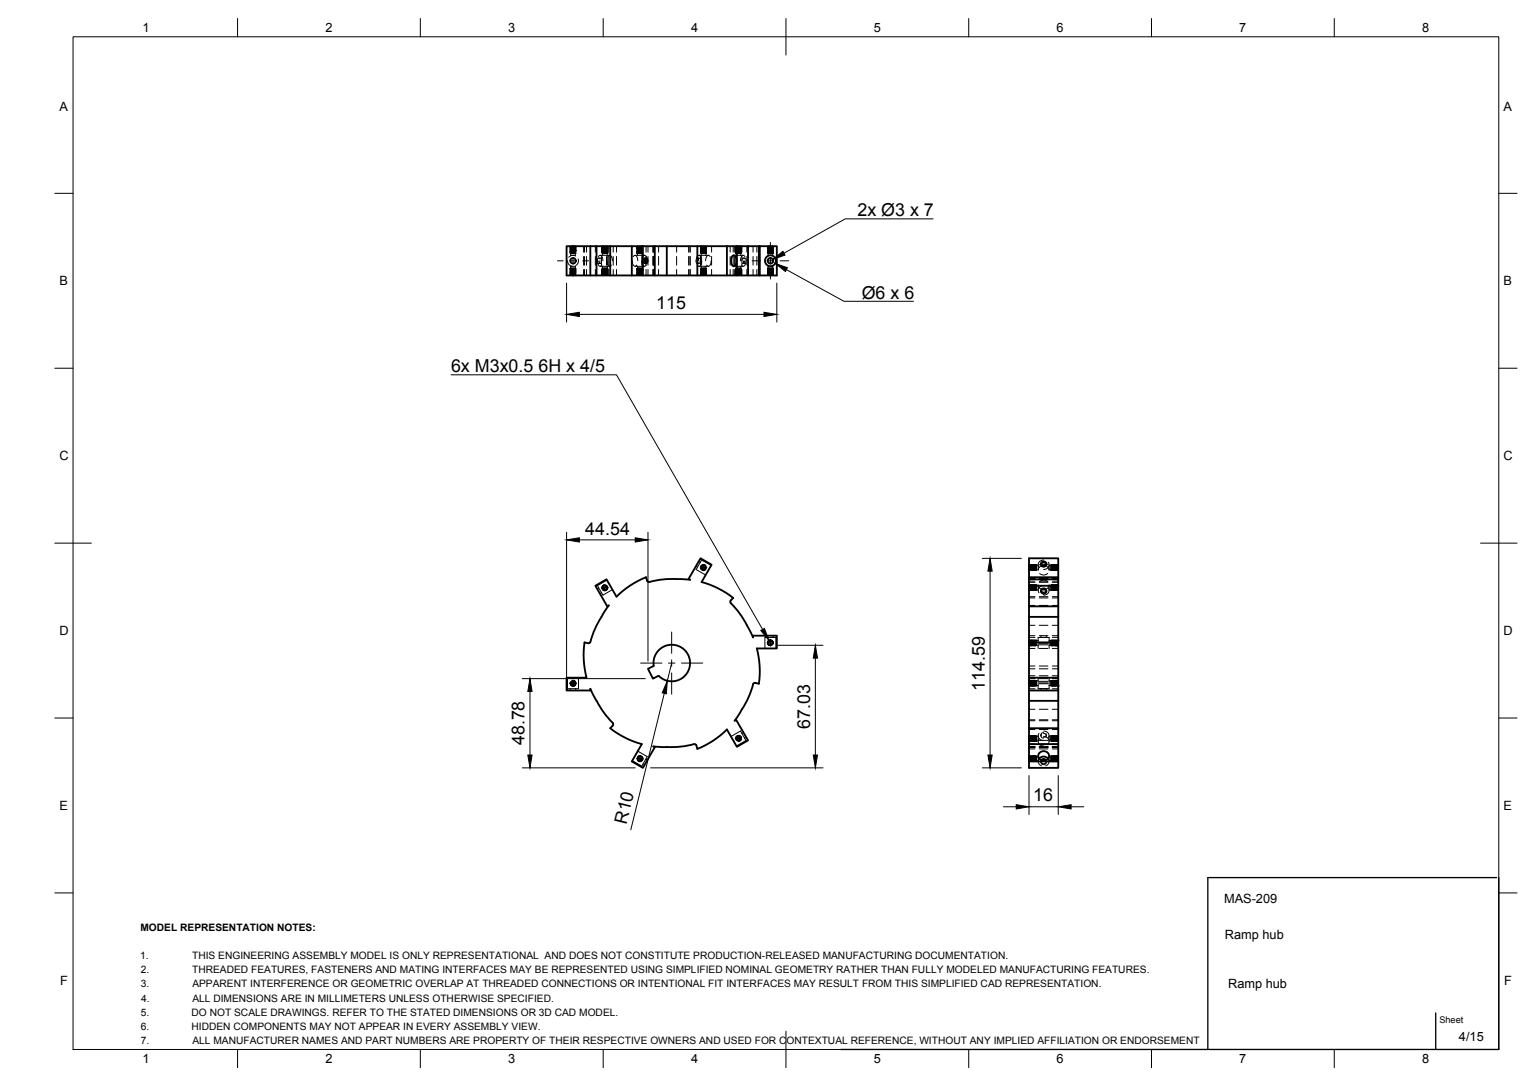
ISO-10303-21;
HEADER;
/* Generated by software containing ST-Developer
 * from STEP Tools, Inc. (www.steptools.com) 
 */

FILE_DESCRIPTION(
/* description */ ('Independent bearing-supported roller-ramp one-way clutch. Six logarit
hmic ramps with plain solid rollers, sprung guided plungers, native Co
il variants, removable shared keepers, rounded parallel key, shaft wit
h complete retaining lips, bronze journal/thrust support and bolted co
vers. Native rotor, roller planar/spin and plunger joints permit manua
l geometric engaged/released inspection. Automatic frictional torque s
witching/contact dynamics are not simulated; no capacity, hardness, fi
t, lubrication, speed, force or life rating. External input driver/cou
pling/anchors outside assembly.'),
/* implementation_level */ '2;1');

FILE_NAME(
/* name */ 'Ramp hub.step',
/* time_stamp */ '2026-11-08T07:04:38-08:00',
/* author */ (''),
/* organization */ (''),
/* preprocessor_version */ 'ST-DEVELOPER v20.2',
/* originating_system */ 'Autodesk Translation Framework v15.17.0.0',
/* authorisation */ '');

FILE_SCHEMA (('AUTOMOTIVE_DESIGN { 1 0 10303 214 3 1 1 }'));
ENDSEC;

DATA;
#10=MECHANICAL_DESIGN_GEOMETRIC_PRESENTATION_REPRESENTATION('',(#301),#99526);
#256=(
BOUNDED_SURFACE()
B_SPLINE_SURFACE(5,1,((#70021,#70022),(#70023,#70024),(#70025,#70026),(#70027,
#70028),(#70029,#70030),(#70031,#70032),(#70033,#70034),(#70035,#70036),
(#70037,#70038),(#70039,#70040),(#70041,#70042),(#70043,#70044),(#70045,
#70046),(#70047,#70048),(#70049,#70050),(#70051,#70052),(#70053,#70054),
(#70055,#70056),(#70057,#70058),(#70059,#70060),(#70061,#70062),(#70063,
#70064),(#70065,#70066),(#70067,#70068),(#70069,#70070),(#70071,#70072),
(#70073,#70074),(#70075,#70076),(#70077,#70078),(#70079,#70080),(#70081,
#70082),(#70083,#70084),(#70085,#70086),(#70087,#70088),(#70089,#70090),
(#70091,#70092),(#70093,#70094),(#70095,#70096),(#70097,#70098),(#70099,
#70100),(#70101,#70102),(#70103,#70104),(#70105,#70106),(#70107,#70108),
(#70109,#70110),(#70111,#70112),(#70113,#70114),(#70115,#70116),(#70117,
#70118),(#70119,#70120),(#70121,#70122),(#70123,#70124),(#70125,#70126),
(#70127,#70128),(#70129,#70130),(#70131,#70132),(#70133,#70134),(#70135,
#70136),(#70137,#70138),(#70139,#70140),(#70141,#70142),(#70143,#70144),
(#70145,#70146),(#70147,#70148),(#70149,#70150),(#70151,#70152),(#70153,
#70154),(#70155,#70156),(#70157,#70158),(#70159,#70160),(#70161,#70162),
(#70163,#70164),(#70165,#70166),(#70167,#70168),(#70169,#70170),(#70171,
#70172),(#70173,#70174),(#70175,#70176),(#70177,#70178),(#70179,#70180),
(#70181,#70182),(#70183,#70184),(#70185,#70186),(#70187,#70188),(#70189,
#70190),(#70191,#70192),(#70193,#70194),(#70195,#70196),(#70197,#70198),
(#70199,#70200),(#70201,#70202),(#70203,#70204),(#70205,#70206),(#70207,
#70208),(#70209,#70210),(#70211,#70212),(#70213,#70214),(#70215,#70216),
(#70217,#70218),(#70219,#70220),(#70221,#70222),(#70223,#70224),(#70225,
#70226),(#70227,#70228),(#70229,#70230),(#70231,#70232),(#70233,#70234),
(#70235,#70236),(#70237,#70238),(#70239,#70240),(#70241,#70242),(#70243,
#70244),(#70245,#70246),(#70247,#70248),(#70249,#70250),(#70251,#70252),
(#70253,#70254),(#70255,#70256),(#70257,#70258),(#70259,#70260),(#70261,
#70262),(#70263,#70264),(#70265,#70266),(#70267,#70268),(#70269,#70270),
(#70271,#70272),(#70273,#70274),(#70275,#70276),(#70277,#70278),(#70279,
#70280),(#70281,#70282),(#70283,#70284),(#70285,#70286),(#70287,#70288),
(#70289,#70290),(#70291,#70292),(#70293,#70294),(#70295,#70296),(#70297,
#70298),(#70299,#70300),(#70301,#70302),(#70303,#70304),(#70305,#70306),
(#70307,#70308),(#70309,#70310),(#70311,#70312),(#70313,#70314),(#70315,
#70316),(#70317,#70318),(#70319,#70320),(#70321,#70322),(#70323,#70324),
(#70325,#70326),(#70327,#70328),(#70329,#70330),(#70331,#70332),(#70333,
#70334),(#70335,#70336),(#70337,#70338),(#70339,#70340),(#70341,#70342),
(#70343,#70344),(#70345,#70346),(#70347,#70348),(#70349,#70350),(#70351,
#70352),(#70353,#70354),(#70355,#70356),(#70357,#70358),(#70359,#70360),
(#70361,#70362),(#70363,#70364),(#70365,#70366),(#70367,#70368),(#70369,
#70370),(#70371,#70372),(#70373,#70374),(#70375,#70376),(#70377,#70378),
(#70379,#70380),(#70381,#70382),(#70383,#70384),(#70385,#70386),(#70387,
#70388),(#70389,#70390),(#70391,#70392),(#70393,#70394),(#70395,#70396),
(#70397,#70398),(#70399,#70400),(#70401,#70402),(#70403,#70404),(#70405,
#70406),(#70407,#70408),(#70409,#70410),(#70411,#70412),(#70413,#70414),
(#70415,#70416),(#70417,#70418),(#70419,#70420),(#70421,#70422),(#70423,
#70424),(#70425,#70426),(#70427,#70428),(#70429,#70430),(#70431,#70432),
(#70433,#70434),(#70435,#70436),(#70437,#70438),(#70439,#70440),(#70441,
#70442),(#70443,#70444),(#70445,#70446),(#70447,#70448),(#70449,#70450),
(#70451,#70452),(#70453,#70454),(#70455,#70456),(#70457,#70458),(#70459,
#70460),(#70461,#70462),(#70463,#70464),(#70465,#70466),(#70467,#70468),
(#70469,#70470),(#70471,#70472),(#70473,#70474),(#70475,#70476),(#70477,
#70478),(#70479,#70480),(#70481,#70482),(#70483,#70484),(#70485,#70486),
(#70487,#70488),(#70489,#70490),(#70491,#70492),(#70493,#70494),(#70495,
#70496),(#70497,#70498),(#70499,#70500),(#70501,#70502),(#70503,#70504),
(#70505,#70506),(#70507,#70508),(#70509,#70510),(#70511,#70512),(#70513,
#70514),(#70515,#70516),(#70517,#70518),(#70519,#70520),(#70521,#70522),
(#70523,#70524),(#70525,#70526),(#70527,#70528),(#70529,#70530),(#70531,
#70532),(#70533,#70534),(#70535,#70536),(#70537,#70538),(#70539,#70540),
(#70541,#70542),(#70543,#70544),(#70545,#70546),(#70547,#70548),(#70549,
#70550),(#70551,#70552),(#70553,#70554),(#70555,#70556),(#70557,#70558),
(#70559,#70560),(#70561,#70562),(#70563,#70564),(#70565,#70566),(#70567,
#70568),(#70569,#70570),(#70571,#70572),(#70573,#70574),(#70575,#70576),
(#70577,#70578),(#70579,#70580),(#70581,#70582),(#70583,#70584),(#70585,
#70586),(#70587,#70588),(#70589,#70590),(#70591,#70592),(#70593,#70594),
(#70595,#70596),(#70597,#70598),(#70599,#70600),(#70601,#70602),(#70603,
#70604),(#70605,#70606),(#70607,#70608),(#70609,#70610),(#70611,#70612),
(#70613,#70614),(#70615,#70616),(#70617,#70618),(#70619,#70620),(#70621,
#70622),(#70623,#70624),(#70625,#70626),(#70627,#70628),(#70629,#70630),
(#70631,#70632),(#70633,#70634),(#70635,#70636),(#70637,#70638),(#70639,
#70640),(#70641,#70642),(#70643,#70644),(#70645,#70646),(#70647,#70648),
(#70649,#70650),(#70651,#70652),(#70653,#70654),(#70655,#70656),(#70657,
#70658),(#70659,#70660),(#70661,#70662),(#70663,#70664),(#70665,#70666),
(#70667,#70668),(#70669,#70670),(#70671,#70672),(#70673,#70674),(#70675,
#70676),(#70677,#70678),(#70679,#70680),(#70681,#70682),(#70683,#70684),
(#70685,#70686),(#70687,#70688),(#70689,#70690),(#70691,#70692),(#70693,
#70694),(#70695,#70696),(#70697,#70698),(#70699,#70700),(#70701,#70702),
(#70703,#70704),(#70705,#70706),(#70707,#70708),(#70709,#70710),(#70711,
#70712),(#70713,#70714),(#70715,#70716),(#70717,#70718),(#70719,#70720),
(#70721,#70722),(#70723,#70724),(#70725,#70726),(#70727,#70728),(#70729,
#70730),(#70731,#70732),(#70733,#70734),(#70735,#70736),(#70737,#70738),
(#70739,#70740),(#70741,#70742),(#70743,#70744),(#70745,#70746),(#70747,
#70748),(#70749,#70750),(#70751,#70752),(#70753,#70754),(#70755,#70756),
(#70757,#70758),(#70759,#70760),(#70761,#70762),(#70763,#70764),(#70765,
#70766),(#70767,#70768),(#70769,#70770),(#70771,#70772),(#70773,#70774),
(#70775,#70776),(#70777,#70778),(#70779,#70780),(#70781,#70782),(#70783,
#70784),(#70785,#70786),(#70787,#70788),(#70789,#70790),(#70791,#70792),
(#70793,#70794),(#70795,#70796),(#70797,#70798),(#70799,#70800),(#70801,
#70802),(#70803,#70804),(#70805,#70806),(#70807,#70808),(#70809,#70810),
(#70811,#70812),(#70813,#70814),(#70815,#70816),(#70817,#70818),(#70819,
#70820),(#70821,#70822),(#70823,#70824),(#70825,#70826),(#70827,#70828),
(#70829,#70830),(#70831,#70832),(#70833,#70834),(#70835,#70836),(#70837,
#70838),(#70839,#70840),(#70841,#70842),(#70843,#70844),(#70845,#70846),
(#70847,#70848),(#70849,#70850),(#70851,#70852),(#70853,#70854),(#70855,
#70856),(#70857,#70858),(#70859,#70860),(#70861,#70862),(#70863,#70864),
(#70865,#70866),(#70867,#70868),(#70869,#70870),(#70871,#70872),(#70873,
#70874),(#70875,#70876),(#70877,#70878),(#70879,#70880),(#70881,#70882),
(#70883,#70884),(#70885,#70886),(#70887,#70888),(#70889,#70890),(#70891,
#70892),(#70893,#70894),(#70895,#70896),(#70897,#70898),(#70899,#70900),
(#70901,#70902),(#70903,#70904),(#70905,#70906),(#70907,#70908),(#70909,
#70910),(#70911,#70912),(#70913,#70914),(#70915,#70916),(#70917,#70918),
(#70919,#70920),(#70921,#70922),(#70923,#70924),(#70925,#70926),(#70927,
#70928),(#70929,#70930),(#70931,#70932),(#70933,#70934),(#70935,#70936),
(#70937,#70938),(#70939,#70940),(#70941,#70942),(#70943,#70944),(#70945,
#70946),(#70947,#70948),(#70949,#70950),(#70951,#70952),(#70953,#70954),
(#70955,#70956),(#70957,#70958),(#70959,#70960),(#70961,#70962),(#70963,
#70964),(#70965,#70966),(#70967,#70968),(#70969,#70970),(#70971,#70972),
(#70973,#70974),(#70975,#70976),(#70977,#70978),(#70979,#70980),(#70981,
#70982),(#70983,#70984),(#70985,#70986),(#70987,#70988),(#70989,#70990),
(#70991,#70992),(#70993,#70994),(#70995,#70996),(#70997,#70998),(#70999,
#71000),(#71001,#71002),(#71003,#71004),(#71005,#71006),(#71007,#71008),
(#71009,#71010),(#71011,#71012),(#71013,#71014),(#71015,#71016),(#71017,
#71018),(#71019,#71020),(#71021,#71022),(#71023,#71024),(#71025,#71026),
(#71027,#71028),(#71029,#71030),(#71031,#71032),(#71033,#71034),(#71035,
#71036),(#71037,#71038),(#71039,#71040),(#71041,#71042),(#71043,#71044),
(#71045,#71046),(#71047,#71048),(#71049,#71050),(#71051,#71052),(#71053,
#71054),(#71055,#71056),(#71057,#71058),(#71059,#71060),(#71061,#71062),
(#71063,#71064),(#71065,#71066),(#71067,#71068),(#71069,#71070),(#71071,
#71072),(#71073,#71074),(#71075,#71076),(#71077,#71078),(#71079,#71080),
(#71081,#71082),(#71083,#71084),(#71085,#71086),(#71087,#71088),(#71089,
#71090),(#71091,#71092),(#71093,#71094),(#71095,#71096),(#71097,#71098),
(#71099,#71100),(#71101,#71102),(#71103,#71104),(#71105,#71106),(#71107,
#71108),(#71109,#71110),(#71111,#71112),(#71113,#71114),(#71115,#71116),
(#71117,#71118),(#71119,#71120),(#71121,#71122),(#71123,#71124),(#71125,
#71126),(#71127,#71128),(#71129,#71130),(#71131,#71132),(#71133,#71134),
(#71135,#71136),(#71137,#71138),(#71139,#71140),(#71141,#71142),(#71143,
#71144),(#71145,#71146),(#71147,#71148),(#71149,#71150),(#71151,#71152),
(#71153,#71154),(#71155,#71156),(#71157,#71158),(#71159,#71160),(#71161,
#71162),(#71163,#71164),(#71165,#71166),(#71167,#71168),(#71169,#71170),
(#71171,#71172),(#71173,#71174),(#71175,#71176),(#71177,#71178),(#71179,
#71180),(#71181,#71182),(#71183,#71184),(#71185,#71186),(#71187,#71188),
(#71189,#71190),(#71191,#71192),(#71193,#71194),(#71195,#71196),(#71197,
#71198),(#71199,#71200),(#71201,#71202),(#71203,#71204),(#71205,#71206),
(#71207,#71208),(#71209,#71210),(#71211,#71212),(#71213,#71214),(#71215,
#71216),(#71217,#71218),(#71219,#71220),(#71221,#71222),(#71223,#71224),
(#71225,#71226),(#71227,#71228),(#71229,#71230),(#71231,#71232),(#71233,
#71234),(#71235,#71236),(#71237,#71238),(#71239,#71240),(#71241,#71242),
(#71243,#71244),(#71245,#71246),(#71247,#71248),(#71249,#71250),(#71251,
#71252),(#71253,#71254),(#71255,#71256),(#71257,#71258),(#71259,#71260),
(#71261,#71262),(#71263,#71264),(#71265,#71266),(#71267,#71268),(#71269,
#71270),(#71271,#71272),(#71273,#71274),(#71275,#71276),(#71277,#71278),
(#71279,#71280),(#71281,#71282),(#71283,#71284),(#71285,#71286),(#71287,
#71288),(#71289,#71290),(#71291,#71292),(#71293,#71294),(#71295,#71296),
(#71297,#71298),(#71299,#71300),(#71301,#71302),(#71303,#71304),(#71305,
#71306),(#71307,#71308),(#71309,#71310),(#71311,#71312),(#71313,#71314),
(#71315,#71316),(#71317,#71318),(#71319,#71320),(#71321,#71322),(#71323,
#71324),(#71325,#71326),(#71327,#71328),(#71329,#71330),(#71331,#71332),
(#71333,#71334),(#71335,#71336),(#71337,#71338),(#71339,#71340),(#71341,
#71342),(#71343,#71344),(#71345,#71346),(#71347,#71348),(#71349,#71350),
(#71351,#71352),(#71353,#71354),(#71355,#71356),(#71357,#71358),(#71359,
#71360),(#71361,#71362),(#71363,#71364),(#71365,#71366),(#71367,#71368),
(#71369,#71370),(#71371,#71372),(#71373,#71374),(#71375,#71376),(#71377,
#71378),(#71379,#71380),(#71381,#71382),(#71383,#71384),(#71385,#71386),
(#71387,#71388),(#71389,#71390),(#71391,#71392),(#71393,#71394),(#71395,
#71396),(#71397,#71398),(#71399,#71400),(#71401,#71402),(#71403,#71404),
(#71405,#71406),(#71407,#71408),(#71409,#71410),(#71411,#71412),(#71413,
#71414),(#71415,#71416),(#71417,#71418),(#71419,#71420),(#71421,#71422),
(#71423,#71424),(#71425,#71426),(#71427,#71428),(#71429,#71430),(#71431,
#71432),(#71433,#71434),(#71435,#71436),(#71437,#71438),(#71439,#71440),
(#71441,#71442),(#71443,#71444),(#71445,#71446),(#71447,#71448),(#71449,
#71450),(#71451,#71452),(#71453,#71454),(#71455,#71456),(#71457,#71458),
(#71459,#71460),(#71461,#71462),(#71463,#71464),(#71465,#71466),(#71467,
#71468),(#71469,#71470),(#71471,#71472),(#71473,#71474),(#71475,#71476),
(#71477,#71478),(#71479,#71480),(#71481,#71482),(#71483,#71484),(#71485,
#71486),(#71487,#71488),(#71489,#71490),(#71491,#71492),(#71493,#71494),
(#71495,#71496),(#71497,#71498),(#71499,#71500),(#71501,#71502),(#71503,
#71504),(#71505,#71506),(#71507,#71508),(#71509,#71510),(#71511,#71512),
(#71513,#71514),(#71515,#71516),(#71517,#71518),(#71519,#71520),(#71521,
#71522),(#71523,#71524),(#71525,#71526),(#71527,#71528),(#71529,#71530),
(#71531,#71532),(#71533,#71534),(#71535,#71536),(#71537,#71538),(#71539,
#71540),(#71541,#71542),(#71543,#71544),(#71545,#71546),(#71547,#71548),
(#71549,#71550),(#71551,#71552),(#71553,#71554),(#71555,#71556),(#71557,
#71558),(#71559,#71560),(#71561,#71562),(#71563,#71564),(#71565,#71566),
(#71567,#71568),(#71569,#71570),(#71571,#71572),(#71573,#71574),(#71575,
#71576),(#71577,#71578),(#71579,#71580),(#71581,#71582),(#71583,#71584),
(#71585,#71586),(#71587,#71588),(#71589,#71590),(#71591,#71592),(#71593,
#71594),(#71595,#71596),(#71597,#71598),(#71599,#71600),(#71601,#71602),
(#71603,#71604),(#71605,#71606),(#71607,#71608),(#71609,#71610),(#71611,
#71612),(#71613,#71614),(#71615,#71616),(#71617,#71618),(#71619,#71620),
(#71621,#71622),(#71623,#71624),(#71625,#71626),(#71627,#71628),(#71629,
#71630),(#71631,#71632),(#71633,#71634),(#71635,#71636),(#71637,#71638),
(#71639,#71640),(#71641,#71642),(#71643,#71644),(#71645,#71646),(#71647,
#71648),(#71649,#71650),(#71651,#71652),(#71653,#71654),(#71655,#71656),
(#71657,#71658),(#71659,#71660),(#71661,#71662),(#71663,#71664),(#71665,
#71666),(#71667,#71668),(#71669,#71670),(#71671,#71672),(#71673,#71674),
(#71675,#71676),(#71677,#71678),(#71679,#71680),(#71681,#71682),(#71683,
#71684),(#71685,#71686),(#71687,#71688),(#71689,#71690),(#71691,#71692),
(#71693,#71694),(#71695,#71696),(#71697,#71698),(#71699,#71700),(#71701,
#71702),(#71703,#71704),(#71705,#71706),(#71707,#71708),(#71709,#71710),
(#71711,#71712),(#71713,#71714),(#71715,#71716),(#71717,#71718),(#71719,
#71720),(#71721,#71722),(#71723,#71724),(#71725,#71726),(#71727,#71728),
(#71729,#71730),(#71731,#71732),(#71733,#71734),(#71735,#71736),(#71737,
#71738),(#71739,#71740),(#71741,#71742),(#71743,#71744),(#71745,#71746),
(#71747,#71748),(#71749,#71750),(#71751,#71752),(#71753,#71754),(#71755,
#71756),(#71757,#71758),(#71759,#71760),(#71761,#71762),(#71763,#71764),
(#71765,#71766),(#71767,#71768),(#71769,#71770),(#71771,#71772),(#71773,
#71774),(#71775,#71776),(#71777,#71778),(#71779,#71780),(#71781,#71782),
(#71783,#71784),(#71785,#71786),(#71787,#71788),(#71789,#71790),(#71791,
#71792),(#71793,#71794),(#71795,#71796),(#71797,#71798),(#71799,#71800),
(#71801,#71802),(#71803,#71804),(#71805,#71806),(#71807,#71808),(#71809,
#71810),(#71811,#71812),(#71813,#71814),(#71815,#71816),(#71817,#71818),
(#71819,#71820),(#71821,#71822),(#71823,#71824),(#71825,#71826),(#71827,
#71828),(#71829,#71830),(#71831,#71832),(#71833,#71834),(#71835,#71836),
(#71837,#71838),(#71839,#71840),(#71841,#71842),(#71843,#71844),(#71845,
#71846),(#71847,#71848),(#71849,#71850),(#71851,#71852),(#71853,#71854),
(#71855,#71856),(#71857,#71858),(#71859,#71860),(#71861,#71862),(#71863,
#71864),(#71865,#71866),(#71867,#71868),(#71869,#71870),(#71871,#71872),
(#71873,#71874),(#71875,#71876),(#71877,#71878),(#71879,#71880),(#71881,
#71882),(#71883,#71884),(#71885,#71886),(#71887,#71888),(#71889,#71890),
(#71891,#71892),(#71893,#71894),(#71895,#71896),(#71897,#71898),(#71899,
#71900),(#71901,#71902),(#71903,#71904),(#71905,#71906),(#71907,#71908),
(#71909,#71910),(#71911,#71912),(#71913,#71914),(#71915,#71916),(#71917,
#71918),(#71919,#71920),(#71921,#71922),(#71923,#71924),(#71925,#71926),
(#71927,#71928),(#71929,#71930),(#71931,#71932),(#71933,#71934),(#71935,
#71936),(#71937,#71938),(#71939,#71940),(#71941,#71942),(#71943,#71944),
(#71945,#71946),(#71947,#71948),(#71949,#71950),(#71951,#71952),(#71953,
#71954),(#71955,#71956),(#71957,#71958),(#71959,#71960),(#71961,#71962),
(#71963,#71964),(#71965,#71966),(#71967,#71968),(#71969,#71970),(#71971,
#71972),(#71973,#71974),(#71975,#71976),(#71977,#71978),(#71979,#71980),
(#71981,#71982),(#71983,#71984),(#71985,#71986),(#71987,#71988),(#71989,
#71990),(#71991,#71992),(#71993,#71994),(#71995,#71996),(#71997,#71998),
(#71999,#72000),(#72001,#72002),(#72003,#72004),(#72005,#72006),(#72007,
#72008),(#72009,#72010),(#72011,#72012),(#72013,#72014),(#72015,#72016),
(#72017,#72018),(#72019,#72020),(#72021,#72022),(#72023,#72024),(#72025,
#72026),(#72027,#72028),(#72029,#72030)),.UNSPECIFIED.,.F.,.F.,.F.)
B_SPLINE_SURFACE_WITH_KNOTS((6,1,1,1,1,1,1,1,1,1,1,1,1,1,1,1,1,1,1,1,1,
1,1,1,1,1,1,1,1,1,1,1,1,1,1,1,1,1,1,1,1,1,1,1,1,1,1,1,1,1,1,1,1,1,1,1,1,
1,1,1,1,1,1,1,1,1,1,1,1,1,1,1,1,1,1,1,1,1,1,1,1,1,1,1,1,1,1,1,1,1,1,1,1,
1,1,1,1,1,1,1,1,1,1,1,1,1,1,1,1,1,1,1,1,1,1,1,1,1,1,1,1,1,1,1,1,1,1,1,1,
1,1,1,1,1,1,1,1,1,1,1,1,1,1,1,1,1,1,1,1,1,1,1,1,1,1,1,1,1,1,1,1,1,1,1,1,
1,1,1,1,1,1,1,1,1,1,1,1,1,1,1,1,1,1,1,1,1,1,1,1,1,1,1,1,1,1,1,1,1,1,1,1,
1,1,1,1,1,1,1,1,1,1,1,1,1,1,1,1,1,1,1,1,1,1,1,1,1,1,1,1,1,1,1,1,1,1,1,1,
1,1,1,1,1,1,1,1,1,1,1,1,1,1,1,1,1,1,1,1,1,1,1,1,1,1,1,1,1,1,1,1,1,1,1,1,
1,1,1,1,1,1,1,1,1,1,1,1,1,1,1,1,1,1,1,1,1,1,1,1,1,1,1,1,1,1,1,1,1,1,1,1,
1,1,1,1,1,1,1,1,1,1,1,1,1,1,1,1,1,1,1,1,1,1,1,1,1,1,1,1,1,1,1,1,1,1,1,1,
1,1,1,1,1,1,1,1,1,1,1,1,1,1,1,1,1,1,1,1,1,1,1,1,1,1,1,1,1,1,1,1,1,1,1,1,
1,1,1,1,1,1,1,1,1,1,1,1,1,1,1,1,1,1,1,1,1,1,1,1,1,1,1,1,1,1,1,1,1,1,1,1,
1,1,1,1,1,1,1,1,1,1,1,1,1,1,1,1,1,1,1,1,1,1,1,1,1,1,1,1,1,1,1,1,1,1,1,1,
1,1,1,1,1,1,1,1,1,1,1,1,1,1,1,1,1,1,1,1,1,1,1,1,1,1,1,1,1,1,1,1,1,1,1,1,
1,1,1,1,1,1,1,1,1,1,1,1,1,1,1,1,1,1,1,1,1,1,1,1,1,1,1,1,1,1,1,1,1,1,1,1,
1,1,1,1,1,1,1,1,1,1,1,1,1,1,1,1,1,1,1,1,1,1,1,1,1,1,1,1,1,1,1,1,1,1,1,1,
1,1,1,1,1,1,1,1,1,1,1,1,1,1,1,1,1,1,1,1,1,1,1,1,1,1,1,1,1,1,1,1,1,1,1,1,
1,1,1,1,1,1,1,1,1,1,1,1,1,1,1,1,1,1,1,1,1,1,1,1,1,1,1,1,1,1,1,1,1,1,1,1,
1,1,1,1,1,1,1,1,1,1,1,1,1,1,1,1,1,1,1,1,1,1,1,1,1,1,1,1,1,1,1,1,1,1,1,1,
1,1,1,1,1,1,1,1,1,1,1,1,1,1,1,1,1,1,1,1,1,1,1,1,1,1,1,1,1,1,1,1,1,1,1,1,
1,1,1,1,1,1,1,1,1,1,1,1,1,1,1,1,1,1,1,1,1,1,1,1,1,1,1,1,1,1,1,1,1,1,1,1,
1,1,1,1,1,1,1,1,1,1,1,1,1,1,1,1,1,1,1,1,1,1,1,1,1,1,1,1,1,1,1,1,1,1,1,1,
1,1,1,1,1,1,1,1,1,1,1,1,1,1,1,1,1,1,1,1,1,1,1,1,1,1,1,1,1,1,1,1,1,1,1,1,
1,1,1,1,1,1,1,1,1,1,1,1,1,1,1,1,1,1,1,1,1,1,1,1,1,1,1,1,1,1,1,1,1,1,1,1,
1,1,1,1,1,1,1,1,1,1,1,1,1,1,1,1,1,1,1,1,1,1,1,1,1,1,1,1,1,1,1,1,1,1,1,1,
1,1,1,1,1,1,1,1,1,1,1,1,1,1,1,1,1,1,1,1,1,1,1,1,1,1,1,1,1,1,1,1,1,1,1,1,
1,1,1,1,1,1,1,1,1,1,1,1,1,1,1,1,1,1,1,1,1,1,1,1,1,1,1,1,1,1,1,1,1,1,1,1,
1,1,1,1,1,1,1,1,1,1,1,1,1,1,1,1,1,1,1,1,1,1,1,1,1,1,1,1,1,1,1,1,1,1,1,1,
1,1,1,1,1,1,1,6),(2,2),(-1.,-0.999000000000001,-0.998000000000001,-0.997000000000001,
-0.996000000000001,-0.995000000000001,-0.994000000000001,-0.993000000000001,
-0.992000000000001,-0.991000000000001,-0.990000000000001,-0.989000000000001,
-0.988000000000001,-0.987000000000001,-0.986000000000001,-0.985000000000001,
-0.984000000000001,-0.983000000000001,-0.982000000000001,-0.981000000000001,
-0.980000000000001,-0.979000000000001,-0.978000000000001,-0.977000000000001,
-0.976000000000001,-0.975000000000001,-0.974000000000001,-0.973000000000001,
-0.972000000000001,-0.971000000000001,-0.970000000000001,-0.969000000000001,
-0.968000000000001,-0.967000000000001,-0.966000000000001,-0.965000000000001,
-0.964000000000001,-0.963000000000001,-0.962000000000001,-0.961000000000001,
-0.960000000000001,-0.959000000000001,-0.958000000000001,-0.957000000000001,
-0.956000000000001,-0.955000000000001,-0.954000000000001,-0.953000000000001,
-0.952000000000001,-0.951000000000001,-0.950000000000001,-0.949000000000001,
-0.948000000000001,-0.947000000000001,-0.946000000000001,-0.945000000000001,
-0.944000000000001,-0.943000000000001,-0.942000000000001,-0.941000000000001,
-0.940000000000001,-0.939000000000001,-0.938000000000001,-0.937000000000001,
-0.936000000000001,-0.935000000000001,-0.934000000000001,-0.933000000000001,
-0.932000000000001,-0.931000000000001,-0.930000000000001,-0.929000000000001,
-0.928000000000001,-0.927000000000001,-0.926000000000001,-0.925000000000001,
-0.924000000000001,-0.923000000000001,-0.922000000000001,-0.921000000000001,
-0.920000000000001,-0.919000000000001,-0.918000000000001,-0.917000000000001,
-0.916000000000001,-0.915000000000001,-0.914000000000001,-0.913000000000001,
-0.912000000000001,-0.911000000000001,-0.910000000000001,-0.909000000000001,
-0.908000000000001,-0.907000000000001,-0.906000000000001,-0.905000000000001,
-0.904000000000001,-0.903000000000001,-0.902000000000001,-0.901000000000001,
-0.900000000000001,-0.899000000000001,-0.898000000000001,-0.897000000000001,
-0.896000000000001,-0.895000000000001,-0.894000000000001,-0.893000000000001,
-0.892000000000001,-0.891000000000001,-0.890000000000001,-0.889000000000001,
-0.888000000000001,-0.887000000000001,-0.886000000000001,-0.885000000000001,
-0.884000000000001,-0.883000000000001,-0.882000000000001,-0.881000000000001,
-0.880000000000001,-0.879000000000001,-0.878000000000001,-0.877000000000001,
-0.876000000000001,-0.875000000000001,-0.874000000000001,-0.873000000000001,
-0.872000000000001,-0.871000000000001,-0.870000000000001,-0.869000000000001,
-0.868000000000001,-0.867000000000001,-0.866000000000001,-0.865000000000001,
-0.864000000000001,-0.863000000000001,-0.862000000000001,-0.861000000000001,
-0.860000000000001,-0.859000000000001,-0.858000000000001,-0.857000000000001,
-0.856000000000001,-0.855000000000001,-0.854000000000001,-0.853000000000001,
-0.852000000000001,-0.851000000000001,-0.850000000000001,-0.849000000000001,
-0.848000000000001,-0.847000000000001,-0.846000000000001,-0.845000000000001,
-0.844000000000001,-0.843000000000001,-0.842000000000001,-0.841000000000001,
-0.840000000000001,-0.839000000000001,-0.838000000000001,-0.837000000000001,
-0.836000000000001,-0.835000000000001,-0.834000000000001,-0.833000000000001,
-0.832000000000001,-0.831000000000001,-0.830000000000001,-0.829000000000001,
-0.828000000000001,-0.827000000000001,-0.826000000000001,-0.825000000000001,
-0.824000000000001,-0.823000000000001,-0.822000000000001,-0.821000000000001,
-0.820000000000001,-0.819000000000001,-0.818000000000001,-0.817000000000001,
-0.816000000000001,-0.815000000000001,-0.814000000000001,-0.813000000000001,
-0.812000000000001,-0.811000000000001,-0.810000000000001,-0.809000000000001,
-0.808000000000001,-0.807000000000001,-0.806000000000001,-0.805000000000001,
-0.804000000000001,-0.803000000000001,-0.802000000000001,-0.801000000000001,
-0.800000000000001,-0.799000000000001,-0.798000000000001,-0.797000000000001,
-0.796000000000001,-0.795000000000001,-0.794000000000001,-0.793000000000001,
-0.792000000000001,-0.791000000000001,-0.790000000000001,-0.789000000000001,
-0.788000000000001,-0.787000000000001,-0.786000000000001,-0.785000000000001,
-0.784000000000001,-0.783000000000001,-0.782000000000001,-0.781000000000001,
-0.780000000000001,-0.779000000000001,-0.778000000000001,-0.777000000000001,
-0.776000000000001,-0.775000000000001,-0.774000000000001,-0.773000000000001,
-0.772000000000001,-0.771000000000001,-0.770000000000001,-0.769000000000001,
-0.768000000000001,-0.767000000000001,-0.766000000000001,-0.765000000000001,
-0.764000000000001,-0.763000000000001,-0.762000000000001,-0.761000000000001,
-0.760000000000001,-0.759000000000001,-0.758000000000001,-0.757000000000001,
-0.756000000000001,-0.755000000000001,-0.754000000000001,-0.753000000000001,
-0.752000000000001,-0.751000000000001,-0.750000000000001,-0.749000000000001,
-0.748000000000001,-0.747000000000001,-0.746000000000001,-0.745000000000001,
-0.744000000000001,-0.743000000000001,-0.742000000000001,-0.741000000000001,
-0.740000000000001,-0.739000000000001,-0.738000000000001,-0.737000000000001,
-0.736000000000001,-0.735000000000001,-0.734000000000001,-0.733000000000001,
-0.732000000000001,-0.731000000000001,-0.730000000000001,-0.729000000000001,
-0.728000000000001,-0.727000000000001,-0.726000000000001,-0.725000000000001,
-0.724000000000001,-0.723000000000001,-0.722000000000001,-0.721000000000001,
-0.720000000000001,-0.719000000000001,-0.718000000000001,-0.717000000000001,
-0.716000000000001,-0.715000000000001,-0.714000000000001,-0.713000000000001,
-0.712000000000001,-0.711000000000001,-0.710000000000001,-0.709000000000001,
-0.708000000000001,-0.707000000000001,-0.706000000000001,-0.705000000000001,
-0.704000000000001,-0.703000000000001,-0.702000000000001,-0.701000000000001,
-0.700000000000001,-0.699000000000001,-0.698000000000001,-0.697000000000001,
-0.696000000000001,-0.695000000000001,-0.694000000000001,-0.693000000000001,
-0.692000000000001,-0.691000000000001,-0.690000000000001,-0.689000000000001,
-0.688000000000001,-0.687,-0.686,-0.685,-0.684,-0.683,-0.682,-0.681,-0.68,
-0.679,-0.678,-0.677,-0.676,-0.675,-0.674,-0.673,-0.672,-0.671,-0.67,-0.669,
-0.668,-0.667,-0.666,-0.665,-0.664,-0.663,-0.662,-0.661,-0.66,-0.659,-0.658,
-0.657,-0.656,-0.655,-0.654,-0.653,-0.652,-0.651,-0.65,-0.649,-0.648,-0.647,
-0.646,-0.645,-0.644,-0.643,-0.642,-0.641,-0.64,-0.639,-0.638,-0.637,-0.636,
-0.635,-0.634,-0.633,-0.632,-0.631,-0.63,-0.629,-0.628,-0.627,-0.626,-0.625,
-0.624,-0.623,-0.622,-0.621,-0.62,-0.619,-0.618,-0.617,-0.616,-0.615,-0.614,
-0.613,-0.612,-0.611,-0.61,-0.609,-0.608,-0.607,-0.606,-0.605,-0.604,-0.603,
-0.602,-0.601,-0.6,-0.599,-0.598,-0.597,-0.596,-0.595,-0.594,-0.593,-0.592,
-0.591,-0.59,-0.589,-0.588,-0.587,-0.586,-0.585,-0.584,-0.583,-0.582,-0.581,
-0.58,-0.579,-0.578,-0.577,-0.576,-0.575,-0.574,-0.573,-0.572,-0.571,-0.57,
-0.569,-0.568,-0.567,-0.566,-0.565,-0.564,-0.563,-0.562,-0.561,-0.56,-0.559,
-0.558,-0.557,-0.556,-0.555,-0.554,-0.553,-0.552,-0.551,-0.55,-0.549,-0.548,
-0.547,-0.546,-0.545,-0.544,-0.543,-0.542,-0.541,-0.54,-0.539,-0.538,-0.537,
-0.536,-0.535,-0.534,-0.533,-0.532,-0.531,-0.53,-0.529,-0.528,-0.527,-0.526,
-0.525,-0.524,-0.523,-0.522,-0.521,-0.52,-0.519,-0.518,-0.517,-0.516,-0.515,
-0.514,-0.513,-0.512,-0.511,-0.51,-0.509,-0.508,-0.507,-0.506,-0.505,-0.504,
-0.503,-0.502,-0.501,-0.5,-0.499,-0.498,-0.497,-0.496,-0.495,-0.494,-0.493,
-0.492,-0.491,-0.49,-0.489,-0.488,-0.487,-0.486,-0.485,-0.484,-0.483,-0.482,
-0.481,-0.48,-0.479,-0.478,-0.477,-0.476,-0.475,-0.474,-0.473,-0.472,-0.471,
-0.47,-0.469,-0.468,-0.467,-0.466,-0.465,-0.464,-0.463,-0.462,-0.461,-0.46,
-0.459,-0.458,-0.457,-0.456,-0.455,-0.454,-0.453,-0.452,-0.451,-0.45,-0.449,
-0.448,-0.447,-0.446,-0.445,-0.444,-0.443,-0.442,-0.441,-0.44,-0.439,-0.438,
-0.437,-0.436,-0.435,-0.434,-0.433,-0.432,-0.431,-0.43,-0.429,-0.428,-0.427,
-0.426,-0.425,-0.424,-0.423,-0.422,-0.421,-0.42,-0.419,-0.418,-0.417,-0.416,
-0.415,-0.414,-0.413,-0.412,-0.411,-0.41,-0.409,-0.408,-0.407,-0.406,-0.405,
-0.404,-0.403,-0.402,-0.401,-0.4,-0.399,-0.398,-0.397,-0.396,-0.395,-0.394,
-0.393,-0.392,-0.391,-0.39,-0.389,-0.388,-0.387,-0.386,-0.385,-0.384,-0.383,
-0.382,-0.381,-0.38,-0.379,-0.378,-0.377,-0.376,-0.375,-0.374,-0.373,-0.372,
-0.371,-0.37,-0.369,-0.368,-0.367,-0.366,-0.365,-0.364,-0.363,-0.362,-0.361,
-0.36,-0.359,-0.358,-0.357,-0.356,-0.355,-0.354,-0.353,-0.352,-0.351,-0.35,
-0.349,-0.348,-0.347,-0.346,-0.345,-0.344,-0.343,-0.342,-0.341,-0.34,-0.339,
-0.338,-0.337,-0.336,-0.335,-0.334,-0.333,-0.332,-0.331,-0.33,-0.329,-0.328,
-0.327,-0.326,-0.325,-0.324,-0.323,-0.322,-0.321,-0.32,-0.319,-0.318,-0.317,
-0.316,-0.315,-0.314,-0.313,-0.312,-0.311,-0.31,-0.309,-0.308,-0.307,-0.306,
-0.305,-0.304,-0.303,-0.302,-0.301,-0.3,-0.299,-0.298,-0.297,-0.296,-0.295,
-0.294,-0.293,-0.292,-0.291,-0.29,-0.289,-0.288,-0.287,-0.286,-0.285,-0.284,
-0.283,-0.282,-0.281,-0.28,-0.279,-0.278,-0.277,-0.276,-0.275,-0.274,-0.273,
-0.272,-0.271,-0.27,-0.269,-0.268,-0.267,-0.266,-0.265,-0.264,-0.263,-0.262,
-0.261,-0.26,-0.259,-0.258,-0.257,-0.256,-0.255,-0.254,-0.253,-0.252,-0.251,
-0.25,-0.249,-0.248,-0.247,-0.246,-0.245,-0.244,-0.243,-0.242,-0.241,-0.24,
-0.239,-0.238,-0.237,-0.236,-0.235,-0.234,-0.233,-0.232,-0.231,-0.23,-0.229,
-0.228,-0.227,-0.226,-0.225,-0.224,-0.223,-0.222,-0.221,-0.22,-0.219,-0.218,
-0.217,-0.216,-0.215,-0.214,-0.213,-0.212,-0.211,-0.21,-0.209,-0.208,-0.207,
-0.206,-0.205,-0.204,-0.203,-0.202,-0.201,-0.2,-0.199,-0.198,-0.197,-0.196,
-0.195,-0.194,-0.193,-0.192,-0.191,-0.19,-0.189,-0.188,-0.187,-0.186,-0.185,
-0.184,-0.183,-0.182,-0.181,-0.18,-0.179,-0.178,-0.177,-0.176,-0.175,-0.174,
-0.173,-0.172,-0.171,-0.17,-0.169,-0.168,-0.167,-0.166,-0.165,-0.164,-0.163,
-0.162,-0.161,-0.16,-0.159,-0.158,-0.157,-0.156,-0.155,-0.154,-0.153,-0.152,
-0.151,-0.15,-0.149,-0.148,-0.147,-0.146,-0.145,-0.144,-0.143,-0.142,-0.141,
-0.14,-0.139,-0.138,-0.137,-0.136,-0.135,-0.134,-0.133,-0.132,-0.131,-0.13,
-0.129,-0.128,-0.127,-0.126,-0.125,-0.124,-0.123,-0.122,-0.121,-0.12,-0.119,
-0.118,-0.117,-0.116,-0.115,-0.114,-0.113,-0.112,-0.111,-0.11,-0.109,-0.108,
-0.107,-0.106,-0.105,-0.104,-0.103,-0.102,-0.101,-0.1,-0.0990000000000001,
-0.0980000000000001,-0.0970000000000001,-0.0960000000000001,-0.0950000000000001,
-0.0940000000000001,-0.0930000000000001,-0.0920000000000001,-0.0910000000000001,
-0.0900000000000001,-0.0890000000000001,-0.0880000000000001,-0.0870000000000001,
-0.0860000000000001,-0.0850000000000001,-0.0840000000000001,-0.0830000000000001,
-0.0820000000000001,-0.0810000000000001,-0.0800000000000001,-0.0790000000000001,
-0.0780000000000001,-0.0770000000000001,-0.0760000000000001,-0.0750000000000001,
-0.0740000000000001,-0.0730000000000001,-0.0720000000000001,-0.071,-0.07,
-0.069,-0.068,-0.067,-0.066,-0.065,-0.064,-0.063,-0.062,-0.061,-0.06,-0.059,
-0.058,-0.057,-0.056,-0.055,-0.054,-0.053,-0.052,-0.051,-0.05,-0.049,-0.048,
-0.047,-0.046,-0.045,-0.044,-0.043,-0.042,-0.041,-0.04,-0.039,-0.038,-0.037,
-0.036,-0.035,-0.034,-0.033,-0.032,-0.031,-0.03,-0.029,-0.028,-0.027,-0.026,
-0.025,-0.024,-0.023,-0.022,-0.021,-0.02,-0.019,-0.018,-0.017,-0.016,-0.015,
-0.014,-0.013,-0.012,-0.011,-0.01,-0.009,-0.008,-0.007,-0.006,-0.005,-0.004,
-0.003,-0.002,-0.001,0.),(0.,2.),.UNSPECIFIED.)
GEOMETRIC_REPRESENTATION_ITEM()
RATIONAL_B_SPLINE_SURFACE(((1.,1.),(1.,1.),(1.,1.),(1.,1.),(1.,1.),(1.,
1.),(1.,1.),(1.,1.),(1.,1.),(1.,1.),(1.,1.),(1.,1.),(1.,1.),(1.,1.),(1.,
1.),(1.,1.),(1.,1.),(1.,1.),(1.,1.),(1.,1.),(1.,1.),(1.,1.),(1.,1.),(1.,
1.),(1.,1.),(1.,1.),(1.,1.),(1.,1.),(1.,1.),(1.,1.),(1.,1.),(1.,1.),(1.,
1.),(1.,1.),(1.,1.),(1.,1.),(1.,1.),(1.,1.),(1.,1.),(1.,1.),(1.,1.),(1.,
1.),(1.,1.),(1.,1.),(1.,1.),(1.,1.),(1.,1.),(1.,1.),(1.,1.),(1.,1.),(1.,
1.),(1.,1.),(1.,1.),(1.,1.),(1.,1.),(1.,1.),(1.,1.),(1.,1.),(1.,1.),(1.,
1.),(1.,1.),(1.,1.),(1.,1.),(1.,1.),(1.,1.),(1.,1.),(1.,1.),(1.,1.),(1.,
1.),(1.,1.),(1.,1.),(1.,1.),(1.,1.),(1.,1.),(1.,1.),(1.,1.),(1.,1.),(1.,
1.),(1.,1.),(1.,1.),(1.,1.),(1.,1.),(1.,1.),(1.,1.),(1.,1.),(1.,1.),(1.,
1.),(1.,1.),(1.,1.),(1.,1.),(1.,1.),(1.,1.),(1.,1.),(1.,1.),(1.,1.),(1.,
1.),(1.,1.),(1.,1.),(1.,1.),(1.,1.),(1.,1.),(1.,1.),(1.,1.),(1.,1.),(1.,
1.),(1.,1.),(1.,1.),(1.,1.),(1.,1.),(1.,1.),(1.,1.),(1.,1.),(1.,1.),(1.,
1.),(1.,1.),(1.,1.),(1.,1.),(1.,1.),(1.,1.),(1.,1.),(1.,1.),(1.,1.),(1.,
1.),(1.,1.),(1.,1.),(1.,1.),(1.,1.),(1.,1.),(1.,1.),(1.,1.),(1.,1.),(1.,
1.),(1.,1.),(1.,1.),(1.,1.),(1.,1.),(1.,1.),(1.,1.),(1.,1.),(1.,1.),(1.,
1.),(1.,1.),(1.,1.),(1.,1.),(1.,1.),(1.,1.),(1.,1.),(1.,1.),(1.,1.),(1.,
1.),(1.,1.),(1.,1.),(1.,1.),(1.,1.),(1.,1.),(1.,1.),(1.,1.),(1.,1.),(1.,
1.),(1.,1.),(1.,1.),(1.,1.),(1.,1.),(1.,1.),(1.,1.),(1.,1.),(1.,1.),(1.,
1.),(1.,1.),(1.,1.),(1.,1.),(1.,1.),(1.,1.),(1.,1.),(1.,1.),(1.,1.),(1.,
1.),(1.,1.),(1.,1.),(1.,1.),(1.,1.),(1.,1.),(1.,1.),(1.,1.),(1.,1.),(1.,
1.),(1.,1.),(1.,1.),(1.,1.),(1.,1.),(1.,1.),(1.,1.),(1.,1.),(1.,1.),(1.,
1.),(1.,1.),(1.,1.),(1.,1.),(1.,1.),(1.,1.),(1.,1.),(1.,1.),(1.,1.),(1.,
1.),(1.,1.),(1.,1.),(1.,1.),(1.,1.),(1.,1.),(1.,1.),(1.,1.),(1.,1.),(1.,
1.),(1.,1.),(1.,1.),(1.,1.),(1.,1.),(1.,1.),(1.,1.),(1.,1.),(1.,1.),(1.,
1.),(1.,1.),(1.,1.),(1.,1.),(1.,1.),(1.,1.),(1.,1.),(1.,1.),(1.,1.),(1.,
1.),(1.,1.),(1.,1.),(1.,1.),(1.,1.),(1.,1.),(1.,1.),(1.,1.),(1.,1.),(1.,
1.),(1.,1.),(1.,1.),(1.,1.),(1.,1.),(1.,1.),(1.,1.),(1.,1.),(1.,1.),(1.,
1.),(1.,1.),(1.,1.),(1.,1.),(1.,1.),(1.,1.),(1.,1.),(1.,1.),(1.,1.),(1.,
1.),(1.,1.),(1.,1.),(1.,1.),(1.,1.),(1.,1.),(1.,1.),(1.,1.),(1.,1.),(1.,
1.),(1.,1.),(1.,1.),(1.,1.),(1.,1.),(1.,1.),(1.,1.),(1.,1.),(1.,1.),(1.,
1.),(1.,1.),(1.,1.),(1.,1.),(1.,1.),(1.,1.),(1.,1.),(1.,1.),(1.,1.),(1.,
1.),(1.,1.),(1.,1.),(1.,1.),(1.,1.),(1.,1.),(1.,1.),(1.,1.),(1.,1.),(1.,
1.),(1.,1.),(1.,1.),(1.,1.),(1.,1.),(1.,1.),(1.,1.),(1.,1.),(1.,1.),(1.,
1.),(1.,1.),(1.,1.),(1.,1.),(1.,1.),(1.,1.),(1.,1.),(1.,1.),(1.,1.),(1.,
1.),(1.,1.),(1.,1.),(1.,1.),(1.,1.),(1.,1.),(1.,1.),(1.,1.),(1.,1.),(1.,
1.),(1.,1.),(1.,1.),(1.,1.),(1.,1.),(1.,1.),(1.,1.),(1.,1.),(1.,1.),(1.,
1.),(1.,1.),(1.,1.),(1.,1.),(1.,1.),(1.,1.),(1.,1.),(1.,1.),(1.,1.),(1.,
1.),(1.,1.),(1.,1.),(1.,1.),(1.,1.),(1.,1.),(1.,1.),(1.,1.),(1.,1.),(1.,
1.),(1.,1.),(1.,1.),(1.,1.),(1.,1.),(1.,1.),(1.,1.),(1.,1.),(1.,1.),(1.,
1.),(1.,1.),(1.,1.),(1.,1.),(1.,1.),(1.,1.),(1.,1.),(1.,1.),(1.,1.),(1.,
1.),(1.,1.),(1.,1.),(1.,1.),(1.,1.),(1.,1.),(1.,1.),(1.,1.),(1.,1.),(1.,
1.),(1.,1.),(1.,1.),(1.,1.),(1.,1.),(1.,1.),(1.,1.),(1.,1.),(1.,1.),(1.,
1.),(1.,1.),(1.,1.),(1.,1.),(1.,1.),(1.,1.),(1.,1.),(1.,1.),(1.,1.),(1.,
1.),(1.,1.),(1.,1.),(1.,1.),(1.,1.),(1.,1.),(1.,1.),(1.,1.),(1.,1.),(1.,
1.),(1.,1.),(1.,1.),(1.,1.),(1.,1.),(1.,1.),(1.,1.),(1.,1.),(1.,1.),(1.,
1.),(1.,1.),(1.,1.),(1.,1.),(1.,1.),(1.,1.),(1.,1.),(1.,1.),(1.,1.),(1.,
1.),(1.,1.),(1.,1.),(1.,1.),(1.,1.),(1.,1.),(1.,1.),(1.,1.),(1.,1.),(1.,
1.),(1.,1.),(1.,1.),(1.,1.),(1.,1.),(1.,1.),(1.,1.),(1.,1.),(1.,1.),(1.,
1.),(1.,1.),(1.,1.),(1.,1.),(1.,1.),(1.,1.),(1.,1.),(1.,1.),(1.,1.),(1.,
1.),(1.,1.),(1.,1.),(1.,1.),(1.,1.),(1.,1.),(1.,1.),(1.,1.),(1.,1.),(1.,
1.),(1.,1.),(1.,1.),(1.,1.),(1.,1.),(1.,1.),(1.,1.),(1.,1.),(1.,1.),(1.,
1.),(1.,1.),(1.,1.),(1.,1.),(1.,1.),(1.,1.),(1.,1.),(1.,1.),(1.,1.),(1.,
1.),(1.,1.),(1.,1.),(1.,1.),(1.,1.),(1.,1.),(1.,1.),(1.,1.),(1.,1.),(1.,
1.),(1.,1.),(1.,1.),(1.,1.),(1.,1.),(1.,1.),(1.,1.),(1.,1.),(1.,1.),(1.,
1.),(1.,1.),(1.,1.),(1.,1.),(1.,1.),(1.,1.),(1.,1.),(1.,1.),(1.,1.),(1.,
1.),(1.,1.),(1.,1.),(1.,1.),(1.,1.),(1.,1.),(1.,1.),(1.,1.),(1.,1.),(1.,
1.),(1.,1.),(1.,1.),(1.,1.),(1.,1.),(1.,1.),(1.,1.),(1.,1.),(1.,1.),(1.,
1.),(1.,1.),(1.,1.),(1.,1.),(1.,1.),(1.,1.),(1.,1.),(1.,1.),(1.,1.),(1.,
1.),(1.,1.),(1.,1.),(1.,1.),(1.,1.),(1.,1.),(1.,1.),(1.,1.),(1.,1.),(1.,
1.),(1.,1.),(1.,1.),(1.,1.),(1.,1.),(1.,1.),(1.,1.),(1.,1.),(1.,1.),(1.,
1.),(1.,1.),(1.,1.),(1.,1.),(1.,1.),(1.,1.),(1.,1.),(1.,1.),(1.,1.),(1.,
1.),(1.,1.),(1.,1.),(1.,1.),(1.,1.),(1.,1.),(1.,1.),(1.,1.),(1.,1.),(1.,
1.),(1.,1.),(1.,1.),(1.,1.),(1.,1.),(1.,1.),(1.,1.),(1.,1.),(1.,1.),(1.,
1.),(1.,1.),(1.,1.),(1.,1.),(1.,1.),(1.,1.),(1.,1.),(1.,1.),(1.,1.),(1.,
1.),(1.,1.),(1.,1.),(1.,1.),(1.,1.),(1.,1.),(1.,1.),(1.,1.),(1.,1.),(1.,
1.),(1.,1.),(1.,1.),(1.,1.),(1.,1.),(1.,1.),(1.,1.),(1.,1.),(1.,1.),(1.,
1.),(1.,1.),(1.,1.),(1.,1.),(1.,1.),(1.,1.),(1.,1.),(1.,1.),(1.,1.),(1.,
1.),(1.,1.),(1.,1.),(1.,1.),(1.,1.),(1.,1.),(1.,1.),(1.,1.),(1.,1.),(1.,
1.),(1.,1.),(1.,1.),(1.,1.),(1.,1.),(1.,1.),(1.,1.),(1.,1.),(1.,1.),(1.,
1.),(1.,1.),(1.,1.),(1.,1.),(1.,1.),(1.,1.),(1.,1.),(1.,1.),(1.,1.),(1.,
1.),(1.,1.),(1.,1.),(1.,1.),(1.,1.),(1.,1.),(1.,1.),(1.,1.),(1.,1.),(1.,
1.),(1.,1.),(1.,1.),(1.,1.),(1.,1.),(1.,1.),(1.,1.),(1.,1.),(1.,1.),(1.,
1.),(1.,1.),(1.,1.),(1.,1.),(1.,1.),(1.,1.),(1.,1.),(1.,1.),(1.,1.),(1.,
1.),(1.,1.),(1.,1.),(1.,1.),(1.,1.),(1.,1.),(1.,1.),(1.,1.),(1.,1.),(1.,
1.),(1.,1.),(1.,1.),(1.,1.),(1.,1.),(1.,1.),(1.,1.),(1.,1.),(1.,1.),(1.,
1.),(1.,1.),(1.,1.),(1.,1.),(1.,1.),(1.,1.),(1.,1.),(1.,1.),(1.,1.),(1.,
1.),(1.,1.),(1.,1.),(1.,1.),(1.,1.),(1.,1.),(1.,1.),(1.,1.),(1.,1.),(1.,
1.),(1.,1.),(1.,1.),(1.,1.),(1.,1.),(1.,1.),(1.,1.),(1.,1.),(1.,1.),(1.,
1.),(1.,1.),(1.,1.),(1.,1.),(1.,1.),(1.,1.),(1.,1.),(1.,1.),(1.,1.),(1.,
1.),(1.,1.),(1.,1.),(1.,1.),(1.,1.),(1.,1.),(1.,1.),(1.,1.),(1.,1.),(1.,
1.),(1.,1.),(1.,1.),(1.,1.),(1.,1.),(1.,1.),(1.,1.),(1.,1.),(1.,1.),(1.,
1.),(1.,1.),(1.,1.),(1.,1.),(1.,1.),(1.,1.),(1.,1.),(1.,1.),(1.,1.),(1.,
1.),(1.,1.),(1.,1.),(1.,1.),(1.,1.),(1.,1.),(1.,1.),(1.,1.),(1.,1.),(1.,
1.),(1.,1.),(1.,1.),(1.,1.),(1.,1.),(1.,1.),(1.,1.),(1.,1.),(1.,1.),(1.,
1.),(1.,1.),(1.,1.),(1.,1.),(1.,1.),(1.,1.),(1.,1.),(1.,1.),(1.,1.),(1.,
1.),(1.,1.),(1.,1.),(1.,1.),(1.,1.),(1.,1.),(1.,1.),(1.,1.),(1.,1.),(1.,
1.),(1.,1.),(1.,1.),(1.,1.),(1.,1.),(1.,1.),(1.,1.),(1.,1.),(1.,1.),(1.,
1.),(1.,1.),(1.,1.),(1.,1.),(1.,1.),(1.,1.),(1.,1.),(1.,1.),(1.,1.),(1.,
1.),(1.,1.),(1.,1.),(1.,1.),(1.,1.),(1.,1.),(1.,1.),(1.,1.),(1.,1.),(1.,
1.),(1.,1.),(1.,1.),(1.,1.),(1.,1.),(1.,1.),(1.,1.),(1.,1.),(1.,1.),(1.,
1.),(1.,1.),(1.,1.),(1.,1.),(1.,1.),(1.,1.),(1.,1.),(1.,1.),(1.,1.),(1.,
1.),(1.,1.),(1.,1.),(1.,1.),(1.,1.),(1.,1.),(1.,1.),(1.,1.),(1.,1.),(1.,
1.),(1.,1.),(1.,1.),(1.,1.),(1.,1.),(1.,1.),(1.,1.),(1.,1.),(1.,1.),(1.,
1.),(1.,1.),(1.,1.),(1.,1.),(1.,1.),(1.,1.),(1.,1.),(1.,1.),(1.,1.),(1.,
1.),(1.,1.),(1.,1.),(1.,1.),(1.,1.),(1.,1.),(1.,1.),(1.,1.),(1.,1.),(1.,
1.),(1.,1.),(1.,1.),(1.,1.),(1.,1.),(1.,1.),(1.,1.),(1.,1.),(1.,1.),(1.,
1.),(1.,1.),(1.,1.),(1.,1.),(1.,1.),(1.,1.),(1.,1.),(1.,1.),(1.,1.),(1.,
1.),(1.,1.),(1.,1.),(1.,1.),(1.,1.),(1.,1.),(1.,1.),(1.,1.),(1.,1.),(1.,
1.),(1.,1.),(1.,1.),(1.,1.),(1.,1.),(1.,1.),(1.,1.),(1.,1.),(1.,1.),(1.,
1.),(1.,1.),(1.,1.),(1.,1.),(1.,1.),(1.,1.),(1.,1.),(1.,1.),(1.,1.),(1.,
1.),(1.,1.),(1.,1.),(1.,1.),(1.,1.),(1.,1.),(1.,1.),(1.,1.),(1.,1.),(1.,
1.),(1.,1.),(1.,1.),(1.,1.),(1.,1.),(1.,1.),(1.,1.),(1.,1.),(1.,1.),(1.,
1.),(1.,1.),(1.,1.),(1.,1.),(1.,1.),(1.,1.),(1.,1.),(1.,1.),(1.,1.),(1.,
1.),(1.,1.),(1.,1.),(1.,1.),(1.,1.),(1.,1.),(1.,1.),(1.,1.),(1.,1.),(1.,
1.),(1.,1.),(1.,1.),(1.,1.),(1.,1.),(1.,1.),(1.,1.),(1.,1.),(1.,1.),(1.,
1.),(1.,1.),(1.,1.),(1.,1.),(1.,1.),(1.,1.),(1.,1.),(1.,1.),(1.,1.),(1.,
1.),(1.,1.),(1.,1.),(1.,1.),(1.,1.),(1.,1.),(1.,1.),(1.,1.),(1.,1.),(1.,
1.),(1.,1.),(1.,1.),(1.,1.),(1.,1.),(1.,1.),(1.,1.),(1.,1.),(1.,1.),(1.,
1.),(1.,1.),(1.,1.),(1.,1.),(1.,1.),(1.,1.),(1.,1.),(1.,1.),(1.,1.),(1.,
1.),(1.,1.),(1.,1.),(1.,1.),(1.,1.),(1.,1.),(1.,1.),(1.,1.),(1.,1.),(1.,
1.),(1.,1.),(1.,1.),(1.,1.),(1.,1.),(1.,1.),(1.,1.),(1.,1.),(1.,1.),(1.,
1.)))
REPRESENTATION_ITEM('')
SURFACE()
);
#257=(
BOUNDED_SURFACE()
B_SPLINE_SURFACE(5,1,((#72061,#72062),(#72063,#72064),(#72065,#72066),(#72067,
#72068),(#72069,#72070),(#72071,#72072),(#72073,#72074),(#72075,#72076),
(#72077,#72078),(#72079,#72080),(#72081,#72082),(#72083,#72084),(#72085,
#72086),(#72087,#72088),(#72089,#72090),(#72091,#72092),(#72093,#72094),
(#72095,#72096),(#72097,#72098),(#72099,#72100),(#72101,#72102),(#72103,
#72104),(#72105,#72106),(#72107,#72108),(#72109,#72110),(#72111,#72112),
(#72113,#72114),(#72115,#72116),(#72117,#72118),(#72119,#72120),(#72121,
#72122),(#72123,#72124),(#72125,#72126),(#72127,#72128),(#72129,#72130),
(#72131,#72132),(#72133,#72134),(#72135,#72136),(#72137,#72138),(#72139,
#72140),(#72141,#72142),(#72143,#72144),(#72145,#72146),(#72147,#72148),
(#72149,#72150),(#72151,#72152),(#72153,#72154),(#72155,#72156),(#72157,
#72158),(#72159,#72160),(#72161,#72162),(#72163,#72164),(#72165,#72166),
(#72167,#72168),(#72169,#72170),(#72171,#72172),(#72173,#72174),(#72175,
#72176),(#72177,#72178),(#72179,#72180),(#72181,#72182),(#72183,#72184),
(#72185,#72186),(#72187,#72188),(#72189,#72190),(#72191,#72192),(#72193,
#72194),(#72195,#72196),(#72197,#72198),(#72199,#72200),(#72201,#72202),
(#72203,#72204),(#72205,#72206),(#72207,#72208),(#72209,#72210),(#72211,
#72212),(#72213,#72214),(#72215,#72216),(#72217,#72218),(#72219,#72220),
(#72221,#72222),(#72223,#72224),(#72225,#72226),(#72227,#72228),(#72229,
#72230),(#72231,#72232),(#72233,#72234),(#72235,#72236),(#72237,#72238),
(#72239,#72240),(#72241,#72242),(#72243,#72244),(#72245,#72246),(#72247,
#72248),(#72249,#72250),(#72251,#72252),(#72253,#72254),(#72255,#72256),
(#72257,#72258),(#72259,#72260),(#72261,#72262),(#72263,#72264),(#72265,
#72266),(#72267,#72268),(#72269,#72270),(#72271,#72272),(#72273,#72274),
(#72275,#72276),(#72277,#72278),(#72279,#72280),(#72281,#72282),(#72283,
#72284),(#72285,#72286),(#72287,#72288),(#72289,#72290),(#72291,#72292),
(#72293,#72294),(#72295,#72296),(#72297,#72298),(#72299,#72300),(#72301,
#72302),(#72303,#72304),(#72305,#72306),(#72307,#72308),(#72309,#72310),
(#72311,#72312),(#72313,#72314),(#72315,#72316),(#72317,#72318),(#72319,
#72320),(#72321,#72322),(#72323,#72324),(#72325,#72326),(#72327,#72328),
(#72329,#72330),(#72331,#72332),(#72333,#72334),(#72335,#72336),(#72337,
#72338),(#72339,#72340),(#72341,#72342),(#72343,#72344),(#72345,#72346),
(#72347,#72348),(#72349,#72350),(#72351,#72352),(#72353,#72354),(#72355,
#72356),(#72357,#72358),(#72359,#72360),(#72361,#72362),(#72363,#72364),
(#72365,#72366),(#72367,#72368),(#72369,#72370),(#72371,#72372),(#72373,
#72374),(#72375,#72376),(#72377,#72378),(#72379,#72380),(#72381,#72382),
(#72383,#72384),(#72385,#72386),(#72387,#72388),(#72389,#72390),(#72391,
#72392),(#72393,#72394),(#72395,#72396),(#72397,#72398),(#72399,#72400),
(#72401,#72402),(#72403,#72404),(#72405,#72406),(#72407,#72408),(#72409,
#72410),(#72411,#72412),(#72413,#72414),(#72415,#72416),(#72417,#72418),
(#72419,#72420),(#72421,#72422),(#72423,#72424),(#72425,#72426),(#72427,
#72428),(#72429,#72430),(#72431,#72432),(#72433,#72434),(#72435,#72436),
(#72437,#72438),(#72439,#72440),(#72441,#72442),(#72443,#72444),(#72445,
#72446),(#72447,#72448),(#72449,#72450),(#72451,#72452),(#72453,#72454),
(#72455,#72456),(#72457,#72458),(#72459,#72460),(#72461,#72462),(#72463,
#72464),(#72465,#72466),(#72467,#72468),(#72469,#72470),(#72471,#72472),
(#72473,#72474),(#72475,#72476),(#72477,#72478),(#72479,#72480),(#72481,
#72482),(#72483,#72484),(#72485,#72486),(#72487,#72488),(#72489,#72490),
(#72491,#72492),(#72493,#72494),(#72495,#72496),(#72497,#72498),(#72499,
#72500),(#72501,#72502),(#72503,#72504),(#72505,#72506),(#72507,#72508),
(#72509,#72510),(#72511,#72512),(#72513,#72514),(#72515,#72516),(#72517,
#72518),(#72519,#72520),(#72521,#72522),(#72523,#72524),(#72525,#72526),
(#72527,#72528),(#72529,#72530),(#72531,#72532),(#72533,#72534),(#72535,
#72536),(#72537,#72538),(#72539,#72540),(#72541,#72542),(#72543,#72544),
(#72545,#72546),(#72547,#72548),(#72549,#72550),(#72551,#72552),(#72553,
#72554),(#72555,#72556),(#72557,#72558),(#72559,#72560),(#72561,#72562),
(#72563,#72564),(#72565,#72566),(#72567,#72568),(#72569,#72570),(#72571,
#72572),(#72573,#72574),(#72575,#72576),(#72577,#72578),(#72579,#72580),
(#72581,#72582),(#72583,#72584),(#72585,#72586),(#72587,#72588),(#72589,
#72590),(#72591,#72592),(#72593,#72594),(#72595,#72596),(#72597,#72598),
(#72599,#72600),(#72601,#72602),(#72603,#72604),(#72605,#72606),(#72607,
#72608),(#72609,#72610),(#72611,#72612),(#72613,#72614),(#72615,#72616),
(#72617,#72618),(#72619,#72620),(#72621,#72622),(#72623,#72624),(#72625,
#72626),(#72627,#72628),(#72629,#72630),(#72631,#72632),(#72633,#72634),
(#72635,#72636),(#72637,#72638),(#72639,#72640),(#72641,#72642),(#72643,
#72644),(#72645,#72646),(#72647,#72648),(#72649,#72650),(#72651,#72652),
(#72653,#72654),(#72655,#72656),(#72657,#72658),(#72659,#72660),(#72661,
#72662),(#72663,#72664),(#72665,#72666),(#72667,#72668),(#72669,#72670),
(#72671,#72672),(#72673,#72674),(#72675,#72676),(#72677,#72678),(#72679,
#72680),(#72681,#72682),(#72683,#72684),(#72685,#72686),(#72687,#72688),
(#72689,#72690),(#72691,#72692),(#72693,#72694),(#72695,#72696),(#72697,
#72698),(#72699,#72700),(#72701,#72702),(#72703,#72704),(#72705,#72706),
(#72707,#72708),(#72709,#72710),(#72711,#72712),(#72713,#72714),(#72715,
#72716),(#72717,#72718),(#72719,#72720),(#72721,#72722),(#72723,#72724),
(#72725,#72726),(#72727,#72728),(#72729,#72730),(#72731,#72732),(#72733,
#72734),(#72735,#72736),(#72737,#72738),(#72739,#72740),(#72741,#72742),
(#72743,#72744),(#72745,#72746),(#72747,#72748),(#72749,#72750),(#72751,
#72752),(#72753,#72754),(#72755,#72756),(#72757,#72758),(#72759,#72760),
(#72761,#72762),(#72763,#72764),(#72765,#72766),(#72767,#72768),(#72769,
#72770),(#72771,#72772),(#72773,#72774),(#72775,#72776),(#72777,#72778),
(#72779,#72780),(#72781,#72782),(#72783,#72784),(#72785,#72786),(#72787,
#72788),(#72789,#72790),(#72791,#72792),(#72793,#72794),(#72795,#72796),
(#72797,#72798),(#72799,#72800),(#72801,#72802),(#72803,#72804),(#72805,
#72806),(#72807,#72808),(#72809,#72810),(#72811,#72812),(#72813,#72814),
(#72815,#72816),(#72817,#72818),(#72819,#72820),(#72821,#72822),(#72823,
#72824),(#72825,#72826),(#72827,#72828),(#72829,#72830),(#72831,#72832),
(#72833,#72834),(#72835,#72836),(#72837,#72838),(#72839,#72840),(#72841,
#72842),(#72843,#72844),(#72845,#72846),(#72847,#72848),(#72849,#72850),
(#72851,#72852),(#72853,#72854),(#72855,#72856),(#72857,#72858),(#72859,
#72860),(#72861,#72862),(#72863,#72864),(#72865,#72866),(#72867,#72868),
(#72869,#72870),(#72871,#72872),(#72873,#72874),(#72875,#72876),(#72877,
#72878),(#72879,#72880),(#72881,#72882),(#72883,#72884),(#72885,#72886),
(#72887,#72888),(#72889,#72890),(#72891,#72892),(#72893,#72894),(#72895,
#72896),(#72897,#72898),(#72899,#72900),(#72901,#72902),(#72903,#72904),
(#72905,#72906),(#72907,#72908),(#72909,#72910),(#72911,#72912),(#72913,
#72914),(#72915,#72916),(#72917,#72918),(#72919,#72920),(#72921,#72922),
(#72923,#72924),(#72925,#72926),(#72927,#72928),(#72929,#72930),(#72931,
#72932),(#72933,#72934),(#72935,#72936),(#72937,#72938),(#72939,#72940),
(#72941,#72942),(#72943,#72944),(#72945,#72946),(#72947,#72948),(#72949,
#72950),(#72951,#72952),(#72953,#72954),(#72955,#72956),(#72957,#72958),
(#72959,#72960),(#72961,#72962),(#72963,#72964),(#72965,#72966),(#72967,
#72968),(#72969,#72970),(#72971,#72972),(#72973,#72974),(#72975,#72976),
(#72977,#72978),(#72979,#72980),(#72981,#72982),(#72983,#72984),(#72985,
#72986),(#72987,#72988),(#72989,#72990),(#72991,#72992),(#72993,#72994),
(#72995,#72996),(#72997,#72998),(#72999,#73000),(#73001,#73002),(#73003,
#73004),(#73005,#73006),(#73007,#73008),(#73009,#73010),(#73011,#73012),
(#73013,#73014),(#73015,#73016),(#73017,#73018),(#73019,#73020),(#73021,
#73022),(#73023,#73024),(#73025,#73026),(#73027,#73028),(#73029,#73030),
(#73031,#73032),(#73033,#73034),(#73035,#73036),(#73037,#73038),(#73039,
#73040),(#73041,#73042),(#73043,#73044),(#73045,#73046),(#73047,#73048),
(#73049,#73050),(#73051,#73052),(#73053,#73054),(#73055,#73056),(#73057,
#73058),(#73059,#73060),(#73061,#73062),(#73063,#73064),(#73065,#73066),
(#73067,#73068),(#73069,#73070),(#73071,#73072),(#73073,#73074),(#73075,
#73076),(#73077,#73078),(#73079,#73080),(#73081,#73082),(#73083,#73084),
(#73085,#73086),(#73087,#73088),(#73089,#73090),(#73091,#73092),(#73093,
#73094),(#73095,#73096),(#73097,#73098),(#73099,#73100),(#73101,#73102),
(#73103,#73104),(#73105,#73106),(#73107,#73108),(#73109,#73110),(#73111,
#73112),(#73113,#73114),(#73115,#73116),(#73117,#73118),(#73119,#73120),
(#73121,#73122),(#73123,#73124),(#73125,#73126),(#73127,#73128),(#73129,
#73130),(#73131,#73132),(#73133,#73134),(#73135,#73136),(#73137,#73138),
(#73139,#73140),(#73141,#73142),(#73143,#73144),(#73145,#73146),(#73147,
#73148),(#73149,#73150),(#73151,#73152),(#73153,#73154),(#73155,#73156),
(#73157,#73158),(#73159,#73160),(#73161,#73162),(#73163,#73164),(#73165,
#73166),(#73167,#73168),(#73169,#73170),(#73171,#73172),(#73173,#73174),
(#73175,#73176),(#73177,#73178),(#73179,#73180),(#73181,#73182),(#73183,
#73184),(#73185,#73186),(#73187,#73188),(#73189,#73190),(#73191,#73192),
(#73193,#73194),(#73195,#73196),(#73197,#73198),(#73199,#73200),(#73201,
#73202),(#73203,#73204),(#73205,#73206),(#73207,#73208),(#73209,#73210),
(#73211,#73212),(#73213,#73214),(#73215,#73216),(#73217,#73218),(#73219,
#73220),(#73221,#73222),(#73223,#73224),(#73225,#73226),(#73227,#73228),
(#73229,#73230),(#73231,#73232),(#73233,#73234),(#73235,#73236),(#73237,
#73238),(#73239,#73240),(#73241,#73242),(#73243,#73244),(#73245,#73246),
(#73247,#73248),(#73249,#73250),(#73251,#73252),(#73253,#73254),(#73255,
#73256),(#73257,#73258),(#73259,#73260),(#73261,#73262),(#73263,#73264),
(#73265,#73266),(#73267,#73268),(#73269,#73270),(#73271,#73272),(#73273,
#73274),(#73275,#73276),(#73277,#73278),(#73279,#73280),(#73281,#73282),
(#73283,#73284),(#73285,#73286),(#73287,#73288),(#73289,#73290),(#73291,
#73292),(#73293,#73294),(#73295,#73296),(#73297,#73298),(#73299,#73300),
(#73301,#73302),(#73303,#73304),(#73305,#73306),(#73307,#73308),(#73309,
#73310),(#73311,#73312),(#73313,#73314),(#73315,#73316),(#73317,#73318),
(#73319,#73320),(#73321,#73322),(#73323,#73324),(#73325,#73326),(#73327,
#73328),(#73329,#73330),(#73331,#73332),(#73333,#73334),(#73335,#73336),
(#73337,#73338),(#73339,#73340),(#73341,#73342),(#73343,#73344),(#73345,
#73346),(#73347,#73348),(#73349,#73350),(#73351,#73352),(#73353,#73354),
(#73355,#73356),(#73357,#73358),(#73359,#73360),(#73361,#73362),(#73363,
#73364),(#73365,#73366),(#73367,#73368),(#73369,#73370),(#73371,#73372),
(#73373,#73374),(#73375,#73376),(#73377,#73378),(#73379,#73380),(#73381,
#73382),(#73383,#73384),(#73385,#73386),(#73387,#73388),(#73389,#73390),
(#73391,#73392),(#73393,#73394),(#73395,#73396),(#73397,#73398),(#73399,
#73400),(#73401,#73402),(#73403,#73404),(#73405,#73406),(#73407,#73408),
(#73409,#73410),(#73411,#73412),(#73413,#73414),(#73415,#73416),(#73417,
#73418),(#73419,#73420),(#73421,#73422),(#73423,#73424),(#73425,#73426),
(#73427,#73428),(#73429,#73430),(#73431,#73432),(#73433,#73434),(#73435,
#73436),(#73437,#73438),(#73439,#73440),(#73441,#73442),(#73443,#73444),
(#73445,#73446),(#73447,#73448),(#73449,#73450),(#73451,#73452),(#73453,
#73454),(#73455,#73456),(#73457,#73458),(#73459,#73460),(#73461,#73462),
(#73463,#73464),(#73465,#73466),(#73467,#73468),(#73469,#73470),(#73471,
#73472),(#73473,#73474),(#73475,#73476),(#73477,#73478),(#73479,#73480),
(#73481,#73482),(#73483,#73484),(#73485,#73486),(#73487,#73488),(#73489,
#73490),(#73491,#73492),(#73493,#73494),(#73495,#73496),(#73497,#73498),
(#73499,#73500),(#73501,#73502),(#73503,#73504),(#73505,#73506),(#73507,
#73508),(#73509,#73510),(#73511,#73512),(#73513,#73514),(#73515,#73516),
(#73517,#73518),(#73519,#73520),(#73521,#73522),(#73523,#73524),(#73525,
#73526),(#73527,#73528),(#73529,#73530),(#73531,#73532),(#73533,#73534),
(#73535,#73536),(#73537,#73538),(#73539,#73540),(#73541,#73542),(#73543,
#73544),(#73545,#73546),(#73547,#73548),(#73549,#73550),(#73551,#73552),
(#73553,#73554),(#73555,#73556),(#73557,#73558),(#73559,#73560),(#73561,
#73562),(#73563,#73564),(#73565,#73566),(#73567,#73568),(#73569,#73570),
(#73571,#73572),(#73573,#73574),(#73575,#73576),(#73577,#73578),(#73579,
#73580),(#73581,#73582),(#73583,#73584),(#73585,#73586),(#73587,#73588),
(#73589,#73590),(#73591,#73592),(#73593,#73594),(#73595,#73596),(#73597,
#73598),(#73599,#73600),(#73601,#73602),(#73603,#73604),(#73605,#73606),
(#73607,#73608),(#73609,#73610),(#73611,#73612),(#73613,#73614),(#73615,
#73616),(#73617,#73618),(#73619,#73620),(#73621,#73622),(#73623,#73624),
(#73625,#73626),(#73627,#73628),(#73629,#73630),(#73631,#73632),(#73633,
#73634),(#73635,#73636),(#73637,#73638),(#73639,#73640),(#73641,#73642),
(#73643,#73644),(#73645,#73646),(#73647,#73648),(#73649,#73650),(#73651,
#73652),(#73653,#73654),(#73655,#73656),(#73657,#73658),(#73659,#73660),
(#73661,#73662),(#73663,#73664),(#73665,#73666),(#73667,#73668),(#73669,
#73670),(#73671,#73672),(#73673,#73674),(#73675,#73676),(#73677,#73678),
(#73679,#73680),(#73681,#73682),(#73683,#73684),(#73685,#73686),(#73687,
#73688),(#73689,#73690),(#73691,#73692),(#73693,#73694),(#73695,#73696),
(#73697,#73698),(#73699,#73700),(#73701,#73702),(#73703,#73704),(#73705,
#73706),(#73707,#73708),(#73709,#73710),(#73711,#73712),(#73713,#73714),
(#73715,#73716),(#73717,#73718),(#73719,#73720),(#73721,#73722),(#73723,
#73724),(#73725,#73726),(#73727,#73728),(#73729,#73730),(#73731,#73732),
(#73733,#73734),(#73735,#73736),(#73737,#73738),(#73739,#73740),(#73741,
#73742),(#73743,#73744),(#73745,#73746),(#73747,#73748),(#73749,#73750),
(#73751,#73752),(#73753,#73754),(#73755,#73756),(#73757,#73758),(#73759,
#73760),(#73761,#73762),(#73763,#73764),(#73765,#73766),(#73767,#73768),
(#73769,#73770),(#73771,#73772),(#73773,#73774),(#73775,#73776),(#73777,
#73778),(#73779,#73780),(#73781,#73782),(#73783,#73784),(#73785,#73786),
(#73787,#73788),(#73789,#73790),(#73791,#73792),(#73793,#73794),(#73795,
#73796),(#73797,#73798),(#73799,#73800),(#73801,#73802),(#73803,#73804),
(#73805,#73806),(#73807,#73808),(#73809,#73810),(#73811,#73812),(#73813,
#73814),(#73815,#73816),(#73817,#73818),(#73819,#73820),(#73821,#73822),
(#73823,#73824),(#73825,#73826),(#73827,#73828),(#73829,#73830),(#73831,
#73832),(#73833,#73834),(#73835,#73836),(#73837,#73838),(#73839,#73840),
(#73841,#73842),(#73843,#73844),(#73845,#73846),(#73847,#73848),(#73849,
#73850),(#73851,#73852),(#73853,#73854),(#73855,#73856),(#73857,#73858),
(#73859,#73860),(#73861,#73862),(#73863,#73864),(#73865,#73866),(#73867,
#73868),(#73869,#73870),(#73871,#73872),(#73873,#73874),(#73875,#73876),
(#73877,#73878),(#73879,#73880),(#73881,#73882),(#73883,#73884),(#73885,
#73886),(#73887,#73888),(#73889,#73890),(#73891,#73892),(#73893,#73894),
(#73895,#73896),(#73897,#73898),(#73899,#73900),(#73901,#73902),(#73903,
#73904),(#73905,#73906),(#73907,#73908),(#73909,#73910),(#73911,#73912),
(#73913,#73914),(#73915,#73916),(#73917,#73918),(#73919,#73920),(#73921,
#73922),(#73923,#73924),(#73925,#73926),(#73927,#73928),(#73929,#73930),
(#73931,#73932),(#73933,#73934),(#73935,#73936),(#73937,#73938),(#73939,
#73940),(#73941,#73942),(#73943,#73944),(#73945,#73946),(#73947,#73948),
(#73949,#73950),(#73951,#73952),(#73953,#73954),(#73955,#73956),(#73957,
#73958),(#73959,#73960),(#73961,#73962),(#73963,#73964),(#73965,#73966),
(#73967,#73968),(#73969,#73970),(#73971,#73972),(#73973,#73974),(#73975,
#73976),(#73977,#73978),(#73979,#73980),(#73981,#73982),(#73983,#73984),
(#73985,#73986),(#73987,#73988),(#73989,#73990),(#73991,#73992),(#73993,
#73994),(#73995,#73996),(#73997,#73998),(#73999,#74000),(#74001,#74002),
(#74003,#74004),(#74005,#74006),(#74007,#74008),(#74009,#74010),(#74011,
#74012),(#74013,#74014),(#74015,#74016),(#74017,#74018),(#74019,#74020),
(#74021,#74022),(#74023,#74024),(#74025,#74026),(#74027,#74028),(#74029,
#74030),(#74031,#74032),(#74033,#74034),(#74035,#74036),(#74037,#74038),
(#74039,#74040),(#74041,#74042),(#74043,#74044),(#74045,#74046),(#74047,
#74048),(#74049,#74050),(#74051,#74052),(#74053,#74054),(#74055,#74056),
(#74057,#74058),(#74059,#74060),(#74061,#74062),(#74063,#74064),(#74065,
#74066),(#74067,#74068),(#74069,#74070)),.UNSPECIFIED.,.F.,.F.,.F.)
B_SPLINE_SURFACE_WITH_KNOTS((6,1,1,1,1,1,1,1,1,1,1,1,1,1,1,1,1,1,1,1,1,
1,1,1,1,1,1,1,1,1,1,1,1,1,1,1,1,1,1,1,1,1,1,1,1,1,1,1,1,1,1,1,1,1,1,1,1,
1,1,1,1,1,1,1,1,1,1,1,1,1,1,1,1,1,1,1,1,1,1,1,1,1,1,1,1,1,1,1,1,1,1,1,1,
1,1,1,1,1,1,1,1,1,1,1,1,1,1,1,1,1,1,1,1,1,1,1,1,1,1,1,1,1,1,1,1,1,1,1,1,
1,1,1,1,1,1,1,1,1,1,1,1,1,1,1,1,1,1,1,1,1,1,1,1,1,1,1,1,1,1,1,1,1,1,1,1,
1,1,1,1,1,1,1,1,1,1,1,1,1,1,1,1,1,1,1,1,1,1,1,1,1,1,1,1,1,1,1,1,1,1,1,1,
1,1,1,1,1,1,1,1,1,1,1,1,1,1,1,1,1,1,1,1,1,1,1,1,1,1,1,1,1,1,1,1,1,1,1,1,
1,1,1,1,1,1,1,1,1,1,1,1,1,1,1,1,1,1,1,1,1,1,1,1,1,1,1,1,1,1,1,1,1,1,1,1,
1,1,1,1,1,1,1,1,1,1,1,1,1,1,1,1,1,1,1,1,1,1,1,1,1,1,1,1,1,1,1,1,1,1,1,1,
1,1,1,1,1,1,1,1,1,1,1,1,1,1,1,1,1,1,1,1,1,1,1,1,1,1,1,1,1,1,1,1,1,1,1,1,
1,1,1,1,1,1,1,1,1,1,1,1,1,1,1,1,1,1,1,1,1,1,1,1,1,1,1,1,1,1,1,1,1,1,1,1,
1,1,1,1,1,1,1,1,1,1,1,1,1,1,1,1,1,1,1,1,1,1,1,1,1,1,1,1,1,1,1,1,1,1,1,1,
1,1,1,1,1,1,1,1,1,1,1,1,1,1,1,1,1,1,1,1,1,1,1,1,1,1,1,1,1,1,1,1,1,1,1,1,
1,1,1,1,1,1,1,1,1,1,1,1,1,1,1,1,1,1,1,1,1,1,1,1,1,1,1,1,1,1,1,1,1,1,1,1,
1,1,1,1,1,1,1,1,1,1,1,1,1,1,1,1,1,1,1,1,1,1,1,1,1,1,1,1,1,1,1,1,1,1,1,1,
1,1,1,1,1,1,1,1,1,1,1,1,1,1,1,1,1,1,1,1,1,1,1,1,1,1,1,1,1,1,1,1,1,1,1,1,
1,1,1,1,1,1,1,1,1,1,1,1,1,1,1,1,1,1,1,1,1,1,1,1,1,1,1,1,1,1,1,1,1,1,1,1,
1,1,1,1,1,1,1,1,1,1,1,1,1,1,1,1,1,1,1,1,1,1,1,1,1,1,1,1,1,1,1,1,1,1,1,1,
1,1,1,1,1,1,1,1,1,1,1,1,1,1,1,1,1,1,1,1,1,1,1,1,1,1,1,1,1,1,1,1,1,1,1,1,
1,1,1,1,1,1,1,1,1,1,1,1,1,1,1,1,1,1,1,1,1,1,1,1,1,1,1,1,1,1,1,1,1,1,1,1,
1,1,1,1,1,1,1,1,1,1,1,1,1,1,1,1,1,1,1,1,1,1,1,1,1,1,1,1,1,1,1,1,1,1,1,1,
1,1,1,1,1,1,1,1,1,1,1,1,1,1,1,1,1,1,1,1,1,1,1,1,1,1,1,1,1,1,1,1,1,1,1,1,
1,1,1,1,1,1,1,1,1,1,1,1,1,1,1,1,1,1,1,1,1,1,1,1,1,1,1,1,1,1,1,1,1,1,1,1,
1,1,1,1,1,1,1,1,1,1,1,1,1,1,1,1,1,1,1,1,1,1,1,1,1,1,1,1,1,1,1,1,1,1,1,1,
1,1,1,1,1,1,1,1,1,1,1,1,1,1,1,1,1,1,1,1,1,1,1,1,1,1,1,1,1,1,1,1,1,1,1,1,
1,1,1,1,1,1,1,1,1,1,1,1,1,1,1,1,1,1,1,1,1,1,1,1,1,1,1,1,1,1,1,1,1,1,1,1,
1,1,1,1,1,1,1,1,1,1,1,1,1,1,1,1,1,1,1,1,1,1,1,1,1,1,1,1,1,1,1,1,1,1,1,1,
1,1,1,1,1,1,1,1,1,1,1,1,1,1,1,1,1,1,1,1,1,1,1,1,1,1,1,1,1,1,1,1,1,1,1,1,
1,1,1,1,1,1,1,6),(2,2),(-1.,-0.999000000000001,-0.998000000000001,-0.997000000000001,
-0.996000000000001,-0.995000000000001,-0.994000000000001,-0.993000000000001,
-0.992000000000001,-0.991000000000001,-0.990000000000001,-0.989000000000001,
-0.988000000000001,-0.987000000000001,-0.986000000000001,-0.985000000000001,
-0.984000000000001,-0.983000000000001,-0.982000000000001,-0.981000000000001,
-0.980000000000001,-0.979000000000001,-0.978000000000001,-0.977000000000001,
-0.976000000000001,-0.975000000000001,-0.974000000000001,-0.973000000000001,
-0.972000000000001,-0.971000000000001,-0.970000000000001,-0.969000000000001,
-0.968000000000001,-0.967000000000001,-0.966000000000001,-0.965000000000001,
-0.964000000000001,-0.963000000000001,-0.962000000000001,-0.961000000000001,
-0.960000000000001,-0.959000000000001,-0.958000000000001,-0.957000000000001,
-0.956000000000001,-0.955000000000001,-0.954000000000001,-0.953000000000001,
-0.952000000000001,-0.951000000000001,-0.950000000000001,-0.949000000000001,
-0.948000000000001,-0.947000000000001,-0.946000000000001,-0.945000000000001,
-0.944000000000001,-0.943000000000001,-0.942000000000001,-0.941000000000001,
-0.940000000000001,-0.939000000000001,-0.938000000000001,-0.937000000000001,
-0.936000000000001,-0.935000000000001,-0.934000000000001,-0.933000000000001,
-0.932000000000001,-0.931000000000001,-0.930000000000001,-0.929000000000001,
-0.928000000000001,-0.927000000000001,-0.926000000000001,-0.925000000000001,
-0.924000000000001,-0.923000000000001,-0.922000000000001,-0.921000000000001,
-0.920000000000001,-0.919000000000001,-0.918000000000001,-0.917000000000001,
-0.916000000000001,-0.915000000000001,-0.914000000000001,-0.913000000000001,
-0.912000000000001,-0.911000000000001,-0.910000000000001,-0.909000000000001,
-0.908000000000001,-0.907000000000001,-0.906000000000001,-0.905000000000001,
-0.904000000000001,-0.903000000000001,-0.902000000000001,-0.901000000000001,
-0.900000000000001,-0.899000000000001,-0.898000000000001,-0.897000000000001,
-0.896000000000001,-0.895000000000001,-0.894000000000001,-0.893000000000001,
-0.892000000000001,-0.891000000000001,-0.890000000000001,-0.889000000000001,
-0.888000000000001,-0.887000000000001,-0.886000000000001,-0.885000000000001,
-0.884000000000001,-0.883000000000001,-0.882000000000001,-0.881000000000001,
-0.880000000000001,-0.879000000000001,-0.878000000000001,-0.877000000000001,
-0.876000000000001,-0.875000000000001,-0.874000000000001,-0.873000000000001,
-0.872000000000001,-0.871000000000001,-0.870000000000001,-0.869000000000001,
-0.868000000000001,-0.867000000000001,-0.866000000000001,-0.865000000000001,
-0.864000000000001,-0.863000000000001,-0.862000000000001,-0.861000000000001,
-0.860000000000001,-0.859000000000001,-0.858000000000001,-0.857000000000001,
-0.856000000000001,-0.855000000000001,-0.854000000000001,-0.853000000000001,
-0.852000000000001,-0.851000000000001,-0.850000000000001,-0.849000000000001,
-0.848000000000001,-0.847000000000001,-0.846000000000001,-0.845000000000001,
-0.844000000000001,-0.843000000000001,-0.842000000000001,-0.841000000000001,
-0.840000000000001,-0.839000000000001,-0.838000000000001,-0.837000000000001,
-0.836000000000001,-0.835000000000001,-0.834000000000001,-0.833000000000001,
-0.832000000000001,-0.831000000000001,-0.830000000000001,-0.829000000000001,
-0.828000000000001,-0.827000000000001,-0.826000000000001,-0.825000000000001,
-0.824000000000001,-0.823000000000001,-0.822000000000001,-0.821000000000001,
-0.820000000000001,-0.819000000000001,-0.818000000000001,-0.817000000000001,
-0.816000000000001,-0.815000000000001,-0.814000000000001,-0.813000000000001,
-0.812000000000001,-0.811000000000001,-0.810000000000001,-0.809000000000001,
-0.808000000000001,-0.807000000000001,-0.806000000000001,-0.805000000000001,
-0.804000000000001,-0.803000000000001,-0.802000000000001,-0.801000000000001,
-0.800000000000001,-0.799000000000001,-0.798000000000001,-0.797000000000001,
-0.796000000000001,-0.795000000000001,-0.794000000000001,-0.793000000000001,
-0.792000000000001,-0.791000000000001,-0.790000000000001,-0.789000000000001,
-0.788000000000001,-0.787000000000001,-0.786000000000001,-0.785000000000001,
-0.784000000000001,-0.783000000000001,-0.782000000000001,-0.781000000000001,
-0.780000000000001,-0.779000000000001,-0.778000000000001,-0.777000000000001,
-0.776000000000001,-0.775000000000001,-0.774000000000001,-0.773000000000001,
-0.772000000000001,-0.771000000000001,-0.770000000000001,-0.769000000000001,
-0.768000000000001,-0.767000000000001,-0.766000000000001,-0.765000000000001,
-0.764000000000001,-0.763000000000001,-0.762000000000001,-0.761000000000001,
-0.760000000000001,-0.759000000000001,-0.758000000000001,-0.757000000000001,
-0.756000000000001,-0.755000000000001,-0.754000000000001,-0.753000000000001,
-0.752000000000001,-0.751000000000001,-0.750000000000001,-0.749000000000001,
-0.748000000000001,-0.747000000000001,-0.746000000000001,-0.745000000000001,
-0.744000000000001,-0.743000000000001,-0.742000000000001,-0.741000000000001,
-0.740000000000001,-0.739000000000001,-0.738000000000001,-0.737000000000001,
-0.736000000000001,-0.735000000000001,-0.734000000000001,-0.733000000000001,
-0.732000000000001,-0.731000000000001,-0.730000000000001,-0.729000000000001,
-0.728000000000001,-0.727000000000001,-0.726000000000001,-0.725000000000001,
-0.724000000000001,-0.723000000000001,-0.722000000000001,-0.721000000000001,
-0.720000000000001,-0.719000000000001,-0.718000000000001,-0.717000000000001,
-0.716000000000001,-0.715000000000001,-0.714000000000001,-0.713000000000001,
-0.712000000000001,-0.711000000000001,-0.710000000000001,-0.709000000000001,
-0.708000000000001,-0.707000000000001,-0.706000000000001,-0.705000000000001,
-0.704000000000001,-0.703000000000001,-0.702000000000001,-0.701000000000001,
-0.700000000000001,-0.699000000000001,-0.698000000000001,-0.697000000000001,
-0.696000000000001,-0.695000000000001,-0.694000000000001,-0.693000000000001,
-0.692000000000001,-0.691000000000001,-0.690000000000001,-0.689000000000001,
-0.688000000000001,-0.687,-0.686,-0.685,-0.684,-0.683,-0.682,-0.681,-0.68,
-0.679,-0.678,-0.677,-0.676,-0.675,-0.674,-0.673,-0.672,-0.671,-0.67,-0.669,
-0.668,-0.667,-0.666,-0.665,-0.664,-0.663,-0.662,-0.661,-0.66,-0.659,-0.658,
-0.657,-0.656,-0.655,-0.654,-0.653,-0.652,-0.651,-0.65,-0.649,-0.648,-0.647,
-0.646,-0.645,-0.644,-0.643,-0.642,-0.641,-0.64,-0.639,-0.638,-0.637,-0.636,
-0.635,-0.634,-0.633,-0.632,-0.631,-0.63,-0.629,-0.628,-0.627,-0.626,-0.625,
-0.624,-0.623,-0.622,-0.621,-0.62,-0.619,-0.618,-0.617,-0.616,-0.615,-0.614,
-0.613,-0.612,-0.611,-0.61,-0.609,-0.608,-0.607,-0.606,-0.605,-0.604,-0.603,
-0.602,-0.601,-0.6,-0.599,-0.598,-0.597,-0.596,-0.595,-0.594,-0.593,-0.592,
-0.591,-0.59,-0.589,-0.588,-0.587,-0.586,-0.585,-0.584,-0.583,-0.582,-0.581,
-0.58,-0.579,-0.578,-0.577,-0.576,-0.575,-0.574,-0.573,-0.572,-0.571,-0.57,
-0.569,-0.568,-0.567,-0.566,-0.565,-0.564,-0.563,-0.562,-0.561,-0.56,-0.559,
-0.558,-0.557,-0.556,-0.555,-0.554,-0.553,-0.552,-0.551,-0.55,-0.549,-0.548,
-0.547,-0.546,-0.545,-0.544,-0.543,-0.542,-0.541,-0.54,-0.539,-0.538,-0.537,
-0.536,-0.535,-0.534,-0.533,-0.532,-0.531,-0.53,-0.529,-0.528,-0.527,-0.526,
-0.525,-0.524,-0.523,-0.522,-0.521,-0.52,-0.519,-0.518,-0.517,-0.516,-0.515,
-0.514,-0.513,-0.512,-0.511,-0.51,-0.509,-0.508,-0.507,-0.506,-0.505,-0.504,
-0.503,-0.502,-0.501,-0.5,-0.499,-0.498,-0.497,-0.496,-0.495,-0.494,-0.493,
-0.492,-0.491,-0.49,-0.489,-0.488,-0.487,-0.486,-0.485,-0.484,-0.483,-0.482,
-0.481,-0.48,-0.479,-0.478,-0.477,-0.476,-0.475,-0.474,-0.473,-0.472,-0.471,
-0.47,-0.469,-0.468,-0.467,-0.466,-0.465,-0.464,-0.463,-0.462,-0.461,-0.46,
-0.459,-0.458,-0.457,-0.456,-0.455,-0.454,-0.453,-0.452,-0.451,-0.45,-0.449,
-0.448,-0.447,-0.446,-0.445,-0.444,-0.443,-0.442,-0.441,-0.44,-0.439,-0.438,
-0.437,-0.436,-0.435,-0.434,-0.433,-0.432,-0.431,-0.43,-0.429,-0.428,-0.427,
-0.426,-0.425,-0.424,-0.423,-0.422,-0.421,-0.42,-0.419,-0.418,-0.417,-0.416,
-0.415,-0.414,-0.413,-0.412,-0.411,-0.41,-0.409,-0.408,-0.407,-0.406,-0.405,
-0.404,-0.403,-0.402,-0.401,-0.4,-0.399,-0.398,-0.397,-0.396,-0.395,-0.394,
-0.393,-0.392,-0.391,-0.39,-0.389,-0.388,-0.387,-0.386,-0.385,-0.384,-0.383,
-0.382,-0.381,-0.38,-0.379,-0.378,-0.377,-0.376,-0.375,-0.374,-0.373,-0.372,
-0.371,-0.37,-0.369,-0.368,-0.367,-0.366,-0.365,-0.364,-0.363,-0.362,-0.361,
-0.36,-0.359,-0.358,-0.357,-0.356,-0.355,-0.354,-0.353,-0.352,-0.351,-0.35,
-0.349,-0.348,-0.347,-0.346,-0.345,-0.344,-0.343,-0.342,-0.341,-0.34,-0.339,
-0.338,-0.337,-0.336,-0.335,-0.334,-0.333,-0.332,-0.331,-0.33,-0.329,-0.328,
-0.327,-0.326,-0.325,-0.324,-0.323,-0.322,-0.321,-0.32,-0.319,-0.318,-0.317,
-0.316,-0.315,-0.314,-0.313,-0.312,-0.311,-0.31,-0.309,-0.308,-0.307,-0.306,
-0.305,-0.304,-0.303,-0.302,-0.301,-0.3,-0.299,-0.298,-0.297,-0.296,-0.295,
-0.294,-0.293,-0.292,-0.291,-0.29,-0.289,-0.288,-0.287,-0.286,-0.285,-0.284,
-0.283,-0.282,-0.281,-0.28,-0.279,-0.278,-0.277,-0.276,-0.275,-0.274,-0.273,
-0.272,-0.271,-0.27,-0.269,-0.268,-0.267,-0.266,-0.265,-0.264,-0.263,-0.262,
-0.261,-0.26,-0.259,-0.258,-0.257,-0.256,-0.255,-0.254,-0.253,-0.252,-0.251,
-0.25,-0.249,-0.248,-0.247,-0.246,-0.245,-0.244,-0.243,-0.242,-0.241,-0.24,
-0.239,-0.238,-0.237,-0.236,-0.235,-0.234,-0.233,-0.232,-0.231,-0.23,-0.229,
-0.228,-0.227,-0.226,-0.225,-0.224,-0.223,-0.222,-0.221,-0.22,-0.219,-0.218,
-0.217,-0.216,-0.215,-0.214,-0.213,-0.212,-0.211,-0.21,-0.209,-0.208,-0.207,
-0.206,-0.205,-0.204,-0.203,-0.202,-0.201,-0.2,-0.199,-0.198,-0.197,-0.196,
-0.195,-0.194,-0.193,-0.192,-0.191,-0.19,-0.189,-0.188,-0.187,-0.186,-0.185,
-0.184,-0.183,-0.182,-0.181,-0.18,-0.179,-0.178,-0.177,-0.176,-0.175,-0.174,
-0.173,-0.172,-0.171,-0.17,-0.169,-0.168,-0.167,-0.166,-0.165,-0.164,-0.163,
-0.162,-0.161,-0.16,-0.159,-0.158,-0.157,-0.156,-0.155,-0.154,-0.153,-0.152,
-0.151,-0.15,-0.149,-0.148,-0.147,-0.146,-0.145,-0.144,-0.143,-0.142,-0.141,
-0.14,-0.139,-0.138,-0.137,-0.136,-0.135,-0.134,-0.133,-0.132,-0.131,-0.13,
-0.129,-0.128,-0.127,-0.126,-0.125,-0.124,-0.123,-0.122,-0.121,-0.12,-0.119,
-0.118,-0.117,-0.116,-0.115,-0.114,-0.113,-0.112,-0.111,-0.11,-0.109,-0.108,
-0.107,-0.106,-0.105,-0.104,-0.103,-0.102,-0.101,-0.1,-0.0990000000000001,
-0.0980000000000001,-0.0970000000000001,-0.0960000000000001,-0.0950000000000001,
-0.0940000000000001,-0.0930000000000001,-0.0920000000000001,-0.0910000000000001,
-0.0900000000000001,-0.0890000000000001,-0.0880000000000001,-0.0870000000000001,
-0.0860000000000001,-0.0850000000000001,-0.0840000000000001,-0.0830000000000001,
-0.0820000000000001,-0.0810000000000001,-0.0800000000000001,-0.0790000000000001,
-0.0780000000000001,-0.0770000000000001,-0.0760000000000001,-0.0750000000000001,
-0.0740000000000001,-0.0730000000000001,-0.0720000000000001,-0.071,-0.07,
-0.069,-0.068,-0.067,-0.066,-0.065,-0.064,-0.063,-0.062,-0.061,-0.06,-0.059,
-0.058,-0.057,-0.056,-0.055,-0.054,-0.053,-0.052,-0.051,-0.05,-0.049,-0.048,
-0.047,-0.046,-0.045,-0.044,-0.043,-0.042,-0.041,-0.04,-0.039,-0.038,-0.037,
-0.036,-0.035,-0.034,-0.033,-0.032,-0.031,-0.03,-0.029,-0.028,-0.027,-0.026,
-0.025,-0.024,-0.023,-0.022,-0.021,-0.02,-0.019,-0.018,-0.017,-0.016,-0.015,
-0.014,-0.013,-0.012,-0.011,-0.01,-0.009,-0.008,-0.007,-0.006,-0.005,-0.004,
-0.003,-0.002,-0.001,0.),(0.,2.),.UNSPECIFIED.)
GEOMETRIC_REPRESENTATION_ITEM()
RATIONAL_B_SPLINE_SURFACE(((1.,1.),(1.,1.),(1.,1.),(1.,1.),(1.,1.),(1.,
1.),(1.,1.),(1.,1.),(1.,1.),(1.,1.),(1.,1.),(1.,1.),(1.,1.),(1.,1.),(1.,
1.),(1.,1.),(1.,1.),(1.,1.),(1.,1.),(1.,1.),(1.,1.),(1.,1.),(1.,1.),(1.,
1.),(1.,1.),(1.,1.),(1.,1.),(1.,1.),(1.,1.),(1.,1.),(1.,1.),(1.,1.),(1.,
1.),(1.,1.),(1.,1.),(1.,1.),(1.,1.),(1.,1.),(1.,1.),(1.,1.),(1.,1.),(1.,
1.),(1.,1.),(1.,1.),(1.,1.),(1.,1.),(1.,1.),(1.,1.),(1.,1.),(1.,1.),(1.,
1.),(1.,1.),(1.,1.),(1.,1.),(1.,1.),(1.,1.),(1.,1.),(1.,1.),(1.,1.),(1.,
1.),(1.,1.),(1.,1.),(1.,1.),(1.,1.),(1.,1.),(1.,1.),(1.,1.),(1.,1.),(1.,
1.),(1.,1.),(1.,1.),(1.,1.),(1.,1.),(1.,1.),(1.,1.),(1.,1.),(1.,1.),(1.,
1.),(1.,1.),(1.,1.),(1.,1.),(1.,1.),(1.,1.),(1.,1.),(1.,1.),(1.,1.),(1.,
1.),(1.,1.),(1.,1.),(1.,1.),(1.,1.),(1.,1.),(1.,1.),(1.,1.),(1.,1.),(1.,
1.),(1.,1.),(1.,1.),(1.,1.),(1.,1.),(1.,1.),(1.,1.),(1.,1.),(1.,1.),(1.,
1.),(1.,1.),(1.,1.),(1.,1.),(1.,1.),(1.,1.),(1.,1.),(1.,1.),(1.,1.),(1.,
1.),(1.,1.),(1.,1.),(1.,1.),(1.,1.),(1.,1.),(1.,1.),(1.,1.),(1.,1.),(1.,
1.),(1.,1.),(1.,1.),(1.,1.),(1.,1.),(1.,1.),(1.,1.),(1.,1.),(1.,1.),(1.,
1.),(1.,1.),(1.,1.),(1.,1.),(1.,1.),(1.,1.),(1.,1.),(1.,1.),(1.,1.),(1.,
1.),(1.,1.),(1.,1.),(1.,1.),(1.,1.),(1.,1.),(1.,1.),(1.,1.),(1.,1.),(1.,
1.),(1.,1.),(1.,1.),(1.,1.),(1.,1.),(1.,1.),(1.,1.),(1.,1.),(1.,1.),(1.,
1.),(1.,1.),(1.,1.),(1.,1.),(1.,1.),(1.,1.),(1.,1.),(1.,1.),(1.,1.),(1.,
1.),(1.,1.),(1.,1.),(1.,1.),(1.,1.),(1.,1.),(1.,1.),(1.,1.),(1.,1.),(1.,
1.),(1.,1.),(1.,1.),(1.,1.),(1.,1.),(1.,1.),(1.,1.),(1.,1.),(1.,1.),(1.,
1.),(1.,1.),(1.,1.),(1.,1.),(1.,1.),(1.,1.),(1.,1.),(1.,1.),(1.,1.),(1.,
1.),(1.,1.),(1.,1.),(1.,1.),(1.,1.),(1.,1.),(1.,1.),(1.,1.),(1.,1.),(1.,
1.),(1.,1.),(1.,1.),(1.,1.),(1.,1.),(1.,1.),(1.,1.),(1.,1.),(1.,1.),(1.,
1.),(1.,1.),(1.,1.),(1.,1.),(1.,1.),(1.,1.),(1.,1.),(1.,1.),(1.,1.),(1.,
1.),(1.,1.),(1.,1.),(1.,1.),(1.,1.),(1.,1.),(1.,1.),(1.,1.),(1.,1.),(1.,
1.),(1.,1.),(1.,1.),(1.,1.),(1.,1.),(1.,1.),(1.,1.),(1.,1.),(1.,1.),(1.,
1.),(1.,1.),(1.,1.),(1.,1.),(1.,1.),(1.,1.),(1.,1.),(1.,1.),(1.,1.),(1.,
1.),(1.,1.),(1.,1.),(1.,1.),(1.,1.),(1.,1.),(1.,1.),(1.,1.),(1.,1.),(1.,
1.),(1.,1.),(1.,1.),(1.,1.),(1.,1.),(1.,1.),(1.,1.),(1.,1.),(1.,1.),(1.,
1.),(1.,1.),(1.,1.),(1.,1.),(1.,1.),(1.,1.),(1.,1.),(1.,1.),(1.,1.),(1.,
1.),(1.,1.),(1.,1.),(1.,1.),(1.,1.),(1.,1.),(1.,1.),(1.,1.),(1.,1.),(1.,
1.),(1.,1.),(1.,1.),(1.,1.),(1.,1.),(1.,1.),(1.,1.),(1.,1.),(1.,1.),(1.,
1.),(1.,1.),(1.,1.),(1.,1.),(1.,1.),(1.,1.),(1.,1.),(1.,1.),(1.,1.),(1.,
1.),(1.,1.),(1.,1.),(1.,1.),(1.,1.),(1.,1.),(1.,1.),(1.,1.),(1.,1.),(1.,
1.),(1.,1.),(1.,1.),(1.,1.),(1.,1.),(1.,1.),(1.,1.),(1.,1.),(1.,1.),(1.,
1.),(1.,1.),(1.,1.),(1.,1.),(1.,1.),(1.,1.),(1.,1.),(1.,1.),(1.,1.),(1.,
1.),(1.,1.),(1.,1.),(1.,1.),(1.,1.),(1.,1.),(1.,1.),(1.,1.),(1.,1.),(1.,
1.),(1.,1.),(1.,1.),(1.,1.),(1.,1.),(1.,1.),(1.,1.),(1.,1.),(1.,1.),(1.,
1.),(1.,1.),(1.,1.),(1.,1.),(1.,1.),(1.,1.),(1.,1.),(1.,1.),(1.,1.),(1.,
1.),(1.,1.),(1.,1.),(1.,1.),(1.,1.),(1.,1.),(1.,1.),(1.,1.),(1.,1.),(1.,
1.),(1.,1.),(1.,1.),(1.,1.),(1.,1.),(1.,1.),(1.,1.),(1.,1.),(1.,1.),(1.,
1.),(1.,1.),(1.,1.),(1.,1.),(1.,1.),(1.,1.),(1.,1.),(1.,1.),(1.,1.),(1.,
1.),(1.,1.),(1.,1.),(1.,1.),(1.,1.),(1.,1.),(1.,1.),(1.,1.),(1.,1.),(1.,
1.),(1.,1.),(1.,1.),(1.,1.),(1.,1.),(1.,1.),(1.,1.),(1.,1.),(1.,1.),(1.,
1.),(1.,1.),(1.,1.),(1.,1.),(1.,1.),(1.,1.),(1.,1.),(1.,1.),(1.,1.),(1.,
1.),(1.,1.),(1.,1.),(1.,1.),(1.,1.),(1.,1.),(1.,1.),(1.,1.),(1.,1.),(1.,
1.),(1.,1.),(1.,1.),(1.,1.),(1.,1.),(1.,1.),(1.,1.),(1.,1.),(1.,1.),(1.,
1.),(1.,1.),(1.,1.),(1.,1.),(1.,1.),(1.,1.),(1.,1.),(1.,1.),(1.,1.),(1.,
1.),(1.,1.),(1.,1.),(1.,1.),(1.,1.),(1.,1.),(1.,1.),(1.,1.),(1.,1.),(1.,
1.),(1.,1.),(1.,1.),(1.,1.),(1.,1.),(1.,1.),(1.,1.),(1.,1.),(1.,1.),(1.,
1.),(1.,1.),(1.,1.),(1.,1.),(1.,1.),(1.,1.),(1.,1.),(1.,1.),(1.,1.),(1.,
1.),(1.,1.),(1.,1.),(1.,1.),(1.,1.),(1.,1.),(1.,1.),(1.,1.),(1.,1.),(1.,
1.),(1.,1.),(1.,1.),(1.,1.),(1.,1.),(1.,1.),(1.,1.),(1.,1.),(1.,1.),(1.,
1.),(1.,1.),(1.,1.),(1.,1.),(1.,1.),(1.,1.),(1.,1.),(1.,1.),(1.,1.),(1.,
1.),(1.,1.),(1.,1.),(1.,1.),(1.,1.),(1.,1.),(1.,1.),(1.,1.),(1.,1.),(1.,
1.),(1.,1.),(1.,1.),(1.,1.),(1.,1.),(1.,1.),(1.,1.),(1.,1.),(1.,1.),(1.,
1.),(1.,1.),(1.,1.),(1.,1.),(1.,1.),(1.,1.),(1.,1.),(1.,1.),(1.,1.),(1.,
1.),(1.,1.),(1.,1.),(1.,1.),(1.,1.),(1.,1.),(1.,1.),(1.,1.),(1.,1.),(1.,
1.),(1.,1.),(1.,1.),(1.,1.),(1.,1.),(1.,1.),(1.,1.),(1.,1.),(1.,1.),(1.,
1.),(1.,1.),(1.,1.),(1.,1.),(1.,1.),(1.,1.),(1.,1.),(1.,1.),(1.,1.),(1.,
1.),(1.,1.),(1.,1.),(1.,1.),(1.,1.),(1.,1.),(1.,1.),(1.,1.),(1.,1.),(1.,
1.),(1.,1.),(1.,1.),(1.,1.),(1.,1.),(1.,1.),(1.,1.),(1.,1.),(1.,1.),(1.,
1.),(1.,1.),(1.,1.),(1.,1.),(1.,1.),(1.,1.),(1.,1.),(1.,1.),(1.,1.),(1.,
1.),(1.,1.),(1.,1.),(1.,1.),(1.,1.),(1.,1.),(1.,1.),(1.,1.),(1.,1.),(1.,
1.),(1.,1.),(1.,1.),(1.,1.),(1.,1.),(1.,1.),(1.,1.),(1.,1.),(1.,1.),(1.,
1.),(1.,1.),(1.,1.),(1.,1.),(1.,1.),(1.,1.),(1.,1.),(1.,1.),(1.,1.),(1.,
1.),(1.,1.),(1.,1.),(1.,1.),(1.,1.),(1.,1.),(1.,1.),(1.,1.),(1.,1.),(1.,
1.),(1.,1.),(1.,1.),(1.,1.),(1.,1.),(1.,1.),(1.,1.),(1.,1.),(1.,1.),(1.,
1.),(1.,1.),(1.,1.),(1.,1.),(1.,1.),(1.,1.),(1.,1.),(1.,1.),(1.,1.),(1.,
1.),(1.,1.),(1.,1.),(1.,1.),(1.,1.),(1.,1.),(1.,1.),(1.,1.),(1.,1.),(1.,
1.),(1.,1.),(1.,1.),(1.,1.),(1.,1.),(1.,1.),(1.,1.),(1.,1.),(1.,1.),(1.,
1.),(1.,1.),(1.,1.),(1.,1.),(1.,1.),(1.,1.),(1.,1.),(1.,1.),(1.,1.),(1.,
1.),(1.,1.),(1.,1.),(1.,1.),(1.,1.),(1.,1.),(1.,1.),(1.,1.),(1.,1.),(1.,
1.),(1.,1.),(1.,1.),(1.,1.),(1.,1.),(1.,1.),(1.,1.),(1.,1.),(1.,1.),(1.,
1.),(1.,1.),(1.,1.),(1.,1.),(1.,1.),(1.,1.),(1.,1.),(1.,1.),(1.,1.),(1.,
1.),(1.,1.),(1.,1.),(1.,1.),(1.,1.),(1.,1.),(1.,1.),(1.,1.),(1.,1.),(1.,
1.),(1.,1.),(1.,1.),(1.,1.),(1.,1.),(1.,1.),(1.,1.),(1.,1.),(1.,1.),(1.,
1.),(1.,1.),(1.,1.),(1.,1.),(1.,1.),(1.,1.),(1.,1.),(1.,1.),(1.,1.),(1.,
1.),(1.,1.),(1.,1.),(1.,1.),(1.,1.),(1.,1.),(1.,1.),(1.,1.),(1.,1.),(1.,
1.),(1.,1.),(1.,1.),(1.,1.),(1.,1.),(1.,1.),(1.,1.),(1.,1.),(1.,1.),(1.,
1.),(1.,1.),(1.,1.),(1.,1.),(1.,1.),(1.,1.),(1.,1.),(1.,1.),(1.,1.),(1.,
1.),(1.,1.),(1.,1.),(1.,1.),(1.,1.),(1.,1.),(1.,1.),(1.,1.),(1.,1.),(1.,
1.),(1.,1.),(1.,1.),(1.,1.),(1.,1.),(1.,1.),(1.,1.),(1.,1.),(1.,1.),(1.,
1.),(1.,1.),(1.,1.),(1.,1.),(1.,1.),(1.,1.),(1.,1.),(1.,1.),(1.,1.),(1.,
1.),(1.,1.),(1.,1.),(1.,1.),(1.,1.),(1.,1.),(1.,1.),(1.,1.),(1.,1.),(1.,
1.),(1.,1.),(1.,1.),(1.,1.),(1.,1.),(1.,1.),(1.,1.),(1.,1.),(1.,1.),(1.,
1.),(1.,1.),(1.,1.),(1.,1.),(1.,1.),(1.,1.),(1.,1.),(1.,1.),(1.,1.),(1.,
1.),(1.,1.),(1.,1.),(1.,1.),(1.,1.),(1.,1.),(1.,1.),(1.,1.),(1.,1.),(1.,
1.),(1.,1.),(1.,1.),(1.,1.),(1.,1.),(1.,1.),(1.,1.),(1.,1.),(1.,1.),(1.,
1.),(1.,1.),(1.,1.),(1.,1.),(1.,1.),(1.,1.),(1.,1.),(1.,1.),(1.,1.),(1.,
1.),(1.,1.),(1.,1.),(1.,1.),(1.,1.),(1.,1.),(1.,1.),(1.,1.),(1.,1.),(1.,
1.),(1.,1.),(1.,1.),(1.,1.),(1.,1.),(1.,1.),(1.,1.),(1.,1.),(1.,1.),(1.,
1.),(1.,1.),(1.,1.),(1.,1.),(1.,1.),(1.,1.),(1.,1.),(1.,1.),(1.,1.),(1.,
1.),(1.,1.),(1.,1.),(1.,1.),(1.,1.),(1.,1.),(1.,1.),(1.,1.),(1.,1.),(1.,
1.),(1.,1.),(1.,1.),(1.,1.),(1.,1.),(1.,1.),(1.,1.),(1.,1.),(1.,1.),(1.,
1.),(1.,1.),(1.,1.),(1.,1.),(1.,1.),(1.,1.),(1.,1.),(1.,1.),(1.,1.),(1.,
1.),(1.,1.),(1.,1.),(1.,1.),(1.,1.),(1.,1.),(1.,1.),(1.,1.),(1.,1.),(1.,
1.),(1.,1.),(1.,1.),(1.,1.),(1.,1.),(1.,1.),(1.,1.),(1.,1.),(1.,1.),(1.,
1.),(1.,1.),(1.,1.),(1.,1.),(1.,1.),(1.,1.),(1.,1.),(1.,1.),(1.,1.),(1.,
1.),(1.,1.),(1.,1.),(1.,1.),(1.,1.),(1.,1.),(1.,1.),(1.,1.),(1.,1.),(1.,
1.),(1.,1.),(1.,1.),(1.,1.),(1.,1.),(1.,1.),(1.,1.),(1.,1.),(1.,1.),(1.,
1.),(1.,1.),(1.,1.),(1.,1.),(1.,1.),(1.,1.),(1.,1.),(1.,1.),(1.,1.),(1.,
1.),(1.,1.),(1.,1.),(1.,1.),(1.,1.),(1.,1.),(1.,1.),(1.,1.),(1.,1.),(1.,
1.),(1.,1.),(1.,1.),(1.,1.),(1.,1.),(1.,1.),(1.,1.),(1.,1.),(1.,1.),(1.,
1.),(1.,1.),(1.,1.),(1.,1.),(1.,1.),(1.,1.),(1.,1.),(1.,1.),(1.,1.),(1.,
1.),(1.,1.),(1.,1.),(1.,1.),(1.,1.),(1.,1.),(1.,1.),(1.,1.),(1.,1.),(1.,
1.),(1.,1.),(1.,1.),(1.,1.),(1.,1.),(1.,1.),(1.,1.),(1.,1.),(1.,1.),(1.,
1.),(1.,1.),(1.,1.),(1.,1.),(1.,1.),(1.,1.),(1.,1.),(1.,1.),(1.,1.),(1.,
1.),(1.,1.),(1.,1.),(1.,1.),(1.,1.),(1.,1.),(1.,1.),(1.,1.),(1.,1.),(1.,
1.),(1.,1.),(1.,1.),(1.,1.),(1.,1.),(1.,1.),(1.,1.),(1.,1.),(1.,1.),(1.,
1.),(1.,1.),(1.,1.),(1.,1.),(1.,1.),(1.,1.),(1.,1.),(1.,1.),(1.,1.),(1.,
1.)))
REPRESENTATION_ITEM('')
SURFACE()
);
#258=(
BOUNDED_SURFACE()
B_SPLINE_SURFACE(5,1,((#74101,#74102),(#74103,#74104),(#74105,#74106),(#74107,
#74108),(#74109,#74110),(#74111,#74112),(#74113,#74114),(#74115,#74116),
(#74117,#74118),(#74119,#74120),(#74121,#74122),(#74123,#74124),(#74125,
#74126),(#74127,#74128),(#74129,#74130),(#74131,#74132),(#74133,#74134),
(#74135,#74136),(#74137,#74138),(#74139,#74140),(#74141,#74142),(#74143,
#74144),(#74145,#74146),(#74147,#74148),(#74149,#74150),(#74151,#74152),
(#74153,#74154),(#74155,#74156),(#74157,#74158),(#74159,#74160),(#74161,
#74162),(#74163,#74164),(#74165,#74166),(#74167,#74168),(#74169,#74170),
(#74171,#74172),(#74173,#74174),(#74175,#74176),(#74177,#74178),(#74179,
#74180),(#74181,#74182),(#74183,#74184),(#74185,#74186),(#74187,#74188),
(#74189,#74190),(#74191,#74192),(#74193,#74194),(#74195,#74196),(#74197,
#74198),(#74199,#74200),(#74201,#74202),(#74203,#74204),(#74205,#74206),
(#74207,#74208),(#74209,#74210),(#74211,#74212),(#74213,#74214),(#74215,
#74216),(#74217,#74218),(#74219,#74220),(#74221,#74222),(#74223,#74224),
(#74225,#74226),(#74227,#74228),(#74229,#74230),(#74231,#74232),(#74233,
#74234),(#74235,#74236),(#74237,#74238),(#74239,#74240),(#74241,#74242),
(#74243,#74244),(#74245,#74246),(#74247,#74248),(#74249,#74250),(#74251,
#74252),(#74253,#74254),(#74255,#74256),(#74257,#74258),(#74259,#74260),
(#74261,#74262),(#74263,#74264),(#74265,#74266),(#74267,#74268),(#74269,
#74270),(#74271,#74272),(#74273,#74274),(#74275,#74276),(#74277,#74278),
(#74279,#74280),(#74281,#74282),(#74283,#74284),(#74285,#74286),(#74287,
#74288),(#74289,#74290),(#74291,#74292),(#74293,#74294),(#74295,#74296),
(#74297,#74298),(#74299,#74300),(#74301,#74302),(#74303,#74304),(#74305,
#74306),(#74307,#74308),(#74309,#74310),(#74311,#74312),(#74313,#74314),
(#74315,#74316),(#74317,#74318),(#74319,#74320),(#74321,#74322),(#74323,
#74324),(#74325,#74326),(#74327,#74328),(#74329,#74330),(#74331,#74332),
(#74333,#74334),(#74335,#74336),(#74337,#74338),(#74339,#74340),(#74341,
#74342),(#74343,#74344),(#74345,#74346),(#74347,#74348),(#74349,#74350),
(#74351,#74352),(#74353,#74354),(#74355,#74356),(#74357,#74358),(#74359,
#74360),(#74361,#74362),(#74363,#74364),(#74365,#74366),(#74367,#74368),
(#74369,#74370),(#74371,#74372),(#74373,#74374),(#74375,#74376),(#74377,
#74378),(#74379,#74380),(#74381,#74382),(#74383,#74384),(#74385,#74386),
(#74387,#74388),(#74389,#74390),(#74391,#74392),(#74393,#74394),(#74395,
#74396),(#74397,#74398),(#74399,#74400),(#74401,#74402),(#74403,#74404),
(#74405,#74406),(#74407,#74408),(#74409,#74410),(#74411,#74412),(#74413,
#74414),(#74415,#74416),(#74417,#74418),(#74419,#74420),(#74421,#74422),
(#74423,#74424),(#74425,#74426),(#74427,#74428),(#74429,#74430),(#74431,
#74432),(#74433,#74434),(#74435,#74436),(#74437,#74438),(#74439,#74440),
(#74441,#74442),(#74443,#74444),(#74445,#74446),(#74447,#74448),(#74449,
#74450),(#74451,#74452),(#74453,#74454),(#74455,#74456),(#74457,#74458),
(#74459,#74460),(#74461,#74462),(#74463,#74464),(#74465,#74466),(#74467,
#74468),(#74469,#74470),(#74471,#74472),(#74473,#74474),(#74475,#74476),
(#74477,#74478),(#74479,#74480),(#74481,#74482),(#74483,#74484),(#74485,
#74486),(#74487,#74488),(#74489,#74490),(#74491,#74492),(#74493,#74494),
(#74495,#74496),(#74497,#74498),(#74499,#74500),(#74501,#74502),(#74503,
#74504),(#74505,#74506),(#74507,#74508),(#74509,#74510),(#74511,#74512),
(#74513,#74514),(#74515,#74516),(#74517,#74518),(#74519,#74520),(#74521,
#74522),(#74523,#74524),(#74525,#74526),(#74527,#74528),(#74529,#74530),
(#74531,#74532),(#74533,#74534),(#74535,#74536),(#74537,#74538),(#74539,
#74540),(#74541,#74542),(#74543,#74544),(#74545,#74546),(#74547,#74548),
(#74549,#74550),(#74551,#74552),(#74553,#74554),(#74555,#74556),(#74557,
#74558),(#74559,#74560),(#74561,#74562),(#74563,#74564),(#74565,#74566),
(#74567,#74568),(#74569,#74570),(#74571,#74572),(#74573,#74574),(#74575,
#74576),(#74577,#74578),(#74579,#74580),(#74581,#74582),(#74583,#74584),
(#74585,#74586),(#74587,#74588),(#74589,#74590),(#74591,#74592),(#74593,
#74594),(#74595,#74596),(#74597,#74598),(#74599,#74600),(#74601,#74602),
(#74603,#74604),(#74605,#74606),(#74607,#74608),(#74609,#74610),(#74611,
#74612),(#74613,#74614),(#74615,#74616),(#74617,#74618),(#74619,#74620),
(#74621,#74622),(#74623,#74624),(#74625,#74626),(#74627,#74628),(#74629,
#74630),(#74631,#74632),(#74633,#74634),(#74635,#74636),(#74637,#74638),
(#74639,#74640),(#74641,#74642),(#74643,#74644),(#74645,#74646),(#74647,
#74648),(#74649,#74650),(#74651,#74652),(#74653,#74654),(#74655,#74656),
(#74657,#74658),(#74659,#74660),(#74661,#74662),(#74663,#74664),(#74665,
#74666),(#74667,#74668),(#74669,#74670),(#74671,#74672),(#74673,#74674),
(#74675,#74676),(#74677,#74678),(#74679,#74680),(#74681,#74682),(#74683,
#74684),(#74685,#74686),(#74687,#74688),(#74689,#74690),(#74691,#74692),
(#74693,#74694),(#74695,#74696),(#74697,#74698),(#74699,#74700),(#74701,
#74702),(#74703,#74704),(#74705,#74706),(#74707,#74708),(#74709,#74710),
(#74711,#74712),(#74713,#74714),(#74715,#74716),(#74717,#74718),(#74719,
#74720),(#74721,#74722),(#74723,#74724),(#74725,#74726),(#74727,#74728),
(#74729,#74730),(#74731,#74732),(#74733,#74734),(#74735,#74736),(#74737,
#74738),(#74739,#74740),(#74741,#74742),(#74743,#74744),(#74745,#74746),
(#74747,#74748),(#74749,#74750),(#74751,#74752),(#74753,#74754),(#74755,
#74756),(#74757,#74758),(#74759,#74760),(#74761,#74762),(#74763,#74764),
(#74765,#74766),(#74767,#74768),(#74769,#74770),(#74771,#74772),(#74773,
#74774),(#74775,#74776),(#74777,#74778),(#74779,#74780),(#74781,#74782),
(#74783,#74784),(#74785,#74786),(#74787,#74788),(#74789,#74790),(#74791,
#74792),(#74793,#74794),(#74795,#74796),(#74797,#74798),(#74799,#74800),
(#74801,#74802),(#74803,#74804),(#74805,#74806),(#74807,#74808),(#74809,
#74810),(#74811,#74812),(#74813,#74814),(#74815,#74816),(#74817,#74818),
(#74819,#74820),(#74821,#74822),(#74823,#74824),(#74825,#74826),(#74827,
#74828),(#74829,#74830),(#74831,#74832),(#74833,#74834),(#74835,#74836),
(#74837,#74838),(#74839,#74840),(#74841,#74842),(#74843,#74844),(#74845,
#74846),(#74847,#74848),(#74849,#74850),(#74851,#74852),(#74853,#74854),
(#74855,#74856),(#74857,#74858),(#74859,#74860),(#74861,#74862),(#74863,
#74864),(#74865,#74866),(#74867,#74868),(#74869,#74870),(#74871,#74872),
(#74873,#74874),(#74875,#74876),(#74877,#74878),(#74879,#74880),(#74881,
#74882),(#74883,#74884),(#74885,#74886),(#74887,#74888),(#74889,#74890),
(#74891,#74892),(#74893,#74894),(#74895,#74896),(#74897,#74898),(#74899,
#74900),(#74901,#74902),(#74903,#74904),(#74905,#74906),(#74907,#74908),
(#74909,#74910),(#74911,#74912),(#74913,#74914),(#74915,#74916),(#74917,
#74918),(#74919,#74920),(#74921,#74922),(#74923,#74924),(#74925,#74926),
(#74927,#74928),(#74929,#74930),(#74931,#74932),(#74933,#74934),(#74935,
#74936),(#74937,#74938),(#74939,#74940),(#74941,#74942),(#74943,#74944),
(#74945,#74946),(#74947,#74948),(#74949,#74950),(#74951,#74952),(#74953,
#74954),(#74955,#74956),(#74957,#74958),(#74959,#74960),(#74961,#74962),
(#74963,#74964),(#74965,#74966),(#74967,#74968),(#74969,#74970),(#74971,
#74972),(#74973,#74974),(#74975,#74976),(#74977,#74978),(#74979,#74980),
(#74981,#74982),(#74983,#74984),(#74985,#74986),(#74987,#74988),(#74989,
#74990),(#74991,#74992),(#74993,#74994),(#74995,#74996),(#74997,#74998),
(#74999,#75000),(#75001,#75002),(#75003,#75004),(#75005,#75006),(#75007,
#75008),(#75009,#75010),(#75011,#75012),(#75013,#75014),(#75015,#75016),
(#75017,#75018),(#75019,#75020),(#75021,#75022),(#75023,#75024),(#75025,
#75026),(#75027,#75028),(#75029,#75030),(#75031,#75032),(#75033,#75034),
(#75035,#75036),(#75037,#75038),(#75039,#75040),(#75041,#75042),(#75043,
#75044),(#75045,#75046),(#75047,#75048),(#75049,#75050),(#75051,#75052),
(#75053,#75054),(#75055,#75056),(#75057,#75058),(#75059,#75060),(#75061,
#75062),(#75063,#75064),(#75065,#75066),(#75067,#75068),(#75069,#75070),
(#75071,#75072),(#75073,#75074),(#75075,#75076),(#75077,#75078),(#75079,
#75080),(#75081,#75082),(#75083,#75084),(#75085,#75086),(#75087,#75088),
(#75089,#75090),(#75091,#75092),(#75093,#75094),(#75095,#75096),(#75097,
#75098),(#75099,#75100),(#75101,#75102),(#75103,#75104),(#75105,#75106),
(#75107,#75108),(#75109,#75110),(#75111,#75112),(#75113,#75114),(#75115,
#75116),(#75117,#75118),(#75119,#75120),(#75121,#75122),(#75123,#75124),
(#75125,#75126),(#75127,#75128),(#75129,#75130),(#75131,#75132),(#75133,
#75134),(#75135,#75136),(#75137,#75138),(#75139,#75140),(#75141,#75142),
(#75143,#75144),(#75145,#75146),(#75147,#75148),(#75149,#75150),(#75151,
#75152),(#75153,#75154),(#75155,#75156),(#75157,#75158),(#75159,#75160),
(#75161,#75162),(#75163,#75164),(#75165,#75166),(#75167,#75168),(#75169,
#75170),(#75171,#75172),(#75173,#75174),(#75175,#75176),(#75177,#75178),
(#75179,#75180),(#75181,#75182),(#75183,#75184),(#75185,#75186),(#75187,
#75188),(#75189,#75190),(#75191,#75192),(#75193,#75194),(#75195,#75196),
(#75197,#75198),(#75199,#75200),(#75201,#75202),(#75203,#75204),(#75205,
#75206),(#75207,#75208),(#75209,#75210),(#75211,#75212),(#75213,#75214),
(#75215,#75216),(#75217,#75218),(#75219,#75220),(#75221,#75222),(#75223,
#75224),(#75225,#75226),(#75227,#75228),(#75229,#75230),(#75231,#75232),
(#75233,#75234),(#75235,#75236),(#75237,#75238),(#75239,#75240),(#75241,
#75242),(#75243,#75244),(#75245,#75246),(#75247,#75248),(#75249,#75250),
(#75251,#75252),(#75253,#75254),(#75255,#75256),(#75257,#75258),(#75259,
#75260),(#75261,#75262),(#75263,#75264),(#75265,#75266),(#75267,#75268),
(#75269,#75270),(#75271,#75272),(#75273,#75274),(#75275,#75276),(#75277,
#75278),(#75279,#75280),(#75281,#75282),(#75283,#75284),(#75285,#75286),
(#75287,#75288),(#75289,#75290),(#75291,#75292),(#75293,#75294),(#75295,
#75296),(#75297,#75298),(#75299,#75300),(#75301,#75302),(#75303,#75304),
(#75305,#75306),(#75307,#75308),(#75309,#75310),(#75311,#75312),(#75313,
#75314),(#75315,#75316),(#75317,#75318),(#75319,#75320),(#75321,#75322),
(#75323,#75324),(#75325,#75326),(#75327,#75328),(#75329,#75330),(#75331,
#75332),(#75333,#75334),(#75335,#75336),(#75337,#75338),(#75339,#75340),
(#75341,#75342),(#75343,#75344),(#75345,#75346),(#75347,#75348),(#75349,
#75350),(#75351,#75352),(#75353,#75354),(#75355,#75356),(#75357,#75358),
(#75359,#75360),(#75361,#75362),(#75363,#75364),(#75365,#75366),(#75367,
#75368),(#75369,#75370),(#75371,#75372),(#75373,#75374),(#75375,#75376),
(#75377,#75378),(#75379,#75380),(#75381,#75382),(#75383,#75384),(#75385,
#75386),(#75387,#75388),(#75389,#75390),(#75391,#75392),(#75393,#75394),
(#75395,#75396),(#75397,#75398),(#75399,#75400),(#75401,#75402),(#75403,
#75404),(#75405,#75406),(#75407,#75408),(#75409,#75410),(#75411,#75412),
(#75413,#75414),(#75415,#75416),(#75417,#75418),(#75419,#75420),(#75421,
#75422),(#75423,#75424),(#75425,#75426),(#75427,#75428),(#75429,#75430),
(#75431,#75432),(#75433,#75434),(#75435,#75436),(#75437,#75438),(#75439,
#75440),(#75441,#75442),(#75443,#75444),(#75445,#75446),(#75447,#75448),
(#75449,#75450),(#75451,#75452),(#75453,#75454),(#75455,#75456),(#75457,
#75458),(#75459,#75460),(#75461,#75462),(#75463,#75464),(#75465,#75466),
(#75467,#75468),(#75469,#75470),(#75471,#75472),(#75473,#75474),(#75475,
#75476),(#75477,#75478),(#75479,#75480),(#75481,#75482),(#75483,#75484),
(#75485,#75486),(#75487,#75488),(#75489,#75490),(#75491,#75492),(#75493,
#75494),(#75495,#75496),(#75497,#75498),(#75499,#75500),(#75501,#75502),
(#75503,#75504),(#75505,#75506),(#75507,#75508),(#75509,#75510),(#75511,
#75512),(#75513,#75514),(#75515,#75516),(#75517,#75518),(#75519,#75520),
(#75521,#75522),(#75523,#75524),(#75525,#75526),(#75527,#75528),(#75529,
#75530),(#75531,#75532),(#75533,#75534),(#75535,#75536),(#75537,#75538),
(#75539,#75540),(#75541,#75542),(#75543,#75544),(#75545,#75546),(#75547,
#75548),(#75549,#75550),(#75551,#75552),(#75553,#75554),(#75555,#75556),
(#75557,#75558),(#75559,#75560),(#75561,#75562),(#75563,#75564),(#75565,
#75566),(#75567,#75568),(#75569,#75570),(#75571,#75572),(#75573,#75574),
(#75575,#75576),(#75577,#75578),(#75579,#75580),(#75581,#75582),(#75583,
#75584),(#75585,#75586),(#75587,#75588),(#75589,#75590),(#75591,#75592),
(#75593,#75594),(#75595,#75596),(#75597,#75598),(#75599,#75600),(#75601,
#75602),(#75603,#75604),(#75605,#75606),(#75607,#75608),(#75609,#75610),
(#75611,#75612),(#75613,#75614),(#75615,#75616),(#75617,#75618),(#75619,
#75620),(#75621,#75622),(#75623,#75624),(#75625,#75626),(#75627,#75628),
(#75629,#75630),(#75631,#75632),(#75633,#75634),(#75635,#75636),(#75637,
#75638),(#75639,#75640),(#75641,#75642),(#75643,#75644),(#75645,#75646),
(#75647,#75648),(#75649,#75650),(#75651,#75652),(#75653,#75654),(#75655,
#75656),(#75657,#75658),(#75659,#75660),(#75661,#75662),(#75663,#75664),
(#75665,#75666),(#75667,#75668),(#75669,#75670),(#75671,#75672),(#75673,
#75674),(#75675,#75676),(#75677,#75678),(#75679,#75680),(#75681,#75682),
(#75683,#75684),(#75685,#75686),(#75687,#75688),(#75689,#75690),(#75691,
#75692),(#75693,#75694),(#75695,#75696),(#75697,#75698),(#75699,#75700),
(#75701,#75702),(#75703,#75704),(#75705,#75706),(#75707,#75708),(#75709,
#75710),(#75711,#75712),(#75713,#75714),(#75715,#75716),(#75717,#75718),
(#75719,#75720),(#75721,#75722),(#75723,#75724),(#75725,#75726),(#75727,
#75728),(#75729,#75730),(#75731,#75732),(#75733,#75734),(#75735,#75736),
(#75737,#75738),(#75739,#75740),(#75741,#75742),(#75743,#75744),(#75745,
#75746),(#75747,#75748),(#75749,#75750),(#75751,#75752),(#75753,#75754),
(#75755,#75756),(#75757,#75758),(#75759,#75760),(#75761,#75762),(#75763,
#75764),(#75765,#75766),(#75767,#75768),(#75769,#75770),(#75771,#75772),
(#75773,#75774),(#75775,#75776),(#75777,#75778),(#75779,#75780),(#75781,
#75782),(#75783,#75784),(#75785,#75786),(#75787,#75788),(#75789,#75790),
(#75791,#75792),(#75793,#75794),(#75795,#75796),(#75797,#75798),(#75799,
#75800),(#75801,#75802),(#75803,#75804),(#75805,#75806),(#75807,#75808),
(#75809,#75810),(#75811,#75812),(#75813,#75814),(#75815,#75816),(#75817,
#75818),(#75819,#75820),(#75821,#75822),(#75823,#75824),(#75825,#75826),
(#75827,#75828),(#75829,#75830),(#75831,#75832),(#75833,#75834),(#75835,
#75836),(#75837,#75838),(#75839,#75840),(#75841,#75842),(#75843,#75844),
(#75845,#75846),(#75847,#75848),(#75849,#75850),(#75851,#75852),(#75853,
#75854),(#75855,#75856),(#75857,#75858),(#75859,#75860),(#75861,#75862),
(#75863,#75864),(#75865,#75866),(#75867,#75868),(#75869,#75870),(#75871,
#75872),(#75873,#75874),(#75875,#75876),(#75877,#75878),(#75879,#75880),
(#75881,#75882),(#75883,#75884),(#75885,#75886),(#75887,#75888),(#75889,
#75890),(#75891,#75892),(#75893,#75894),(#75895,#75896),(#75897,#75898),
(#75899,#75900),(#75901,#75902),(#75903,#75904),(#75905,#75906),(#75907,
#75908),(#75909,#75910),(#75911,#75912),(#75913,#75914),(#75915,#75916),
(#75917,#75918),(#75919,#75920),(#75921,#75922),(#75923,#75924),(#75925,
#75926),(#75927,#75928),(#75929,#75930),(#75931,#75932),(#75933,#75934),
(#75935,#75936),(#75937,#75938),(#75939,#75940),(#75941,#75942),(#75943,
#75944),(#75945,#75946),(#75947,#75948),(#75949,#75950),(#75951,#75952),
(#75953,#75954),(#75955,#75956),(#75957,#75958),(#75959,#75960),(#75961,
#75962),(#75963,#75964),(#75965,#75966),(#75967,#75968),(#75969,#75970),
(#75971,#75972),(#75973,#75974),(#75975,#75976),(#75977,#75978),(#75979,
#75980),(#75981,#75982),(#75983,#75984),(#75985,#75986),(#75987,#75988),
(#75989,#75990),(#75991,#75992),(#75993,#75994),(#75995,#75996),(#75997,
#75998),(#75999,#76000),(#76001,#76002),(#76003,#76004),(#76005,#76006),
(#76007,#76008),(#76009,#76010),(#76011,#76012),(#76013,#76014),(#76015,
#76016),(#76017,#76018),(#76019,#76020),(#76021,#76022),(#76023,#76024),
(#76025,#76026),(#76027,#76028),(#76029,#76030),(#76031,#76032),(#76033,
#76034),(#76035,#76036),(#76037,#76038),(#76039,#76040),(#76041,#76042),
(#76043,#76044),(#76045,#76046),(#76047,#76048),(#76049,#76050),(#76051,
#76052),(#76053,#76054),(#76055,#76056),(#76057,#76058),(#76059,#76060),
(#76061,#76062),(#76063,#76064),(#76065,#76066),(#76067,#76068),(#76069,
#76070),(#76071,#76072),(#76073,#76074),(#76075,#76076),(#76077,#76078),
(#76079,#76080),(#76081,#76082),(#76083,#76084),(#76085,#76086),(#76087,
#76088),(#76089,#76090),(#76091,#76092),(#76093,#76094),(#76095,#76096),
(#76097,#76098),(#76099,#76100),(#76101,#76102),(#76103,#76104),(#76105,
#76106),(#76107,#76108),(#76109,#76110)),.UNSPECIFIED.,.F.,.F.,.F.)
B_SPLINE_SURFACE_WITH_KNOTS((6,1,1,1,1,1,1,1,1,1,1,1,1,1,1,1,1,1,1,1,1,
1,1,1,1,1,1,1,1,1,1,1,1,1,1,1,1,1,1,1,1,1,1,1,1,1,1,1,1,1,1,1,1,1,1,1,1,
1,1,1,1,1,1,1,1,1,1,1,1,1,1,1,1,1,1,1,1,1,1,1,1,1,1,1,1,1,1,1,1,1,1,1,1,
1,1,1,1,1,1,1,1,1,1,1,1,1,1,1,1,1,1,1,1,1,1,1,1,1,1,1,1,1,1,1,1,1,1,1,1,
1,1,1,1,1,1,1,1,1,1,1,1,1,1,1,1,1,1,1,1,1,1,1,1,1,1,1,1,1,1,1,1,1,1,1,1,
1,1,1,1,1,1,1,1,1,1,1,1,1,1,1,1,1,1,1,1,1,1,1,1,1,1,1,1,1,1,1,1,1,1,1,1,
1,1,1,1,1,1,1,1,1,1,1,1,1,1,1,1,1,1,1,1,1,1,1,1,1,1,1,1,1,1,1,1,1,1,1,1,
1,1,1,1,1,1,1,1,1,1,1,1,1,1,1,1,1,1,1,1,1,1,1,1,1,1,1,1,1,1,1,1,1,1,1,1,
1,1,1,1,1,1,1,1,1,1,1,1,1,1,1,1,1,1,1,1,1,1,1,1,1,1,1,1,1,1,1,1,1,1,1,1,
1,1,1,1,1,1,1,1,1,1,1,1,1,1,1,1,1,1,1,1,1,1,1,1,1,1,1,1,1,1,1,1,1,1,1,1,
1,1,1,1,1,1,1,1,1,1,1,1,1,1,1,1,1,1,1,1,1,1,1,1,1,1,1,1,1,1,1,1,1,1,1,1,
1,1,1,1,1,1,1,1,1,1,1,1,1,1,1,1,1,1,1,1,1,1,1,1,1,1,1,1,1,1,1,1,1,1,1,1,
1,1,1,1,1,1,1,1,1,1,1,1,1,1,1,1,1,1,1,1,1,1,1,1,1,1,1,1,1,1,1,1,1,1,1,1,
1,1,1,1,1,1,1,1,1,1,1,1,1,1,1,1,1,1,1,1,1,1,1,1,1,1,1,1,1,1,1,1,1,1,1,1,
1,1,1,1,1,1,1,1,1,1,1,1,1,1,1,1,1,1,1,1,1,1,1,1,1,1,1,1,1,1,1,1,1,1,1,1,
1,1,1,1,1,1,1,1,1,1,1,1,1,1,1,1,1,1,1,1,1,1,1,1,1,1,1,1,1,1,1,1,1,1,1,1,
1,1,1,1,1,1,1,1,1,1,1,1,1,1,1,1,1,1,1,1,1,1,1,1,1,1,1,1,1,1,1,1,1,1,1,1,
1,1,1,1,1,1,1,1,1,1,1,1,1,1,1,1,1,1,1,1,1,1,1,1,1,1,1,1,1,1,1,1,1,1,1,1,
1,1,1,1,1,1,1,1,1,1,1,1,1,1,1,1,1,1,1,1,1,1,1,1,1,1,1,1,1,1,1,1,1,1,1,1,
1,1,1,1,1,1,1,1,1,1,1,1,1,1,1,1,1,1,1,1,1,1,1,1,1,1,1,1,1,1,1,1,1,1,1,1,
1,1,1,1,1,1,1,1,1,1,1,1,1,1,1,1,1,1,1,1,1,1,1,1,1,1,1,1,1,1,1,1,1,1,1,1,
1,1,1,1,1,1,1,1,1,1,1,1,1,1,1,1,1,1,1,1,1,1,1,1,1,1,1,1,1,1,1,1,1,1,1,1,
1,1,1,1,1,1,1,1,1,1,1,1,1,1,1,1,1,1,1,1,1,1,1,1,1,1,1,1,1,1,1,1,1,1,1,1,
1,1,1,1,1,1,1,1,1,1,1,1,1,1,1,1,1,1,1,1,1,1,1,1,1,1,1,1,1,1,1,1,1,1,1,1,
1,1,1,1,1,1,1,1,1,1,1,1,1,1,1,1,1,1,1,1,1,1,1,1,1,1,1,1,1,1,1,1,1,1,1,1,
1,1,1,1,1,1,1,1,1,1,1,1,1,1,1,1,1,1,1,1,1,1,1,1,1,1,1,1,1,1,1,1,1,1,1,1,
1,1,1,1,1,1,1,1,1,1,1,1,1,1,1,1,1,1,1,1,1,1,1,1,1,1,1,1,1,1,1,1,1,1,1,1,
1,1,1,1,1,1,1,1,1,1,1,1,1,1,1,1,1,1,1,1,1,1,1,1,1,1,1,1,1,1,1,1,1,1,1,1,
1,1,1,1,1,1,1,6),(2,2),(-1.,-0.999000000000001,-0.998000000000001,-0.997000000000001,
-0.996000000000001,-0.995000000000001,-0.994000000000001,-0.993000000000001,
-0.992000000000001,-0.991000000000001,-0.990000000000001,-0.989000000000001,
-0.988000000000001,-0.987000000000001,-0.986000000000001,-0.985000000000001,
-0.984000000000001,-0.983000000000001,-0.982000000000001,-0.981000000000001,
-0.980000000000001,-0.979000000000001,-0.978000000000001,-0.977000000000001,
-0.976000000000001,-0.975000000000001,-0.974000000000001,-0.973000000000001,
-0.972000000000001,-0.971000000000001,-0.970000000000001,-0.969000000000001,
-0.968000000000001,-0.967000000000001,-0.966000000000001,-0.965000000000001,
-0.964000000000001,-0.963000000000001,-0.962000000000001,-0.961000000000001,
-0.960000000000001,-0.959000000000001,-0.958000000000001,-0.957000000000001,
-0.956000000000001,-0.955000000000001,-0.954000000000001,-0.953000000000001,
-0.952000000000001,-0.951000000000001,-0.950000000000001,-0.949000000000001,
-0.948000000000001,-0.947000000000001,-0.946000000000001,-0.945000000000001,
-0.944000000000001,-0.943000000000001,-0.942000000000001,-0.941000000000001,
-0.940000000000001,-0.939000000000001,-0.938000000000001,-0.937000000000001,
-0.936000000000001,-0.935000000000001,-0.934000000000001,-0.933000000000001,
-0.932000000000001,-0.931000000000001,-0.930000000000001,-0.929000000000001,
-0.928000000000001,-0.927000000000001,-0.926000000000001,-0.925000000000001,
-0.924000000000001,-0.923000000000001,-0.922000000000001,-0.921000000000001,
-0.920000000000001,-0.919000000000001,-0.918000000000001,-0.917000000000001,
-0.916000000000001,-0.915000000000001,-0.914000000000001,-0.913000000000001,
-0.912000000000001,-0.911000000000001,-0.910000000000001,-0.909000000000001,
-0.908000000000001,-0.907000000000001,-0.906000000000001,-0.905000000000001,
-0.904000000000001,-0.903000000000001,-0.902000000000001,-0.901000000000001,
-0.900000000000001,-0.899000000000001,-0.898000000000001,-0.897000000000001,
-0.896000000000001,-0.895000000000001,-0.894000000000001,-0.893000000000001,
-0.892000000000001,-0.891000000000001,-0.890000000000001,-0.889000000000001,
-0.888000000000001,-0.887000000000001,-0.886000000000001,-0.885000000000001,
-0.884000000000001,-0.883000000000001,-0.882000000000001,-0.881000000000001,
-0.880000000000001,-0.879000000000001,-0.878000000000001,-0.877000000000001,
-0.876000000000001,-0.875000000000001,-0.874000000000001,-0.873000000000001,
-0.872000000000001,-0.871000000000001,-0.870000000000001,-0.869000000000001,
-0.868000000000001,-0.867000000000001,-0.866000000000001,-0.865000000000001,
-0.864000000000001,-0.863000000000001,-0.862000000000001,-0.861000000000001,
-0.860000000000001,-0.859000000000001,-0.858000000000001,-0.857000000000001,
-0.856000000000001,-0.855000000000001,-0.854000000000001,-0.853000000000001,
-0.852000000000001,-0.851000000000001,-0.850000000000001,-0.849000000000001,
-0.848000000000001,-0.847000000000001,-0.846000000000001,-0.845000000000001,
-0.844000000000001,-0.843000000000001,-0.842000000000001,-0.841000000000001,
-0.840000000000001,-0.839000000000001,-0.838000000000001,-0.837000000000001,
-0.836000000000001,-0.835000000000001,-0.834000000000001,-0.833000000000001,
-0.832000000000001,-0.831000000000001,-0.830000000000001,-0.829000000000001,
-0.828000000000001,-0.827000000000001,-0.826000000000001,-0.825000000000001,
-0.824000000000001,-0.823000000000001,-0.822000000000001,-0.821000000000001,
-0.820000000000001,-0.819000000000001,-0.818000000000001,-0.817000000000001,
-0.816000000000001,-0.815000000000001,-0.814000000000001,-0.813000000000001,
-0.812000000000001,-0.811000000000001,-0.810000000000001,-0.809000000000001,
-0.808000000000001,-0.807000000000001,-0.806000000000001,-0.805000000000001,
-0.804000000000001,-0.803000000000001,-0.802000000000001,-0.801000000000001,
-0.800000000000001,-0.799000000000001,-0.798000000000001,-0.797000000000001,
-0.796000000000001,-0.795000000000001,-0.794000000000001,-0.793000000000001,
-0.792000000000001,-0.791000000000001,-0.790000000000001,-0.789000000000001,
-0.788000000000001,-0.787000000000001,-0.786000000000001,-0.785000000000001,
-0.784000000000001,-0.783000000000001,-0.782000000000001,-0.781000000000001,
-0.780000000000001,-0.779000000000001,-0.778000000000001,-0.777000000000001,
-0.776000000000001,-0.775000000000001,-0.774000000000001,-0.773000000000001,
-0.772000000000001,-0.771000000000001,-0.770000000000001,-0.769000000000001,
-0.768000000000001,-0.767000000000001,-0.766000000000001,-0.765000000000001,
-0.764000000000001,-0.763000000000001,-0.762000000000001,-0.761000000000001,
-0.760000000000001,-0.759000000000001,-0.758000000000001,-0.757000000000001,
-0.756000000000001,-0.755000000000001,-0.754000000000001,-0.753000000000001,
-0.752000000000001,-0.751000000000001,-0.750000000000001,-0.749000000000001,
-0.748000000000001,-0.747000000000001,-0.746000000000001,-0.745000000000001,
-0.744000000000001,-0.743000000000001,-0.742000000000001,-0.741000000000001,
-0.740000000000001,-0.739000000000001,-0.738000000000001,-0.737000000000001,
-0.736000000000001,-0.735000000000001,-0.734000000000001,-0.733000000000001,
-0.732000000000001,-0.731000000000001,-0.730000000000001,-0.729000000000001,
-0.728000000000001,-0.727000000000001,-0.726000000000001,-0.725000000000001,
-0.724000000000001,-0.723000000000001,-0.722000000000001,-0.721000000000001,
-0.720000000000001,-0.719000000000001,-0.718000000000001,-0.717000000000001,
-0.716000000000001,-0.715000000000001,-0.714000000000001,-0.713000000000001,
-0.712000000000001,-0.711000000000001,-0.710000000000001,-0.709000000000001,
-0.708000000000001,-0.707000000000001,-0.706000000000001,-0.705000000000001,
-0.704000000000001,-0.703000000000001,-0.702000000000001,-0.701000000000001,
-0.700000000000001,-0.699000000000001,-0.698000000000001,-0.697000000000001,
-0.696000000000001,-0.695000000000001,-0.694000000000001,-0.693000000000001,
-0.692000000000001,-0.691000000000001,-0.690000000000001,-0.689000000000001,
-0.688000000000001,-0.687,-0.686,-0.685,-0.684,-0.683,-0.682,-0.681,-0.68,
-0.679,-0.678,-0.677,-0.676,-0.675,-0.674,-0.673,-0.672,-0.671,-0.67,-0.669,
-0.668,-0.667,-0.666,-0.665,-0.664,-0.663,-0.662,-0.661,-0.66,-0.659,-0.658,
-0.657,-0.656,-0.655,-0.654,-0.653,-0.652,-0.651,-0.65,-0.649,-0.648,-0.647,
-0.646,-0.645,-0.644,-0.643,-0.642,-0.641,-0.64,-0.639,-0.638,-0.637,-0.636,
-0.635,-0.634,-0.633,-0.632,-0.631,-0.63,-0.629,-0.628,-0.627,-0.626,-0.625,
-0.624,-0.623,-0.622,-0.621,-0.62,-0.619,-0.618,-0.617,-0.616,-0.615,-0.614,
-0.613,-0.612,-0.611,-0.61,-0.609,-0.608,-0.607,-0.606,-0.605,-0.604,-0.603,
-0.602,-0.601,-0.6,-0.599,-0.598,-0.597,-0.596,-0.595,-0.594,-0.593,-0.592,
-0.591,-0.59,-0.589,-0.588,-0.587,-0.586,-0.585,-0.584,-0.583,-0.582,-0.581,
-0.58,-0.579,-0.578,-0.577,-0.576,-0.575,-0.574,-0.573,-0.572,-0.571,-0.57,
-0.569,-0.568,-0.567,-0.566,-0.565,-0.564,-0.563,-0.562,-0.561,-0.56,-0.559,
-0.558,-0.557,-0.556,-0.555,-0.554,-0.553,-0.552,-0.551,-0.55,-0.549,-0.548,
-0.547,-0.546,-0.545,-0.544,-0.543,-0.542,-0.541,-0.54,-0.539,-0.538,-0.537,
-0.536,-0.535,-0.534,-0.533,-0.532,-0.531,-0.53,-0.529,-0.528,-0.527,-0.526,
-0.525,-0.524,-0.523,-0.522,-0.521,-0.52,-0.519,-0.518,-0.517,-0.516,-0.515,
-0.514,-0.513,-0.512,-0.511,-0.51,-0.509,-0.508,-0.507,-0.506,-0.505,-0.504,
-0.503,-0.502,-0.501,-0.5,-0.499,-0.498,-0.497,-0.496,-0.495,-0.494,-0.493,
-0.492,-0.491,-0.49,-0.489,-0.488,-0.487,-0.486,-0.485,-0.484,-0.483,-0.482,
-0.481,-0.48,-0.479,-0.478,-0.477,-0.476,-0.475,-0.474,-0.473,-0.472,-0.471,
-0.47,-0.469,-0.468,-0.467,-0.466,-0.465,-0.464,-0.463,-0.462,-0.461,-0.46,
-0.459,-0.458,-0.457,-0.456,-0.455,-0.454,-0.453,-0.452,-0.451,-0.45,-0.449,
-0.448,-0.447,-0.446,-0.445,-0.444,-0.443,-0.442,-0.441,-0.44,-0.439,-0.438,
-0.437,-0.436,-0.435,-0.434,-0.433,-0.432,-0.431,-0.43,-0.429,-0.428,-0.427,
-0.426,-0.425,-0.424,-0.423,-0.422,-0.421,-0.42,-0.419,-0.418,-0.417,-0.416,
-0.415,-0.414,-0.413,-0.412,-0.411,-0.41,-0.409,-0.408,-0.407,-0.406,-0.405,
-0.404,-0.403,-0.402,-0.401,-0.4,-0.399,-0.398,-0.397,-0.396,-0.395,-0.394,
-0.393,-0.392,-0.391,-0.39,-0.389,-0.388,-0.387,-0.386,-0.385,-0.384,-0.383,
-0.382,-0.381,-0.38,-0.379,-0.378,-0.377,-0.376,-0.375,-0.374,-0.373,-0.372,
-0.371,-0.37,-0.369,-0.368,-0.367,-0.366,-0.365,-0.364,-0.363,-0.362,-0.361,
-0.36,-0.359,-0.358,-0.357,-0.356,-0.355,-0.354,-0.353,-0.352,-0.351,-0.35,
-0.349,-0.348,-0.347,-0.346,-0.345,-0.344,-0.343,-0.342,-0.341,-0.34,-0.339,
-0.338,-0.337,-0.336,-0.335,-0.334,-0.333,-0.332,-0.331,-0.33,-0.329,-0.328,
-0.327,-0.326,-0.325,-0.324,-0.323,-0.322,-0.321,-0.32,-0.319,-0.318,-0.317,
-0.316,-0.315,-0.314,-0.313,-0.312,-0.311,-0.31,-0.309,-0.308,-0.307,-0.306,
-0.305,-0.304,-0.303,-0.302,-0.301,-0.3,-0.299,-0.298,-0.297,-0.296,-0.295,
-0.294,-0.293,-0.292,-0.291,-0.29,-0.289,-0.288,-0.287,-0.286,-0.285,-0.284,
-0.283,-0.282,-0.281,-0.28,-0.279,-0.278,-0.277,-0.276,-0.275,-0.274,-0.273,
-0.272,-0.271,-0.27,-0.269,-0.268,-0.267,-0.266,-0.265,-0.264,-0.263,-0.262,
-0.261,-0.26,-0.259,-0.258,-0.257,-0.256,-0.255,-0.254,-0.253,-0.252,-0.251,
-0.25,-0.249,-0.248,-0.247,-0.246,-0.245,-0.244,-0.243,-0.242,-0.241,-0.24,
-0.239,-0.238,-0.237,-0.236,-0.235,-0.234,-0.233,-0.232,-0.231,-0.23,-0.229,
-0.228,-0.227,-0.226,-0.225,-0.224,-0.223,-0.222,-0.221,-0.22,-0.219,-0.218,
-0.217,-0.216,-0.215,-0.214,-0.213,-0.212,-0.211,-0.21,-0.209,-0.208,-0.207,
-0.206,-0.205,-0.204,-0.203,-0.202,-0.201,-0.2,-0.199,-0.198,-0.197,-0.196,
-0.195,-0.194,-0.193,-0.192,-0.191,-0.19,-0.189,-0.188,-0.187,-0.186,-0.185,
-0.184,-0.183,-0.182,-0.181,-0.18,-0.179,-0.178,-0.177,-0.176,-0.175,-0.174,
-0.173,-0.172,-0.171,-0.17,-0.169,-0.168,-0.167,-0.166,-0.165,-0.164,-0.163,
-0.162,-0.161,-0.16,-0.159,-0.158,-0.157,-0.156,-0.155,-0.154,-0.153,-0.152,
-0.151,-0.15,-0.149,-0.148,-0.147,-0.146,-0.145,-0.144,-0.143,-0.142,-0.141,
-0.14,-0.139,-0.138,-0.137,-0.136,-0.135,-0.134,-0.133,-0.132,-0.131,-0.13,
-0.129,-0.128,-0.127,-0.126,-0.125,-0.124,-0.123,-0.122,-0.121,-0.12,-0.119,
-0.118,-0.117,-0.116,-0.115,-0.114,-0.113,-0.112,-0.111,-0.11,-0.109,-0.108,
-0.107,-0.106,-0.105,-0.104,-0.103,-0.102,-0.101,-0.1,-0.0990000000000001,
-0.0980000000000001,-0.0970000000000001,-0.0960000000000001,-0.0950000000000001,
-0.0940000000000001,-0.0930000000000001,-0.0920000000000001,-0.0910000000000001,
-0.0900000000000001,-0.0890000000000001,-0.0880000000000001,-0.0870000000000001,
-0.0860000000000001,-0.0850000000000001,-0.0840000000000001,-0.0830000000000001,
-0.0820000000000001,-0.0810000000000001,-0.0800000000000001,-0.0790000000000001,
-0.0780000000000001,-0.0770000000000001,-0.0760000000000001,-0.0750000000000001,
-0.0740000000000001,-0.0730000000000001,-0.0720000000000001,-0.071,-0.07,
-0.069,-0.068,-0.067,-0.066,-0.065,-0.064,-0.063,-0.062,-0.061,-0.06,-0.059,
-0.058,-0.057,-0.056,-0.055,-0.054,-0.053,-0.052,-0.051,-0.05,-0.049,-0.048,
-0.047,-0.046,-0.045,-0.044,-0.043,-0.042,-0.041,-0.04,-0.039,-0.038,-0.037,
-0.036,-0.035,-0.034,-0.033,-0.032,-0.031,-0.03,-0.029,-0.028,-0.027,-0.026,
-0.025,-0.024,-0.023,-0.022,-0.021,-0.02,-0.019,-0.018,-0.017,-0.016,-0.015,
-0.014,-0.013,-0.012,-0.011,-0.01,-0.009,-0.008,-0.007,-0.006,-0.005,-0.004,
-0.003,-0.002,-0.001,0.),(0.,2.),.UNSPECIFIED.)
GEOMETRIC_REPRESENTATION_ITEM()
RATIONAL_B_SPLINE_SURFACE(((1.,1.),(1.,1.),(1.,1.),(1.,1.),(1.,1.),(1.,
1.),(1.,1.),(1.,1.),(1.,1.),(1.,1.),(1.,1.),(1.,1.),(1.,1.),(1.,1.),(1.,
1.),(1.,1.),(1.,1.),(1.,1.),(1.,1.),(1.,1.),(1.,1.),(1.,1.),(1.,1.),(1.,
1.),(1.,1.),(1.,1.),(1.,1.),(1.,1.),(1.,1.),(1.,1.),(1.,1.),(1.,1.),(1.,
1.),(1.,1.),(1.,1.),(1.,1.),(1.,1.),(1.,1.),(1.,1.),(1.,1.),(1.,1.),(1.,
1.),(1.,1.),(1.,1.),(1.,1.),(1.,1.),(1.,1.),(1.,1.),(1.,1.),(1.,1.),(1.,
1.),(1.,1.),(1.,1.),(1.,1.),(1.,1.),(1.,1.),(1.,1.),(1.,1.),(1.,1.),(1.,
1.),(1.,1.),(1.,1.),(1.,1.),(1.,1.),(1.,1.),(1.,1.),(1.,1.),(1.,1.),(1.,
1.),(1.,1.),(1.,1.),(1.,1.),(1.,1.),(1.,1.),(1.,1.),(1.,1.),(1.,1.),(1.,
1.),(1.,1.),(1.,1.),(1.,1.),(1.,1.),(1.,1.),(1.,1.),(1.,1.),(1.,1.),(1.,
1.),(1.,1.),(1.,1.),(1.,1.),(1.,1.),(1.,1.),(1.,1.),(1.,1.),(1.,1.),(1.,
1.),(1.,1.),(1.,1.),(1.,1.),(1.,1.),(1.,1.),(1.,1.),(1.,1.),(1.,1.),(1.,
1.),(1.,1.),(1.,1.),(1.,1.),(1.,1.),(1.,1.),(1.,1.),(1.,1.),(1.,1.),(1.,
1.),(1.,1.),(1.,1.),(1.,1.),(1.,1.),(1.,1.),(1.,1.),(1.,1.),(1.,1.),(1.,
1.),(1.,1.),(1.,1.),(1.,1.),(1.,1.),(1.,1.),(1.,1.),(1.,1.),(1.,1.),(1.,
1.),(1.,1.),(1.,1.),(1.,1.),(1.,1.),(1.,1.),(1.,1.),(1.,1.),(1.,1.),(1.,
1.),(1.,1.),(1.,1.),(1.,1.),(1.,1.),(1.,1.),(1.,1.),(1.,1.),(1.,1.),(1.,
1.),(1.,1.),(1.,1.),(1.,1.),(1.,1.),(1.,1.),(1.,1.),(1.,1.),(1.,1.),(1.,
1.),(1.,1.),(1.,1.),(1.,1.),(1.,1.),(1.,1.),(1.,1.),(1.,1.),(1.,1.),(1.,
1.),(1.,1.),(1.,1.),(1.,1.),(1.,1.),(1.,1.),(1.,1.),(1.,1.),(1.,1.),(1.,
1.),(1.,1.),(1.,1.),(1.,1.),(1.,1.),(1.,1.),(1.,1.),(1.,1.),(1.,1.),(1.,
1.),(1.,1.),(1.,1.),(1.,1.),(1.,1.),(1.,1.),(1.,1.),(1.,1.),(1.,1.),(1.,
1.),(1.,1.),(1.,1.),(1.,1.),(1.,1.),(1.,1.),(1.,1.),(1.,1.),(1.,1.),(1.,
1.),(1.,1.),(1.,1.),(1.,1.),(1.,1.),(1.,1.),(1.,1.),(1.,1.),(1.,1.),(1.,
1.),(1.,1.),(1.,1.),(1.,1.),(1.,1.),(1.,1.),(1.,1.),(1.,1.),(1.,1.),(1.,
1.),(1.,1.),(1.,1.),(1.,1.),(1.,1.),(1.,1.),(1.,1.),(1.,1.),(1.,1.),(1.,
1.),(1.,1.),(1.,1.),(1.,1.),(1.,1.),(1.,1.),(1.,1.),(1.,1.),(1.,1.),(1.,
1.),(1.,1.),(1.,1.),(1.,1.),(1.,1.),(1.,1.),(1.,1.),(1.,1.),(1.,1.),(1.,
1.),(1.,1.),(1.,1.),(1.,1.),(1.,1.),(1.,1.),(1.,1.),(1.,1.),(1.,1.),(1.,
1.),(1.,1.),(1.,1.),(1.,1.),(1.,1.),(1.,1.),(1.,1.),(1.,1.),(1.,1.),(1.,
1.),(1.,1.),(1.,1.),(1.,1.),(1.,1.),(1.,1.),(1.,1.),(1.,1.),(1.,1.),(1.,
1.),(1.,1.),(1.,1.),(1.,1.),(1.,1.),(1.,1.),(1.,1.),(1.,1.),(1.,1.),(1.,
1.),(1.,1.),(1.,1.),(1.,1.),(1.,1.),(1.,1.),(1.,1.),(1.,1.),(1.,1.),(1.,
1.),(1.,1.),(1.,1.),(1.,1.),(1.,1.),(1.,1.),(1.,1.),(1.,1.),(1.,1.),(1.,
1.),(1.,1.),(1.,1.),(1.,1.),(1.,1.),(1.,1.),(1.,1.),(1.,1.),(1.,1.),(1.,
1.),(1.,1.),(1.,1.),(1.,1.),(1.,1.),(1.,1.),(1.,1.),(1.,1.),(1.,1.),(1.,
1.),(1.,1.),(1.,1.),(1.,1.),(1.,1.),(1.,1.),(1.,1.),(1.,1.),(1.,1.),(1.,
1.),(1.,1.),(1.,1.),(1.,1.),(1.,1.),(1.,1.),(1.,1.),(1.,1.),(1.,1.),(1.,
1.),(1.,1.),(1.,1.),(1.,1.),(1.,1.),(1.,1.),(1.,1.),(1.,1.),(1.,1.),(1.,
1.),(1.,1.),(1.,1.),(1.,1.),(1.,1.),(1.,1.),(1.,1.),(1.,1.),(1.,1.),(1.,
1.),(1.,1.),(1.,1.),(1.,1.),(1.,1.),(1.,1.),(1.,1.),(1.,1.),(1.,1.),(1.,
1.),(1.,1.),(1.,1.),(1.,1.),(1.,1.),(1.,1.),(1.,1.),(1.,1.),(1.,1.),(1.,
1.),(1.,1.),(1.,1.),(1.,1.),(1.,1.),(1.,1.),(1.,1.),(1.,1.),(1.,1.),(1.,
1.),(1.,1.),(1.,1.),(1.,1.),(1.,1.),(1.,1.),(1.,1.),(1.,1.),(1.,1.),(1.,
1.),(1.,1.),(1.,1.),(1.,1.),(1.,1.),(1.,1.),(1.,1.),(1.,1.),(1.,1.),(1.,
1.),(1.,1.),(1.,1.),(1.,1.),(1.,1.),(1.,1.),(1.,1.),(1.,1.),(1.,1.),(1.,
1.),(1.,1.),(1.,1.),(1.,1.),(1.,1.),(1.,1.),(1.,1.),(1.,1.),(1.,1.),(1.,
1.),(1.,1.),(1.,1.),(1.,1.),(1.,1.),(1.,1.),(1.,1.),(1.,1.),(1.,1.),(1.,
1.),(1.,1.),(1.,1.),(1.,1.),(1.,1.),(1.,1.),(1.,1.),(1.,1.),(1.,1.),(1.,
1.),(1.,1.),(1.,1.),(1.,1.),(1.,1.),(1.,1.),(1.,1.),(1.,1.),(1.,1.),(1.,
1.),(1.,1.),(1.,1.),(1.,1.),(1.,1.),(1.,1.),(1.,1.),(1.,1.),(1.,1.),(1.,
1.),(1.,1.),(1.,1.),(1.,1.),(1.,1.),(1.,1.),(1.,1.),(1.,1.),(1.,1.),(1.,
1.),(1.,1.),(1.,1.),(1.,1.),(1.,1.),(1.,1.),(1.,1.),(1.,1.),(1.,1.),(1.,
1.),(1.,1.),(1.,1.),(1.,1.),(1.,1.),(1.,1.),(1.,1.),(1.,1.),(1.,1.),(1.,
1.),(1.,1.),(1.,1.),(1.,1.),(1.,1.),(1.,1.),(1.,1.),(1.,1.),(1.,1.),(1.,
1.),(1.,1.),(1.,1.),(1.,1.),(1.,1.),(1.,1.),(1.,1.),(1.,1.),(1.,1.),(1.,
1.),(1.,1.),(1.,1.),(1.,1.),(1.,1.),(1.,1.),(1.,1.),(1.,1.),(1.,1.),(1.,
1.),(1.,1.),(1.,1.),(1.,1.),(1.,1.),(1.,1.),(1.,1.),(1.,1.),(1.,1.),(1.,
1.),(1.,1.),(1.,1.),(1.,1.),(1.,1.),(1.,1.),(1.,1.),(1.,1.),(1.,1.),(1.,
1.),(1.,1.),(1.,1.),(1.,1.),(1.,1.),(1.,1.),(1.,1.),(1.,1.),(1.,1.),(1.,
1.),(1.,1.),(1.,1.),(1.,1.),(1.,1.),(1.,1.),(1.,1.),(1.,1.),(1.,1.),(1.,
1.),(1.,1.),(1.,1.),(1.,1.),(1.,1.),(1.,1.),(1.,1.),(1.,1.),(1.,1.),(1.,
1.),(1.,1.),(1.,1.),(1.,1.),(1.,1.),(1.,1.),(1.,1.),(1.,1.),(1.,1.),(1.,
1.),(1.,1.),(1.,1.),(1.,1.),(1.,1.),(1.,1.),(1.,1.),(1.,1.),(1.,1.),(1.,
1.),(1.,1.),(1.,1.),(1.,1.),(1.,1.),(1.,1.),(1.,1.),(1.,1.),(1.,1.),(1.,
1.),(1.,1.),(1.,1.),(1.,1.),(1.,1.),(1.,1.),(1.,1.),(1.,1.),(1.,1.),(1.,
1.),(1.,1.),(1.,1.),(1.,1.),(1.,1.),(1.,1.),(1.,1.),(1.,1.),(1.,1.),(1.,
1.),(1.,1.),(1.,1.),(1.,1.),(1.,1.),(1.,1.),(1.,1.),(1.,1.),(1.,1.),(1.,
1.),(1.,1.),(1.,1.),(1.,1.),(1.,1.),(1.,1.),(1.,1.),(1.,1.),(1.,1.),(1.,
1.),(1.,1.),(1.,1.),(1.,1.),(1.,1.),(1.,1.),(1.,1.),(1.,1.),(1.,1.),(1.,
1.),(1.,1.),(1.,1.),(1.,1.),(1.,1.),(1.,1.),(1.,1.),(1.,1.),(1.,1.),(1.,
1.),(1.,1.),(1.,1.),(1.,1.),(1.,1.),(1.,1.),(1.,1.),(1.,1.),(1.,1.),(1.,
1.),(1.,1.),(1.,1.),(1.,1.),(1.,1.),(1.,1.),(1.,1.),(1.,1.),(1.,1.),(1.,
1.),(1.,1.),(1.,1.),(1.,1.),(1.,1.),(1.,1.),(1.,1.),(1.,1.),(1.,1.),(1.,
1.),(1.,1.),(1.,1.),(1.,1.),(1.,1.),(1.,1.),(1.,1.),(1.,1.),(1.,1.),(1.,
1.),(1.,1.),(1.,1.),(1.,1.),(1.,1.),(1.,1.),(1.,1.),(1.,1.),(1.,1.),(1.,
1.),(1.,1.),(1.,1.),(1.,1.),(1.,1.),(1.,1.),(1.,1.),(1.,1.),(1.,1.),(1.,
1.),(1.,1.),(1.,1.),(1.,1.),(1.,1.),(1.,1.),(1.,1.),(1.,1.),(1.,1.),(1.,
1.),(1.,1.),(1.,1.),(1.,1.),(1.,1.),(1.,1.),(1.,1.),(1.,1.),(1.,1.),(1.,
1.),(1.,1.),(1.,1.),(1.,1.),(1.,1.),(1.,1.),(1.,1.),(1.,1.),(1.,1.),(1.,
1.),(1.,1.),(1.,1.),(1.,1.),(1.,1.),(1.,1.),(1.,1.),(1.,1.),(1.,1.),(1.,
1.),(1.,1.),(1.,1.),(1.,1.),(1.,1.),(1.,1.),(1.,1.),(1.,1.),(1.,1.),(1.,
1.),(1.,1.),(1.,1.),(1.,1.),(1.,1.),(1.,1.),(1.,1.),(1.,1.),(1.,1.),(1.,
1.),(1.,1.),(1.,1.),(1.,1.),(1.,1.),(1.,1.),(1.,1.),(1.,1.),(1.,1.),(1.,
1.),(1.,1.),(1.,1.),(1.,1.),(1.,1.),(1.,1.),(1.,1.),(1.,1.),(1.,1.),(1.,
1.),(1.,1.),(1.,1.),(1.,1.),(1.,1.),(1.,1.),(1.,1.),(1.,1.),(1.,1.),(1.,
1.),(1.,1.),(1.,1.),(1.,1.),(1.,1.),(1.,1.),(1.,1.),(1.,1.),(1.,1.),(1.,
1.),(1.,1.),(1.,1.),(1.,1.),(1.,1.),(1.,1.),(1.,1.),(1.,1.),(1.,1.),(1.,
1.),(1.,1.),(1.,1.),(1.,1.),(1.,1.),(1.,1.),(1.,1.),(1.,1.),(1.,1.),(1.,
1.),(1.,1.),(1.,1.),(1.,1.),(1.,1.),(1.,1.),(1.,1.),(1.,1.),(1.,1.),(1.,
1.),(1.,1.),(1.,1.),(1.,1.),(1.,1.),(1.,1.),(1.,1.),(1.,1.),(1.,1.),(1.,
1.),(1.,1.),(1.,1.),(1.,1.),(1.,1.),(1.,1.),(1.,1.),(1.,1.),(1.,1.),(1.,
1.),(1.,1.),(1.,1.),(1.,1.),(1.,1.),(1.,1.),(1.,1.),(1.,1.),(1.,1.),(1.,
1.),(1.,1.),(1.,1.),(1.,1.),(1.,1.),(1.,1.),(1.,1.),(1.,1.),(1.,1.),(1.,
1.),(1.,1.),(1.,1.),(1.,1.),(1.,1.),(1.,1.),(1.,1.),(1.,1.),(1.,1.),(1.,
1.),(1.,1.),(1.,1.),(1.,1.),(1.,1.),(1.,1.),(1.,1.),(1.,1.),(1.,1.),(1.,
1.),(1.,1.),(1.,1.),(1.,1.),(1.,1.),(1.,1.),(1.,1.),(1.,1.),(1.,1.),(1.,
1.),(1.,1.),(1.,1.),(1.,1.),(1.,1.),(1.,1.),(1.,1.),(1.,1.),(1.,1.),(1.,
1.),(1.,1.),(1.,1.),(1.,1.),(1.,1.),(1.,1.),(1.,1.),(1.,1.),(1.,1.),(1.,
1.),(1.,1.),(1.,1.),(1.,1.),(1.,1.),(1.,1.),(1.,1.),(1.,1.),(1.,1.),(1.,
1.),(1.,1.),(1.,1.),(1.,1.),(1.,1.),(1.,1.),(1.,1.),(1.,1.),(1.,1.),(1.,
1.),(1.,1.),(1.,1.),(1.,1.),(1.,1.),(1.,1.),(1.,1.),(1.,1.),(1.,1.),(1.,
1.),(1.,1.),(1.,1.),(1.,1.),(1.,1.),(1.,1.),(1.,1.),(1.,1.),(1.,1.),(1.,
1.),(1.,1.),(1.,1.),(1.,1.),(1.,1.),(1.,1.),(1.,1.),(1.,1.),(1.,1.),(1.,
1.),(1.,1.),(1.,1.),(1.,1.),(1.,1.),(1.,1.),(1.,1.),(1.,1.),(1.,1.),(1.,
1.),(1.,1.),(1.,1.),(1.,1.),(1.,1.),(1.,1.),(1.,1.),(1.,1.),(1.,1.),(1.,
1.),(1.,1.),(1.,1.),(1.,1.),(1.,1.),(1.,1.),(1.,1.),(1.,1.),(1.,1.),(1.,
1.),(1.,1.),(1.,1.),(1.,1.),(1.,1.),(1.,1.),(1.,1.),(1.,1.),(1.,1.),(1.,
1.),(1.,1.),(1.,1.),(1.,1.),(1.,1.),(1.,1.),(1.,1.),(1.,1.),(1.,1.),(1.,
1.),(1.,1.),(1.,1.),(1.,1.),(1.,1.),(1.,1.),(1.,1.),(1.,1.),(1.,1.),(1.,
1.),(1.,1.),(1.,1.),(1.,1.),(1.,1.),(1.,1.),(1.,1.),(1.,1.),(1.,1.),(1.,
1.),(1.,1.),(1.,1.),(1.,1.),(1.,1.),(1.,1.),(1.,1.),(1.,1.),(1.,1.),(1.,
1.)))
REPRESENTATION_ITEM('')
SURFACE()
);
#259=(
BOUNDED_SURFACE()
B_SPLINE_SURFACE(5,1,((#76117,#76118),(#76119,#76120),(#76121,#76122),(#76123,
#76124),(#76125,#76126),(#76127,#76128),(#76129,#76130),(#76131,#76132),
(#76133,#76134),(#76135,#76136),(#76137,#76138),(#76139,#76140),(#76141,
#76142),(#76143,#76144),(#76145,#76146),(#76147,#76148),(#76149,#76150),
(#76151,#76152),(#76153,#76154),(#76155,#76156),(#76157,#76158),(#76159,
#76160),(#76161,#76162),(#76163,#76164),(#76165,#76166),(#76167,#76168),
(#76169,#76170),(#76171,#76172),(#76173,#76174),(#76175,#76176),(#76177,
#76178),(#76179,#76180),(#76181,#76182),(#76183,#76184),(#76185,#76186),
(#76187,#76188),(#76189,#76190),(#76191,#76192),(#76193,#76194),(#76195,
#76196),(#76197,#76198),(#76199,#76200),(#76201,#76202),(#76203,#76204),
(#76205,#76206),(#76207,#76208),(#76209,#76210),(#76211,#76212),(#76213,
#76214),(#76215,#76216),(#76217,#76218),(#76219,#76220),(#76221,#76222),
(#76223,#76224),(#76225,#76226),(#76227,#76228),(#76229,#76230),(#76231,
#76232),(#76233,#76234),(#76235,#76236),(#76237,#76238),(#76239,#76240),
(#76241,#76242),(#76243,#76244),(#76245,#76246),(#76247,#76248),(#76249,
#76250),(#76251,#76252),(#76253,#76254),(#76255,#76256),(#76257,#76258),
(#76259,#76260),(#76261,#76262),(#76263,#76264),(#76265,#76266),(#76267,
#76268),(#76269,#76270),(#76271,#76272),(#76273,#76274),(#76275,#76276),
(#76277,#76278),(#76279,#76280),(#76281,#76282),(#76283,#76284),(#76285,
#76286),(#76287,#76288),(#76289,#76290),(#76291,#76292),(#76293,#76294),
(#76295,#76296),(#76297,#76298),(#76299,#76300),(#76301,#76302),(#76303,
#76304),(#76305,#76306),(#76307,#76308),(#76309,#76310),(#76311,#76312),
(#76313,#76314),(#76315,#76316),(#76317,#76318),(#76319,#76320),(#76321,
#76322),(#76323,#76324),(#76325,#76326),(#76327,#76328),(#76329,#76330),
(#76331,#76332),(#76333,#76334),(#76335,#76336),(#76337,#76338),(#76339,
#76340),(#76341,#76342),(#76343,#76344),(#76345,#76346),(#76347,#76348),
(#76349,#76350),(#76351,#76352),(#76353,#76354),(#76355,#76356),(#76357,
#76358),(#76359,#76360),(#76361,#76362),(#76363,#76364),(#76365,#76366),
(#76367,#76368),(#76369,#76370),(#76371,#76372),(#76373,#76374),(#76375,
#76376),(#76377,#76378),(#76379,#76380),(#76381,#76382),(#76383,#76384),
(#76385,#76386),(#76387,#76388),(#76389,#76390),(#76391,#76392),(#76393,
#76394),(#76395,#76396),(#76397,#76398),(#76399,#76400),(#76401,#76402),
(#76403,#76404),(#76405,#76406),(#76407,#76408),(#76409,#76410),(#76411,
#76412),(#76413,#76414),(#76415,#76416),(#76417,#76418),(#76419,#76420),
(#76421,#76422),(#76423,#76424),(#76425,#76426),(#76427,#76428),(#76429,
#76430),(#76431,#76432),(#76433,#76434),(#76435,#76436),(#76437,#76438),
(#76439,#76440),(#76441,#76442),(#76443,#76444),(#76445,#76446),(#76447,
#76448),(#76449,#76450),(#76451,#76452),(#76453,#76454),(#76455,#76456),
(#76457,#76458),(#76459,#76460),(#76461,#76462),(#76463,#76464),(#76465,
#76466),(#76467,#76468),(#76469,#76470),(#76471,#76472),(#76473,#76474),
(#76475,#76476),(#76477,#76478),(#76479,#76480),(#76481,#76482),(#76483,
#76484),(#76485,#76486),(#76487,#76488),(#76489,#76490),(#76491,#76492),
(#76493,#76494),(#76495,#76496),(#76497,#76498),(#76499,#76500),(#76501,
#76502),(#76503,#76504),(#76505,#76506),(#76507,#76508),(#76509,#76510),
(#76511,#76512),(#76513,#76514),(#76515,#76516),(#76517,#76518),(#76519,
#76520),(#76521,#76522),(#76523,#76524),(#76525,#76526),(#76527,#76528),
(#76529,#76530),(#76531,#76532),(#76533,#76534),(#76535,#76536),(#76537,
#76538),(#76539,#76540),(#76541,#76542),(#76543,#76544),(#76545,#76546),
(#76547,#76548),(#76549,#76550),(#76551,#76552),(#76553,#76554),(#76555,
#76556),(#76557,#76558),(#76559,#76560),(#76561,#76562),(#76563,#76564),
(#76565,#76566),(#76567,#76568),(#76569,#76570),(#76571,#76572),(#76573,
#76574),(#76575,#76576),(#76577,#76578),(#76579,#76580),(#76581,#76582),
(#76583,#76584),(#76585,#76586),(#76587,#76588),(#76589,#76590),(#76591,
#76592),(#76593,#76594),(#76595,#76596),(#76597,#76598),(#76599,#76600),
(#76601,#76602),(#76603,#76604),(#76605,#76606),(#76607,#76608),(#76609,
#76610),(#76611,#76612),(#76613,#76614),(#76615,#76616),(#76617,#76618),
(#76619,#76620),(#76621,#76622),(#76623,#76624),(#76625,#76626),(#76627,
#76628),(#76629,#76630),(#76631,#76632),(#76633,#76634),(#76635,#76636),
(#76637,#76638),(#76639,#76640),(#76641,#76642),(#76643,#76644),(#76645,
#76646),(#76647,#76648),(#76649,#76650),(#76651,#76652),(#76653,#76654),
(#76655,#76656),(#76657,#76658),(#76659,#76660),(#76661,#76662),(#76663,
#76664),(#76665,#76666),(#76667,#76668),(#76669,#76670),(#76671,#76672),
(#76673,#76674),(#76675,#76676),(#76677,#76678),(#76679,#76680),(#76681,
#76682),(#76683,#76684),(#76685,#76686),(#76687,#76688),(#76689,#76690),
(#76691,#76692),(#76693,#76694),(#76695,#76696),(#76697,#76698),(#76699,
#76700),(#76701,#76702),(#76703,#76704),(#76705,#76706),(#76707,#76708),
(#76709,#76710),(#76711,#76712),(#76713,#76714),(#76715,#76716),(#76717,
#76718),(#76719,#76720),(#76721,#76722),(#76723,#76724),(#76725,#76726),
(#76727,#76728),(#76729,#76730),(#76731,#76732),(#76733,#76734),(#76735,
#76736),(#76737,#76738),(#76739,#76740),(#76741,#76742),(#76743,#76744),
(#76745,#76746),(#76747,#76748),(#76749,#76750),(#76751,#76752),(#76753,
#76754),(#76755,#76756),(#76757,#76758),(#76759,#76760),(#76761,#76762),
(#76763,#76764),(#76765,#76766),(#76767,#76768),(#76769,#76770),(#76771,
#76772),(#76773,#76774),(#76775,#76776),(#76777,#76778),(#76779,#76780),
(#76781,#76782),(#76783,#76784),(#76785,#76786),(#76787,#76788),(#76789,
#76790),(#76791,#76792),(#76793,#76794),(#76795,#76796),(#76797,#76798),
(#76799,#76800),(#76801,#76802),(#76803,#76804),(#76805,#76806),(#76807,
#76808),(#76809,#76810),(#76811,#76812),(#76813,#76814),(#76815,#76816),
(#76817,#76818),(#76819,#76820),(#76821,#76822),(#76823,#76824),(#76825,
#76826),(#76827,#76828),(#76829,#76830),(#76831,#76832),(#76833,#76834),
(#76835,#76836),(#76837,#76838),(#76839,#76840),(#76841,#76842),(#76843,
#76844),(#76845,#76846),(#76847,#76848),(#76849,#76850),(#76851,#76852),
(#76853,#76854),(#76855,#76856),(#76857,#76858),(#76859,#76860),(#76861,
#76862),(#76863,#76864),(#76865,#76866),(#76867,#76868),(#76869,#76870),
(#76871,#76872),(#76873,#76874),(#76875,#76876),(#76877,#76878),(#76879,
#76880),(#76881,#76882),(#76883,#76884),(#76885,#76886),(#76887,#76888),
(#76889,#76890),(#76891,#76892),(#76893,#76894),(#76895,#76896),(#76897,
#76898),(#76899,#76900),(#76901,#76902),(#76903,#76904),(#76905,#76906),
(#76907,#76908),(#76909,#76910),(#76911,#76912),(#76913,#76914),(#76915,
#76916),(#76917,#76918),(#76919,#76920),(#76921,#76922),(#76923,#76924),
(#76925,#76926),(#76927,#76928),(#76929,#76930),(#76931,#76932),(#76933,
#76934),(#76935,#76936),(#76937,#76938),(#76939,#76940),(#76941,#76942),
(#76943,#76944),(#76945,#76946),(#76947,#76948),(#76949,#76950),(#76951,
#76952),(#76953,#76954),(#76955,#76956),(#76957,#76958),(#76959,#76960),
(#76961,#76962),(#76963,#76964),(#76965,#76966),(#76967,#76968),(#76969,
#76970),(#76971,#76972),(#76973,#76974),(#76975,#76976),(#76977,#76978),
(#76979,#76980),(#76981,#76982),(#76983,#76984),(#76985,#76986),(#76987,
#76988),(#76989,#76990),(#76991,#76992),(#76993,#76994),(#76995,#76996),
(#76997,#76998),(#76999,#77000),(#77001,#77002),(#77003,#77004),(#77005,
#77006),(#77007,#77008),(#77009,#77010),(#77011,#77012),(#77013,#77014),
(#77015,#77016),(#77017,#77018),(#77019,#77020),(#77021,#77022),(#77023,
#77024),(#77025,#77026),(#77027,#77028),(#77029,#77030),(#77031,#77032),
(#77033,#77034),(#77035,#77036),(#77037,#77038),(#77039,#77040),(#77041,
#77042),(#77043,#77044),(#77045,#77046),(#77047,#77048),(#77049,#77050),
(#77051,#77052),(#77053,#77054),(#77055,#77056),(#77057,#77058),(#77059,
#77060),(#77061,#77062),(#77063,#77064),(#77065,#77066),(#77067,#77068),
(#77069,#77070),(#77071,#77072),(#77073,#77074),(#77075,#77076),(#77077,
#77078),(#77079,#77080),(#77081,#77082),(#77083,#77084),(#77085,#77086),
(#77087,#77088),(#77089,#77090),(#77091,#77092),(#77093,#77094),(#77095,
#77096),(#77097,#77098),(#77099,#77100),(#77101,#77102),(#77103,#77104),
(#77105,#77106),(#77107,#77108),(#77109,#77110),(#77111,#77112),(#77113,
#77114),(#77115,#77116),(#77117,#77118),(#77119,#77120),(#77121,#77122),
(#77123,#77124),(#77125,#77126),(#77127,#77128),(#77129,#77130),(#77131,
#77132),(#77133,#77134),(#77135,#77136),(#77137,#77138),(#77139,#77140),
(#77141,#77142),(#77143,#77144),(#77145,#77146),(#77147,#77148),(#77149,
#77150),(#77151,#77152),(#77153,#77154),(#77155,#77156),(#77157,#77158),
(#77159,#77160),(#77161,#77162),(#77163,#77164),(#77165,#77166),(#77167,
#77168),(#77169,#77170),(#77171,#77172),(#77173,#77174),(#77175,#77176),
(#77177,#77178),(#77179,#77180),(#77181,#77182),(#77183,#77184),(#77185,
#77186),(#77187,#77188),(#77189,#77190),(#77191,#77192),(#77193,#77194),
(#77195,#77196),(#77197,#77198),(#77199,#77200),(#77201,#77202),(#77203,
#77204),(#77205,#77206),(#77207,#77208),(#77209,#77210),(#77211,#77212),
(#77213,#77214),(#77215,#77216),(#77217,#77218),(#77219,#77220),(#77221,
#77222),(#77223,#77224),(#77225,#77226),(#77227,#77228),(#77229,#77230),
(#77231,#77232),(#77233,#77234),(#77235,#77236),(#77237,#77238),(#77239,
#77240),(#77241,#77242),(#77243,#77244),(#77245,#77246),(#77247,#77248),
(#77249,#77250),(#77251,#77252),(#77253,#77254),(#77255,#77256),(#77257,
#77258),(#77259,#77260),(#77261,#77262),(#77263,#77264),(#77265,#77266),
(#77267,#77268),(#77269,#77270),(#77271,#77272),(#77273,#77274),(#77275,
#77276),(#77277,#77278),(#77279,#77280),(#77281,#77282),(#77283,#77284),
(#77285,#77286),(#77287,#77288),(#77289,#77290),(#77291,#77292),(#77293,
#77294),(#77295,#77296),(#77297,#77298),(#77299,#77300),(#77301,#77302),
(#77303,#77304),(#77305,#77306),(#77307,#77308),(#77309,#77310),(#77311,
#77312),(#77313,#77314),(#77315,#77316),(#77317,#77318),(#77319,#77320),
(#77321,#77322),(#77323,#77324),(#77325,#77326),(#77327,#77328),(#77329,
#77330),(#77331,#77332),(#77333,#77334),(#77335,#77336),(#77337,#77338),
(#77339,#77340),(#77341,#77342),(#77343,#77344),(#77345,#77346),(#77347,
#77348),(#77349,#77350),(#77351,#77352),(#77353,#77354),(#77355,#77356),
(#77357,#77358),(#77359,#77360),(#77361,#77362),(#77363,#77364),(#77365,
#77366),(#77367,#77368),(#77369,#77370),(#77371,#77372),(#77373,#77374),
(#77375,#77376),(#77377,#77378),(#77379,#77380),(#77381,#77382),(#77383,
#77384),(#77385,#77386),(#77387,#77388),(#77389,#77390),(#77391,#77392),
(#77393,#77394),(#77395,#77396),(#77397,#77398),(#77399,#77400),(#77401,
#77402),(#77403,#77404),(#77405,#77406),(#77407,#77408),(#77409,#77410),
(#77411,#77412),(#77413,#77414),(#77415,#77416),(#77417,#77418),(#77419,
#77420),(#77421,#77422),(#77423,#77424),(#77425,#77426),(#77427,#77428),
(#77429,#77430),(#77431,#77432),(#77433,#77434),(#77435,#77436),(#77437,
#77438),(#77439,#77440),(#77441,#77442),(#77443,#77444),(#77445,#77446),
(#77447,#77448),(#77449,#77450),(#77451,#77452),(#77453,#77454),(#77455,
#77456),(#77457,#77458),(#77459,#77460),(#77461,#77462),(#77463,#77464),
(#77465,#77466),(#77467,#77468),(#77469,#77470),(#77471,#77472),(#77473,
#77474),(#77475,#77476),(#77477,#77478),(#77479,#77480),(#77481,#77482),
(#77483,#77484),(#77485,#77486),(#77487,#77488),(#77489,#77490),(#77491,
#77492),(#77493,#77494),(#77495,#77496),(#77497,#77498),(#77499,#77500),
(#77501,#77502),(#77503,#77504),(#77505,#77506),(#77507,#77508),(#77509,
#77510),(#77511,#77512),(#77513,#77514),(#77515,#77516),(#77517,#77518),
(#77519,#77520),(#77521,#77522),(#77523,#77524),(#77525,#77526),(#77527,
#77528),(#77529,#77530),(#77531,#77532),(#77533,#77534),(#77535,#77536),
(#77537,#77538),(#77539,#77540),(#77541,#77542),(#77543,#77544),(#77545,
#77546),(#77547,#77548),(#77549,#77550),(#77551,#77552),(#77553,#77554),
(#77555,#77556),(#77557,#77558),(#77559,#77560),(#77561,#77562),(#77563,
#77564),(#77565,#77566),(#77567,#77568),(#77569,#77570),(#77571,#77572),
(#77573,#77574),(#77575,#77576),(#77577,#77578),(#77579,#77580),(#77581,
#77582),(#77583,#77584),(#77585,#77586),(#77587,#77588),(#77589,#77590),
(#77591,#77592),(#77593,#77594),(#77595,#77596),(#77597,#77598),(#77599,
#77600),(#77601,#77602),(#77603,#77604),(#77605,#77606),(#77607,#77608),
(#77609,#77610),(#77611,#77612),(#77613,#77614),(#77615,#77616),(#77617,
#77618),(#77619,#77620),(#77621,#77622),(#77623,#77624),(#77625,#77626),
(#77627,#77628),(#77629,#77630),(#77631,#77632),(#77633,#77634),(#77635,
#77636),(#77637,#77638),(#77639,#77640),(#77641,#77642),(#77643,#77644),
(#77645,#77646),(#77647,#77648),(#77649,#77650),(#77651,#77652),(#77653,
#77654),(#77655,#77656),(#77657,#77658),(#77659,#77660),(#77661,#77662),
(#77663,#77664),(#77665,#77666),(#77667,#77668),(#77669,#77670),(#77671,
#77672),(#77673,#77674),(#77675,#77676),(#77677,#77678),(#77679,#77680),
(#77681,#77682),(#77683,#77684),(#77685,#77686),(#77687,#77688),(#77689,
#77690),(#77691,#77692),(#77693,#77694),(#77695,#77696),(#77697,#77698),
(#77699,#77700),(#77701,#77702),(#77703,#77704),(#77705,#77706),(#77707,
#77708),(#77709,#77710),(#77711,#77712),(#77713,#77714),(#77715,#77716),
(#77717,#77718),(#77719,#77720),(#77721,#77722),(#77723,#77724),(#77725,
#77726),(#77727,#77728),(#77729,#77730),(#77731,#77732),(#77733,#77734),
(#77735,#77736),(#77737,#77738),(#77739,#77740),(#77741,#77742),(#77743,
#77744),(#77745,#77746),(#77747,#77748),(#77749,#77750),(#77751,#77752),
(#77753,#77754),(#77755,#77756),(#77757,#77758),(#77759,#77760),(#77761,
#77762),(#77763,#77764),(#77765,#77766),(#77767,#77768),(#77769,#77770),
(#77771,#77772),(#77773,#77774),(#77775,#77776),(#77777,#77778),(#77779,
#77780),(#77781,#77782),(#77783,#77784),(#77785,#77786),(#77787,#77788),
(#77789,#77790),(#77791,#77792),(#77793,#77794),(#77795,#77796),(#77797,
#77798),(#77799,#77800),(#77801,#77802),(#77803,#77804),(#77805,#77806),
(#77807,#77808),(#77809,#77810),(#77811,#77812),(#77813,#77814),(#77815,
#77816),(#77817,#77818),(#77819,#77820),(#77821,#77822),(#77823,#77824),
(#77825,#77826),(#77827,#77828),(#77829,#77830),(#77831,#77832),(#77833,
#77834),(#77835,#77836),(#77837,#77838),(#77839,#77840),(#77841,#77842),
(#77843,#77844),(#77845,#77846),(#77847,#77848),(#77849,#77850),(#77851,
#77852),(#77853,#77854),(#77855,#77856),(#77857,#77858),(#77859,#77860),
(#77861,#77862),(#77863,#77864),(#77865,#77866),(#77867,#77868),(#77869,
#77870),(#77871,#77872),(#77873,#77874),(#77875,#77876),(#77877,#77878),
(#77879,#77880),(#77881,#77882),(#77883,#77884),(#77885,#77886),(#77887,
#77888),(#77889,#77890),(#77891,#77892),(#77893,#77894),(#77895,#77896),
(#77897,#77898),(#77899,#77900),(#77901,#77902),(#77903,#77904),(#77905,
#77906),(#77907,#77908),(#77909,#77910),(#77911,#77912),(#77913,#77914),
(#77915,#77916),(#77917,#77918),(#77919,#77920),(#77921,#77922),(#77923,
#77924),(#77925,#77926),(#77927,#77928),(#77929,#77930),(#77931,#77932),
(#77933,#77934),(#77935,#77936),(#77937,#77938),(#77939,#77940),(#77941,
#77942),(#77943,#77944),(#77945,#77946),(#77947,#77948),(#77949,#77950),
(#77951,#77952),(#77953,#77954),(#77955,#77956),(#77957,#77958),(#77959,
#77960),(#77961,#77962),(#77963,#77964),(#77965,#77966),(#77967,#77968),
(#77969,#77970),(#77971,#77972),(#77973,#77974),(#77975,#77976),(#77977,
#77978),(#77979,#77980),(#77981,#77982),(#77983,#77984),(#77985,#77986),
(#77987,#77988),(#77989,#77990),(#77991,#77992),(#77993,#77994),(#77995,
#77996),(#77997,#77998),(#77999,#78000),(#78001,#78002),(#78003,#78004),
(#78005,#78006),(#78007,#78008),(#78009,#78010),(#78011,#78012),(#78013,
#78014),(#78015,#78016),(#78017,#78018),(#78019,#78020),(#78021,#78022),
(#78023,#78024),(#78025,#78026),(#78027,#78028),(#78029,#78030),(#78031,
#78032),(#78033,#78034),(#78035,#78036),(#78037,#78038),(#78039,#78040),
(#78041,#78042),(#78043,#78044),(#78045,#78046),(#78047,#78048),(#78049,
#78050),(#78051,#78052),(#78053,#78054),(#78055,#78056),(#78057,#78058),
(#78059,#78060),(#78061,#78062),(#78063,#78064),(#78065,#78066),(#78067,
#78068),(#78069,#78070),(#78071,#78072),(#78073,#78074),(#78075,#78076),
(#78077,#78078),(#78079,#78080),(#78081,#78082),(#78083,#78084),(#78085,
#78086),(#78087,#78088),(#78089,#78090),(#78091,#78092),(#78093,#78094),
(#78095,#78096),(#78097,#78098),(#78099,#78100),(#78101,#78102),(#78103,
#78104),(#78105,#78106),(#78107,#78108),(#78109,#78110),(#78111,#78112),
(#78113,#78114),(#78115,#78116),(#78117,#78118),(#78119,#78120),(#78121,
#78122),(#78123,#78124),(#78125,#78126)),.UNSPECIFIED.,.F.,.F.,.F.)
B_SPLINE_SURFACE_WITH_KNOTS((6,1,1,1,1,1,1,1,1,1,1,1,1,1,1,1,1,1,1,1,1,
1,1,1,1,1,1,1,1,1,1,1,1,1,1,1,1,1,1,1,1,1,1,1,1,1,1,1,1,1,1,1,1,1,1,1,1,
1,1,1,1,1,1,1,1,1,1,1,1,1,1,1,1,1,1,1,1,1,1,1,1,1,1,1,1,1,1,1,1,1,1,1,1,
1,1,1,1,1,1,1,1,1,1,1,1,1,1,1,1,1,1,1,1,1,1,1,1,1,1,1,1,1,1,1,1,1,1,1,1,
1,1,1,1,1,1,1,1,1,1,1,1,1,1,1,1,1,1,1,1,1,1,1,1,1,1,1,1,1,1,1,1,1,1,1,1,
1,1,1,1,1,1,1,1,1,1,1,1,1,1,1,1,1,1,1,1,1,1,1,1,1,1,1,1,1,1,1,1,1,1,1,1,
1,1,1,1,1,1,1,1,1,1,1,1,1,1,1,1,1,1,1,1,1,1,1,1,1,1,1,1,1,1,1,1,1,1,1,1,
1,1,1,1,1,1,1,1,1,1,1,1,1,1,1,1,1,1,1,1,1,1,1,1,1,1,1,1,1,1,1,1,1,1,1,1,
1,1,1,1,1,1,1,1,1,1,1,1,1,1,1,1,1,1,1,1,1,1,1,1,1,1,1,1,1,1,1,1,1,1,1,1,
1,1,1,1,1,1,1,1,1,1,1,1,1,1,1,1,1,1,1,1,1,1,1,1,1,1,1,1,1,1,1,1,1,1,1,1,
1,1,1,1,1,1,1,1,1,1,1,1,1,1,1,1,1,1,1,1,1,1,1,1,1,1,1,1,1,1,1,1,1,1,1,1,
1,1,1,1,1,1,1,1,1,1,1,1,1,1,1,1,1,1,1,1,1,1,1,1,1,1,1,1,1,1,1,1,1,1,1,1,
1,1,1,1,1,1,1,1,1,1,1,1,1,1,1,1,1,1,1,1,1,1,1,1,1,1,1,1,1,1,1,1,1,1,1,1,
1,1,1,1,1,1,1,1,1,1,1,1,1,1,1,1,1,1,1,1,1,1,1,1,1,1,1,1,1,1,1,1,1,1,1,1,
1,1,1,1,1,1,1,1,1,1,1,1,1,1,1,1,1,1,1,1,1,1,1,1,1,1,1,1,1,1,1,1,1,1,1,1,
1,1,1,1,1,1,1,1,1,1,1,1,1,1,1,1,1,1,1,1,1,1,1,1,1,1,1,1,1,1,1,1,1,1,1,1,
1,1,1,1,1,1,1,1,1,1,1,1,1,1,1,1,1,1,1,1,1,1,1,1,1,1,1,1,1,1,1,1,1,1,1,1,
1,1,1,1,1,1,1,1,1,1,1,1,1,1,1,1,1,1,1,1,1,1,1,1,1,1,1,1,1,1,1,1,1,1,1,1,
1,1,1,1,1,1,1,1,1,1,1,1,1,1,1,1,1,1,1,1,1,1,1,1,1,1,1,1,1,1,1,1,1,1,1,1,
1,1,1,1,1,1,1,1,1,1,1,1,1,1,1,1,1,1,1,1,1,1,1,1,1,1,1,1,1,1,1,1,1,1,1,1,
1,1,1,1,1,1,1,1,1,1,1,1,1,1,1,1,1,1,1,1,1,1,1,1,1,1,1,1,1,1,1,1,1,1,1,1,
1,1,1,1,1,1,1,1,1,1,1,1,1,1,1,1,1,1,1,1,1,1,1,1,1,1,1,1,1,1,1,1,1,1,1,1,
1,1,1,1,1,1,1,1,1,1,1,1,1,1,1,1,1,1,1,1,1,1,1,1,1,1,1,1,1,1,1,1,1,1,1,1,
1,1,1,1,1,1,1,1,1,1,1,1,1,1,1,1,1,1,1,1,1,1,1,1,1,1,1,1,1,1,1,1,1,1,1,1,
1,1,1,1,1,1,1,1,1,1,1,1,1,1,1,1,1,1,1,1,1,1,1,1,1,1,1,1,1,1,1,1,1,1,1,1,
1,1,1,1,1,1,1,1,1,1,1,1,1,1,1,1,1,1,1,1,1,1,1,1,1,1,1,1,1,1,1,1,1,1,1,1,
1,1,1,1,1,1,1,1,1,1,1,1,1,1,1,1,1,1,1,1,1,1,1,1,1,1,1,1,1,1,1,1,1,1,1,1,
1,1,1,1,1,1,1,1,1,1,1,1,1,1,1,1,1,1,1,1,1,1,1,1,1,1,1,1,1,1,1,1,1,1,1,1,
1,1,1,1,1,1,1,6),(2,2),(-1.,-0.999000000000001,-0.998000000000001,-0.997000000000001,
-0.996000000000001,-0.995000000000001,-0.994000000000001,-0.993000000000001,
-0.992000000000001,-0.991000000000001,-0.990000000000001,-0.989000000000001,
-0.988000000000001,-0.987000000000001,-0.986000000000001,-0.985000000000001,
-0.984000000000001,-0.983000000000001,-0.982000000000001,-0.981000000000001,
-0.980000000000001,-0.979000000000001,-0.978000000000001,-0.977000000000001,
-0.976000000000001,-0.975000000000001,-0.974000000000001,-0.973000000000001,
-0.972000000000001,-0.971000000000001,-0.970000000000001,-0.969000000000001,
-0.968000000000001,-0.967000000000001,-0.966000000000001,-0.965000000000001,
-0.964000000000001,-0.963000000000001,-0.962000000000001,-0.961000000000001,
-0.960000000000001,-0.959000000000001,-0.958000000000001,-0.957000000000001,
-0.956000000000001,-0.955000000000001,-0.954000000000001,-0.953000000000001,
-0.952000000000001,-0.951000000000001,-0.950000000000001,-0.949000000000001,
-0.948000000000001,-0.947000000000001,-0.946000000000001,-0.945000000000001,
-0.944000000000001,-0.943000000000001,-0.942000000000001,-0.941000000000001,
-0.940000000000001,-0.939000000000001,-0.938000000000001,-0.937000000000001,
-0.936000000000001,-0.935000000000001,-0.934000000000001,-0.933000000000001,
-0.932000000000001,-0.931000000000001,-0.930000000000001,-0.929000000000001,
-0.928000000000001,-0.927000000000001,-0.926000000000001,-0.925000000000001,
-0.924000000000001,-0.923000000000001,-0.922000000000001,-0.921000000000001,
-0.920000000000001,-0.919000000000001,-0.918000000000001,-0.917000000000001,
-0.916000000000001,-0.915000000000001,-0.914000000000001,-0.913000000000001,
-0.912000000000001,-0.911000000000001,-0.910000000000001,-0.909000000000001,
-0.908000000000001,-0.907000000000001,-0.906000000000001,-0.905000000000001,
-0.904000000000001,-0.903000000000001,-0.902000000000001,-0.901000000000001,
-0.900000000000001,-0.899000000000001,-0.898000000000001,-0.897000000000001,
-0.896000000000001,-0.895000000000001,-0.894000000000001,-0.893000000000001,
-0.892000000000001,-0.891000000000001,-0.890000000000001,-0.889000000000001,
-0.888000000000001,-0.887000000000001,-0.886000000000001,-0.885000000000001,
-0.884000000000001,-0.883000000000001,-0.882000000000001,-0.881000000000001,
-0.880000000000001,-0.879000000000001,-0.878000000000001,-0.877000000000001,
-0.876000000000001,-0.875000000000001,-0.874000000000001,-0.873000000000001,
-0.872000000000001,-0.871000000000001,-0.870000000000001,-0.869000000000001,
-0.868000000000001,-0.867000000000001,-0.866000000000001,-0.865000000000001,
-0.864000000000001,-0.863000000000001,-0.862000000000001,-0.861000000000001,
-0.860000000000001,-0.859000000000001,-0.858000000000001,-0.857000000000001,
-0.856000000000001,-0.855000000000001,-0.854000000000001,-0.853000000000001,
-0.852000000000001,-0.851000000000001,-0.850000000000001,-0.849000000000001,
-0.848000000000001,-0.847000000000001,-0.846000000000001,-0.845000000000001,
-0.844000000000001,-0.843000000000001,-0.842000000000001,-0.841000000000001,
-0.840000000000001,-0.839000000000001,-0.838000000000001,-0.837000000000001,
-0.836000000000001,-0.835000000000001,-0.834000000000001,-0.833000000000001,
-0.832000000000001,-0.831000000000001,-0.830000000000001,-0.829000000000001,
-0.828000000000001,-0.827000000000001,-0.826000000000001,-0.825000000000001,
-0.824000000000001,-0.823000000000001,-0.822000000000001,-0.821000000000001,
-0.820000000000001,-0.819000000000001,-0.818000000000001,-0.817000000000001,
-0.816000000000001,-0.815000000000001,-0.814000000000001,-0.813000000000001,
-0.812000000000001,-0.811000000000001,-0.810000000000001,-0.809000000000001,
-0.808000000000001,-0.807000000000001,-0.806000000000001,-0.805000000000001,
-0.804000000000001,-0.803000000000001,-0.802000000000001,-0.801000000000001,
-0.800000000000001,-0.799000000000001,-0.798000000000001,-0.797000000000001,
-0.796000000000001,-0.795000000000001,-0.794000000000001,-0.793000000000001,
-0.792000000000001,-0.791000000000001,-0.790000000000001,-0.789000000000001,
-0.788000000000001,-0.787000000000001,-0.786000000000001,-0.785000000000001,
-0.784000000000001,-0.783000000000001,-0.782000000000001,-0.781000000000001,
-0.780000000000001,-0.779000000000001,-0.778000000000001,-0.777000000000001,
-0.776000000000001,-0.775000000000001,-0.774000000000001,-0.773000000000001,
-0.772000000000001,-0.771000000000001,-0.770000000000001,-0.769000000000001,
-0.768000000000001,-0.767000000000001,-0.766000000000001,-0.765000000000001,
-0.764000000000001,-0.763000000000001,-0.762000000000001,-0.761000000000001,
-0.760000000000001,-0.759000000000001,-0.758000000000001,-0.757000000000001,
-0.756000000000001,-0.755000000000001,-0.754000000000001,-0.753000000000001,
-0.752000000000001,-0.751000000000001,-0.750000000000001,-0.749000000000001,
-0.748000000000001,-0.747000000000001,-0.746000000000001,-0.745000000000001,
-0.744000000000001,-0.743000000000001,-0.742000000000001,-0.741000000000001,
-0.740000000000001,-0.739000000000001,-0.738000000000001,-0.737000000000001,
-0.736000000000001,-0.735000000000001,-0.734000000000001,-0.733000000000001,
-0.732000000000001,-0.731000000000001,-0.730000000000001,-0.729000000000001,
-0.728000000000001,-0.727000000000001,-0.726000000000001,-0.725000000000001,
-0.724000000000001,-0.723000000000001,-0.722000000000001,-0.721000000000001,
-0.720000000000001,-0.719000000000001,-0.718000000000001,-0.717000000000001,
-0.716000000000001,-0.715000000000001,-0.714000000000001,-0.713000000000001,
-0.712000000000001,-0.711000000000001,-0.710000000000001,-0.709000000000001,
-0.708000000000001,-0.707000000000001,-0.706000000000001,-0.705000000000001,
-0.704000000000001,-0.703000000000001,-0.702000000000001,-0.701000000000001,
-0.700000000000001,-0.699000000000001,-0.698000000000001,-0.697000000000001,
-0.696000000000001,-0.695000000000001,-0.694000000000001,-0.693000000000001,
-0.692000000000001,-0.691000000000001,-0.690000000000001,-0.689000000000001,
-0.688000000000001,-0.687,-0.686,-0.685,-0.684,-0.683,-0.682,-0.681,-0.68,
-0.679,-0.678,-0.677,-0.676,-0.675,-0.674,-0.673,-0.672,-0.671,-0.67,-0.669,
-0.668,-0.667,-0.666,-0.665,-0.664,-0.663,-0.662,-0.661,-0.66,-0.659,-0.658,
-0.657,-0.656,-0.655,-0.654,-0.653,-0.652,-0.651,-0.65,-0.649,-0.648,-0.647,
-0.646,-0.645,-0.644,-0.643,-0.642,-0.641,-0.64,-0.639,-0.638,-0.637,-0.636,
-0.635,-0.634,-0.633,-0.632,-0.631,-0.63,-0.629,-0.628,-0.627,-0.626,-0.625,
-0.624,-0.623,-0.622,-0.621,-0.62,-0.619,-0.618,-0.617,-0.616,-0.615,-0.614,
-0.613,-0.612,-0.611,-0.61,-0.609,-0.608,-0.607,-0.606,-0.605,-0.604,-0.603,
-0.602,-0.601,-0.6,-0.599,-0.598,-0.597,-0.596,-0.595,-0.594,-0.593,-0.592,
-0.591,-0.59,-0.589,-0.588,-0.587,-0.586,-0.585,-0.584,-0.583,-0.582,-0.581,
-0.58,-0.579,-0.578,-0.577,-0.576,-0.575,-0.574,-0.573,-0.572,-0.571,-0.57,
-0.569,-0.568,-0.567,-0.566,-0.565,-0.564,-0.563,-0.562,-0.561,-0.56,-0.559,
-0.558,-0.557,-0.556,-0.555,-0.554,-0.553,-0.552,-0.551,-0.55,-0.549,-0.548,
-0.547,-0.546,-0.545,-0.544,-0.543,-0.542,-0.541,-0.54,-0.539,-0.538,-0.537,
-0.536,-0.535,-0.534,-0.533,-0.532,-0.531,-0.53,-0.529,-0.528,-0.527,-0.526,
-0.525,-0.524,-0.523,-0.522,-0.521,-0.52,-0.519,-0.518,-0.517,-0.516,-0.515,
-0.514,-0.513,-0.512,-0.511,-0.51,-0.509,-0.508,-0.507,-0.506,-0.505,-0.504,
-0.503,-0.502,-0.501,-0.5,-0.499,-0.498,-0.497,-0.496,-0.495,-0.494,-0.493,
-0.492,-0.491,-0.49,-0.489,-0.488,-0.487,-0.486,-0.485,-0.484,-0.483,-0.482,
-0.481,-0.48,-0.479,-0.478,-0.477,-0.476,-0.475,-0.474,-0.473,-0.472,-0.471,
-0.47,-0.469,-0.468,-0.467,-0.466,-0.465,-0.464,-0.463,-0.462,-0.461,-0.46,
-0.459,-0.458,-0.457,-0.456,-0.455,-0.454,-0.453,-0.452,-0.451,-0.45,-0.449,
-0.448,-0.447,-0.446,-0.445,-0.444,-0.443,-0.442,-0.441,-0.44,-0.439,-0.438,
-0.437,-0.436,-0.435,-0.434,-0.433,-0.432,-0.431,-0.43,-0.429,-0.428,-0.427,
-0.426,-0.425,-0.424,-0.423,-0.422,-0.421,-0.42,-0.419,-0.418,-0.417,-0.416,
-0.415,-0.414,-0.413,-0.412,-0.411,-0.41,-0.409,-0.408,-0.407,-0.406,-0.405,
-0.404,-0.403,-0.402,-0.401,-0.4,-0.399,-0.398,-0.397,-0.396,-0.395,-0.394,
-0.393,-0.392,-0.391,-0.39,-0.389,-0.388,-0.387,-0.386,-0.385,-0.384,-0.383,
-0.382,-0.381,-0.38,-0.379,-0.378,-0.377,-0.376,-0.375,-0.374,-0.373,-0.372,
-0.371,-0.37,-0.369,-0.368,-0.367,-0.366,-0.365,-0.364,-0.363,-0.362,-0.361,
-0.36,-0.359,-0.358,-0.357,-0.356,-0.355,-0.354,-0.353,-0.352,-0.351,-0.35,
-0.349,-0.348,-0.347,-0.346,-0.345,-0.344,-0.343,-0.342,-0.341,-0.34,-0.339,
-0.338,-0.337,-0.336,-0.335,-0.334,-0.333,-0.332,-0.331,-0.33,-0.329,-0.328,
-0.327,-0.326,-0.325,-0.324,-0.323,-0.322,-0.321,-0.32,-0.319,-0.318,-0.317,
-0.316,-0.315,-0.314,-0.313,-0.312,-0.311,-0.31,-0.309,-0.308,-0.307,-0.306,
-0.305,-0.304,-0.303,-0.302,-0.301,-0.3,-0.299,-0.298,-0.297,-0.296,-0.295,
-0.294,-0.293,-0.292,-0.291,-0.29,-0.289,-0.288,-0.287,-0.286,-0.285,-0.284,
-0.283,-0.282,-0.281,-0.28,-0.279,-0.278,-0.277,-0.276,-0.275,-0.274,-0.273,
-0.272,-0.271,-0.27,-0.269,-0.268,-0.267,-0.266,-0.265,-0.264,-0.263,-0.262,
-0.261,-0.26,-0.259,-0.258,-0.257,-0.256,-0.255,-0.254,-0.253,-0.252,-0.251,
-0.25,-0.249,-0.248,-0.247,-0.246,-0.245,-0.244,-0.243,-0.242,-0.241,-0.24,
-0.239,-0.238,-0.237,-0.236,-0.235,-0.234,-0.233,-0.232,-0.231,-0.23,-0.229,
-0.228,-0.227,-0.226,-0.225,-0.224,-0.223,-0.222,-0.221,-0.22,-0.219,-0.218,
-0.217,-0.216,-0.215,-0.214,-0.213,-0.212,-0.211,-0.21,-0.209,-0.208,-0.207,
-0.206,-0.205,-0.204,-0.203,-0.202,-0.201,-0.2,-0.199,-0.198,-0.197,-0.196,
-0.195,-0.194,-0.193,-0.192,-0.191,-0.19,-0.189,-0.188,-0.187,-0.186,-0.185,
-0.184,-0.183,-0.182,-0.181,-0.18,-0.179,-0.178,-0.177,-0.176,-0.175,-0.174,
-0.173,-0.172,-0.171,-0.17,-0.169,-0.168,-0.167,-0.166,-0.165,-0.164,-0.163,
-0.162,-0.161,-0.16,-0.159,-0.158,-0.157,-0.156,-0.155,-0.154,-0.153,-0.152,
-0.151,-0.15,-0.149,-0.148,-0.147,-0.146,-0.145,-0.144,-0.143,-0.142,-0.141,
-0.14,-0.139,-0.138,-0.137,-0.136,-0.135,-0.134,-0.133,-0.132,-0.131,-0.13,
-0.129,-0.128,-0.127,-0.126,-0.125,-0.124,-0.123,-0.122,-0.121,-0.12,-0.119,
-0.118,-0.117,-0.116,-0.115,-0.114,-0.113,-0.112,-0.111,-0.11,-0.109,-0.108,
-0.107,-0.106,-0.105,-0.104,-0.103,-0.102,-0.101,-0.1,-0.0990000000000001,
-0.0980000000000001,-0.0970000000000001,-0.0960000000000001,-0.0950000000000001,
-0.0940000000000001,-0.0930000000000001,-0.0920000000000001,-0.0910000000000001,
-0.0900000000000001,-0.0890000000000001,-0.0880000000000001,-0.0870000000000001,
-0.0860000000000001,-0.0850000000000001,-0.0840000000000001,-0.0830000000000001,
-0.0820000000000001,-0.0810000000000001,-0.0800000000000001,-0.0790000000000001,
-0.0780000000000001,-0.0770000000000001,-0.0760000000000001,-0.0750000000000001,
-0.0740000000000001,-0.0730000000000001,-0.0720000000000001,-0.071,-0.07,
-0.069,-0.068,-0.067,-0.066,-0.065,-0.064,-0.063,-0.062,-0.061,-0.06,-0.059,
-0.058,-0.057,-0.056,-0.055,-0.054,-0.053,-0.052,-0.051,-0.05,-0.049,-0.048,
-0.047,-0.046,-0.045,-0.044,-0.043,-0.042,-0.041,-0.04,-0.039,-0.038,-0.037,
-0.036,-0.035,-0.034,-0.033,-0.032,-0.031,-0.03,-0.029,-0.028,-0.027,-0.026,
-0.025,-0.024,-0.023,-0.022,-0.021,-0.02,-0.019,-0.018,-0.017,-0.016,-0.015,
-0.014,-0.013,-0.012,-0.011,-0.01,-0.009,-0.008,-0.007,-0.006,-0.005,-0.004,
-0.003,-0.002,-0.001,0.),(0.,2.),.UNSPECIFIED.)
GEOMETRIC_REPRESENTATION_ITEM()
RATIONAL_B_SPLINE_SURFACE(((1.,1.),(1.,1.),(1.,1.),(1.,1.),(1.,1.),(1.,
1.),(1.,1.),(1.,1.),(1.,1.),(1.,1.),(1.,1.),(1.,1.),(1.,1.),(1.,1.),(1.,
1.),(1.,1.),(1.,1.),(1.,1.),(1.,1.),(1.,1.),(1.,1.),(1.,1.),(1.,1.),(1.,
1.),(1.,1.),(1.,1.),(1.,1.),(1.,1.),(1.,1.),(1.,1.),(1.,1.),(1.,1.),(1.,
1.),(1.,1.),(1.,1.),(1.,1.),(1.,1.),(1.,1.),(1.,1.),(1.,1.),(1.,1.),(1.,
1.),(1.,1.),(1.,1.),(1.,1.),(1.,1.),(1.,1.),(1.,1.),(1.,1.),(1.,1.),(1.,
1.),(1.,1.),(1.,1.),(1.,1.),(1.,1.),(1.,1.),(1.,1.),(1.,1.),(1.,1.),(1.,
1.),(1.,1.),(1.,1.),(1.,1.),(1.,1.),(1.,1.),(1.,1.),(1.,1.),(1.,1.),(1.,
1.),(1.,1.),(1.,1.),(1.,1.),(1.,1.),(1.,1.),(1.,1.),(1.,1.),(1.,1.),(1.,
1.),(1.,1.),(1.,1.),(1.,1.),(1.,1.),(1.,1.),(1.,1.),(1.,1.),(1.,1.),(1.,
1.),(1.,1.),(1.,1.),(1.,1.),(1.,1.),(1.,1.),(1.,1.),(1.,1.),(1.,1.),(1.,
1.),(1.,1.),(1.,1.),(1.,1.),(1.,1.),(1.,1.),(1.,1.),(1.,1.),(1.,1.),(1.,
1.),(1.,1.),(1.,1.),(1.,1.),(1.,1.),(1.,1.),(1.,1.),(1.,1.),(1.,1.),(1.,
1.),(1.,1.),(1.,1.),(1.,1.),(1.,1.),(1.,1.),(1.,1.),(1.,1.),(1.,1.),(1.,
1.),(1.,1.),(1.,1.),(1.,1.),(1.,1.),(1.,1.),(1.,1.),(1.,1.),(1.,1.),(1.,
1.),(1.,1.),(1.,1.),(1.,1.),(1.,1.),(1.,1.),(1.,1.),(1.,1.),(1.,1.),(1.,
1.),(1.,1.),(1.,1.),(1.,1.),(1.,1.),(1.,1.),(1.,1.),(1.,1.),(1.,1.),(1.,
1.),(1.,1.),(1.,1.),(1.,1.),(1.,1.),(1.,1.),(1.,1.),(1.,1.),(1.,1.),(1.,
1.),(1.,1.),(1.,1.),(1.,1.),(1.,1.),(1.,1.),(1.,1.),(1.,1.),(1.,1.),(1.,
1.),(1.,1.),(1.,1.),(1.,1.),(1.,1.),(1.,1.),(1.,1.),(1.,1.),(1.,1.),(1.,
1.),(1.,1.),(1.,1.),(1.,1.),(1.,1.),(1.,1.),(1.,1.),(1.,1.),(1.,1.),(1.,
1.),(1.,1.),(1.,1.),(1.,1.),(1.,1.),(1.,1.),(1.,1.),(1.,1.),(1.,1.),(1.,
1.),(1.,1.),(1.,1.),(1.,1.),(1.,1.),(1.,1.),(1.,1.),(1.,1.),(1.,1.),(1.,
1.),(1.,1.),(1.,1.),(1.,1.),(1.,1.),(1.,1.),(1.,1.),(1.,1.),(1.,1.),(1.,
1.),(1.,1.),(1.,1.),(1.,1.),(1.,1.),(1.,1.),(1.,1.),(1.,1.),(1.,1.),(1.,
1.),(1.,1.),(1.,1.),(1.,1.),(1.,1.),(1.,1.),(1.,1.),(1.,1.),(1.,1.),(1.,
1.),(1.,1.),(1.,1.),(1.,1.),(1.,1.),(1.,1.),(1.,1.),(1.,1.),(1.,1.),(1.,
1.),(1.,1.),(1.,1.),(1.,1.),(1.,1.),(1.,1.),(1.,1.),(1.,1.),(1.,1.),(1.,
1.),(1.,1.),(1.,1.),(1.,1.),(1.,1.),(1.,1.),(1.,1.),(1.,1.),(1.,1.),(1.,
1.),(1.,1.),(1.,1.),(1.,1.),(1.,1.),(1.,1.),(1.,1.),(1.,1.),(1.,1.),(1.,
1.),(1.,1.),(1.,1.),(1.,1.),(1.,1.),(1.,1.),(1.,1.),(1.,1.),(1.,1.),(1.,
1.),(1.,1.),(1.,1.),(1.,1.),(1.,1.),(1.,1.),(1.,1.),(1.,1.),(1.,1.),(1.,
1.),(1.,1.),(1.,1.),(1.,1.),(1.,1.),(1.,1.),(1.,1.),(1.,1.),(1.,1.),(1.,
1.),(1.,1.),(1.,1.),(1.,1.),(1.,1.),(1.,1.),(1.,1.),(1.,1.),(1.,1.),(1.,
1.),(1.,1.),(1.,1.),(1.,1.),(1.,1.),(1.,1.),(1.,1.),(1.,1.),(1.,1.),(1.,
1.),(1.,1.),(1.,1.),(1.,1.),(1.,1.),(1.,1.),(1.,1.),(1.,1.),(1.,1.),(1.,
1.),(1.,1.),(1.,1.),(1.,1.),(1.,1.),(1.,1.),(1.,1.),(1.,1.),(1.,1.),(1.,
1.),(1.,1.),(1.,1.),(1.,1.),(1.,1.),(1.,1.),(1.,1.),(1.,1.),(1.,1.),(1.,
1.),(1.,1.),(1.,1.),(1.,1.),(1.,1.),(1.,1.),(1.,1.),(1.,1.),(1.,1.),(1.,
1.),(1.,1.),(1.,1.),(1.,1.),(1.,1.),(1.,1.),(1.,1.),(1.,1.),(1.,1.),(1.,
1.),(1.,1.),(1.,1.),(1.,1.),(1.,1.),(1.,1.),(1.,1.),(1.,1.),(1.,1.),(1.,
1.),(1.,1.),(1.,1.),(1.,1.),(1.,1.),(1.,1.),(1.,1.),(1.,1.),(1.,1.),(1.,
1.),(1.,1.),(1.,1.),(1.,1.),(1.,1.),(1.,1.),(1.,1.),(1.,1.),(1.,1.),(1.,
1.),(1.,1.),(1.,1.),(1.,1.),(1.,1.),(1.,1.),(1.,1.),(1.,1.),(1.,1.),(1.,
1.),(1.,1.),(1.,1.),(1.,1.),(1.,1.),(1.,1.),(1.,1.),(1.,1.),(1.,1.),(1.,
1.),(1.,1.),(1.,1.),(1.,1.),(1.,1.),(1.,1.),(1.,1.),(1.,1.),(1.,1.),(1.,
1.),(1.,1.),(1.,1.),(1.,1.),(1.,1.),(1.,1.),(1.,1.),(1.,1.),(1.,1.),(1.,
1.),(1.,1.),(1.,1.),(1.,1.),(1.,1.),(1.,1.),(1.,1.),(1.,1.),(1.,1.),(1.,
1.),(1.,1.),(1.,1.),(1.,1.),(1.,1.),(1.,1.),(1.,1.),(1.,1.),(1.,1.),(1.,
1.),(1.,1.),(1.,1.),(1.,1.),(1.,1.),(1.,1.),(1.,1.),(1.,1.),(1.,1.),(1.,
1.),(1.,1.),(1.,1.),(1.,1.),(1.,1.),(1.,1.),(1.,1.),(1.,1.),(1.,1.),(1.,
1.),(1.,1.),(1.,1.),(1.,1.),(1.,1.),(1.,1.),(1.,1.),(1.,1.),(1.,1.),(1.,
1.),(1.,1.),(1.,1.),(1.,1.),(1.,1.),(1.,1.),(1.,1.),(1.,1.),(1.,1.),(1.,
1.),(1.,1.),(1.,1.),(1.,1.),(1.,1.),(1.,1.),(1.,1.),(1.,1.),(1.,1.),(1.,
1.),(1.,1.),(1.,1.),(1.,1.),(1.,1.),(1.,1.),(1.,1.),(1.,1.),(1.,1.),(1.,
1.),(1.,1.),(1.,1.),(1.,1.),(1.,1.),(1.,1.),(1.,1.),(1.,1.),(1.,1.),(1.,
1.),(1.,1.),(1.,1.),(1.,1.),(1.,1.),(1.,1.),(1.,1.),(1.,1.),(1.,1.),(1.,
1.),(1.,1.),(1.,1.),(1.,1.),(1.,1.),(1.,1.),(1.,1.),(1.,1.),(1.,1.),(1.,
1.),(1.,1.),(1.,1.),(1.,1.),(1.,1.),(1.,1.),(1.,1.),(1.,1.),(1.,1.),(1.,
1.),(1.,1.),(1.,1.),(1.,1.),(1.,1.),(1.,1.),(1.,1.),(1.,1.),(1.,1.),(1.,
1.),(1.,1.),(1.,1.),(1.,1.),(1.,1.),(1.,1.),(1.,1.),(1.,1.),(1.,1.),(1.,
1.),(1.,1.),(1.,1.),(1.,1.),(1.,1.),(1.,1.),(1.,1.),(1.,1.),(1.,1.),(1.,
1.),(1.,1.),(1.,1.),(1.,1.),(1.,1.),(1.,1.),(1.,1.),(1.,1.),(1.,1.),(1.,
1.),(1.,1.),(1.,1.),(1.,1.),(1.,1.),(1.,1.),(1.,1.),(1.,1.),(1.,1.),(1.,
1.),(1.,1.),(1.,1.),(1.,1.),(1.,1.),(1.,1.),(1.,1.),(1.,1.),(1.,1.),(1.,
1.),(1.,1.),(1.,1.),(1.,1.),(1.,1.),(1.,1.),(1.,1.),(1.,1.),(1.,1.),(1.,
1.),(1.,1.),(1.,1.),(1.,1.),(1.,1.),(1.,1.),(1.,1.),(1.,1.),(1.,1.),(1.,
1.),(1.,1.),(1.,1.),(1.,1.),(1.,1.),(1.,1.),(1.,1.),(1.,1.),(1.,1.),(1.,
1.),(1.,1.),(1.,1.),(1.,1.),(1.,1.),(1.,1.),(1.,1.),(1.,1.),(1.,1.),(1.,
1.),(1.,1.),(1.,1.),(1.,1.),(1.,1.),(1.,1.),(1.,1.),(1.,1.),(1.,1.),(1.,
1.),(1.,1.),(1.,1.),(1.,1.),(1.,1.),(1.,1.),(1.,1.),(1.,1.),(1.,1.),(1.,
1.),(1.,1.),(1.,1.),(1.,1.),(1.,1.),(1.,1.),(1.,1.),(1.,1.),(1.,1.),(1.,
1.),(1.,1.),(1.,1.),(1.,1.),(1.,1.),(1.,1.),(1.,1.),(1.,1.),(1.,1.),(1.,
1.),(1.,1.),(1.,1.),(1.,1.),(1.,1.),(1.,1.),(1.,1.),(1.,1.),(1.,1.),(1.,
1.),(1.,1.),(1.,1.),(1.,1.),(1.,1.),(1.,1.),(1.,1.),(1.,1.),(1.,1.),(1.,
1.),(1.,1.),(1.,1.),(1.,1.),(1.,1.),(1.,1.),(1.,1.),(1.,1.),(1.,1.),(1.,
1.),(1.,1.),(1.,1.),(1.,1.),(1.,1.),(1.,1.),(1.,1.),(1.,1.),(1.,1.),(1.,
1.),(1.,1.),(1.,1.),(1.,1.),(1.,1.),(1.,1.),(1.,1.),(1.,1.),(1.,1.),(1.,
1.),(1.,1.),(1.,1.),(1.,1.),(1.,1.),(1.,1.),(1.,1.),(1.,1.),(1.,1.),(1.,
1.),(1.,1.),(1.,1.),(1.,1.),(1.,1.),(1.,1.),(1.,1.),(1.,1.),(1.,1.),(1.,
1.),(1.,1.),(1.,1.),(1.,1.),(1.,1.),(1.,1.),(1.,1.),(1.,1.),(1.,1.),(1.,
1.),(1.,1.),(1.,1.),(1.,1.),(1.,1.),(1.,1.),(1.,1.),(1.,1.),(1.,1.),(1.,
1.),(1.,1.),(1.,1.),(1.,1.),(1.,1.),(1.,1.),(1.,1.),(1.,1.),(1.,1.),(1.,
1.),(1.,1.),(1.,1.),(1.,1.),(1.,1.),(1.,1.),(1.,1.),(1.,1.),(1.,1.),(1.,
1.),(1.,1.),(1.,1.),(1.,1.),(1.,1.),(1.,1.),(1.,1.),(1.,1.),(1.,1.),(1.,
1.),(1.,1.),(1.,1.),(1.,1.),(1.,1.),(1.,1.),(1.,1.),(1.,1.),(1.,1.),(1.,
1.),(1.,1.),(1.,1.),(1.,1.),(1.,1.),(1.,1.),(1.,1.),(1.,1.),(1.,1.),(1.,
1.),(1.,1.),(1.,1.),(1.,1.),(1.,1.),(1.,1.),(1.,1.),(1.,1.),(1.,1.),(1.,
1.),(1.,1.),(1.,1.),(1.,1.),(1.,1.),(1.,1.),(1.,1.),(1.,1.),(1.,1.),(1.,
1.),(1.,1.),(1.,1.),(1.,1.),(1.,1.),(1.,1.),(1.,1.),(1.,1.),(1.,1.),(1.,
1.),(1.,1.),(1.,1.),(1.,1.),(1.,1.),(1.,1.),(1.,1.),(1.,1.),(1.,1.),(1.,
1.),(1.,1.),(1.,1.),(1.,1.),(1.,1.),(1.,1.),(1.,1.),(1.,1.),(1.,1.),(1.,
1.),(1.,1.),(1.,1.),(1.,1.),(1.,1.),(1.,1.),(1.,1.),(1.,1.),(1.,1.),(1.,
1.),(1.,1.),(1.,1.),(1.,1.),(1.,1.),(1.,1.),(1.,1.),(1.,1.),(1.,1.),(1.,
1.),(1.,1.),(1.,1.),(1.,1.),(1.,1.),(1.,1.),(1.,1.),(1.,1.),(1.,1.),(1.,
1.),(1.,1.),(1.,1.),(1.,1.),(1.,1.),(1.,1.),(1.,1.),(1.,1.),(1.,1.),(1.,
1.),(1.,1.),(1.,1.),(1.,1.),(1.,1.),(1.,1.),(1.,1.),(1.,1.),(1.,1.),(1.,
1.),(1.,1.),(1.,1.),(1.,1.),(1.,1.),(1.,1.),(1.,1.),(1.,1.),(1.,1.),(1.,
1.),(1.,1.),(1.,1.),(1.,1.),(1.,1.),(1.,1.),(1.,1.),(1.,1.),(1.,1.),(1.,
1.),(1.,1.),(1.,1.),(1.,1.),(1.,1.),(1.,1.),(1.,1.),(1.,1.),(1.,1.),(1.,
1.),(1.,1.),(1.,1.),(1.,1.),(1.,1.),(1.,1.),(1.,1.),(1.,1.),(1.,1.),(1.,
1.),(1.,1.),(1.,1.),(1.,1.),(1.,1.),(1.,1.),(1.,1.),(1.,1.),(1.,1.),(1.,
1.),(1.,1.),(1.,1.),(1.,1.),(1.,1.),(1.,1.),(1.,1.),(1.,1.),(1.,1.),(1.,
1.),(1.,1.),(1.,1.),(1.,1.),(1.,1.),(1.,1.),(1.,1.),(1.,1.),(1.,1.),(1.,
1.),(1.,1.),(1.,1.),(1.,1.),(1.,1.),(1.,1.),(1.,1.),(1.,1.),(1.,1.),(1.,
1.),(1.,1.),(1.,1.),(1.,1.),(1.,1.),(1.,1.),(1.,1.),(1.,1.),(1.,1.),(1.,
1.),(1.,1.),(1.,1.),(1.,1.),(1.,1.),(1.,1.),(1.,1.),(1.,1.),(1.,1.),(1.,
1.),(1.,1.),(1.,1.),(1.,1.),(1.,1.),(1.,1.),(1.,1.),(1.,1.),(1.,1.),(1.,
1.),(1.,1.),(1.,1.),(1.,1.),(1.,1.),(1.,1.),(1.,1.),(1.,1.),(1.,1.),(1.,
1.),(1.,1.),(1.,1.),(1.,1.),(1.,1.),(1.,1.),(1.,1.),(1.,1.),(1.,1.),(1.,
1.),(1.,1.),(1.,1.),(1.,1.),(1.,1.),(1.,1.),(1.,1.),(1.,1.),(1.,1.),(1.,
1.),(1.,1.),(1.,1.),(1.,1.),(1.,1.),(1.,1.),(1.,1.),(1.,1.),(1.,1.),(1.,
1.)))
REPRESENTATION_ITEM('')
SURFACE()
);
#260=(
BOUNDED_SURFACE()
B_SPLINE_SURFACE(5,1,((#78157,#78158),(#78159,#78160),(#78161,#78162),(#78163,
#78164),(#78165,#78166),(#78167,#78168),(#78169,#78170),(#78171,#78172),
(#78173,#78174),(#78175,#78176),(#78177,#78178),(#78179,#78180),(#78181,
#78182),(#78183,#78184),(#78185,#78186),(#78187,#78188),(#78189,#78190),
(#78191,#78192),(#78193,#78194),(#78195,#78196),(#78197,#78198),(#78199,
#78200),(#78201,#78202),(#78203,#78204),(#78205,#78206),(#78207,#78208),
(#78209,#78210),(#78211,#78212),(#78213,#78214),(#78215,#78216),(#78217,
#78218),(#78219,#78220),(#78221,#78222),(#78223,#78224),(#78225,#78226),
(#78227,#78228),(#78229,#78230),(#78231,#78232),(#78233,#78234),(#78235,
#78236),(#78237,#78238),(#78239,#78240),(#78241,#78242),(#78243,#78244),
(#78245,#78246),(#78247,#78248),(#78249,#78250),(#78251,#78252),(#78253,
#78254),(#78255,#78256),(#78257,#78258),(#78259,#78260),(#78261,#78262),
(#78263,#78264),(#78265,#78266),(#78267,#78268),(#78269,#78270),(#78271,
#78272),(#78273,#78274),(#78275,#78276),(#78277,#78278),(#78279,#78280),
(#78281,#78282),(#78283,#78284),(#78285,#78286),(#78287,#78288),(#78289,
#78290),(#78291,#78292),(#78293,#78294),(#78295,#78296),(#78297,#78298),
(#78299,#78300),(#78301,#78302),(#78303,#78304),(#78305,#78306),(#78307,
#78308),(#78309,#78310),(#78311,#78312),(#78313,#78314),(#78315,#78316),
(#78317,#78318),(#78319,#78320),(#78321,#78322),(#78323,#78324),(#78325,
#78326),(#78327,#78328),(#78329,#78330),(#78331,#78332),(#78333,#78334),
(#78335,#78336),(#78337,#78338),(#78339,#78340),(#78341,#78342),(#78343,
#78344),(#78345,#78346),(#78347,#78348),(#78349,#78350),(#78351,#78352),
(#78353,#78354),(#78355,#78356),(#78357,#78358),(#78359,#78360),(#78361,
#78362),(#78363,#78364),(#78365,#78366),(#78367,#78368),(#78369,#78370),
(#78371,#78372),(#78373,#78374),(#78375,#78376),(#78377,#78378),(#78379,
#78380),(#78381,#78382),(#78383,#78384),(#78385,#78386),(#78387,#78388),
(#78389,#78390),(#78391,#78392),(#78393,#78394),(#78395,#78396),(#78397,
#78398),(#78399,#78400),(#78401,#78402),(#78403,#78404),(#78405,#78406),
(#78407,#78408),(#78409,#78410),(#78411,#78412),(#78413,#78414),(#78415,
#78416),(#78417,#78418),(#78419,#78420),(#78421,#78422),(#78423,#78424),
(#78425,#78426),(#78427,#78428),(#78429,#78430),(#78431,#78432),(#78433,
#78434),(#78435,#78436),(#78437,#78438),(#78439,#78440),(#78441,#78442),
(#78443,#78444),(#78445,#78446),(#78447,#78448),(#78449,#78450),(#78451,
#78452),(#78453,#78454),(#78455,#78456),(#78457,#78458),(#78459,#78460),
(#78461,#78462),(#78463,#78464),(#78465,#78466),(#78467,#78468),(#78469,
#78470),(#78471,#78472),(#78473,#78474),(#78475,#78476),(#78477,#78478),
(#78479,#78480),(#78481,#78482),(#78483,#78484),(#78485,#78486),(#78487,
#78488),(#78489,#78490),(#78491,#78492),(#78493,#78494),(#78495,#78496),
(#78497,#78498),(#78499,#78500),(#78501,#78502),(#78503,#78504),(#78505,
#78506),(#78507,#78508),(#78509,#78510),(#78511,#78512),(#78513,#78514),
(#78515,#78516),(#78517,#78518),(#78519,#78520),(#78521,#78522),(#78523,
#78524),(#78525,#78526),(#78527,#78528),(#78529,#78530),(#78531,#78532),
(#78533,#78534),(#78535,#78536),(#78537,#78538),(#78539,#78540),(#78541,
#78542),(#78543,#78544),(#78545,#78546),(#78547,#78548),(#78549,#78550),
(#78551,#78552),(#78553,#78554),(#78555,#78556),(#78557,#78558),(#78559,
#78560),(#78561,#78562),(#78563,#78564),(#78565,#78566),(#78567,#78568),
(#78569,#78570),(#78571,#78572),(#78573,#78574),(#78575,#78576),(#78577,
#78578),(#78579,#78580),(#78581,#78582),(#78583,#78584),(#78585,#78586),
(#78587,#78588),(#78589,#78590),(#78591,#78592),(#78593,#78594),(#78595,
#78596),(#78597,#78598),(#78599,#78600),(#78601,#78602),(#78603,#78604),
(#78605,#78606),(#78607,#78608),(#78609,#78610),(#78611,#78612),(#78613,
#78614),(#78615,#78616),(#78617,#78618),(#78619,#78620),(#78621,#78622),
(#78623,#78624),(#78625,#78626),(#78627,#78628),(#78629,#78630),(#78631,
#78632),(#78633,#78634),(#78635,#78636),(#78637,#78638),(#78639,#78640),
(#78641,#78642),(#78643,#78644),(#78645,#78646),(#78647,#78648),(#78649,
#78650),(#78651,#78652),(#78653,#78654),(#78655,#78656),(#78657,#78658),
(#78659,#78660),(#78661,#78662),(#78663,#78664),(#78665,#78666),(#78667,
#78668),(#78669,#78670),(#78671,#78672),(#78673,#78674),(#78675,#78676),
(#78677,#78678),(#78679,#78680),(#78681,#78682),(#78683,#78684),(#78685,
#78686),(#78687,#78688),(#78689,#78690),(#78691,#78692),(#78693,#78694),
(#78695,#78696),(#78697,#78698),(#78699,#78700),(#78701,#78702),(#78703,
#78704),(#78705,#78706),(#78707,#78708),(#78709,#78710),(#78711,#78712),
(#78713,#78714),(#78715,#78716),(#78717,#78718),(#78719,#78720),(#78721,
#78722),(#78723,#78724),(#78725,#78726),(#78727,#78728),(#78729,#78730),
(#78731,#78732),(#78733,#78734),(#78735,#78736),(#78737,#78738),(#78739,
#78740),(#78741,#78742),(#78743,#78744),(#78745,#78746),(#78747,#78748),
(#78749,#78750),(#78751,#78752),(#78753,#78754),(#78755,#78756),(#78757,
#78758),(#78759,#78760),(#78761,#78762),(#78763,#78764),(#78765,#78766),
(#78767,#78768),(#78769,#78770),(#78771,#78772),(#78773,#78774),(#78775,
#78776),(#78777,#78778),(#78779,#78780),(#78781,#78782),(#78783,#78784),
(#78785,#78786),(#78787,#78788),(#78789,#78790),(#78791,#78792),(#78793,
#78794),(#78795,#78796),(#78797,#78798),(#78799,#78800),(#78801,#78802),
(#78803,#78804),(#78805,#78806),(#78807,#78808),(#78809,#78810),(#78811,
#78812),(#78813,#78814),(#78815,#78816),(#78817,#78818),(#78819,#78820),
(#78821,#78822),(#78823,#78824),(#78825,#78826),(#78827,#78828),(#78829,
#78830),(#78831,#78832),(#78833,#78834),(#78835,#78836),(#78837,#78838),
(#78839,#78840),(#78841,#78842),(#78843,#78844),(#78845,#78846),(#78847,
#78848),(#78849,#78850),(#78851,#78852),(#78853,#78854),(#78855,#78856),
(#78857,#78858),(#78859,#78860),(#78861,#78862),(#78863,#78864),(#78865,
#78866),(#78867,#78868),(#78869,#78870),(#78871,#78872),(#78873,#78874),
(#78875,#78876),(#78877,#78878),(#78879,#78880),(#78881,#78882),(#78883,
#78884),(#78885,#78886),(#78887,#78888),(#78889,#78890),(#78891,#78892),
(#78893,#78894),(#78895,#78896),(#78897,#78898),(#78899,#78900),(#78901,
#78902),(#78903,#78904),(#78905,#78906),(#78907,#78908),(#78909,#78910),
(#78911,#78912),(#78913,#78914),(#78915,#78916),(#78917,#78918),(#78919,
#78920),(#78921,#78922),(#78923,#78924),(#78925,#78926),(#78927,#78928),
(#78929,#78930),(#78931,#78932),(#78933,#78934),(#78935,#78936),(#78937,
#78938),(#78939,#78940),(#78941,#78942),(#78943,#78944),(#78945,#78946),
(#78947,#78948),(#78949,#78950),(#78951,#78952),(#78953,#78954),(#78955,
#78956),(#78957,#78958),(#78959,#78960),(#78961,#78962),(#78963,#78964),
(#78965,#78966),(#78967,#78968),(#78969,#78970),(#78971,#78972),(#78973,
#78974),(#78975,#78976),(#78977,#78978),(#78979,#78980),(#78981,#78982),
(#78983,#78984),(#78985,#78986),(#78987,#78988),(#78989,#78990),(#78991,
#78992),(#78993,#78994),(#78995,#78996),(#78997,#78998),(#78999,#79000),
(#79001,#79002),(#79003,#79004),(#79005,#79006),(#79007,#79008),(#79009,
#79010),(#79011,#79012),(#79013,#79014),(#79015,#79016),(#79017,#79018),
(#79019,#79020),(#79021,#79022),(#79023,#79024),(#79025,#79026),(#79027,
#79028),(#79029,#79030),(#79031,#79032),(#79033,#79034),(#79035,#79036),
(#79037,#79038),(#79039,#79040),(#79041,#79042),(#79043,#79044),(#79045,
#79046),(#79047,#79048),(#79049,#79050),(#79051,#79052),(#79053,#79054),
(#79055,#79056),(#79057,#79058),(#79059,#79060),(#79061,#79062),(#79063,
#79064),(#79065,#79066),(#79067,#79068),(#79069,#79070),(#79071,#79072),
(#79073,#79074),(#79075,#79076),(#79077,#79078),(#79079,#79080),(#79081,
#79082),(#79083,#79084),(#79085,#79086),(#79087,#79088),(#79089,#79090),
(#79091,#79092),(#79093,#79094),(#79095,#79096),(#79097,#79098),(#79099,
#79100),(#79101,#79102),(#79103,#79104),(#79105,#79106),(#79107,#79108),
(#79109,#79110),(#79111,#79112),(#79113,#79114),(#79115,#79116),(#79117,
#79118),(#79119,#79120),(#79121,#79122),(#79123,#79124),(#79125,#79126),
(#79127,#79128),(#79129,#79130),(#79131,#79132),(#79133,#79134),(#79135,
#79136),(#79137,#79138),(#79139,#79140),(#79141,#79142),(#79143,#79144),
(#79145,#79146),(#79147,#79148),(#79149,#79150),(#79151,#79152),(#79153,
#79154),(#79155,#79156),(#79157,#79158),(#79159,#79160),(#79161,#79162),
(#79163,#79164),(#79165,#79166),(#79167,#79168),(#79169,#79170),(#79171,
#79172),(#79173,#79174),(#79175,#79176),(#79177,#79178),(#79179,#79180),
(#79181,#79182),(#79183,#79184),(#79185,#79186),(#79187,#79188),(#79189,
#79190),(#79191,#79192),(#79193,#79194),(#79195,#79196),(#79197,#79198),
(#79199,#79200),(#79201,#79202),(#79203,#79204),(#79205,#79206),(#79207,
#79208),(#79209,#79210),(#79211,#79212),(#79213,#79214),(#79215,#79216),
(#79217,#79218),(#79219,#79220),(#79221,#79222),(#79223,#79224),(#79225,
#79226),(#79227,#79228),(#79229,#79230),(#79231,#79232),(#79233,#79234),
(#79235,#79236),(#79237,#79238),(#79239,#79240),(#79241,#79242),(#79243,
#79244),(#79245,#79246),(#79247,#79248),(#79249,#79250),(#79251,#79252),
(#79253,#79254),(#79255,#79256),(#79257,#79258),(#79259,#79260),(#79261,
#79262),(#79263,#79264),(#79265,#79266),(#79267,#79268),(#79269,#79270),
(#79271,#79272),(#79273,#79274),(#79275,#79276),(#79277,#79278),(#79279,
#79280),(#79281,#79282),(#79283,#79284),(#79285,#79286),(#79287,#79288),
(#79289,#79290),(#79291,#79292),(#79293,#79294),(#79295,#79296),(#79297,
#79298),(#79299,#79300),(#79301,#79302),(#79303,#79304),(#79305,#79306),
(#79307,#79308),(#79309,#79310),(#79311,#79312),(#79313,#79314),(#79315,
#79316),(#79317,#79318),(#79319,#79320),(#79321,#79322),(#79323,#79324),
(#79325,#79326),(#79327,#79328),(#79329,#79330),(#79331,#79332),(#79333,
#79334),(#79335,#79336),(#79337,#79338),(#79339,#79340),(#79341,#79342),
(#79343,#79344),(#79345,#79346),(#79347,#79348),(#79349,#79350),(#79351,
#79352),(#79353,#79354),(#79355,#79356),(#79357,#79358),(#79359,#79360),
(#79361,#79362),(#79363,#79364),(#79365,#79366),(#79367,#79368),(#79369,
#79370),(#79371,#79372),(#79373,#79374),(#79375,#79376),(#79377,#79378),
(#79379,#79380),(#79381,#79382),(#79383,#79384),(#79385,#79386),(#79387,
#79388),(#79389,#79390),(#79391,#79392),(#79393,#79394),(#79395,#79396),
(#79397,#79398),(#79399,#79400),(#79401,#79402),(#79403,#79404),(#79405,
#79406),(#79407,#79408),(#79409,#79410),(#79411,#79412),(#79413,#79414),
(#79415,#79416),(#79417,#79418),(#79419,#79420),(#79421,#79422),(#79423,
#79424),(#79425,#79426),(#79427,#79428),(#79429,#79430),(#79431,#79432),
(#79433,#79434),(#79435,#79436),(#79437,#79438),(#79439,#79440),(#79441,
#79442),(#79443,#79444),(#79445,#79446),(#79447,#79448),(#79449,#79450),
(#79451,#79452),(#79453,#79454),(#79455,#79456),(#79457,#79458),(#79459,
#79460),(#79461,#79462),(#79463,#79464),(#79465,#79466),(#79467,#79468),
(#79469,#79470),(#79471,#79472),(#79473,#79474),(#79475,#79476),(#79477,
#79478),(#79479,#79480),(#79481,#79482),(#79483,#79484),(#79485,#79486),
(#79487,#79488),(#79489,#79490),(#79491,#79492),(#79493,#79494),(#79495,
#79496),(#79497,#79498),(#79499,#79500),(#79501,#79502),(#79503,#79504),
(#79505,#79506),(#79507,#79508),(#79509,#79510),(#79511,#79512),(#79513,
#79514),(#79515,#79516),(#79517,#79518),(#79519,#79520),(#79521,#79522),
(#79523,#79524),(#79525,#79526),(#79527,#79528),(#79529,#79530),(#79531,
#79532),(#79533,#79534),(#79535,#79536),(#79537,#79538),(#79539,#79540),
(#79541,#79542),(#79543,#79544),(#79545,#79546),(#79547,#79548),(#79549,
#79550),(#79551,#79552),(#79553,#79554),(#79555,#79556),(#79557,#79558),
(#79559,#79560),(#79561,#79562),(#79563,#79564),(#79565,#79566),(#79567,
#79568),(#79569,#79570),(#79571,#79572),(#79573,#79574),(#79575,#79576),
(#79577,#79578),(#79579,#79580),(#79581,#79582),(#79583,#79584),(#79585,
#79586),(#79587,#79588),(#79589,#79590),(#79591,#79592),(#79593,#79594),
(#79595,#79596),(#79597,#79598),(#79599,#79600),(#79601,#79602),(#79603,
#79604),(#79605,#79606),(#79607,#79608),(#79609,#79610),(#79611,#79612),
(#79613,#79614),(#79615,#79616),(#79617,#79618),(#79619,#79620),(#79621,
#79622),(#79623,#79624),(#79625,#79626),(#79627,#79628),(#79629,#79630),
(#79631,#79632),(#79633,#79634),(#79635,#79636),(#79637,#79638),(#79639,
#79640),(#79641,#79642),(#79643,#79644),(#79645,#79646),(#79647,#79648),
(#79649,#79650),(#79651,#79652),(#79653,#79654),(#79655,#79656),(#79657,
#79658),(#79659,#79660),(#79661,#79662),(#79663,#79664),(#79665,#79666),
(#79667,#79668),(#79669,#79670),(#79671,#79672),(#79673,#79674),(#79675,
#79676),(#79677,#79678),(#79679,#79680),(#79681,#79682),(#79683,#79684),
(#79685,#79686),(#79687,#79688),(#79689,#79690),(#79691,#79692),(#79693,
#79694),(#79695,#79696),(#79697,#79698),(#79699,#79700),(#79701,#79702),
(#79703,#79704),(#79705,#79706),(#79707,#79708),(#79709,#79710),(#79711,
#79712),(#79713,#79714),(#79715,#79716),(#79717,#79718),(#79719,#79720),
(#79721,#79722),(#79723,#79724),(#79725,#79726),(#79727,#79728),(#79729,
#79730),(#79731,#79732),(#79733,#79734),(#79735,#79736),(#79737,#79738),
(#79739,#79740),(#79741,#79742),(#79743,#79744),(#79745,#79746),(#79747,
#79748),(#79749,#79750),(#79751,#79752),(#79753,#79754),(#79755,#79756),
(#79757,#79758),(#79759,#79760),(#79761,#79762),(#79763,#79764),(#79765,
#79766),(#79767,#79768),(#79769,#79770),(#79771,#79772),(#79773,#79774),
(#79775,#79776),(#79777,#79778),(#79779,#79780),(#79781,#79782),(#79783,
#79784),(#79785,#79786),(#79787,#79788),(#79789,#79790),(#79791,#79792),
(#79793,#79794),(#79795,#79796),(#79797,#79798),(#79799,#79800),(#79801,
#79802),(#79803,#79804),(#79805,#79806),(#79807,#79808),(#79809,#79810),
(#79811,#79812),(#79813,#79814),(#79815,#79816),(#79817,#79818),(#79819,
#79820),(#79821,#79822),(#79823,#79824),(#79825,#79826),(#79827,#79828),
(#79829,#79830),(#79831,#79832),(#79833,#79834),(#79835,#79836),(#79837,
#79838),(#79839,#79840),(#79841,#79842),(#79843,#79844),(#79845,#79846),
(#79847,#79848),(#79849,#79850),(#79851,#79852),(#79853,#79854),(#79855,
#79856),(#79857,#79858),(#79859,#79860),(#79861,#79862),(#79863,#79864),
(#79865,#79866),(#79867,#79868),(#79869,#79870),(#79871,#79872),(#79873,
#79874),(#79875,#79876),(#79877,#79878),(#79879,#79880),(#79881,#79882),
(#79883,#79884),(#79885,#79886),(#79887,#79888),(#79889,#79890),(#79891,
#79892),(#79893,#79894),(#79895,#79896),(#79897,#79898),(#79899,#79900),
(#79901,#79902),(#79903,#79904),(#79905,#79906),(#79907,#79908),(#79909,
#79910),(#79911,#79912),(#79913,#79914),(#79915,#79916),(#79917,#79918),
(#79919,#79920),(#79921,#79922),(#79923,#79924),(#79925,#79926),(#79927,
#79928),(#79929,#79930),(#79931,#79932),(#79933,#79934),(#79935,#79936),
(#79937,#79938),(#79939,#79940),(#79941,#79942),(#79943,#79944),(#79945,
#79946),(#79947,#79948),(#79949,#79950),(#79951,#79952),(#79953,#79954),
(#79955,#79956),(#79957,#79958),(#79959,#79960),(#79961,#79962),(#79963,
#79964),(#79965,#79966),(#79967,#79968),(#79969,#79970),(#79971,#79972),
(#79973,#79974),(#79975,#79976),(#79977,#79978),(#79979,#79980),(#79981,
#79982),(#79983,#79984),(#79985,#79986),(#79987,#79988),(#79989,#79990),
(#79991,#79992),(#79993,#79994),(#79995,#79996),(#79997,#79998),(#79999,
#80000),(#80001,#80002),(#80003,#80004),(#80005,#80006),(#80007,#80008),
(#80009,#80010),(#80011,#80012),(#80013,#80014),(#80015,#80016),(#80017,
#80018),(#80019,#80020),(#80021,#80022),(#80023,#80024),(#80025,#80026),
(#80027,#80028),(#80029,#80030),(#80031,#80032),(#80033,#80034),(#80035,
#80036),(#80037,#80038),(#80039,#80040),(#80041,#80042),(#80043,#80044),
(#80045,#80046),(#80047,#80048),(#80049,#80050),(#80051,#80052),(#80053,
#80054),(#80055,#80056),(#80057,#80058),(#80059,#80060),(#80061,#80062),
(#80063,#80064),(#80065,#80066),(#80067,#80068),(#80069,#80070),(#80071,
#80072),(#80073,#80074),(#80075,#80076),(#80077,#80078),(#80079,#80080),
(#80081,#80082),(#80083,#80084),(#80085,#80086),(#80087,#80088),(#80089,
#80090),(#80091,#80092),(#80093,#80094),(#80095,#80096),(#80097,#80098),
(#80099,#80100),(#80101,#80102),(#80103,#80104),(#80105,#80106),(#80107,
#80108),(#80109,#80110),(#80111,#80112),(#80113,#80114),(#80115,#80116),
(#80117,#80118),(#80119,#80120),(#80121,#80122),(#80123,#80124),(#80125,
#80126),(#80127,#80128),(#80129,#80130),(#80131,#80132),(#80133,#80134),
(#80135,#80136),(#80137,#80138),(#80139,#80140),(#80141,#80142),(#80143,
#80144),(#80145,#80146),(#80147,#80148),(#80149,#80150),(#80151,#80152),
(#80153,#80154),(#80155,#80156),(#80157,#80158),(#80159,#80160),(#80161,
#80162),(#80163,#80164),(#80165,#80166)),.UNSPECIFIED.,.F.,.F.,.F.)
B_SPLINE_SURFACE_WITH_KNOTS((6,1,1,1,1,1,1,1,1,1,1,1,1,1,1,1,1,1,1,1,1,
1,1,1,1,1,1,1,1,1,1,1,1,1,1,1,1,1,1,1,1,1,1,1,1,1,1,1,1,1,1,1,1,1,1,1,1,
1,1,1,1,1,1,1,1,1,1,1,1,1,1,1,1,1,1,1,1,1,1,1,1,1,1,1,1,1,1,1,1,1,1,1,1,
1,1,1,1,1,1,1,1,1,1,1,1,1,1,1,1,1,1,1,1,1,1,1,1,1,1,1,1,1,1,1,1,1,1,1,1,
1,1,1,1,1,1,1,1,1,1,1,1,1,1,1,1,1,1,1,1,1,1,1,1,1,1,1,1,1,1,1,1,1,1,1,1,
1,1,1,1,1,1,1,1,1,1,1,1,1,1,1,1,1,1,1,1,1,1,1,1,1,1,1,1,1,1,1,1,1,1,1,1,
1,1,1,1,1,1,1,1,1,1,1,1,1,1,1,1,1,1,1,1,1,1,1,1,1,1,1,1,1,1,1,1,1,1,1,1,
1,1,1,1,1,1,1,1,1,1,1,1,1,1,1,1,1,1,1,1,1,1,1,1,1,1,1,1,1,1,1,1,1,1,1,1,
1,1,1,1,1,1,1,1,1,1,1,1,1,1,1,1,1,1,1,1,1,1,1,1,1,1,1,1,1,1,1,1,1,1,1,1,
1,1,1,1,1,1,1,1,1,1,1,1,1,1,1,1,1,1,1,1,1,1,1,1,1,1,1,1,1,1,1,1,1,1,1,1,
1,1,1,1,1,1,1,1,1,1,1,1,1,1,1,1,1,1,1,1,1,1,1,1,1,1,1,1,1,1,1,1,1,1,1,1,
1,1,1,1,1,1,1,1,1,1,1,1,1,1,1,1,1,1,1,1,1,1,1,1,1,1,1,1,1,1,1,1,1,1,1,1,
1,1,1,1,1,1,1,1,1,1,1,1,1,1,1,1,1,1,1,1,1,1,1,1,1,1,1,1,1,1,1,1,1,1,1,1,
1,1,1,1,1,1,1,1,1,1,1,1,1,1,1,1,1,1,1,1,1,1,1,1,1,1,1,1,1,1,1,1,1,1,1,1,
1,1,1,1,1,1,1,1,1,1,1,1,1,1,1,1,1,1,1,1,1,1,1,1,1,1,1,1,1,1,1,1,1,1,1,1,
1,1,1,1,1,1,1,1,1,1,1,1,1,1,1,1,1,1,1,1,1,1,1,1,1,1,1,1,1,1,1,1,1,1,1,1,
1,1,1,1,1,1,1,1,1,1,1,1,1,1,1,1,1,1,1,1,1,1,1,1,1,1,1,1,1,1,1,1,1,1,1,1,
1,1,1,1,1,1,1,1,1,1,1,1,1,1,1,1,1,1,1,1,1,1,1,1,1,1,1,1,1,1,1,1,1,1,1,1,
1,1,1,1,1,1,1,1,1,1,1,1,1,1,1,1,1,1,1,1,1,1,1,1,1,1,1,1,1,1,1,1,1,1,1,1,
1,1,1,1,1,1,1,1,1,1,1,1,1,1,1,1,1,1,1,1,1,1,1,1,1,1,1,1,1,1,1,1,1,1,1,1,
1,1,1,1,1,1,1,1,1,1,1,1,1,1,1,1,1,1,1,1,1,1,1,1,1,1,1,1,1,1,1,1,1,1,1,1,
1,1,1,1,1,1,1,1,1,1,1,1,1,1,1,1,1,1,1,1,1,1,1,1,1,1,1,1,1,1,1,1,1,1,1,1,
1,1,1,1,1,1,1,1,1,1,1,1,1,1,1,1,1,1,1,1,1,1,1,1,1,1,1,1,1,1,1,1,1,1,1,1,
1,1,1,1,1,1,1,1,1,1,1,1,1,1,1,1,1,1,1,1,1,1,1,1,1,1,1,1,1,1,1,1,1,1,1,1,
1,1,1,1,1,1,1,1,1,1,1,1,1,1,1,1,1,1,1,1,1,1,1,1,1,1,1,1,1,1,1,1,1,1,1,1,
1,1,1,1,1,1,1,1,1,1,1,1,1,1,1,1,1,1,1,1,1,1,1,1,1,1,1,1,1,1,1,1,1,1,1,1,
1,1,1,1,1,1,1,1,1,1,1,1,1,1,1,1,1,1,1,1,1,1,1,1,1,1,1,1,1,1,1,1,1,1,1,1,
1,1,1,1,1,1,1,1,1,1,1,1,1,1,1,1,1,1,1,1,1,1,1,1,1,1,1,1,1,1,1,1,1,1,1,1,
1,1,1,1,1,1,1,6),(2,2),(-1.,-0.999000000000001,-0.998000000000001,-0.997000000000001,
-0.996000000000001,-0.995000000000001,-0.994000000000001,-0.993000000000001,
-0.992000000000001,-0.991000000000001,-0.990000000000001,-0.989000000000001,
-0.988000000000001,-0.987000000000001,-0.986000000000001,-0.985000000000001,
-0.984000000000001,-0.983000000000001,-0.982000000000001,-0.981000000000001,
-0.980000000000001,-0.979000000000001,-0.978000000000001,-0.977000000000001,
-0.976000000000001,-0.975000000000001,-0.974000000000001,-0.973000000000001,
-0.972000000000001,-0.971000000000001,-0.970000000000001,-0.969000000000001,
-0.968000000000001,-0.967000000000001,-0.966000000000001,-0.965000000000001,
-0.964000000000001,-0.963000000000001,-0.962000000000001,-0.961000000000001,
-0.960000000000001,-0.959000000000001,-0.958000000000001,-0.957000000000001,
-0.956000000000001,-0.955000000000001,-0.954000000000001,-0.953000000000001,
-0.952000000000001,-0.951000000000001,-0.950000000000001,-0.949000000000001,
-0.948000000000001,-0.947000000000001,-0.946000000000001,-0.945000000000001,
-0.944000000000001,-0.943000000000001,-0.942000000000001,-0.941000000000001,
-0.940000000000001,-0.939000000000001,-0.938000000000001,-0.937000000000001,
-0.936000000000001,-0.935000000000001,-0.934000000000001,-0.933000000000001,
-0.932000000000001,-0.931000000000001,-0.930000000000001,-0.929000000000001,
-0.928000000000001,-0.927000000000001,-0.926000000000001,-0.925000000000001,
-0.924000000000001,-0.923000000000001,-0.922000000000001,-0.921000000000001,
-0.920000000000001,-0.919000000000001,-0.918000000000001,-0.917000000000001,
-0.916000000000001,-0.915000000000001,-0.914000000000001,-0.913000000000001,
-0.912000000000001,-0.911000000000001,-0.910000000000001,-0.909000000000001,
-0.908000000000001,-0.907000000000001,-0.906000000000001,-0.905000000000001,
-0.904000000000001,-0.903000000000001,-0.902000000000001,-0.901000000000001,
-0.900000000000001,-0.899000000000001,-0.898000000000001,-0.897000000000001,
-0.896000000000001,-0.895000000000001,-0.894000000000001,-0.893000000000001,
-0.892000000000001,-0.891000000000001,-0.890000000000001,-0.889000000000001,
-0.888000000000001,-0.887000000000001,-0.886000000000001,-0.885000000000001,
-0.884000000000001,-0.883000000000001,-0.882000000000001,-0.881000000000001,
-0.880000000000001,-0.879000000000001,-0.878000000000001,-0.877000000000001,
-0.876000000000001,-0.875000000000001,-0.874000000000001,-0.873000000000001,
-0.872000000000001,-0.871000000000001,-0.870000000000001,-0.869000000000001,
-0.868000000000001,-0.867000000000001,-0.866000000000001,-0.865000000000001,
-0.864000000000001,-0.863000000000001,-0.862000000000001,-0.861000000000001,
-0.860000000000001,-0.859000000000001,-0.858000000000001,-0.857000000000001,
-0.856000000000001,-0.855000000000001,-0.854000000000001,-0.853000000000001,
-0.852000000000001,-0.851000000000001,-0.850000000000001,-0.849000000000001,
-0.848000000000001,-0.847000000000001,-0.846000000000001,-0.845000000000001,
-0.844000000000001,-0.843000000000001,-0.842000000000001,-0.841000000000001,
-0.840000000000001,-0.839000000000001,-0.838000000000001,-0.837000000000001,
-0.836000000000001,-0.835000000000001,-0.834000000000001,-0.833000000000001,
-0.832000000000001,-0.831000000000001,-0.830000000000001,-0.829000000000001,
-0.828000000000001,-0.827000000000001,-0.826000000000001,-0.825000000000001,
-0.824000000000001,-0.823000000000001,-0.822000000000001,-0.821000000000001,
-0.820000000000001,-0.819000000000001,-0.818000000000001,-0.817000000000001,
-0.816000000000001,-0.815000000000001,-0.814000000000001,-0.813000000000001,
-0.812000000000001,-0.811000000000001,-0.810000000000001,-0.809000000000001,
-0.808000000000001,-0.807000000000001,-0.806000000000001,-0.805000000000001,
-0.804000000000001,-0.803000000000001,-0.802000000000001,-0.801000000000001,
-0.800000000000001,-0.799000000000001,-0.798000000000001,-0.797000000000001,
-0.796000000000001,-0.795000000000001,-0.794000000000001,-0.793000000000001,
-0.792000000000001,-0.791000000000001,-0.790000000000001,-0.789000000000001,
-0.788000000000001,-0.787000000000001,-0.786000000000001,-0.785000000000001,
-0.784000000000001,-0.783000000000001,-0.782000000000001,-0.781000000000001,
-0.780000000000001,-0.779000000000001,-0.778000000000001,-0.777000000000001,
-0.776000000000001,-0.775000000000001,-0.774000000000001,-0.773000000000001,
-0.772000000000001,-0.771000000000001,-0.770000000000001,-0.769000000000001,
-0.768000000000001,-0.767000000000001,-0.766000000000001,-0.765000000000001,
-0.764000000000001,-0.763000000000001,-0.762000000000001,-0.761000000000001,
-0.760000000000001,-0.759000000000001,-0.758000000000001,-0.757000000000001,
-0.756000000000001,-0.755000000000001,-0.754000000000001,-0.753000000000001,
-0.752000000000001,-0.751000000000001,-0.750000000000001,-0.749000000000001,
-0.748000000000001,-0.747000000000001,-0.746000000000001,-0.745000000000001,
-0.744000000000001,-0.743000000000001,-0.742000000000001,-0.741000000000001,
-0.740000000000001,-0.739000000000001,-0.738000000000001,-0.737000000000001,
-0.736000000000001,-0.735000000000001,-0.734000000000001,-0.733000000000001,
-0.732000000000001,-0.731000000000001,-0.730000000000001,-0.729000000000001,
-0.728000000000001,-0.727000000000001,-0.726000000000001,-0.725000000000001,
-0.724000000000001,-0.723000000000001,-0.722000000000001,-0.721000000000001,
-0.720000000000001,-0.719000000000001,-0.718000000000001,-0.717000000000001,
-0.716000000000001,-0.715000000000001,-0.714000000000001,-0.713000000000001,
-0.712000000000001,-0.711000000000001,-0.710000000000001,-0.709000000000001,
-0.708000000000001,-0.707000000000001,-0.706000000000001,-0.705000000000001,
-0.704000000000001,-0.703000000000001,-0.702000000000001,-0.701000000000001,
-0.700000000000001,-0.699000000000001,-0.698000000000001,-0.697000000000001,
-0.696000000000001,-0.695000000000001,-0.694000000000001,-0.693000000000001,
-0.692000000000001,-0.691000000000001,-0.690000000000001,-0.689000000000001,
-0.688000000000001,-0.687,-0.686,-0.685,-0.684,-0.683,-0.682,-0.681,-0.68,
-0.679,-0.678,-0.677,-0.676,-0.675,-0.674,-0.673,-0.672,-0.671,-0.67,-0.669,
-0.668,-0.667,-0.666,-0.665,-0.664,-0.663,-0.662,-0.661,-0.66,-0.659,-0.658,
-0.657,-0.656,-0.655,-0.654,-0.653,-0.652,-0.651,-0.65,-0.649,-0.648,-0.647,
-0.646,-0.645,-0.644,-0.643,-0.642,-0.641,-0.64,-0.639,-0.638,-0.637,-0.636,
-0.635,-0.634,-0.633,-0.632,-0.631,-0.63,-0.629,-0.628,-0.627,-0.626,-0.625,
-0.624,-0.623,-0.622,-0.621,-0.62,-0.619,-0.618,-0.617,-0.616,-0.615,-0.614,
-0.613,-0.612,-0.611,-0.61,-0.609,-0.608,-0.607,-0.606,-0.605,-0.604,-0.603,
-0.602,-0.601,-0.6,-0.599,-0.598,-0.597,-0.596,-0.595,-0.594,-0.593,-0.592,
-0.591,-0.59,-0.589,-0.588,-0.587,-0.586,-0.585,-0.584,-0.583,-0.582,-0.581,
-0.58,-0.579,-0.578,-0.577,-0.576,-0.575,-0.574,-0.573,-0.572,-0.571,-0.57,
-0.569,-0.568,-0.567,-0.566,-0.565,-0.564,-0.563,-0.562,-0.561,-0.56,-0.559,
-0.558,-0.557,-0.556,-0.555,-0.554,-0.553,-0.552,-0.551,-0.55,-0.549,-0.548,
-0.547,-0.546,-0.545,-0.544,-0.543,-0.542,-0.541,-0.54,-0.539,-0.538,-0.537,
-0.536,-0.535,-0.534,-0.533,-0.532,-0.531,-0.53,-0.529,-0.528,-0.527,-0.526,
-0.525,-0.524,-0.523,-0.522,-0.521,-0.52,-0.519,-0.518,-0.517,-0.516,-0.515,
-0.514,-0.513,-0.512,-0.511,-0.51,-0.509,-0.508,-0.507,-0.506,-0.505,-0.504,
-0.503,-0.502,-0.501,-0.5,-0.499,-0.498,-0.497,-0.496,-0.495,-0.494,-0.493,
-0.492,-0.491,-0.49,-0.489,-0.488,-0.487,-0.486,-0.485,-0.484,-0.483,-0.482,
-0.481,-0.48,-0.479,-0.478,-0.477,-0.476,-0.475,-0.474,-0.473,-0.472,-0.471,
-0.47,-0.469,-0.468,-0.467,-0.466,-0.465,-0.464,-0.463,-0.462,-0.461,-0.46,
-0.459,-0.458,-0.457,-0.456,-0.455,-0.454,-0.453,-0.452,-0.451,-0.45,-0.449,
-0.448,-0.447,-0.446,-0.445,-0.444,-0.443,-0.442,-0.441,-0.44,-0.439,-0.438,
-0.437,-0.436,-0.435,-0.434,-0.433,-0.432,-0.431,-0.43,-0.429,-0.428,-0.427,
-0.426,-0.425,-0.424,-0.423,-0.422,-0.421,-0.42,-0.419,-0.418,-0.417,-0.416,
-0.415,-0.414,-0.413,-0.412,-0.411,-0.41,-0.409,-0.408,-0.407,-0.406,-0.405,
-0.404,-0.403,-0.402,-0.401,-0.4,-0.399,-0.398,-0.397,-0.396,-0.395,-0.394,
-0.393,-0.392,-0.391,-0.39,-0.389,-0.388,-0.387,-0.386,-0.385,-0.384,-0.383,
-0.382,-0.381,-0.38,-0.379,-0.378,-0.377,-0.376,-0.375,-0.374,-0.373,-0.372,
-0.371,-0.37,-0.369,-0.368,-0.367,-0.366,-0.365,-0.364,-0.363,-0.362,-0.361,
-0.36,-0.359,-0.358,-0.357,-0.356,-0.355,-0.354,-0.353,-0.352,-0.351,-0.35,
-0.349,-0.348,-0.347,-0.346,-0.345,-0.344,-0.343,-0.342,-0.341,-0.34,-0.339,
-0.338,-0.337,-0.336,-0.335,-0.334,-0.333,-0.332,-0.331,-0.33,-0.329,-0.328,
-0.327,-0.326,-0.325,-0.324,-0.323,-0.322,-0.321,-0.32,-0.319,-0.318,-0.317,
-0.316,-0.315,-0.314,-0.313,-0.312,-0.311,-0.31,-0.309,-0.308,-0.307,-0.306,
-0.305,-0.304,-0.303,-0.302,-0.301,-0.3,-0.299,-0.298,-0.297,-0.296,-0.295,
-0.294,-0.293,-0.292,-0.291,-0.29,-0.289,-0.288,-0.287,-0.286,-0.285,-0.284,
-0.283,-0.282,-0.281,-0.28,-0.279,-0.278,-0.277,-0.276,-0.275,-0.274,-0.273,
-0.272,-0.271,-0.27,-0.269,-0.268,-0.267,-0.266,-0.265,-0.264,-0.263,-0.262,
-0.261,-0.26,-0.259,-0.258,-0.257,-0.256,-0.255,-0.254,-0.253,-0.252,-0.251,
-0.25,-0.249,-0.248,-0.247,-0.246,-0.245,-0.244,-0.243,-0.242,-0.241,-0.24,
-0.239,-0.238,-0.237,-0.236,-0.235,-0.234,-0.233,-0.232,-0.231,-0.23,-0.229,
-0.228,-0.227,-0.226,-0.225,-0.224,-0.223,-0.222,-0.221,-0.22,-0.219,-0.218,
-0.217,-0.216,-0.215,-0.214,-0.213,-0.212,-0.211,-0.21,-0.209,-0.208,-0.207,
-0.206,-0.205,-0.204,-0.203,-0.202,-0.201,-0.2,-0.199,-0.198,-0.197,-0.196,
-0.195,-0.194,-0.193,-0.192,-0.191,-0.19,-0.189,-0.188,-0.187,-0.186,-0.185,
-0.184,-0.183,-0.182,-0.181,-0.18,-0.179,-0.178,-0.177,-0.176,-0.175,-0.174,
-0.173,-0.172,-0.171,-0.17,-0.169,-0.168,-0.167,-0.166,-0.165,-0.164,-0.163,
-0.162,-0.161,-0.16,-0.159,-0.158,-0.157,-0.156,-0.155,-0.154,-0.153,-0.152,
-0.151,-0.15,-0.149,-0.148,-0.147,-0.146,-0.145,-0.144,-0.143,-0.142,-0.141,
-0.14,-0.139,-0.138,-0.137,-0.136,-0.135,-0.134,-0.133,-0.132,-0.131,-0.13,
-0.129,-0.128,-0.127,-0.126,-0.125,-0.124,-0.123,-0.122,-0.121,-0.12,-0.119,
-0.118,-0.117,-0.116,-0.115,-0.114,-0.113,-0.112,-0.111,-0.11,-0.109,-0.108,
-0.107,-0.106,-0.105,-0.104,-0.103,-0.102,-0.101,-0.1,-0.0990000000000001,
-0.0980000000000001,-0.0970000000000001,-0.0960000000000001,-0.0950000000000001,
-0.0940000000000001,-0.0930000000000001,-0.0920000000000001,-0.0910000000000001,
-0.0900000000000001,-0.0890000000000001,-0.0880000000000001,-0.0870000000000001,
-0.0860000000000001,-0.0850000000000001,-0.0840000000000001,-0.0830000000000001,
-0.0820000000000001,-0.0810000000000001,-0.0800000000000001,-0.0790000000000001,
-0.0780000000000001,-0.0770000000000001,-0.0760000000000001,-0.0750000000000001,
-0.0740000000000001,-0.0730000000000001,-0.0720000000000001,-0.071,-0.07,
-0.069,-0.068,-0.067,-0.066,-0.065,-0.064,-0.063,-0.062,-0.061,-0.06,-0.059,
-0.058,-0.057,-0.056,-0.055,-0.054,-0.053,-0.052,-0.051,-0.05,-0.049,-0.048,
-0.047,-0.046,-0.045,-0.044,-0.043,-0.042,-0.041,-0.04,-0.039,-0.038,-0.037,
-0.036,-0.035,-0.034,-0.033,-0.032,-0.031,-0.03,-0.029,-0.028,-0.027,-0.026,
-0.025,-0.024,-0.023,-0.022,-0.021,-0.02,-0.019,-0.018,-0.017,-0.016,-0.015,
-0.014,-0.013,-0.012,-0.011,-0.01,-0.009,-0.008,-0.007,-0.006,-0.005,-0.004,
-0.003,-0.002,-0.001,0.),(0.,2.),.UNSPECIFIED.)
GEOMETRIC_REPRESENTATION_ITEM()
RATIONAL_B_SPLINE_SURFACE(((1.,1.),(1.,1.),(1.,1.),(1.,1.),(1.,1.),(1.,
1.),(1.,1.),(1.,1.),(1.,1.),(1.,1.),(1.,1.),(1.,1.),(1.,1.),(1.,1.),(1.,
1.),(1.,1.),(1.,1.),(1.,1.),(1.,1.),(1.,1.),(1.,1.),(1.,1.),(1.,1.),(1.,
1.),(1.,1.),(1.,1.),(1.,1.),(1.,1.),(1.,1.),(1.,1.),(1.,1.),(1.,1.),(1.,
1.),(1.,1.),(1.,1.),(1.,1.),(1.,1.),(1.,1.),(1.,1.),(1.,1.),(1.,1.),(1.,
1.),(1.,1.),(1.,1.),(1.,1.),(1.,1.),(1.,1.),(1.,1.),(1.,1.),(1.,1.),(1.,
1.),(1.,1.),(1.,1.),(1.,1.),(1.,1.),(1.,1.),(1.,1.),(1.,1.),(1.,1.),(1.,
1.),(1.,1.),(1.,1.),(1.,1.),(1.,1.),(1.,1.),(1.,1.),(1.,1.),(1.,1.),(1.,
1.),(1.,1.),(1.,1.),(1.,1.),(1.,1.),(1.,1.),(1.,1.),(1.,1.),(1.,1.),(1.,
1.),(1.,1.),(1.,1.),(1.,1.),(1.,1.),(1.,1.),(1.,1.),(1.,1.),(1.,1.),(1.,
1.),(1.,1.),(1.,1.),(1.,1.),(1.,1.),(1.,1.),(1.,1.),(1.,1.),(1.,1.),(1.,
1.),(1.,1.),(1.,1.),(1.,1.),(1.,1.),(1.,1.),(1.,1.),(1.,1.),(1.,1.),(1.,
1.),(1.,1.),(1.,1.),(1.,1.),(1.,1.),(1.,1.),(1.,1.),(1.,1.),(1.,1.),(1.,
1.),(1.,1.),(1.,1.),(1.,1.),(1.,1.),(1.,1.),(1.,1.),(1.,1.),(1.,1.),(1.,
1.),(1.,1.),(1.,1.),(1.,1.),(1.,1.),(1.,1.),(1.,1.),(1.,1.),(1.,1.),(1.,
1.),(1.,1.),(1.,1.),(1.,1.),(1.,1.),(1.,1.),(1.,1.),(1.,1.),(1.,1.),(1.,
1.),(1.,1.),(1.,1.),(1.,1.),(1.,1.),(1.,1.),(1.,1.),(1.,1.),(1.,1.),(1.,
1.),(1.,1.),(1.,1.),(1.,1.),(1.,1.),(1.,1.),(1.,1.),(1.,1.),(1.,1.),(1.,
1.),(1.,1.),(1.,1.),(1.,1.),(1.,1.),(1.,1.),(1.,1.),(1.,1.),(1.,1.),(1.,
1.),(1.,1.),(1.,1.),(1.,1.),(1.,1.),(1.,1.),(1.,1.),(1.,1.),(1.,1.),(1.,
1.),(1.,1.),(1.,1.),(1.,1.),(1.,1.),(1.,1.),(1.,1.),(1.,1.),(1.,1.),(1.,
1.),(1.,1.),(1.,1.),(1.,1.),(1.,1.),(1.,1.),(1.,1.),(1.,1.),(1.,1.),(1.,
1.),(1.,1.),(1.,1.),(1.,1.),(1.,1.),(1.,1.),(1.,1.),(1.,1.),(1.,1.),(1.,
1.),(1.,1.),(1.,1.),(1.,1.),(1.,1.),(1.,1.),(1.,1.),(1.,1.),(1.,1.),(1.,
1.),(1.,1.),(1.,1.),(1.,1.),(1.,1.),(1.,1.),(1.,1.),(1.,1.),(1.,1.),(1.,
1.),(1.,1.),(1.,1.),(1.,1.),(1.,1.),(1.,1.),(1.,1.),(1.,1.),(1.,1.),(1.,
1.),(1.,1.),(1.,1.),(1.,1.),(1.,1.),(1.,1.),(1.,1.),(1.,1.),(1.,1.),(1.,
1.),(1.,1.),(1.,1.),(1.,1.),(1.,1.),(1.,1.),(1.,1.),(1.,1.),(1.,1.),(1.,
1.),(1.,1.),(1.,1.),(1.,1.),(1.,1.),(1.,1.),(1.,1.),(1.,1.),(1.,1.),(1.,
1.),(1.,1.),(1.,1.),(1.,1.),(1.,1.),(1.,1.),(1.,1.),(1.,1.),(1.,1.),(1.,
1.),(1.,1.),(1.,1.),(1.,1.),(1.,1.),(1.,1.),(1.,1.),(1.,1.),(1.,1.),(1.,
1.),(1.,1.),(1.,1.),(1.,1.),(1.,1.),(1.,1.),(1.,1.),(1.,1.),(1.,1.),(1.,
1.),(1.,1.),(1.,1.),(1.,1.),(1.,1.),(1.,1.),(1.,1.),(1.,1.),(1.,1.),(1.,
1.),(1.,1.),(1.,1.),(1.,1.),(1.,1.),(1.,1.),(1.,1.),(1.,1.),(1.,1.),(1.,
1.),(1.,1.),(1.,1.),(1.,1.),(1.,1.),(1.,1.),(1.,1.),(1.,1.),(1.,1.),(1.,
1.),(1.,1.),(1.,1.),(1.,1.),(1.,1.),(1.,1.),(1.,1.),(1.,1.),(1.,1.),(1.,
1.),(1.,1.),(1.,1.),(1.,1.),(1.,1.),(1.,1.),(1.,1.),(1.,1.),(1.,1.),(1.,
1.),(1.,1.),(1.,1.),(1.,1.),(1.,1.),(1.,1.),(1.,1.),(1.,1.),(1.,1.),(1.,
1.),(1.,1.),(1.,1.),(1.,1.),(1.,1.),(1.,1.),(1.,1.),(1.,1.),(1.,1.),(1.,
1.),(1.,1.),(1.,1.),(1.,1.),(1.,1.),(1.,1.),(1.,1.),(1.,1.),(1.,1.),(1.,
1.),(1.,1.),(1.,1.),(1.,1.),(1.,1.),(1.,1.),(1.,1.),(1.,1.),(1.,1.),(1.,
1.),(1.,1.),(1.,1.),(1.,1.),(1.,1.),(1.,1.),(1.,1.),(1.,1.),(1.,1.),(1.,
1.),(1.,1.),(1.,1.),(1.,1.),(1.,1.),(1.,1.),(1.,1.),(1.,1.),(1.,1.),(1.,
1.),(1.,1.),(1.,1.),(1.,1.),(1.,1.),(1.,1.),(1.,1.),(1.,1.),(1.,1.),(1.,
1.),(1.,1.),(1.,1.),(1.,1.),(1.,1.),(1.,1.),(1.,1.),(1.,1.),(1.,1.),(1.,
1.),(1.,1.),(1.,1.),(1.,1.),(1.,1.),(1.,1.),(1.,1.),(1.,1.),(1.,1.),(1.,
1.),(1.,1.),(1.,1.),(1.,1.),(1.,1.),(1.,1.),(1.,1.),(1.,1.),(1.,1.),(1.,
1.),(1.,1.),(1.,1.),(1.,1.),(1.,1.),(1.,1.),(1.,1.),(1.,1.),(1.,1.),(1.,
1.),(1.,1.),(1.,1.),(1.,1.),(1.,1.),(1.,1.),(1.,1.),(1.,1.),(1.,1.),(1.,
1.),(1.,1.),(1.,1.),(1.,1.),(1.,1.),(1.,1.),(1.,1.),(1.,1.),(1.,1.),(1.,
1.),(1.,1.),(1.,1.),(1.,1.),(1.,1.),(1.,1.),(1.,1.),(1.,1.),(1.,1.),(1.,
1.),(1.,1.),(1.,1.),(1.,1.),(1.,1.),(1.,1.),(1.,1.),(1.,1.),(1.,1.),(1.,
1.),(1.,1.),(1.,1.),(1.,1.),(1.,1.),(1.,1.),(1.,1.),(1.,1.),(1.,1.),(1.,
1.),(1.,1.),(1.,1.),(1.,1.),(1.,1.),(1.,1.),(1.,1.),(1.,1.),(1.,1.),(1.,
1.),(1.,1.),(1.,1.),(1.,1.),(1.,1.),(1.,1.),(1.,1.),(1.,1.),(1.,1.),(1.,
1.),(1.,1.),(1.,1.),(1.,1.),(1.,1.),(1.,1.),(1.,1.),(1.,1.),(1.,1.),(1.,
1.),(1.,1.),(1.,1.),(1.,1.),(1.,1.),(1.,1.),(1.,1.),(1.,1.),(1.,1.),(1.,
1.),(1.,1.),(1.,1.),(1.,1.),(1.,1.),(1.,1.),(1.,1.),(1.,1.),(1.,1.),(1.,
1.),(1.,1.),(1.,1.),(1.,1.),(1.,1.),(1.,1.),(1.,1.),(1.,1.),(1.,1.),(1.,
1.),(1.,1.),(1.,1.),(1.,1.),(1.,1.),(1.,1.),(1.,1.),(1.,1.),(1.,1.),(1.,
1.),(1.,1.),(1.,1.),(1.,1.),(1.,1.),(1.,1.),(1.,1.),(1.,1.),(1.,1.),(1.,
1.),(1.,1.),(1.,1.),(1.,1.),(1.,1.),(1.,1.),(1.,1.),(1.,1.),(1.,1.),(1.,
1.),(1.,1.),(1.,1.),(1.,1.),(1.,1.),(1.,1.),(1.,1.),(1.,1.),(1.,1.),(1.,
1.),(1.,1.),(1.,1.),(1.,1.),(1.,1.),(1.,1.),(1.,1.),(1.,1.),(1.,1.),(1.,
1.),(1.,1.),(1.,1.),(1.,1.),(1.,1.),(1.,1.),(1.,1.),(1.,1.),(1.,1.),(1.,
1.),(1.,1.),(1.,1.),(1.,1.),(1.,1.),(1.,1.),(1.,1.),(1.,1.),(1.,1.),(1.,
1.),(1.,1.),(1.,1.),(1.,1.),(1.,1.),(1.,1.),(1.,1.),(1.,1.),(1.,1.),(1.,
1.),(1.,1.),(1.,1.),(1.,1.),(1.,1.),(1.,1.),(1.,1.),(1.,1.),(1.,1.),(1.,
1.),(1.,1.),(1.,1.),(1.,1.),(1.,1.),(1.,1.),(1.,1.),(1.,1.),(1.,1.),(1.,
1.),(1.,1.),(1.,1.),(1.,1.),(1.,1.),(1.,1.),(1.,1.),(1.,1.),(1.,1.),(1.,
1.),(1.,1.),(1.,1.),(1.,1.),(1.,1.),(1.,1.),(1.,1.),(1.,1.),(1.,1.),(1.,
1.),(1.,1.),(1.,1.),(1.,1.),(1.,1.),(1.,1.),(1.,1.),(1.,1.),(1.,1.),(1.,
1.),(1.,1.),(1.,1.),(1.,1.),(1.,1.),(1.,1.),(1.,1.),(1.,1.),(1.,1.),(1.,
1.),(1.,1.),(1.,1.),(1.,1.),(1.,1.),(1.,1.),(1.,1.),(1.,1.),(1.,1.),(1.,
1.),(1.,1.),(1.,1.),(1.,1.),(1.,1.),(1.,1.),(1.,1.),(1.,1.),(1.,1.),(1.,
1.),(1.,1.),(1.,1.),(1.,1.),(1.,1.),(1.,1.),(1.,1.),(1.,1.),(1.,1.),(1.,
1.),(1.,1.),(1.,1.),(1.,1.),(1.,1.),(1.,1.),(1.,1.),(1.,1.),(1.,1.),(1.,
1.),(1.,1.),(1.,1.),(1.,1.),(1.,1.),(1.,1.),(1.,1.),(1.,1.),(1.,1.),(1.,
1.),(1.,1.),(1.,1.),(1.,1.),(1.,1.),(1.,1.),(1.,1.),(1.,1.),(1.,1.),(1.,
1.),(1.,1.),(1.,1.),(1.,1.),(1.,1.),(1.,1.),(1.,1.),(1.,1.),(1.,1.),(1.,
1.),(1.,1.),(1.,1.),(1.,1.),(1.,1.),(1.,1.),(1.,1.),(1.,1.),(1.,1.),(1.,
1.),(1.,1.),(1.,1.),(1.,1.),(1.,1.),(1.,1.),(1.,1.),(1.,1.),(1.,1.),(1.,
1.),(1.,1.),(1.,1.),(1.,1.),(1.,1.),(1.,1.),(1.,1.),(1.,1.),(1.,1.),(1.,
1.),(1.,1.),(1.,1.),(1.,1.),(1.,1.),(1.,1.),(1.,1.),(1.,1.),(1.,1.),(1.,
1.),(1.,1.),(1.,1.),(1.,1.),(1.,1.),(1.,1.),(1.,1.),(1.,1.),(1.,1.),(1.,
1.),(1.,1.),(1.,1.),(1.,1.),(1.,1.),(1.,1.),(1.,1.),(1.,1.),(1.,1.),(1.,
1.),(1.,1.),(1.,1.),(1.,1.),(1.,1.),(1.,1.),(1.,1.),(1.,1.),(1.,1.),(1.,
1.),(1.,1.),(1.,1.),(1.,1.),(1.,1.),(1.,1.),(1.,1.),(1.,1.),(1.,1.),(1.,
1.),(1.,1.),(1.,1.),(1.,1.),(1.,1.),(1.,1.),(1.,1.),(1.,1.),(1.,1.),(1.,
1.),(1.,1.),(1.,1.),(1.,1.),(1.,1.),(1.,1.),(1.,1.),(1.,1.),(1.,1.),(1.,
1.),(1.,1.),(1.,1.),(1.,1.),(1.,1.),(1.,1.),(1.,1.),(1.,1.),(1.,1.),(1.,
1.),(1.,1.),(1.,1.),(1.,1.),(1.,1.),(1.,1.),(1.,1.),(1.,1.),(1.,1.),(1.,
1.),(1.,1.),(1.,1.),(1.,1.),(1.,1.),(1.,1.),(1.,1.),(1.,1.),(1.,1.),(1.,
1.),(1.,1.),(1.,1.),(1.,1.),(1.,1.),(1.,1.),(1.,1.),(1.,1.),(1.,1.),(1.,
1.),(1.,1.),(1.,1.),(1.,1.),(1.,1.),(1.,1.),(1.,1.),(1.,1.),(1.,1.),(1.,
1.),(1.,1.),(1.,1.),(1.,1.),(1.,1.),(1.,1.),(1.,1.),(1.,1.),(1.,1.),(1.,
1.),(1.,1.),(1.,1.),(1.,1.),(1.,1.),(1.,1.),(1.,1.),(1.,1.),(1.,1.),(1.,
1.),(1.,1.),(1.,1.),(1.,1.),(1.,1.),(1.,1.),(1.,1.),(1.,1.),(1.,1.),(1.,
1.),(1.,1.),(1.,1.),(1.,1.),(1.,1.),(1.,1.),(1.,1.),(1.,1.),(1.,1.),(1.,
1.),(1.,1.),(1.,1.),(1.,1.),(1.,1.),(1.,1.),(1.,1.),(1.,1.),(1.,1.),(1.,
1.),(1.,1.),(1.,1.),(1.,1.),(1.,1.),(1.,1.),(1.,1.),(1.,1.),(1.,1.),(1.,
1.),(1.,1.),(1.,1.),(1.,1.),(1.,1.),(1.,1.),(1.,1.),(1.,1.),(1.,1.),(1.,
1.),(1.,1.),(1.,1.),(1.,1.),(1.,1.),(1.,1.),(1.,1.),(1.,1.),(1.,1.),(1.,
1.),(1.,1.),(1.,1.),(1.,1.),(1.,1.),(1.,1.),(1.,1.),(1.,1.),(1.,1.),(1.,
1.),(1.,1.),(1.,1.),(1.,1.),(1.,1.),(1.,1.),(1.,1.),(1.,1.),(1.,1.),(1.,
1.),(1.,1.),(1.,1.),(1.,1.),(1.,1.),(1.,1.),(1.,1.),(1.,1.),(1.,1.),(1.,
1.),(1.,1.),(1.,1.),(1.,1.),(1.,1.),(1.,1.),(1.,1.),(1.,1.),(1.,1.),(1.,
1.),(1.,1.),(1.,1.),(1.,1.),(1.,1.),(1.,1.),(1.,1.),(1.,1.),(1.,1.),(1.,
1.),(1.,1.),(1.,1.),(1.,1.),(1.,1.),(1.,1.),(1.,1.),(1.,1.),(1.,1.),(1.,
1.),(1.,1.),(1.,1.),(1.,1.),(1.,1.),(1.,1.),(1.,1.),(1.,1.),(1.,1.),(1.,
1.),(1.,1.),(1.,1.),(1.,1.),(1.,1.),(1.,1.),(1.,1.),(1.,1.),(1.,1.),(1.,
1.),(1.,1.),(1.,1.),(1.,1.),(1.,1.),(1.,1.),(1.,1.),(1.,1.),(1.,1.),(1.,
1.)))
REPRESENTATION_ITEM('')
SURFACE()
);
#261=(
BOUNDED_SURFACE()
B_SPLINE_SURFACE(5,1,((#80173,#80174),(#80175,#80176),(#80177,#80178),(#80179,
#80180),(#80181,#80182),(#80183,#80184),(#80185,#80186),(#80187,#80188),
(#80189,#80190),(#80191,#80192),(#80193,#80194),(#80195,#80196),(#80197,
#80198),(#80199,#80200),(#80201,#80202),(#80203,#80204),(#80205,#80206),
(#80207,#80208),(#80209,#80210),(#80211,#80212),(#80213,#80214),(#80215,
#80216),(#80217,#80218),(#80219,#80220),(#80221,#80222),(#80223,#80224),
(#80225,#80226),(#80227,#80228),(#80229,#80230),(#80231,#80232),(#80233,
#80234),(#80235,#80236),(#80237,#80238),(#80239,#80240),(#80241,#80242),
(#80243,#80244),(#80245,#80246),(#80247,#80248),(#80249,#80250),(#80251,
#80252),(#80253,#80254),(#80255,#80256),(#80257,#80258),(#80259,#80260),
(#80261,#80262),(#80263,#80264),(#80265,#80266),(#80267,#80268),(#80269,
#80270),(#80271,#80272),(#80273,#80274),(#80275,#80276),(#80277,#80278),
(#80279,#80280),(#80281,#80282),(#80283,#80284),(#80285,#80286),(#80287,
#80288),(#80289,#80290),(#80291,#80292),(#80293,#80294),(#80295,#80296),
(#80297,#80298),(#80299,#80300),(#80301,#80302),(#80303,#80304),(#80305,
#80306),(#80307,#80308),(#80309,#80310),(#80311,#80312),(#80313,#80314),
(#80315,#80316),(#80317,#80318),(#80319,#80320),(#80321,#80322),(#80323,
#80324),(#80325,#80326),(#80327,#80328),(#80329,#80330),(#80331,#80332),
(#80333,#80334),(#80335,#80336),(#80337,#80338),(#80339,#80340),(#80341,
#80342),(#80343,#80344),(#80345,#80346),(#80347,#80348),(#80349,#80350),
(#80351,#80352),(#80353,#80354),(#80355,#80356),(#80357,#80358),(#80359,
#80360),(#80361,#80362),(#80363,#80364),(#80365,#80366),(#80367,#80368),
(#80369,#80370),(#80371,#80372),(#80373,#80374),(#80375,#80376),(#80377,
#80378),(#80379,#80380),(#80381,#80382),(#80383,#80384),(#80385,#80386),
(#80387,#80388),(#80389,#80390),(#80391,#80392),(#80393,#80394),(#80395,
#80396),(#80397,#80398),(#80399,#80400),(#80401,#80402),(#80403,#80404),
(#80405,#80406),(#80407,#80408),(#80409,#80410),(#80411,#80412),(#80413,
#80414),(#80415,#80416),(#80417,#80418),(#80419,#80420),(#80421,#80422),
(#80423,#80424),(#80425,#80426),(#80427,#80428),(#80429,#80430),(#80431,
#80432),(#80433,#80434),(#80435,#80436),(#80437,#80438),(#80439,#80440),
(#80441,#80442),(#80443,#80444),(#80445,#80446),(#80447,#80448),(#80449,
#80450),(#80451,#80452),(#80453,#80454),(#80455,#80456),(#80457,#80458),
(#80459,#80460),(#80461,#80462),(#80463,#80464),(#80465,#80466),(#80467,
#80468),(#80469,#80470),(#80471,#80472),(#80473,#80474),(#80475,#80476),
(#80477,#80478),(#80479,#80480),(#80481,#80482),(#80483,#80484),(#80485,
#80486),(#80487,#80488),(#80489,#80490),(#80491,#80492),(#80493,#80494),
(#80495,#80496),(#80497,#80498),(#80499,#80500),(#80501,#80502),(#80503,
#80504),(#80505,#80506),(#80507,#80508),(#80509,#80510),(#80511,#80512),
(#80513,#80514),(#80515,#80516),(#80517,#80518),(#80519,#80520),(#80521,
#80522),(#80523,#80524),(#80525,#80526),(#80527,#80528),(#80529,#80530),
(#80531,#80532),(#80533,#80534),(#80535,#80536),(#80537,#80538),(#80539,
#80540),(#80541,#80542),(#80543,#80544),(#80545,#80546),(#80547,#80548),
(#80549,#80550),(#80551,#80552),(#80553,#80554),(#80555,#80556),(#80557,
#80558),(#80559,#80560),(#80561,#80562),(#80563,#80564),(#80565,#80566),
(#80567,#80568),(#80569,#80570),(#80571,#80572),(#80573,#80574),(#80575,
#80576),(#80577,#80578),(#80579,#80580),(#80581,#80582),(#80583,#80584),
(#80585,#80586),(#80587,#80588),(#80589,#80590),(#80591,#80592),(#80593,
#80594),(#80595,#80596),(#80597,#80598),(#80599,#80600),(#80601,#80602),
(#80603,#80604),(#80605,#80606),(#80607,#80608),(#80609,#80610),(#80611,
#80612),(#80613,#80614),(#80615,#80616),(#80617,#80618),(#80619,#80620),
(#80621,#80622),(#80623,#80624),(#80625,#80626),(#80627,#80628),(#80629,
#80630),(#80631,#80632),(#80633,#80634),(#80635,#80636),(#80637,#80638),
(#80639,#80640),(#80641,#80642),(#80643,#80644),(#80645,#80646),(#80647,
#80648),(#80649,#80650),(#80651,#80652),(#80653,#80654),(#80655,#80656),
(#80657,#80658),(#80659,#80660),(#80661,#80662),(#80663,#80664),(#80665,
#80666),(#80667,#80668),(#80669,#80670),(#80671,#80672),(#80673,#80674),
(#80675,#80676),(#80677,#80678),(#80679,#80680),(#80681,#80682),(#80683,
#80684),(#80685,#80686),(#80687,#80688),(#80689,#80690),(#80691,#80692),
(#80693,#80694),(#80695,#80696),(#80697,#80698),(#80699,#80700),(#80701,
#80702),(#80703,#80704),(#80705,#80706),(#80707,#80708),(#80709,#80710),
(#80711,#80712),(#80713,#80714),(#80715,#80716),(#80717,#80718),(#80719,
#80720),(#80721,#80722),(#80723,#80724),(#80725,#80726),(#80727,#80728),
(#80729,#80730),(#80731,#80732),(#80733,#80734),(#80735,#80736),(#80737,
#80738),(#80739,#80740),(#80741,#80742),(#80743,#80744),(#80745,#80746),
(#80747,#80748),(#80749,#80750),(#80751,#80752),(#80753,#80754),(#80755,
#80756),(#80757,#80758),(#80759,#80760),(#80761,#80762),(#80763,#80764),
(#80765,#80766),(#80767,#80768),(#80769,#80770),(#80771,#80772),(#80773,
#80774),(#80775,#80776),(#80777,#80778),(#80779,#80780),(#80781,#80782),
(#80783,#80784),(#80785,#80786),(#80787,#80788),(#80789,#80790),(#80791,
#80792),(#80793,#80794),(#80795,#80796),(#80797,#80798),(#80799,#80800),
(#80801,#80802),(#80803,#80804),(#80805,#80806),(#80807,#80808),(#80809,
#80810),(#80811,#80812),(#80813,#80814),(#80815,#80816),(#80817,#80818),
(#80819,#80820),(#80821,#80822),(#80823,#80824),(#80825,#80826),(#80827,
#80828),(#80829,#80830),(#80831,#80832),(#80833,#80834),(#80835,#80836),
(#80837,#80838),(#80839,#80840),(#80841,#80842),(#80843,#80844),(#80845,
#80846),(#80847,#80848),(#80849,#80850),(#80851,#80852),(#80853,#80854),
(#80855,#80856),(#80857,#80858),(#80859,#80860),(#80861,#80862),(#80863,
#80864),(#80865,#80866),(#80867,#80868),(#80869,#80870),(#80871,#80872),
(#80873,#80874),(#80875,#80876),(#80877,#80878),(#80879,#80880),(#80881,
#80882),(#80883,#80884),(#80885,#80886),(#80887,#80888),(#80889,#80890),
(#80891,#80892),(#80893,#80894),(#80895,#80896),(#80897,#80898),(#80899,
#80900),(#80901,#80902),(#80903,#80904),(#80905,#80906),(#80907,#80908),
(#80909,#80910),(#80911,#80912),(#80913,#80914),(#80915,#80916),(#80917,
#80918),(#80919,#80920),(#80921,#80922),(#80923,#80924),(#80925,#80926),
(#80927,#80928),(#80929,#80930),(#80931,#80932),(#80933,#80934),(#80935,
#80936),(#80937,#80938),(#80939,#80940),(#80941,#80942),(#80943,#80944),
(#80945,#80946),(#80947,#80948),(#80949,#80950),(#80951,#80952),(#80953,
#80954),(#80955,#80956),(#80957,#80958),(#80959,#80960),(#80961,#80962),
(#80963,#80964),(#80965,#80966),(#80967,#80968),(#80969,#80970),(#80971,
#80972),(#80973,#80974),(#80975,#80976),(#80977,#80978),(#80979,#80980),
(#80981,#80982),(#80983,#80984),(#80985,#80986),(#80987,#80988),(#80989,
#80990),(#80991,#80992),(#80993,#80994),(#80995,#80996),(#80997,#80998),
(#80999,#81000),(#81001,#81002),(#81003,#81004),(#81005,#81006),(#81007,
#81008),(#81009,#81010),(#81011,#81012),(#81013,#81014),(#81015,#81016),
(#81017,#81018),(#81019,#81020),(#81021,#81022),(#81023,#81024),(#81025,
#81026),(#81027,#81028),(#81029,#81030),(#81031,#81032),(#81033,#81034),
(#81035,#81036),(#81037,#81038),(#81039,#81040),(#81041,#81042),(#81043,
#81044),(#81045,#81046),(#81047,#81048),(#81049,#81050),(#81051,#81052),
(#81053,#81054),(#81055,#81056),(#81057,#81058),(#81059,#81060),(#81061,
#81062),(#81063,#81064),(#81065,#81066),(#81067,#81068),(#81069,#81070),
(#81071,#81072),(#81073,#81074),(#81075,#81076),(#81077,#81078),(#81079,
#81080),(#81081,#81082),(#81083,#81084),(#81085,#81086),(#81087,#81088),
(#81089,#81090),(#81091,#81092),(#81093,#81094),(#81095,#81096),(#81097,
#81098),(#81099,#81100),(#81101,#81102),(#81103,#81104),(#81105,#81106),
(#81107,#81108),(#81109,#81110),(#81111,#81112),(#81113,#81114),(#81115,
#81116),(#81117,#81118),(#81119,#81120),(#81121,#81122),(#81123,#81124),
(#81125,#81126),(#81127,#81128),(#81129,#81130),(#81131,#81132),(#81133,
#81134),(#81135,#81136),(#81137,#81138),(#81139,#81140),(#81141,#81142),
(#81143,#81144),(#81145,#81146),(#81147,#81148),(#81149,#81150),(#81151,
#81152),(#81153,#81154),(#81155,#81156),(#81157,#81158),(#81159,#81160),
(#81161,#81162),(#81163,#81164),(#81165,#81166),(#81167,#81168),(#81169,
#81170),(#81171,#81172),(#81173,#81174),(#81175,#81176),(#81177,#81178),
(#81179,#81180),(#81181,#81182),(#81183,#81184),(#81185,#81186),(#81187,
#81188),(#81189,#81190),(#81191,#81192),(#81193,#81194),(#81195,#81196),
(#81197,#81198),(#81199,#81200),(#81201,#81202),(#81203,#81204),(#81205,
#81206),(#81207,#81208),(#81209,#81210),(#81211,#81212),(#81213,#81214),
(#81215,#81216),(#81217,#81218),(#81219,#81220),(#81221,#81222),(#81223,
#81224),(#81225,#81226),(#81227,#81228),(#81229,#81230),(#81231,#81232),
(#81233,#81234),(#81235,#81236),(#81237,#81238),(#81239,#81240),(#81241,
#81242),(#81243,#81244),(#81245,#81246),(#81247,#81248),(#81249,#81250),
(#81251,#81252),(#81253,#81254),(#81255,#81256),(#81257,#81258),(#81259,
#81260),(#81261,#81262),(#81263,#81264),(#81265,#81266),(#81267,#81268),
(#81269,#81270),(#81271,#81272),(#81273,#81274),(#81275,#81276),(#81277,
#81278),(#81279,#81280),(#81281,#81282),(#81283,#81284),(#81285,#81286),
(#81287,#81288),(#81289,#81290),(#81291,#81292),(#81293,#81294),(#81295,
#81296),(#81297,#81298),(#81299,#81300),(#81301,#81302),(#81303,#81304),
(#81305,#81306),(#81307,#81308),(#81309,#81310),(#81311,#81312),(#81313,
#81314),(#81315,#81316),(#81317,#81318),(#81319,#81320),(#81321,#81322),
(#81323,#81324),(#81325,#81326),(#81327,#81328),(#81329,#81330),(#81331,
#81332),(#81333,#81334),(#81335,#81336),(#81337,#81338),(#81339,#81340),
(#81341,#81342),(#81343,#81344),(#81345,#81346),(#81347,#81348),(#81349,
#81350),(#81351,#81352),(#81353,#81354),(#81355,#81356),(#81357,#81358),
(#81359,#81360),(#81361,#81362),(#81363,#81364),(#81365,#81366),(#81367,
#81368),(#81369,#81370),(#81371,#81372),(#81373,#81374),(#81375,#81376),
(#81377,#81378),(#81379,#81380),(#81381,#81382),(#81383,#81384),(#81385,
#81386),(#81387,#81388),(#81389,#81390),(#81391,#81392),(#81393,#81394),
(#81395,#81396),(#81397,#81398),(#81399,#81400),(#81401,#81402),(#81403,
#81404),(#81405,#81406),(#81407,#81408),(#81409,#81410),(#81411,#81412),
(#81413,#81414),(#81415,#81416),(#81417,#81418),(#81419,#81420),(#81421,
#81422),(#81423,#81424),(#81425,#81426),(#81427,#81428),(#81429,#81430),
(#81431,#81432),(#81433,#81434),(#81435,#81436),(#81437,#81438),(#81439,
#81440),(#81441,#81442),(#81443,#81444),(#81445,#81446),(#81447,#81448),
(#81449,#81450),(#81451,#81452),(#81453,#81454),(#81455,#81456),(#81457,
#81458),(#81459,#81460),(#81461,#81462),(#81463,#81464),(#81465,#81466),
(#81467,#81468),(#81469,#81470),(#81471,#81472),(#81473,#81474),(#81475,
#81476),(#81477,#81478),(#81479,#81480),(#81481,#81482),(#81483,#81484),
(#81485,#81486),(#81487,#81488),(#81489,#81490),(#81491,#81492),(#81493,
#81494),(#81495,#81496),(#81497,#81498),(#81499,#81500),(#81501,#81502),
(#81503,#81504),(#81505,#81506),(#81507,#81508),(#81509,#81510),(#81511,
#81512),(#81513,#81514),(#81515,#81516),(#81517,#81518),(#81519,#81520),
(#81521,#81522),(#81523,#81524),(#81525,#81526),(#81527,#81528),(#81529,
#81530),(#81531,#81532),(#81533,#81534),(#81535,#81536),(#81537,#81538),
(#81539,#81540),(#81541,#81542),(#81543,#81544),(#81545,#81546),(#81547,
#81548),(#81549,#81550),(#81551,#81552),(#81553,#81554),(#81555,#81556),
(#81557,#81558),(#81559,#81560),(#81561,#81562),(#81563,#81564),(#81565,
#81566),(#81567,#81568),(#81569,#81570),(#81571,#81572),(#81573,#81574),
(#81575,#81576),(#81577,#81578),(#81579,#81580),(#81581,#81582),(#81583,
#81584),(#81585,#81586),(#81587,#81588),(#81589,#81590),(#81591,#81592),
(#81593,#81594),(#81595,#81596),(#81597,#81598),(#81599,#81600),(#81601,
#81602),(#81603,#81604),(#81605,#81606),(#81607,#81608),(#81609,#81610),
(#81611,#81612),(#81613,#81614),(#81615,#81616),(#81617,#81618),(#81619,
#81620),(#81621,#81622),(#81623,#81624),(#81625,#81626),(#81627,#81628),
(#81629,#81630),(#81631,#81632),(#81633,#81634),(#81635,#81636),(#81637,
#81638),(#81639,#81640),(#81641,#81642),(#81643,#81644),(#81645,#81646),
(#81647,#81648),(#81649,#81650),(#81651,#81652),(#81653,#81654),(#81655,
#81656),(#81657,#81658),(#81659,#81660),(#81661,#81662),(#81663,#81664),
(#81665,#81666),(#81667,#81668),(#81669,#81670),(#81671,#81672),(#81673,
#81674),(#81675,#81676),(#81677,#81678),(#81679,#81680),(#81681,#81682),
(#81683,#81684),(#81685,#81686),(#81687,#81688),(#81689,#81690),(#81691,
#81692),(#81693,#81694),(#81695,#81696),(#81697,#81698),(#81699,#81700),
(#81701,#81702),(#81703,#81704),(#81705,#81706),(#81707,#81708),(#81709,
#81710),(#81711,#81712),(#81713,#81714),(#81715,#81716),(#81717,#81718),
(#81719,#81720),(#81721,#81722),(#81723,#81724),(#81725,#81726),(#81727,
#81728),(#81729,#81730),(#81731,#81732),(#81733,#81734),(#81735,#81736),
(#81737,#81738),(#81739,#81740),(#81741,#81742),(#81743,#81744),(#81745,
#81746),(#81747,#81748),(#81749,#81750),(#81751,#81752),(#81753,#81754),
(#81755,#81756),(#81757,#81758),(#81759,#81760),(#81761,#81762),(#81763,
#81764),(#81765,#81766),(#81767,#81768),(#81769,#81770),(#81771,#81772),
(#81773,#81774),(#81775,#81776),(#81777,#81778),(#81779,#81780),(#81781,
#81782),(#81783,#81784),(#81785,#81786),(#81787,#81788),(#81789,#81790),
(#81791,#81792),(#81793,#81794),(#81795,#81796),(#81797,#81798),(#81799,
#81800),(#81801,#81802),(#81803,#81804),(#81805,#81806),(#81807,#81808),
(#81809,#81810),(#81811,#81812),(#81813,#81814),(#81815,#81816),(#81817,
#81818),(#81819,#81820),(#81821,#81822),(#81823,#81824),(#81825,#81826),
(#81827,#81828),(#81829,#81830),(#81831,#81832),(#81833,#81834),(#81835,
#81836),(#81837,#81838),(#81839,#81840),(#81841,#81842),(#81843,#81844),
(#81845,#81846),(#81847,#81848),(#81849,#81850),(#81851,#81852),(#81853,
#81854),(#81855,#81856),(#81857,#81858),(#81859,#81860),(#81861,#81862),
(#81863,#81864),(#81865,#81866),(#81867,#81868),(#81869,#81870),(#81871,
#81872),(#81873,#81874),(#81875,#81876),(#81877,#81878),(#81879,#81880),
(#81881,#81882),(#81883,#81884),(#81885,#81886),(#81887,#81888),(#81889,
#81890),(#81891,#81892),(#81893,#81894),(#81895,#81896),(#81897,#81898),
(#81899,#81900),(#81901,#81902),(#81903,#81904),(#81905,#81906),(#81907,
#81908),(#81909,#81910),(#81911,#81912),(#81913,#81914),(#81915,#81916),
(#81917,#81918),(#81919,#81920),(#81921,#81922),(#81923,#81924),(#81925,
#81926),(#81927,#81928),(#81929,#81930),(#81931,#81932),(#81933,#81934),
(#81935,#81936),(#81937,#81938),(#81939,#81940),(#81941,#81942),(#81943,
#81944),(#81945,#81946),(#81947,#81948),(#81949,#81950),(#81951,#81952),
(#81953,#81954),(#81955,#81956),(#81957,#81958),(#81959,#81960),(#81961,
#81962),(#81963,#81964),(#81965,#81966),(#81967,#81968),(#81969,#81970),
(#81971,#81972),(#81973,#81974),(#81975,#81976),(#81977,#81978),(#81979,
#81980),(#81981,#81982),(#81983,#81984),(#81985,#81986),(#81987,#81988),
(#81989,#81990),(#81991,#81992),(#81993,#81994),(#81995,#81996),(#81997,
#81998),(#81999,#82000),(#82001,#82002),(#82003,#82004),(#82005,#82006),
(#82007,#82008),(#82009,#82010),(#82011,#82012),(#82013,#82014),(#82015,
#82016),(#82017,#82018),(#82019,#82020),(#82021,#82022),(#82023,#82024),
(#82025,#82026),(#82027,#82028),(#82029,#82030),(#82031,#82032),(#82033,
#82034),(#82035,#82036),(#82037,#82038),(#82039,#82040),(#82041,#82042),
(#82043,#82044),(#82045,#82046),(#82047,#82048),(#82049,#82050),(#82051,
#82052),(#82053,#82054),(#82055,#82056),(#82057,#82058),(#82059,#82060),
(#82061,#82062),(#82063,#82064),(#82065,#82066),(#82067,#82068),(#82069,
#82070),(#82071,#82072),(#82073,#82074),(#82075,#82076),(#82077,#82078),
(#82079,#82080),(#82081,#82082),(#82083,#82084),(#82085,#82086),(#82087,
#82088),(#82089,#82090),(#82091,#82092),(#82093,#82094),(#82095,#82096),
(#82097,#82098),(#82099,#82100),(#82101,#82102),(#82103,#82104),(#82105,
#82106),(#82107,#82108),(#82109,#82110),(#82111,#82112),(#82113,#82114),
(#82115,#82116),(#82117,#82118),(#82119,#82120),(#82121,#82122),(#82123,
#82124),(#82125,#82126),(#82127,#82128),(#82129,#82130),(#82131,#82132),
(#82133,#82134),(#82135,#82136),(#82137,#82138),(#82139,#82140),(#82141,
#82142),(#82143,#82144),(#82145,#82146),(#82147,#82148),(#82149,#82150),
(#82151,#82152),(#82153,#82154),(#82155,#82156),(#82157,#82158),(#82159,
#82160),(#82161,#82162),(#82163,#82164),(#82165,#82166),(#82167,#82168),
(#82169,#82170),(#82171,#82172),(#82173,#82174),(#82175,#82176),(#82177,
#82178),(#82179,#82180),(#82181,#82182)),.UNSPECIFIED.,.F.,.F.,.F.)
B_SPLINE_SURFACE_WITH_KNOTS((6,1,1,1,1,1,1,1,1,1,1,1,1,1,1,1,1,1,1,1,1,
1,1,1,1,1,1,1,1,1,1,1,1,1,1,1,1,1,1,1,1,1,1,1,1,1,1,1,1,1,1,1,1,1,1,1,1,
1,1,1,1,1,1,1,1,1,1,1,1,1,1,1,1,1,1,1,1,1,1,1,1,1,1,1,1,1,1,1,1,1,1,1,1,
1,1,1,1,1,1,1,1,1,1,1,1,1,1,1,1,1,1,1,1,1,1,1,1,1,1,1,1,1,1,1,1,1,1,1,1,
1,1,1,1,1,1,1,1,1,1,1,1,1,1,1,1,1,1,1,1,1,1,1,1,1,1,1,1,1,1,1,1,1,1,1,1,
1,1,1,1,1,1,1,1,1,1,1,1,1,1,1,1,1,1,1,1,1,1,1,1,1,1,1,1,1,1,1,1,1,1,1,1,
1,1,1,1,1,1,1,1,1,1,1,1,1,1,1,1,1,1,1,1,1,1,1,1,1,1,1,1,1,1,1,1,1,1,1,1,
1,1,1,1,1,1,1,1,1,1,1,1,1,1,1,1,1,1,1,1,1,1,1,1,1,1,1,1,1,1,1,1,1,1,1,1,
1,1,1,1,1,1,1,1,1,1,1,1,1,1,1,1,1,1,1,1,1,1,1,1,1,1,1,1,1,1,1,1,1,1,1,1,
1,1,1,1,1,1,1,1,1,1,1,1,1,1,1,1,1,1,1,1,1,1,1,1,1,1,1,1,1,1,1,1,1,1,1,1,
1,1,1,1,1,1,1,1,1,1,1,1,1,1,1,1,1,1,1,1,1,1,1,1,1,1,1,1,1,1,1,1,1,1,1,1,
1,1,1,1,1,1,1,1,1,1,1,1,1,1,1,1,1,1,1,1,1,1,1,1,1,1,1,1,1,1,1,1,1,1,1,1,
1,1,1,1,1,1,1,1,1,1,1,1,1,1,1,1,1,1,1,1,1,1,1,1,1,1,1,1,1,1,1,1,1,1,1,1,
1,1,1,1,1,1,1,1,1,1,1,1,1,1,1,1,1,1,1,1,1,1,1,1,1,1,1,1,1,1,1,1,1,1,1,1,
1,1,1,1,1,1,1,1,1,1,1,1,1,1,1,1,1,1,1,1,1,1,1,1,1,1,1,1,1,1,1,1,1,1,1,1,
1,1,1,1,1,1,1,1,1,1,1,1,1,1,1,1,1,1,1,1,1,1,1,1,1,1,1,1,1,1,1,1,1,1,1,1,
1,1,1,1,1,1,1,1,1,1,1,1,1,1,1,1,1,1,1,1,1,1,1,1,1,1,1,1,1,1,1,1,1,1,1,1,
1,1,1,1,1,1,1,1,1,1,1,1,1,1,1,1,1,1,1,1,1,1,1,1,1,1,1,1,1,1,1,1,1,1,1,1,
1,1,1,1,1,1,1,1,1,1,1,1,1,1,1,1,1,1,1,1,1,1,1,1,1,1,1,1,1,1,1,1,1,1,1,1,
1,1,1,1,1,1,1,1,1,1,1,1,1,1,1,1,1,1,1,1,1,1,1,1,1,1,1,1,1,1,1,1,1,1,1,1,
1,1,1,1,1,1,1,1,1,1,1,1,1,1,1,1,1,1,1,1,1,1,1,1,1,1,1,1,1,1,1,1,1,1,1,1,
1,1,1,1,1,1,1,1,1,1,1,1,1,1,1,1,1,1,1,1,1,1,1,1,1,1,1,1,1,1,1,1,1,1,1,1,
1,1,1,1,1,1,1,1,1,1,1,1,1,1,1,1,1,1,1,1,1,1,1,1,1,1,1,1,1,1,1,1,1,1,1,1,
1,1,1,1,1,1,1,1,1,1,1,1,1,1,1,1,1,1,1,1,1,1,1,1,1,1,1,1,1,1,1,1,1,1,1,1,
1,1,1,1,1,1,1,1,1,1,1,1,1,1,1,1,1,1,1,1,1,1,1,1,1,1,1,1,1,1,1,1,1,1,1,1,
1,1,1,1,1,1,1,1,1,1,1,1,1,1,1,1,1,1,1,1,1,1,1,1,1,1,1,1,1,1,1,1,1,1,1,1,
1,1,1,1,1,1,1,1,1,1,1,1,1,1,1,1,1,1,1,1,1,1,1,1,1,1,1,1,1,1,1,1,1,1,1,1,
1,1,1,1,1,1,1,1,1,1,1,1,1,1,1,1,1,1,1,1,1,1,1,1,1,1,1,1,1,1,1,1,1,1,1,1,
1,1,1,1,1,1,1,6),(2,2),(-1.,-0.999000000000001,-0.998000000000001,-0.997000000000001,
-0.996000000000001,-0.995000000000001,-0.994000000000001,-0.993000000000001,
-0.992000000000001,-0.991000000000001,-0.990000000000001,-0.989000000000001,
-0.988000000000001,-0.987000000000001,-0.986000000000001,-0.985000000000001,
-0.984000000000001,-0.983000000000001,-0.982000000000001,-0.981000000000001,
-0.980000000000001,-0.979000000000001,-0.978000000000001,-0.977000000000001,
-0.976000000000001,-0.975000000000001,-0.974000000000001,-0.973000000000001,
-0.972000000000001,-0.971000000000001,-0.970000000000001,-0.969000000000001,
-0.968000000000001,-0.967000000000001,-0.966000000000001,-0.965000000000001,
-0.964000000000001,-0.963000000000001,-0.962000000000001,-0.961000000000001,
-0.960000000000001,-0.959000000000001,-0.958000000000001,-0.957000000000001,
-0.956000000000001,-0.955000000000001,-0.954000000000001,-0.953000000000001,
-0.952000000000001,-0.951000000000001,-0.950000000000001,-0.949000000000001,
-0.948000000000001,-0.947000000000001,-0.946000000000001,-0.945000000000001,
-0.944000000000001,-0.943000000000001,-0.942000000000001,-0.941000000000001,
-0.940000000000001,-0.939000000000001,-0.938000000000001,-0.937000000000001,
-0.936000000000001,-0.935000000000001,-0.934000000000001,-0.933000000000001,
-0.932000000000001,-0.931000000000001,-0.930000000000001,-0.929000000000001,
-0.928000000000001,-0.927000000000001,-0.926000000000001,-0.925000000000001,
-0.924000000000001,-0.923000000000001,-0.922000000000001,-0.921000000000001,
-0.920000000000001,-0.919000000000001,-0.918000000000001,-0.917000000000001,
-0.916000000000001,-0.915000000000001,-0.914000000000001,-0.913000000000001,
-0.912000000000001,-0.911000000000001,-0.910000000000001,-0.909000000000001,
-0.908000000000001,-0.907000000000001,-0.906000000000001,-0.905000000000001,
-0.904000000000001,-0.903000000000001,-0.902000000000001,-0.901000000000001,
-0.900000000000001,-0.899000000000001,-0.898000000000001,-0.897000000000001,
-0.896000000000001,-0.895000000000001,-0.894000000000001,-0.893000000000001,
-0.892000000000001,-0.891000000000001,-0.890000000000001,-0.889000000000001,
-0.888000000000001,-0.887000000000001,-0.886000000000001,-0.885000000000001,
-0.884000000000001,-0.883000000000001,-0.882000000000001,-0.881000000000001,
-0.880000000000001,-0.879000000000001,-0.878000000000001,-0.877000000000001,
-0.876000000000001,-0.875000000000001,-0.874000000000001,-0.873000000000001,
-0.872000000000001,-0.871000000000001,-0.870000000000001,-0.869000000000001,
-0.868000000000001,-0.867000000000001,-0.866000000000001,-0.865000000000001,
-0.864000000000001,-0.863000000000001,-0.862000000000001,-0.861000000000001,
-0.860000000000001,-0.859000000000001,-0.858000000000001,-0.857000000000001,
-0.856000000000001,-0.855000000000001,-0.854000000000001,-0.853000000000001,
-0.852000000000001,-0.851000000000001,-0.850000000000001,-0.849000000000001,
-0.848000000000001,-0.847000000000001,-0.846000000000001,-0.845000000000001,
-0.844000000000001,-0.843000000000001,-0.842000000000001,-0.841000000000001,
-0.840000000000001,-0.839000000000001,-0.838000000000001,-0.837000000000001,
-0.836000000000001,-0.835000000000001,-0.834000000000001,-0.833000000000001,
-0.832000000000001,-0.831000000000001,-0.830000000000001,-0.829000000000001,
-0.828000000000001,-0.827000000000001,-0.826000000000001,-0.825000000000001,
-0.824000000000001,-0.823000000000001,-0.822000000000001,-0.821000000000001,
-0.820000000000001,-0.819000000000001,-0.818000000000001,-0.817000000000001,
-0.816000000000001,-0.815000000000001,-0.814000000000001,-0.813000000000001,
-0.812000000000001,-0.811000000000001,-0.810000000000001,-0.809000000000001,
-0.808000000000001,-0.807000000000001,-0.806000000000001,-0.805000000000001,
-0.804000000000001,-0.803000000000001,-0.802000000000001,-0.801000000000001,
-0.800000000000001,-0.799000000000001,-0.798000000000001,-0.797000000000001,
-0.796000000000001,-0.795000000000001,-0.794000000000001,-0.793000000000001,
-0.792000000000001,-0.791000000000001,-0.790000000000001,-0.789000000000001,
-0.788000000000001,-0.787000000000001,-0.786000000000001,-0.785000000000001,
-0.784000000000001,-0.783000000000001,-0.782000000000001,-0.781000000000001,
-0.780000000000001,-0.779000000000001,-0.778000000000001,-0.777000000000001,
-0.776000000000001,-0.775000000000001,-0.774000000000001,-0.773000000000001,
-0.772000000000001,-0.771000000000001,-0.770000000000001,-0.769000000000001,
-0.768000000000001,-0.767000000000001,-0.766000000000001,-0.765000000000001,
-0.764000000000001,-0.763000000000001,-0.762000000000001,-0.761000000000001,
-0.760000000000001,-0.759000000000001,-0.758000000000001,-0.757000000000001,
-0.756000000000001,-0.755000000000001,-0.754000000000001,-0.753000000000001,
-0.752000000000001,-0.751000000000001,-0.750000000000001,-0.749000000000001,
-0.748000000000001,-0.747000000000001,-0.746000000000001,-0.745000000000001,
-0.744000000000001,-0.743000000000001,-0.742000000000001,-0.741000000000001,
-0.740000000000001,-0.739000000000001,-0.738000000000001,-0.737000000000001,
-0.736000000000001,-0.735000000000001,-0.734000000000001,-0.733000000000001,
-0.732000000000001,-0.731000000000001,-0.730000000000001,-0.729000000000001,
-0.728000000000001,-0.727000000000001,-0.726000000000001,-0.725000000000001,
-0.724000000000001,-0.723000000000001,-0.722000000000001,-0.721000000000001,
-0.720000000000001,-0.719000000000001,-0.718000000000001,-0.717000000000001,
-0.716000000000001,-0.715000000000001,-0.714000000000001,-0.713000000000001,
-0.712000000000001,-0.711000000000001,-0.710000000000001,-0.709000000000001,
-0.708000000000001,-0.707000000000001,-0.706000000000001,-0.705000000000001,
-0.704000000000001,-0.703000000000001,-0.702000000000001,-0.701000000000001,
-0.700000000000001,-0.699000000000001,-0.698000000000001,-0.697000000000001,
-0.696000000000001,-0.695000000000001,-0.694000000000001,-0.693000000000001,
-0.692000000000001,-0.691000000000001,-0.690000000000001,-0.689000000000001,
-0.688000000000001,-0.687,-0.686,-0.685,-0.684,-0.683,-0.682,-0.681,-0.68,
-0.679,-0.678,-0.677,-0.676,-0.675,-0.674,-0.673,-0.672,-0.671,-0.67,-0.669,
-0.668,-0.667,-0.666,-0.665,-0.664,-0.663,-0.662,-0.661,-0.66,-0.659,-0.658,
-0.657,-0.656,-0.655,-0.654,-0.653,-0.652,-0.651,-0.65,-0.649,-0.648,-0.647,
-0.646,-0.645,-0.644,-0.643,-0.642,-0.641,-0.64,-0.639,-0.638,-0.637,-0.636,
-0.635,-0.634,-0.633,-0.632,-0.631,-0.63,-0.629,-0.628,-0.627,-0.626,-0.625,
-0.624,-0.623,-0.622,-0.621,-0.62,-0.619,-0.618,-0.617,-0.616,-0.615,-0.614,
-0.613,-0.612,-0.611,-0.61,-0.609,-0.608,-0.607,-0.606,-0.605,-0.604,-0.603,
-0.602,-0.601,-0.6,-0.599,-0.598,-0.597,-0.596,-0.595,-0.594,-0.593,-0.592,
-0.591,-0.59,-0.589,-0.588,-0.587,-0.586,-0.585,-0.584,-0.583,-0.582,-0.581,
-0.58,-0.579,-0.578,-0.577,-0.576,-0.575,-0.574,-0.573,-0.572,-0.571,-0.57,
-0.569,-0.568,-0.567,-0.566,-0.565,-0.564,-0.563,-0.562,-0.561,-0.56,-0.559,
-0.558,-0.557,-0.556,-0.555,-0.554,-0.553,-0.552,-0.551,-0.55,-0.549,-0.548,
-0.547,-0.546,-0.545,-0.544,-0.543,-0.542,-0.541,-0.54,-0.539,-0.538,-0.537,
-0.536,-0.535,-0.534,-0.533,-0.532,-0.531,-0.53,-0.529,-0.528,-0.527,-0.526,
-0.525,-0.524,-0.523,-0.522,-0.521,-0.52,-0.519,-0.518,-0.517,-0.516,-0.515,
-0.514,-0.513,-0.512,-0.511,-0.51,-0.509,-0.508,-0.507,-0.506,-0.505,-0.504,
-0.503,-0.502,-0.501,-0.5,-0.499,-0.498,-0.497,-0.496,-0.495,-0.494,-0.493,
-0.492,-0.491,-0.49,-0.489,-0.488,-0.487,-0.486,-0.485,-0.484,-0.483,-0.482,
-0.481,-0.48,-0.479,-0.478,-0.477,-0.476,-0.475,-0.474,-0.473,-0.472,-0.471,
-0.47,-0.469,-0.468,-0.467,-0.466,-0.465,-0.464,-0.463,-0.462,-0.461,-0.46,
-0.459,-0.458,-0.457,-0.456,-0.455,-0.454,-0.453,-0.452,-0.451,-0.45,-0.449,
-0.448,-0.447,-0.446,-0.445,-0.444,-0.443,-0.442,-0.441,-0.44,-0.439,-0.438,
-0.437,-0.436,-0.435,-0.434,-0.433,-0.432,-0.431,-0.43,-0.429,-0.428,-0.427,
-0.426,-0.425,-0.424,-0.423,-0.422,-0.421,-0.42,-0.419,-0.418,-0.417,-0.416,
-0.415,-0.414,-0.413,-0.412,-0.411,-0.41,-0.409,-0.408,-0.407,-0.406,-0.405,
-0.404,-0.403,-0.402,-0.401,-0.4,-0.399,-0.398,-0.397,-0.396,-0.395,-0.394,
-0.393,-0.392,-0.391,-0.39,-0.389,-0.388,-0.387,-0.386,-0.385,-0.384,-0.383,
-0.382,-0.381,-0.38,-0.379,-0.378,-0.377,-0.376,-0.375,-0.374,-0.373,-0.372,
-0.371,-0.37,-0.369,-0.368,-0.367,-0.366,-0.365,-0.364,-0.363,-0.362,-0.361,
-0.36,-0.359,-0.358,-0.357,-0.356,-0.355,-0.354,-0.353,-0.352,-0.351,-0.35,
-0.349,-0.348,-0.347,-0.346,-0.345,-0.344,-0.343,-0.342,-0.341,-0.34,-0.339,
-0.338,-0.337,-0.336,-0.335,-0.334,-0.333,-0.332,-0.331,-0.33,-0.329,-0.328,
-0.327,-0.326,-0.325,-0.324,-0.323,-0.322,-0.321,-0.32,-0.319,-0.318,-0.317,
-0.316,-0.315,-0.314,-0.313,-0.312,-0.311,-0.31,-0.309,-0.308,-0.307,-0.306,
-0.305,-0.304,-0.303,-0.302,-0.301,-0.3,-0.299,-0.298,-0.297,-0.296,-0.295,
-0.294,-0.293,-0.292,-0.291,-0.29,-0.289,-0.288,-0.287,-0.286,-0.285,-0.284,
-0.283,-0.282,-0.281,-0.28,-0.279,-0.278,-0.277,-0.276,-0.275,-0.274,-0.273,
-0.272,-0.271,-0.27,-0.269,-0.268,-0.267,-0.266,-0.265,-0.264,-0.263,-0.262,
-0.261,-0.26,-0.259,-0.258,-0.257,-0.256,-0.255,-0.254,-0.253,-0.252,-0.251,
-0.25,-0.249,-0.248,-0.247,-0.246,-0.245,-0.244,-0.243,-0.242,-0.241,-0.24,
-0.239,-0.238,-0.237,-0.236,-0.235,-0.234,-0.233,-0.232,-0.231,-0.23,-0.229,
-0.228,-0.227,-0.226,-0.225,-0.224,-0.223,-0.222,-0.221,-0.22,-0.219,-0.218,
-0.217,-0.216,-0.215,-0.214,-0.213,-0.212,-0.211,-0.21,-0.209,-0.208,-0.207,
-0.206,-0.205,-0.204,-0.203,-0.202,-0.201,-0.2,-0.199,-0.198,-0.197,-0.196,
-0.195,-0.194,-0.193,-0.192,-0.191,-0.19,-0.189,-0.188,-0.187,-0.186,-0.185,
-0.184,-0.183,-0.182,-0.181,-0.18,-0.179,-0.178,-0.177,-0.176,-0.175,-0.174,
-0.173,-0.172,-0.171,-0.17,-0.169,-0.168,-0.167,-0.166,-0.165,-0.164,-0.163,
-0.162,-0.161,-0.16,-0.159,-0.158,-0.157,-0.156,-0.155,-0.154,-0.153,-0.152,
-0.151,-0.15,-0.149,-0.148,-0.147,-0.146,-0.145,-0.144,-0.143,-0.142,-0.141,
-0.14,-0.139,-0.138,-0.137,-0.136,-0.135,-0.134,-0.133,-0.132,-0.131,-0.13,
-0.129,-0.128,-0.127,-0.126,-0.125,-0.124,-0.123,-0.122,-0.121,-0.12,-0.119,
-0.118,-0.117,-0.116,-0.115,-0.114,-0.113,-0.112,-0.111,-0.11,-0.109,-0.108,
-0.107,-0.106,-0.105,-0.104,-0.103,-0.102,-0.101,-0.1,-0.0990000000000001,
-0.0980000000000001,-0.0970000000000001,-0.0960000000000001,-0.0950000000000001,
-0.0940000000000001,-0.0930000000000001,-0.0920000000000001,-0.0910000000000001,
-0.0900000000000001,-0.0890000000000001,-0.0880000000000001,-0.0870000000000001,
-0.0860000000000001,-0.0850000000000001,-0.0840000000000001,-0.0830000000000001,
-0.0820000000000001,-0.0810000000000001,-0.0800000000000001,-0.0790000000000001,
-0.0780000000000001,-0.0770000000000001,-0.0760000000000001,-0.0750000000000001,
-0.0740000000000001,-0.0730000000000001,-0.0720000000000001,-0.071,-0.07,
-0.069,-0.068,-0.067,-0.066,-0.065,-0.064,-0.063,-0.062,-0.061,-0.06,-0.059,
-0.058,-0.057,-0.056,-0.055,-0.054,-0.053,-0.052,-0.051,-0.05,-0.049,-0.048,
-0.047,-0.046,-0.045,-0.044,-0.043,-0.042,-0.041,-0.04,-0.039,-0.038,-0.037,
-0.036,-0.035,-0.034,-0.033,-0.032,-0.031,-0.03,-0.029,-0.028,-0.027,-0.026,
-0.025,-0.024,-0.023,-0.022,-0.021,-0.02,-0.019,-0.018,-0.017,-0.016,-0.015,
-0.014,-0.013,-0.012,-0.011,-0.01,-0.009,-0.008,-0.007,-0.006,-0.005,-0.004,
-0.003,-0.002,-0.001,0.),(0.,2.),.UNSPECIFIED.)
GEOMETRIC_REPRESENTATION_ITEM()
RATIONAL_B_SPLINE_SURFACE(((1.,1.),(1.,1.),(1.,1.),(1.,1.),(1.,1.),(1.,
1.),(1.,1.),(1.,1.),(1.,1.),(1.,1.),(1.,1.),(1.,1.),(1.,1.),(1.,1.),(1.,
1.),(1.,1.),(1.,1.),(1.,1.),(1.,1.),(1.,1.),(1.,1.),(1.,1.),(1.,1.),(1.,
1.),(1.,1.),(1.,1.),(1.,1.),(1.,1.),(1.,1.),(1.,1.),(1.,1.),(1.,1.),(1.,
1.),(1.,1.),(1.,1.),(1.,1.),(1.,1.),(1.,1.),(1.,1.),(1.,1.),(1.,1.),(1.,
1.),(1.,1.),(1.,1.),(1.,1.),(1.,1.),(1.,1.),(1.,1.),(1.,1.),(1.,1.),(1.,
1.),(1.,1.),(1.,1.),(1.,1.),(1.,1.),(1.,1.),(1.,1.),(1.,1.),(1.,1.),(1.,
1.),(1.,1.),(1.,1.),(1.,1.),(1.,1.),(1.,1.),(1.,1.),(1.,1.),(1.,1.),(1.,
1.),(1.,1.),(1.,1.),(1.,1.),(1.,1.),(1.,1.),(1.,1.),(1.,1.),(1.,1.),(1.,
1.),(1.,1.),(1.,1.),(1.,1.),(1.,1.),(1.,1.),(1.,1.),(1.,1.),(1.,1.),(1.,
1.),(1.,1.),(1.,1.),(1.,1.),(1.,1.),(1.,1.),(1.,1.),(1.,1.),(1.,1.),(1.,
1.),(1.,1.),(1.,1.),(1.,1.),(1.,1.),(1.,1.),(1.,1.),(1.,1.),(1.,1.),(1.,
1.),(1.,1.),(1.,1.),(1.,1.),(1.,1.),(1.,1.),(1.,1.),(1.,1.),(1.,1.),(1.,
1.),(1.,1.),(1.,1.),(1.,1.),(1.,1.),(1.,1.),(1.,1.),(1.,1.),(1.,1.),(1.,
1.),(1.,1.),(1.,1.),(1.,1.),(1.,1.),(1.,1.),(1.,1.),(1.,1.),(1.,1.),(1.,
1.),(1.,1.),(1.,1.),(1.,1.),(1.,1.),(1.,1.),(1.,1.),(1.,1.),(1.,1.),(1.,
1.),(1.,1.),(1.,1.),(1.,1.),(1.,1.),(1.,1.),(1.,1.),(1.,1.),(1.,1.),(1.,
1.),(1.,1.),(1.,1.),(1.,1.),(1.,1.),(1.,1.),(1.,1.),(1.,1.),(1.,1.),(1.,
1.),(1.,1.),(1.,1.),(1.,1.),(1.,1.),(1.,1.),(1.,1.),(1.,1.),(1.,1.),(1.,
1.),(1.,1.),(1.,1.),(1.,1.),(1.,1.),(1.,1.),(1.,1.),(1.,1.),(1.,1.),(1.,
1.),(1.,1.),(1.,1.),(1.,1.),(1.,1.),(1.,1.),(1.,1.),(1.,1.),(1.,1.),(1.,
1.),(1.,1.),(1.,1.),(1.,1.),(1.,1.),(1.,1.),(1.,1.),(1.,1.),(1.,1.),(1.,
1.),(1.,1.),(1.,1.),(1.,1.),(1.,1.),(1.,1.),(1.,1.),(1.,1.),(1.,1.),(1.,
1.),(1.,1.),(1.,1.),(1.,1.),(1.,1.),(1.,1.),(1.,1.),(1.,1.),(1.,1.),(1.,
1.),(1.,1.),(1.,1.),(1.,1.),(1.,1.),(1.,1.),(1.,1.),(1.,1.),(1.,1.),(1.,
1.),(1.,1.),(1.,1.),(1.,1.),(1.,1.),(1.,1.),(1.,1.),(1.,1.),(1.,1.),(1.,
1.),(1.,1.),(1.,1.),(1.,1.),(1.,1.),(1.,1.),(1.,1.),(1.,1.),(1.,1.),(1.,
1.),(1.,1.),(1.,1.),(1.,1.),(1.,1.),(1.,1.),(1.,1.),(1.,1.),(1.,1.),(1.,
1.),(1.,1.),(1.,1.),(1.,1.),(1.,1.),(1.,1.),(1.,1.),(1.,1.),(1.,1.),(1.,
1.),(1.,1.),(1.,1.),(1.,1.),(1.,1.),(1.,1.),(1.,1.),(1.,1.),(1.,1.),(1.,
1.),(1.,1.),(1.,1.),(1.,1.),(1.,1.),(1.,1.),(1.,1.),(1.,1.),(1.,1.),(1.,
1.),(1.,1.),(1.,1.),(1.,1.),(1.,1.),(1.,1.),(1.,1.),(1.,1.),(1.,1.),(1.,
1.),(1.,1.),(1.,1.),(1.,1.),(1.,1.),(1.,1.),(1.,1.),(1.,1.),(1.,1.),(1.,
1.),(1.,1.),(1.,1.),(1.,1.),(1.,1.),(1.,1.),(1.,1.),(1.,1.),(1.,1.),(1.,
1.),(1.,1.),(1.,1.),(1.,1.),(1.,1.),(1.,1.),(1.,1.),(1.,1.),(1.,1.),(1.,
1.),(1.,1.),(1.,1.),(1.,1.),(1.,1.),(1.,1.),(1.,1.),(1.,1.),(1.,1.),(1.,
1.),(1.,1.),(1.,1.),(1.,1.),(1.,1.),(1.,1.),(1.,1.),(1.,1.),(1.,1.),(1.,
1.),(1.,1.),(1.,1.),(1.,1.),(1.,1.),(1.,1.),(1.,1.),(1.,1.),(1.,1.),(1.,
1.),(1.,1.),(1.,1.),(1.,1.),(1.,1.),(1.,1.),(1.,1.),(1.,1.),(1.,1.),(1.,
1.),(1.,1.),(1.,1.),(1.,1.),(1.,1.),(1.,1.),(1.,1.),(1.,1.),(1.,1.),(1.,
1.),(1.,1.),(1.,1.),(1.,1.),(1.,1.),(1.,1.),(1.,1.),(1.,1.),(1.,1.),(1.,
1.),(1.,1.),(1.,1.),(1.,1.),(1.,1.),(1.,1.),(1.,1.),(1.,1.),(1.,1.),(1.,
1.),(1.,1.),(1.,1.),(1.,1.),(1.,1.),(1.,1.),(1.,1.),(1.,1.),(1.,1.),(1.,
1.),(1.,1.),(1.,1.),(1.,1.),(1.,1.),(1.,1.),(1.,1.),(1.,1.),(1.,1.),(1.,
1.),(1.,1.),(1.,1.),(1.,1.),(1.,1.),(1.,1.),(1.,1.),(1.,1.),(1.,1.),(1.,
1.),(1.,1.),(1.,1.),(1.,1.),(1.,1.),(1.,1.),(1.,1.),(1.,1.),(1.,1.),(1.,
1.),(1.,1.),(1.,1.),(1.,1.),(1.,1.),(1.,1.),(1.,1.),(1.,1.),(1.,1.),(1.,
1.),(1.,1.),(1.,1.),(1.,1.),(1.,1.),(1.,1.),(1.,1.),(1.,1.),(1.,1.),(1.,
1.),(1.,1.),(1.,1.),(1.,1.),(1.,1.),(1.,1.),(1.,1.),(1.,1.),(1.,1.),(1.,
1.),(1.,1.),(1.,1.),(1.,1.),(1.,1.),(1.,1.),(1.,1.),(1.,1.),(1.,1.),(1.,
1.),(1.,1.),(1.,1.),(1.,1.),(1.,1.),(1.,1.),(1.,1.),(1.,1.),(1.,1.),(1.,
1.),(1.,1.),(1.,1.),(1.,1.),(1.,1.),(1.,1.),(1.,1.),(1.,1.),(1.,1.),(1.,
1.),(1.,1.),(1.,1.),(1.,1.),(1.,1.),(1.,1.),(1.,1.),(1.,1.),(1.,1.),(1.,
1.),(1.,1.),(1.,1.),(1.,1.),(1.,1.),(1.,1.),(1.,1.),(1.,1.),(1.,1.),(1.,
1.),(1.,1.),(1.,1.),(1.,1.),(1.,1.),(1.,1.),(1.,1.),(1.,1.),(1.,1.),(1.,
1.),(1.,1.),(1.,1.),(1.,1.),(1.,1.),(1.,1.),(1.,1.),(1.,1.),(1.,1.),(1.,
1.),(1.,1.),(1.,1.),(1.,1.),(1.,1.),(1.,1.),(1.,1.),(1.,1.),(1.,1.),(1.,
1.),(1.,1.),(1.,1.),(1.,1.),(1.,1.),(1.,1.),(1.,1.),(1.,1.),(1.,1.),(1.,
1.),(1.,1.),(1.,1.),(1.,1.),(1.,1.),(1.,1.),(1.,1.),(1.,1.),(1.,1.),(1.,
1.),(1.,1.),(1.,1.),(1.,1.),(1.,1.),(1.,1.),(1.,1.),(1.,1.),(1.,1.),(1.,
1.),(1.,1.),(1.,1.),(1.,1.),(1.,1.),(1.,1.),(1.,1.),(1.,1.),(1.,1.),(1.,
1.),(1.,1.),(1.,1.),(1.,1.),(1.,1.),(1.,1.),(1.,1.),(1.,1.),(1.,1.),(1.,
1.),(1.,1.),(1.,1.),(1.,1.),(1.,1.),(1.,1.),(1.,1.),(1.,1.),(1.,1.),(1.,
1.),(1.,1.),(1.,1.),(1.,1.),(1.,1.),(1.,1.),(1.,1.),(1.,1.),(1.,1.),(1.,
1.),(1.,1.),(1.,1.),(1.,1.),(1.,1.),(1.,1.),(1.,1.),(1.,1.),(1.,1.),(1.,
1.),(1.,1.),(1.,1.),(1.,1.),(1.,1.),(1.,1.),(1.,1.),(1.,1.),(1.,1.),(1.,
1.),(1.,1.),(1.,1.),(1.,1.),(1.,1.),(1.,1.),(1.,1.),(1.,1.),(1.,1.),(1.,
1.),(1.,1.),(1.,1.),(1.,1.),(1.,1.),(1.,1.),(1.,1.),(1.,1.),(1.,1.),(1.,
1.),(1.,1.),(1.,1.),(1.,1.),(1.,1.),(1.,1.),(1.,1.),(1.,1.),(1.,1.),(1.,
1.),(1.,1.),(1.,1.),(1.,1.),(1.,1.),(1.,1.),(1.,1.),(1.,1.),(1.,1.),(1.,
1.),(1.,1.),(1.,1.),(1.,1.),(1.,1.),(1.,1.),(1.,1.),(1.,1.),(1.,1.),(1.,
1.),(1.,1.),(1.,1.),(1.,1.),(1.,1.),(1.,1.),(1.,1.),(1.,1.),(1.,1.),(1.,
1.),(1.,1.),(1.,1.),(1.,1.),(1.,1.),(1.,1.),(1.,1.),(1.,1.),(1.,1.),(1.,
1.),(1.,1.),(1.,1.),(1.,1.),(1.,1.),(1.,1.),(1.,1.),(1.,1.),(1.,1.),(1.,
1.),(1.,1.),(1.,1.),(1.,1.),(1.,1.),(1.,1.),(1.,1.),(1.,1.),(1.,1.),(1.,
1.),(1.,1.),(1.,1.),(1.,1.),(1.,1.),(1.,1.),(1.,1.),(1.,1.),(1.,1.),(1.,
1.),(1.,1.),(1.,1.),(1.,1.),(1.,1.),(1.,1.),(1.,1.),(1.,1.),(1.,1.),(1.,
1.),(1.,1.),(1.,1.),(1.,1.),(1.,1.),(1.,1.),(1.,1.),(1.,1.),(1.,1.),(1.,
1.),(1.,1.),(1.,1.),(1.,1.),(1.,1.),(1.,1.),(1.,1.),(1.,1.),(1.,1.),(1.,
1.),(1.,1.),(1.,1.),(1.,1.),(1.,1.),(1.,1.),(1.,1.),(1.,1.),(1.,1.),(1.,
1.),(1.,1.),(1.,1.),(1.,1.),(1.,1.),(1.,1.),(1.,1.),(1.,1.),(1.,1.),(1.,
1.),(1.,1.),(1.,1.),(1.,1.),(1.,1.),(1.,1.),(1.,1.),(1.,1.),(1.,1.),(1.,
1.),(1.,1.),(1.,1.),(1.,1.),(1.,1.),(1.,1.),(1.,1.),(1.,1.),(1.,1.),(1.,
1.),(1.,1.),(1.,1.),(1.,1.),(1.,1.),(1.,1.),(1.,1.),(1.,1.),(1.,1.),(1.,
1.),(1.,1.),(1.,1.),(1.,1.),(1.,1.),(1.,1.),(1.,1.),(1.,1.),(1.,1.),(1.,
1.),(1.,1.),(1.,1.),(1.,1.),(1.,1.),(1.,1.),(1.,1.),(1.,1.),(1.,1.),(1.,
1.),(1.,1.),(1.,1.),(1.,1.),(1.,1.),(1.,1.),(1.,1.),(1.,1.),(1.,1.),(1.,
1.),(1.,1.),(1.,1.),(1.,1.),(1.,1.),(1.,1.),(1.,1.),(1.,1.),(1.,1.),(1.,
1.),(1.,1.),(1.,1.),(1.,1.),(1.,1.),(1.,1.),(1.,1.),(1.,1.),(1.,1.),(1.,
1.),(1.,1.),(1.,1.),(1.,1.),(1.,1.),(1.,1.),(1.,1.),(1.,1.),(1.,1.),(1.,
1.),(1.,1.),(1.,1.),(1.,1.),(1.,1.),(1.,1.),(1.,1.),(1.,1.),(1.,1.),(1.,
1.),(1.,1.),(1.,1.),(1.,1.),(1.,1.),(1.,1.),(1.,1.),(1.,1.),(1.,1.),(1.,
1.),(1.,1.),(1.,1.),(1.,1.),(1.,1.),(1.,1.),(1.,1.),(1.,1.),(1.,1.),(1.,
1.),(1.,1.),(1.,1.),(1.,1.),(1.,1.),(1.,1.),(1.,1.),(1.,1.),(1.,1.),(1.,
1.),(1.,1.),(1.,1.),(1.,1.),(1.,1.),(1.,1.),(1.,1.),(1.,1.),(1.,1.),(1.,
1.),(1.,1.),(1.,1.),(1.,1.),(1.,1.),(1.,1.),(1.,1.),(1.,1.),(1.,1.),(1.,
1.),(1.,1.),(1.,1.),(1.,1.),(1.,1.),(1.,1.),(1.,1.),(1.,1.),(1.,1.),(1.,
1.),(1.,1.),(1.,1.),(1.,1.),(1.,1.),(1.,1.),(1.,1.),(1.,1.),(1.,1.),(1.,
1.),(1.,1.),(1.,1.),(1.,1.),(1.,1.),(1.,1.),(1.,1.),(1.,1.),(1.,1.),(1.,
1.),(1.,1.),(1.,1.),(1.,1.),(1.,1.),(1.,1.),(1.,1.),(1.,1.),(1.,1.),(1.,
1.),(1.,1.),(1.,1.),(1.,1.),(1.,1.),(1.,1.),(1.,1.),(1.,1.),(1.,1.),(1.,
1.),(1.,1.),(1.,1.),(1.,1.),(1.,1.),(1.,1.),(1.,1.),(1.,1.),(1.,1.),(1.,
1.),(1.,1.),(1.,1.),(1.,1.),(1.,1.),(1.,1.),(1.,1.),(1.,1.),(1.,1.),(1.,
1.),(1.,1.),(1.,1.),(1.,1.),(1.,1.),(1.,1.),(1.,1.),(1.,1.),(1.,1.),(1.,
1.),(1.,1.),(1.,1.),(1.,1.),(1.,1.),(1.,1.),(1.,1.),(1.,1.),(1.,1.),(1.,
1.),(1.,1.),(1.,1.),(1.,1.),(1.,1.),(1.,1.),(1.,1.),(1.,1.),(1.,1.),(1.,
1.),(1.,1.),(1.,1.),(1.,1.),(1.,1.),(1.,1.),(1.,1.),(1.,1.),(1.,1.),(1.,
1.),(1.,1.),(1.,1.),(1.,1.),(1.,1.),(1.,1.),(1.,1.),(1.,1.),(1.,1.),(1.,
1.),(1.,1.),(1.,1.),(1.,1.),(1.,1.),(1.,1.),(1.,1.),(1.,1.),(1.,1.),(1.,
1.),(1.,1.),(1.,1.),(1.,1.),(1.,1.),(1.,1.),(1.,1.),(1.,1.),(1.,1.),(1.,
1.),(1.,1.),(1.,1.),(1.,1.),(1.,1.),(1.,1.),(1.,1.),(1.,1.),(1.,1.),(1.,
1.),(1.,1.),(1.,1.),(1.,1.),(1.,1.),(1.,1.),(1.,1.),(1.,1.),(1.,1.),(1.,
1.)))
REPRESENTATION_ITEM('')
SURFACE()
);
#262=(
BOUNDED_SURFACE()
B_SPLINE_SURFACE(5,1,((#82213,#82214),(#82215,#82216),(#82217,#82218),(#82219,
#82220),(#82221,#82222),(#82223,#82224),(#82225,#82226),(#82227,#82228),
(#82229,#82230),(#82231,#82232),(#82233,#82234),(#82235,#82236),(#82237,
#82238),(#82239,#82240),(#82241,#82242),(#82243,#82244),(#82245,#82246),
(#82247,#82248),(#82249,#82250),(#82251,#82252),(#82253,#82254),(#82255,
#82256),(#82257,#82258),(#82259,#82260),(#82261,#82262),(#82263,#82264),
(#82265,#82266),(#82267,#82268),(#82269,#82270),(#82271,#82272),(#82273,
#82274),(#82275,#82276),(#82277,#82278),(#82279,#82280),(#82281,#82282),
(#82283,#82284),(#82285,#82286),(#82287,#82288),(#82289,#82290),(#82291,
#82292),(#82293,#82294),(#82295,#82296),(#82297,#82298),(#82299,#82300),
(#82301,#82302),(#82303,#82304),(#82305,#82306),(#82307,#82308),(#82309,
#82310),(#82311,#82312),(#82313,#82314),(#82315,#82316),(#82317,#82318),
(#82319,#82320),(#82321,#82322),(#82323,#82324),(#82325,#82326),(#82327,
#82328),(#82329,#82330),(#82331,#82332),(#82333,#82334),(#82335,#82336),
(#82337,#82338),(#82339,#82340),(#82341,#82342),(#82343,#82344),(#82345,
#82346),(#82347,#82348),(#82349,#82350),(#82351,#82352),(#82353,#82354),
(#82355,#82356),(#82357,#82358),(#82359,#82360),(#82361,#82362),(#82363,
#82364),(#82365,#82366),(#82367,#82368),(#82369,#82370),(#82371,#82372),
(#82373,#82374),(#82375,#82376),(#82377,#82378),(#82379,#82380),(#82381,
#82382),(#82383,#82384),(#82385,#82386),(#82387,#82388),(#82389,#82390),
(#82391,#82392),(#82393,#82394),(#82395,#82396),(#82397,#82398),(#82399,
#82400),(#82401,#82402),(#82403,#82404),(#82405,#82406),(#82407,#82408),
(#82409,#82410),(#82411,#82412),(#82413,#82414),(#82415,#82416),(#82417,
#82418),(#82419,#82420),(#82421,#82422),(#82423,#82424),(#82425,#82426),
(#82427,#82428),(#82429,#82430),(#82431,#82432),(#82433,#82434),(#82435,
#82436),(#82437,#82438),(#82439,#82440),(#82441,#82442),(#82443,#82444),
(#82445,#82446),(#82447,#82448),(#82449,#82450),(#82451,#82452),(#82453,
#82454),(#82455,#82456),(#82457,#82458),(#82459,#82460),(#82461,#82462),
(#82463,#82464),(#82465,#82466),(#82467,#82468),(#82469,#82470),(#82471,
#82472),(#82473,#82474),(#82475,#82476),(#82477,#82478),(#82479,#82480),
(#82481,#82482),(#82483,#82484),(#82485,#82486),(#82487,#82488),(#82489,
#82490),(#82491,#82492),(#82493,#82494),(#82495,#82496),(#82497,#82498),
(#82499,#82500),(#82501,#82502),(#82503,#82504),(#82505,#82506),(#82507,
#82508),(#82509,#82510),(#82511,#82512),(#82513,#82514),(#82515,#82516),
(#82517,#82518),(#82519,#82520),(#82521,#82522),(#82523,#82524),(#82525,
#82526),(#82527,#82528),(#82529,#82530),(#82531,#82532),(#82533,#82534),
(#82535,#82536),(#82537,#82538),(#82539,#82540),(#82541,#82542),(#82543,
#82544),(#82545,#82546),(#82547,#82548),(#82549,#82550),(#82551,#82552),
(#82553,#82554),(#82555,#82556),(#82557,#82558),(#82559,#82560),(#82561,
#82562),(#82563,#82564),(#82565,#82566),(#82567,#82568),(#82569,#82570),
(#82571,#82572),(#82573,#82574),(#82575,#82576),(#82577,#82578),(#82579,
#82580),(#82581,#82582),(#82583,#82584),(#82585,#82586),(#82587,#82588),
(#82589,#82590),(#82591,#82592),(#82593,#82594),(#82595,#82596),(#82597,
#82598),(#82599,#82600),(#82601,#82602),(#82603,#82604),(#82605,#82606),
(#82607,#82608),(#82609,#82610),(#82611,#82612),(#82613,#82614),(#82615,
#82616),(#82617,#82618),(#82619,#82620),(#82621,#82622),(#82623,#82624),
(#82625,#82626),(#82627,#82628),(#82629,#82630),(#82631,#82632),(#82633,
#82634),(#82635,#82636),(#82637,#82638),(#82639,#82640),(#82641,#82642),
(#82643,#82644),(#82645,#82646),(#82647,#82648),(#82649,#82650),(#82651,
#82652),(#82653,#82654),(#82655,#82656),(#82657,#82658),(#82659,#82660),
(#82661,#82662),(#82663,#82664),(#82665,#82666),(#82667,#82668),(#82669,
#82670),(#82671,#82672),(#82673,#82674),(#82675,#82676),(#82677,#82678),
(#82679,#82680),(#82681,#82682),(#82683,#82684),(#82685,#82686),(#82687,
#82688),(#82689,#82690),(#82691,#82692),(#82693,#82694),(#82695,#82696),
(#82697,#82698),(#82699,#82700),(#82701,#82702),(#82703,#82704),(#82705,
#82706),(#82707,#82708),(#82709,#82710),(#82711,#82712),(#82713,#82714),
(#82715,#82716),(#82717,#82718),(#82719,#82720),(#82721,#82722),(#82723,
#82724),(#82725,#82726),(#82727,#82728),(#82729,#82730),(#82731,#82732),
(#82733,#82734),(#82735,#82736),(#82737,#82738),(#82739,#82740),(#82741,
#82742),(#82743,#82744),(#82745,#82746),(#82747,#82748),(#82749,#82750),
(#82751,#82752),(#82753,#82754),(#82755,#82756),(#82757,#82758),(#82759,
#82760),(#82761,#82762),(#82763,#82764),(#82765,#82766),(#82767,#82768),
(#82769,#82770),(#82771,#82772),(#82773,#82774),(#82775,#82776),(#82777,
#82778),(#82779,#82780),(#82781,#82782),(#82783,#82784),(#82785,#82786),
(#82787,#82788),(#82789,#82790),(#82791,#82792),(#82793,#82794),(#82795,
#82796),(#82797,#82798),(#82799,#82800),(#82801,#82802),(#82803,#82804),
(#82805,#82806),(#82807,#82808),(#82809,#82810),(#82811,#82812),(#82813,
#82814),(#82815,#82816),(#82817,#82818),(#82819,#82820),(#82821,#82822),
(#82823,#82824),(#82825,#82826),(#82827,#82828),(#82829,#82830),(#82831,
#82832),(#82833,#82834),(#82835,#82836),(#82837,#82838),(#82839,#82840),
(#82841,#82842),(#82843,#82844),(#82845,#82846),(#82847,#82848),(#82849,
#82850),(#82851,#82852),(#82853,#82854),(#82855,#82856),(#82857,#82858),
(#82859,#82860),(#82861,#82862),(#82863,#82864),(#82865,#82866),(#82867,
#82868),(#82869,#82870),(#82871,#82872),(#82873,#82874),(#82875,#82876),
(#82877,#82878),(#82879,#82880),(#82881,#82882),(#82883,#82884),(#82885,
#82886),(#82887,#82888),(#82889,#82890),(#82891,#82892),(#82893,#82894),
(#82895,#82896),(#82897,#82898),(#82899,#82900),(#82901,#82902),(#82903,
#82904),(#82905,#82906),(#82907,#82908),(#82909,#82910),(#82911,#82912),
(#82913,#82914),(#82915,#82916),(#82917,#82918),(#82919,#82920),(#82921,
#82922),(#82923,#82924),(#82925,#82926),(#82927,#82928),(#82929,#82930),
(#82931,#82932),(#82933,#82934),(#82935,#82936),(#82937,#82938),(#82939,
#82940),(#82941,#82942),(#82943,#82944),(#82945,#82946),(#82947,#82948),
(#82949,#82950),(#82951,#82952),(#82953,#82954),(#82955,#82956),(#82957,
#82958),(#82959,#82960),(#82961,#82962),(#82963,#82964),(#82965,#82966),
(#82967,#82968),(#82969,#82970),(#82971,#82972),(#82973,#82974),(#82975,
#82976),(#82977,#82978),(#82979,#82980),(#82981,#82982),(#82983,#82984),
(#82985,#82986),(#82987,#82988),(#82989,#82990),(#82991,#82992),(#82993,
#82994),(#82995,#82996),(#82997,#82998),(#82999,#83000),(#83001,#83002),
(#83003,#83004),(#83005,#83006),(#83007,#83008),(#83009,#83010),(#83011,
#83012),(#83013,#83014),(#83015,#83016),(#83017,#83018),(#83019,#83020),
(#83021,#83022),(#83023,#83024),(#83025,#83026),(#83027,#83028),(#83029,
#83030),(#83031,#83032),(#83033,#83034),(#83035,#83036),(#83037,#83038),
(#83039,#83040),(#83041,#83042),(#83043,#83044),(#83045,#83046),(#83047,
#83048),(#83049,#83050),(#83051,#83052),(#83053,#83054),(#83055,#83056),
(#83057,#83058),(#83059,#83060),(#83061,#83062),(#83063,#83064),(#83065,
#83066),(#83067,#83068),(#83069,#83070),(#83071,#83072),(#83073,#83074),
(#83075,#83076),(#83077,#83078),(#83079,#83080),(#83081,#83082),(#83083,
#83084),(#83085,#83086),(#83087,#83088),(#83089,#83090),(#83091,#83092),
(#83093,#83094),(#83095,#83096),(#83097,#83098),(#83099,#83100),(#83101,
#83102),(#83103,#83104),(#83105,#83106),(#83107,#83108),(#83109,#83110),
(#83111,#83112),(#83113,#83114),(#83115,#83116),(#83117,#83118),(#83119,
#83120),(#83121,#83122),(#83123,#83124),(#83125,#83126),(#83127,#83128),
(#83129,#83130),(#83131,#83132),(#83133,#83134),(#83135,#83136),(#83137,
#83138),(#83139,#83140),(#83141,#83142),(#83143,#83144),(#83145,#83146),
(#83147,#83148),(#83149,#83150),(#83151,#83152),(#83153,#83154),(#83155,
#83156),(#83157,#83158),(#83159,#83160),(#83161,#83162),(#83163,#83164),
(#83165,#83166),(#83167,#83168),(#83169,#83170),(#83171,#83172),(#83173,
#83174),(#83175,#83176),(#83177,#83178),(#83179,#83180),(#83181,#83182),
(#83183,#83184),(#83185,#83186),(#83187,#83188),(#83189,#83190),(#83191,
#83192),(#83193,#83194),(#83195,#83196),(#83197,#83198),(#83199,#83200),
(#83201,#83202),(#83203,#83204),(#83205,#83206),(#83207,#83208),(#83209,
#83210),(#83211,#83212),(#83213,#83214),(#83215,#83216),(#83217,#83218),
(#83219,#83220),(#83221,#83222),(#83223,#83224),(#83225,#83226),(#83227,
#83228),(#83229,#83230),(#83231,#83232),(#83233,#83234),(#83235,#83236),
(#83237,#83238),(#83239,#83240),(#83241,#83242),(#83243,#83244),(#83245,
#83246),(#83247,#83248),(#83249,#83250),(#83251,#83252),(#83253,#83254),
(#83255,#83256),(#83257,#83258),(#83259,#83260),(#83261,#83262),(#83263,
#83264),(#83265,#83266),(#83267,#83268),(#83269,#83270),(#83271,#83272),
(#83273,#83274),(#83275,#83276),(#83277,#83278),(#83279,#83280),(#83281,
#83282),(#83283,#83284),(#83285,#83286),(#83287,#83288),(#83289,#83290),
(#83291,#83292),(#83293,#83294),(#83295,#83296),(#83297,#83298),(#83299,
#83300),(#83301,#83302),(#83303,#83304),(#83305,#83306),(#83307,#83308),
(#83309,#83310),(#83311,#83312),(#83313,#83314),(#83315,#83316),(#83317,
#83318),(#83319,#83320),(#83321,#83322),(#83323,#83324),(#83325,#83326),
(#83327,#83328),(#83329,#83330),(#83331,#83332),(#83333,#83334),(#83335,
#83336),(#83337,#83338),(#83339,#83340),(#83341,#83342),(#83343,#83344),
(#83345,#83346),(#83347,#83348),(#83349,#83350),(#83351,#83352),(#83353,
#83354),(#83355,#83356),(#83357,#83358),(#83359,#83360),(#83361,#83362),
(#83363,#83364),(#83365,#83366),(#83367,#83368),(#83369,#83370),(#83371,
#83372),(#83373,#83374),(#83375,#83376),(#83377,#83378),(#83379,#83380),
(#83381,#83382),(#83383,#83384),(#83385,#83386),(#83387,#83388),(#83389,
#83390),(#83391,#83392),(#83393,#83394),(#83395,#83396),(#83397,#83398),
(#83399,#83400),(#83401,#83402),(#83403,#83404),(#83405,#83406),(#83407,
#83408),(#83409,#83410),(#83411,#83412),(#83413,#83414),(#83415,#83416),
(#83417,#83418),(#83419,#83420),(#83421,#83422),(#83423,#83424),(#83425,
#83426),(#83427,#83428),(#83429,#83430),(#83431,#83432),(#83433,#83434),
(#83435,#83436),(#83437,#83438),(#83439,#83440),(#83441,#83442),(#83443,
#83444),(#83445,#83446),(#83447,#83448),(#83449,#83450),(#83451,#83452),
(#83453,#83454),(#83455,#83456),(#83457,#83458),(#83459,#83460),(#83461,
#83462),(#83463,#83464),(#83465,#83466),(#83467,#83468),(#83469,#83470),
(#83471,#83472),(#83473,#83474),(#83475,#83476),(#83477,#83478),(#83479,
#83480),(#83481,#83482),(#83483,#83484),(#83485,#83486),(#83487,#83488),
(#83489,#83490),(#83491,#83492),(#83493,#83494),(#83495,#83496),(#83497,
#83498),(#83499,#83500),(#83501,#83502),(#83503,#83504),(#83505,#83506),
(#83507,#83508),(#83509,#83510),(#83511,#83512),(#83513,#83514),(#83515,
#83516),(#83517,#83518),(#83519,#83520),(#83521,#83522),(#83523,#83524),
(#83525,#83526),(#83527,#83528),(#83529,#83530),(#83531,#83532),(#83533,
#83534),(#83535,#83536),(#83537,#83538),(#83539,#83540),(#83541,#83542),
(#83543,#83544),(#83545,#83546),(#83547,#83548),(#83549,#83550),(#83551,
#83552),(#83553,#83554),(#83555,#83556),(#83557,#83558),(#83559,#83560),
(#83561,#83562),(#83563,#83564),(#83565,#83566),(#83567,#83568),(#83569,
#83570),(#83571,#83572),(#83573,#83574),(#83575,#83576),(#83577,#83578),
(#83579,#83580),(#83581,#83582),(#83583,#83584),(#83585,#83586),(#83587,
#83588),(#83589,#83590),(#83591,#83592),(#83593,#83594),(#83595,#83596),
(#83597,#83598),(#83599,#83600),(#83601,#83602),(#83603,#83604),(#83605,
#83606),(#83607,#83608),(#83609,#83610),(#83611,#83612),(#83613,#83614),
(#83615,#83616),(#83617,#83618),(#83619,#83620),(#83621,#83622),(#83623,
#83624),(#83625,#83626),(#83627,#83628),(#83629,#83630),(#83631,#83632),
(#83633,#83634),(#83635,#83636),(#83637,#83638),(#83639,#83640),(#83641,
#83642),(#83643,#83644),(#83645,#83646),(#83647,#83648),(#83649,#83650),
(#83651,#83652),(#83653,#83654),(#83655,#83656),(#83657,#83658),(#83659,
#83660),(#83661,#83662),(#83663,#83664),(#83665,#83666),(#83667,#83668),
(#83669,#83670),(#83671,#83672),(#83673,#83674),(#83675,#83676),(#83677,
#83678),(#83679,#83680),(#83681,#83682),(#83683,#83684),(#83685,#83686),
(#83687,#83688),(#83689,#83690),(#83691,#83692),(#83693,#83694),(#83695,
#83696),(#83697,#83698),(#83699,#83700),(#83701,#83702),(#83703,#83704),
(#83705,#83706),(#83707,#83708),(#83709,#83710),(#83711,#83712),(#83713,
#83714),(#83715,#83716),(#83717,#83718),(#83719,#83720),(#83721,#83722),
(#83723,#83724),(#83725,#83726),(#83727,#83728),(#83729,#83730),(#83731,
#83732),(#83733,#83734),(#83735,#83736),(#83737,#83738),(#83739,#83740),
(#83741,#83742),(#83743,#83744),(#83745,#83746),(#83747,#83748),(#83749,
#83750),(#83751,#83752),(#83753,#83754),(#83755,#83756),(#83757,#83758),
(#83759,#83760),(#83761,#83762),(#83763,#83764),(#83765,#83766),(#83767,
#83768),(#83769,#83770),(#83771,#83772),(#83773,#83774),(#83775,#83776),
(#83777,#83778),(#83779,#83780),(#83781,#83782),(#83783,#83784),(#83785,
#83786),(#83787,#83788),(#83789,#83790),(#83791,#83792),(#83793,#83794),
(#83795,#83796),(#83797,#83798),(#83799,#83800),(#83801,#83802),(#83803,
#83804),(#83805,#83806),(#83807,#83808),(#83809,#83810),(#83811,#83812),
(#83813,#83814),(#83815,#83816),(#83817,#83818),(#83819,#83820),(#83821,
#83822),(#83823,#83824),(#83825,#83826),(#83827,#83828),(#83829,#83830),
(#83831,#83832),(#83833,#83834),(#83835,#83836),(#83837,#83838),(#83839,
#83840),(#83841,#83842),(#83843,#83844),(#83845,#83846),(#83847,#83848),
(#83849,#83850),(#83851,#83852),(#83853,#83854),(#83855,#83856),(#83857,
#83858),(#83859,#83860),(#83861,#83862),(#83863,#83864),(#83865,#83866),
(#83867,#83868),(#83869,#83870),(#83871,#83872),(#83873,#83874),(#83875,
#83876),(#83877,#83878),(#83879,#83880),(#83881,#83882),(#83883,#83884),
(#83885,#83886),(#83887,#83888),(#83889,#83890),(#83891,#83892),(#83893,
#83894),(#83895,#83896),(#83897,#83898),(#83899,#83900),(#83901,#83902),
(#83903,#83904),(#83905,#83906),(#83907,#83908),(#83909,#83910),(#83911,
#83912),(#83913,#83914),(#83915,#83916),(#83917,#83918),(#83919,#83920),
(#83921,#83922),(#83923,#83924),(#83925,#83926),(#83927,#83928),(#83929,
#83930),(#83931,#83932),(#83933,#83934),(#83935,#83936),(#83937,#83938),
(#83939,#83940),(#83941,#83942),(#83943,#83944),(#83945,#83946),(#83947,
#83948),(#83949,#83950),(#83951,#83952),(#83953,#83954),(#83955,#83956),
(#83957,#83958),(#83959,#83960),(#83961,#83962),(#83963,#83964),(#83965,
#83966),(#83967,#83968),(#83969,#83970),(#83971,#83972),(#83973,#83974),
(#83975,#83976),(#83977,#83978),(#83979,#83980),(#83981,#83982),(#83983,
#83984),(#83985,#83986),(#83987,#83988),(#83989,#83990),(#83991,#83992),
(#83993,#83994),(#83995,#83996),(#83997,#83998),(#83999,#84000),(#84001,
#84002),(#84003,#84004),(#84005,#84006),(#84007,#84008),(#84009,#84010),
(#84011,#84012),(#84013,#84014),(#84015,#84016),(#84017,#84018),(#84019,
#84020),(#84021,#84022),(#84023,#84024),(#84025,#84026),(#84027,#84028),
(#84029,#84030),(#84031,#84032),(#84033,#84034),(#84035,#84036),(#84037,
#84038),(#84039,#84040),(#84041,#84042),(#84043,#84044),(#84045,#84046),
(#84047,#84048),(#84049,#84050),(#84051,#84052),(#84053,#84054),(#84055,
#84056),(#84057,#84058),(#84059,#84060),(#84061,#84062),(#84063,#84064),
(#84065,#84066),(#84067,#84068),(#84069,#84070),(#84071,#84072),(#84073,
#84074),(#84075,#84076),(#84077,#84078),(#84079,#84080),(#84081,#84082),
(#84083,#84084),(#84085,#84086),(#84087,#84088),(#84089,#84090),(#84091,
#84092),(#84093,#84094),(#84095,#84096),(#84097,#84098),(#84099,#84100),
(#84101,#84102),(#84103,#84104),(#84105,#84106),(#84107,#84108),(#84109,
#84110),(#84111,#84112),(#84113,#84114),(#84115,#84116),(#84117,#84118),
(#84119,#84120),(#84121,#84122),(#84123,#84124),(#84125,#84126),(#84127,
#84128),(#84129,#84130),(#84131,#84132),(#84133,#84134),(#84135,#84136),
(#84137,#84138),(#84139,#84140),(#84141,#84142),(#84143,#84144),(#84145,
#84146),(#84147,#84148),(#84149,#84150),(#84151,#84152),(#84153,#84154),
(#84155,#84156),(#84157,#84158),(#84159,#84160),(#84161,#84162),(#84163,
#84164),(#84165,#84166),(#84167,#84168),(#84169,#84170),(#84171,#84172),
(#84173,#84174),(#84175,#84176),(#84177,#84178),(#84179,#84180),(#84181,
#84182),(#84183,#84184),(#84185,#84186),(#84187,#84188),(#84189,#84190),
(#84191,#84192),(#84193,#84194),(#84195,#84196),(#84197,#84198),(#84199,
#84200),(#84201,#84202),(#84203,#84204),(#84205,#84206),(#84207,#84208),
(#84209,#84210),(#84211,#84212),(#84213,#84214),(#84215,#84216),(#84217,
#84218),(#84219,#84220),(#84221,#84222)),.UNSPECIFIED.,.F.,.F.,.F.)
B_SPLINE_SURFACE_WITH_KNOTS((6,1,1,1,1,1,1,1,1,1,1,1,1,1,1,1,1,1,1,1,1,
1,1,1,1,1,1,1,1,1,1,1,1,1,1,1,1,1,1,1,1,1,1,1,1,1,1,1,1,1,1,1,1,1,1,1,1,
1,1,1,1,1,1,1,1,1,1,1,1,1,1,1,1,1,1,1,1,1,1,1,1,1,1,1,1,1,1,1,1,1,1,1,1,
1,1,1,1,1,1,1,1,1,1,1,1,1,1,1,1,1,1,1,1,1,1,1,1,1,1,1,1,1,1,1,1,1,1,1,1,
1,1,1,1,1,1,1,1,1,1,1,1,1,1,1,1,1,1,1,1,1,1,1,1,1,1,1,1,1,1,1,1,1,1,1,1,
1,1,1,1,1,1,1,1,1,1,1,1,1,1,1,1,1,1,1,1,1,1,1,1,1,1,1,1,1,1,1,1,1,1,1,1,
1,1,1,1,1,1,1,1,1,1,1,1,1,1,1,1,1,1,1,1,1,1,1,1,1,1,1,1,1,1,1,1,1,1,1,1,
1,1,1,1,1,1,1,1,1,1,1,1,1,1,1,1,1,1,1,1,1,1,1,1,1,1,1,1,1,1,1,1,1,1,1,1,
1,1,1,1,1,1,1,1,1,1,1,1,1,1,1,1,1,1,1,1,1,1,1,1,1,1,1,1,1,1,1,1,1,1,1,1,
1,1,1,1,1,1,1,1,1,1,1,1,1,1,1,1,1,1,1,1,1,1,1,1,1,1,1,1,1,1,1,1,1,1,1,1,
1,1,1,1,1,1,1,1,1,1,1,1,1,1,1,1,1,1,1,1,1,1,1,1,1,1,1,1,1,1,1,1,1,1,1,1,
1,1,1,1,1,1,1,1,1,1,1,1,1,1,1,1,1,1,1,1,1,1,1,1,1,1,1,1,1,1,1,1,1,1,1,1,
1,1,1,1,1,1,1,1,1,1,1,1,1,1,1,1,1,1,1,1,1,1,1,1,1,1,1,1,1,1,1,1,1,1,1,1,
1,1,1,1,1,1,1,1,1,1,1,1,1,1,1,1,1,1,1,1,1,1,1,1,1,1,1,1,1,1,1,1,1,1,1,1,
1,1,1,1,1,1,1,1,1,1,1,1,1,1,1,1,1,1,1,1,1,1,1,1,1,1,1,1,1,1,1,1,1,1,1,1,
1,1,1,1,1,1,1,1,1,1,1,1,1,1,1,1,1,1,1,1,1,1,1,1,1,1,1,1,1,1,1,1,1,1,1,1,
1,1,1,1,1,1,1,1,1,1,1,1,1,1,1,1,1,1,1,1,1,1,1,1,1,1,1,1,1,1,1,1,1,1,1,1,
1,1,1,1,1,1,1,1,1,1,1,1,1,1,1,1,1,1,1,1,1,1,1,1,1,1,1,1,1,1,1,1,1,1,1,1,
1,1,1,1,1,1,1,1,1,1,1,1,1,1,1,1,1,1,1,1,1,1,1,1,1,1,1,1,1,1,1,1,1,1,1,1,
1,1,1,1,1,1,1,1,1,1,1,1,1,1,1,1,1,1,1,1,1,1,1,1,1,1,1,1,1,1,1,1,1,1,1,1,
1,1,1,1,1,1,1,1,1,1,1,1,1,1,1,1,1,1,1,1,1,1,1,1,1,1,1,1,1,1,1,1,1,1,1,1,
1,1,1,1,1,1,1,1,1,1,1,1,1,1,1,1,1,1,1,1,1,1,1,1,1,1,1,1,1,1,1,1,1,1,1,1,
1,1,1,1,1,1,1,1,1,1,1,1,1,1,1,1,1,1,1,1,1,1,1,1,1,1,1,1,1,1,1,1,1,1,1,1,
1,1,1,1,1,1,1,1,1,1,1,1,1,1,1,1,1,1,1,1,1,1,1,1,1,1,1,1,1,1,1,1,1,1,1,1,
1,1,1,1,1,1,1,1,1,1,1,1,1,1,1,1,1,1,1,1,1,1,1,1,1,1,1,1,1,1,1,1,1,1,1,1,
1,1,1,1,1,1,1,1,1,1,1,1,1,1,1,1,1,1,1,1,1,1,1,1,1,1,1,1,1,1,1,1,1,1,1,1,
1,1,1,1,1,1,1,1,1,1,1,1,1,1,1,1,1,1,1,1,1,1,1,1,1,1,1,1,1,1,1,1,1,1,1,1,
1,1,1,1,1,1,1,1,1,1,1,1,1,1,1,1,1,1,1,1,1,1,1,1,1,1,1,1,1,1,1,1,1,1,1,1,
1,1,1,1,1,1,1,6),(2,2),(-1.,-0.999000000000001,-0.998000000000001,-0.997000000000001,
-0.996000000000001,-0.995000000000001,-0.994000000000001,-0.993000000000001,
-0.992000000000001,-0.991000000000001,-0.990000000000001,-0.989000000000001,
-0.988000000000001,-0.987000000000001,-0.986000000000001,-0.985000000000001,
-0.984000000000001,-0.983000000000001,-0.982000000000001,-0.981000000000001,
-0.980000000000001,-0.979000000000001,-0.978000000000001,-0.977000000000001,
-0.976000000000001,-0.975000000000001,-0.974000000000001,-0.973000000000001,
-0.972000000000001,-0.971000000000001,-0.970000000000001,-0.969000000000001,
-0.968000000000001,-0.967000000000001,-0.966000000000001,-0.965000000000001,
-0.964000000000001,-0.963000000000001,-0.962000000000001,-0.961000000000001,
-0.960000000000001,-0.959000000000001,-0.958000000000001,-0.957000000000001,
-0.956000000000001,-0.955000000000001,-0.954000000000001,-0.953000000000001,
-0.952000000000001,-0.951000000000001,-0.950000000000001,-0.949000000000001,
-0.948000000000001,-0.947000000000001,-0.946000000000001,-0.945000000000001,
-0.944000000000001,-0.943000000000001,-0.942000000000001,-0.941000000000001,
-0.940000000000001,-0.939000000000001,-0.938000000000001,-0.937000000000001,
-0.936000000000001,-0.935000000000001,-0.934000000000001,-0.933000000000001,
-0.932000000000001,-0.931000000000001,-0.930000000000001,-0.929000000000001,
-0.928000000000001,-0.927000000000001,-0.926000000000001,-0.925000000000001,
-0.924000000000001,-0.923000000000001,-0.922000000000001,-0.921000000000001,
-0.920000000000001,-0.919000000000001,-0.918000000000001,-0.917000000000001,
-0.916000000000001,-0.915000000000001,-0.914000000000001,-0.913000000000001,
-0.912000000000001,-0.911000000000001,-0.910000000000001,-0.909000000000001,
-0.908000000000001,-0.907000000000001,-0.906000000000001,-0.905000000000001,
-0.904000000000001,-0.903000000000001,-0.902000000000001,-0.901000000000001,
-0.900000000000001,-0.899000000000001,-0.898000000000001,-0.897000000000001,
-0.896000000000001,-0.895000000000001,-0.894000000000001,-0.893000000000001,
-0.892000000000001,-0.891000000000001,-0.890000000000001,-0.889000000000001,
-0.888000000000001,-0.887000000000001,-0.886000000000001,-0.885000000000001,
-0.884000000000001,-0.883000000000001,-0.882000000000001,-0.881000000000001,
-0.880000000000001,-0.879000000000001,-0.878000000000001,-0.877000000000001,
-0.876000000000001,-0.875000000000001,-0.874000000000001,-0.873000000000001,
-0.872000000000001,-0.871000000000001,-0.870000000000001,-0.869000000000001,
-0.868000000000001,-0.867000000000001,-0.866000000000001,-0.865000000000001,
-0.864000000000001,-0.863000000000001,-0.862000000000001,-0.861000000000001,
-0.860000000000001,-0.859000000000001,-0.858000000000001,-0.857000000000001,
-0.856000000000001,-0.855000000000001,-0.854000000000001,-0.853000000000001,
-0.852000000000001,-0.851000000000001,-0.850000000000001,-0.849000000000001,
-0.848000000000001,-0.847000000000001,-0.846000000000001,-0.845000000000001,
-0.844000000000001,-0.843000000000001,-0.842000000000001,-0.841000000000001,
-0.840000000000001,-0.839000000000001,-0.838000000000001,-0.837000000000001,
-0.836000000000001,-0.835000000000001,-0.834000000000001,-0.833000000000001,
-0.832000000000001,-0.831000000000001,-0.830000000000001,-0.829000000000001,
-0.828000000000001,-0.827000000000001,-0.826000000000001,-0.825000000000001,
-0.824000000000001,-0.823000000000001,-0.822000000000001,-0.821000000000001,
-0.820000000000001,-0.819000000000001,-0.818000000000001,-0.817000000000001,
-0.816000000000001,-0.815000000000001,-0.814000000000001,-0.813000000000001,
-0.812000000000001,-0.811000000000001,-0.810000000000001,-0.809000000000001,
-0.808000000000001,-0.807000000000001,-0.806000000000001,-0.805000000000001,
-0.804000000000001,-0.803000000000001,-0.802000000000001,-0.801000000000001,
-0.800000000000001,-0.799000000000001,-0.798000000000001,-0.797000000000001,
-0.796000000000001,-0.795000000000001,-0.794000000000001,-0.793000000000001,
-0.792000000000001,-0.791000000000001,-0.790000000000001,-0.789000000000001,
-0.788000000000001,-0.787000000000001,-0.786000000000001,-0.785000000000001,
-0.784000000000001,-0.783000000000001,-0.782000000000001,-0.781000000000001,
-0.780000000000001,-0.779000000000001,-0.778000000000001,-0.777000000000001,
-0.776000000000001,-0.775000000000001,-0.774000000000001,-0.773000000000001,
-0.772000000000001,-0.771000000000001,-0.770000000000001,-0.769000000000001,
-0.768000000000001,-0.767000000000001,-0.766000000000001,-0.765000000000001,
-0.764000000000001,-0.763000000000001,-0.762000000000001,-0.761000000000001,
-0.760000000000001,-0.759000000000001,-0.758000000000001,-0.757000000000001,
-0.756000000000001,-0.755000000000001,-0.754000000000001,-0.753000000000001,
-0.752000000000001,-0.751000000000001,-0.750000000000001,-0.749000000000001,
-0.748000000000001,-0.747000000000001,-0.746000000000001,-0.745000000000001,
-0.744000000000001,-0.743000000000001,-0.742000000000001,-0.741000000000001,
-0.740000000000001,-0.739000000000001,-0.738000000000001,-0.737000000000001,
-0.736000000000001,-0.735000000000001,-0.734000000000001,-0.733000000000001,
-0.732000000000001,-0.731000000000001,-0.730000000000001,-0.729000000000001,
-0.728000000000001,-0.727000000000001,-0.726000000000001,-0.725000000000001,
-0.724000000000001,-0.723000000000001,-0.722000000000001,-0.721000000000001,
-0.720000000000001,-0.719000000000001,-0.718000000000001,-0.717000000000001,
-0.716000000000001,-0.715000000000001,-0.714000000000001,-0.713000000000001,
-0.712000000000001,-0.711000000000001,-0.710000000000001,-0.709000000000001,
-0.708000000000001,-0.707000000000001,-0.706000000000001,-0.705000000000001,
-0.704000000000001,-0.703000000000001,-0.702000000000001,-0.701000000000001,
-0.700000000000001,-0.699000000000001,-0.698000000000001,-0.697000000000001,
-0.696000000000001,-0.695000000000001,-0.694000000000001,-0.693000000000001,
-0.692000000000001,-0.691000000000001,-0.690000000000001,-0.689000000000001,
-0.688000000000001,-0.687,-0.686,-0.685,-0.684,-0.683,-0.682,-0.681,-0.68,
-0.679,-0.678,-0.677,-0.676,-0.675,-0.674,-0.673,-0.672,-0.671,-0.67,-0.669,
-0.668,-0.667,-0.666,-0.665,-0.664,-0.663,-0.662,-0.661,-0.66,-0.659,-0.658,
-0.657,-0.656,-0.655,-0.654,-0.653,-0.652,-0.651,-0.65,-0.649,-0.648,-0.647,
-0.646,-0.645,-0.644,-0.643,-0.642,-0.641,-0.64,-0.639,-0.638,-0.637,-0.636,
-0.635,-0.634,-0.633,-0.632,-0.631,-0.63,-0.629,-0.628,-0.627,-0.626,-0.625,
-0.624,-0.623,-0.622,-0.621,-0.62,-0.619,-0.618,-0.617,-0.616,-0.615,-0.614,
-0.613,-0.612,-0.611,-0.61,-0.609,-0.608,-0.607,-0.606,-0.605,-0.604,-0.603,
-0.602,-0.601,-0.6,-0.599,-0.598,-0.597,-0.596,-0.595,-0.594,-0.593,-0.592,
-0.591,-0.59,-0.589,-0.588,-0.587,-0.586,-0.585,-0.584,-0.583,-0.582,-0.581,
-0.58,-0.579,-0.578,-0.577,-0.576,-0.575,-0.574,-0.573,-0.572,-0.571,-0.57,
-0.569,-0.568,-0.567,-0.566,-0.565,-0.564,-0.563,-0.562,-0.561,-0.56,-0.559,
-0.558,-0.557,-0.556,-0.555,-0.554,-0.553,-0.552,-0.551,-0.55,-0.549,-0.548,
-0.547,-0.546,-0.545,-0.544,-0.543,-0.542,-0.541,-0.54,-0.539,-0.538,-0.537,
-0.536,-0.535,-0.534,-0.533,-0.532,-0.531,-0.53,-0.529,-0.528,-0.527,-0.526,
-0.525,-0.524,-0.523,-0.522,-0.521,-0.52,-0.519,-0.518,-0.517,-0.516,-0.515,
-0.514,-0.513,-0.512,-0.511,-0.51,-0.509,-0.508,-0.507,-0.506,-0.505,-0.504,
-0.503,-0.502,-0.501,-0.5,-0.499,-0.498,-0.497,-0.496,-0.495,-0.494,-0.493,
-0.492,-0.491,-0.49,-0.489,-0.488,-0.487,-0.486,-0.485,-0.484,-0.483,-0.482,
-0.481,-0.48,-0.479,-0.478,-0.477,-0.476,-0.475,-0.474,-0.473,-0.472,-0.471,
-0.47,-0.469,-0.468,-0.467,-0.466,-0.465,-0.464,-0.463,-0.462,-0.461,-0.46,
-0.459,-0.458,-0.457,-0.456,-0.455,-0.454,-0.453,-0.452,-0.451,-0.45,-0.449,
-0.448,-0.447,-0.446,-0.445,-0.444,-0.443,-0.442,-0.441,-0.44,-0.439,-0.438,
-0.437,-0.436,-0.435,-0.434,-0.433,-0.432,-0.431,-0.43,-0.429,-0.428,-0.427,
-0.426,-0.425,-0.424,-0.423,-0.422,-0.421,-0.42,-0.419,-0.418,-0.417,-0.416,
-0.415,-0.414,-0.413,-0.412,-0.411,-0.41,-0.409,-0.408,-0.407,-0.406,-0.405,
-0.404,-0.403,-0.402,-0.401,-0.4,-0.399,-0.398,-0.397,-0.396,-0.395,-0.394,
-0.393,-0.392,-0.391,-0.39,-0.389,-0.388,-0.387,-0.386,-0.385,-0.384,-0.383,
-0.382,-0.381,-0.38,-0.379,-0.378,-0.377,-0.376,-0.375,-0.374,-0.373,-0.372,
-0.371,-0.37,-0.369,-0.368,-0.367,-0.366,-0.365,-0.364,-0.363,-0.362,-0.361,
-0.36,-0.359,-0.358,-0.357,-0.356,-0.355,-0.354,-0.353,-0.352,-0.351,-0.35,
-0.349,-0.348,-0.347,-0.346,-0.345,-0.344,-0.343,-0.342,-0.341,-0.34,-0.339,
-0.338,-0.337,-0.336,-0.335,-0.334,-0.333,-0.332,-0.331,-0.33,-0.329,-0.328,
-0.327,-0.326,-0.325,-0.324,-0.323,-0.322,-0.321,-0.32,-0.319,-0.318,-0.317,
-0.316,-0.315,-0.314,-0.313,-0.312,-0.311,-0.31,-0.309,-0.308,-0.307,-0.306,
-0.305,-0.304,-0.303,-0.302,-0.301,-0.3,-0.299,-0.298,-0.297,-0.296,-0.295,
-0.294,-0.293,-0.292,-0.291,-0.29,-0.289,-0.288,-0.287,-0.286,-0.285,-0.284,
-0.283,-0.282,-0.281,-0.28,-0.279,-0.278,-0.277,-0.276,-0.275,-0.274,-0.273,
-0.272,-0.271,-0.27,-0.269,-0.268,-0.267,-0.266,-0.265,-0.264,-0.263,-0.262,
-0.261,-0.26,-0.259,-0.258,-0.257,-0.256,-0.255,-0.254,-0.253,-0.252,-0.251,
-0.25,-0.249,-0.248,-0.247,-0.246,-0.245,-0.244,-0.243,-0.242,-0.241,-0.24,
-0.239,-0.238,-0.237,-0.236,-0.235,-0.234,-0.233,-0.232,-0.231,-0.23,-0.229,
-0.228,-0.227,-0.226,-0.225,-0.224,-0.223,-0.222,-0.221,-0.22,-0.219,-0.218,
-0.217,-0.216,-0.215,-0.214,-0.213,-0.212,-0.211,-0.21,-0.209,-0.208,-0.207,
-0.206,-0.205,-0.204,-0.203,-0.202,-0.201,-0.2,-0.199,-0.198,-0.197,-0.196,
-0.195,-0.194,-0.193,-0.192,-0.191,-0.19,-0.189,-0.188,-0.187,-0.186,-0.185,
-0.184,-0.183,-0.182,-0.181,-0.18,-0.179,-0.178,-0.177,-0.176,-0.175,-0.174,
-0.173,-0.172,-0.171,-0.17,-0.169,-0.168,-0.167,-0.166,-0.165,-0.164,-0.163,
-0.162,-0.161,-0.16,-0.159,-0.158,-0.157,-0.156,-0.155,-0.154,-0.153,-0.152,
-0.151,-0.15,-0.149,-0.148,-0.147,-0.146,-0.145,-0.144,-0.143,-0.142,-0.141,
-0.14,-0.139,-0.138,-0.137,-0.136,-0.135,-0.134,-0.133,-0.132,-0.131,-0.13,
-0.129,-0.128,-0.127,-0.126,-0.125,-0.124,-0.123,-0.122,-0.121,-0.12,-0.119,
-0.118,-0.117,-0.116,-0.115,-0.114,-0.113,-0.112,-0.111,-0.11,-0.109,-0.108,
-0.107,-0.106,-0.105,-0.104,-0.103,-0.102,-0.101,-0.1,-0.0990000000000001,
-0.0980000000000001,-0.0970000000000001,-0.0960000000000001,-0.0950000000000001,
-0.0940000000000001,-0.0930000000000001,-0.0920000000000001,-0.0910000000000001,
-0.0900000000000001,-0.0890000000000001,-0.0880000000000001,-0.0870000000000001,
-0.0860000000000001,-0.0850000000000001,-0.0840000000000001,-0.0830000000000001,
-0.0820000000000001,-0.0810000000000001,-0.0800000000000001,-0.0790000000000001,
-0.0780000000000001,-0.0770000000000001,-0.0760000000000001,-0.0750000000000001,
-0.0740000000000001,-0.0730000000000001,-0.0720000000000001,-0.071,-0.07,
-0.069,-0.068,-0.067,-0.066,-0.065,-0.064,-0.063,-0.062,-0.061,-0.06,-0.059,
-0.058,-0.057,-0.056,-0.055,-0.054,-0.053,-0.052,-0.051,-0.05,-0.049,-0.048,
-0.047,-0.046,-0.045,-0.044,-0.043,-0.042,-0.041,-0.04,-0.039,-0.038,-0.037,
-0.036,-0.035,-0.034,-0.033,-0.032,-0.031,-0.03,-0.029,-0.028,-0.027,-0.026,
-0.025,-0.024,-0.023,-0.022,-0.021,-0.02,-0.019,-0.018,-0.017,-0.016,-0.015,
-0.014,-0.013,-0.012,-0.011,-0.01,-0.009,-0.008,-0.007,-0.006,-0.005,-0.004,
-0.003,-0.002,-0.001,0.),(0.,2.),.UNSPECIFIED.)
GEOMETRIC_REPRESENTATION_ITEM()
RATIONAL_B_SPLINE_SURFACE(((1.,1.),(1.,1.),(1.,1.),(1.,1.),(1.,1.),(1.,
1.),(1.,1.),(1.,1.),(1.,1.),(1.,1.),(1.,1.),(1.,1.),(1.,1.),(1.,1.),(1.,
1.),(1.,1.),(1.,1.),(1.,1.),(1.,1.),(1.,1.),(1.,1.),(1.,1.),(1.,1.),(1.,
1.),(1.,1.),(1.,1.),(1.,1.),(1.,1.),(1.,1.),(1.,1.),(1.,1.),(1.,1.),(1.,
1.),(1.,1.),(1.,1.),(1.,1.),(1.,1.),(1.,1.),(1.,1.),(1.,1.),(1.,1.),(1.,
1.),(1.,1.),(1.,1.),(1.,1.),(1.,1.),(1.,1.),(1.,1.),(1.,1.),(1.,1.),(1.,
1.),(1.,1.),(1.,1.),(1.,1.),(1.,1.),(1.,1.),(1.,1.),(1.,1.),(1.,1.),(1.,
1.),(1.,1.),(1.,1.),(1.,1.),(1.,1.),(1.,1.),(1.,1.),(1.,1.),(1.,1.),(1.,
1.),(1.,1.),(1.,1.),(1.,1.),(1.,1.),(1.,1.),(1.,1.),(1.,1.),(1.,1.),(1.,
1.),(1.,1.),(1.,1.),(1.,1.),(1.,1.),(1.,1.),(1.,1.),(1.,1.),(1.,1.),(1.,
1.),(1.,1.),(1.,1.),(1.,1.),(1.,1.),(1.,1.),(1.,1.),(1.,1.),(1.,1.),(1.,
1.),(1.,1.),(1.,1.),(1.,1.),(1.,1.),(1.,1.),(1.,1.),(1.,1.),(1.,1.),(1.,
1.),(1.,1.),(1.,1.),(1.,1.),(1.,1.),(1.,1.),(1.,1.),(1.,1.),(1.,1.),(1.,
1.),(1.,1.),(1.,1.),(1.,1.),(1.,1.),(1.,1.),(1.,1.),(1.,1.),(1.,1.),(1.,
1.),(1.,1.),(1.,1.),(1.,1.),(1.,1.),(1.,1.),(1.,1.),(1.,1.),(1.,1.),(1.,
1.),(1.,1.),(1.,1.),(1.,1.),(1.,1.),(1.,1.),(1.,1.),(1.,1.),(1.,1.),(1.,
1.),(1.,1.),(1.,1.),(1.,1.),(1.,1.),(1.,1.),(1.,1.),(1.,1.),(1.,1.),(1.,
1.),(1.,1.),(1.,1.),(1.,1.),(1.,1.),(1.,1.),(1.,1.),(1.,1.),(1.,1.),(1.,
1.),(1.,1.),(1.,1.),(1.,1.),(1.,1.),(1.,1.),(1.,1.),(1.,1.),(1.,1.),(1.,
1.),(1.,1.),(1.,1.),(1.,1.),(1.,1.),(1.,1.),(1.,1.),(1.,1.),(1.,1.),(1.,
1.),(1.,1.),(1.,1.),(1.,1.),(1.,1.),(1.,1.),(1.,1.),(1.,1.),(1.,1.),(1.,
1.),(1.,1.),(1.,1.),(1.,1.),(1.,1.),(1.,1.),(1.,1.),(1.,1.),(1.,1.),(1.,
1.),(1.,1.),(1.,1.),(1.,1.),(1.,1.),(1.,1.),(1.,1.),(1.,1.),(1.,1.),(1.,
1.),(1.,1.),(1.,1.),(1.,1.),(1.,1.),(1.,1.),(1.,1.),(1.,1.),(1.,1.),(1.,
1.),(1.,1.),(1.,1.),(1.,1.),(1.,1.),(1.,1.),(1.,1.),(1.,1.),(1.,1.),(1.,
1.),(1.,1.),(1.,1.),(1.,1.),(1.,1.),(1.,1.),(1.,1.),(1.,1.),(1.,1.),(1.,
1.),(1.,1.),(1.,1.),(1.,1.),(1.,1.),(1.,1.),(1.,1.),(1.,1.),(1.,1.),(1.,
1.),(1.,1.),(1.,1.),(1.,1.),(1.,1.),(1.,1.),(1.,1.),(1.,1.),(1.,1.),(1.,
1.),(1.,1.),(1.,1.),(1.,1.),(1.,1.),(1.,1.),(1.,1.),(1.,1.),(1.,1.),(1.,
1.),(1.,1.),(1.,1.),(1.,1.),(1.,1.),(1.,1.),(1.,1.),(1.,1.),(1.,1.),(1.,
1.),(1.,1.),(1.,1.),(1.,1.),(1.,1.),(1.,1.),(1.,1.),(1.,1.),(1.,1.),(1.,
1.),(1.,1.),(1.,1.),(1.,1.),(1.,1.),(1.,1.),(1.,1.),(1.,1.),(1.,1.),(1.,
1.),(1.,1.),(1.,1.),(1.,1.),(1.,1.),(1.,1.),(1.,1.),(1.,1.),(1.,1.),(1.,
1.),(1.,1.),(1.,1.),(1.,1.),(1.,1.),(1.,1.),(1.,1.),(1.,1.),(1.,1.),(1.,
1.),(1.,1.),(1.,1.),(1.,1.),(1.,1.),(1.,1.),(1.,1.),(1.,1.),(1.,1.),(1.,
1.),(1.,1.),(1.,1.),(1.,1.),(1.,1.),(1.,1.),(1.,1.),(1.,1.),(1.,1.),(1.,
1.),(1.,1.),(1.,1.),(1.,1.),(1.,1.),(1.,1.),(1.,1.),(1.,1.),(1.,1.),(1.,
1.),(1.,1.),(1.,1.),(1.,1.),(1.,1.),(1.,1.),(1.,1.),(1.,1.),(1.,1.),(1.,
1.),(1.,1.),(1.,1.),(1.,1.),(1.,1.),(1.,1.),(1.,1.),(1.,1.),(1.,1.),(1.,
1.),(1.,1.),(1.,1.),(1.,1.),(1.,1.),(1.,1.),(1.,1.),(1.,1.),(1.,1.),(1.,
1.),(1.,1.),(1.,1.),(1.,1.),(1.,1.),(1.,1.),(1.,1.),(1.,1.),(1.,1.),(1.,
1.),(1.,1.),(1.,1.),(1.,1.),(1.,1.),(1.,1.),(1.,1.),(1.,1.),(1.,1.),(1.,
1.),(1.,1.),(1.,1.),(1.,1.),(1.,1.),(1.,1.),(1.,1.),(1.,1.),(1.,1.),(1.,
1.),(1.,1.),(1.,1.),(1.,1.),(1.,1.),(1.,1.),(1.,1.),(1.,1.),(1.,1.),(1.,
1.),(1.,1.),(1.,1.),(1.,1.),(1.,1.),(1.,1.),(1.,1.),(1.,1.),(1.,1.),(1.,
1.),(1.,1.),(1.,1.),(1.,1.),(1.,1.),(1.,1.),(1.,1.),(1.,1.),(1.,1.),(1.,
1.),(1.,1.),(1.,1.),(1.,1.),(1.,1.),(1.,1.),(1.,1.),(1.,1.),(1.,1.),(1.,
1.),(1.,1.),(1.,1.),(1.,1.),(1.,1.),(1.,1.),(1.,1.),(1.,1.),(1.,1.),(1.,
1.),(1.,1.),(1.,1.),(1.,1.),(1.,1.),(1.,1.),(1.,1.),(1.,1.),(1.,1.),(1.,
1.),(1.,1.),(1.,1.),(1.,1.),(1.,1.),(1.,1.),(1.,1.),(1.,1.),(1.,1.),(1.,
1.),(1.,1.),(1.,1.),(1.,1.),(1.,1.),(1.,1.),(1.,1.),(1.,1.),(1.,1.),(1.,
1.),(1.,1.),(1.,1.),(1.,1.),(1.,1.),(1.,1.),(1.,1.),(1.,1.),(1.,1.),(1.,
1.),(1.,1.),(1.,1.),(1.,1.),(1.,1.),(1.,1.),(1.,1.),(1.,1.),(1.,1.),(1.,
1.),(1.,1.),(1.,1.),(1.,1.),(1.,1.),(1.,1.),(1.,1.),(1.,1.),(1.,1.),(1.,
1.),(1.,1.),(1.,1.),(1.,1.),(1.,1.),(1.,1.),(1.,1.),(1.,1.),(1.,1.),(1.,
1.),(1.,1.),(1.,1.),(1.,1.),(1.,1.),(1.,1.),(1.,1.),(1.,1.),(1.,1.),(1.,
1.),(1.,1.),(1.,1.),(1.,1.),(1.,1.),(1.,1.),(1.,1.),(1.,1.),(1.,1.),(1.,
1.),(1.,1.),(1.,1.),(1.,1.),(1.,1.),(1.,1.),(1.,1.),(1.,1.),(1.,1.),(1.,
1.),(1.,1.),(1.,1.),(1.,1.),(1.,1.),(1.,1.),(1.,1.),(1.,1.),(1.,1.),(1.,
1.),(1.,1.),(1.,1.),(1.,1.),(1.,1.),(1.,1.),(1.,1.),(1.,1.),(1.,1.),(1.,
1.),(1.,1.),(1.,1.),(1.,1.),(1.,1.),(1.,1.),(1.,1.),(1.,1.),(1.,1.),(1.,
1.),(1.,1.),(1.,1.),(1.,1.),(1.,1.),(1.,1.),(1.,1.),(1.,1.),(1.,1.),(1.,
1.),(1.,1.),(1.,1.),(1.,1.),(1.,1.),(1.,1.),(1.,1.),(1.,1.),(1.,1.),(1.,
1.),(1.,1.),(1.,1.),(1.,1.),(1.,1.),(1.,1.),(1.,1.),(1.,1.),(1.,1.),(1.,
1.),(1.,1.),(1.,1.),(1.,1.),(1.,1.),(1.,1.),(1.,1.),(1.,1.),(1.,1.),(1.,
1.),(1.,1.),(1.,1.),(1.,1.),(1.,1.),(1.,1.),(1.,1.),(1.,1.),(1.,1.),(1.,
1.),(1.,1.),(1.,1.),(1.,1.),(1.,1.),(1.,1.),(1.,1.),(1.,1.),(1.,1.),(1.,
1.),(1.,1.),(1.,1.),(1.,1.),(1.,1.),(1.,1.),(1.,1.),(1.,1.),(1.,1.),(1.,
1.),(1.,1.),(1.,1.),(1.,1.),(1.,1.),(1.,1.),(1.,1.),(1.,1.),(1.,1.),(1.,
1.),(1.,1.),(1.,1.),(1.,1.),(1.,1.),(1.,1.),(1.,1.),(1.,1.),(1.,1.),(1.,
1.),(1.,1.),(1.,1.),(1.,1.),(1.,1.),(1.,1.),(1.,1.),(1.,1.),(1.,1.),(1.,
1.),(1.,1.),(1.,1.),(1.,1.),(1.,1.),(1.,1.),(1.,1.),(1.,1.),(1.,1.),(1.,
1.),(1.,1.),(1.,1.),(1.,1.),(1.,1.),(1.,1.),(1.,1.),(1.,1.),(1.,1.),(1.,
1.),(1.,1.),(1.,1.),(1.,1.),(1.,1.),(1.,1.),(1.,1.),(1.,1.),(1.,1.),(1.,
1.),(1.,1.),(1.,1.),(1.,1.),(1.,1.),(1.,1.),(1.,1.),(1.,1.),(1.,1.),(1.,
1.),(1.,1.),(1.,1.),(1.,1.),(1.,1.),(1.,1.),(1.,1.),(1.,1.),(1.,1.),(1.,
1.),(1.,1.),(1.,1.),(1.,1.),(1.,1.),(1.,1.),(1.,1.),(1.,1.),(1.,1.),(1.,
1.),(1.,1.),(1.,1.),(1.,1.),(1.,1.),(1.,1.),(1.,1.),(1.,1.),(1.,1.),(1.,
1.),(1.,1.),(1.,1.),(1.,1.),(1.,1.),(1.,1.),(1.,1.),(1.,1.),(1.,1.),(1.,
1.),(1.,1.),(1.,1.),(1.,1.),(1.,1.),(1.,1.),(1.,1.),(1.,1.),(1.,1.),(1.,
1.),(1.,1.),(1.,1.),(1.,1.),(1.,1.),(1.,1.),(1.,1.),(1.,1.),(1.,1.),(1.,
1.),(1.,1.),(1.,1.),(1.,1.),(1.,1.),(1.,1.),(1.,1.),(1.,1.),(1.,1.),(1.,
1.),(1.,1.),(1.,1.),(1.,1.),(1.,1.),(1.,1.),(1.,1.),(1.,1.),(1.,1.),(1.,
1.),(1.,1.),(1.,1.),(1.,1.),(1.,1.),(1.,1.),(1.,1.),(1.,1.),(1.,1.),(1.,
1.),(1.,1.),(1.,1.),(1.,1.),(1.,1.),(1.,1.),(1.,1.),(1.,1.),(1.,1.),(1.,
1.),(1.,1.),(1.,1.),(1.,1.),(1.,1.),(1.,1.),(1.,1.),(1.,1.),(1.,1.),(1.,
1.),(1.,1.),(1.,1.),(1.,1.),(1.,1.),(1.,1.),(1.,1.),(1.,1.),(1.,1.),(1.,
1.),(1.,1.),(1.,1.),(1.,1.),(1.,1.),(1.,1.),(1.,1.),(1.,1.),(1.,1.),(1.,
1.),(1.,1.),(1.,1.),(1.,1.),(1.,1.),(1.,1.),(1.,1.),(1.,1.),(1.,1.),(1.,
1.),(1.,1.),(1.,1.),(1.,1.),(1.,1.),(1.,1.),(1.,1.),(1.,1.),(1.,1.),(1.,
1.),(1.,1.),(1.,1.),(1.,1.),(1.,1.),(1.,1.),(1.,1.),(1.,1.),(1.,1.),(1.,
1.),(1.,1.),(1.,1.),(1.,1.),(1.,1.),(1.,1.),(1.,1.),(1.,1.),(1.,1.),(1.,
1.),(1.,1.),(1.,1.),(1.,1.),(1.,1.),(1.,1.),(1.,1.),(1.,1.),(1.,1.),(1.,
1.),(1.,1.),(1.,1.),(1.,1.),(1.,1.),(1.,1.),(1.,1.),(1.,1.),(1.,1.),(1.,
1.),(1.,1.),(1.,1.),(1.,1.),(1.,1.),(1.,1.),(1.,1.),(1.,1.),(1.,1.),(1.,
1.),(1.,1.),(1.,1.),(1.,1.),(1.,1.),(1.,1.),(1.,1.),(1.,1.),(1.,1.),(1.,
1.),(1.,1.),(1.,1.),(1.,1.),(1.,1.),(1.,1.),(1.,1.),(1.,1.),(1.,1.),(1.,
1.),(1.,1.),(1.,1.),(1.,1.),(1.,1.),(1.,1.),(1.,1.),(1.,1.),(1.,1.),(1.,
1.),(1.,1.),(1.,1.),(1.,1.),(1.,1.),(1.,1.),(1.,1.),(1.,1.),(1.,1.),(1.,
1.),(1.,1.),(1.,1.),(1.,1.),(1.,1.),(1.,1.),(1.,1.),(1.,1.),(1.,1.),(1.,
1.),(1.,1.),(1.,1.),(1.,1.),(1.,1.),(1.,1.),(1.,1.),(1.,1.),(1.,1.),(1.,
1.),(1.,1.),(1.,1.),(1.,1.),(1.,1.),(1.,1.),(1.,1.),(1.,1.),(1.,1.),(1.,
1.),(1.,1.),(1.,1.),(1.,1.),(1.,1.),(1.,1.),(1.,1.),(1.,1.),(1.,1.),(1.,
1.),(1.,1.),(1.,1.),(1.,1.),(1.,1.),(1.,1.),(1.,1.),(1.,1.),(1.,1.),(1.,
1.),(1.,1.),(1.,1.),(1.,1.),(1.,1.),(1.,1.),(1.,1.),(1.,1.),(1.,1.),(1.,
1.),(1.,1.),(1.,1.),(1.,1.),(1.,1.),(1.,1.),(1.,1.),(1.,1.),(1.,1.),(1.,
1.),(1.,1.),(1.,1.),(1.,1.),(1.,1.),(1.,1.),(1.,1.),(1.,1.),(1.,1.),(1.,
1.),(1.,1.),(1.,1.),(1.,1.),(1.,1.),(1.,1.),(1.,1.),(1.,1.),(1.,1.),(1.,
1.),(1.,1.),(1.,1.),(1.,1.),(1.,1.),(1.,1.),(1.,1.),(1.,1.),(1.,1.),(1.,
1.),(1.,1.),(1.,1.),(1.,1.),(1.,1.),(1.,1.),(1.,1.),(1.,1.),(1.,1.),(1.,
1.),(1.,1.),(1.,1.),(1.,1.),(1.,1.),(1.,1.),(1.,1.),(1.,1.),(1.,1.),(1.,
1.),(1.,1.),(1.,1.),(1.,1.),(1.,1.),(1.,1.),(1.,1.),(1.,1.),(1.,1.),(1.,
1.)))
REPRESENTATION_ITEM('')
SURFACE()
);
#263=(
BOUNDED_SURFACE()
B_SPLINE_SURFACE(5,1,((#84229,#84230),(#84231,#84232),(#84233,#84234),(#84235,
#84236),(#84237,#84238),(#84239,#84240),(#84241,#84242),(#84243,#84244),
(#84245,#84246),(#84247,#84248),(#84249,#84250),(#84251,#84252),(#84253,
#84254),(#84255,#84256),(#84257,#84258),(#84259,#84260),(#84261,#84262),
(#84263,#84264),(#84265,#84266),(#84267,#84268),(#84269,#84270),(#84271,
#84272),(#84273,#84274),(#84275,#84276),(#84277,#84278),(#84279,#84280),
(#84281,#84282),(#84283,#84284),(#84285,#84286),(#84287,#84288),(#84289,
#84290),(#84291,#84292),(#84293,#84294),(#84295,#84296),(#84297,#84298),
(#84299,#84300),(#84301,#84302),(#84303,#84304),(#84305,#84306),(#84307,
#84308),(#84309,#84310),(#84311,#84312),(#84313,#84314),(#84315,#84316),
(#84317,#84318),(#84319,#84320),(#84321,#84322),(#84323,#84324),(#84325,
#84326),(#84327,#84328),(#84329,#84330),(#84331,#84332),(#84333,#84334),
(#84335,#84336),(#84337,#84338),(#84339,#84340),(#84341,#84342),(#84343,
#84344),(#84345,#84346),(#84347,#84348),(#84349,#84350),(#84351,#84352),
(#84353,#84354),(#84355,#84356),(#84357,#84358),(#84359,#84360),(#84361,
#84362),(#84363,#84364),(#84365,#84366),(#84367,#84368),(#84369,#84370),
(#84371,#84372),(#84373,#84374),(#84375,#84376),(#84377,#84378),(#84379,
#84380),(#84381,#84382),(#84383,#84384),(#84385,#84386),(#84387,#84388),
(#84389,#84390),(#84391,#84392),(#84393,#84394),(#84395,#84396),(#84397,
#84398),(#84399,#84400),(#84401,#84402),(#84403,#84404),(#84405,#84406),
(#84407,#84408),(#84409,#84410),(#84411,#84412),(#84413,#84414),(#84415,
#84416),(#84417,#84418),(#84419,#84420),(#84421,#84422),(#84423,#84424),
(#84425,#84426),(#84427,#84428),(#84429,#84430),(#84431,#84432),(#84433,
#84434),(#84435,#84436),(#84437,#84438),(#84439,#84440),(#84441,#84442),
(#84443,#84444),(#84445,#84446),(#84447,#84448),(#84449,#84450),(#84451,
#84452),(#84453,#84454),(#84455,#84456),(#84457,#84458),(#84459,#84460),
(#84461,#84462),(#84463,#84464),(#84465,#84466),(#84467,#84468),(#84469,
#84470),(#84471,#84472),(#84473,#84474),(#84475,#84476),(#84477,#84478),
(#84479,#84480),(#84481,#84482),(#84483,#84484),(#84485,#84486),(#84487,
#84488),(#84489,#84490),(#84491,#84492),(#84493,#84494),(#84495,#84496),
(#84497,#84498),(#84499,#84500),(#84501,#84502),(#84503,#84504),(#84505,
#84506),(#84507,#84508),(#84509,#84510),(#84511,#84512),(#84513,#84514),
(#84515,#84516),(#84517,#84518),(#84519,#84520),(#84521,#84522),(#84523,
#84524),(#84525,#84526),(#84527,#84528),(#84529,#84530),(#84531,#84532),
(#84533,#84534),(#84535,#84536),(#84537,#84538),(#84539,#84540),(#84541,
#84542),(#84543,#84544),(#84545,#84546),(#84547,#84548),(#84549,#84550),
(#84551,#84552),(#84553,#84554),(#84555,#84556),(#84557,#84558),(#84559,
#84560),(#84561,#84562),(#84563,#84564),(#84565,#84566),(#84567,#84568),
(#84569,#84570),(#84571,#84572),(#84573,#84574),(#84575,#84576),(#84577,
#84578),(#84579,#84580),(#84581,#84582),(#84583,#84584),(#84585,#84586),
(#84587,#84588),(#84589,#84590),(#84591,#84592),(#84593,#84594),(#84595,
#84596),(#84597,#84598),(#84599,#84600),(#84601,#84602),(#84603,#84604),
(#84605,#84606),(#84607,#84608),(#84609,#84610),(#84611,#84612),(#84613,
#84614),(#84615,#84616),(#84617,#84618),(#84619,#84620),(#84621,#84622),
(#84623,#84624),(#84625,#84626),(#84627,#84628),(#84629,#84630),(#84631,
#84632),(#84633,#84634),(#84635,#84636),(#84637,#84638),(#84639,#84640),
(#84641,#84642),(#84643,#84644),(#84645,#84646),(#84647,#84648),(#84649,
#84650),(#84651,#84652),(#84653,#84654),(#84655,#84656),(#84657,#84658),
(#84659,#84660),(#84661,#84662),(#84663,#84664),(#84665,#84666),(#84667,
#84668),(#84669,#84670),(#84671,#84672),(#84673,#84674),(#84675,#84676),
(#84677,#84678),(#84679,#84680),(#84681,#84682),(#84683,#84684),(#84685,
#84686),(#84687,#84688),(#84689,#84690),(#84691,#84692),(#84693,#84694),
(#84695,#84696),(#84697,#84698),(#84699,#84700),(#84701,#84702),(#84703,
#84704),(#84705,#84706),(#84707,#84708),(#84709,#84710),(#84711,#84712),
(#84713,#84714),(#84715,#84716),(#84717,#84718),(#84719,#84720),(#84721,
#84722),(#84723,#84724),(#84725,#84726),(#84727,#84728),(#84729,#84730),
(#84731,#84732),(#84733,#84734),(#84735,#84736),(#84737,#84738),(#84739,
#84740),(#84741,#84742),(#84743,#84744),(#84745,#84746),(#84747,#84748),
(#84749,#84750),(#84751,#84752),(#84753,#84754),(#84755,#84756),(#84757,
#84758),(#84759,#84760),(#84761,#84762),(#84763,#84764),(#84765,#84766),
(#84767,#84768),(#84769,#84770),(#84771,#84772),(#84773,#84774),(#84775,
#84776),(#84777,#84778),(#84779,#84780),(#84781,#84782),(#84783,#84784),
(#84785,#84786),(#84787,#84788),(#84789,#84790),(#84791,#84792),(#84793,
#84794),(#84795,#84796),(#84797,#84798),(#84799,#84800),(#84801,#84802),
(#84803,#84804),(#84805,#84806),(#84807,#84808),(#84809,#84810),(#84811,
#84812),(#84813,#84814),(#84815,#84816),(#84817,#84818),(#84819,#84820),
(#84821,#84822),(#84823,#84824),(#84825,#84826),(#84827,#84828),(#84829,
#84830),(#84831,#84832),(#84833,#84834),(#84835,#84836),(#84837,#84838),
(#84839,#84840),(#84841,#84842),(#84843,#84844),(#84845,#84846),(#84847,
#84848),(#84849,#84850),(#84851,#84852),(#84853,#84854),(#84855,#84856),
(#84857,#84858),(#84859,#84860),(#84861,#84862),(#84863,#84864),(#84865,
#84866),(#84867,#84868),(#84869,#84870),(#84871,#84872),(#84873,#84874),
(#84875,#84876),(#84877,#84878),(#84879,#84880),(#84881,#84882),(#84883,
#84884),(#84885,#84886),(#84887,#84888),(#84889,#84890),(#84891,#84892),
(#84893,#84894),(#84895,#84896),(#84897,#84898),(#84899,#84900),(#84901,
#84902),(#84903,#84904),(#84905,#84906),(#84907,#84908),(#84909,#84910),
(#84911,#84912),(#84913,#84914),(#84915,#84916),(#84917,#84918),(#84919,
#84920),(#84921,#84922),(#84923,#84924),(#84925,#84926),(#84927,#84928),
(#84929,#84930),(#84931,#84932),(#84933,#84934),(#84935,#84936),(#84937,
#84938),(#84939,#84940),(#84941,#84942),(#84943,#84944),(#84945,#84946),
(#84947,#84948),(#84949,#84950),(#84951,#84952),(#84953,#84954),(#84955,
#84956),(#84957,#84958),(#84959,#84960),(#84961,#84962),(#84963,#84964),
(#84965,#84966),(#84967,#84968),(#84969,#84970),(#84971,#84972),(#84973,
#84974),(#84975,#84976),(#84977,#84978),(#84979,#84980),(#84981,#84982),
(#84983,#84984),(#84985,#84986),(#84987,#84988),(#84989,#84990),(#84991,
#84992),(#84993,#84994),(#84995,#84996),(#84997,#84998),(#84999,#85000),
(#85001,#85002),(#85003,#85004),(#85005,#85006),(#85007,#85008),(#85009,
#85010),(#85011,#85012),(#85013,#85014),(#85015,#85016),(#85017,#85018),
(#85019,#85020),(#85021,#85022),(#85023,#85024),(#85025,#85026),(#85027,
#85028),(#85029,#85030),(#85031,#85032),(#85033,#85034),(#85035,#85036),
(#85037,#85038),(#85039,#85040),(#85041,#85042),(#85043,#85044),(#85045,
#85046),(#85047,#85048),(#85049,#85050),(#85051,#85052),(#85053,#85054),
(#85055,#85056),(#85057,#85058),(#85059,#85060),(#85061,#85062),(#85063,
#85064),(#85065,#85066),(#85067,#85068),(#85069,#85070),(#85071,#85072),
(#85073,#85074),(#85075,#85076),(#85077,#85078),(#85079,#85080),(#85081,
#85082),(#85083,#85084),(#85085,#85086),(#85087,#85088),(#85089,#85090),
(#85091,#85092),(#85093,#85094),(#85095,#85096),(#85097,#85098),(#85099,
#85100),(#85101,#85102),(#85103,#85104),(#85105,#85106),(#85107,#85108),
(#85109,#85110),(#85111,#85112),(#85113,#85114),(#85115,#85116),(#85117,
#85118),(#85119,#85120),(#85121,#85122),(#85123,#85124),(#85125,#85126),
(#85127,#85128),(#85129,#85130),(#85131,#85132),(#85133,#85134),(#85135,
#85136),(#85137,#85138),(#85139,#85140),(#85141,#85142),(#85143,#85144),
(#85145,#85146),(#85147,#85148),(#85149,#85150),(#85151,#85152),(#85153,
#85154),(#85155,#85156),(#85157,#85158),(#85159,#85160),(#85161,#85162),
(#85163,#85164),(#85165,#85166),(#85167,#85168),(#85169,#85170),(#85171,
#85172),(#85173,#85174),(#85175,#85176),(#85177,#85178),(#85179,#85180),
(#85181,#85182),(#85183,#85184),(#85185,#85186),(#85187,#85188),(#85189,
#85190),(#85191,#85192),(#85193,#85194),(#85195,#85196),(#85197,#85198),
(#85199,#85200),(#85201,#85202),(#85203,#85204),(#85205,#85206),(#85207,
#85208),(#85209,#85210),(#85211,#85212),(#85213,#85214),(#85215,#85216),
(#85217,#85218),(#85219,#85220),(#85221,#85222),(#85223,#85224),(#85225,
#85226),(#85227,#85228),(#85229,#85230),(#85231,#85232),(#85233,#85234),
(#85235,#85236),(#85237,#85238),(#85239,#85240),(#85241,#85242),(#85243,
#85244),(#85245,#85246),(#85247,#85248),(#85249,#85250),(#85251,#85252),
(#85253,#85254),(#85255,#85256),(#85257,#85258),(#85259,#85260),(#85261,
#85262),(#85263,#85264),(#85265,#85266),(#85267,#85268),(#85269,#85270),
(#85271,#85272),(#85273,#85274),(#85275,#85276),(#85277,#85278),(#85279,
#85280),(#85281,#85282),(#85283,#85284),(#85285,#85286),(#85287,#85288),
(#85289,#85290),(#85291,#85292),(#85293,#85294),(#85295,#85296),(#85297,
#85298),(#85299,#85300),(#85301,#85302),(#85303,#85304),(#85305,#85306),
(#85307,#85308),(#85309,#85310),(#85311,#85312),(#85313,#85314),(#85315,
#85316),(#85317,#85318),(#85319,#85320),(#85321,#85322),(#85323,#85324),
(#85325,#85326),(#85327,#85328),(#85329,#85330),(#85331,#85332),(#85333,
#85334),(#85335,#85336),(#85337,#85338),(#85339,#85340),(#85341,#85342),
(#85343,#85344),(#85345,#85346),(#85347,#85348),(#85349,#85350),(#85351,
#85352),(#85353,#85354),(#85355,#85356),(#85357,#85358),(#85359,#85360),
(#85361,#85362),(#85363,#85364),(#85365,#85366),(#85367,#85368),(#85369,
#85370),(#85371,#85372),(#85373,#85374),(#85375,#85376),(#85377,#85378),
(#85379,#85380),(#85381,#85382),(#85383,#85384),(#85385,#85386),(#85387,
#85388),(#85389,#85390),(#85391,#85392),(#85393,#85394),(#85395,#85396),
(#85397,#85398),(#85399,#85400),(#85401,#85402),(#85403,#85404),(#85405,
#85406),(#85407,#85408),(#85409,#85410),(#85411,#85412),(#85413,#85414),
(#85415,#85416),(#85417,#85418),(#85419,#85420),(#85421,#85422),(#85423,
#85424),(#85425,#85426),(#85427,#85428),(#85429,#85430),(#85431,#85432),
(#85433,#85434),(#85435,#85436),(#85437,#85438),(#85439,#85440),(#85441,
#85442),(#85443,#85444),(#85445,#85446),(#85447,#85448),(#85449,#85450),
(#85451,#85452),(#85453,#85454),(#85455,#85456),(#85457,#85458),(#85459,
#85460),(#85461,#85462),(#85463,#85464),(#85465,#85466),(#85467,#85468),
(#85469,#85470),(#85471,#85472),(#85473,#85474),(#85475,#85476),(#85477,
#85478),(#85479,#85480),(#85481,#85482),(#85483,#85484),(#85485,#85486),
(#85487,#85488),(#85489,#85490),(#85491,#85492),(#85493,#85494),(#85495,
#85496),(#85497,#85498),(#85499,#85500),(#85501,#85502),(#85503,#85504),
(#85505,#85506),(#85507,#85508),(#85509,#85510),(#85511,#85512),(#85513,
#85514),(#85515,#85516),(#85517,#85518),(#85519,#85520),(#85521,#85522),
(#85523,#85524),(#85525,#85526),(#85527,#85528),(#85529,#85530),(#85531,
#85532),(#85533,#85534),(#85535,#85536),(#85537,#85538),(#85539,#85540),
(#85541,#85542),(#85543,#85544),(#85545,#85546),(#85547,#85548),(#85549,
#85550),(#85551,#85552),(#85553,#85554),(#85555,#85556),(#85557,#85558),
(#85559,#85560),(#85561,#85562),(#85563,#85564),(#85565,#85566),(#85567,
#85568),(#85569,#85570),(#85571,#85572),(#85573,#85574),(#85575,#85576),
(#85577,#85578),(#85579,#85580),(#85581,#85582),(#85583,#85584),(#85585,
#85586),(#85587,#85588),(#85589,#85590),(#85591,#85592),(#85593,#85594),
(#85595,#85596),(#85597,#85598),(#85599,#85600),(#85601,#85602),(#85603,
#85604),(#85605,#85606),(#85607,#85608),(#85609,#85610),(#85611,#85612),
(#85613,#85614),(#85615,#85616),(#85617,#85618),(#85619,#85620),(#85621,
#85622),(#85623,#85624),(#85625,#85626),(#85627,#85628),(#85629,#85630),
(#85631,#85632),(#85633,#85634),(#85635,#85636),(#85637,#85638),(#85639,
#85640),(#85641,#85642),(#85643,#85644),(#85645,#85646),(#85647,#85648),
(#85649,#85650),(#85651,#85652),(#85653,#85654),(#85655,#85656),(#85657,
#85658),(#85659,#85660),(#85661,#85662),(#85663,#85664),(#85665,#85666),
(#85667,#85668),(#85669,#85670),(#85671,#85672),(#85673,#85674),(#85675,
#85676),(#85677,#85678),(#85679,#85680),(#85681,#85682),(#85683,#85684),
(#85685,#85686),(#85687,#85688),(#85689,#85690),(#85691,#85692),(#85693,
#85694),(#85695,#85696),(#85697,#85698),(#85699,#85700),(#85701,#85702),
(#85703,#85704),(#85705,#85706),(#85707,#85708),(#85709,#85710),(#85711,
#85712),(#85713,#85714),(#85715,#85716),(#85717,#85718),(#85719,#85720),
(#85721,#85722),(#85723,#85724),(#85725,#85726),(#85727,#85728),(#85729,
#85730),(#85731,#85732),(#85733,#85734),(#85735,#85736),(#85737,#85738),
(#85739,#85740),(#85741,#85742),(#85743,#85744),(#85745,#85746),(#85747,
#85748),(#85749,#85750),(#85751,#85752),(#85753,#85754),(#85755,#85756),
(#85757,#85758),(#85759,#85760),(#85761,#85762),(#85763,#85764),(#85765,
#85766),(#85767,#85768),(#85769,#85770),(#85771,#85772),(#85773,#85774),
(#85775,#85776),(#85777,#85778),(#85779,#85780),(#85781,#85782),(#85783,
#85784),(#85785,#85786),(#85787,#85788),(#85789,#85790),(#85791,#85792),
(#85793,#85794),(#85795,#85796),(#85797,#85798),(#85799,#85800),(#85801,
#85802),(#85803,#85804),(#85805,#85806),(#85807,#85808),(#85809,#85810),
(#85811,#85812),(#85813,#85814),(#85815,#85816),(#85817,#85818),(#85819,
#85820),(#85821,#85822),(#85823,#85824),(#85825,#85826),(#85827,#85828),
(#85829,#85830),(#85831,#85832),(#85833,#85834),(#85835,#85836),(#85837,
#85838),(#85839,#85840),(#85841,#85842),(#85843,#85844),(#85845,#85846),
(#85847,#85848),(#85849,#85850),(#85851,#85852),(#85853,#85854),(#85855,
#85856),(#85857,#85858),(#85859,#85860),(#85861,#85862),(#85863,#85864),
(#85865,#85866),(#85867,#85868),(#85869,#85870),(#85871,#85872),(#85873,
#85874),(#85875,#85876),(#85877,#85878),(#85879,#85880),(#85881,#85882),
(#85883,#85884),(#85885,#85886),(#85887,#85888),(#85889,#85890),(#85891,
#85892),(#85893,#85894),(#85895,#85896),(#85897,#85898),(#85899,#85900),
(#85901,#85902),(#85903,#85904),(#85905,#85906),(#85907,#85908),(#85909,
#85910),(#85911,#85912),(#85913,#85914),(#85915,#85916),(#85917,#85918),
(#85919,#85920),(#85921,#85922),(#85923,#85924),(#85925,#85926),(#85927,
#85928),(#85929,#85930),(#85931,#85932),(#85933,#85934),(#85935,#85936),
(#85937,#85938),(#85939,#85940),(#85941,#85942),(#85943,#85944),(#85945,
#85946),(#85947,#85948),(#85949,#85950),(#85951,#85952),(#85953,#85954),
(#85955,#85956),(#85957,#85958),(#85959,#85960),(#85961,#85962),(#85963,
#85964),(#85965,#85966),(#85967,#85968),(#85969,#85970),(#85971,#85972),
(#85973,#85974),(#85975,#85976),(#85977,#85978),(#85979,#85980),(#85981,
#85982),(#85983,#85984),(#85985,#85986),(#85987,#85988),(#85989,#85990),
(#85991,#85992),(#85993,#85994),(#85995,#85996),(#85997,#85998),(#85999,
#86000),(#86001,#86002),(#86003,#86004),(#86005,#86006),(#86007,#86008),
(#86009,#86010),(#86011,#86012),(#86013,#86014),(#86015,#86016),(#86017,
#86018),(#86019,#86020),(#86021,#86022),(#86023,#86024),(#86025,#86026),
(#86027,#86028),(#86029,#86030),(#86031,#86032),(#86033,#86034),(#86035,
#86036),(#86037,#86038),(#86039,#86040),(#86041,#86042),(#86043,#86044),
(#86045,#86046),(#86047,#86048),(#86049,#86050),(#86051,#86052),(#86053,
#86054),(#86055,#86056),(#86057,#86058),(#86059,#86060),(#86061,#86062),
(#86063,#86064),(#86065,#86066),(#86067,#86068),(#86069,#86070),(#86071,
#86072),(#86073,#86074),(#86075,#86076),(#86077,#86078),(#86079,#86080),
(#86081,#86082),(#86083,#86084),(#86085,#86086),(#86087,#86088),(#86089,
#86090),(#86091,#86092),(#86093,#86094),(#86095,#86096),(#86097,#86098),
(#86099,#86100),(#86101,#86102),(#86103,#86104),(#86105,#86106),(#86107,
#86108),(#86109,#86110),(#86111,#86112),(#86113,#86114),(#86115,#86116),
(#86117,#86118),(#86119,#86120),(#86121,#86122),(#86123,#86124),(#86125,
#86126),(#86127,#86128),(#86129,#86130),(#86131,#86132),(#86133,#86134),
(#86135,#86136),(#86137,#86138),(#86139,#86140),(#86141,#86142),(#86143,
#86144),(#86145,#86146),(#86147,#86148),(#86149,#86150),(#86151,#86152),
(#86153,#86154),(#86155,#86156),(#86157,#86158),(#86159,#86160),(#86161,
#86162),(#86163,#86164),(#86165,#86166),(#86167,#86168),(#86169,#86170),
(#86171,#86172),(#86173,#86174),(#86175,#86176),(#86177,#86178),(#86179,
#86180),(#86181,#86182),(#86183,#86184),(#86185,#86186),(#86187,#86188),
(#86189,#86190),(#86191,#86192),(#86193,#86194),(#86195,#86196),(#86197,
#86198),(#86199,#86200),(#86201,#86202),(#86203,#86204),(#86205,#86206),
(#86207,#86208),(#86209,#86210),(#86211,#86212),(#86213,#86214),(#86215,
#86216),(#86217,#86218),(#86219,#86220),(#86221,#86222),(#86223,#86224),
(#86225,#86226),(#86227,#86228),(#86229,#86230),(#86231,#86232),(#86233,
#86234),(#86235,#86236),(#86237,#86238)),.UNSPECIFIED.,.F.,.F.,.F.)
B_SPLINE_SURFACE_WITH_KNOTS((6,1,1,1,1,1,1,1,1,1,1,1,1,1,1,1,1,1,1,1,1,
1,1,1,1,1,1,1,1,1,1,1,1,1,1,1,1,1,1,1,1,1,1,1,1,1,1,1,1,1,1,1,1,1,1,1,1,
1,1,1,1,1,1,1,1,1,1,1,1,1,1,1,1,1,1,1,1,1,1,1,1,1,1,1,1,1,1,1,1,1,1,1,1,
1,1,1,1,1,1,1,1,1,1,1,1,1,1,1,1,1,1,1,1,1,1,1,1,1,1,1,1,1,1,1,1,1,1,1,1,
1,1,1,1,1,1,1,1,1,1,1,1,1,1,1,1,1,1,1,1,1,1,1,1,1,1,1,1,1,1,1,1,1,1,1,1,
1,1,1,1,1,1,1,1,1,1,1,1,1,1,1,1,1,1,1,1,1,1,1,1,1,1,1,1,1,1,1,1,1,1,1,1,
1,1,1,1,1,1,1,1,1,1,1,1,1,1,1,1,1,1,1,1,1,1,1,1,1,1,1,1,1,1,1,1,1,1,1,1,
1,1,1,1,1,1,1,1,1,1,1,1,1,1,1,1,1,1,1,1,1,1,1,1,1,1,1,1,1,1,1,1,1,1,1,1,
1,1,1,1,1,1,1,1,1,1,1,1,1,1,1,1,1,1,1,1,1,1,1,1,1,1,1,1,1,1,1,1,1,1,1,1,
1,1,1,1,1,1,1,1,1,1,1,1,1,1,1,1,1,1,1,1,1,1,1,1,1,1,1,1,1,1,1,1,1,1,1,1,
1,1,1,1,1,1,1,1,1,1,1,1,1,1,1,1,1,1,1,1,1,1,1,1,1,1,1,1,1,1,1,1,1,1,1,1,
1,1,1,1,1,1,1,1,1,1,1,1,1,1,1,1,1,1,1,1,1,1,1,1,1,1,1,1,1,1,1,1,1,1,1,1,
1,1,1,1,1,1,1,1,1,1,1,1,1,1,1,1,1,1,1,1,1,1,1,1,1,1,1,1,1,1,1,1,1,1,1,1,
1,1,1,1,1,1,1,1,1,1,1,1,1,1,1,1,1,1,1,1,1,1,1,1,1,1,1,1,1,1,1,1,1,1,1,1,
1,1,1,1,1,1,1,1,1,1,1,1,1,1,1,1,1,1,1,1,1,1,1,1,1,1,1,1,1,1,1,1,1,1,1,1,
1,1,1,1,1,1,1,1,1,1,1,1,1,1,1,1,1,1,1,1,1,1,1,1,1,1,1,1,1,1,1,1,1,1,1,1,
1,1,1,1,1,1,1,1,1,1,1,1,1,1,1,1,1,1,1,1,1,1,1,1,1,1,1,1,1,1,1,1,1,1,1,1,
1,1,1,1,1,1,1,1,1,1,1,1,1,1,1,1,1,1,1,1,1,1,1,1,1,1,1,1,1,1,1,1,1,1,1,1,
1,1,1,1,1,1,1,1,1,1,1,1,1,1,1,1,1,1,1,1,1,1,1,1,1,1,1,1,1,1,1,1,1,1,1,1,
1,1,1,1,1,1,1,1,1,1,1,1,1,1,1,1,1,1,1,1,1,1,1,1,1,1,1,1,1,1,1,1,1,1,1,1,
1,1,1,1,1,1,1,1,1,1,1,1,1,1,1,1,1,1,1,1,1,1,1,1,1,1,1,1,1,1,1,1,1,1,1,1,
1,1,1,1,1,1,1,1,1,1,1,1,1,1,1,1,1,1,1,1,1,1,1,1,1,1,1,1,1,1,1,1,1,1,1,1,
1,1,1,1,1,1,1,1,1,1,1,1,1,1,1,1,1,1,1,1,1,1,1,1,1,1,1,1,1,1,1,1,1,1,1,1,
1,1,1,1,1,1,1,1,1,1,1,1,1,1,1,1,1,1,1,1,1,1,1,1,1,1,1,1,1,1,1,1,1,1,1,1,
1,1,1,1,1,1,1,1,1,1,1,1,1,1,1,1,1,1,1,1,1,1,1,1,1,1,1,1,1,1,1,1,1,1,1,1,
1,1,1,1,1,1,1,1,1,1,1,1,1,1,1,1,1,1,1,1,1,1,1,1,1,1,1,1,1,1,1,1,1,1,1,1,
1,1,1,1,1,1,1,1,1,1,1,1,1,1,1,1,1,1,1,1,1,1,1,1,1,1,1,1,1,1,1,1,1,1,1,1,
1,1,1,1,1,1,1,1,1,1,1,1,1,1,1,1,1,1,1,1,1,1,1,1,1,1,1,1,1,1,1,1,1,1,1,1,
1,1,1,1,1,1,1,6),(2,2),(-1.,-0.999000000000001,-0.998000000000001,-0.997000000000001,
-0.996000000000001,-0.995000000000001,-0.994000000000001,-0.993000000000001,
-0.992000000000001,-0.991000000000001,-0.990000000000001,-0.989000000000001,
-0.988000000000001,-0.987000000000001,-0.986000000000001,-0.985000000000001,
-0.984000000000001,-0.983000000000001,-0.982000000000001,-0.981000000000001,
-0.980000000000001,-0.979000000000001,-0.978000000000001,-0.977000000000001,
-0.976000000000001,-0.975000000000001,-0.974000000000001,-0.973000000000001,
-0.972000000000001,-0.971000000000001,-0.970000000000001,-0.969000000000001,
-0.968000000000001,-0.967000000000001,-0.966000000000001,-0.965000000000001,
-0.964000000000001,-0.963000000000001,-0.962000000000001,-0.961000000000001,
-0.960000000000001,-0.959000000000001,-0.958000000000001,-0.957000000000001,
-0.956000000000001,-0.955000000000001,-0.954000000000001,-0.953000000000001,
-0.952000000000001,-0.951000000000001,-0.950000000000001,-0.949000000000001,
-0.948000000000001,-0.947000000000001,-0.946000000000001,-0.945000000000001,
-0.944000000000001,-0.943000000000001,-0.942000000000001,-0.941000000000001,
-0.940000000000001,-0.939000000000001,-0.938000000000001,-0.937000000000001,
-0.936000000000001,-0.935000000000001,-0.934000000000001,-0.933000000000001,
-0.932000000000001,-0.931000000000001,-0.930000000000001,-0.929000000000001,
-0.928000000000001,-0.927000000000001,-0.926000000000001,-0.925000000000001,
-0.924000000000001,-0.923000000000001,-0.922000000000001,-0.921000000000001,
-0.920000000000001,-0.919000000000001,-0.918000000000001,-0.917000000000001,
-0.916000000000001,-0.915000000000001,-0.914000000000001,-0.913000000000001,
-0.912000000000001,-0.911000000000001,-0.910000000000001,-0.909000000000001,
-0.908000000000001,-0.907000000000001,-0.906000000000001,-0.905000000000001,
-0.904000000000001,-0.903000000000001,-0.902000000000001,-0.901000000000001,
-0.900000000000001,-0.899000000000001,-0.898000000000001,-0.897000000000001,
-0.896000000000001,-0.895000000000001,-0.894000000000001,-0.893000000000001,
-0.892000000000001,-0.891000000000001,-0.890000000000001,-0.889000000000001,
-0.888000000000001,-0.887000000000001,-0.886000000000001,-0.885000000000001,
-0.884000000000001,-0.883000000000001,-0.882000000000001,-0.881000000000001,
-0.880000000000001,-0.879000000000001,-0.878000000000001,-0.877000000000001,
-0.876000000000001,-0.875000000000001,-0.874000000000001,-0.873000000000001,
-0.872000000000001,-0.871000000000001,-0.870000000000001,-0.869000000000001,
-0.868000000000001,-0.867000000000001,-0.866000000000001,-0.865000000000001,
-0.864000000000001,-0.863000000000001,-0.862000000000001,-0.861000000000001,
-0.860000000000001,-0.859000000000001,-0.858000000000001,-0.857000000000001,
-0.856000000000001,-0.855000000000001,-0.854000000000001,-0.853000000000001,
-0.852000000000001,-0.851000000000001,-0.850000000000001,-0.849000000000001,
-0.848000000000001,-0.847000000000001,-0.846000000000001,-0.845000000000001,
-0.844000000000001,-0.843000000000001,-0.842000000000001,-0.841000000000001,
-0.840000000000001,-0.839000000000001,-0.838000000000001,-0.837000000000001,
-0.836000000000001,-0.835000000000001,-0.834000000000001,-0.833000000000001,
-0.832000000000001,-0.831000000000001,-0.830000000000001,-0.829000000000001,
-0.828000000000001,-0.827000000000001,-0.826000000000001,-0.825000000000001,
-0.824000000000001,-0.823000000000001,-0.822000000000001,-0.821000000000001,
-0.820000000000001,-0.819000000000001,-0.818000000000001,-0.817000000000001,
-0.816000000000001,-0.815000000000001,-0.814000000000001,-0.813000000000001,
-0.812000000000001,-0.811000000000001,-0.810000000000001,-0.809000000000001,
-0.808000000000001,-0.807000000000001,-0.806000000000001,-0.805000000000001,
-0.804000000000001,-0.803000000000001,-0.802000000000001,-0.801000000000001,
-0.800000000000001,-0.799000000000001,-0.798000000000001,-0.797000000000001,
-0.796000000000001,-0.795000000000001,-0.794000000000001,-0.793000000000001,
-0.792000000000001,-0.791000000000001,-0.790000000000001,-0.789000000000001,
-0.788000000000001,-0.787000000000001,-0.786000000000001,-0.785000000000001,
-0.784000000000001,-0.783000000000001,-0.782000000000001,-0.781000000000001,
-0.780000000000001,-0.779000000000001,-0.778000000000001,-0.777000000000001,
-0.776000000000001,-0.775000000000001,-0.774000000000001,-0.773000000000001,
-0.772000000000001,-0.771000000000001,-0.770000000000001,-0.769000000000001,
-0.768000000000001,-0.767000000000001,-0.766000000000001,-0.765000000000001,
-0.764000000000001,-0.763000000000001,-0.762000000000001,-0.761000000000001,
-0.760000000000001,-0.759000000000001,-0.758000000000001,-0.757000000000001,
-0.756000000000001,-0.755000000000001,-0.754000000000001,-0.753000000000001,
-0.752000000000001,-0.751000000000001,-0.750000000000001,-0.749000000000001,
-0.748000000000001,-0.747000000000001,-0.746000000000001,-0.745000000000001,
-0.744000000000001,-0.743000000000001,-0.742000000000001,-0.741000000000001,
-0.740000000000001,-0.739000000000001,-0.738000000000001,-0.737000000000001,
-0.736000000000001,-0.735000000000001,-0.734000000000001,-0.733000000000001,
-0.732000000000001,-0.731000000000001,-0.730000000000001,-0.729000000000001,
-0.728000000000001,-0.727000000000001,-0.726000000000001,-0.725000000000001,
-0.724000000000001,-0.723000000000001,-0.722000000000001,-0.721000000000001,
-0.720000000000001,-0.719000000000001,-0.718000000000001,-0.717000000000001,
-0.716000000000001,-0.715000000000001,-0.714000000000001,-0.713000000000001,
-0.712000000000001,-0.711000000000001,-0.710000000000001,-0.709000000000001,
-0.708000000000001,-0.707000000000001,-0.706000000000001,-0.705000000000001,
-0.704000000000001,-0.703000000000001,-0.702000000000001,-0.701000000000001,
-0.700000000000001,-0.699000000000001,-0.698000000000001,-0.697000000000001,
-0.696000000000001,-0.695000000000001,-0.694000000000001,-0.693000000000001,
-0.692000000000001,-0.691000000000001,-0.690000000000001,-0.689000000000001,
-0.688000000000001,-0.687,-0.686,-0.685,-0.684,-0.683,-0.682,-0.681,-0.68,
-0.679,-0.678,-0.677,-0.676,-0.675,-0.674,-0.673,-0.672,-0.671,-0.67,-0.669,
-0.668,-0.667,-0.666,-0.665,-0.664,-0.663,-0.662,-0.661,-0.66,-0.659,-0.658,
-0.657,-0.656,-0.655,-0.654,-0.653,-0.652,-0.651,-0.65,-0.649,-0.648,-0.647,
-0.646,-0.645,-0.644,-0.643,-0.642,-0.641,-0.64,-0.639,-0.638,-0.637,-0.636,
-0.635,-0.634,-0.633,-0.632,-0.631,-0.63,-0.629,-0.628,-0.627,-0.626,-0.625,
-0.624,-0.623,-0.622,-0.621,-0.62,-0.619,-0.618,-0.617,-0.616,-0.615,-0.614,
-0.613,-0.612,-0.611,-0.61,-0.609,-0.608,-0.607,-0.606,-0.605,-0.604,-0.603,
-0.602,-0.601,-0.6,-0.599,-0.598,-0.597,-0.596,-0.595,-0.594,-0.593,-0.592,
-0.591,-0.59,-0.589,-0.588,-0.587,-0.586,-0.585,-0.584,-0.583,-0.582,-0.581,
-0.58,-0.579,-0.578,-0.577,-0.576,-0.575,-0.574,-0.573,-0.572,-0.571,-0.57,
-0.569,-0.568,-0.567,-0.566,-0.565,-0.564,-0.563,-0.562,-0.561,-0.56,-0.559,
-0.558,-0.557,-0.556,-0.555,-0.554,-0.553,-0.552,-0.551,-0.55,-0.549,-0.548,
-0.547,-0.546,-0.545,-0.544,-0.543,-0.542,-0.541,-0.54,-0.539,-0.538,-0.537,
-0.536,-0.535,-0.534,-0.533,-0.532,-0.531,-0.53,-0.529,-0.528,-0.527,-0.526,
-0.525,-0.524,-0.523,-0.522,-0.521,-0.52,-0.519,-0.518,-0.517,-0.516,-0.515,
-0.514,-0.513,-0.512,-0.511,-0.51,-0.509,-0.508,-0.507,-0.506,-0.505,-0.504,
-0.503,-0.502,-0.501,-0.5,-0.499,-0.498,-0.497,-0.496,-0.495,-0.494,-0.493,
-0.492,-0.491,-0.49,-0.489,-0.488,-0.487,-0.486,-0.485,-0.484,-0.483,-0.482,
-0.481,-0.48,-0.479,-0.478,-0.477,-0.476,-0.475,-0.474,-0.473,-0.472,-0.471,
-0.47,-0.469,-0.468,-0.467,-0.466,-0.465,-0.464,-0.463,-0.462,-0.461,-0.46,
-0.459,-0.458,-0.457,-0.456,-0.455,-0.454,-0.453,-0.452,-0.451,-0.45,-0.449,
-0.448,-0.447,-0.446,-0.445,-0.444,-0.443,-0.442,-0.441,-0.44,-0.439,-0.438,
-0.437,-0.436,-0.435,-0.434,-0.433,-0.432,-0.431,-0.43,-0.429,-0.428,-0.427,
-0.426,-0.425,-0.424,-0.423,-0.422,-0.421,-0.42,-0.419,-0.418,-0.417,-0.416,
-0.415,-0.414,-0.413,-0.412,-0.411,-0.41,-0.409,-0.408,-0.407,-0.406,-0.405,
-0.404,-0.403,-0.402,-0.401,-0.4,-0.399,-0.398,-0.397,-0.396,-0.395,-0.394,
-0.393,-0.392,-0.391,-0.39,-0.389,-0.388,-0.387,-0.386,-0.385,-0.384,-0.383,
-0.382,-0.381,-0.38,-0.379,-0.378,-0.377,-0.376,-0.375,-0.374,-0.373,-0.372,
-0.371,-0.37,-0.369,-0.368,-0.367,-0.366,-0.365,-0.364,-0.363,-0.362,-0.361,
-0.36,-0.359,-0.358,-0.357,-0.356,-0.355,-0.354,-0.353,-0.352,-0.351,-0.35,
-0.349,-0.348,-0.347,-0.346,-0.345,-0.344,-0.343,-0.342,-0.341,-0.34,-0.339,
-0.338,-0.337,-0.336,-0.335,-0.334,-0.333,-0.332,-0.331,-0.33,-0.329,-0.328,
-0.327,-0.326,-0.325,-0.324,-0.323,-0.322,-0.321,-0.32,-0.319,-0.318,-0.317,
-0.316,-0.315,-0.314,-0.313,-0.312,-0.311,-0.31,-0.309,-0.308,-0.307,-0.306,
-0.305,-0.304,-0.303,-0.302,-0.301,-0.3,-0.299,-0.298,-0.297,-0.296,-0.295,
-0.294,-0.293,-0.292,-0.291,-0.29,-0.289,-0.288,-0.287,-0.286,-0.285,-0.284,
-0.283,-0.282,-0.281,-0.28,-0.279,-0.278,-0.277,-0.276,-0.275,-0.274,-0.273,
-0.272,-0.271,-0.27,-0.269,-0.268,-0.267,-0.266,-0.265,-0.264,-0.263,-0.262,
-0.261,-0.26,-0.259,-0.258,-0.257,-0.256,-0.255,-0.254,-0.253,-0.252,-0.251,
-0.25,-0.249,-0.248,-0.247,-0.246,-0.245,-0.244,-0.243,-0.242,-0.241,-0.24,
-0.239,-0.238,-0.237,-0.236,-0.235,-0.234,-0.233,-0.232,-0.231,-0.23,-0.229,
-0.228,-0.227,-0.226,-0.225,-0.224,-0.223,-0.222,-0.221,-0.22,-0.219,-0.218,
-0.217,-0.216,-0.215,-0.214,-0.213,-0.212,-0.211,-0.21,-0.209,-0.208,-0.207,
-0.206,-0.205,-0.204,-0.203,-0.202,-0.201,-0.2,-0.199,-0.198,-0.197,-0.196,
-0.195,-0.194,-0.193,-0.192,-0.191,-0.19,-0.189,-0.188,-0.187,-0.186,-0.185,
-0.184,-0.183,-0.182,-0.181,-0.18,-0.179,-0.178,-0.177,-0.176,-0.175,-0.174,
-0.173,-0.172,-0.171,-0.17,-0.169,-0.168,-0.167,-0.166,-0.165,-0.164,-0.163,
-0.162,-0.161,-0.16,-0.159,-0.158,-0.157,-0.156,-0.155,-0.154,-0.153,-0.152,
-0.151,-0.15,-0.149,-0.148,-0.147,-0.146,-0.145,-0.144,-0.143,-0.142,-0.141,
-0.14,-0.139,-0.138,-0.137,-0.136,-0.135,-0.134,-0.133,-0.132,-0.131,-0.13,
-0.129,-0.128,-0.127,-0.126,-0.125,-0.124,-0.123,-0.122,-0.121,-0.12,-0.119,
-0.118,-0.117,-0.116,-0.115,-0.114,-0.113,-0.112,-0.111,-0.11,-0.109,-0.108,
-0.107,-0.106,-0.105,-0.104,-0.103,-0.102,-0.101,-0.1,-0.0990000000000001,
-0.0980000000000001,-0.0970000000000001,-0.0960000000000001,-0.0950000000000001,
-0.0940000000000001,-0.0930000000000001,-0.0920000000000001,-0.0910000000000001,
-0.0900000000000001,-0.0890000000000001,-0.0880000000000001,-0.0870000000000001,
-0.0860000000000001,-0.0850000000000001,-0.0840000000000001,-0.0830000000000001,
-0.0820000000000001,-0.0810000000000001,-0.0800000000000001,-0.0790000000000001,
-0.0780000000000001,-0.0770000000000001,-0.0760000000000001,-0.0750000000000001,
-0.0740000000000001,-0.0730000000000001,-0.0720000000000001,-0.071,-0.07,
-0.069,-0.068,-0.067,-0.066,-0.065,-0.064,-0.063,-0.062,-0.061,-0.06,-0.059,
-0.058,-0.057,-0.056,-0.055,-0.054,-0.053,-0.052,-0.051,-0.05,-0.049,-0.048,
-0.047,-0.046,-0.045,-0.044,-0.043,-0.042,-0.041,-0.04,-0.039,-0.038,-0.037,
-0.036,-0.035,-0.034,-0.033,-0.032,-0.031,-0.03,-0.029,-0.028,-0.027,-0.026,
-0.025,-0.024,-0.023,-0.022,-0.021,-0.02,-0.019,-0.018,-0.017,-0.016,-0.015,
-0.014,-0.013,-0.012,-0.011,-0.01,-0.009,-0.008,-0.007,-0.006,-0.005,-0.004,
-0.003,-0.002,-0.001,0.),(0.,2.),.UNSPECIFIED.)
GEOMETRIC_REPRESENTATION_ITEM()
RATIONAL_B_SPLINE_SURFACE(((1.,1.),(1.,1.),(1.,1.),(1.,1.),(1.,1.),(1.,
1.),(1.,1.),(1.,1.),(1.,1.),(1.,1.),(1.,1.),(1.,1.),(1.,1.),(1.,1.),(1.,
1.),(1.,1.),(1.,1.),(1.,1.),(1.,1.),(1.,1.),(1.,1.),(1.,1.),(1.,1.),(1.,
1.),(1.,1.),(1.,1.),(1.,1.),(1.,1.),(1.,1.),(1.,1.),(1.,1.),(1.,1.),(1.,
1.),(1.,1.),(1.,1.),(1.,1.),(1.,1.),(1.,1.),(1.,1.),(1.,1.),(1.,1.),(1.,
1.),(1.,1.),(1.,1.),(1.,1.),(1.,1.),(1.,1.),(1.,1.),(1.,1.),(1.,1.),(1.,
1.),(1.,1.),(1.,1.),(1.,1.),(1.,1.),(1.,1.),(1.,1.),(1.,1.),(1.,1.),(1.,
1.),(1.,1.),(1.,1.),(1.,1.),(1.,1.),(1.,1.),(1.,1.),(1.,1.),(1.,1.),(1.,
1.),(1.,1.),(1.,1.),(1.,1.),(1.,1.),(1.,1.),(1.,1.),(1.,1.),(1.,1.),(1.,
1.),(1.,1.),(1.,1.),(1.,1.),(1.,1.),(1.,1.),(1.,1.),(1.,1.),(1.,1.),(1.,
1.),(1.,1.),(1.,1.),(1.,1.),(1.,1.),(1.,1.),(1.,1.),(1.,1.),(1.,1.),(1.,
1.),(1.,1.),(1.,1.),(1.,1.),(1.,1.),(1.,1.),(1.,1.),(1.,1.),(1.,1.),(1.,
1.),(1.,1.),(1.,1.),(1.,1.),(1.,1.),(1.,1.),(1.,1.),(1.,1.),(1.,1.),(1.,
1.),(1.,1.),(1.,1.),(1.,1.),(1.,1.),(1.,1.),(1.,1.),(1.,1.),(1.,1.),(1.,
1.),(1.,1.),(1.,1.),(1.,1.),(1.,1.),(1.,1.),(1.,1.),(1.,1.),(1.,1.),(1.,
1.),(1.,1.),(1.,1.),(1.,1.),(1.,1.),(1.,1.),(1.,1.),(1.,1.),(1.,1.),(1.,
1.),(1.,1.),(1.,1.),(1.,1.),(1.,1.),(1.,1.),(1.,1.),(1.,1.),(1.,1.),(1.,
1.),(1.,1.),(1.,1.),(1.,1.),(1.,1.),(1.,1.),(1.,1.),(1.,1.),(1.,1.),(1.,
1.),(1.,1.),(1.,1.),(1.,1.),(1.,1.),(1.,1.),(1.,1.),(1.,1.),(1.,1.),(1.,
1.),(1.,1.),(1.,1.),(1.,1.),(1.,1.),(1.,1.),(1.,1.),(1.,1.),(1.,1.),(1.,
1.),(1.,1.),(1.,1.),(1.,1.),(1.,1.),(1.,1.),(1.,1.),(1.,1.),(1.,1.),(1.,
1.),(1.,1.),(1.,1.),(1.,1.),(1.,1.),(1.,1.),(1.,1.),(1.,1.),(1.,1.),(1.,
1.),(1.,1.),(1.,1.),(1.,1.),(1.,1.),(1.,1.),(1.,1.),(1.,1.),(1.,1.),(1.,
1.),(1.,1.),(1.,1.),(1.,1.),(1.,1.),(1.,1.),(1.,1.),(1.,1.),(1.,1.),(1.,
1.),(1.,1.),(1.,1.),(1.,1.),(1.,1.),(1.,1.),(1.,1.),(1.,1.),(1.,1.),(1.,
1.),(1.,1.),(1.,1.),(1.,1.),(1.,1.),(1.,1.),(1.,1.),(1.,1.),(1.,1.),(1.,
1.),(1.,1.),(1.,1.),(1.,1.),(1.,1.),(1.,1.),(1.,1.),(1.,1.),(1.,1.),(1.,
1.),(1.,1.),(1.,1.),(1.,1.),(1.,1.),(1.,1.),(1.,1.),(1.,1.),(1.,1.),(1.,
1.),(1.,1.),(1.,1.),(1.,1.),(1.,1.),(1.,1.),(1.,1.),(1.,1.),(1.,1.),(1.,
1.),(1.,1.),(1.,1.),(1.,1.),(1.,1.),(1.,1.),(1.,1.),(1.,1.),(1.,1.),(1.,
1.),(1.,1.),(1.,1.),(1.,1.),(1.,1.),(1.,1.),(1.,1.),(1.,1.),(1.,1.),(1.,
1.),(1.,1.),(1.,1.),(1.,1.),(1.,1.),(1.,1.),(1.,1.),(1.,1.),(1.,1.),(1.,
1.),(1.,1.),(1.,1.),(1.,1.),(1.,1.),(1.,1.),(1.,1.),(1.,1.),(1.,1.),(1.,
1.),(1.,1.),(1.,1.),(1.,1.),(1.,1.),(1.,1.),(1.,1.),(1.,1.),(1.,1.),(1.,
1.),(1.,1.),(1.,1.),(1.,1.),(1.,1.),(1.,1.),(1.,1.),(1.,1.),(1.,1.),(1.,
1.),(1.,1.),(1.,1.),(1.,1.),(1.,1.),(1.,1.),(1.,1.),(1.,1.),(1.,1.),(1.,
1.),(1.,1.),(1.,1.),(1.,1.),(1.,1.),(1.,1.),(1.,1.),(1.,1.),(1.,1.),(1.,
1.),(1.,1.),(1.,1.),(1.,1.),(1.,1.),(1.,1.),(1.,1.),(1.,1.),(1.,1.),(1.,
1.),(1.,1.),(1.,1.),(1.,1.),(1.,1.),(1.,1.),(1.,1.),(1.,1.),(1.,1.),(1.,
1.),(1.,1.),(1.,1.),(1.,1.),(1.,1.),(1.,1.),(1.,1.),(1.,1.),(1.,1.),(1.,
1.),(1.,1.),(1.,1.),(1.,1.),(1.,1.),(1.,1.),(1.,1.),(1.,1.),(1.,1.),(1.,
1.),(1.,1.),(1.,1.),(1.,1.),(1.,1.),(1.,1.),(1.,1.),(1.,1.),(1.,1.),(1.,
1.),(1.,1.),(1.,1.),(1.,1.),(1.,1.),(1.,1.),(1.,1.),(1.,1.),(1.,1.),(1.,
1.),(1.,1.),(1.,1.),(1.,1.),(1.,1.),(1.,1.),(1.,1.),(1.,1.),(1.,1.),(1.,
1.),(1.,1.),(1.,1.),(1.,1.),(1.,1.),(1.,1.),(1.,1.),(1.,1.),(1.,1.),(1.,
1.),(1.,1.),(1.,1.),(1.,1.),(1.,1.),(1.,1.),(1.,1.),(1.,1.),(1.,1.),(1.,
1.),(1.,1.),(1.,1.),(1.,1.),(1.,1.),(1.,1.),(1.,1.),(1.,1.),(1.,1.),(1.,
1.),(1.,1.),(1.,1.),(1.,1.),(1.,1.),(1.,1.),(1.,1.),(1.,1.),(1.,1.),(1.,
1.),(1.,1.),(1.,1.),(1.,1.),(1.,1.),(1.,1.),(1.,1.),(1.,1.),(1.,1.),(1.,
1.),(1.,1.),(1.,1.),(1.,1.),(1.,1.),(1.,1.),(1.,1.),(1.,1.),(1.,1.),(1.,
1.),(1.,1.),(1.,1.),(1.,1.),(1.,1.),(1.,1.),(1.,1.),(1.,1.),(1.,1.),(1.,
1.),(1.,1.),(1.,1.),(1.,1.),(1.,1.),(1.,1.),(1.,1.),(1.,1.),(1.,1.),(1.,
1.),(1.,1.),(1.,1.),(1.,1.),(1.,1.),(1.,1.),(1.,1.),(1.,1.),(1.,1.),(1.,
1.),(1.,1.),(1.,1.),(1.,1.),(1.,1.),(1.,1.),(1.,1.),(1.,1.),(1.,1.),(1.,
1.),(1.,1.),(1.,1.),(1.,1.),(1.,1.),(1.,1.),(1.,1.),(1.,1.),(1.,1.),(1.,
1.),(1.,1.),(1.,1.),(1.,1.),(1.,1.),(1.,1.),(1.,1.),(1.,1.),(1.,1.),(1.,
1.),(1.,1.),(1.,1.),(1.,1.),(1.,1.),(1.,1.),(1.,1.),(1.,1.),(1.,1.),(1.,
1.),(1.,1.),(1.,1.),(1.,1.),(1.,1.),(1.,1.),(1.,1.),(1.,1.),(1.,1.),(1.,
1.),(1.,1.),(1.,1.),(1.,1.),(1.,1.),(1.,1.),(1.,1.),(1.,1.),(1.,1.),(1.,
1.),(1.,1.),(1.,1.),(1.,1.),(1.,1.),(1.,1.),(1.,1.),(1.,1.),(1.,1.),(1.,
1.),(1.,1.),(1.,1.),(1.,1.),(1.,1.),(1.,1.),(1.,1.),(1.,1.),(1.,1.),(1.,
1.),(1.,1.),(1.,1.),(1.,1.),(1.,1.),(1.,1.),(1.,1.),(1.,1.),(1.,1.),(1.,
1.),(1.,1.),(1.,1.),(1.,1.),(1.,1.),(1.,1.),(1.,1.),(1.,1.),(1.,1.),(1.,
1.),(1.,1.),(1.,1.),(1.,1.),(1.,1.),(1.,1.),(1.,1.),(1.,1.),(1.,1.),(1.,
1.),(1.,1.),(1.,1.),(1.,1.),(1.,1.),(1.,1.),(1.,1.),(1.,1.),(1.,1.),(1.,
1.),(1.,1.),(1.,1.),(1.,1.),(1.,1.),(1.,1.),(1.,1.),(1.,1.),(1.,1.),(1.,
1.),(1.,1.),(1.,1.),(1.,1.),(1.,1.),(1.,1.),(1.,1.),(1.,1.),(1.,1.),(1.,
1.),(1.,1.),(1.,1.),(1.,1.),(1.,1.),(1.,1.),(1.,1.),(1.,1.),(1.,1.),(1.,
1.),(1.,1.),(1.,1.),(1.,1.),(1.,1.),(1.,1.),(1.,1.),(1.,1.),(1.,1.),(1.,
1.),(1.,1.),(1.,1.),(1.,1.),(1.,1.),(1.,1.),(1.,1.),(1.,1.),(1.,1.),(1.,
1.),(1.,1.),(1.,1.),(1.,1.),(1.,1.),(1.,1.),(1.,1.),(1.,1.),(1.,1.),(1.,
1.),(1.,1.),(1.,1.),(1.,1.),(1.,1.),(1.,1.),(1.,1.),(1.,1.),(1.,1.),(1.,
1.),(1.,1.),(1.,1.),(1.,1.),(1.,1.),(1.,1.),(1.,1.),(1.,1.),(1.,1.),(1.,
1.),(1.,1.),(1.,1.),(1.,1.),(1.,1.),(1.,1.),(1.,1.),(1.,1.),(1.,1.),(1.,
1.),(1.,1.),(1.,1.),(1.,1.),(1.,1.),(1.,1.),(1.,1.),(1.,1.),(1.,1.),(1.,
1.),(1.,1.),(1.,1.),(1.,1.),(1.,1.),(1.,1.),(1.,1.),(1.,1.),(1.,1.),(1.,
1.),(1.,1.),(1.,1.),(1.,1.),(1.,1.),(1.,1.),(1.,1.),(1.,1.),(1.,1.),(1.,
1.),(1.,1.),(1.,1.),(1.,1.),(1.,1.),(1.,1.),(1.,1.),(1.,1.),(1.,1.),(1.,
1.),(1.,1.),(1.,1.),(1.,1.),(1.,1.),(1.,1.),(1.,1.),(1.,1.),(1.,1.),(1.,
1.),(1.,1.),(1.,1.),(1.,1.),(1.,1.),(1.,1.),(1.,1.),(1.,1.),(1.,1.),(1.,
1.),(1.,1.),(1.,1.),(1.,1.),(1.,1.),(1.,1.),(1.,1.),(1.,1.),(1.,1.),(1.,
1.),(1.,1.),(1.,1.),(1.,1.),(1.,1.),(1.,1.),(1.,1.),(1.,1.),(1.,1.),(1.,
1.),(1.,1.),(1.,1.),(1.,1.),(1.,1.),(1.,1.),(1.,1.),(1.,1.),(1.,1.),(1.,
1.),(1.,1.),(1.,1.),(1.,1.),(1.,1.),(1.,1.),(1.,1.),(1.,1.),(1.,1.),(1.,
1.),(1.,1.),(1.,1.),(1.,1.),(1.,1.),(1.,1.),(1.,1.),(1.,1.),(1.,1.),(1.,
1.),(1.,1.),(1.,1.),(1.,1.),(1.,1.),(1.,1.),(1.,1.),(1.,1.),(1.,1.),(1.,
1.),(1.,1.),(1.,1.),(1.,1.),(1.,1.),(1.,1.),(1.,1.),(1.,1.),(1.,1.),(1.,
1.),(1.,1.),(1.,1.),(1.,1.),(1.,1.),(1.,1.),(1.,1.),(1.,1.),(1.,1.),(1.,
1.),(1.,1.),(1.,1.),(1.,1.),(1.,1.),(1.,1.),(1.,1.),(1.,1.),(1.,1.),(1.,
1.),(1.,1.),(1.,1.),(1.,1.),(1.,1.),(1.,1.),(1.,1.),(1.,1.),(1.,1.),(1.,
1.),(1.,1.),(1.,1.),(1.,1.),(1.,1.),(1.,1.),(1.,1.),(1.,1.),(1.,1.),(1.,
1.),(1.,1.),(1.,1.),(1.,1.),(1.,1.),(1.,1.),(1.,1.),(1.,1.),(1.,1.),(1.,
1.),(1.,1.),(1.,1.),(1.,1.),(1.,1.),(1.,1.),(1.,1.),(1.,1.),(1.,1.),(1.,
1.),(1.,1.),(1.,1.),(1.,1.),(1.,1.),(1.,1.),(1.,1.),(1.,1.),(1.,1.),(1.,
1.),(1.,1.),(1.,1.),(1.,1.),(1.,1.),(1.,1.),(1.,1.),(1.,1.),(1.,1.),(1.,
1.),(1.,1.),(1.,1.),(1.,1.),(1.,1.),(1.,1.),(1.,1.),(1.,1.),(1.,1.),(1.,
1.),(1.,1.),(1.,1.),(1.,1.),(1.,1.),(1.,1.),(1.,1.),(1.,1.),(1.,1.),(1.,
1.),(1.,1.),(1.,1.),(1.,1.),(1.,1.),(1.,1.),(1.,1.),(1.,1.),(1.,1.),(1.,
1.),(1.,1.),(1.,1.),(1.,1.),(1.,1.),(1.,1.),(1.,1.),(1.,1.),(1.,1.),(1.,
1.),(1.,1.),(1.,1.),(1.,1.),(1.,1.),(1.,1.),(1.,1.),(1.,1.),(1.,1.),(1.,
1.),(1.,1.),(1.,1.),(1.,1.),(1.,1.),(1.,1.),(1.,1.),(1.,1.),(1.,1.),(1.,
1.),(1.,1.),(1.,1.),(1.,1.),(1.,1.),(1.,1.),(1.,1.),(1.,1.),(1.,1.),(1.,
1.),(1.,1.),(1.,1.),(1.,1.),(1.,1.),(1.,1.),(1.,1.),(1.,1.),(1.,1.),(1.,
1.),(1.,1.),(1.,1.),(1.,1.),(1.,1.),(1.,1.),(1.,1.),(1.,1.),(1.,1.),(1.,
1.),(1.,1.),(1.,1.),(1.,1.),(1.,1.),(1.,1.),(1.,1.),(1.,1.),(1.,1.),(1.,
1.),(1.,1.),(1.,1.),(1.,1.),(1.,1.),(1.,1.),(1.,1.),(1.,1.),(1.,1.),(1.,
1.),(1.,1.),(1.,1.),(1.,1.),(1.,1.),(1.,1.),(1.,1.),(1.,1.),(1.,1.),(1.,
1.),(1.,1.),(1.,1.),(1.,1.),(1.,1.),(1.,1.),(1.,1.),(1.,1.),(1.,1.),(1.,
1.),(1.,1.),(1.,1.),(1.,1.),(1.,1.),(1.,1.),(1.,1.),(1.,1.),(1.,1.),(1.,
1.),(1.,1.),(1.,1.),(1.,1.),(1.,1.),(1.,1.),(1.,1.),(1.,1.),(1.,1.),(1.,
1.),(1.,1.),(1.,1.),(1.,1.),(1.,1.),(1.,1.),(1.,1.),(1.,1.),(1.,1.),(1.,
1.),(1.,1.),(1.,1.),(1.,1.),(1.,1.),(1.,1.),(1.,1.),(1.,1.),(1.,1.),(1.,
1.)))
REPRESENTATION_ITEM('')
SURFACE()
);
#264=(
BOUNDED_SURFACE()
B_SPLINE_SURFACE(5,1,((#86297,#86298),(#86299,#86300),(#86301,#86302),(#86303,
#86304),(#86305,#86306),(#86307,#86308),(#86309,#86310),(#86311,#86312),
(#86313,#86314),(#86315,#86316),(#86317,#86318),(#86319,#86320),(#86321,
#86322),(#86323,#86324),(#86325,#86326),(#86327,#86328),(#86329,#86330),
(#86331,#86332),(#86333,#86334),(#86335,#86336),(#86337,#86338),(#86339,
#86340),(#86341,#86342),(#86343,#86344),(#86345,#86346),(#86347,#86348),
(#86349,#86350),(#86351,#86352),(#86353,#86354),(#86355,#86356),(#86357,
#86358),(#86359,#86360),(#86361,#86362),(#86363,#86364),(#86365,#86366),
(#86367,#86368),(#86369,#86370),(#86371,#86372),(#86373,#86374),(#86375,
#86376),(#86377,#86378),(#86379,#86380),(#86381,#86382),(#86383,#86384),
(#86385,#86386),(#86387,#86388),(#86389,#86390),(#86391,#86392),(#86393,
#86394),(#86395,#86396),(#86397,#86398),(#86399,#86400),(#86401,#86402),
(#86403,#86404),(#86405,#86406),(#86407,#86408),(#86409,#86410),(#86411,
#86412),(#86413,#86414),(#86415,#86416),(#86417,#86418),(#86419,#86420),
(#86421,#86422),(#86423,#86424),(#86425,#86426),(#86427,#86428),(#86429,
#86430),(#86431,#86432),(#86433,#86434),(#86435,#86436),(#86437,#86438),
(#86439,#86440),(#86441,#86442),(#86443,#86444),(#86445,#86446),(#86447,
#86448),(#86449,#86450),(#86451,#86452),(#86453,#86454),(#86455,#86456),
(#86457,#86458),(#86459,#86460),(#86461,#86462),(#86463,#86464),(#86465,
#86466),(#86467,#86468),(#86469,#86470),(#86471,#86472),(#86473,#86474),
(#86475,#86476),(#86477,#86478),(#86479,#86480),(#86481,#86482),(#86483,
#86484),(#86485,#86486),(#86487,#86488),(#86489,#86490),(#86491,#86492),
(#86493,#86494),(#86495,#86496),(#86497,#86498),(#86499,#86500),(#86501,
#86502),(#86503,#86504),(#86505,#86506),(#86507,#86508),(#86509,#86510),
(#86511,#86512),(#86513,#86514),(#86515,#86516),(#86517,#86518),(#86519,
#86520),(#86521,#86522),(#86523,#86524),(#86525,#86526),(#86527,#86528),
(#86529,#86530),(#86531,#86532),(#86533,#86534),(#86535,#86536),(#86537,
#86538),(#86539,#86540),(#86541,#86542),(#86543,#86544),(#86545,#86546),
(#86547,#86548),(#86549,#86550),(#86551,#86552),(#86553,#86554),(#86555,
#86556),(#86557,#86558),(#86559,#86560),(#86561,#86562),(#86563,#86564),
(#86565,#86566),(#86567,#86568),(#86569,#86570),(#86571,#86572),(#86573,
#86574),(#86575,#86576),(#86577,#86578),(#86579,#86580),(#86581,#86582),
(#86583,#86584),(#86585,#86586),(#86587,#86588),(#86589,#86590),(#86591,
#86592),(#86593,#86594),(#86595,#86596),(#86597,#86598),(#86599,#86600),
(#86601,#86602),(#86603,#86604),(#86605,#86606),(#86607,#86608),(#86609,
#86610),(#86611,#86612),(#86613,#86614),(#86615,#86616),(#86617,#86618),
(#86619,#86620),(#86621,#86622),(#86623,#86624),(#86625,#86626),(#86627,
#86628),(#86629,#86630),(#86631,#86632),(#86633,#86634),(#86635,#86636),
(#86637,#86638),(#86639,#86640),(#86641,#86642),(#86643,#86644),(#86645,
#86646),(#86647,#86648),(#86649,#86650),(#86651,#86652),(#86653,#86654),
(#86655,#86656),(#86657,#86658),(#86659,#86660),(#86661,#86662),(#86663,
#86664),(#86665,#86666),(#86667,#86668),(#86669,#86670),(#86671,#86672),
(#86673,#86674),(#86675,#86676),(#86677,#86678),(#86679,#86680),(#86681,
#86682),(#86683,#86684),(#86685,#86686),(#86687,#86688),(#86689,#86690),
(#86691,#86692),(#86693,#86694),(#86695,#86696),(#86697,#86698),(#86699,
#86700),(#86701,#86702),(#86703,#86704),(#86705,#86706),(#86707,#86708),
(#86709,#86710),(#86711,#86712),(#86713,#86714),(#86715,#86716),(#86717,
#86718),(#86719,#86720),(#86721,#86722),(#86723,#86724),(#86725,#86726),
(#86727,#86728),(#86729,#86730),(#86731,#86732),(#86733,#86734),(#86735,
#86736),(#86737,#86738),(#86739,#86740),(#86741,#86742),(#86743,#86744),
(#86745,#86746),(#86747,#86748),(#86749,#86750),(#86751,#86752),(#86753,
#86754),(#86755,#86756),(#86757,#86758),(#86759,#86760),(#86761,#86762),
(#86763,#86764),(#86765,#86766),(#86767,#86768),(#86769,#86770),(#86771,
#86772),(#86773,#86774),(#86775,#86776),(#86777,#86778),(#86779,#86780),
(#86781,#86782),(#86783,#86784),(#86785,#86786),(#86787,#86788),(#86789,
#86790),(#86791,#86792),(#86793,#86794),(#86795,#86796),(#86797,#86798),
(#86799,#86800),(#86801,#86802),(#86803,#86804),(#86805,#86806),(#86807,
#86808),(#86809,#86810),(#86811,#86812),(#86813,#86814),(#86815,#86816),
(#86817,#86818),(#86819,#86820),(#86821,#86822),(#86823,#86824),(#86825,
#86826),(#86827,#86828),(#86829,#86830),(#86831,#86832),(#86833,#86834),
(#86835,#86836),(#86837,#86838),(#86839,#86840),(#86841,#86842),(#86843,
#86844),(#86845,#86846),(#86847,#86848),(#86849,#86850),(#86851,#86852),
(#86853,#86854),(#86855,#86856),(#86857,#86858),(#86859,#86860),(#86861,
#86862),(#86863,#86864),(#86865,#86866),(#86867,#86868),(#86869,#86870),
(#86871,#86872),(#86873,#86874),(#86875,#86876),(#86877,#86878),(#86879,
#86880),(#86881,#86882),(#86883,#86884),(#86885,#86886),(#86887,#86888),
(#86889,#86890),(#86891,#86892),(#86893,#86894),(#86895,#86896),(#86897,
#86898),(#86899,#86900),(#86901,#86902),(#86903,#86904),(#86905,#86906),
(#86907,#86908),(#86909,#86910),(#86911,#86912),(#86913,#86914),(#86915,
#86916),(#86917,#86918),(#86919,#86920),(#86921,#86922),(#86923,#86924),
(#86925,#86926),(#86927,#86928),(#86929,#86930),(#86931,#86932),(#86933,
#86934),(#86935,#86936),(#86937,#86938),(#86939,#86940),(#86941,#86942),
(#86943,#86944),(#86945,#86946),(#86947,#86948),(#86949,#86950),(#86951,
#86952),(#86953,#86954),(#86955,#86956),(#86957,#86958),(#86959,#86960),
(#86961,#86962),(#86963,#86964),(#86965,#86966),(#86967,#86968),(#86969,
#86970),(#86971,#86972),(#86973,#86974),(#86975,#86976),(#86977,#86978),
(#86979,#86980),(#86981,#86982),(#86983,#86984),(#86985,#86986),(#86987,
#86988),(#86989,#86990),(#86991,#86992),(#86993,#86994),(#86995,#86996),
(#86997,#86998),(#86999,#87000),(#87001,#87002),(#87003,#87004),(#87005,
#87006),(#87007,#87008),(#87009,#87010),(#87011,#87012),(#87013,#87014),
(#87015,#87016),(#87017,#87018),(#87019,#87020),(#87021,#87022),(#87023,
#87024),(#87025,#87026),(#87027,#87028),(#87029,#87030),(#87031,#87032),
(#87033,#87034),(#87035,#87036),(#87037,#87038),(#87039,#87040),(#87041,
#87042),(#87043,#87044),(#87045,#87046),(#87047,#87048),(#87049,#87050),
(#87051,#87052),(#87053,#87054),(#87055,#87056),(#87057,#87058),(#87059,
#87060),(#87061,#87062),(#87063,#87064),(#87065,#87066),(#87067,#87068),
(#87069,#87070),(#87071,#87072),(#87073,#87074),(#87075,#87076),(#87077,
#87078),(#87079,#87080),(#87081,#87082),(#87083,#87084),(#87085,#87086),
(#87087,#87088),(#87089,#87090),(#87091,#87092),(#87093,#87094),(#87095,
#87096),(#87097,#87098),(#87099,#87100),(#87101,#87102),(#87103,#87104),
(#87105,#87106),(#87107,#87108),(#87109,#87110),(#87111,#87112),(#87113,
#87114),(#87115,#87116),(#87117,#87118),(#87119,#87120),(#87121,#87122),
(#87123,#87124),(#87125,#87126),(#87127,#87128),(#87129,#87130),(#87131,
#87132),(#87133,#87134),(#87135,#87136),(#87137,#87138),(#87139,#87140),
(#87141,#87142),(#87143,#87144),(#87145,#87146),(#87147,#87148),(#87149,
#87150),(#87151,#87152),(#87153,#87154),(#87155,#87156),(#87157,#87158),
(#87159,#87160),(#87161,#87162),(#87163,#87164),(#87165,#87166),(#87167,
#87168),(#87169,#87170),(#87171,#87172),(#87173,#87174),(#87175,#87176),
(#87177,#87178),(#87179,#87180),(#87181,#87182),(#87183,#87184),(#87185,
#87186),(#87187,#87188),(#87189,#87190),(#87191,#87192),(#87193,#87194),
(#87195,#87196),(#87197,#87198),(#87199,#87200),(#87201,#87202),(#87203,
#87204),(#87205,#87206),(#87207,#87208),(#87209,#87210),(#87211,#87212),
(#87213,#87214),(#87215,#87216),(#87217,#87218),(#87219,#87220),(#87221,
#87222),(#87223,#87224),(#87225,#87226),(#87227,#87228),(#87229,#87230),
(#87231,#87232),(#87233,#87234),(#87235,#87236),(#87237,#87238),(#87239,
#87240),(#87241,#87242),(#87243,#87244),(#87245,#87246),(#87247,#87248),
(#87249,#87250),(#87251,#87252),(#87253,#87254),(#87255,#87256),(#87257,
#87258),(#87259,#87260),(#87261,#87262),(#87263,#87264),(#87265,#87266),
(#87267,#87268),(#87269,#87270),(#87271,#87272),(#87273,#87274),(#87275,
#87276),(#87277,#87278),(#87279,#87280),(#87281,#87282),(#87283,#87284),
(#87285,#87286),(#87287,#87288),(#87289,#87290),(#87291,#87292),(#87293,
#87294),(#87295,#87296),(#87297,#87298),(#87299,#87300),(#87301,#87302),
(#87303,#87304),(#87305,#87306),(#87307,#87308),(#87309,#87310),(#87311,
#87312),(#87313,#87314),(#87315,#87316),(#87317,#87318),(#87319,#87320),
(#87321,#87322),(#87323,#87324),(#87325,#87326),(#87327,#87328),(#87329,
#87330),(#87331,#87332),(#87333,#87334),(#87335,#87336),(#87337,#87338),
(#87339,#87340),(#87341,#87342),(#87343,#87344),(#87345,#87346),(#87347,
#87348),(#87349,#87350),(#87351,#87352),(#87353,#87354),(#87355,#87356),
(#87357,#87358),(#87359,#87360),(#87361,#87362),(#87363,#87364),(#87365,
#87366),(#87367,#87368),(#87369,#87370),(#87371,#87372),(#87373,#87374),
(#87375,#87376),(#87377,#87378),(#87379,#87380),(#87381,#87382),(#87383,
#87384),(#87385,#87386),(#87387,#87388),(#87389,#87390),(#87391,#87392),
(#87393,#87394),(#87395,#87396),(#87397,#87398),(#87399,#87400),(#87401,
#87402),(#87403,#87404),(#87405,#87406),(#87407,#87408),(#87409,#87410),
(#87411,#87412),(#87413,#87414),(#87415,#87416),(#87417,#87418),(#87419,
#87420),(#87421,#87422),(#87423,#87424),(#87425,#87426),(#87427,#87428),
(#87429,#87430),(#87431,#87432),(#87433,#87434),(#87435,#87436),(#87437,
#87438),(#87439,#87440),(#87441,#87442),(#87443,#87444),(#87445,#87446),
(#87447,#87448),(#87449,#87450),(#87451,#87452),(#87453,#87454),(#87455,
#87456),(#87457,#87458),(#87459,#87460),(#87461,#87462),(#87463,#87464),
(#87465,#87466),(#87467,#87468),(#87469,#87470),(#87471,#87472),(#87473,
#87474),(#87475,#87476),(#87477,#87478),(#87479,#87480),(#87481,#87482),
(#87483,#87484),(#87485,#87486),(#87487,#87488),(#87489,#87490),(#87491,
#87492),(#87493,#87494),(#87495,#87496),(#87497,#87498),(#87499,#87500),
(#87501,#87502),(#87503,#87504),(#87505,#87506),(#87507,#87508),(#87509,
#87510),(#87511,#87512),(#87513,#87514),(#87515,#87516),(#87517,#87518),
(#87519,#87520),(#87521,#87522),(#87523,#87524),(#87525,#87526),(#87527,
#87528),(#87529,#87530),(#87531,#87532),(#87533,#87534),(#87535,#87536),
(#87537,#87538),(#87539,#87540),(#87541,#87542),(#87543,#87544),(#87545,
#87546),(#87547,#87548),(#87549,#87550),(#87551,#87552),(#87553,#87554),
(#87555,#87556),(#87557,#87558),(#87559,#87560),(#87561,#87562),(#87563,
#87564),(#87565,#87566),(#87567,#87568),(#87569,#87570),(#87571,#87572),
(#87573,#87574),(#87575,#87576),(#87577,#87578),(#87579,#87580),(#87581,
#87582),(#87583,#87584),(#87585,#87586),(#87587,#87588),(#87589,#87590),
(#87591,#87592),(#87593,#87594),(#87595,#87596),(#87597,#87598),(#87599,
#87600),(#87601,#87602),(#87603,#87604),(#87605,#87606),(#87607,#87608),
(#87609,#87610),(#87611,#87612),(#87613,#87614),(#87615,#87616),(#87617,
#87618),(#87619,#87620),(#87621,#87622),(#87623,#87624),(#87625,#87626),
(#87627,#87628),(#87629,#87630),(#87631,#87632),(#87633,#87634),(#87635,
#87636),(#87637,#87638),(#87639,#87640),(#87641,#87642),(#87643,#87644),
(#87645,#87646),(#87647,#87648),(#87649,#87650),(#87651,#87652),(#87653,
#87654),(#87655,#87656),(#87657,#87658),(#87659,#87660),(#87661,#87662),
(#87663,#87664),(#87665,#87666),(#87667,#87668),(#87669,#87670),(#87671,
#87672),(#87673,#87674),(#87675,#87676),(#87677,#87678),(#87679,#87680),
(#87681,#87682),(#87683,#87684),(#87685,#87686),(#87687,#87688),(#87689,
#87690),(#87691,#87692),(#87693,#87694),(#87695,#87696),(#87697,#87698),
(#87699,#87700),(#87701,#87702),(#87703,#87704),(#87705,#87706),(#87707,
#87708),(#87709,#87710),(#87711,#87712),(#87713,#87714),(#87715,#87716),
(#87717,#87718),(#87719,#87720),(#87721,#87722),(#87723,#87724),(#87725,
#87726),(#87727,#87728),(#87729,#87730),(#87731,#87732),(#87733,#87734),
(#87735,#87736),(#87737,#87738),(#87739,#87740),(#87741,#87742),(#87743,
#87744),(#87745,#87746),(#87747,#87748),(#87749,#87750),(#87751,#87752),
(#87753,#87754),(#87755,#87756),(#87757,#87758),(#87759,#87760),(#87761,
#87762),(#87763,#87764),(#87765,#87766),(#87767,#87768),(#87769,#87770),
(#87771,#87772),(#87773,#87774),(#87775,#87776),(#87777,#87778),(#87779,
#87780),(#87781,#87782),(#87783,#87784),(#87785,#87786),(#87787,#87788),
(#87789,#87790),(#87791,#87792),(#87793,#87794),(#87795,#87796),(#87797,
#87798),(#87799,#87800),(#87801,#87802),(#87803,#87804),(#87805,#87806),
(#87807,#87808),(#87809,#87810),(#87811,#87812),(#87813,#87814),(#87815,
#87816),(#87817,#87818),(#87819,#87820),(#87821,#87822),(#87823,#87824),
(#87825,#87826),(#87827,#87828),(#87829,#87830),(#87831,#87832),(#87833,
#87834),(#87835,#87836),(#87837,#87838),(#87839,#87840),(#87841,#87842),
(#87843,#87844),(#87845,#87846),(#87847,#87848),(#87849,#87850),(#87851,
#87852),(#87853,#87854),(#87855,#87856),(#87857,#87858),(#87859,#87860),
(#87861,#87862),(#87863,#87864),(#87865,#87866),(#87867,#87868),(#87869,
#87870),(#87871,#87872),(#87873,#87874),(#87875,#87876),(#87877,#87878),
(#87879,#87880),(#87881,#87882),(#87883,#87884),(#87885,#87886),(#87887,
#87888),(#87889,#87890),(#87891,#87892),(#87893,#87894),(#87895,#87896),
(#87897,#87898),(#87899,#87900),(#87901,#87902),(#87903,#87904),(#87905,
#87906),(#87907,#87908),(#87909,#87910),(#87911,#87912),(#87913,#87914),
(#87915,#87916),(#87917,#87918),(#87919,#87920),(#87921,#87922),(#87923,
#87924),(#87925,#87926),(#87927,#87928),(#87929,#87930),(#87931,#87932),
(#87933,#87934),(#87935,#87936),(#87937,#87938),(#87939,#87940),(#87941,
#87942),(#87943,#87944),(#87945,#87946),(#87947,#87948),(#87949,#87950),
(#87951,#87952),(#87953,#87954),(#87955,#87956),(#87957,#87958),(#87959,
#87960),(#87961,#87962),(#87963,#87964),(#87965,#87966),(#87967,#87968),
(#87969,#87970),(#87971,#87972),(#87973,#87974),(#87975,#87976),(#87977,
#87978),(#87979,#87980),(#87981,#87982),(#87983,#87984),(#87985,#87986),
(#87987,#87988),(#87989,#87990),(#87991,#87992),(#87993,#87994),(#87995,
#87996),(#87997,#87998),(#87999,#88000),(#88001,#88002),(#88003,#88004),
(#88005,#88006),(#88007,#88008),(#88009,#88010),(#88011,#88012),(#88013,
#88014),(#88015,#88016),(#88017,#88018),(#88019,#88020),(#88021,#88022),
(#88023,#88024),(#88025,#88026),(#88027,#88028),(#88029,#88030),(#88031,
#88032),(#88033,#88034),(#88035,#88036),(#88037,#88038),(#88039,#88040),
(#88041,#88042),(#88043,#88044),(#88045,#88046),(#88047,#88048),(#88049,
#88050),(#88051,#88052),(#88053,#88054),(#88055,#88056),(#88057,#88058),
(#88059,#88060),(#88061,#88062),(#88063,#88064),(#88065,#88066),(#88067,
#88068),(#88069,#88070),(#88071,#88072),(#88073,#88074),(#88075,#88076),
(#88077,#88078),(#88079,#88080),(#88081,#88082),(#88083,#88084),(#88085,
#88086),(#88087,#88088),(#88089,#88090),(#88091,#88092),(#88093,#88094),
(#88095,#88096),(#88097,#88098),(#88099,#88100),(#88101,#88102),(#88103,
#88104),(#88105,#88106),(#88107,#88108),(#88109,#88110),(#88111,#88112),
(#88113,#88114),(#88115,#88116),(#88117,#88118),(#88119,#88120),(#88121,
#88122),(#88123,#88124),(#88125,#88126),(#88127,#88128),(#88129,#88130),
(#88131,#88132),(#88133,#88134),(#88135,#88136),(#88137,#88138),(#88139,
#88140),(#88141,#88142),(#88143,#88144),(#88145,#88146),(#88147,#88148),
(#88149,#88150),(#88151,#88152),(#88153,#88154),(#88155,#88156),(#88157,
#88158),(#88159,#88160),(#88161,#88162),(#88163,#88164),(#88165,#88166),
(#88167,#88168),(#88169,#88170),(#88171,#88172),(#88173,#88174),(#88175,
#88176),(#88177,#88178),(#88179,#88180),(#88181,#88182),(#88183,#88184),
(#88185,#88186),(#88187,#88188),(#88189,#88190),(#88191,#88192),(#88193,
#88194),(#88195,#88196),(#88197,#88198),(#88199,#88200),(#88201,#88202),
(#88203,#88204),(#88205,#88206),(#88207,#88208),(#88209,#88210),(#88211,
#88212),(#88213,#88214),(#88215,#88216),(#88217,#88218),(#88219,#88220),
(#88221,#88222),(#88223,#88224),(#88225,#88226),(#88227,#88228),(#88229,
#88230),(#88231,#88232),(#88233,#88234),(#88235,#88236),(#88237,#88238),
(#88239,#88240),(#88241,#88242),(#88243,#88244),(#88245,#88246),(#88247,
#88248),(#88249,#88250),(#88251,#88252),(#88253,#88254),(#88255,#88256),
(#88257,#88258),(#88259,#88260),(#88261,#88262),(#88263,#88264),(#88265,
#88266),(#88267,#88268),(#88269,#88270),(#88271,#88272),(#88273,#88274),
(#88275,#88276),(#88277,#88278),(#88279,#88280),(#88281,#88282),(#88283,
#88284),(#88285,#88286),(#88287,#88288),(#88289,#88290),(#88291,#88292),
(#88293,#88294),(#88295,#88296),(#88297,#88298),(#88299,#88300),(#88301,
#88302),(#88303,#88304),(#88305,#88306)),.UNSPECIFIED.,.F.,.F.,.F.)
B_SPLINE_SURFACE_WITH_KNOTS((6,1,1,1,1,1,1,1,1,1,1,1,1,1,1,1,1,1,1,1,1,
1,1,1,1,1,1,1,1,1,1,1,1,1,1,1,1,1,1,1,1,1,1,1,1,1,1,1,1,1,1,1,1,1,1,1,1,
1,1,1,1,1,1,1,1,1,1,1,1,1,1,1,1,1,1,1,1,1,1,1,1,1,1,1,1,1,1,1,1,1,1,1,1,
1,1,1,1,1,1,1,1,1,1,1,1,1,1,1,1,1,1,1,1,1,1,1,1,1,1,1,1,1,1,1,1,1,1,1,1,
1,1,1,1,1,1,1,1,1,1,1,1,1,1,1,1,1,1,1,1,1,1,1,1,1,1,1,1,1,1,1,1,1,1,1,1,
1,1,1,1,1,1,1,1,1,1,1,1,1,1,1,1,1,1,1,1,1,1,1,1,1,1,1,1,1,1,1,1,1,1,1,1,
1,1,1,1,1,1,1,1,1,1,1,1,1,1,1,1,1,1,1,1,1,1,1,1,1,1,1,1,1,1,1,1,1,1,1,1,
1,1,1,1,1,1,1,1,1,1,1,1,1,1,1,1,1,1,1,1,1,1,1,1,1,1,1,1,1,1,1,1,1,1,1,1,
1,1,1,1,1,1,1,1,1,1,1,1,1,1,1,1,1,1,1,1,1,1,1,1,1,1,1,1,1,1,1,1,1,1,1,1,
1,1,1,1,1,1,1,1,1,1,1,1,1,1,1,1,1,1,1,1,1,1,1,1,1,1,1,1,1,1,1,1,1,1,1,1,
1,1,1,1,1,1,1,1,1,1,1,1,1,1,1,1,1,1,1,1,1,1,1,1,1,1,1,1,1,1,1,1,1,1,1,1,
1,1,1,1,1,1,1,1,1,1,1,1,1,1,1,1,1,1,1,1,1,1,1,1,1,1,1,1,1,1,1,1,1,1,1,1,
1,1,1,1,1,1,1,1,1,1,1,1,1,1,1,1,1,1,1,1,1,1,1,1,1,1,1,1,1,1,1,1,1,1,1,1,
1,1,1,1,1,1,1,1,1,1,1,1,1,1,1,1,1,1,1,1,1,1,1,1,1,1,1,1,1,1,1,1,1,1,1,1,
1,1,1,1,1,1,1,1,1,1,1,1,1,1,1,1,1,1,1,1,1,1,1,1,1,1,1,1,1,1,1,1,1,1,1,1,
1,1,1,1,1,1,1,1,1,1,1,1,1,1,1,1,1,1,1,1,1,1,1,1,1,1,1,1,1,1,1,1,1,1,1,1,
1,1,1,1,1,1,1,1,1,1,1,1,1,1,1,1,1,1,1,1,1,1,1,1,1,1,1,1,1,1,1,1,1,1,1,1,
1,1,1,1,1,1,1,1,1,1,1,1,1,1,1,1,1,1,1,1,1,1,1,1,1,1,1,1,1,1,1,1,1,1,1,1,
1,1,1,1,1,1,1,1,1,1,1,1,1,1,1,1,1,1,1,1,1,1,1,1,1,1,1,1,1,1,1,1,1,1,1,1,
1,1,1,1,1,1,1,1,1,1,1,1,1,1,1,1,1,1,1,1,1,1,1,1,1,1,1,1,1,1,1,1,1,1,1,1,
1,1,1,1,1,1,1,1,1,1,1,1,1,1,1,1,1,1,1,1,1,1,1,1,1,1,1,1,1,1,1,1,1,1,1,1,
1,1,1,1,1,1,1,1,1,1,1,1,1,1,1,1,1,1,1,1,1,1,1,1,1,1,1,1,1,1,1,1,1,1,1,1,
1,1,1,1,1,1,1,1,1,1,1,1,1,1,1,1,1,1,1,1,1,1,1,1,1,1,1,1,1,1,1,1,1,1,1,1,
1,1,1,1,1,1,1,1,1,1,1,1,1,1,1,1,1,1,1,1,1,1,1,1,1,1,1,1,1,1,1,1,1,1,1,1,
1,1,1,1,1,1,1,1,1,1,1,1,1,1,1,1,1,1,1,1,1,1,1,1,1,1,1,1,1,1,1,1,1,1,1,1,
1,1,1,1,1,1,1,1,1,1,1,1,1,1,1,1,1,1,1,1,1,1,1,1,1,1,1,1,1,1,1,1,1,1,1,1,
1,1,1,1,1,1,1,1,1,1,1,1,1,1,1,1,1,1,1,1,1,1,1,1,1,1,1,1,1,1,1,1,1,1,1,1,
1,1,1,1,1,1,1,1,1,1,1,1,1,1,1,1,1,1,1,1,1,1,1,1,1,1,1,1,1,1,1,1,1,1,1,1,
1,1,1,1,1,1,1,6),(2,2),(-1.,-0.999000000000001,-0.998000000000001,-0.997000000000001,
-0.996000000000001,-0.995000000000001,-0.994000000000001,-0.993000000000001,
-0.992000000000001,-0.991000000000001,-0.990000000000001,-0.989000000000001,
-0.988000000000001,-0.987000000000001,-0.986000000000001,-0.985000000000001,
-0.984000000000001,-0.983000000000001,-0.982000000000001,-0.981000000000001,
-0.980000000000001,-0.979000000000001,-0.978000000000001,-0.977000000000001,
-0.976000000000001,-0.975000000000001,-0.974000000000001,-0.973000000000001,
-0.972000000000001,-0.971000000000001,-0.970000000000001,-0.969000000000001,
-0.968000000000001,-0.967000000000001,-0.966000000000001,-0.965000000000001,
-0.964000000000001,-0.963000000000001,-0.962000000000001,-0.961000000000001,
-0.960000000000001,-0.959000000000001,-0.958000000000001,-0.957000000000001,
-0.956000000000001,-0.955000000000001,-0.954000000000001,-0.953000000000001,
-0.952000000000001,-0.951000000000001,-0.950000000000001,-0.949000000000001,
-0.948000000000001,-0.947000000000001,-0.946000000000001,-0.945000000000001,
-0.944000000000001,-0.943000000000001,-0.942000000000001,-0.941000000000001,
-0.940000000000001,-0.939000000000001,-0.938000000000001,-0.937000000000001,
-0.936000000000001,-0.935000000000001,-0.934000000000001,-0.933000000000001,
-0.932000000000001,-0.931000000000001,-0.930000000000001,-0.929000000000001,
-0.928000000000001,-0.927000000000001,-0.926000000000001,-0.925000000000001,
-0.924000000000001,-0.923000000000001,-0.922000000000001,-0.921000000000001,
-0.920000000000001,-0.919000000000001,-0.918000000000001,-0.917000000000001,
-0.916000000000001,-0.915000000000001,-0.914000000000001,-0.913000000000001,
-0.912000000000001,-0.911000000000001,-0.910000000000001,-0.909000000000001,
-0.908000000000001,-0.907000000000001,-0.906000000000001,-0.905000000000001,
-0.904000000000001,-0.903000000000001,-0.902000000000001,-0.901000000000001,
-0.900000000000001,-0.899000000000001,-0.898000000000001,-0.897000000000001,
-0.896000000000001,-0.895000000000001,-0.894000000000001,-0.893000000000001,
-0.892000000000001,-0.891000000000001,-0.890000000000001,-0.889000000000001,
-0.888000000000001,-0.887000000000001,-0.886000000000001,-0.885000000000001,
-0.884000000000001,-0.883000000000001,-0.882000000000001,-0.881000000000001,
-0.880000000000001,-0.879000000000001,-0.878000000000001,-0.877000000000001,
-0.876000000000001,-0.875000000000001,-0.874000000000001,-0.873000000000001,
-0.872000000000001,-0.871000000000001,-0.870000000000001,-0.869000000000001,
-0.868000000000001,-0.867000000000001,-0.866000000000001,-0.865000000000001,
-0.864000000000001,-0.863000000000001,-0.862000000000001,-0.861000000000001,
-0.860000000000001,-0.859000000000001,-0.858000000000001,-0.857000000000001,
-0.856000000000001,-0.855000000000001,-0.854000000000001,-0.853000000000001,
-0.852000000000001,-0.851000000000001,-0.850000000000001,-0.849000000000001,
-0.848000000000001,-0.847000000000001,-0.846000000000001,-0.845000000000001,
-0.844000000000001,-0.843000000000001,-0.842000000000001,-0.841000000000001,
-0.840000000000001,-0.839000000000001,-0.838000000000001,-0.837000000000001,
-0.836000000000001,-0.835000000000001,-0.834000000000001,-0.833000000000001,
-0.832000000000001,-0.831000000000001,-0.830000000000001,-0.829000000000001,
-0.828000000000001,-0.827000000000001,-0.826000000000001,-0.825000000000001,
-0.824000000000001,-0.823000000000001,-0.822000000000001,-0.821000000000001,
-0.820000000000001,-0.819000000000001,-0.818000000000001,-0.817000000000001,
-0.816000000000001,-0.815000000000001,-0.814000000000001,-0.813000000000001,
-0.812000000000001,-0.811000000000001,-0.810000000000001,-0.809000000000001,
-0.808000000000001,-0.807000000000001,-0.806000000000001,-0.805000000000001,
-0.804000000000001,-0.803000000000001,-0.802000000000001,-0.801000000000001,
-0.800000000000001,-0.799000000000001,-0.798000000000001,-0.797000000000001,
-0.796000000000001,-0.795000000000001,-0.794000000000001,-0.793000000000001,
-0.792000000000001,-0.791000000000001,-0.790000000000001,-0.789000000000001,
-0.788000000000001,-0.787000000000001,-0.786000000000001,-0.785000000000001,
-0.784000000000001,-0.783000000000001,-0.782000000000001,-0.781000000000001,
-0.780000000000001,-0.779000000000001,-0.778000000000001,-0.777000000000001,
-0.776000000000001,-0.775000000000001,-0.774000000000001,-0.773000000000001,
-0.772000000000001,-0.771000000000001,-0.770000000000001,-0.769000000000001,
-0.768000000000001,-0.767000000000001,-0.766000000000001,-0.765000000000001,
-0.764000000000001,-0.763000000000001,-0.762000000000001,-0.761000000000001,
-0.760000000000001,-0.759000000000001,-0.758000000000001,-0.757000000000001,
-0.756000000000001,-0.755000000000001,-0.754000000000001,-0.753000000000001,
-0.752000000000001,-0.751000000000001,-0.750000000000001,-0.749000000000001,
-0.748000000000001,-0.747000000000001,-0.746000000000001,-0.745000000000001,
-0.744000000000001,-0.743000000000001,-0.742000000000001,-0.741000000000001,
-0.740000000000001,-0.739000000000001,-0.738000000000001,-0.737000000000001,
-0.736000000000001,-0.735000000000001,-0.734000000000001,-0.733000000000001,
-0.732000000000001,-0.731000000000001,-0.730000000000001,-0.729000000000001,
-0.728000000000001,-0.727000000000001,-0.726000000000001,-0.725000000000001,
-0.724000000000001,-0.723000000000001,-0.722000000000001,-0.721000000000001,
-0.720000000000001,-0.719000000000001,-0.718000000000001,-0.717000000000001,
-0.716000000000001,-0.715000000000001,-0.714000000000001,-0.713000000000001,
-0.712000000000001,-0.711000000000001,-0.710000000000001,-0.709000000000001,
-0.708000000000001,-0.707000000000001,-0.706000000000001,-0.705000000000001,
-0.704000000000001,-0.703000000000001,-0.702000000000001,-0.701000000000001,
-0.700000000000001,-0.699000000000001,-0.698000000000001,-0.697000000000001,
-0.696000000000001,-0.695000000000001,-0.694000000000001,-0.693000000000001,
-0.692000000000001,-0.691000000000001,-0.690000000000001,-0.689000000000001,
-0.688000000000001,-0.687,-0.686,-0.685,-0.684,-0.683,-0.682,-0.681,-0.68,
-0.679,-0.678,-0.677,-0.676,-0.675,-0.674,-0.673,-0.672,-0.671,-0.67,-0.669,
-0.668,-0.667,-0.666,-0.665,-0.664,-0.663,-0.662,-0.661,-0.66,-0.659,-0.658,
-0.657,-0.656,-0.655,-0.654,-0.653,-0.652,-0.651,-0.65,-0.649,-0.648,-0.647,
-0.646,-0.645,-0.644,-0.643,-0.642,-0.641,-0.64,-0.639,-0.638,-0.637,-0.636,
-0.635,-0.634,-0.633,-0.632,-0.631,-0.63,-0.629,-0.628,-0.627,-0.626,-0.625,
-0.624,-0.623,-0.622,-0.621,-0.62,-0.619,-0.618,-0.617,-0.616,-0.615,-0.614,
-0.613,-0.612,-0.611,-0.61,-0.609,-0.608,-0.607,-0.606,-0.605,-0.604,-0.603,
-0.602,-0.601,-0.6,-0.599,-0.598,-0.597,-0.596,-0.595,-0.594,-0.593,-0.592,
-0.591,-0.59,-0.589,-0.588,-0.587,-0.586,-0.585,-0.584,-0.583,-0.582,-0.581,
-0.58,-0.579,-0.578,-0.577,-0.576,-0.575,-0.574,-0.573,-0.572,-0.571,-0.57,
-0.569,-0.568,-0.567,-0.566,-0.565,-0.564,-0.563,-0.562,-0.561,-0.56,-0.559,
-0.558,-0.557,-0.556,-0.555,-0.554,-0.553,-0.552,-0.551,-0.55,-0.549,-0.548,
-0.547,-0.546,-0.545,-0.544,-0.543,-0.542,-0.541,-0.54,-0.539,-0.538,-0.537,
-0.536,-0.535,-0.534,-0.533,-0.532,-0.531,-0.53,-0.529,-0.528,-0.527,-0.526,
-0.525,-0.524,-0.523,-0.522,-0.521,-0.52,-0.519,-0.518,-0.517,-0.516,-0.515,
-0.514,-0.513,-0.512,-0.511,-0.51,-0.509,-0.508,-0.507,-0.506,-0.505,-0.504,
-0.503,-0.502,-0.501,-0.5,-0.499,-0.498,-0.497,-0.496,-0.495,-0.494,-0.493,
-0.492,-0.491,-0.49,-0.489,-0.488,-0.487,-0.486,-0.485,-0.484,-0.483,-0.482,
-0.481,-0.48,-0.479,-0.478,-0.477,-0.476,-0.475,-0.474,-0.473,-0.472,-0.471,
-0.47,-0.469,-0.468,-0.467,-0.466,-0.465,-0.464,-0.463,-0.462,-0.461,-0.46,
-0.459,-0.458,-0.457,-0.456,-0.455,-0.454,-0.453,-0.452,-0.451,-0.45,-0.449,
-0.448,-0.447,-0.446,-0.445,-0.444,-0.443,-0.442,-0.441,-0.44,-0.439,-0.438,
-0.437,-0.436,-0.435,-0.434,-0.433,-0.432,-0.431,-0.43,-0.429,-0.428,-0.427,
-0.426,-0.425,-0.424,-0.423,-0.422,-0.421,-0.42,-0.419,-0.418,-0.417,-0.416,
-0.415,-0.414,-0.413,-0.412,-0.411,-0.41,-0.409,-0.408,-0.407,-0.406,-0.405,
-0.404,-0.403,-0.402,-0.401,-0.4,-0.399,-0.398,-0.397,-0.396,-0.395,-0.394,
-0.393,-0.392,-0.391,-0.39,-0.389,-0.388,-0.387,-0.386,-0.385,-0.384,-0.383,
-0.382,-0.381,-0.38,-0.379,-0.378,-0.377,-0.376,-0.375,-0.374,-0.373,-0.372,
-0.371,-0.37,-0.369,-0.368,-0.367,-0.366,-0.365,-0.364,-0.363,-0.362,-0.361,
-0.36,-0.359,-0.358,-0.357,-0.356,-0.355,-0.354,-0.353,-0.352,-0.351,-0.35,
-0.349,-0.348,-0.347,-0.346,-0.345,-0.344,-0.343,-0.342,-0.341,-0.34,-0.339,
-0.338,-0.337,-0.336,-0.335,-0.334,-0.333,-0.332,-0.331,-0.33,-0.329,-0.328,
-0.327,-0.326,-0.325,-0.324,-0.323,-0.322,-0.321,-0.32,-0.319,-0.318,-0.317,
-0.316,-0.315,-0.314,-0.313,-0.312,-0.311,-0.31,-0.309,-0.308,-0.307,-0.306,
-0.305,-0.304,-0.303,-0.302,-0.301,-0.3,-0.299,-0.298,-0.297,-0.296,-0.295,
-0.294,-0.293,-0.292,-0.291,-0.29,-0.289,-0.288,-0.287,-0.286,-0.285,-0.284,
-0.283,-0.282,-0.281,-0.28,-0.279,-0.278,-0.277,-0.276,-0.275,-0.274,-0.273,
-0.272,-0.271,-0.27,-0.269,-0.268,-0.267,-0.266,-0.265,-0.264,-0.263,-0.262,
-0.261,-0.26,-0.259,-0.258,-0.257,-0.256,-0.255,-0.254,-0.253,-0.252,-0.251,
-0.25,-0.249,-0.248,-0.247,-0.246,-0.245,-0.244,-0.243,-0.242,-0.241,-0.24,
-0.239,-0.238,-0.237,-0.236,-0.235,-0.234,-0.233,-0.232,-0.231,-0.23,-0.229,
-0.228,-0.227,-0.226,-0.225,-0.224,-0.223,-0.222,-0.221,-0.22,-0.219,-0.218,
-0.217,-0.216,-0.215,-0.214,-0.213,-0.212,-0.211,-0.21,-0.209,-0.208,-0.207,
-0.206,-0.205,-0.204,-0.203,-0.202,-0.201,-0.2,-0.199,-0.198,-0.197,-0.196,
-0.195,-0.194,-0.193,-0.192,-0.191,-0.19,-0.189,-0.188,-0.187,-0.186,-0.185,
-0.184,-0.183,-0.182,-0.181,-0.18,-0.179,-0.178,-0.177,-0.176,-0.175,-0.174,
-0.173,-0.172,-0.171,-0.17,-0.169,-0.168,-0.167,-0.166,-0.165,-0.164,-0.163,
-0.162,-0.161,-0.16,-0.159,-0.158,-0.157,-0.156,-0.155,-0.154,-0.153,-0.152,
-0.151,-0.15,-0.149,-0.148,-0.147,-0.146,-0.145,-0.144,-0.143,-0.142,-0.141,
-0.14,-0.139,-0.138,-0.137,-0.136,-0.135,-0.134,-0.133,-0.132,-0.131,-0.13,
-0.129,-0.128,-0.127,-0.126,-0.125,-0.124,-0.123,-0.122,-0.121,-0.12,-0.119,
-0.118,-0.117,-0.116,-0.115,-0.114,-0.113,-0.112,-0.111,-0.11,-0.109,-0.108,
-0.107,-0.106,-0.105,-0.104,-0.103,-0.102,-0.101,-0.1,-0.0990000000000001,
-0.0980000000000001,-0.0970000000000001,-0.0960000000000001,-0.0950000000000001,
-0.0940000000000001,-0.0930000000000001,-0.0920000000000001,-0.0910000000000001,
-0.0900000000000001,-0.0890000000000001,-0.0880000000000001,-0.0870000000000001,
-0.0860000000000001,-0.0850000000000001,-0.0840000000000001,-0.0830000000000001,
-0.0820000000000001,-0.0810000000000001,-0.0800000000000001,-0.0790000000000001,
-0.0780000000000001,-0.0770000000000001,-0.0760000000000001,-0.0750000000000001,
-0.0740000000000001,-0.0730000000000001,-0.0720000000000001,-0.071,-0.07,
-0.069,-0.068,-0.067,-0.066,-0.065,-0.064,-0.063,-0.062,-0.061,-0.06,-0.059,
-0.058,-0.057,-0.056,-0.055,-0.054,-0.053,-0.052,-0.051,-0.05,-0.049,-0.048,
-0.047,-0.046,-0.045,-0.044,-0.043,-0.042,-0.041,-0.04,-0.039,-0.038,-0.037,
-0.036,-0.035,-0.034,-0.033,-0.032,-0.031,-0.03,-0.029,-0.028,-0.027,-0.026,
-0.025,-0.024,-0.023,-0.022,-0.021,-0.02,-0.019,-0.018,-0.017,-0.016,-0.015,
-0.014,-0.013,-0.012,-0.011,-0.01,-0.009,-0.008,-0.007,-0.006,-0.005,-0.004,
-0.003,-0.002,-0.001,0.),(0.,2.),.UNSPECIFIED.)
GEOMETRIC_REPRESENTATION_ITEM()
RATIONAL_B_SPLINE_SURFACE(((1.,1.),(1.,1.),(1.,1.),(1.,1.),(1.,1.),(1.,
1.),(1.,1.),(1.,1.),(1.,1.),(1.,1.),(1.,1.),(1.,1.),(1.,1.),(1.,1.),(1.,
1.),(1.,1.),(1.,1.),(1.,1.),(1.,1.),(1.,1.),(1.,1.),(1.,1.),(1.,1.),(1.,
1.),(1.,1.),(1.,1.),(1.,1.),(1.,1.),(1.,1.),(1.,1.),(1.,1.),(1.,1.),(1.,
1.),(1.,1.),(1.,1.),(1.,1.),(1.,1.),(1.,1.),(1.,1.),(1.,1.),(1.,1.),(1.,
1.),(1.,1.),(1.,1.),(1.,1.),(1.,1.),(1.,1.),(1.,1.),(1.,1.),(1.,1.),(1.,
1.),(1.,1.),(1.,1.),(1.,1.),(1.,1.),(1.,1.),(1.,1.),(1.,1.),(1.,1.),(1.,
1.),(1.,1.),(1.,1.),(1.,1.),(1.,1.),(1.,1.),(1.,1.),(1.,1.),(1.,1.),(1.,
1.),(1.,1.),(1.,1.),(1.,1.),(1.,1.),(1.,1.),(1.,1.),(1.,1.),(1.,1.),(1.,
1.),(1.,1.),(1.,1.),(1.,1.),(1.,1.),(1.,1.),(1.,1.),(1.,1.),(1.,1.),(1.,
1.),(1.,1.),(1.,1.),(1.,1.),(1.,1.),(1.,1.),(1.,1.),(1.,1.),(1.,1.),(1.,
1.),(1.,1.),(1.,1.),(1.,1.),(1.,1.),(1.,1.),(1.,1.),(1.,1.),(1.,1.),(1.,
1.),(1.,1.),(1.,1.),(1.,1.),(1.,1.),(1.,1.),(1.,1.),(1.,1.),(1.,1.),(1.,
1.),(1.,1.),(1.,1.),(1.,1.),(1.,1.),(1.,1.),(1.,1.),(1.,1.),(1.,1.),(1.,
1.),(1.,1.),(1.,1.),(1.,1.),(1.,1.),(1.,1.),(1.,1.),(1.,1.),(1.,1.),(1.,
1.),(1.,1.),(1.,1.),(1.,1.),(1.,1.),(1.,1.),(1.,1.),(1.,1.),(1.,1.),(1.,
1.),(1.,1.),(1.,1.),(1.,1.),(1.,1.),(1.,1.),(1.,1.),(1.,1.),(1.,1.),(1.,
1.),(1.,1.),(1.,1.),(1.,1.),(1.,1.),(1.,1.),(1.,1.),(1.,1.),(1.,1.),(1.,
1.),(1.,1.),(1.,1.),(1.,1.),(1.,1.),(1.,1.),(1.,1.),(1.,1.),(1.,1.),(1.,
1.),(1.,1.),(1.,1.),(1.,1.),(1.,1.),(1.,1.),(1.,1.),(1.,1.),(1.,1.),(1.,
1.),(1.,1.),(1.,1.),(1.,1.),(1.,1.),(1.,1.),(1.,1.),(1.,1.),(1.,1.),(1.,
1.),(1.,1.),(1.,1.),(1.,1.),(1.,1.),(1.,1.),(1.,1.),(1.,1.),(1.,1.),(1.,
1.),(1.,1.),(1.,1.),(1.,1.),(1.,1.),(1.,1.),(1.,1.),(1.,1.),(1.,1.),(1.,
1.),(1.,1.),(1.,1.),(1.,1.),(1.,1.),(1.,1.),(1.,1.),(1.,1.),(1.,1.),(1.,
1.),(1.,1.),(1.,1.),(1.,1.),(1.,1.),(1.,1.),(1.,1.),(1.,1.),(1.,1.),(1.,
1.),(1.,1.),(1.,1.),(1.,1.),(1.,1.),(1.,1.),(1.,1.),(1.,1.),(1.,1.),(1.,
1.),(1.,1.),(1.,1.),(1.,1.),(1.,1.),(1.,1.),(1.,1.),(1.,1.),(1.,1.),(1.,
1.),(1.,1.),(1.,1.),(1.,1.),(1.,1.),(1.,1.),(1.,1.),(1.,1.),(1.,1.),(1.,
1.),(1.,1.),(1.,1.),(1.,1.),(1.,1.),(1.,1.),(1.,1.),(1.,1.),(1.,1.),(1.,
1.),(1.,1.),(1.,1.),(1.,1.),(1.,1.),(1.,1.),(1.,1.),(1.,1.),(1.,1.),(1.,
1.),(1.,1.),(1.,1.),(1.,1.),(1.,1.),(1.,1.),(1.,1.),(1.,1.),(1.,1.),(1.,
1.),(1.,1.),(1.,1.),(1.,1.),(1.,1.),(1.,1.),(1.,1.),(1.,1.),(1.,1.),(1.,
1.),(1.,1.),(1.,1.),(1.,1.),(1.,1.),(1.,1.),(1.,1.),(1.,1.),(1.,1.),(1.,
1.),(1.,1.),(1.,1.),(1.,1.),(1.,1.),(1.,1.),(1.,1.),(1.,1.),(1.,1.),(1.,
1.),(1.,1.),(1.,1.),(1.,1.),(1.,1.),(1.,1.),(1.,1.),(1.,1.),(1.,1.),(1.,
1.),(1.,1.),(1.,1.),(1.,1.),(1.,1.),(1.,1.),(1.,1.),(1.,1.),(1.,1.),(1.,
1.),(1.,1.),(1.,1.),(1.,1.),(1.,1.),(1.,1.),(1.,1.),(1.,1.),(1.,1.),(1.,
1.),(1.,1.),(1.,1.),(1.,1.),(1.,1.),(1.,1.),(1.,1.),(1.,1.),(1.,1.),(1.,
1.),(1.,1.),(1.,1.),(1.,1.),(1.,1.),(1.,1.),(1.,1.),(1.,1.),(1.,1.),(1.,
1.),(1.,1.),(1.,1.),(1.,1.),(1.,1.),(1.,1.),(1.,1.),(1.,1.),(1.,1.),(1.,
1.),(1.,1.),(1.,1.),(1.,1.),(1.,1.),(1.,1.),(1.,1.),(1.,1.),(1.,1.),(1.,
1.),(1.,1.),(1.,1.),(1.,1.),(1.,1.),(1.,1.),(1.,1.),(1.,1.),(1.,1.),(1.,
1.),(1.,1.),(1.,1.),(1.,1.),(1.,1.),(1.,1.),(1.,1.),(1.,1.),(1.,1.),(1.,
1.),(1.,1.),(1.,1.),(1.,1.),(1.,1.),(1.,1.),(1.,1.),(1.,1.),(1.,1.),(1.,
1.),(1.,1.),(1.,1.),(1.,1.),(1.,1.),(1.,1.),(1.,1.),(1.,1.),(1.,1.),(1.,
1.),(1.,1.),(1.,1.),(1.,1.),(1.,1.),(1.,1.),(1.,1.),(1.,1.),(1.,1.),(1.,
1.),(1.,1.),(1.,1.),(1.,1.),(1.,1.),(1.,1.),(1.,1.),(1.,1.),(1.,1.),(1.,
1.),(1.,1.),(1.,1.),(1.,1.),(1.,1.),(1.,1.),(1.,1.),(1.,1.),(1.,1.),(1.,
1.),(1.,1.),(1.,1.),(1.,1.),(1.,1.),(1.,1.),(1.,1.),(1.,1.),(1.,1.),(1.,
1.),(1.,1.),(1.,1.),(1.,1.),(1.,1.),(1.,1.),(1.,1.),(1.,1.),(1.,1.),(1.,
1.),(1.,1.),(1.,1.),(1.,1.),(1.,1.),(1.,1.),(1.,1.),(1.,1.),(1.,1.),(1.,
1.),(1.,1.),(1.,1.),(1.,1.),(1.,1.),(1.,1.),(1.,1.),(1.,1.),(1.,1.),(1.,
1.),(1.,1.),(1.,1.),(1.,1.),(1.,1.),(1.,1.),(1.,1.),(1.,1.),(1.,1.),(1.,
1.),(1.,1.),(1.,1.),(1.,1.),(1.,1.),(1.,1.),(1.,1.),(1.,1.),(1.,1.),(1.,
1.),(1.,1.),(1.,1.),(1.,1.),(1.,1.),(1.,1.),(1.,1.),(1.,1.),(1.,1.),(1.,
1.),(1.,1.),(1.,1.),(1.,1.),(1.,1.),(1.,1.),(1.,1.),(1.,1.),(1.,1.),(1.,
1.),(1.,1.),(1.,1.),(1.,1.),(1.,1.),(1.,1.),(1.,1.),(1.,1.),(1.,1.),(1.,
1.),(1.,1.),(1.,1.),(1.,1.),(1.,1.),(1.,1.),(1.,1.),(1.,1.),(1.,1.),(1.,
1.),(1.,1.),(1.,1.),(1.,1.),(1.,1.),(1.,1.),(1.,1.),(1.,1.),(1.,1.),(1.,
1.),(1.,1.),(1.,1.),(1.,1.),(1.,1.),(1.,1.),(1.,1.),(1.,1.),(1.,1.),(1.,
1.),(1.,1.),(1.,1.),(1.,1.),(1.,1.),(1.,1.),(1.,1.),(1.,1.),(1.,1.),(1.,
1.),(1.,1.),(1.,1.),(1.,1.),(1.,1.),(1.,1.),(1.,1.),(1.,1.),(1.,1.),(1.,
1.),(1.,1.),(1.,1.),(1.,1.),(1.,1.),(1.,1.),(1.,1.),(1.,1.),(1.,1.),(1.,
1.),(1.,1.),(1.,1.),(1.,1.),(1.,1.),(1.,1.),(1.,1.),(1.,1.),(1.,1.),(1.,
1.),(1.,1.),(1.,1.),(1.,1.),(1.,1.),(1.,1.),(1.,1.),(1.,1.),(1.,1.),(1.,
1.),(1.,1.),(1.,1.),(1.,1.),(1.,1.),(1.,1.),(1.,1.),(1.,1.),(1.,1.),(1.,
1.),(1.,1.),(1.,1.),(1.,1.),(1.,1.),(1.,1.),(1.,1.),(1.,1.),(1.,1.),(1.,
1.),(1.,1.),(1.,1.),(1.,1.),(1.,1.),(1.,1.),(1.,1.),(1.,1.),(1.,1.),(1.,
1.),(1.,1.),(1.,1.),(1.,1.),(1.,1.),(1.,1.),(1.,1.),(1.,1.),(1.,1.),(1.,
1.),(1.,1.),(1.,1.),(1.,1.),(1.,1.),(1.,1.),(1.,1.),(1.,1.),(1.,1.),(1.,
1.),(1.,1.),(1.,1.),(1.,1.),(1.,1.),(1.,1.),(1.,1.),(1.,1.),(1.,1.),(1.,
1.),(1.,1.),(1.,1.),(1.,1.),(1.,1.),(1.,1.),(1.,1.),(1.,1.),(1.,1.),(1.,
1.),(1.,1.),(1.,1.),(1.,1.),(1.,1.),(1.,1.),(1.,1.),(1.,1.),(1.,1.),(1.,
1.),(1.,1.),(1.,1.),(1.,1.),(1.,1.),(1.,1.),(1.,1.),(1.,1.),(1.,1.),(1.,
1.),(1.,1.),(1.,1.),(1.,1.),(1.,1.),(1.,1.),(1.,1.),(1.,1.),(1.,1.),(1.,
1.),(1.,1.),(1.,1.),(1.,1.),(1.,1.),(1.,1.),(1.,1.),(1.,1.),(1.,1.),(1.,
1.),(1.,1.),(1.,1.),(1.,1.),(1.,1.),(1.,1.),(1.,1.),(1.,1.),(1.,1.),(1.,
1.),(1.,1.),(1.,1.),(1.,1.),(1.,1.),(1.,1.),(1.,1.),(1.,1.),(1.,1.),(1.,
1.),(1.,1.),(1.,1.),(1.,1.),(1.,1.),(1.,1.),(1.,1.),(1.,1.),(1.,1.),(1.,
1.),(1.,1.),(1.,1.),(1.,1.),(1.,1.),(1.,1.),(1.,1.),(1.,1.),(1.,1.),(1.,
1.),(1.,1.),(1.,1.),(1.,1.),(1.,1.),(1.,1.),(1.,1.),(1.,1.),(1.,1.),(1.,
1.),(1.,1.),(1.,1.),(1.,1.),(1.,1.),(1.,1.),(1.,1.),(1.,1.),(1.,1.),(1.,
1.),(1.,1.),(1.,1.),(1.,1.),(1.,1.),(1.,1.),(1.,1.),(1.,1.),(1.,1.),(1.,
1.),(1.,1.),(1.,1.),(1.,1.),(1.,1.),(1.,1.),(1.,1.),(1.,1.),(1.,1.),(1.,
1.),(1.,1.),(1.,1.),(1.,1.),(1.,1.),(1.,1.),(1.,1.),(1.,1.),(1.,1.),(1.,
1.),(1.,1.),(1.,1.),(1.,1.),(1.,1.),(1.,1.),(1.,1.),(1.,1.),(1.,1.),(1.,
1.),(1.,1.),(1.,1.),(1.,1.),(1.,1.),(1.,1.),(1.,1.),(1.,1.),(1.,1.),(1.,
1.),(1.,1.),(1.,1.),(1.,1.),(1.,1.),(1.,1.),(1.,1.),(1.,1.),(1.,1.),(1.,
1.),(1.,1.),(1.,1.),(1.,1.),(1.,1.),(1.,1.),(1.,1.),(1.,1.),(1.,1.),(1.,
1.),(1.,1.),(1.,1.),(1.,1.),(1.,1.),(1.,1.),(1.,1.),(1.,1.),(1.,1.),(1.,
1.),(1.,1.),(1.,1.),(1.,1.),(1.,1.),(1.,1.),(1.,1.),(1.,1.),(1.,1.),(1.,
1.),(1.,1.),(1.,1.),(1.,1.),(1.,1.),(1.,1.),(1.,1.),(1.,1.),(1.,1.),(1.,
1.),(1.,1.),(1.,1.),(1.,1.),(1.,1.),(1.,1.),(1.,1.),(1.,1.),(1.,1.),(1.,
1.),(1.,1.),(1.,1.),(1.,1.),(1.,1.),(1.,1.),(1.,1.),(1.,1.),(1.,1.),(1.,
1.),(1.,1.),(1.,1.),(1.,1.),(1.,1.),(1.,1.),(1.,1.),(1.,1.),(1.,1.),(1.,
1.),(1.,1.),(1.,1.),(1.,1.),(1.,1.),(1.,1.),(1.,1.),(1.,1.),(1.,1.),(1.,
1.),(1.,1.),(1.,1.),(1.,1.),(1.,1.),(1.,1.),(1.,1.),(1.,1.),(1.,1.),(1.,
1.),(1.,1.),(1.,1.),(1.,1.),(1.,1.),(1.,1.),(1.,1.),(1.,1.),(1.,1.),(1.,
1.),(1.,1.),(1.,1.),(1.,1.),(1.,1.),(1.,1.),(1.,1.),(1.,1.),(1.,1.),(1.,
1.),(1.,1.),(1.,1.),(1.,1.),(1.,1.),(1.,1.),(1.,1.),(1.,1.),(1.,1.),(1.,
1.),(1.,1.),(1.,1.),(1.,1.),(1.,1.),(1.,1.),(1.,1.),(1.,1.),(1.,1.),(1.,
1.),(1.,1.),(1.,1.),(1.,1.),(1.,1.),(1.,1.),(1.,1.),(1.,1.),(1.,1.),(1.,
1.),(1.,1.),(1.,1.),(1.,1.),(1.,1.),(1.,1.),(1.,1.),(1.,1.),(1.,1.),(1.,
1.),(1.,1.),(1.,1.),(1.,1.),(1.,1.),(1.,1.),(1.,1.),(1.,1.),(1.,1.),(1.,
1.),(1.,1.),(1.,1.),(1.,1.),(1.,1.),(1.,1.),(1.,1.),(1.,1.),(1.,1.),(1.,
1.),(1.,1.),(1.,1.),(1.,1.),(1.,1.),(1.,1.),(1.,1.),(1.,1.),(1.,1.),(1.,
1.),(1.,1.),(1.,1.),(1.,1.),(1.,1.),(1.,1.),(1.,1.),(1.,1.),(1.,1.),(1.,
1.),(1.,1.),(1.,1.),(1.,1.),(1.,1.),(1.,1.),(1.,1.),(1.,1.),(1.,1.),(1.,
1.),(1.,1.),(1.,1.),(1.,1.),(1.,1.),(1.,1.),(1.,1.),(1.,1.),(1.,1.),(1.,
1.),(1.,1.),(1.,1.),(1.,1.),(1.,1.),(1.,1.),(1.,1.),(1.,1.),(1.,1.),(1.,
1.),(1.,1.),(1.,1.),(1.,1.),(1.,1.),(1.,1.),(1.,1.),(1.,1.),(1.,1.),(1.,
1.),(1.,1.),(1.,1.),(1.,1.),(1.,1.),(1.,1.),(1.,1.),(1.,1.),(1.,1.),(1.,
1.)))
REPRESENTATION_ITEM('')
SURFACE()
);
#265=(
BOUNDED_SURFACE()
B_SPLINE_SURFACE(5,1,((#88405,#88406),(#88407,#88408),(#88409,#88410),(#88411,
#88412),(#88413,#88414),(#88415,#88416),(#88417,#88418),(#88419,#88420),
(#88421,#88422),(#88423,#88424),(#88425,#88426),(#88427,#88428),(#88429,
#88430),(#88431,#88432),(#88433,#88434),(#88435,#88436),(#88437,#88438),
(#88439,#88440),(#88441,#88442),(#88443,#88444),(#88445,#88446),(#88447,
#88448),(#88449,#88450),(#88451,#88452),(#88453,#88454),(#88455,#88456),
(#88457,#88458),(#88459,#88460),(#88461,#88462),(#88463,#88464),(#88465,
#88466),(#88467,#88468),(#88469,#88470),(#88471,#88472),(#88473,#88474),
(#88475,#88476),(#88477,#88478),(#88479,#88480),(#88481,#88482),(#88483,
#88484),(#88485,#88486),(#88487,#88488),(#88489,#88490),(#88491,#88492),
(#88493,#88494),(#88495,#88496),(#88497,#88498),(#88499,#88500),(#88501,
#88502),(#88503,#88504),(#88505,#88506),(#88507,#88508),(#88509,#88510),
(#88511,#88512),(#88513,#88514),(#88515,#88516),(#88517,#88518),(#88519,
#88520),(#88521,#88522),(#88523,#88524),(#88525,#88526),(#88527,#88528),
(#88529,#88530),(#88531,#88532),(#88533,#88534),(#88535,#88536),(#88537,
#88538),(#88539,#88540),(#88541,#88542),(#88543,#88544),(#88545,#88546),
(#88547,#88548),(#88549,#88550),(#88551,#88552),(#88553,#88554),(#88555,
#88556),(#88557,#88558),(#88559,#88560),(#88561,#88562),(#88563,#88564),
(#88565,#88566),(#88567,#88568),(#88569,#88570),(#88571,#88572),(#88573,
#88574),(#88575,#88576),(#88577,#88578),(#88579,#88580),(#88581,#88582),
(#88583,#88584),(#88585,#88586),(#88587,#88588),(#88589,#88590),(#88591,
#88592),(#88593,#88594),(#88595,#88596),(#88597,#88598),(#88599,#88600),
(#88601,#88602),(#88603,#88604),(#88605,#88606),(#88607,#88608),(#88609,
#88610),(#88611,#88612),(#88613,#88614),(#88615,#88616),(#88617,#88618),
(#88619,#88620),(#88621,#88622),(#88623,#88624),(#88625,#88626),(#88627,
#88628),(#88629,#88630),(#88631,#88632),(#88633,#88634),(#88635,#88636),
(#88637,#88638),(#88639,#88640),(#88641,#88642),(#88643,#88644),(#88645,
#88646),(#88647,#88648),(#88649,#88650),(#88651,#88652),(#88653,#88654),
(#88655,#88656),(#88657,#88658),(#88659,#88660),(#88661,#88662),(#88663,
#88664),(#88665,#88666),(#88667,#88668),(#88669,#88670),(#88671,#88672),
(#88673,#88674),(#88675,#88676),(#88677,#88678),(#88679,#88680),(#88681,
#88682),(#88683,#88684),(#88685,#88686),(#88687,#88688),(#88689,#88690),
(#88691,#88692),(#88693,#88694),(#88695,#88696),(#88697,#88698),(#88699,
#88700),(#88701,#88702),(#88703,#88704),(#88705,#88706),(#88707,#88708),
(#88709,#88710),(#88711,#88712),(#88713,#88714),(#88715,#88716),(#88717,
#88718),(#88719,#88720),(#88721,#88722),(#88723,#88724),(#88725,#88726),
(#88727,#88728),(#88729,#88730),(#88731,#88732),(#88733,#88734),(#88735,
#88736),(#88737,#88738),(#88739,#88740),(#88741,#88742),(#88743,#88744),
(#88745,#88746),(#88747,#88748),(#88749,#88750),(#88751,#88752),(#88753,
#88754),(#88755,#88756),(#88757,#88758),(#88759,#88760),(#88761,#88762),
(#88763,#88764),(#88765,#88766),(#88767,#88768),(#88769,#88770),(#88771,
#88772),(#88773,#88774),(#88775,#88776),(#88777,#88778),(#88779,#88780),
(#88781,#88782),(#88783,#88784),(#88785,#88786),(#88787,#88788),(#88789,
#88790),(#88791,#88792),(#88793,#88794),(#88795,#88796),(#88797,#88798),
(#88799,#88800),(#88801,#88802),(#88803,#88804),(#88805,#88806),(#88807,
#88808),(#88809,#88810),(#88811,#88812),(#88813,#88814),(#88815,#88816),
(#88817,#88818),(#88819,#88820),(#88821,#88822),(#88823,#88824),(#88825,
#88826),(#88827,#88828),(#88829,#88830),(#88831,#88832),(#88833,#88834),
(#88835,#88836),(#88837,#88838),(#88839,#88840),(#88841,#88842),(#88843,
#88844),(#88845,#88846),(#88847,#88848),(#88849,#88850),(#88851,#88852),
(#88853,#88854),(#88855,#88856),(#88857,#88858),(#88859,#88860),(#88861,
#88862),(#88863,#88864),(#88865,#88866),(#88867,#88868),(#88869,#88870),
(#88871,#88872),(#88873,#88874),(#88875,#88876),(#88877,#88878),(#88879,
#88880),(#88881,#88882),(#88883,#88884),(#88885,#88886),(#88887,#88888),
(#88889,#88890),(#88891,#88892),(#88893,#88894),(#88895,#88896),(#88897,
#88898),(#88899,#88900),(#88901,#88902),(#88903,#88904),(#88905,#88906),
(#88907,#88908),(#88909,#88910),(#88911,#88912),(#88913,#88914),(#88915,
#88916),(#88917,#88918),(#88919,#88920),(#88921,#88922),(#88923,#88924),
(#88925,#88926),(#88927,#88928),(#88929,#88930),(#88931,#88932),(#88933,
#88934),(#88935,#88936),(#88937,#88938),(#88939,#88940),(#88941,#88942),
(#88943,#88944),(#88945,#88946),(#88947,#88948),(#88949,#88950),(#88951,
#88952),(#88953,#88954),(#88955,#88956),(#88957,#88958),(#88959,#88960),
(#88961,#88962),(#88963,#88964),(#88965,#88966),(#88967,#88968),(#88969,
#88970),(#88971,#88972),(#88973,#88974),(#88975,#88976),(#88977,#88978),
(#88979,#88980),(#88981,#88982),(#88983,#88984),(#88985,#88986),(#88987,
#88988),(#88989,#88990),(#88991,#88992),(#88993,#88994),(#88995,#88996),
(#88997,#88998),(#88999,#89000),(#89001,#89002),(#89003,#89004),(#89005,
#89006),(#89007,#89008),(#89009,#89010),(#89011,#89012),(#89013,#89014),
(#89015,#89016),(#89017,#89018),(#89019,#89020),(#89021,#89022),(#89023,
#89024),(#89025,#89026),(#89027,#89028),(#89029,#89030),(#89031,#89032),
(#89033,#89034),(#89035,#89036),(#89037,#89038),(#89039,#89040),(#89041,
#89042),(#89043,#89044),(#89045,#89046),(#89047,#89048),(#89049,#89050),
(#89051,#89052),(#89053,#89054),(#89055,#89056),(#89057,#89058),(#89059,
#89060),(#89061,#89062),(#89063,#89064),(#89065,#89066),(#89067,#89068),
(#89069,#89070),(#89071,#89072),(#89073,#89074),(#89075,#89076),(#89077,
#89078),(#89079,#89080),(#89081,#89082),(#89083,#89084),(#89085,#89086),
(#89087,#89088),(#89089,#89090),(#89091,#89092),(#89093,#89094),(#89095,
#89096),(#89097,#89098),(#89099,#89100),(#89101,#89102),(#89103,#89104),
(#89105,#89106),(#89107,#89108),(#89109,#89110),(#89111,#89112),(#89113,
#89114),(#89115,#89116),(#89117,#89118),(#89119,#89120),(#89121,#89122),
(#89123,#89124),(#89125,#89126),(#89127,#89128),(#89129,#89130),(#89131,
#89132),(#89133,#89134),(#89135,#89136),(#89137,#89138),(#89139,#89140),
(#89141,#89142),(#89143,#89144),(#89145,#89146),(#89147,#89148),(#89149,
#89150),(#89151,#89152),(#89153,#89154),(#89155,#89156),(#89157,#89158),
(#89159,#89160),(#89161,#89162),(#89163,#89164),(#89165,#89166),(#89167,
#89168),(#89169,#89170),(#89171,#89172),(#89173,#89174),(#89175,#89176),
(#89177,#89178),(#89179,#89180),(#89181,#89182),(#89183,#89184),(#89185,
#89186),(#89187,#89188),(#89189,#89190),(#89191,#89192),(#89193,#89194),
(#89195,#89196),(#89197,#89198),(#89199,#89200),(#89201,#89202),(#89203,
#89204),(#89205,#89206),(#89207,#89208),(#89209,#89210),(#89211,#89212),
(#89213,#89214),(#89215,#89216),(#89217,#89218),(#89219,#89220),(#89221,
#89222),(#89223,#89224),(#89225,#89226),(#89227,#89228),(#89229,#89230),
(#89231,#89232),(#89233,#89234),(#89235,#89236),(#89237,#89238),(#89239,
#89240),(#89241,#89242),(#89243,#89244),(#89245,#89246),(#89247,#89248),
(#89249,#89250),(#89251,#89252),(#89253,#89254),(#89255,#89256),(#89257,
#89258),(#89259,#89260),(#89261,#89262),(#89263,#89264),(#89265,#89266),
(#89267,#89268),(#89269,#89270),(#89271,#89272),(#89273,#89274),(#89275,
#89276),(#89277,#89278),(#89279,#89280),(#89281,#89282),(#89283,#89284),
(#89285,#89286),(#89287,#89288),(#89289,#89290),(#89291,#89292),(#89293,
#89294),(#89295,#89296),(#89297,#89298),(#89299,#89300),(#89301,#89302),
(#89303,#89304),(#89305,#89306),(#89307,#89308),(#89309,#89310),(#89311,
#89312),(#89313,#89314),(#89315,#89316),(#89317,#89318),(#89319,#89320),
(#89321,#89322),(#89323,#89324),(#89325,#89326),(#89327,#89328),(#89329,
#89330),(#89331,#89332),(#89333,#89334),(#89335,#89336),(#89337,#89338),
(#89339,#89340),(#89341,#89342),(#89343,#89344),(#89345,#89346),(#89347,
#89348),(#89349,#89350),(#89351,#89352),(#89353,#89354),(#89355,#89356),
(#89357,#89358),(#89359,#89360),(#89361,#89362),(#89363,#89364),(#89365,
#89366),(#89367,#89368),(#89369,#89370),(#89371,#89372),(#89373,#89374),
(#89375,#89376),(#89377,#89378),(#89379,#89380),(#89381,#89382),(#89383,
#89384),(#89385,#89386),(#89387,#89388),(#89389,#89390),(#89391,#89392),
(#89393,#89394),(#89395,#89396),(#89397,#89398),(#89399,#89400),(#89401,
#89402),(#89403,#89404),(#89405,#89406),(#89407,#89408),(#89409,#89410),
(#89411,#89412),(#89413,#89414),(#89415,#89416),(#89417,#89418),(#89419,
#89420),(#89421,#89422),(#89423,#89424),(#89425,#89426),(#89427,#89428),
(#89429,#89430),(#89431,#89432),(#89433,#89434),(#89435,#89436),(#89437,
#89438),(#89439,#89440),(#89441,#89442),(#89443,#89444),(#89445,#89446),
(#89447,#89448),(#89449,#89450),(#89451,#89452),(#89453,#89454),(#89455,
#89456),(#89457,#89458),(#89459,#89460),(#89461,#89462),(#89463,#89464),
(#89465,#89466),(#89467,#89468),(#89469,#89470),(#89471,#89472),(#89473,
#89474),(#89475,#89476),(#89477,#89478),(#89479,#89480),(#89481,#89482),
(#89483,#89484),(#89485,#89486),(#89487,#89488),(#89489,#89490),(#89491,
#89492),(#89493,#89494),(#89495,#89496),(#89497,#89498),(#89499,#89500),
(#89501,#89502),(#89503,#89504),(#89505,#89506),(#89507,#89508),(#89509,
#89510),(#89511,#89512),(#89513,#89514),(#89515,#89516),(#89517,#89518),
(#89519,#89520),(#89521,#89522),(#89523,#89524),(#89525,#89526),(#89527,
#89528),(#89529,#89530),(#89531,#89532),(#89533,#89534),(#89535,#89536),
(#89537,#89538),(#89539,#89540),(#89541,#89542),(#89543,#89544),(#89545,
#89546),(#89547,#89548),(#89549,#89550),(#89551,#89552),(#89553,#89554),
(#89555,#89556),(#89557,#89558),(#89559,#89560),(#89561,#89562),(#89563,
#89564),(#89565,#89566),(#89567,#89568),(#89569,#89570),(#89571,#89572),
(#89573,#89574),(#89575,#89576),(#89577,#89578),(#89579,#89580),(#89581,
#89582),(#89583,#89584),(#89585,#89586),(#89587,#89588),(#89589,#89590),
(#89591,#89592),(#89593,#89594),(#89595,#89596),(#89597,#89598),(#89599,
#89600),(#89601,#89602),(#89603,#89604),(#89605,#89606),(#89607,#89608),
(#89609,#89610),(#89611,#89612),(#89613,#89614),(#89615,#89616),(#89617,
#89618),(#89619,#89620),(#89621,#89622),(#89623,#89624),(#89625,#89626),
(#89627,#89628),(#89629,#89630),(#89631,#89632),(#89633,#89634),(#89635,
#89636),(#89637,#89638),(#89639,#89640),(#89641,#89642),(#89643,#89644),
(#89645,#89646),(#89647,#89648),(#89649,#89650),(#89651,#89652),(#89653,
#89654),(#89655,#89656),(#89657,#89658),(#89659,#89660),(#89661,#89662),
(#89663,#89664),(#89665,#89666),(#89667,#89668),(#89669,#89670),(#89671,
#89672),(#89673,#89674),(#89675,#89676),(#89677,#89678),(#89679,#89680),
(#89681,#89682),(#89683,#89684),(#89685,#89686),(#89687,#89688),(#89689,
#89690),(#89691,#89692),(#89693,#89694),(#89695,#89696),(#89697,#89698),
(#89699,#89700),(#89701,#89702),(#89703,#89704),(#89705,#89706),(#89707,
#89708),(#89709,#89710),(#89711,#89712),(#89713,#89714),(#89715,#89716),
(#89717,#89718),(#89719,#89720),(#89721,#89722),(#89723,#89724),(#89725,
#89726),(#89727,#89728),(#89729,#89730),(#89731,#89732),(#89733,#89734),
(#89735,#89736),(#89737,#89738),(#89739,#89740),(#89741,#89742),(#89743,
#89744),(#89745,#89746),(#89747,#89748),(#89749,#89750),(#89751,#89752),
(#89753,#89754),(#89755,#89756),(#89757,#89758),(#89759,#89760),(#89761,
#89762),(#89763,#89764),(#89765,#89766),(#89767,#89768),(#89769,#89770),
(#89771,#89772),(#89773,#89774),(#89775,#89776),(#89777,#89778),(#89779,
#89780),(#89781,#89782),(#89783,#89784),(#89785,#89786),(#89787,#89788),
(#89789,#89790),(#89791,#89792),(#89793,#89794),(#89795,#89796),(#89797,
#89798),(#89799,#89800),(#89801,#89802),(#89803,#89804),(#89805,#89806),
(#89807,#89808),(#89809,#89810),(#89811,#89812),(#89813,#89814),(#89815,
#89816),(#89817,#89818),(#89819,#89820),(#89821,#89822),(#89823,#89824),
(#89825,#89826),(#89827,#89828),(#89829,#89830),(#89831,#89832),(#89833,
#89834),(#89835,#89836),(#89837,#89838),(#89839,#89840),(#89841,#89842),
(#89843,#89844),(#89845,#89846),(#89847,#89848),(#89849,#89850),(#89851,
#89852),(#89853,#89854),(#89855,#89856),(#89857,#89858),(#89859,#89860),
(#89861,#89862),(#89863,#89864),(#89865,#89866),(#89867,#89868),(#89869,
#89870),(#89871,#89872),(#89873,#89874),(#89875,#89876),(#89877,#89878),
(#89879,#89880),(#89881,#89882),(#89883,#89884),(#89885,#89886),(#89887,
#89888),(#89889,#89890),(#89891,#89892),(#89893,#89894),(#89895,#89896),
(#89897,#89898),(#89899,#89900),(#89901,#89902),(#89903,#89904),(#89905,
#89906),(#89907,#89908),(#89909,#89910),(#89911,#89912),(#89913,#89914),
(#89915,#89916),(#89917,#89918),(#89919,#89920),(#89921,#89922),(#89923,
#89924),(#89925,#89926),(#89927,#89928),(#89929,#89930),(#89931,#89932),
(#89933,#89934),(#89935,#89936),(#89937,#89938),(#89939,#89940),(#89941,
#89942),(#89943,#89944),(#89945,#89946),(#89947,#89948),(#89949,#89950),
(#89951,#89952),(#89953,#89954),(#89955,#89956),(#89957,#89958),(#89959,
#89960),(#89961,#89962),(#89963,#89964),(#89965,#89966),(#89967,#89968),
(#89969,#89970),(#89971,#89972),(#89973,#89974),(#89975,#89976),(#89977,
#89978),(#89979,#89980),(#89981,#89982),(#89983,#89984),(#89985,#89986),
(#89987,#89988),(#89989,#89990),(#89991,#89992),(#89993,#89994),(#89995,
#89996),(#89997,#89998),(#89999,#90000),(#90001,#90002),(#90003,#90004),
(#90005,#90006),(#90007,#90008),(#90009,#90010),(#90011,#90012),(#90013,
#90014),(#90015,#90016),(#90017,#90018),(#90019,#90020),(#90021,#90022),
(#90023,#90024),(#90025,#90026),(#90027,#90028),(#90029,#90030),(#90031,
#90032),(#90033,#90034),(#90035,#90036),(#90037,#90038),(#90039,#90040),
(#90041,#90042),(#90043,#90044),(#90045,#90046),(#90047,#90048),(#90049,
#90050),(#90051,#90052),(#90053,#90054),(#90055,#90056),(#90057,#90058),
(#90059,#90060),(#90061,#90062),(#90063,#90064),(#90065,#90066),(#90067,
#90068),(#90069,#90070),(#90071,#90072),(#90073,#90074),(#90075,#90076),
(#90077,#90078),(#90079,#90080),(#90081,#90082),(#90083,#90084),(#90085,
#90086),(#90087,#90088),(#90089,#90090),(#90091,#90092),(#90093,#90094),
(#90095,#90096),(#90097,#90098),(#90099,#90100),(#90101,#90102),(#90103,
#90104),(#90105,#90106),(#90107,#90108),(#90109,#90110),(#90111,#90112),
(#90113,#90114),(#90115,#90116),(#90117,#90118),(#90119,#90120),(#90121,
#90122),(#90123,#90124),(#90125,#90126),(#90127,#90128),(#90129,#90130),
(#90131,#90132),(#90133,#90134),(#90135,#90136),(#90137,#90138),(#90139,
#90140),(#90141,#90142),(#90143,#90144),(#90145,#90146),(#90147,#90148),
(#90149,#90150),(#90151,#90152),(#90153,#90154),(#90155,#90156),(#90157,
#90158),(#90159,#90160),(#90161,#90162),(#90163,#90164),(#90165,#90166),
(#90167,#90168),(#90169,#90170),(#90171,#90172),(#90173,#90174),(#90175,
#90176),(#90177,#90178),(#90179,#90180),(#90181,#90182),(#90183,#90184),
(#90185,#90186),(#90187,#90188),(#90189,#90190),(#90191,#90192),(#90193,
#90194),(#90195,#90196),(#90197,#90198),(#90199,#90200),(#90201,#90202),
(#90203,#90204),(#90205,#90206),(#90207,#90208),(#90209,#90210),(#90211,
#90212),(#90213,#90214),(#90215,#90216),(#90217,#90218),(#90219,#90220),
(#90221,#90222),(#90223,#90224),(#90225,#90226),(#90227,#90228),(#90229,
#90230),(#90231,#90232),(#90233,#90234),(#90235,#90236),(#90237,#90238),
(#90239,#90240),(#90241,#90242),(#90243,#90244),(#90245,#90246),(#90247,
#90248),(#90249,#90250),(#90251,#90252),(#90253,#90254),(#90255,#90256),
(#90257,#90258),(#90259,#90260),(#90261,#90262),(#90263,#90264),(#90265,
#90266),(#90267,#90268),(#90269,#90270),(#90271,#90272),(#90273,#90274),
(#90275,#90276),(#90277,#90278),(#90279,#90280),(#90281,#90282),(#90283,
#90284),(#90285,#90286),(#90287,#90288),(#90289,#90290),(#90291,#90292),
(#90293,#90294),(#90295,#90296),(#90297,#90298),(#90299,#90300),(#90301,
#90302),(#90303,#90304),(#90305,#90306),(#90307,#90308),(#90309,#90310),
(#90311,#90312),(#90313,#90314),(#90315,#90316),(#90317,#90318),(#90319,
#90320),(#90321,#90322),(#90323,#90324),(#90325,#90326),(#90327,#90328),
(#90329,#90330),(#90331,#90332),(#90333,#90334),(#90335,#90336),(#90337,
#90338),(#90339,#90340),(#90341,#90342),(#90343,#90344),(#90345,#90346),
(#90347,#90348),(#90349,#90350),(#90351,#90352),(#90353,#90354),(#90355,
#90356),(#90357,#90358),(#90359,#90360),(#90361,#90362),(#90363,#90364),
(#90365,#90366),(#90367,#90368),(#90369,#90370),(#90371,#90372),(#90373,
#90374),(#90375,#90376),(#90377,#90378),(#90379,#90380),(#90381,#90382),
(#90383,#90384),(#90385,#90386),(#90387,#90388),(#90389,#90390),(#90391,
#90392),(#90393,#90394),(#90395,#90396),(#90397,#90398),(#90399,#90400),
(#90401,#90402),(#90403,#90404),(#90405,#90406),(#90407,#90408),(#90409,
#90410),(#90411,#90412),(#90413,#90414)),.UNSPECIFIED.,.F.,.F.,.F.)
B_SPLINE_SURFACE_WITH_KNOTS((6,1,1,1,1,1,1,1,1,1,1,1,1,1,1,1,1,1,1,1,1,
1,1,1,1,1,1,1,1,1,1,1,1,1,1,1,1,1,1,1,1,1,1,1,1,1,1,1,1,1,1,1,1,1,1,1,1,
1,1,1,1,1,1,1,1,1,1,1,1,1,1,1,1,1,1,1,1,1,1,1,1,1,1,1,1,1,1,1,1,1,1,1,1,
1,1,1,1,1,1,1,1,1,1,1,1,1,1,1,1,1,1,1,1,1,1,1,1,1,1,1,1,1,1,1,1,1,1,1,1,
1,1,1,1,1,1,1,1,1,1,1,1,1,1,1,1,1,1,1,1,1,1,1,1,1,1,1,1,1,1,1,1,1,1,1,1,
1,1,1,1,1,1,1,1,1,1,1,1,1,1,1,1,1,1,1,1,1,1,1,1,1,1,1,1,1,1,1,1,1,1,1,1,
1,1,1,1,1,1,1,1,1,1,1,1,1,1,1,1,1,1,1,1,1,1,1,1,1,1,1,1,1,1,1,1,1,1,1,1,
1,1,1,1,1,1,1,1,1,1,1,1,1,1,1,1,1,1,1,1,1,1,1,1,1,1,1,1,1,1,1,1,1,1,1,1,
1,1,1,1,1,1,1,1,1,1,1,1,1,1,1,1,1,1,1,1,1,1,1,1,1,1,1,1,1,1,1,1,1,1,1,1,
1,1,1,1,1,1,1,1,1,1,1,1,1,1,1,1,1,1,1,1,1,1,1,1,1,1,1,1,1,1,1,1,1,1,1,1,
1,1,1,1,1,1,1,1,1,1,1,1,1,1,1,1,1,1,1,1,1,1,1,1,1,1,1,1,1,1,1,1,1,1,1,1,
1,1,1,1,1,1,1,1,1,1,1,1,1,1,1,1,1,1,1,1,1,1,1,1,1,1,1,1,1,1,1,1,1,1,1,1,
1,1,1,1,1,1,1,1,1,1,1,1,1,1,1,1,1,1,1,1,1,1,1,1,1,1,1,1,1,1,1,1,1,1,1,1,
1,1,1,1,1,1,1,1,1,1,1,1,1,1,1,1,1,1,1,1,1,1,1,1,1,1,1,1,1,1,1,1,1,1,1,1,
1,1,1,1,1,1,1,1,1,1,1,1,1,1,1,1,1,1,1,1,1,1,1,1,1,1,1,1,1,1,1,1,1,1,1,1,
1,1,1,1,1,1,1,1,1,1,1,1,1,1,1,1,1,1,1,1,1,1,1,1,1,1,1,1,1,1,1,1,1,1,1,1,
1,1,1,1,1,1,1,1,1,1,1,1,1,1,1,1,1,1,1,1,1,1,1,1,1,1,1,1,1,1,1,1,1,1,1,1,
1,1,1,1,1,1,1,1,1,1,1,1,1,1,1,1,1,1,1,1,1,1,1,1,1,1,1,1,1,1,1,1,1,1,1,1,
1,1,1,1,1,1,1,1,1,1,1,1,1,1,1,1,1,1,1,1,1,1,1,1,1,1,1,1,1,1,1,1,1,1,1,1,
1,1,1,1,1,1,1,1,1,1,1,1,1,1,1,1,1,1,1,1,1,1,1,1,1,1,1,1,1,1,1,1,1,1,1,1,
1,1,1,1,1,1,1,1,1,1,1,1,1,1,1,1,1,1,1,1,1,1,1,1,1,1,1,1,1,1,1,1,1,1,1,1,
1,1,1,1,1,1,1,1,1,1,1,1,1,1,1,1,1,1,1,1,1,1,1,1,1,1,1,1,1,1,1,1,1,1,1,1,
1,1,1,1,1,1,1,1,1,1,1,1,1,1,1,1,1,1,1,1,1,1,1,1,1,1,1,1,1,1,1,1,1,1,1,1,
1,1,1,1,1,1,1,1,1,1,1,1,1,1,1,1,1,1,1,1,1,1,1,1,1,1,1,1,1,1,1,1,1,1,1,1,
1,1,1,1,1,1,1,1,1,1,1,1,1,1,1,1,1,1,1,1,1,1,1,1,1,1,1,1,1,1,1,1,1,1,1,1,
1,1,1,1,1,1,1,1,1,1,1,1,1,1,1,1,1,1,1,1,1,1,1,1,1,1,1,1,1,1,1,1,1,1,1,1,
1,1,1,1,1,1,1,1,1,1,1,1,1,1,1,1,1,1,1,1,1,1,1,1,1,1,1,1,1,1,1,1,1,1,1,1,
1,1,1,1,1,1,1,1,1,1,1,1,1,1,1,1,1,1,1,1,1,1,1,1,1,1,1,1,1,1,1,1,1,1,1,1,
1,1,1,1,1,1,1,6),(2,2),(-1.,-0.999000000000001,-0.998000000000001,-0.997000000000001,
-0.996000000000001,-0.995000000000001,-0.994000000000001,-0.993000000000001,
-0.992000000000001,-0.991000000000001,-0.990000000000001,-0.989000000000001,
-0.988000000000001,-0.987000000000001,-0.986000000000001,-0.985000000000001,
-0.984000000000001,-0.983000000000001,-0.982000000000001,-0.981000000000001,
-0.980000000000001,-0.979000000000001,-0.978000000000001,-0.977000000000001,
-0.976000000000001,-0.975000000000001,-0.974000000000001,-0.973000000000001,
-0.972000000000001,-0.971000000000001,-0.970000000000001,-0.969000000000001,
-0.968000000000001,-0.967000000000001,-0.966000000000001,-0.965000000000001,
-0.964000000000001,-0.963000000000001,-0.962000000000001,-0.961000000000001,
-0.960000000000001,-0.959000000000001,-0.958000000000001,-0.957000000000001,
-0.956000000000001,-0.955000000000001,-0.954000000000001,-0.953000000000001,
-0.952000000000001,-0.951000000000001,-0.950000000000001,-0.949000000000001,
-0.948000000000001,-0.947000000000001,-0.946000000000001,-0.945000000000001,
-0.944000000000001,-0.943000000000001,-0.942000000000001,-0.941000000000001,
-0.940000000000001,-0.939000000000001,-0.938000000000001,-0.937000000000001,
-0.936000000000001,-0.935000000000001,-0.934000000000001,-0.933000000000001,
-0.932000000000001,-0.931000000000001,-0.930000000000001,-0.929000000000001,
-0.928000000000001,-0.927000000000001,-0.926000000000001,-0.925000000000001,
-0.924000000000001,-0.923000000000001,-0.922000000000001,-0.921000000000001,
-0.920000000000001,-0.919000000000001,-0.918000000000001,-0.917000000000001,
-0.916000000000001,-0.915000000000001,-0.914000000000001,-0.913000000000001,
-0.912000000000001,-0.911000000000001,-0.910000000000001,-0.909000000000001,
-0.908000000000001,-0.907000000000001,-0.906000000000001,-0.905000000000001,
-0.904000000000001,-0.903000000000001,-0.902000000000001,-0.901000000000001,
-0.900000000000001,-0.899000000000001,-0.898000000000001,-0.897000000000001,
-0.896000000000001,-0.895000000000001,-0.894000000000001,-0.893000000000001,
-0.892000000000001,-0.891000000000001,-0.890000000000001,-0.889000000000001,
-0.888000000000001,-0.887000000000001,-0.886000000000001,-0.885000000000001,
-0.884000000000001,-0.883000000000001,-0.882000000000001,-0.881000000000001,
-0.880000000000001,-0.879000000000001,-0.878000000000001,-0.877000000000001,
-0.876000000000001,-0.875000000000001,-0.874000000000001,-0.873000000000001,
-0.872000000000001,-0.871000000000001,-0.870000000000001,-0.869000000000001,
-0.868000000000001,-0.867000000000001,-0.866000000000001,-0.865000000000001,
-0.864000000000001,-0.863000000000001,-0.862000000000001,-0.861000000000001,
-0.860000000000001,-0.859000000000001,-0.858000000000001,-0.857000000000001,
-0.856000000000001,-0.855000000000001,-0.854000000000001,-0.853000000000001,
-0.852000000000001,-0.851000000000001,-0.850000000000001,-0.849000000000001,
-0.848000000000001,-0.847000000000001,-0.846000000000001,-0.845000000000001,
-0.844000000000001,-0.843000000000001,-0.842000000000001,-0.841000000000001,
-0.840000000000001,-0.839000000000001,-0.838000000000001,-0.837000000000001,
-0.836000000000001,-0.835000000000001,-0.834000000000001,-0.833000000000001,
-0.832000000000001,-0.831000000000001,-0.830000000000001,-0.829000000000001,
-0.828000000000001,-0.827000000000001,-0.826000000000001,-0.825000000000001,
-0.824000000000001,-0.823000000000001,-0.822000000000001,-0.821000000000001,
-0.820000000000001,-0.819000000000001,-0.818000000000001,-0.817000000000001,
-0.816000000000001,-0.815000000000001,-0.814000000000001,-0.813000000000001,
-0.812000000000001,-0.811000000000001,-0.810000000000001,-0.809000000000001,
-0.808000000000001,-0.807000000000001,-0.806000000000001,-0.805000000000001,
-0.804000000000001,-0.803000000000001,-0.802000000000001,-0.801000000000001,
-0.800000000000001,-0.799000000000001,-0.798000000000001,-0.797000000000001,
-0.796000000000001,-0.795000000000001,-0.794000000000001,-0.793000000000001,
-0.792000000000001,-0.791000000000001,-0.790000000000001,-0.789000000000001,
-0.788000000000001,-0.787000000000001,-0.786000000000001,-0.785000000000001,
-0.784000000000001,-0.783000000000001,-0.782000000000001,-0.781000000000001,
-0.780000000000001,-0.779000000000001,-0.778000000000001,-0.777000000000001,
-0.776000000000001,-0.775000000000001,-0.774000000000001,-0.773000000000001,
-0.772000000000001,-0.771000000000001,-0.770000000000001,-0.769000000000001,
-0.768000000000001,-0.767000000000001,-0.766000000000001,-0.765000000000001,
-0.764000000000001,-0.763000000000001,-0.762000000000001,-0.761000000000001,
-0.760000000000001,-0.759000000000001,-0.758000000000001,-0.757000000000001,
-0.756000000000001,-0.755000000000001,-0.754000000000001,-0.753000000000001,
-0.752000000000001,-0.751000000000001,-0.750000000000001,-0.749000000000001,
-0.748000000000001,-0.747000000000001,-0.746000000000001,-0.745000000000001,
-0.744000000000001,-0.743000000000001,-0.742000000000001,-0.741000000000001,
-0.740000000000001,-0.739000000000001,-0.738000000000001,-0.737000000000001,
-0.736000000000001,-0.735000000000001,-0.734000000000001,-0.733000000000001,
-0.732000000000001,-0.731000000000001,-0.730000000000001,-0.729000000000001,
-0.728000000000001,-0.727000000000001,-0.726000000000001,-0.725000000000001,
-0.724000000000001,-0.723000000000001,-0.722000000000001,-0.721000000000001,
-0.720000000000001,-0.719000000000001,-0.718000000000001,-0.717000000000001,
-0.716000000000001,-0.715000000000001,-0.714000000000001,-0.713000000000001,
-0.712000000000001,-0.711000000000001,-0.710000000000001,-0.709000000000001,
-0.708000000000001,-0.707000000000001,-0.706000000000001,-0.705000000000001,
-0.704000000000001,-0.703000000000001,-0.702000000000001,-0.701000000000001,
-0.700000000000001,-0.699000000000001,-0.698000000000001,-0.697000000000001,
-0.696000000000001,-0.695000000000001,-0.694000000000001,-0.693000000000001,
-0.692000000000001,-0.691000000000001,-0.690000000000001,-0.689000000000001,
-0.688000000000001,-0.687,-0.686,-0.685,-0.684,-0.683,-0.682,-0.681,-0.68,
-0.679,-0.678,-0.677,-0.676,-0.675,-0.674,-0.673,-0.672,-0.671,-0.67,-0.669,
-0.668,-0.667,-0.666,-0.665,-0.664,-0.663,-0.662,-0.661,-0.66,-0.659,-0.658,
-0.657,-0.656,-0.655,-0.654,-0.653,-0.652,-0.651,-0.65,-0.649,-0.648,-0.647,
-0.646,-0.645,-0.644,-0.643,-0.642,-0.641,-0.64,-0.639,-0.638,-0.637,-0.636,
-0.635,-0.634,-0.633,-0.632,-0.631,-0.63,-0.629,-0.628,-0.627,-0.626,-0.625,
-0.624,-0.623,-0.622,-0.621,-0.62,-0.619,-0.618,-0.617,-0.616,-0.615,-0.614,
-0.613,-0.612,-0.611,-0.61,-0.609,-0.608,-0.607,-0.606,-0.605,-0.604,-0.603,
-0.602,-0.601,-0.6,-0.599,-0.598,-0.597,-0.596,-0.595,-0.594,-0.593,-0.592,
-0.591,-0.59,-0.589,-0.588,-0.587,-0.586,-0.585,-0.584,-0.583,-0.582,-0.581,
-0.58,-0.579,-0.578,-0.577,-0.576,-0.575,-0.574,-0.573,-0.572,-0.571,-0.57,
-0.569,-0.568,-0.567,-0.566,-0.565,-0.564,-0.563,-0.562,-0.561,-0.56,-0.559,
-0.558,-0.557,-0.556,-0.555,-0.554,-0.553,-0.552,-0.551,-0.55,-0.549,-0.548,
-0.547,-0.546,-0.545,-0.544,-0.543,-0.542,-0.541,-0.54,-0.539,-0.538,-0.537,
-0.536,-0.535,-0.534,-0.533,-0.532,-0.531,-0.53,-0.529,-0.528,-0.527,-0.526,
-0.525,-0.524,-0.523,-0.522,-0.521,-0.52,-0.519,-0.518,-0.517,-0.516,-0.515,
-0.514,-0.513,-0.512,-0.511,-0.51,-0.509,-0.508,-0.507,-0.506,-0.505,-0.504,
-0.503,-0.502,-0.501,-0.5,-0.499,-0.498,-0.497,-0.496,-0.495,-0.494,-0.493,
-0.492,-0.491,-0.49,-0.489,-0.488,-0.487,-0.486,-0.485,-0.484,-0.483,-0.482,
-0.481,-0.48,-0.479,-0.478,-0.477,-0.476,-0.475,-0.474,-0.473,-0.472,-0.471,
-0.47,-0.469,-0.468,-0.467,-0.466,-0.465,-0.464,-0.463,-0.462,-0.461,-0.46,
-0.459,-0.458,-0.457,-0.456,-0.455,-0.454,-0.453,-0.452,-0.451,-0.45,-0.449,
-0.448,-0.447,-0.446,-0.445,-0.444,-0.443,-0.442,-0.441,-0.44,-0.439,-0.438,
-0.437,-0.436,-0.435,-0.434,-0.433,-0.432,-0.431,-0.43,-0.429,-0.428,-0.427,
-0.426,-0.425,-0.424,-0.423,-0.422,-0.421,-0.42,-0.419,-0.418,-0.417,-0.416,
-0.415,-0.414,-0.413,-0.412,-0.411,-0.41,-0.409,-0.408,-0.407,-0.406,-0.405,
-0.404,-0.403,-0.402,-0.401,-0.4,-0.399,-0.398,-0.397,-0.396,-0.395,-0.394,
-0.393,-0.392,-0.391,-0.39,-0.389,-0.388,-0.387,-0.386,-0.385,-0.384,-0.383,
-0.382,-0.381,-0.38,-0.379,-0.378,-0.377,-0.376,-0.375,-0.374,-0.373,-0.372,
-0.371,-0.37,-0.369,-0.368,-0.367,-0.366,-0.365,-0.364,-0.363,-0.362,-0.361,
-0.36,-0.359,-0.358,-0.357,-0.356,-0.355,-0.354,-0.353,-0.352,-0.351,-0.35,
-0.349,-0.348,-0.347,-0.346,-0.345,-0.344,-0.343,-0.342,-0.341,-0.34,-0.339,
-0.338,-0.337,-0.336,-0.335,-0.334,-0.333,-0.332,-0.331,-0.33,-0.329,-0.328,
-0.327,-0.326,-0.325,-0.324,-0.323,-0.322,-0.321,-0.32,-0.319,-0.318,-0.317,
-0.316,-0.315,-0.314,-0.313,-0.312,-0.311,-0.31,-0.309,-0.308,-0.307,-0.306,
-0.305,-0.304,-0.303,-0.302,-0.301,-0.3,-0.299,-0.298,-0.297,-0.296,-0.295,
-0.294,-0.293,-0.292,-0.291,-0.29,-0.289,-0.288,-0.287,-0.286,-0.285,-0.284,
-0.283,-0.282,-0.281,-0.28,-0.279,-0.278,-0.277,-0.276,-0.275,-0.274,-0.273,
-0.272,-0.271,-0.27,-0.269,-0.268,-0.267,-0.266,-0.265,-0.264,-0.263,-0.262,
-0.261,-0.26,-0.259,-0.258,-0.257,-0.256,-0.255,-0.254,-0.253,-0.252,-0.251,
-0.25,-0.249,-0.248,-0.247,-0.246,-0.245,-0.244,-0.243,-0.242,-0.241,-0.24,
-0.239,-0.238,-0.237,-0.236,-0.235,-0.234,-0.233,-0.232,-0.231,-0.23,-0.229,
-0.228,-0.227,-0.226,-0.225,-0.224,-0.223,-0.222,-0.221,-0.22,-0.219,-0.218,
-0.217,-0.216,-0.215,-0.214,-0.213,-0.212,-0.211,-0.21,-0.209,-0.208,-0.207,
-0.206,-0.205,-0.204,-0.203,-0.202,-0.201,-0.2,-0.199,-0.198,-0.197,-0.196,
-0.195,-0.194,-0.193,-0.192,-0.191,-0.19,-0.189,-0.188,-0.187,-0.186,-0.185,
-0.184,-0.183,-0.182,-0.181,-0.18,-0.179,-0.178,-0.177,-0.176,-0.175,-0.174,
-0.173,-0.172,-0.171,-0.17,-0.169,-0.168,-0.167,-0.166,-0.165,-0.164,-0.163,
-0.162,-0.161,-0.16,-0.159,-0.158,-0.157,-0.156,-0.155,-0.154,-0.153,-0.152,
-0.151,-0.15,-0.149,-0.148,-0.147,-0.146,-0.145,-0.144,-0.143,-0.142,-0.141,
-0.14,-0.139,-0.138,-0.137,-0.136,-0.135,-0.134,-0.133,-0.132,-0.131,-0.13,
-0.129,-0.128,-0.127,-0.126,-0.125,-0.124,-0.123,-0.122,-0.121,-0.12,-0.119,
-0.118,-0.117,-0.116,-0.115,-0.114,-0.113,-0.112,-0.111,-0.11,-0.109,-0.108,
-0.107,-0.106,-0.105,-0.104,-0.103,-0.102,-0.101,-0.1,-0.0990000000000001,
-0.0980000000000001,-0.0970000000000001,-0.0960000000000001,-0.0950000000000001,
-0.0940000000000001,-0.0930000000000001,-0.0920000000000001,-0.0910000000000001,
-0.0900000000000001,-0.0890000000000001,-0.0880000000000001,-0.0870000000000001,
-0.0860000000000001,-0.0850000000000001,-0.0840000000000001,-0.0830000000000001,
-0.0820000000000001,-0.0810000000000001,-0.0800000000000001,-0.0790000000000001,
-0.0780000000000001,-0.0770000000000001,-0.0760000000000001,-0.0750000000000001,
-0.0740000000000001,-0.0730000000000001,-0.0720000000000001,-0.071,-0.07,
-0.069,-0.068,-0.067,-0.066,-0.065,-0.064,-0.063,-0.062,-0.061,-0.06,-0.059,
-0.058,-0.057,-0.056,-0.055,-0.054,-0.053,-0.052,-0.051,-0.05,-0.049,-0.048,
-0.047,-0.046,-0.045,-0.044,-0.043,-0.042,-0.041,-0.04,-0.039,-0.038,-0.037,
-0.036,-0.035,-0.034,-0.033,-0.032,-0.031,-0.03,-0.029,-0.028,-0.027,-0.026,
-0.025,-0.024,-0.023,-0.022,-0.021,-0.02,-0.019,-0.018,-0.017,-0.016,-0.015,
-0.014,-0.013,-0.012,-0.011,-0.01,-0.009,-0.008,-0.007,-0.006,-0.005,-0.004,
-0.003,-0.002,-0.001,0.),(0.,2.),.UNSPECIFIED.)
GEOMETRIC_REPRESENTATION_ITEM()
RATIONAL_B_SPLINE_SURFACE(((1.,1.),(1.,1.),(1.,1.),(1.,1.),(1.,1.),(1.,
1.),(1.,1.),(1.,1.),(1.,1.),(1.,1.),(1.,1.),(1.,1.),(1.,1.),(1.,1.),(1.,
1.),(1.,1.),(1.,1.),(1.,1.),(1.,1.),(1.,1.),(1.,1.),(1.,1.),(1.,1.),(1.,
1.),(1.,1.),(1.,1.),(1.,1.),(1.,1.),(1.,1.),(1.,1.),(1.,1.),(1.,1.),(1.,
1.),(1.,1.),(1.,1.),(1.,1.),(1.,1.),(1.,1.),(1.,1.),(1.,1.),(1.,1.),(1.,
1.),(1.,1.),(1.,1.),(1.,1.),(1.,1.),(1.,1.),(1.,1.),(1.,1.),(1.,1.),(1.,
1.),(1.,1.),(1.,1.),(1.,1.),(1.,1.),(1.,1.),(1.,1.),(1.,1.),(1.,1.),(1.,
1.),(1.,1.),(1.,1.),(1.,1.),(1.,1.),(1.,1.),(1.,1.),(1.,1.),(1.,1.),(1.,
1.),(1.,1.),(1.,1.),(1.,1.),(1.,1.),(1.,1.),(1.,1.),(1.,1.),(1.,1.),(1.,
1.),(1.,1.),(1.,1.),(1.,1.),(1.,1.),(1.,1.),(1.,1.),(1.,1.),(1.,1.),(1.,
1.),(1.,1.),(1.,1.),(1.,1.),(1.,1.),(1.,1.),(1.,1.),(1.,1.),(1.,1.),(1.,
1.),(1.,1.),(1.,1.),(1.,1.),(1.,1.),(1.,1.),(1.,1.),(1.,1.),(1.,1.),(1.,
1.),(1.,1.),(1.,1.),(1.,1.),(1.,1.),(1.,1.),(1.,1.),(1.,1.),(1.,1.),(1.,
1.),(1.,1.),(1.,1.),(1.,1.),(1.,1.),(1.,1.),(1.,1.),(1.,1.),(1.,1.),(1.,
1.),(1.,1.),(1.,1.),(1.,1.),(1.,1.),(1.,1.),(1.,1.),(1.,1.),(1.,1.),(1.,
1.),(1.,1.),(1.,1.),(1.,1.),(1.,1.),(1.,1.),(1.,1.),(1.,1.),(1.,1.),(1.,
1.),(1.,1.),(1.,1.),(1.,1.),(1.,1.),(1.,1.),(1.,1.),(1.,1.),(1.,1.),(1.,
1.),(1.,1.),(1.,1.),(1.,1.),(1.,1.),(1.,1.),(1.,1.),(1.,1.),(1.,1.),(1.,
1.),(1.,1.),(1.,1.),(1.,1.),(1.,1.),(1.,1.),(1.,1.),(1.,1.),(1.,1.),(1.,
1.),(1.,1.),(1.,1.),(1.,1.),(1.,1.),(1.,1.),(1.,1.),(1.,1.),(1.,1.),(1.,
1.),(1.,1.),(1.,1.),(1.,1.),(1.,1.),(1.,1.),(1.,1.),(1.,1.),(1.,1.),(1.,
1.),(1.,1.),(1.,1.),(1.,1.),(1.,1.),(1.,1.),(1.,1.),(1.,1.),(1.,1.),(1.,
1.),(1.,1.),(1.,1.),(1.,1.),(1.,1.),(1.,1.),(1.,1.),(1.,1.),(1.,1.),(1.,
1.),(1.,1.),(1.,1.),(1.,1.),(1.,1.),(1.,1.),(1.,1.),(1.,1.),(1.,1.),(1.,
1.),(1.,1.),(1.,1.),(1.,1.),(1.,1.),(1.,1.),(1.,1.),(1.,1.),(1.,1.),(1.,
1.),(1.,1.),(1.,1.),(1.,1.),(1.,1.),(1.,1.),(1.,1.),(1.,1.),(1.,1.),(1.,
1.),(1.,1.),(1.,1.),(1.,1.),(1.,1.),(1.,1.),(1.,1.),(1.,1.),(1.,1.),(1.,
1.),(1.,1.),(1.,1.),(1.,1.),(1.,1.),(1.,1.),(1.,1.),(1.,1.),(1.,1.),(1.,
1.),(1.,1.),(1.,1.),(1.,1.),(1.,1.),(1.,1.),(1.,1.),(1.,1.),(1.,1.),(1.,
1.),(1.,1.),(1.,1.),(1.,1.),(1.,1.),(1.,1.),(1.,1.),(1.,1.),(1.,1.),(1.,
1.),(1.,1.),(1.,1.),(1.,1.),(1.,1.),(1.,1.),(1.,1.),(1.,1.),(1.,1.),(1.,
1.),(1.,1.),(1.,1.),(1.,1.),(1.,1.),(1.,1.),(1.,1.),(1.,1.),(1.,1.),(1.,
1.),(1.,1.),(1.,1.),(1.,1.),(1.,1.),(1.,1.),(1.,1.),(1.,1.),(1.,1.),(1.,
1.),(1.,1.),(1.,1.),(1.,1.),(1.,1.),(1.,1.),(1.,1.),(1.,1.),(1.,1.),(1.,
1.),(1.,1.),(1.,1.),(1.,1.),(1.,1.),(1.,1.),(1.,1.),(1.,1.),(1.,1.),(1.,
1.),(1.,1.),(1.,1.),(1.,1.),(1.,1.),(1.,1.),(1.,1.),(1.,1.),(1.,1.),(1.,
1.),(1.,1.),(1.,1.),(1.,1.),(1.,1.),(1.,1.),(1.,1.),(1.,1.),(1.,1.),(1.,
1.),(1.,1.),(1.,1.),(1.,1.),(1.,1.),(1.,1.),(1.,1.),(1.,1.),(1.,1.),(1.,
1.),(1.,1.),(1.,1.),(1.,1.),(1.,1.),(1.,1.),(1.,1.),(1.,1.),(1.,1.),(1.,
1.),(1.,1.),(1.,1.),(1.,1.),(1.,1.),(1.,1.),(1.,1.),(1.,1.),(1.,1.),(1.,
1.),(1.,1.),(1.,1.),(1.,1.),(1.,1.),(1.,1.),(1.,1.),(1.,1.),(1.,1.),(1.,
1.),(1.,1.),(1.,1.),(1.,1.),(1.,1.),(1.,1.),(1.,1.),(1.,1.),(1.,1.),(1.,
1.),(1.,1.),(1.,1.),(1.,1.),(1.,1.),(1.,1.),(1.,1.),(1.,1.),(1.,1.),(1.,
1.),(1.,1.),(1.,1.),(1.,1.),(1.,1.),(1.,1.),(1.,1.),(1.,1.),(1.,1.),(1.,
1.),(1.,1.),(1.,1.),(1.,1.),(1.,1.),(1.,1.),(1.,1.),(1.,1.),(1.,1.),(1.,
1.),(1.,1.),(1.,1.),(1.,1.),(1.,1.),(1.,1.),(1.,1.),(1.,1.),(1.,1.),(1.,
1.),(1.,1.),(1.,1.),(1.,1.),(1.,1.),(1.,1.),(1.,1.),(1.,1.),(1.,1.),(1.,
1.),(1.,1.),(1.,1.),(1.,1.),(1.,1.),(1.,1.),(1.,1.),(1.,1.),(1.,1.),(1.,
1.),(1.,1.),(1.,1.),(1.,1.),(1.,1.),(1.,1.),(1.,1.),(1.,1.),(1.,1.),(1.,
1.),(1.,1.),(1.,1.),(1.,1.),(1.,1.),(1.,1.),(1.,1.),(1.,1.),(1.,1.),(1.,
1.),(1.,1.),(1.,1.),(1.,1.),(1.,1.),(1.,1.),(1.,1.),(1.,1.),(1.,1.),(1.,
1.),(1.,1.),(1.,1.),(1.,1.),(1.,1.),(1.,1.),(1.,1.),(1.,1.),(1.,1.),(1.,
1.),(1.,1.),(1.,1.),(1.,1.),(1.,1.),(1.,1.),(1.,1.),(1.,1.),(1.,1.),(1.,
1.),(1.,1.),(1.,1.),(1.,1.),(1.,1.),(1.,1.),(1.,1.),(1.,1.),(1.,1.),(1.,
1.),(1.,1.),(1.,1.),(1.,1.),(1.,1.),(1.,1.),(1.,1.),(1.,1.),(1.,1.),(1.,
1.),(1.,1.),(1.,1.),(1.,1.),(1.,1.),(1.,1.),(1.,1.),(1.,1.),(1.,1.),(1.,
1.),(1.,1.),(1.,1.),(1.,1.),(1.,1.),(1.,1.),(1.,1.),(1.,1.),(1.,1.),(1.,
1.),(1.,1.),(1.,1.),(1.,1.),(1.,1.),(1.,1.),(1.,1.),(1.,1.),(1.,1.),(1.,
1.),(1.,1.),(1.,1.),(1.,1.),(1.,1.),(1.,1.),(1.,1.),(1.,1.),(1.,1.),(1.,
1.),(1.,1.),(1.,1.),(1.,1.),(1.,1.),(1.,1.),(1.,1.),(1.,1.),(1.,1.),(1.,
1.),(1.,1.),(1.,1.),(1.,1.),(1.,1.),(1.,1.),(1.,1.),(1.,1.),(1.,1.),(1.,
1.),(1.,1.),(1.,1.),(1.,1.),(1.,1.),(1.,1.),(1.,1.),(1.,1.),(1.,1.),(1.,
1.),(1.,1.),(1.,1.),(1.,1.),(1.,1.),(1.,1.),(1.,1.),(1.,1.),(1.,1.),(1.,
1.),(1.,1.),(1.,1.),(1.,1.),(1.,1.),(1.,1.),(1.,1.),(1.,1.),(1.,1.),(1.,
1.),(1.,1.),(1.,1.),(1.,1.),(1.,1.),(1.,1.),(1.,1.),(1.,1.),(1.,1.),(1.,
1.),(1.,1.),(1.,1.),(1.,1.),(1.,1.),(1.,1.),(1.,1.),(1.,1.),(1.,1.),(1.,
1.),(1.,1.),(1.,1.),(1.,1.),(1.,1.),(1.,1.),(1.,1.),(1.,1.),(1.,1.),(1.,
1.),(1.,1.),(1.,1.),(1.,1.),(1.,1.),(1.,1.),(1.,1.),(1.,1.),(1.,1.),(1.,
1.),(1.,1.),(1.,1.),(1.,1.),(1.,1.),(1.,1.),(1.,1.),(1.,1.),(1.,1.),(1.,
1.),(1.,1.),(1.,1.),(1.,1.),(1.,1.),(1.,1.),(1.,1.),(1.,1.),(1.,1.),(1.,
1.),(1.,1.),(1.,1.),(1.,1.),(1.,1.),(1.,1.),(1.,1.),(1.,1.),(1.,1.),(1.,
1.),(1.,1.),(1.,1.),(1.,1.),(1.,1.),(1.,1.),(1.,1.),(1.,1.),(1.,1.),(1.,
1.),(1.,1.),(1.,1.),(1.,1.),(1.,1.),(1.,1.),(1.,1.),(1.,1.),(1.,1.),(1.,
1.),(1.,1.),(1.,1.),(1.,1.),(1.,1.),(1.,1.),(1.,1.),(1.,1.),(1.,1.),(1.,
1.),(1.,1.),(1.,1.),(1.,1.),(1.,1.),(1.,1.),(1.,1.),(1.,1.),(1.,1.),(1.,
1.),(1.,1.),(1.,1.),(1.,1.),(1.,1.),(1.,1.),(1.,1.),(1.,1.),(1.,1.),(1.,
1.),(1.,1.),(1.,1.),(1.,1.),(1.,1.),(1.,1.),(1.,1.),(1.,1.),(1.,1.),(1.,
1.),(1.,1.),(1.,1.),(1.,1.),(1.,1.),(1.,1.),(1.,1.),(1.,1.),(1.,1.),(1.,
1.),(1.,1.),(1.,1.),(1.,1.),(1.,1.),(1.,1.),(1.,1.),(1.,1.),(1.,1.),(1.,
1.),(1.,1.),(1.,1.),(1.,1.),(1.,1.),(1.,1.),(1.,1.),(1.,1.),(1.,1.),(1.,
1.),(1.,1.),(1.,1.),(1.,1.),(1.,1.),(1.,1.),(1.,1.),(1.,1.),(1.,1.),(1.,
1.),(1.,1.),(1.,1.),(1.,1.),(1.,1.),(1.,1.),(1.,1.),(1.,1.),(1.,1.),(1.,
1.),(1.,1.),(1.,1.),(1.,1.),(1.,1.),(1.,1.),(1.,1.),(1.,1.),(1.,1.),(1.,
1.),(1.,1.),(1.,1.),(1.,1.),(1.,1.),(1.,1.),(1.,1.),(1.,1.),(1.,1.),(1.,
1.),(1.,1.),(1.,1.),(1.,1.),(1.,1.),(1.,1.),(1.,1.),(1.,1.),(1.,1.),(1.,
1.),(1.,1.),(1.,1.),(1.,1.),(1.,1.),(1.,1.),(1.,1.),(1.,1.),(1.,1.),(1.,
1.),(1.,1.),(1.,1.),(1.,1.),(1.,1.),(1.,1.),(1.,1.),(1.,1.),(1.,1.),(1.,
1.),(1.,1.),(1.,1.),(1.,1.),(1.,1.),(1.,1.),(1.,1.),(1.,1.),(1.,1.),(1.,
1.),(1.,1.),(1.,1.),(1.,1.),(1.,1.),(1.,1.),(1.,1.),(1.,1.),(1.,1.),(1.,
1.),(1.,1.),(1.,1.),(1.,1.),(1.,1.),(1.,1.),(1.,1.),(1.,1.),(1.,1.),(1.,
1.),(1.,1.),(1.,1.),(1.,1.),(1.,1.),(1.,1.),(1.,1.),(1.,1.),(1.,1.),(1.,
1.),(1.,1.),(1.,1.),(1.,1.),(1.,1.),(1.,1.),(1.,1.),(1.,1.),(1.,1.),(1.,
1.),(1.,1.),(1.,1.),(1.,1.),(1.,1.),(1.,1.),(1.,1.),(1.,1.),(1.,1.),(1.,
1.),(1.,1.),(1.,1.),(1.,1.),(1.,1.),(1.,1.),(1.,1.),(1.,1.),(1.,1.),(1.,
1.),(1.,1.),(1.,1.),(1.,1.),(1.,1.),(1.,1.),(1.,1.),(1.,1.),(1.,1.),(1.,
1.),(1.,1.),(1.,1.),(1.,1.),(1.,1.),(1.,1.),(1.,1.),(1.,1.),(1.,1.),(1.,
1.),(1.,1.),(1.,1.),(1.,1.),(1.,1.),(1.,1.),(1.,1.),(1.,1.),(1.,1.),(1.,
1.),(1.,1.),(1.,1.),(1.,1.),(1.,1.),(1.,1.),(1.,1.),(1.,1.),(1.,1.),(1.,
1.),(1.,1.),(1.,1.),(1.,1.),(1.,1.),(1.,1.),(1.,1.),(1.,1.),(1.,1.),(1.,
1.),(1.,1.),(1.,1.),(1.,1.),(1.,1.),(1.,1.),(1.,1.),(1.,1.),(1.,1.),(1.,
1.),(1.,1.),(1.,1.),(1.,1.),(1.,1.),(1.,1.),(1.,1.),(1.,1.),(1.,1.),(1.,
1.),(1.,1.),(1.,1.),(1.,1.),(1.,1.),(1.,1.),(1.,1.),(1.,1.),(1.,1.),(1.,
1.),(1.,1.),(1.,1.),(1.,1.),(1.,1.),(1.,1.),(1.,1.),(1.,1.),(1.,1.),(1.,
1.),(1.,1.),(1.,1.),(1.,1.),(1.,1.),(1.,1.),(1.,1.),(1.,1.),(1.,1.),(1.,
1.),(1.,1.),(1.,1.),(1.,1.),(1.,1.),(1.,1.),(1.,1.),(1.,1.),(1.,1.),(1.,
1.),(1.,1.),(1.,1.),(1.,1.),(1.,1.),(1.,1.),(1.,1.),(1.,1.),(1.,1.),(1.,
1.),(1.,1.),(1.,1.),(1.,1.),(1.,1.),(1.,1.),(1.,1.),(1.,1.),(1.,1.),(1.,
1.),(1.,1.),(1.,1.),(1.,1.),(1.,1.),(1.,1.),(1.,1.),(1.,1.),(1.,1.),(1.,
1.),(1.,1.),(1.,1.),(1.,1.),(1.,1.),(1.,1.),(1.,1.),(1.,1.),(1.,1.),(1.,
1.),(1.,1.),(1.,1.),(1.,1.),(1.,1.),(1.,1.),(1.,1.),(1.,1.),(1.,1.),(1.,
1.),(1.,1.),(1.,1.),(1.,1.),(1.,1.),(1.,1.),(1.,1.),(1.,1.),(1.,1.),(1.,
1.),(1.,1.),(1.,1.),(1.,1.),(1.,1.),(1.,1.),(1.,1.),(1.,1.),(1.,1.),(1.,
1.)))
REPRESENTATION_ITEM('')
SURFACE()
);
#266=(
BOUNDED_SURFACE()
B_SPLINE_SURFACE(5,1,((#90421,#90422),(#90423,#90424),(#90425,#90426),(#90427,
#90428),(#90429,#90430),(#90431,#90432),(#90433,#90434),(#90435,#90436),
(#90437,#90438),(#90439,#90440),(#90441,#90442),(#90443,#90444),(#90445,
#90446),(#90447,#90448),(#90449,#90450),(#90451,#90452),(#90453,#90454),
(#90455,#90456),(#90457,#90458),(#90459,#90460),(#90461,#90462),(#90463,
#90464),(#90465,#90466),(#90467,#90468),(#90469,#90470),(#90471,#90472),
(#90473,#90474),(#90475,#90476),(#90477,#90478),(#90479,#90480),(#90481,
#90482),(#90483,#90484),(#90485,#90486),(#90487,#90488),(#90489,#90490),
(#90491,#90492),(#90493,#90494),(#90495,#90496),(#90497,#90498),(#90499,
#90500),(#90501,#90502),(#90503,#90504),(#90505,#90506),(#90507,#90508),
(#90509,#90510),(#90511,#90512),(#90513,#90514),(#90515,#90516),(#90517,
#90518),(#90519,#90520),(#90521,#90522),(#90523,#90524),(#90525,#90526),
(#90527,#90528),(#90529,#90530),(#90531,#90532),(#90533,#90534),(#90535,
#90536),(#90537,#90538),(#90539,#90540),(#90541,#90542),(#90543,#90544),
(#90545,#90546),(#90547,#90548),(#90549,#90550),(#90551,#90552),(#90553,
#90554),(#90555,#90556),(#90557,#90558),(#90559,#90560),(#90561,#90562),
(#90563,#90564),(#90565,#90566),(#90567,#90568),(#90569,#90570),(#90571,
#90572),(#90573,#90574),(#90575,#90576),(#90577,#90578),(#90579,#90580),
(#90581,#90582),(#90583,#90584),(#90585,#90586),(#90587,#90588),(#90589,
#90590),(#90591,#90592),(#90593,#90594),(#90595,#90596),(#90597,#90598),
(#90599,#90600),(#90601,#90602),(#90603,#90604),(#90605,#90606),(#90607,
#90608),(#90609,#90610),(#90611,#90612),(#90613,#90614),(#90615,#90616),
(#90617,#90618),(#90619,#90620),(#90621,#90622),(#90623,#90624),(#90625,
#90626),(#90627,#90628),(#90629,#90630),(#90631,#90632),(#90633,#90634),
(#90635,#90636),(#90637,#90638),(#90639,#90640),(#90641,#90642),(#90643,
#90644),(#90645,#90646),(#90647,#90648),(#90649,#90650),(#90651,#90652),
(#90653,#90654),(#90655,#90656),(#90657,#90658),(#90659,#90660),(#90661,
#90662),(#90663,#90664),(#90665,#90666),(#90667,#90668),(#90669,#90670),
(#90671,#90672),(#90673,#90674),(#90675,#90676),(#90677,#90678),(#90679,
#90680),(#90681,#90682),(#90683,#90684),(#90685,#90686),(#90687,#90688),
(#90689,#90690),(#90691,#90692),(#90693,#90694),(#90695,#90696),(#90697,
#90698),(#90699,#90700),(#90701,#90702),(#90703,#90704),(#90705,#90706),
(#90707,#90708),(#90709,#90710),(#90711,#90712),(#90713,#90714),(#90715,
#90716),(#90717,#90718),(#90719,#90720),(#90721,#90722),(#90723,#90724),
(#90725,#90726),(#90727,#90728),(#90729,#90730),(#90731,#90732),(#90733,
#90734),(#90735,#90736),(#90737,#90738),(#90739,#90740),(#90741,#90742),
(#90743,#90744),(#90745,#90746),(#90747,#90748),(#90749,#90750),(#90751,
#90752),(#90753,#90754),(#90755,#90756),(#90757,#90758),(#90759,#90760),
(#90761,#90762),(#90763,#90764),(#90765,#90766),(#90767,#90768),(#90769,
#90770),(#90771,#90772),(#90773,#90774),(#90775,#90776),(#90777,#90778),
(#90779,#90780),(#90781,#90782),(#90783,#90784),(#90785,#90786),(#90787,
#90788),(#90789,#90790),(#90791,#90792),(#90793,#90794),(#90795,#90796),
(#90797,#90798),(#90799,#90800),(#90801,#90802),(#90803,#90804),(#90805,
#90806),(#90807,#90808),(#90809,#90810),(#90811,#90812),(#90813,#90814),
(#90815,#90816),(#90817,#90818),(#90819,#90820),(#90821,#90822),(#90823,
#90824),(#90825,#90826),(#90827,#90828),(#90829,#90830),(#90831,#90832),
(#90833,#90834),(#90835,#90836),(#90837,#90838),(#90839,#90840),(#90841,
#90842),(#90843,#90844),(#90845,#90846),(#90847,#90848),(#90849,#90850),
(#90851,#90852),(#90853,#90854),(#90855,#90856),(#90857,#90858),(#90859,
#90860),(#90861,#90862),(#90863,#90864),(#90865,#90866),(#90867,#90868),
(#90869,#90870),(#90871,#90872),(#90873,#90874),(#90875,#90876),(#90877,
#90878),(#90879,#90880),(#90881,#90882),(#90883,#90884),(#90885,#90886),
(#90887,#90888),(#90889,#90890),(#90891,#90892),(#90893,#90894),(#90895,
#90896),(#90897,#90898),(#90899,#90900),(#90901,#90902),(#90903,#90904),
(#90905,#90906),(#90907,#90908),(#90909,#90910),(#90911,#90912),(#90913,
#90914),(#90915,#90916),(#90917,#90918),(#90919,#90920),(#90921,#90922),
(#90923,#90924),(#90925,#90926),(#90927,#90928),(#90929,#90930),(#90931,
#90932),(#90933,#90934),(#90935,#90936),(#90937,#90938),(#90939,#90940),
(#90941,#90942),(#90943,#90944),(#90945,#90946),(#90947,#90948),(#90949,
#90950),(#90951,#90952),(#90953,#90954),(#90955,#90956),(#90957,#90958),
(#90959,#90960),(#90961,#90962),(#90963,#90964),(#90965,#90966),(#90967,
#90968),(#90969,#90970),(#90971,#90972),(#90973,#90974),(#90975,#90976),
(#90977,#90978),(#90979,#90980),(#90981,#90982),(#90983,#90984),(#90985,
#90986),(#90987,#90988),(#90989,#90990),(#90991,#90992),(#90993,#90994),
(#90995,#90996),(#90997,#90998),(#90999,#91000),(#91001,#91002),(#91003,
#91004),(#91005,#91006),(#91007,#91008),(#91009,#91010),(#91011,#91012),
(#91013,#91014),(#91015,#91016),(#91017,#91018),(#91019,#91020),(#91021,
#91022),(#91023,#91024),(#91025,#91026),(#91027,#91028),(#91029,#91030),
(#91031,#91032),(#91033,#91034),(#91035,#91036),(#91037,#91038),(#91039,
#91040),(#91041,#91042),(#91043,#91044),(#91045,#91046),(#91047,#91048),
(#91049,#91050),(#91051,#91052),(#91053,#91054),(#91055,#91056),(#91057,
#91058),(#91059,#91060),(#91061,#91062),(#91063,#91064),(#91065,#91066),
(#91067,#91068),(#91069,#91070),(#91071,#91072),(#91073,#91074),(#91075,
#91076),(#91077,#91078),(#91079,#91080),(#91081,#91082),(#91083,#91084),
(#91085,#91086),(#91087,#91088),(#91089,#91090),(#91091,#91092),(#91093,
#91094),(#91095,#91096),(#91097,#91098),(#91099,#91100),(#91101,#91102),
(#91103,#91104),(#91105,#91106),(#91107,#91108),(#91109,#91110),(#91111,
#91112),(#91113,#91114),(#91115,#91116),(#91117,#91118),(#91119,#91120),
(#91121,#91122),(#91123,#91124),(#91125,#91126),(#91127,#91128),(#91129,
#91130),(#91131,#91132),(#91133,#91134),(#91135,#91136),(#91137,#91138),
(#91139,#91140),(#91141,#91142),(#91143,#91144),(#91145,#91146),(#91147,
#91148),(#91149,#91150),(#91151,#91152),(#91153,#91154),(#91155,#91156),
(#91157,#91158),(#91159,#91160),(#91161,#91162),(#91163,#91164),(#91165,
#91166),(#91167,#91168),(#91169,#91170),(#91171,#91172),(#91173,#91174),
(#91175,#91176),(#91177,#91178),(#91179,#91180),(#91181,#91182),(#91183,
#91184),(#91185,#91186),(#91187,#91188),(#91189,#91190),(#91191,#91192),
(#91193,#91194),(#91195,#91196),(#91197,#91198),(#91199,#91200),(#91201,
#91202),(#91203,#91204),(#91205,#91206),(#91207,#91208),(#91209,#91210),
(#91211,#91212),(#91213,#91214),(#91215,#91216),(#91217,#91218),(#91219,
#91220),(#91221,#91222),(#91223,#91224),(#91225,#91226),(#91227,#91228),
(#91229,#91230),(#91231,#91232),(#91233,#91234),(#91235,#91236),(#91237,
#91238),(#91239,#91240),(#91241,#91242),(#91243,#91244),(#91245,#91246),
(#91247,#91248),(#91249,#91250),(#91251,#91252),(#91253,#91254),(#91255,
#91256),(#91257,#91258),(#91259,#91260),(#91261,#91262),(#91263,#91264),
(#91265,#91266),(#91267,#91268),(#91269,#91270),(#91271,#91272),(#91273,
#91274),(#91275,#91276),(#91277,#91278),(#91279,#91280),(#91281,#91282),
(#91283,#91284),(#91285,#91286),(#91287,#91288),(#91289,#91290),(#91291,
#91292),(#91293,#91294),(#91295,#91296),(#91297,#91298),(#91299,#91300),
(#91301,#91302),(#91303,#91304),(#91305,#91306),(#91307,#91308),(#91309,
#91310),(#91311,#91312),(#91313,#91314),(#91315,#91316),(#91317,#91318),
(#91319,#91320),(#91321,#91322),(#91323,#91324),(#91325,#91326),(#91327,
#91328),(#91329,#91330),(#91331,#91332),(#91333,#91334),(#91335,#91336),
(#91337,#91338),(#91339,#91340),(#91341,#91342),(#91343,#91344),(#91345,
#91346),(#91347,#91348),(#91349,#91350),(#91351,#91352),(#91353,#91354),
(#91355,#91356),(#91357,#91358),(#91359,#91360),(#91361,#91362),(#91363,
#91364),(#91365,#91366),(#91367,#91368),(#91369,#91370),(#91371,#91372),
(#91373,#91374),(#91375,#91376),(#91377,#91378),(#91379,#91380),(#91381,
#91382),(#91383,#91384),(#91385,#91386),(#91387,#91388),(#91389,#91390),
(#91391,#91392),(#91393,#91394),(#91395,#91396),(#91397,#91398),(#91399,
#91400),(#91401,#91402),(#91403,#91404),(#91405,#91406),(#91407,#91408),
(#91409,#91410),(#91411,#91412),(#91413,#91414),(#91415,#91416),(#91417,
#91418),(#91419,#91420),(#91421,#91422),(#91423,#91424),(#91425,#91426),
(#91427,#91428),(#91429,#91430),(#91431,#91432),(#91433,#91434),(#91435,
#91436),(#91437,#91438),(#91439,#91440),(#91441,#91442),(#91443,#91444),
(#91445,#91446),(#91447,#91448),(#91449,#91450),(#91451,#91452),(#91453,
#91454),(#91455,#91456),(#91457,#91458),(#91459,#91460),(#91461,#91462),
(#91463,#91464),(#91465,#91466),(#91467,#91468),(#91469,#91470),(#91471,
#91472),(#91473,#91474),(#91475,#91476),(#91477,#91478),(#91479,#91480),
(#91481,#91482),(#91483,#91484),(#91485,#91486),(#91487,#91488),(#91489,
#91490),(#91491,#91492),(#91493,#91494),(#91495,#91496),(#91497,#91498),
(#91499,#91500),(#91501,#91502),(#91503,#91504),(#91505,#91506),(#91507,
#91508),(#91509,#91510),(#91511,#91512),(#91513,#91514),(#91515,#91516),
(#91517,#91518),(#91519,#91520),(#91521,#91522),(#91523,#91524),(#91525,
#91526),(#91527,#91528),(#91529,#91530),(#91531,#91532),(#91533,#91534),
(#91535,#91536),(#91537,#91538),(#91539,#91540),(#91541,#91542),(#91543,
#91544),(#91545,#91546),(#91547,#91548),(#91549,#91550),(#91551,#91552),
(#91553,#91554),(#91555,#91556),(#91557,#91558),(#91559,#91560),(#91561,
#91562),(#91563,#91564),(#91565,#91566),(#91567,#91568),(#91569,#91570),
(#91571,#91572),(#91573,#91574),(#91575,#91576),(#91577,#91578),(#91579,
#91580),(#91581,#91582),(#91583,#91584),(#91585,#91586),(#91587,#91588),
(#91589,#91590),(#91591,#91592),(#91593,#91594),(#91595,#91596),(#91597,
#91598),(#91599,#91600),(#91601,#91602),(#91603,#91604),(#91605,#91606),
(#91607,#91608),(#91609,#91610),(#91611,#91612),(#91613,#91614),(#91615,
#91616),(#91617,#91618),(#91619,#91620),(#91621,#91622),(#91623,#91624),
(#91625,#91626),(#91627,#91628),(#91629,#91630),(#91631,#91632),(#91633,
#91634),(#91635,#91636),(#91637,#91638),(#91639,#91640),(#91641,#91642),
(#91643,#91644),(#91645,#91646),(#91647,#91648),(#91649,#91650),(#91651,
#91652),(#91653,#91654),(#91655,#91656),(#91657,#91658),(#91659,#91660),
(#91661,#91662),(#91663,#91664),(#91665,#91666),(#91667,#91668),(#91669,
#91670),(#91671,#91672),(#91673,#91674),(#91675,#91676),(#91677,#91678),
(#91679,#91680),(#91681,#91682),(#91683,#91684),(#91685,#91686),(#91687,
#91688),(#91689,#91690),(#91691,#91692),(#91693,#91694),(#91695,#91696),
(#91697,#91698),(#91699,#91700),(#91701,#91702),(#91703,#91704),(#91705,
#91706),(#91707,#91708),(#91709,#91710),(#91711,#91712),(#91713,#91714),
(#91715,#91716),(#91717,#91718),(#91719,#91720),(#91721,#91722),(#91723,
#91724),(#91725,#91726),(#91727,#91728),(#91729,#91730),(#91731,#91732),
(#91733,#91734),(#91735,#91736),(#91737,#91738),(#91739,#91740),(#91741,
#91742),(#91743,#91744),(#91745,#91746),(#91747,#91748),(#91749,#91750),
(#91751,#91752),(#91753,#91754),(#91755,#91756),(#91757,#91758),(#91759,
#91760),(#91761,#91762),(#91763,#91764),(#91765,#91766),(#91767,#91768),
(#91769,#91770),(#91771,#91772),(#91773,#91774),(#91775,#91776),(#91777,
#91778),(#91779,#91780),(#91781,#91782),(#91783,#91784),(#91785,#91786),
(#91787,#91788),(#91789,#91790),(#91791,#91792),(#91793,#91794),(#91795,
#91796),(#91797,#91798),(#91799,#91800),(#91801,#91802),(#91803,#91804),
(#91805,#91806),(#91807,#91808),(#91809,#91810),(#91811,#91812),(#91813,
#91814),(#91815,#91816),(#91817,#91818),(#91819,#91820),(#91821,#91822),
(#91823,#91824),(#91825,#91826),(#91827,#91828),(#91829,#91830),(#91831,
#91832),(#91833,#91834),(#91835,#91836),(#91837,#91838),(#91839,#91840),
(#91841,#91842),(#91843,#91844),(#91845,#91846),(#91847,#91848),(#91849,
#91850),(#91851,#91852),(#91853,#91854),(#91855,#91856),(#91857,#91858),
(#91859,#91860),(#91861,#91862),(#91863,#91864),(#91865,#91866),(#91867,
#91868),(#91869,#91870),(#91871,#91872),(#91873,#91874),(#91875,#91876),
(#91877,#91878),(#91879,#91880),(#91881,#91882),(#91883,#91884),(#91885,
#91886),(#91887,#91888),(#91889,#91890),(#91891,#91892),(#91893,#91894),
(#91895,#91896),(#91897,#91898),(#91899,#91900),(#91901,#91902),(#91903,
#91904),(#91905,#91906),(#91907,#91908),(#91909,#91910),(#91911,#91912),
(#91913,#91914),(#91915,#91916),(#91917,#91918),(#91919,#91920),(#91921,
#91922),(#91923,#91924),(#91925,#91926),(#91927,#91928),(#91929,#91930),
(#91931,#91932),(#91933,#91934),(#91935,#91936),(#91937,#91938),(#91939,
#91940),(#91941,#91942),(#91943,#91944),(#91945,#91946),(#91947,#91948),
(#91949,#91950),(#91951,#91952),(#91953,#91954),(#91955,#91956),(#91957,
#91958),(#91959,#91960),(#91961,#91962),(#91963,#91964),(#91965,#91966),
(#91967,#91968),(#91969,#91970),(#91971,#91972),(#91973,#91974),(#91975,
#91976),(#91977,#91978),(#91979,#91980),(#91981,#91982),(#91983,#91984),
(#91985,#91986),(#91987,#91988),(#91989,#91990),(#91991,#91992),(#91993,
#91994),(#91995,#91996),(#91997,#91998),(#91999,#92000),(#92001,#92002),
(#92003,#92004),(#92005,#92006),(#92007,#92008),(#92009,#92010),(#92011,
#92012),(#92013,#92014),(#92015,#92016),(#92017,#92018),(#92019,#92020),
(#92021,#92022),(#92023,#92024),(#92025,#92026),(#92027,#92028),(#92029,
#92030),(#92031,#92032),(#92033,#92034),(#92035,#92036),(#92037,#92038),
(#92039,#92040),(#92041,#92042),(#92043,#92044),(#92045,#92046),(#92047,
#92048),(#92049,#92050),(#92051,#92052),(#92053,#92054),(#92055,#92056),
(#92057,#92058),(#92059,#92060),(#92061,#92062),(#92063,#92064),(#92065,
#92066),(#92067,#92068),(#92069,#92070),(#92071,#92072),(#92073,#92074),
(#92075,#92076),(#92077,#92078),(#92079,#92080),(#92081,#92082),(#92083,
#92084),(#92085,#92086),(#92087,#92088),(#92089,#92090),(#92091,#92092),
(#92093,#92094),(#92095,#92096),(#92097,#92098),(#92099,#92100),(#92101,
#92102),(#92103,#92104),(#92105,#92106),(#92107,#92108),(#92109,#92110),
(#92111,#92112),(#92113,#92114),(#92115,#92116),(#92117,#92118),(#92119,
#92120),(#92121,#92122),(#92123,#92124),(#92125,#92126),(#92127,#92128),
(#92129,#92130),(#92131,#92132),(#92133,#92134),(#92135,#92136),(#92137,
#92138),(#92139,#92140),(#92141,#92142),(#92143,#92144),(#92145,#92146),
(#92147,#92148),(#92149,#92150),(#92151,#92152),(#92153,#92154),(#92155,
#92156),(#92157,#92158),(#92159,#92160),(#92161,#92162),(#92163,#92164),
(#92165,#92166),(#92167,#92168),(#92169,#92170),(#92171,#92172),(#92173,
#92174),(#92175,#92176),(#92177,#92178),(#92179,#92180),(#92181,#92182),
(#92183,#92184),(#92185,#92186),(#92187,#92188),(#92189,#92190),(#92191,
#92192),(#92193,#92194),(#92195,#92196),(#92197,#92198),(#92199,#92200),
(#92201,#92202),(#92203,#92204),(#92205,#92206),(#92207,#92208),(#92209,
#92210),(#92211,#92212),(#92213,#92214),(#92215,#92216),(#92217,#92218),
(#92219,#92220),(#92221,#92222),(#92223,#92224),(#92225,#92226),(#92227,
#92228),(#92229,#92230),(#92231,#92232),(#92233,#92234),(#92235,#92236),
(#92237,#92238),(#92239,#92240),(#92241,#92242),(#92243,#92244),(#92245,
#92246),(#92247,#92248),(#92249,#92250),(#92251,#92252),(#92253,#92254),
(#92255,#92256),(#92257,#92258),(#92259,#92260),(#92261,#92262),(#92263,
#92264),(#92265,#92266),(#92267,#92268),(#92269,#92270),(#92271,#92272),
(#92273,#92274),(#92275,#92276),(#92277,#92278),(#92279,#92280),(#92281,
#92282),(#92283,#92284),(#92285,#92286),(#92287,#92288),(#92289,#92290),
(#92291,#92292),(#92293,#92294),(#92295,#92296),(#92297,#92298),(#92299,
#92300),(#92301,#92302),(#92303,#92304),(#92305,#92306),(#92307,#92308),
(#92309,#92310),(#92311,#92312),(#92313,#92314),(#92315,#92316),(#92317,
#92318),(#92319,#92320),(#92321,#92322),(#92323,#92324),(#92325,#92326),
(#92327,#92328),(#92329,#92330),(#92331,#92332),(#92333,#92334),(#92335,
#92336),(#92337,#92338),(#92339,#92340),(#92341,#92342),(#92343,#92344),
(#92345,#92346),(#92347,#92348),(#92349,#92350),(#92351,#92352),(#92353,
#92354),(#92355,#92356),(#92357,#92358),(#92359,#92360),(#92361,#92362),
(#92363,#92364),(#92365,#92366),(#92367,#92368),(#92369,#92370),(#92371,
#92372),(#92373,#92374),(#92375,#92376),(#92377,#92378),(#92379,#92380),
(#92381,#92382),(#92383,#92384),(#92385,#92386),(#92387,#92388),(#92389,
#92390),(#92391,#92392),(#92393,#92394),(#92395,#92396),(#92397,#92398),
(#92399,#92400),(#92401,#92402),(#92403,#92404),(#92405,#92406),(#92407,
#92408),(#92409,#92410),(#92411,#92412),(#92413,#92414),(#92415,#92416),
(#92417,#92418),(#92419,#92420),(#92421,#92422),(#92423,#92424),(#92425,
#92426),(#92427,#92428),(#92429,#92430)),.UNSPECIFIED.,.F.,.F.,.F.)
B_SPLINE_SURFACE_WITH_KNOTS((6,1,1,1,1,1,1,1,1,1,1,1,1,1,1,1,1,1,1,1,1,
1,1,1,1,1,1,1,1,1,1,1,1,1,1,1,1,1,1,1,1,1,1,1,1,1,1,1,1,1,1,1,1,1,1,1,1,
1,1,1,1,1,1,1,1,1,1,1,1,1,1,1,1,1,1,1,1,1,1,1,1,1,1,1,1,1,1,1,1,1,1,1,1,
1,1,1,1,1,1,1,1,1,1,1,1,1,1,1,1,1,1,1,1,1,1,1,1,1,1,1,1,1,1,1,1,1,1,1,1,
1,1,1,1,1,1,1,1,1,1,1,1,1,1,1,1,1,1,1,1,1,1,1,1,1,1,1,1,1,1,1,1,1,1,1,1,
1,1,1,1,1,1,1,1,1,1,1,1,1,1,1,1,1,1,1,1,1,1,1,1,1,1,1,1,1,1,1,1,1,1,1,1,
1,1,1,1,1,1,1,1,1,1,1,1,1,1,1,1,1,1,1,1,1,1,1,1,1,1,1,1,1,1,1,1,1,1,1,1,
1,1,1,1,1,1,1,1,1,1,1,1,1,1,1,1,1,1,1,1,1,1,1,1,1,1,1,1,1,1,1,1,1,1,1,1,
1,1,1,1,1,1,1,1,1,1,1,1,1,1,1,1,1,1,1,1,1,1,1,1,1,1,1,1,1,1,1,1,1,1,1,1,
1,1,1,1,1,1,1,1,1,1,1,1,1,1,1,1,1,1,1,1,1,1,1,1,1,1,1,1,1,1,1,1,1,1,1,1,
1,1,1,1,1,1,1,1,1,1,1,1,1,1,1,1,1,1,1,1,1,1,1,1,1,1,1,1,1,1,1,1,1,1,1,1,
1,1,1,1,1,1,1,1,1,1,1,1,1,1,1,1,1,1,1,1,1,1,1,1,1,1,1,1,1,1,1,1,1,1,1,1,
1,1,1,1,1,1,1,1,1,1,1,1,1,1,1,1,1,1,1,1,1,1,1,1,1,1,1,1,1,1,1,1,1,1,1,1,
1,1,1,1,1,1,1,1,1,1,1,1,1,1,1,1,1,1,1,1,1,1,1,1,1,1,1,1,1,1,1,1,1,1,1,1,
1,1,1,1,1,1,1,1,1,1,1,1,1,1,1,1,1,1,1,1,1,1,1,1,1,1,1,1,1,1,1,1,1,1,1,1,
1,1,1,1,1,1,1,1,1,1,1,1,1,1,1,1,1,1,1,1,1,1,1,1,1,1,1,1,1,1,1,1,1,1,1,1,
1,1,1,1,1,1,1,1,1,1,1,1,1,1,1,1,1,1,1,1,1,1,1,1,1,1,1,1,1,1,1,1,1,1,1,1,
1,1,1,1,1,1,1,1,1,1,1,1,1,1,1,1,1,1,1,1,1,1,1,1,1,1,1,1,1,1,1,1,1,1,1,1,
1,1,1,1,1,1,1,1,1,1,1,1,1,1,1,1,1,1,1,1,1,1,1,1,1,1,1,1,1,1,1,1,1,1,1,1,
1,1,1,1,1,1,1,1,1,1,1,1,1,1,1,1,1,1,1,1,1,1,1,1,1,1,1,1,1,1,1,1,1,1,1,1,
1,1,1,1,1,1,1,1,1,1,1,1,1,1,1,1,1,1,1,1,1,1,1,1,1,1,1,1,1,1,1,1,1,1,1,1,
1,1,1,1,1,1,1,1,1,1,1,1,1,1,1,1,1,1,1,1,1,1,1,1,1,1,1,1,1,1,1,1,1,1,1,1,
1,1,1,1,1,1,1,1,1,1,1,1,1,1,1,1,1,1,1,1,1,1,1,1,1,1,1,1,1,1,1,1,1,1,1,1,
1,1,1,1,1,1,1,1,1,1,1,1,1,1,1,1,1,1,1,1,1,1,1,1,1,1,1,1,1,1,1,1,1,1,1,1,
1,1,1,1,1,1,1,1,1,1,1,1,1,1,1,1,1,1,1,1,1,1,1,1,1,1,1,1,1,1,1,1,1,1,1,1,
1,1,1,1,1,1,1,1,1,1,1,1,1,1,1,1,1,1,1,1,1,1,1,1,1,1,1,1,1,1,1,1,1,1,1,1,
1,1,1,1,1,1,1,1,1,1,1,1,1,1,1,1,1,1,1,1,1,1,1,1,1,1,1,1,1,1,1,1,1,1,1,1,
1,1,1,1,1,1,1,1,1,1,1,1,1,1,1,1,1,1,1,1,1,1,1,1,1,1,1,1,1,1,1,1,1,1,1,1,
1,1,1,1,1,1,1,6),(2,2),(-1.,-0.999000000000001,-0.998000000000001,-0.997000000000001,
-0.996000000000001,-0.995000000000001,-0.994000000000001,-0.993000000000001,
-0.992000000000001,-0.991000000000001,-0.990000000000001,-0.989000000000001,
-0.988000000000001,-0.987000000000001,-0.986000000000001,-0.985000000000001,
-0.984000000000001,-0.983000000000001,-0.982000000000001,-0.981000000000001,
-0.980000000000001,-0.979000000000001,-0.978000000000001,-0.977000000000001,
-0.976000000000001,-0.975000000000001,-0.974000000000001,-0.973000000000001,
-0.972000000000001,-0.971000000000001,-0.970000000000001,-0.969000000000001,
-0.968000000000001,-0.967000000000001,-0.966000000000001,-0.965000000000001,
-0.964000000000001,-0.963000000000001,-0.962000000000001,-0.961000000000001,
-0.960000000000001,-0.959000000000001,-0.958000000000001,-0.957000000000001,
-0.956000000000001,-0.955000000000001,-0.954000000000001,-0.953000000000001,
-0.952000000000001,-0.951000000000001,-0.950000000000001,-0.949000000000001,
-0.948000000000001,-0.947000000000001,-0.946000000000001,-0.945000000000001,
-0.944000000000001,-0.943000000000001,-0.942000000000001,-0.941000000000001,
-0.940000000000001,-0.939000000000001,-0.938000000000001,-0.937000000000001,
-0.936000000000001,-0.935000000000001,-0.934000000000001,-0.933000000000001,
-0.932000000000001,-0.931000000000001,-0.930000000000001,-0.929000000000001,
-0.928000000000001,-0.927000000000001,-0.926000000000001,-0.925000000000001,
-0.924000000000001,-0.923000000000001,-0.922000000000001,-0.921000000000001,
-0.920000000000001,-0.919000000000001,-0.918000000000001,-0.917000000000001,
-0.916000000000001,-0.915000000000001,-0.914000000000001,-0.913000000000001,
-0.912000000000001,-0.911000000000001,-0.910000000000001,-0.909000000000001,
-0.908000000000001,-0.907000000000001,-0.906000000000001,-0.905000000000001,
-0.904000000000001,-0.903000000000001,-0.902000000000001,-0.901000000000001,
-0.900000000000001,-0.899000000000001,-0.898000000000001,-0.897000000000001,
-0.896000000000001,-0.895000000000001,-0.894000000000001,-0.893000000000001,
-0.892000000000001,-0.891000000000001,-0.890000000000001,-0.889000000000001,
-0.888000000000001,-0.887000000000001,-0.886000000000001,-0.885000000000001,
-0.884000000000001,-0.883000000000001,-0.882000000000001,-0.881000000000001,
-0.880000000000001,-0.879000000000001,-0.878000000000001,-0.877000000000001,
-0.876000000000001,-0.875000000000001,-0.874000000000001,-0.873000000000001,
-0.872000000000001,-0.871000000000001,-0.870000000000001,-0.869000000000001,
-0.868000000000001,-0.867000000000001,-0.866000000000001,-0.865000000000001,
-0.864000000000001,-0.863000000000001,-0.862000000000001,-0.861000000000001,
-0.860000000000001,-0.859000000000001,-0.858000000000001,-0.857000000000001,
-0.856000000000001,-0.855000000000001,-0.854000000000001,-0.853000000000001,
-0.852000000000001,-0.851000000000001,-0.850000000000001,-0.849000000000001,
-0.848000000000001,-0.847000000000001,-0.846000000000001,-0.845000000000001,
-0.844000000000001,-0.843000000000001,-0.842000000000001,-0.841000000000001,
-0.840000000000001,-0.839000000000001,-0.838000000000001,-0.837000000000001,
-0.836000000000001,-0.835000000000001,-0.834000000000001,-0.833000000000001,
-0.832000000000001,-0.831000000000001,-0.830000000000001,-0.829000000000001,
-0.828000000000001,-0.827000000000001,-0.826000000000001,-0.825000000000001,
-0.824000000000001,-0.823000000000001,-0.822000000000001,-0.821000000000001,
-0.820000000000001,-0.819000000000001,-0.818000000000001,-0.817000000000001,
-0.816000000000001,-0.815000000000001,-0.814000000000001,-0.813000000000001,
-0.812000000000001,-0.811000000000001,-0.810000000000001,-0.809000000000001,
-0.808000000000001,-0.807000000000001,-0.806000000000001,-0.805000000000001,
-0.804000000000001,-0.803000000000001,-0.802000000000001,-0.801000000000001,
-0.800000000000001,-0.799000000000001,-0.798000000000001,-0.797000000000001,
-0.796000000000001,-0.795000000000001,-0.794000000000001,-0.793000000000001,
-0.792000000000001,-0.791000000000001,-0.790000000000001,-0.789000000000001,
-0.788000000000001,-0.787000000000001,-0.786000000000001,-0.785000000000001,
-0.784000000000001,-0.783000000000001,-0.782000000000001,-0.781000000000001,
-0.780000000000001,-0.779000000000001,-0.778000000000001,-0.777000000000001,
-0.776000000000001,-0.775000000000001,-0.774000000000001,-0.773000000000001,
-0.772000000000001,-0.771000000000001,-0.770000000000001,-0.769000000000001,
-0.768000000000001,-0.767000000000001,-0.766000000000001,-0.765000000000001,
-0.764000000000001,-0.763000000000001,-0.762000000000001,-0.761000000000001,
-0.760000000000001,-0.759000000000001,-0.758000000000001,-0.757000000000001,
-0.756000000000001,-0.755000000000001,-0.754000000000001,-0.753000000000001,
-0.752000000000001,-0.751000000000001,-0.750000000000001,-0.749000000000001,
-0.748000000000001,-0.747000000000001,-0.746000000000001,-0.745000000000001,
-0.744000000000001,-0.743000000000001,-0.742000000000001,-0.741000000000001,
-0.740000000000001,-0.739000000000001,-0.738000000000001,-0.737000000000001,
-0.736000000000001,-0.735000000000001,-0.734000000000001,-0.733000000000001,
-0.732000000000001,-0.731000000000001,-0.730000000000001,-0.729000000000001,
-0.728000000000001,-0.727000000000001,-0.726000000000001,-0.725000000000001,
-0.724000000000001,-0.723000000000001,-0.722000000000001,-0.721000000000001,
-0.720000000000001,-0.719000000000001,-0.718000000000001,-0.717000000000001,
-0.716000000000001,-0.715000000000001,-0.714000000000001,-0.713000000000001,
-0.712000000000001,-0.711000000000001,-0.710000000000001,-0.709000000000001,
-0.708000000000001,-0.707000000000001,-0.706000000000001,-0.705000000000001,
-0.704000000000001,-0.703000000000001,-0.702000000000001,-0.701000000000001,
-0.700000000000001,-0.699000000000001,-0.698000000000001,-0.697000000000001,
-0.696000000000001,-0.695000000000001,-0.694000000000001,-0.693000000000001,
-0.692000000000001,-0.691000000000001,-0.690000000000001,-0.689000000000001,
-0.688000000000001,-0.687,-0.686,-0.685,-0.684,-0.683,-0.682,-0.681,-0.68,
-0.679,-0.678,-0.677,-0.676,-0.675,-0.674,-0.673,-0.672,-0.671,-0.67,-0.669,
-0.668,-0.667,-0.666,-0.665,-0.664,-0.663,-0.662,-0.661,-0.66,-0.659,-0.658,
-0.657,-0.656,-0.655,-0.654,-0.653,-0.652,-0.651,-0.65,-0.649,-0.648,-0.647,
-0.646,-0.645,-0.644,-0.643,-0.642,-0.641,-0.64,-0.639,-0.638,-0.637,-0.636,
-0.635,-0.634,-0.633,-0.632,-0.631,-0.63,-0.629,-0.628,-0.627,-0.626,-0.625,
-0.624,-0.623,-0.622,-0.621,-0.62,-0.619,-0.618,-0.617,-0.616,-0.615,-0.614,
-0.613,-0.612,-0.611,-0.61,-0.609,-0.608,-0.607,-0.606,-0.605,-0.604,-0.603,
-0.602,-0.601,-0.6,-0.599,-0.598,-0.597,-0.596,-0.595,-0.594,-0.593,-0.592,
-0.591,-0.59,-0.589,-0.588,-0.587,-0.586,-0.585,-0.584,-0.583,-0.582,-0.581,
-0.58,-0.579,-0.578,-0.577,-0.576,-0.575,-0.574,-0.573,-0.572,-0.571,-0.57,
-0.569,-0.568,-0.567,-0.566,-0.565,-0.564,-0.563,-0.562,-0.561,-0.56,-0.559,
-0.558,-0.557,-0.556,-0.555,-0.554,-0.553,-0.552,-0.551,-0.55,-0.549,-0.548,
-0.547,-0.546,-0.545,-0.544,-0.543,-0.542,-0.541,-0.54,-0.539,-0.538,-0.537,
-0.536,-0.535,-0.534,-0.533,-0.532,-0.531,-0.53,-0.529,-0.528,-0.527,-0.526,
-0.525,-0.524,-0.523,-0.522,-0.521,-0.52,-0.519,-0.518,-0.517,-0.516,-0.515,
-0.514,-0.513,-0.512,-0.511,-0.51,-0.509,-0.508,-0.507,-0.506,-0.505,-0.504,
-0.503,-0.502,-0.501,-0.5,-0.499,-0.498,-0.497,-0.496,-0.495,-0.494,-0.493,
-0.492,-0.491,-0.49,-0.489,-0.488,-0.487,-0.486,-0.485,-0.484,-0.483,-0.482,
-0.481,-0.48,-0.479,-0.478,-0.477,-0.476,-0.475,-0.474,-0.473,-0.472,-0.471,
-0.47,-0.469,-0.468,-0.467,-0.466,-0.465,-0.464,-0.463,-0.462,-0.461,-0.46,
-0.459,-0.458,-0.457,-0.456,-0.455,-0.454,-0.453,-0.452,-0.451,-0.45,-0.449,
-0.448,-0.447,-0.446,-0.445,-0.444,-0.443,-0.442,-0.441,-0.44,-0.439,-0.438,
-0.437,-0.436,-0.435,-0.434,-0.433,-0.432,-0.431,-0.43,-0.429,-0.428,-0.427,
-0.426,-0.425,-0.424,-0.423,-0.422,-0.421,-0.42,-0.419,-0.418,-0.417,-0.416,
-0.415,-0.414,-0.413,-0.412,-0.411,-0.41,-0.409,-0.408,-0.407,-0.406,-0.405,
-0.404,-0.403,-0.402,-0.401,-0.4,-0.399,-0.398,-0.397,-0.396,-0.395,-0.394,
-0.393,-0.392,-0.391,-0.39,-0.389,-0.388,-0.387,-0.386,-0.385,-0.384,-0.383,
-0.382,-0.381,-0.38,-0.379,-0.378,-0.377,-0.376,-0.375,-0.374,-0.373,-0.372,
-0.371,-0.37,-0.369,-0.368,-0.367,-0.366,-0.365,-0.364,-0.363,-0.362,-0.361,
-0.36,-0.359,-0.358,-0.357,-0.356,-0.355,-0.354,-0.353,-0.352,-0.351,-0.35,
-0.349,-0.348,-0.347,-0.346,-0.345,-0.344,-0.343,-0.342,-0.341,-0.34,-0.339,
-0.338,-0.337,-0.336,-0.335,-0.334,-0.333,-0.332,-0.331,-0.33,-0.329,-0.328,
-0.327,-0.326,-0.325,-0.324,-0.323,-0.322,-0.321,-0.32,-0.319,-0.318,-0.317,
-0.316,-0.315,-0.314,-0.313,-0.312,-0.311,-0.31,-0.309,-0.308,-0.307,-0.306,
-0.305,-0.304,-0.303,-0.302,-0.301,-0.3,-0.299,-0.298,-0.297,-0.296,-0.295,
-0.294,-0.293,-0.292,-0.291,-0.29,-0.289,-0.288,-0.287,-0.286,-0.285,-0.284,
-0.283,-0.282,-0.281,-0.28,-0.279,-0.278,-0.277,-0.276,-0.275,-0.274,-0.273,
-0.272,-0.271,-0.27,-0.269,-0.268,-0.267,-0.266,-0.265,-0.264,-0.263,-0.262,
-0.261,-0.26,-0.259,-0.258,-0.257,-0.256,-0.255,-0.254,-0.253,-0.252,-0.251,
-0.25,-0.249,-0.248,-0.247,-0.246,-0.245,-0.244,-0.243,-0.242,-0.241,-0.24,
-0.239,-0.238,-0.237,-0.236,-0.235,-0.234,-0.233,-0.232,-0.231,-0.23,-0.229,
-0.228,-0.227,-0.226,-0.225,-0.224,-0.223,-0.222,-0.221,-0.22,-0.219,-0.218,
-0.217,-0.216,-0.215,-0.214,-0.213,-0.212,-0.211,-0.21,-0.209,-0.208,-0.207,
-0.206,-0.205,-0.204,-0.203,-0.202,-0.201,-0.2,-0.199,-0.198,-0.197,-0.196,
-0.195,-0.194,-0.193,-0.192,-0.191,-0.19,-0.189,-0.188,-0.187,-0.186,-0.185,
-0.184,-0.183,-0.182,-0.181,-0.18,-0.179,-0.178,-0.177,-0.176,-0.175,-0.174,
-0.173,-0.172,-0.171,-0.17,-0.169,-0.168,-0.167,-0.166,-0.165,-0.164,-0.163,
-0.162,-0.161,-0.16,-0.159,-0.158,-0.157,-0.156,-0.155,-0.154,-0.153,-0.152,
-0.151,-0.15,-0.149,-0.148,-0.147,-0.146,-0.145,-0.144,-0.143,-0.142,-0.141,
-0.14,-0.139,-0.138,-0.137,-0.136,-0.135,-0.134,-0.133,-0.132,-0.131,-0.13,
-0.129,-0.128,-0.127,-0.126,-0.125,-0.124,-0.123,-0.122,-0.121,-0.12,-0.119,
-0.118,-0.117,-0.116,-0.115,-0.114,-0.113,-0.112,-0.111,-0.11,-0.109,-0.108,
-0.107,-0.106,-0.105,-0.104,-0.103,-0.102,-0.101,-0.1,-0.0990000000000001,
-0.0980000000000001,-0.0970000000000001,-0.0960000000000001,-0.0950000000000001,
-0.0940000000000001,-0.0930000000000001,-0.0920000000000001,-0.0910000000000001,
-0.0900000000000001,-0.0890000000000001,-0.0880000000000001,-0.0870000000000001,
-0.0860000000000001,-0.0850000000000001,-0.0840000000000001,-0.0830000000000001,
-0.0820000000000001,-0.0810000000000001,-0.0800000000000001,-0.0790000000000001,
-0.0780000000000001,-0.0770000000000001,-0.0760000000000001,-0.0750000000000001,
-0.0740000000000001,-0.0730000000000001,-0.0720000000000001,-0.071,-0.07,
-0.069,-0.068,-0.067,-0.066,-0.065,-0.064,-0.063,-0.062,-0.061,-0.06,-0.059,
-0.058,-0.057,-0.056,-0.055,-0.054,-0.053,-0.052,-0.051,-0.05,-0.049,-0.048,
-0.047,-0.046,-0.045,-0.044,-0.043,-0.042,-0.041,-0.04,-0.039,-0.038,-0.037,
-0.036,-0.035,-0.034,-0.033,-0.032,-0.031,-0.03,-0.029,-0.028,-0.027,-0.026,
-0.025,-0.024,-0.023,-0.022,-0.021,-0.02,-0.019,-0.018,-0.017,-0.016,-0.015,
-0.014,-0.013,-0.012,-0.011,-0.01,-0.009,-0.008,-0.007,-0.006,-0.005,-0.004,
-0.003,-0.002,-0.001,0.),(0.,2.),.UNSPECIFIED.)
GEOMETRIC_REPRESENTATION_ITEM()
RATIONAL_B_SPLINE_SURFACE(((1.,1.),(1.,1.),(1.,1.),(1.,1.),(1.,1.),(1.,
1.),(1.,1.),(1.,1.),(1.,1.),(1.,1.),(1.,1.),(1.,1.),(1.,1.),(1.,1.),(1.,
1.),(1.,1.),(1.,1.),(1.,1.),(1.,1.),(1.,1.),(1.,1.),(1.,1.),(1.,1.),(1.,
1.),(1.,1.),(1.,1.),(1.,1.),(1.,1.),(1.,1.),(1.,1.),(1.,1.),(1.,1.),(1.,
1.),(1.,1.),(1.,1.),(1.,1.),(1.,1.),(1.,1.),(1.,1.),(1.,1.),(1.,1.),(1.,
1.),(1.,1.),(1.,1.),(1.,1.),(1.,1.),(1.,1.),(1.,1.),(1.,1.),(1.,1.),(1.,
1.),(1.,1.),(1.,1.),(1.,1.),(1.,1.),(1.,1.),(1.,1.),(1.,1.),(1.,1.),(1.,
1.),(1.,1.),(1.,1.),(1.,1.),(1.,1.),(1.,1.),(1.,1.),(1.,1.),(1.,1.),(1.,
1.),(1.,1.),(1.,1.),(1.,1.),(1.,1.),(1.,1.),(1.,1.),(1.,1.),(1.,1.),(1.,
1.),(1.,1.),(1.,1.),(1.,1.),(1.,1.),(1.,1.),(1.,1.),(1.,1.),(1.,1.),(1.,
1.),(1.,1.),(1.,1.),(1.,1.),(1.,1.),(1.,1.),(1.,1.),(1.,1.),(1.,1.),(1.,
1.),(1.,1.),(1.,1.),(1.,1.),(1.,1.),(1.,1.),(1.,1.),(1.,1.),(1.,1.),(1.,
1.),(1.,1.),(1.,1.),(1.,1.),(1.,1.),(1.,1.),(1.,1.),(1.,1.),(1.,1.),(1.,
1.),(1.,1.),(1.,1.),(1.,1.),(1.,1.),(1.,1.),(1.,1.),(1.,1.),(1.,1.),(1.,
1.),(1.,1.),(1.,1.),(1.,1.),(1.,1.),(1.,1.),(1.,1.),(1.,1.),(1.,1.),(1.,
1.),(1.,1.),(1.,1.),(1.,1.),(1.,1.),(1.,1.),(1.,1.),(1.,1.),(1.,1.),(1.,
1.),(1.,1.),(1.,1.),(1.,1.),(1.,1.),(1.,1.),(1.,1.),(1.,1.),(1.,1.),(1.,
1.),(1.,1.),(1.,1.),(1.,1.),(1.,1.),(1.,1.),(1.,1.),(1.,1.),(1.,1.),(1.,
1.),(1.,1.),(1.,1.),(1.,1.),(1.,1.),(1.,1.),(1.,1.),(1.,1.),(1.,1.),(1.,
1.),(1.,1.),(1.,1.),(1.,1.),(1.,1.),(1.,1.),(1.,1.),(1.,1.),(1.,1.),(1.,
1.),(1.,1.),(1.,1.),(1.,1.),(1.,1.),(1.,1.),(1.,1.),(1.,1.),(1.,1.),(1.,
1.),(1.,1.),(1.,1.),(1.,1.),(1.,1.),(1.,1.),(1.,1.),(1.,1.),(1.,1.),(1.,
1.),(1.,1.),(1.,1.),(1.,1.),(1.,1.),(1.,1.),(1.,1.),(1.,1.),(1.,1.),(1.,
1.),(1.,1.),(1.,1.),(1.,1.),(1.,1.),(1.,1.),(1.,1.),(1.,1.),(1.,1.),(1.,
1.),(1.,1.),(1.,1.),(1.,1.),(1.,1.),(1.,1.),(1.,1.),(1.,1.),(1.,1.),(1.,
1.),(1.,1.),(1.,1.),(1.,1.),(1.,1.),(1.,1.),(1.,1.),(1.,1.),(1.,1.),(1.,
1.),(1.,1.),(1.,1.),(1.,1.),(1.,1.),(1.,1.),(1.,1.),(1.,1.),(1.,1.),(1.,
1.),(1.,1.),(1.,1.),(1.,1.),(1.,1.),(1.,1.),(1.,1.),(1.,1.),(1.,1.),(1.,
1.),(1.,1.),(1.,1.),(1.,1.),(1.,1.),(1.,1.),(1.,1.),(1.,1.),(1.,1.),(1.,
1.),(1.,1.),(1.,1.),(1.,1.),(1.,1.),(1.,1.),(1.,1.),(1.,1.),(1.,1.),(1.,
1.),(1.,1.),(1.,1.),(1.,1.),(1.,1.),(1.,1.),(1.,1.),(1.,1.),(1.,1.),(1.,
1.),(1.,1.),(1.,1.),(1.,1.),(1.,1.),(1.,1.),(1.,1.),(1.,1.),(1.,1.),(1.,
1.),(1.,1.),(1.,1.),(1.,1.),(1.,1.),(1.,1.),(1.,1.),(1.,1.),(1.,1.),(1.,
1.),(1.,1.),(1.,1.),(1.,1.),(1.,1.),(1.,1.),(1.,1.),(1.,1.),(1.,1.),(1.,
1.),(1.,1.),(1.,1.),(1.,1.),(1.,1.),(1.,1.),(1.,1.),(1.,1.),(1.,1.),(1.,
1.),(1.,1.),(1.,1.),(1.,1.),(1.,1.),(1.,1.),(1.,1.),(1.,1.),(1.,1.),(1.,
1.),(1.,1.),(1.,1.),(1.,1.),(1.,1.),(1.,1.),(1.,1.),(1.,1.),(1.,1.),(1.,
1.),(1.,1.),(1.,1.),(1.,1.),(1.,1.),(1.,1.),(1.,1.),(1.,1.),(1.,1.),(1.,
1.),(1.,1.),(1.,1.),(1.,1.),(1.,1.),(1.,1.),(1.,1.),(1.,1.),(1.,1.),(1.,
1.),(1.,1.),(1.,1.),(1.,1.),(1.,1.),(1.,1.),(1.,1.),(1.,1.),(1.,1.),(1.,
1.),(1.,1.),(1.,1.),(1.,1.),(1.,1.),(1.,1.),(1.,1.),(1.,1.),(1.,1.),(1.,
1.),(1.,1.),(1.,1.),(1.,1.),(1.,1.),(1.,1.),(1.,1.),(1.,1.),(1.,1.),(1.,
1.),(1.,1.),(1.,1.),(1.,1.),(1.,1.),(1.,1.),(1.,1.),(1.,1.),(1.,1.),(1.,
1.),(1.,1.),(1.,1.),(1.,1.),(1.,1.),(1.,1.),(1.,1.),(1.,1.),(1.,1.),(1.,
1.),(1.,1.),(1.,1.),(1.,1.),(1.,1.),(1.,1.),(1.,1.),(1.,1.),(1.,1.),(1.,
1.),(1.,1.),(1.,1.),(1.,1.),(1.,1.),(1.,1.),(1.,1.),(1.,1.),(1.,1.),(1.,
1.),(1.,1.),(1.,1.),(1.,1.),(1.,1.),(1.,1.),(1.,1.),(1.,1.),(1.,1.),(1.,
1.),(1.,1.),(1.,1.),(1.,1.),(1.,1.),(1.,1.),(1.,1.),(1.,1.),(1.,1.),(1.,
1.),(1.,1.),(1.,1.),(1.,1.),(1.,1.),(1.,1.),(1.,1.),(1.,1.),(1.,1.),(1.,
1.),(1.,1.),(1.,1.),(1.,1.),(1.,1.),(1.,1.),(1.,1.),(1.,1.),(1.,1.),(1.,
1.),(1.,1.),(1.,1.),(1.,1.),(1.,1.),(1.,1.),(1.,1.),(1.,1.),(1.,1.),(1.,
1.),(1.,1.),(1.,1.),(1.,1.),(1.,1.),(1.,1.),(1.,1.),(1.,1.),(1.,1.),(1.,
1.),(1.,1.),(1.,1.),(1.,1.),(1.,1.),(1.,1.),(1.,1.),(1.,1.),(1.,1.),(1.,
1.),(1.,1.),(1.,1.),(1.,1.),(1.,1.),(1.,1.),(1.,1.),(1.,1.),(1.,1.),(1.,
1.),(1.,1.),(1.,1.),(1.,1.),(1.,1.),(1.,1.),(1.,1.),(1.,1.),(1.,1.),(1.,
1.),(1.,1.),(1.,1.),(1.,1.),(1.,1.),(1.,1.),(1.,1.),(1.,1.),(1.,1.),(1.,
1.),(1.,1.),(1.,1.),(1.,1.),(1.,1.),(1.,1.),(1.,1.),(1.,1.),(1.,1.),(1.,
1.),(1.,1.),(1.,1.),(1.,1.),(1.,1.),(1.,1.),(1.,1.),(1.,1.),(1.,1.),(1.,
1.),(1.,1.),(1.,1.),(1.,1.),(1.,1.),(1.,1.),(1.,1.),(1.,1.),(1.,1.),(1.,
1.),(1.,1.),(1.,1.),(1.,1.),(1.,1.),(1.,1.),(1.,1.),(1.,1.),(1.,1.),(1.,
1.),(1.,1.),(1.,1.),(1.,1.),(1.,1.),(1.,1.),(1.,1.),(1.,1.),(1.,1.),(1.,
1.),(1.,1.),(1.,1.),(1.,1.),(1.,1.),(1.,1.),(1.,1.),(1.,1.),(1.,1.),(1.,
1.),(1.,1.),(1.,1.),(1.,1.),(1.,1.),(1.,1.),(1.,1.),(1.,1.),(1.,1.),(1.,
1.),(1.,1.),(1.,1.),(1.,1.),(1.,1.),(1.,1.),(1.,1.),(1.,1.),(1.,1.),(1.,
1.),(1.,1.),(1.,1.),(1.,1.),(1.,1.),(1.,1.),(1.,1.),(1.,1.),(1.,1.),(1.,
1.),(1.,1.),(1.,1.),(1.,1.),(1.,1.),(1.,1.),(1.,1.),(1.,1.),(1.,1.),(1.,
1.),(1.,1.),(1.,1.),(1.,1.),(1.,1.),(1.,1.),(1.,1.),(1.,1.),(1.,1.),(1.,
1.),(1.,1.),(1.,1.),(1.,1.),(1.,1.),(1.,1.),(1.,1.),(1.,1.),(1.,1.),(1.,
1.),(1.,1.),(1.,1.),(1.,1.),(1.,1.),(1.,1.),(1.,1.),(1.,1.),(1.,1.),(1.,
1.),(1.,1.),(1.,1.),(1.,1.),(1.,1.),(1.,1.),(1.,1.),(1.,1.),(1.,1.),(1.,
1.),(1.,1.),(1.,1.),(1.,1.),(1.,1.),(1.,1.),(1.,1.),(1.,1.),(1.,1.),(1.,
1.),(1.,1.),(1.,1.),(1.,1.),(1.,1.),(1.,1.),(1.,1.),(1.,1.),(1.,1.),(1.,
1.),(1.,1.),(1.,1.),(1.,1.),(1.,1.),(1.,1.),(1.,1.),(1.,1.),(1.,1.),(1.,
1.),(1.,1.),(1.,1.),(1.,1.),(1.,1.),(1.,1.),(1.,1.),(1.,1.),(1.,1.),(1.,
1.),(1.,1.),(1.,1.),(1.,1.),(1.,1.),(1.,1.),(1.,1.),(1.,1.),(1.,1.),(1.,
1.),(1.,1.),(1.,1.),(1.,1.),(1.,1.),(1.,1.),(1.,1.),(1.,1.),(1.,1.),(1.,
1.),(1.,1.),(1.,1.),(1.,1.),(1.,1.),(1.,1.),(1.,1.),(1.,1.),(1.,1.),(1.,
1.),(1.,1.),(1.,1.),(1.,1.),(1.,1.),(1.,1.),(1.,1.),(1.,1.),(1.,1.),(1.,
1.),(1.,1.),(1.,1.),(1.,1.),(1.,1.),(1.,1.),(1.,1.),(1.,1.),(1.,1.),(1.,
1.),(1.,1.),(1.,1.),(1.,1.),(1.,1.),(1.,1.),(1.,1.),(1.,1.),(1.,1.),(1.,
1.),(1.,1.),(1.,1.),(1.,1.),(1.,1.),(1.,1.),(1.,1.),(1.,1.),(1.,1.),(1.,
1.),(1.,1.),(1.,1.),(1.,1.),(1.,1.),(1.,1.),(1.,1.),(1.,1.),(1.,1.),(1.,
1.),(1.,1.),(1.,1.),(1.,1.),(1.,1.),(1.,1.),(1.,1.),(1.,1.),(1.,1.),(1.,
1.),(1.,1.),(1.,1.),(1.,1.),(1.,1.),(1.,1.),(1.,1.),(1.,1.),(1.,1.),(1.,
1.),(1.,1.),(1.,1.),(1.,1.),(1.,1.),(1.,1.),(1.,1.),(1.,1.),(1.,1.),(1.,
1.),(1.,1.),(1.,1.),(1.,1.),(1.,1.),(1.,1.),(1.,1.),(1.,1.),(1.,1.),(1.,
1.),(1.,1.),(1.,1.),(1.,1.),(1.,1.),(1.,1.),(1.,1.),(1.,1.),(1.,1.),(1.,
1.),(1.,1.),(1.,1.),(1.,1.),(1.,1.),(1.,1.),(1.,1.),(1.,1.),(1.,1.),(1.,
1.),(1.,1.),(1.,1.),(1.,1.),(1.,1.),(1.,1.),(1.,1.),(1.,1.),(1.,1.),(1.,
1.),(1.,1.),(1.,1.),(1.,1.),(1.,1.),(1.,1.),(1.,1.),(1.,1.),(1.,1.),(1.,
1.),(1.,1.),(1.,1.),(1.,1.),(1.,1.),(1.,1.),(1.,1.),(1.,1.),(1.,1.),(1.,
1.),(1.,1.),(1.,1.),(1.,1.),(1.,1.),(1.,1.),(1.,1.),(1.,1.),(1.,1.),(1.,
1.),(1.,1.),(1.,1.),(1.,1.),(1.,1.),(1.,1.),(1.,1.),(1.,1.),(1.,1.),(1.,
1.),(1.,1.),(1.,1.),(1.,1.),(1.,1.),(1.,1.),(1.,1.),(1.,1.),(1.,1.),(1.,
1.),(1.,1.),(1.,1.),(1.,1.),(1.,1.),(1.,1.),(1.,1.),(1.,1.),(1.,1.),(1.,
1.),(1.,1.),(1.,1.),(1.,1.),(1.,1.),(1.,1.),(1.,1.),(1.,1.),(1.,1.),(1.,
1.),(1.,1.),(1.,1.),(1.,1.),(1.,1.),(1.,1.),(1.,1.),(1.,1.),(1.,1.),(1.,
1.),(1.,1.),(1.,1.),(1.,1.),(1.,1.),(1.,1.),(1.,1.),(1.,1.),(1.,1.),(1.,
1.),(1.,1.),(1.,1.),(1.,1.),(1.,1.),(1.,1.),(1.,1.),(1.,1.),(1.,1.),(1.,
1.),(1.,1.),(1.,1.),(1.,1.),(1.,1.),(1.,1.),(1.,1.),(1.,1.),(1.,1.),(1.,
1.),(1.,1.),(1.,1.),(1.,1.),(1.,1.),(1.,1.),(1.,1.),(1.,1.),(1.,1.),(1.,
1.),(1.,1.),(1.,1.),(1.,1.),(1.,1.),(1.,1.),(1.,1.),(1.,1.),(1.,1.),(1.,
1.),(1.,1.),(1.,1.),(1.,1.),(1.,1.),(1.,1.),(1.,1.),(1.,1.),(1.,1.),(1.,
1.),(1.,1.),(1.,1.),(1.,1.),(1.,1.),(1.,1.),(1.,1.),(1.,1.),(1.,1.),(1.,
1.),(1.,1.),(1.,1.),(1.,1.),(1.,1.),(1.,1.),(1.,1.),(1.,1.),(1.,1.),(1.,
1.),(1.,1.),(1.,1.),(1.,1.),(1.,1.),(1.,1.),(1.,1.),(1.,1.),(1.,1.),(1.,
1.),(1.,1.),(1.,1.),(1.,1.),(1.,1.),(1.,1.),(1.,1.),(1.,1.),(1.,1.),(1.,
1.),(1.,1.),(1.,1.),(1.,1.),(1.,1.),(1.,1.),(1.,1.),(1.,1.),(1.,1.),(1.,
1.),(1.,1.),(1.,1.),(1.,1.),(1.,1.),(1.,1.),(1.,1.),(1.,1.),(1.,1.),(1.,
1.),(1.,1.),(1.,1.),(1.,1.),(1.,1.),(1.,1.),(1.,1.),(1.,1.),(1.,1.),(1.,
1.),(1.,1.),(1.,1.),(1.,1.),(1.,1.),(1.,1.),(1.,1.),(1.,1.),(1.,1.),(1.,
1.),(1.,1.),(1.,1.),(1.,1.),(1.,1.),(1.,1.),(1.,1.),(1.,1.),(1.,1.),(1.,
1.)))
REPRESENTATION_ITEM('')
SURFACE()
);
#267=(
BOUNDED_SURFACE()
B_SPLINE_SURFACE(5,1,((#92433,#92434),(#92435,#92436),(#92437,#92438),(#92439,
#92440),(#92441,#92442),(#92443,#92444),(#92445,#92446),(#92447,#92448),
(#92449,#92450),(#92451,#92452),(#92453,#92454),(#92455,#92456),(#92457,
#92458),(#92459,#92460),(#92461,#92462),(#92463,#92464),(#92465,#92466),
(#92467,#92468),(#92469,#92470),(#92471,#92472),(#92473,#92474),(#92475,
#92476),(#92477,#92478),(#92479,#92480),(#92481,#92482),(#92483,#92484),
(#92485,#92486),(#92487,#92488),(#92489,#92490),(#92491,#92492),(#92493,
#92494),(#92495,#92496),(#92497,#92498),(#92499,#92500),(#92501,#92502),
(#92503,#92504),(#92505,#92506),(#92507,#92508),(#92509,#92510),(#92511,
#92512),(#92513,#92514),(#92515,#92516),(#92517,#92518),(#92519,#92520),
(#92521,#92522),(#92523,#92524),(#92525,#92526),(#92527,#92528),(#92529,
#92530),(#92531,#92532),(#92533,#92534),(#92535,#92536),(#92537,#92538),
(#92539,#92540),(#92541,#92542),(#92543,#92544),(#92545,#92546),(#92547,
#92548),(#92549,#92550),(#92551,#92552),(#92553,#92554),(#92555,#92556),
(#92557,#92558),(#92559,#92560),(#92561,#92562),(#92563,#92564),(#92565,
#92566),(#92567,#92568),(#92569,#92570),(#92571,#92572),(#92573,#92574),
(#92575,#92576),(#92577,#92578),(#92579,#92580),(#92581,#92582),(#92583,
#92584),(#92585,#92586),(#92587,#92588),(#92589,#92590),(#92591,#92592),
(#92593,#92594),(#92595,#92596),(#92597,#92598),(#92599,#92600),(#92601,
#92602),(#92603,#92604),(#92605,#92606),(#92607,#92608),(#92609,#92610),
(#92611,#92612),(#92613,#92614),(#92615,#92616),(#92617,#92618),(#92619,
#92620),(#92621,#92622),(#92623,#92624),(#92625,#92626),(#92627,#92628),
(#92629,#92630),(#92631,#92632),(#92633,#92634),(#92635,#92636),(#92637,
#92638),(#92639,#92640),(#92641,#92642),(#92643,#92644),(#92645,#92646),
(#92647,#92648),(#92649,#92650),(#92651,#92652),(#92653,#92654),(#92655,
#92656),(#92657,#92658),(#92659,#92660),(#92661,#92662),(#92663,#92664),
(#92665,#92666),(#92667,#92668),(#92669,#92670),(#92671,#92672),(#92673,
#92674),(#92675,#92676),(#92677,#92678),(#92679,#92680),(#92681,#92682),
(#92683,#92684),(#92685,#92686),(#92687,#92688),(#92689,#92690),(#92691,
#92692),(#92693,#92694),(#92695,#92696),(#92697,#92698),(#92699,#92700),
(#92701,#92702),(#92703,#92704),(#92705,#92706),(#92707,#92708),(#92709,
#92710),(#92711,#92712),(#92713,#92714),(#92715,#92716),(#92717,#92718),
(#92719,#92720),(#92721,#92722),(#92723,#92724),(#92725,#92726),(#92727,
#92728),(#92729,#92730),(#92731,#92732),(#92733,#92734),(#92735,#92736),
(#92737,#92738),(#92739,#92740),(#92741,#92742),(#92743,#92744),(#92745,
#92746),(#92747,#92748),(#92749,#92750),(#92751,#92752),(#92753,#92754),
(#92755,#92756),(#92757,#92758),(#92759,#92760),(#92761,#92762),(#92763,
#92764),(#92765,#92766),(#92767,#92768),(#92769,#92770),(#92771,#92772),
(#92773,#92774),(#92775,#92776),(#92777,#92778),(#92779,#92780),(#92781,
#92782),(#92783,#92784),(#92785,#92786),(#92787,#92788),(#92789,#92790),
(#92791,#92792),(#92793,#92794),(#92795,#92796),(#92797,#92798),(#92799,
#92800),(#92801,#92802),(#92803,#92804),(#92805,#92806),(#92807,#92808),
(#92809,#92810),(#92811,#92812),(#92813,#92814),(#92815,#92816),(#92817,
#92818),(#92819,#92820),(#92821,#92822),(#92823,#92824),(#92825,#92826),
(#92827,#92828),(#92829,#92830),(#92831,#92832),(#92833,#92834),(#92835,
#92836),(#92837,#92838),(#92839,#92840),(#92841,#92842),(#92843,#92844),
(#92845,#92846),(#92847,#92848),(#92849,#92850),(#92851,#92852),(#92853,
#92854),(#92855,#92856),(#92857,#92858),(#92859,#92860),(#92861,#92862),
(#92863,#92864),(#92865,#92866),(#92867,#92868),(#92869,#92870),(#92871,
#92872),(#92873,#92874),(#92875,#92876),(#92877,#92878),(#92879,#92880),
(#92881,#92882),(#92883,#92884),(#92885,#92886),(#92887,#92888),(#92889,
#92890),(#92891,#92892),(#92893,#92894),(#92895,#92896),(#92897,#92898),
(#92899,#92900),(#92901,#92902),(#92903,#92904),(#92905,#92906),(#92907,
#92908),(#92909,#92910),(#92911,#92912),(#92913,#92914),(#92915,#92916),
(#92917,#92918),(#92919,#92920),(#92921,#92922),(#92923,#92924),(#92925,
#92926),(#92927,#92928),(#92929,#92930),(#92931,#92932),(#92933,#92934),
(#92935,#92936),(#92937,#92938),(#92939,#92940),(#92941,#92942),(#92943,
#92944),(#92945,#92946),(#92947,#92948),(#92949,#92950),(#92951,#92952),
(#92953,#92954),(#92955,#92956),(#92957,#92958),(#92959,#92960),(#92961,
#92962),(#92963,#92964),(#92965,#92966),(#92967,#92968),(#92969,#92970),
(#92971,#92972),(#92973,#92974),(#92975,#92976),(#92977,#92978),(#92979,
#92980),(#92981,#92982),(#92983,#92984),(#92985,#92986),(#92987,#92988),
(#92989,#92990),(#92991,#92992),(#92993,#92994),(#92995,#92996),(#92997,
#92998),(#92999,#93000),(#93001,#93002),(#93003,#93004),(#93005,#93006),
(#93007,#93008),(#93009,#93010),(#93011,#93012),(#93013,#93014),(#93015,
#93016),(#93017,#93018),(#93019,#93020),(#93021,#93022),(#93023,#93024),
(#93025,#93026),(#93027,#93028),(#93029,#93030),(#93031,#93032),(#93033,
#93034),(#93035,#93036),(#93037,#93038),(#93039,#93040),(#93041,#93042),
(#93043,#93044),(#93045,#93046),(#93047,#93048),(#93049,#93050),(#93051,
#93052),(#93053,#93054),(#93055,#93056),(#93057,#93058),(#93059,#93060),
(#93061,#93062),(#93063,#93064),(#93065,#93066),(#93067,#93068),(#93069,
#93070),(#93071,#93072),(#93073,#93074),(#93075,#93076),(#93077,#93078),
(#93079,#93080),(#93081,#93082),(#93083,#93084),(#93085,#93086),(#93087,
#93088),(#93089,#93090),(#93091,#93092),(#93093,#93094),(#93095,#93096),
(#93097,#93098),(#93099,#93100),(#93101,#93102),(#93103,#93104),(#93105,
#93106),(#93107,#93108),(#93109,#93110),(#93111,#93112),(#93113,#93114),
(#93115,#93116),(#93117,#93118),(#93119,#93120),(#93121,#93122),(#93123,
#93124),(#93125,#93126),(#93127,#93128),(#93129,#93130),(#93131,#93132),
(#93133,#93134),(#93135,#93136),(#93137,#93138),(#93139,#93140),(#93141,
#93142),(#93143,#93144),(#93145,#93146),(#93147,#93148),(#93149,#93150),
(#93151,#93152),(#93153,#93154),(#93155,#93156),(#93157,#93158),(#93159,
#93160),(#93161,#93162),(#93163,#93164),(#93165,#93166),(#93167,#93168),
(#93169,#93170),(#93171,#93172),(#93173,#93174),(#93175,#93176),(#93177,
#93178),(#93179,#93180),(#93181,#93182),(#93183,#93184),(#93185,#93186),
(#93187,#93188),(#93189,#93190),(#93191,#93192),(#93193,#93194),(#93195,
#93196),(#93197,#93198),(#93199,#93200),(#93201,#93202),(#93203,#93204),
(#93205,#93206),(#93207,#93208),(#93209,#93210),(#93211,#93212),(#93213,
#93214),(#93215,#93216),(#93217,#93218),(#93219,#93220),(#93221,#93222),
(#93223,#93224),(#93225,#93226),(#93227,#93228),(#93229,#93230),(#93231,
#93232),(#93233,#93234),(#93235,#93236),(#93237,#93238),(#93239,#93240),
(#93241,#93242),(#93243,#93244),(#93245,#93246),(#93247,#93248),(#93249,
#93250),(#93251,#93252),(#93253,#93254),(#93255,#93256),(#93257,#93258),
(#93259,#93260),(#93261,#93262),(#93263,#93264),(#93265,#93266),(#93267,
#93268),(#93269,#93270),(#93271,#93272),(#93273,#93274),(#93275,#93276),
(#93277,#93278),(#93279,#93280),(#93281,#93282),(#93283,#93284),(#93285,
#93286),(#93287,#93288),(#93289,#93290),(#93291,#93292),(#93293,#93294),
(#93295,#93296),(#93297,#93298),(#93299,#93300),(#93301,#93302),(#93303,
#93304),(#93305,#93306),(#93307,#93308),(#93309,#93310),(#93311,#93312),
(#93313,#93314),(#93315,#93316),(#93317,#93318),(#93319,#93320),(#93321,
#93322),(#93323,#93324),(#93325,#93326),(#93327,#93328),(#93329,#93330),
(#93331,#93332),(#93333,#93334),(#93335,#93336),(#93337,#93338),(#93339,
#93340),(#93341,#93342),(#93343,#93344),(#93345,#93346),(#93347,#93348),
(#93349,#93350),(#93351,#93352),(#93353,#93354),(#93355,#93356),(#93357,
#93358),(#93359,#93360),(#93361,#93362),(#93363,#93364),(#93365,#93366),
(#93367,#93368),(#93369,#93370),(#93371,#93372),(#93373,#93374),(#93375,
#93376),(#93377,#93378),(#93379,#93380),(#93381,#93382),(#93383,#93384),
(#93385,#93386),(#93387,#93388),(#93389,#93390),(#93391,#93392),(#93393,
#93394),(#93395,#93396),(#93397,#93398),(#93399,#93400),(#93401,#93402),
(#93403,#93404),(#93405,#93406),(#93407,#93408),(#93409,#93410),(#93411,
#93412),(#93413,#93414),(#93415,#93416),(#93417,#93418),(#93419,#93420),
(#93421,#93422),(#93423,#93424),(#93425,#93426),(#93427,#93428),(#93429,
#93430),(#93431,#93432),(#93433,#93434),(#93435,#93436),(#93437,#93438),
(#93439,#93440),(#93441,#93442),(#93443,#93444),(#93445,#93446),(#93447,
#93448),(#93449,#93450),(#93451,#93452),(#93453,#93454),(#93455,#93456),
(#93457,#93458),(#93459,#93460),(#93461,#93462),(#93463,#93464),(#93465,
#93466),(#93467,#93468),(#93469,#93470),(#93471,#93472),(#93473,#93474),
(#93475,#93476),(#93477,#93478),(#93479,#93480),(#93481,#93482),(#93483,
#93484),(#93485,#93486),(#93487,#93488),(#93489,#93490),(#93491,#93492),
(#93493,#93494),(#93495,#93496),(#93497,#93498),(#93499,#93500),(#93501,
#93502),(#93503,#93504),(#93505,#93506),(#93507,#93508),(#93509,#93510),
(#93511,#93512),(#93513,#93514),(#93515,#93516),(#93517,#93518),(#93519,
#93520),(#93521,#93522),(#93523,#93524),(#93525,#93526),(#93527,#93528),
(#93529,#93530),(#93531,#93532),(#93533,#93534),(#93535,#93536),(#93537,
#93538),(#93539,#93540),(#93541,#93542),(#93543,#93544),(#93545,#93546),
(#93547,#93548),(#93549,#93550),(#93551,#93552),(#93553,#93554),(#93555,
#93556),(#93557,#93558),(#93559,#93560),(#93561,#93562),(#93563,#93564),
(#93565,#93566),(#93567,#93568),(#93569,#93570),(#93571,#93572),(#93573,
#93574),(#93575,#93576),(#93577,#93578),(#93579,#93580),(#93581,#93582),
(#93583,#93584),(#93585,#93586),(#93587,#93588),(#93589,#93590),(#93591,
#93592),(#93593,#93594),(#93595,#93596),(#93597,#93598),(#93599,#93600),
(#93601,#93602),(#93603,#93604),(#93605,#93606),(#93607,#93608),(#93609,
#93610),(#93611,#93612),(#93613,#93614),(#93615,#93616),(#93617,#93618),
(#93619,#93620),(#93621,#93622),(#93623,#93624),(#93625,#93626),(#93627,
#93628),(#93629,#93630),(#93631,#93632),(#93633,#93634),(#93635,#93636),
(#93637,#93638),(#93639,#93640),(#93641,#93642),(#93643,#93644),(#93645,
#93646),(#93647,#93648),(#93649,#93650),(#93651,#93652),(#93653,#93654),
(#93655,#93656),(#93657,#93658),(#93659,#93660),(#93661,#93662),(#93663,
#93664),(#93665,#93666),(#93667,#93668),(#93669,#93670),(#93671,#93672),
(#93673,#93674),(#93675,#93676),(#93677,#93678),(#93679,#93680),(#93681,
#93682),(#93683,#93684),(#93685,#93686),(#93687,#93688),(#93689,#93690),
(#93691,#93692),(#93693,#93694),(#93695,#93696),(#93697,#93698),(#93699,
#93700),(#93701,#93702),(#93703,#93704),(#93705,#93706),(#93707,#93708),
(#93709,#93710),(#93711,#93712),(#93713,#93714),(#93715,#93716),(#93717,
#93718),(#93719,#93720),(#93721,#93722),(#93723,#93724),(#93725,#93726),
(#93727,#93728),(#93729,#93730),(#93731,#93732),(#93733,#93734),(#93735,
#93736),(#93737,#93738),(#93739,#93740),(#93741,#93742),(#93743,#93744),
(#93745,#93746),(#93747,#93748),(#93749,#93750),(#93751,#93752),(#93753,
#93754),(#93755,#93756),(#93757,#93758),(#93759,#93760),(#93761,#93762),
(#93763,#93764),(#93765,#93766),(#93767,#93768),(#93769,#93770),(#93771,
#93772),(#93773,#93774),(#93775,#93776),(#93777,#93778),(#93779,#93780),
(#93781,#93782),(#93783,#93784),(#93785,#93786),(#93787,#93788),(#93789,
#93790),(#93791,#93792),(#93793,#93794),(#93795,#93796),(#93797,#93798),
(#93799,#93800),(#93801,#93802),(#93803,#93804),(#93805,#93806),(#93807,
#93808),(#93809,#93810),(#93811,#93812),(#93813,#93814),(#93815,#93816),
(#93817,#93818),(#93819,#93820),(#93821,#93822),(#93823,#93824),(#93825,
#93826),(#93827,#93828),(#93829,#93830),(#93831,#93832),(#93833,#93834),
(#93835,#93836),(#93837,#93838),(#93839,#93840),(#93841,#93842),(#93843,
#93844),(#93845,#93846),(#93847,#93848),(#93849,#93850),(#93851,#93852),
(#93853,#93854),(#93855,#93856),(#93857,#93858),(#93859,#93860),(#93861,
#93862),(#93863,#93864),(#93865,#93866),(#93867,#93868),(#93869,#93870),
(#93871,#93872),(#93873,#93874),(#93875,#93876),(#93877,#93878),(#93879,
#93880),(#93881,#93882),(#93883,#93884),(#93885,#93886),(#93887,#93888),
(#93889,#93890),(#93891,#93892),(#93893,#93894),(#93895,#93896),(#93897,
#93898),(#93899,#93900),(#93901,#93902),(#93903,#93904),(#93905,#93906),
(#93907,#93908),(#93909,#93910),(#93911,#93912),(#93913,#93914),(#93915,
#93916),(#93917,#93918),(#93919,#93920),(#93921,#93922),(#93923,#93924),
(#93925,#93926),(#93927,#93928),(#93929,#93930),(#93931,#93932),(#93933,
#93934),(#93935,#93936),(#93937,#93938),(#93939,#93940),(#93941,#93942),
(#93943,#93944),(#93945,#93946),(#93947,#93948),(#93949,#93950),(#93951,
#93952),(#93953,#93954),(#93955,#93956),(#93957,#93958),(#93959,#93960),
(#93961,#93962),(#93963,#93964),(#93965,#93966),(#93967,#93968),(#93969,
#93970),(#93971,#93972),(#93973,#93974),(#93975,#93976),(#93977,#93978),
(#93979,#93980),(#93981,#93982),(#93983,#93984),(#93985,#93986),(#93987,
#93988),(#93989,#93990),(#93991,#93992),(#93993,#93994),(#93995,#93996),
(#93997,#93998),(#93999,#94000),(#94001,#94002),(#94003,#94004),(#94005,
#94006),(#94007,#94008),(#94009,#94010),(#94011,#94012),(#94013,#94014),
(#94015,#94016),(#94017,#94018),(#94019,#94020),(#94021,#94022),(#94023,
#94024),(#94025,#94026),(#94027,#94028),(#94029,#94030),(#94031,#94032),
(#94033,#94034),(#94035,#94036),(#94037,#94038),(#94039,#94040),(#94041,
#94042),(#94043,#94044),(#94045,#94046),(#94047,#94048),(#94049,#94050),
(#94051,#94052),(#94053,#94054),(#94055,#94056),(#94057,#94058),(#94059,
#94060),(#94061,#94062),(#94063,#94064),(#94065,#94066),(#94067,#94068),
(#94069,#94070),(#94071,#94072),(#94073,#94074),(#94075,#94076),(#94077,
#94078),(#94079,#94080),(#94081,#94082),(#94083,#94084),(#94085,#94086),
(#94087,#94088),(#94089,#94090),(#94091,#94092),(#94093,#94094),(#94095,
#94096),(#94097,#94098),(#94099,#94100),(#94101,#94102),(#94103,#94104),
(#94105,#94106),(#94107,#94108),(#94109,#94110),(#94111,#94112),(#94113,
#94114),(#94115,#94116),(#94117,#94118),(#94119,#94120),(#94121,#94122),
(#94123,#94124),(#94125,#94126),(#94127,#94128),(#94129,#94130),(#94131,
#94132),(#94133,#94134),(#94135,#94136),(#94137,#94138),(#94139,#94140),
(#94141,#94142),(#94143,#94144),(#94145,#94146),(#94147,#94148),(#94149,
#94150),(#94151,#94152),(#94153,#94154),(#94155,#94156),(#94157,#94158),
(#94159,#94160),(#94161,#94162),(#94163,#94164),(#94165,#94166),(#94167,
#94168),(#94169,#94170),(#94171,#94172),(#94173,#94174),(#94175,#94176),
(#94177,#94178),(#94179,#94180),(#94181,#94182),(#94183,#94184),(#94185,
#94186),(#94187,#94188),(#94189,#94190),(#94191,#94192),(#94193,#94194),
(#94195,#94196),(#94197,#94198),(#94199,#94200),(#94201,#94202),(#94203,
#94204),(#94205,#94206),(#94207,#94208),(#94209,#94210),(#94211,#94212),
(#94213,#94214),(#94215,#94216),(#94217,#94218),(#94219,#94220),(#94221,
#94222),(#94223,#94224),(#94225,#94226),(#94227,#94228),(#94229,#94230),
(#94231,#94232),(#94233,#94234),(#94235,#94236),(#94237,#94238),(#94239,
#94240),(#94241,#94242),(#94243,#94244),(#94245,#94246),(#94247,#94248),
(#94249,#94250),(#94251,#94252),(#94253,#94254),(#94255,#94256),(#94257,
#94258),(#94259,#94260),(#94261,#94262),(#94263,#94264),(#94265,#94266),
(#94267,#94268),(#94269,#94270),(#94271,#94272),(#94273,#94274),(#94275,
#94276),(#94277,#94278),(#94279,#94280),(#94281,#94282),(#94283,#94284),
(#94285,#94286),(#94287,#94288),(#94289,#94290),(#94291,#94292),(#94293,
#94294),(#94295,#94296),(#94297,#94298),(#94299,#94300),(#94301,#94302),
(#94303,#94304),(#94305,#94306),(#94307,#94308),(#94309,#94310),(#94311,
#94312),(#94313,#94314),(#94315,#94316),(#94317,#94318),(#94319,#94320),
(#94321,#94322),(#94323,#94324),(#94325,#94326),(#94327,#94328),(#94329,
#94330),(#94331,#94332),(#94333,#94334),(#94335,#94336),(#94337,#94338),
(#94339,#94340),(#94341,#94342),(#94343,#94344),(#94345,#94346),(#94347,
#94348),(#94349,#94350),(#94351,#94352),(#94353,#94354),(#94355,#94356),
(#94357,#94358),(#94359,#94360),(#94361,#94362),(#94363,#94364),(#94365,
#94366),(#94367,#94368),(#94369,#94370),(#94371,#94372),(#94373,#94374),
(#94375,#94376),(#94377,#94378),(#94379,#94380),(#94381,#94382),(#94383,
#94384),(#94385,#94386),(#94387,#94388),(#94389,#94390),(#94391,#94392),
(#94393,#94394),(#94395,#94396),(#94397,#94398),(#94399,#94400),(#94401,
#94402),(#94403,#94404),(#94405,#94406),(#94407,#94408),(#94409,#94410),
(#94411,#94412),(#94413,#94414),(#94415,#94416),(#94417,#94418),(#94419,
#94420),(#94421,#94422),(#94423,#94424),(#94425,#94426),(#94427,#94428),
(#94429,#94430),(#94431,#94432),(#94433,#94434),(#94435,#94436),(#94437,
#94438),(#94439,#94440),(#94441,#94442)),.UNSPECIFIED.,.F.,.F.,.F.)
B_SPLINE_SURFACE_WITH_KNOTS((6,1,1,1,1,1,1,1,1,1,1,1,1,1,1,1,1,1,1,1,1,
1,1,1,1,1,1,1,1,1,1,1,1,1,1,1,1,1,1,1,1,1,1,1,1,1,1,1,1,1,1,1,1,1,1,1,1,
1,1,1,1,1,1,1,1,1,1,1,1,1,1,1,1,1,1,1,1,1,1,1,1,1,1,1,1,1,1,1,1,1,1,1,1,
1,1,1,1,1,1,1,1,1,1,1,1,1,1,1,1,1,1,1,1,1,1,1,1,1,1,1,1,1,1,1,1,1,1,1,1,
1,1,1,1,1,1,1,1,1,1,1,1,1,1,1,1,1,1,1,1,1,1,1,1,1,1,1,1,1,1,1,1,1,1,1,1,
1,1,1,1,1,1,1,1,1,1,1,1,1,1,1,1,1,1,1,1,1,1,1,1,1,1,1,1,1,1,1,1,1,1,1,1,
1,1,1,1,1,1,1,1,1,1,1,1,1,1,1,1,1,1,1,1,1,1,1,1,1,1,1,1,1,1,1,1,1,1,1,1,
1,1,1,1,1,1,1,1,1,1,1,1,1,1,1,1,1,1,1,1,1,1,1,1,1,1,1,1,1,1,1,1,1,1,1,1,
1,1,1,1,1,1,1,1,1,1,1,1,1,1,1,1,1,1,1,1,1,1,1,1,1,1,1,1,1,1,1,1,1,1,1,1,
1,1,1,1,1,1,1,1,1,1,1,1,1,1,1,1,1,1,1,1,1,1,1,1,1,1,1,1,1,1,1,1,1,1,1,1,
1,1,1,1,1,1,1,1,1,1,1,1,1,1,1,1,1,1,1,1,1,1,1,1,1,1,1,1,1,1,1,1,1,1,1,1,
1,1,1,1,1,1,1,1,1,1,1,1,1,1,1,1,1,1,1,1,1,1,1,1,1,1,1,1,1,1,1,1,1,1,1,1,
1,1,1,1,1,1,1,1,1,1,1,1,1,1,1,1,1,1,1,1,1,1,1,1,1,1,1,1,1,1,1,1,1,1,1,1,
1,1,1,1,1,1,1,1,1,1,1,1,1,1,1,1,1,1,1,1,1,1,1,1,1,1,1,1,1,1,1,1,1,1,1,1,
1,1,1,1,1,1,1,1,1,1,1,1,1,1,1,1,1,1,1,1,1,1,1,1,1,1,1,1,1,1,1,1,1,1,1,1,
1,1,1,1,1,1,1,1,1,1,1,1,1,1,1,1,1,1,1,1,1,1,1,1,1,1,1,1,1,1,1,1,1,1,1,1,
1,1,1,1,1,1,1,1,1,1,1,1,1,1,1,1,1,1,1,1,1,1,1,1,1,1,1,1,1,1,1,1,1,1,1,1,
1,1,1,1,1,1,1,1,1,1,1,1,1,1,1,1,1,1,1,1,1,1,1,1,1,1,1,1,1,1,1,1,1,1,1,1,
1,1,1,1,1,1,1,1,1,1,1,1,1,1,1,1,1,1,1,1,1,1,1,1,1,1,1,1,1,1,1,1,1,1,1,1,
1,1,1,1,1,1,1,1,1,1,1,1,1,1,1,1,1,1,1,1,1,1,1,1,1,1,1,1,1,1,1,1,1,1,1,1,
1,1,1,1,1,1,1,1,1,1,1,1,1,1,1,1,1,1,1,1,1,1,1,1,1,1,1,1,1,1,1,1,1,1,1,1,
1,1,1,1,1,1,1,1,1,1,1,1,1,1,1,1,1,1,1,1,1,1,1,1,1,1,1,1,1,1,1,1,1,1,1,1,
1,1,1,1,1,1,1,1,1,1,1,1,1,1,1,1,1,1,1,1,1,1,1,1,1,1,1,1,1,1,1,1,1,1,1,1,
1,1,1,1,1,1,1,1,1,1,1,1,1,1,1,1,1,1,1,1,1,1,1,1,1,1,1,1,1,1,1,1,1,1,1,1,
1,1,1,1,1,1,1,1,1,1,1,1,1,1,1,1,1,1,1,1,1,1,1,1,1,1,1,1,1,1,1,1,1,1,1,1,
1,1,1,1,1,1,1,1,1,1,1,1,1,1,1,1,1,1,1,1,1,1,1,1,1,1,1,1,1,1,1,1,1,1,1,1,
1,1,1,1,1,1,1,1,1,1,1,1,1,1,1,1,1,1,1,1,1,1,1,1,1,1,1,1,1,1,1,1,1,1,1,1,
1,1,1,1,1,1,1,1,1,1,1,1,1,1,1,1,1,1,1,1,1,1,1,1,1,1,1,1,1,1,1,1,1,1,1,1,
1,1,1,1,1,1,1,6),(2,2),(-1.,-0.999000000000001,-0.998000000000001,-0.997000000000001,
-0.996000000000001,-0.995000000000001,-0.994000000000001,-0.993000000000001,
-0.992000000000001,-0.991000000000001,-0.990000000000001,-0.989000000000001,
-0.988000000000001,-0.987000000000001,-0.986000000000001,-0.985000000000001,
-0.984000000000001,-0.983000000000001,-0.982000000000001,-0.981000000000001,
-0.980000000000001,-0.979000000000001,-0.978000000000001,-0.977000000000001,
-0.976000000000001,-0.975000000000001,-0.974000000000001,-0.973000000000001,
-0.972000000000001,-0.971000000000001,-0.970000000000001,-0.969000000000001,
-0.968000000000001,-0.967000000000001,-0.966000000000001,-0.965000000000001,
-0.964000000000001,-0.963000000000001,-0.962000000000001,-0.961000000000001,
-0.960000000000001,-0.959000000000001,-0.958000000000001,-0.957000000000001,
-0.956000000000001,-0.955000000000001,-0.954000000000001,-0.953000000000001,
-0.952000000000001,-0.951000000000001,-0.950000000000001,-0.949000000000001,
-0.948000000000001,-0.947000000000001,-0.946000000000001,-0.945000000000001,
-0.944000000000001,-0.943000000000001,-0.942000000000001,-0.941000000000001,
-0.940000000000001,-0.939000000000001,-0.938000000000001,-0.937000000000001,
-0.936000000000001,-0.935000000000001,-0.934000000000001,-0.933000000000001,
-0.932000000000001,-0.931000000000001,-0.930000000000001,-0.929000000000001,
-0.928000000000001,-0.927000000000001,-0.926000000000001,-0.925000000000001,
-0.924000000000001,-0.923000000000001,-0.922000000000001,-0.921000000000001,
-0.920000000000001,-0.919000000000001,-0.918000000000001,-0.917000000000001,
-0.916000000000001,-0.915000000000001,-0.914000000000001,-0.913000000000001,
-0.912000000000001,-0.911000000000001,-0.910000000000001,-0.909000000000001,
-0.908000000000001,-0.907000000000001,-0.906000000000001,-0.905000000000001,
-0.904000000000001,-0.903000000000001,-0.902000000000001,-0.901000000000001,
-0.900000000000001,-0.899000000000001,-0.898000000000001,-0.897000000000001,
-0.896000000000001,-0.895000000000001,-0.894000000000001,-0.893000000000001,
-0.892000000000001,-0.891000000000001,-0.890000000000001,-0.889000000000001,
-0.888000000000001,-0.887000000000001,-0.886000000000001,-0.885000000000001,
-0.884000000000001,-0.883000000000001,-0.882000000000001,-0.881000000000001,
-0.880000000000001,-0.879000000000001,-0.878000000000001,-0.877000000000001,
-0.876000000000001,-0.875000000000001,-0.874000000000001,-0.873000000000001,
-0.872000000000001,-0.871000000000001,-0.870000000000001,-0.869000000000001,
-0.868000000000001,-0.867000000000001,-0.866000000000001,-0.865000000000001,
-0.864000000000001,-0.863000000000001,-0.862000000000001,-0.861000000000001,
-0.860000000000001,-0.859000000000001,-0.858000000000001,-0.857000000000001,
-0.856000000000001,-0.855000000000001,-0.854000000000001,-0.853000000000001,
-0.852000000000001,-0.851000000000001,-0.850000000000001,-0.849000000000001,
-0.848000000000001,-0.847000000000001,-0.846000000000001,-0.845000000000001,
-0.844000000000001,-0.843000000000001,-0.842000000000001,-0.841000000000001,
-0.840000000000001,-0.839000000000001,-0.838000000000001,-0.837000000000001,
-0.836000000000001,-0.835000000000001,-0.834000000000001,-0.833000000000001,
-0.832000000000001,-0.831000000000001,-0.830000000000001,-0.829000000000001,
-0.828000000000001,-0.827000000000001,-0.826000000000001,-0.825000000000001,
-0.824000000000001,-0.823000000000001,-0.822000000000001,-0.821000000000001,
-0.820000000000001,-0.819000000000001,-0.818000000000001,-0.817000000000001,
-0.816000000000001,-0.815000000000001,-0.814000000000001,-0.813000000000001,
-0.812000000000001,-0.811000000000001,-0.810000000000001,-0.809000000000001,
-0.808000000000001,-0.807000000000001,-0.806000000000001,-0.805000000000001,
-0.804000000000001,-0.803000000000001,-0.802000000000001,-0.801000000000001,
-0.800000000000001,-0.799000000000001,-0.798000000000001,-0.797000000000001,
-0.796000000000001,-0.795000000000001,-0.794000000000001,-0.793000000000001,
-0.792000000000001,-0.791000000000001,-0.790000000000001,-0.789000000000001,
-0.788000000000001,-0.787000000000001,-0.786000000000001,-0.785000000000001,
-0.784000000000001,-0.783000000000001,-0.782000000000001,-0.781000000000001,
-0.780000000000001,-0.779000000000001,-0.778000000000001,-0.777000000000001,
-0.776000000000001,-0.775000000000001,-0.774000000000001,-0.773000000000001,
-0.772000000000001,-0.771000000000001,-0.770000000000001,-0.769000000000001,
-0.768000000000001,-0.767000000000001,-0.766000000000001,-0.765000000000001,
-0.764000000000001,-0.763000000000001,-0.762000000000001,-0.761000000000001,
-0.760000000000001,-0.759000000000001,-0.758000000000001,-0.757000000000001,
-0.756000000000001,-0.755000000000001,-0.754000000000001,-0.753000000000001,
-0.752000000000001,-0.751000000000001,-0.750000000000001,-0.749000000000001,
-0.748000000000001,-0.747000000000001,-0.746000000000001,-0.745000000000001,
-0.744000000000001,-0.743000000000001,-0.742000000000001,-0.741000000000001,
-0.740000000000001,-0.739000000000001,-0.738000000000001,-0.737000000000001,
-0.736000000000001,-0.735000000000001,-0.734000000000001,-0.733000000000001,
-0.732000000000001,-0.731000000000001,-0.730000000000001,-0.729000000000001,
-0.728000000000001,-0.727000000000001,-0.726000000000001,-0.725000000000001,
-0.724000000000001,-0.723000000000001,-0.722000000000001,-0.721000000000001,
-0.720000000000001,-0.719000000000001,-0.718000000000001,-0.717000000000001,
-0.716000000000001,-0.715000000000001,-0.714000000000001,-0.713000000000001,
-0.712000000000001,-0.711000000000001,-0.710000000000001,-0.709000000000001,
-0.708000000000001,-0.707000000000001,-0.706000000000001,-0.705000000000001,
-0.704000000000001,-0.703000000000001,-0.702000000000001,-0.701000000000001,
-0.700000000000001,-0.699000000000001,-0.698000000000001,-0.697000000000001,
-0.696000000000001,-0.695000000000001,-0.694000000000001,-0.693000000000001,
-0.692000000000001,-0.691000000000001,-0.690000000000001,-0.689000000000001,
-0.688000000000001,-0.687,-0.686,-0.685,-0.684,-0.683,-0.682,-0.681,-0.68,
-0.679,-0.678,-0.677,-0.676,-0.675,-0.674,-0.673,-0.672,-0.671,-0.67,-0.669,
-0.668,-0.667,-0.666,-0.665,-0.664,-0.663,-0.662,-0.661,-0.66,-0.659,-0.658,
-0.657,-0.656,-0.655,-0.654,-0.653,-0.652,-0.651,-0.65,-0.649,-0.648,-0.647,
-0.646,-0.645,-0.644,-0.643,-0.642,-0.641,-0.64,-0.639,-0.638,-0.637,-0.636,
-0.635,-0.634,-0.633,-0.632,-0.631,-0.63,-0.629,-0.628,-0.627,-0.626,-0.625,
-0.624,-0.623,-0.622,-0.621,-0.62,-0.619,-0.618,-0.617,-0.616,-0.615,-0.614,
-0.613,-0.612,-0.611,-0.61,-0.609,-0.608,-0.607,-0.606,-0.605,-0.604,-0.603,
-0.602,-0.601,-0.6,-0.599,-0.598,-0.597,-0.596,-0.595,-0.594,-0.593,-0.592,
-0.591,-0.59,-0.589,-0.588,-0.587,-0.586,-0.585,-0.584,-0.583,-0.582,-0.581,
-0.58,-0.579,-0.578,-0.577,-0.576,-0.575,-0.574,-0.573,-0.572,-0.571,-0.57,
-0.569,-0.568,-0.567,-0.566,-0.565,-0.564,-0.563,-0.562,-0.561,-0.56,-0.559,
-0.558,-0.557,-0.556,-0.555,-0.554,-0.553,-0.552,-0.551,-0.55,-0.549,-0.548,
-0.547,-0.546,-0.545,-0.544,-0.543,-0.542,-0.541,-0.54,-0.539,-0.538,-0.537,
-0.536,-0.535,-0.534,-0.533,-0.532,-0.531,-0.53,-0.529,-0.528,-0.527,-0.526,
-0.525,-0.524,-0.523,-0.522,-0.521,-0.52,-0.519,-0.518,-0.517,-0.516,-0.515,
-0.514,-0.513,-0.512,-0.511,-0.51,-0.509,-0.508,-0.507,-0.506,-0.505,-0.504,
-0.503,-0.502,-0.501,-0.5,-0.499,-0.498,-0.497,-0.496,-0.495,-0.494,-0.493,
-0.492,-0.491,-0.49,-0.489,-0.488,-0.487,-0.486,-0.485,-0.484,-0.483,-0.482,
-0.481,-0.48,-0.479,-0.478,-0.477,-0.476,-0.475,-0.474,-0.473,-0.472,-0.471,
-0.47,-0.469,-0.468,-0.467,-0.466,-0.465,-0.464,-0.463,-0.462,-0.461,-0.46,
-0.459,-0.458,-0.457,-0.456,-0.455,-0.454,-0.453,-0.452,-0.451,-0.45,-0.449,
-0.448,-0.447,-0.446,-0.445,-0.444,-0.443,-0.442,-0.441,-0.44,-0.439,-0.438,
-0.437,-0.436,-0.435,-0.434,-0.433,-0.432,-0.431,-0.43,-0.429,-0.428,-0.427,
-0.426,-0.425,-0.424,-0.423,-0.422,-0.421,-0.42,-0.419,-0.418,-0.417,-0.416,
-0.415,-0.414,-0.413,-0.412,-0.411,-0.41,-0.409,-0.408,-0.407,-0.406,-0.405,
-0.404,-0.403,-0.402,-0.401,-0.4,-0.399,-0.398,-0.397,-0.396,-0.395,-0.394,
-0.393,-0.392,-0.391,-0.39,-0.389,-0.388,-0.387,-0.386,-0.385,-0.384,-0.383,
-0.382,-0.381,-0.38,-0.379,-0.378,-0.377,-0.376,-0.375,-0.374,-0.373,-0.372,
-0.371,-0.37,-0.369,-0.368,-0.367,-0.366,-0.365,-0.364,-0.363,-0.362,-0.361,
-0.36,-0.359,-0.358,-0.357,-0.356,-0.355,-0.354,-0.353,-0.352,-0.351,-0.35,
-0.349,-0.348,-0.347,-0.346,-0.345,-0.344,-0.343,-0.342,-0.341,-0.34,-0.339,
-0.338,-0.337,-0.336,-0.335,-0.334,-0.333,-0.332,-0.331,-0.33,-0.329,-0.328,
-0.327,-0.326,-0.325,-0.324,-0.323,-0.322,-0.321,-0.32,-0.319,-0.318,-0.317,
-0.316,-0.315,-0.314,-0.313,-0.312,-0.311,-0.31,-0.309,-0.308,-0.307,-0.306,
-0.305,-0.304,-0.303,-0.302,-0.301,-0.3,-0.299,-0.298,-0.297,-0.296,-0.295,
-0.294,-0.293,-0.292,-0.291,-0.29,-0.289,-0.288,-0.287,-0.286,-0.285,-0.284,
-0.283,-0.282,-0.281,-0.28,-0.279,-0.278,-0.277,-0.276,-0.275,-0.274,-0.273,
-0.272,-0.271,-0.27,-0.269,-0.268,-0.267,-0.266,-0.265,-0.264,-0.263,-0.262,
-0.261,-0.26,-0.259,-0.258,-0.257,-0.256,-0.255,-0.254,-0.253,-0.252,-0.251,
-0.25,-0.249,-0.248,-0.247,-0.246,-0.245,-0.244,-0.243,-0.242,-0.241,-0.24,
-0.239,-0.238,-0.237,-0.236,-0.235,-0.234,-0.233,-0.232,-0.231,-0.23,-0.229,
-0.228,-0.227,-0.226,-0.225,-0.224,-0.223,-0.222,-0.221,-0.22,-0.219,-0.218,
-0.217,-0.216,-0.215,-0.214,-0.213,-0.212,-0.211,-0.21,-0.209,-0.208,-0.207,
-0.206,-0.205,-0.204,-0.203,-0.202,-0.201,-0.2,-0.199,-0.198,-0.197,-0.196,
-0.195,-0.194,-0.193,-0.192,-0.191,-0.19,-0.189,-0.188,-0.187,-0.186,-0.185,
-0.184,-0.183,-0.182,-0.181,-0.18,-0.179,-0.178,-0.177,-0.176,-0.175,-0.174,
-0.173,-0.172,-0.171,-0.17,-0.169,-0.168,-0.167,-0.166,-0.165,-0.164,-0.163,
-0.162,-0.161,-0.16,-0.159,-0.158,-0.157,-0.156,-0.155,-0.154,-0.153,-0.152,
-0.151,-0.15,-0.149,-0.148,-0.147,-0.146,-0.145,-0.144,-0.143,-0.142,-0.141,
-0.14,-0.139,-0.138,-0.137,-0.136,-0.135,-0.134,-0.133,-0.132,-0.131,-0.13,
-0.129,-0.128,-0.127,-0.126,-0.125,-0.124,-0.123,-0.122,-0.121,-0.12,-0.119,
-0.118,-0.117,-0.116,-0.115,-0.114,-0.113,-0.112,-0.111,-0.11,-0.109,-0.108,
-0.107,-0.106,-0.105,-0.104,-0.103,-0.102,-0.101,-0.1,-0.0990000000000001,
-0.0980000000000001,-0.0970000000000001,-0.0960000000000001,-0.0950000000000001,
-0.0940000000000001,-0.0930000000000001,-0.0920000000000001,-0.0910000000000001,
-0.0900000000000001,-0.0890000000000001,-0.0880000000000001,-0.0870000000000001,
-0.0860000000000001,-0.0850000000000001,-0.0840000000000001,-0.0830000000000001,
-0.0820000000000001,-0.0810000000000001,-0.0800000000000001,-0.0790000000000001,
-0.0780000000000001,-0.0770000000000001,-0.0760000000000001,-0.0750000000000001,
-0.0740000000000001,-0.0730000000000001,-0.0720000000000001,-0.071,-0.07,
-0.069,-0.068,-0.067,-0.066,-0.065,-0.064,-0.063,-0.062,-0.061,-0.06,-0.059,
-0.058,-0.057,-0.056,-0.055,-0.054,-0.053,-0.052,-0.051,-0.05,-0.049,-0.048,
-0.047,-0.046,-0.045,-0.044,-0.043,-0.042,-0.041,-0.04,-0.039,-0.038,-0.037,
-0.036,-0.035,-0.034,-0.033,-0.032,-0.031,-0.03,-0.029,-0.028,-0.027,-0.026,
-0.025,-0.024,-0.023,-0.022,-0.021,-0.02,-0.019,-0.018,-0.017,-0.016,-0.015,
-0.014,-0.013,-0.012,-0.011,-0.01,-0.009,-0.008,-0.007,-0.006,-0.005,-0.004,
-0.003,-0.002,-0.001,0.),(0.,2.),.UNSPECIFIED.)
GEOMETRIC_REPRESENTATION_ITEM()
RATIONAL_B_SPLINE_SURFACE(((1.,1.),(1.,1.),(1.,1.),(1.,1.),(1.,1.),(1.,
1.),(1.,1.),(1.,1.),(1.,1.),(1.,1.),(1.,1.),(1.,1.),(1.,1.),(1.,1.),(1.,
1.),(1.,1.),(1.,1.),(1.,1.),(1.,1.),(1.,1.),(1.,1.),(1.,1.),(1.,1.),(1.,
1.),(1.,1.),(1.,1.),(1.,1.),(1.,1.),(1.,1.),(1.,1.),(1.,1.),(1.,1.),(1.,
1.),(1.,1.),(1.,1.),(1.,1.),(1.,1.),(1.,1.),(1.,1.),(1.,1.),(1.,1.),(1.,
1.),(1.,1.),(1.,1.),(1.,1.),(1.,1.),(1.,1.),(1.,1.),(1.,1.),(1.,1.),(1.,
1.),(1.,1.),(1.,1.),(1.,1.),(1.,1.),(1.,1.),(1.,1.),(1.,1.),(1.,1.),(1.,
1.),(1.,1.),(1.,1.),(1.,1.),(1.,1.),(1.,1.),(1.,1.),(1.,1.),(1.,1.),(1.,
1.),(1.,1.),(1.,1.),(1.,1.),(1.,1.),(1.,1.),(1.,1.),(1.,1.),(1.,1.),(1.,
1.),(1.,1.),(1.,1.),(1.,1.),(1.,1.),(1.,1.),(1.,1.),(1.,1.),(1.,1.),(1.,
1.),(1.,1.),(1.,1.),(1.,1.),(1.,1.),(1.,1.),(1.,1.),(1.,1.),(1.,1.),(1.,
1.),(1.,1.),(1.,1.),(1.,1.),(1.,1.),(1.,1.),(1.,1.),(1.,1.),(1.,1.),(1.,
1.),(1.,1.),(1.,1.),(1.,1.),(1.,1.),(1.,1.),(1.,1.),(1.,1.),(1.,1.),(1.,
1.),(1.,1.),(1.,1.),(1.,1.),(1.,1.),(1.,1.),(1.,1.),(1.,1.),(1.,1.),(1.,
1.),(1.,1.),(1.,1.),(1.,1.),(1.,1.),(1.,1.),(1.,1.),(1.,1.),(1.,1.),(1.,
1.),(1.,1.),(1.,1.),(1.,1.),(1.,1.),(1.,1.),(1.,1.),(1.,1.),(1.,1.),(1.,
1.),(1.,1.),(1.,1.),(1.,1.),(1.,1.),(1.,1.),(1.,1.),(1.,1.),(1.,1.),(1.,
1.),(1.,1.),(1.,1.),(1.,1.),(1.,1.),(1.,1.),(1.,1.),(1.,1.),(1.,1.),(1.,
1.),(1.,1.),(1.,1.),(1.,1.),(1.,1.),(1.,1.),(1.,1.),(1.,1.),(1.,1.),(1.,
1.),(1.,1.),(1.,1.),(1.,1.),(1.,1.),(1.,1.),(1.,1.),(1.,1.),(1.,1.),(1.,
1.),(1.,1.),(1.,1.),(1.,1.),(1.,1.),(1.,1.),(1.,1.),(1.,1.),(1.,1.),(1.,
1.),(1.,1.),(1.,1.),(1.,1.),(1.,1.),(1.,1.),(1.,1.),(1.,1.),(1.,1.),(1.,
1.),(1.,1.),(1.,1.),(1.,1.),(1.,1.),(1.,1.),(1.,1.),(1.,1.),(1.,1.),(1.,
1.),(1.,1.),(1.,1.),(1.,1.),(1.,1.),(1.,1.),(1.,1.),(1.,1.),(1.,1.),(1.,
1.),(1.,1.),(1.,1.),(1.,1.),(1.,1.),(1.,1.),(1.,1.),(1.,1.),(1.,1.),(1.,
1.),(1.,1.),(1.,1.),(1.,1.),(1.,1.),(1.,1.),(1.,1.),(1.,1.),(1.,1.),(1.,
1.),(1.,1.),(1.,1.),(1.,1.),(1.,1.),(1.,1.),(1.,1.),(1.,1.),(1.,1.),(1.,
1.),(1.,1.),(1.,1.),(1.,1.),(1.,1.),(1.,1.),(1.,1.),(1.,1.),(1.,1.),(1.,
1.),(1.,1.),(1.,1.),(1.,1.),(1.,1.),(1.,1.),(1.,1.),(1.,1.),(1.,1.),(1.,
1.),(1.,1.),(1.,1.),(1.,1.),(1.,1.),(1.,1.),(1.,1.),(1.,1.),(1.,1.),(1.,
1.),(1.,1.),(1.,1.),(1.,1.),(1.,1.),(1.,1.),(1.,1.),(1.,1.),(1.,1.),(1.,
1.),(1.,1.),(1.,1.),(1.,1.),(1.,1.),(1.,1.),(1.,1.),(1.,1.),(1.,1.),(1.,
1.),(1.,1.),(1.,1.),(1.,1.),(1.,1.),(1.,1.),(1.,1.),(1.,1.),(1.,1.),(1.,
1.),(1.,1.),(1.,1.),(1.,1.),(1.,1.),(1.,1.),(1.,1.),(1.,1.),(1.,1.),(1.,
1.),(1.,1.),(1.,1.),(1.,1.),(1.,1.),(1.,1.),(1.,1.),(1.,1.),(1.,1.),(1.,
1.),(1.,1.),(1.,1.),(1.,1.),(1.,1.),(1.,1.),(1.,1.),(1.,1.),(1.,1.),(1.,
1.),(1.,1.),(1.,1.),(1.,1.),(1.,1.),(1.,1.),(1.,1.),(1.,1.),(1.,1.),(1.,
1.),(1.,1.),(1.,1.),(1.,1.),(1.,1.),(1.,1.),(1.,1.),(1.,1.),(1.,1.),(1.,
1.),(1.,1.),(1.,1.),(1.,1.),(1.,1.),(1.,1.),(1.,1.),(1.,1.),(1.,1.),(1.,
1.),(1.,1.),(1.,1.),(1.,1.),(1.,1.),(1.,1.),(1.,1.),(1.,1.),(1.,1.),(1.,
1.),(1.,1.),(1.,1.),(1.,1.),(1.,1.),(1.,1.),(1.,1.),(1.,1.),(1.,1.),(1.,
1.),(1.,1.),(1.,1.),(1.,1.),(1.,1.),(1.,1.),(1.,1.),(1.,1.),(1.,1.),(1.,
1.),(1.,1.),(1.,1.),(1.,1.),(1.,1.),(1.,1.),(1.,1.),(1.,1.),(1.,1.),(1.,
1.),(1.,1.),(1.,1.),(1.,1.),(1.,1.),(1.,1.),(1.,1.),(1.,1.),(1.,1.),(1.,
1.),(1.,1.),(1.,1.),(1.,1.),(1.,1.),(1.,1.),(1.,1.),(1.,1.),(1.,1.),(1.,
1.),(1.,1.),(1.,1.),(1.,1.),(1.,1.),(1.,1.),(1.,1.),(1.,1.),(1.,1.),(1.,
1.),(1.,1.),(1.,1.),(1.,1.),(1.,1.),(1.,1.),(1.,1.),(1.,1.),(1.,1.),(1.,
1.),(1.,1.),(1.,1.),(1.,1.),(1.,1.),(1.,1.),(1.,1.),(1.,1.),(1.,1.),(1.,
1.),(1.,1.),(1.,1.),(1.,1.),(1.,1.),(1.,1.),(1.,1.),(1.,1.),(1.,1.),(1.,
1.),(1.,1.),(1.,1.),(1.,1.),(1.,1.),(1.,1.),(1.,1.),(1.,1.),(1.,1.),(1.,
1.),(1.,1.),(1.,1.),(1.,1.),(1.,1.),(1.,1.),(1.,1.),(1.,1.),(1.,1.),(1.,
1.),(1.,1.),(1.,1.),(1.,1.),(1.,1.),(1.,1.),(1.,1.),(1.,1.),(1.,1.),(1.,
1.),(1.,1.),(1.,1.),(1.,1.),(1.,1.),(1.,1.),(1.,1.),(1.,1.),(1.,1.),(1.,
1.),(1.,1.),(1.,1.),(1.,1.),(1.,1.),(1.,1.),(1.,1.),(1.,1.),(1.,1.),(1.,
1.),(1.,1.),(1.,1.),(1.,1.),(1.,1.),(1.,1.),(1.,1.),(1.,1.),(1.,1.),(1.,
1.),(1.,1.),(1.,1.),(1.,1.),(1.,1.),(1.,1.),(1.,1.),(1.,1.),(1.,1.),(1.,
1.),(1.,1.),(1.,1.),(1.,1.),(1.,1.),(1.,1.),(1.,1.),(1.,1.),(1.,1.),(1.,
1.),(1.,1.),(1.,1.),(1.,1.),(1.,1.),(1.,1.),(1.,1.),(1.,1.),(1.,1.),(1.,
1.),(1.,1.),(1.,1.),(1.,1.),(1.,1.),(1.,1.),(1.,1.),(1.,1.),(1.,1.),(1.,
1.),(1.,1.),(1.,1.),(1.,1.),(1.,1.),(1.,1.),(1.,1.),(1.,1.),(1.,1.),(1.,
1.),(1.,1.),(1.,1.),(1.,1.),(1.,1.),(1.,1.),(1.,1.),(1.,1.),(1.,1.),(1.,
1.),(1.,1.),(1.,1.),(1.,1.),(1.,1.),(1.,1.),(1.,1.),(1.,1.),(1.,1.),(1.,
1.),(1.,1.),(1.,1.),(1.,1.),(1.,1.),(1.,1.),(1.,1.),(1.,1.),(1.,1.),(1.,
1.),(1.,1.),(1.,1.),(1.,1.),(1.,1.),(1.,1.),(1.,1.),(1.,1.),(1.,1.),(1.,
1.),(1.,1.),(1.,1.),(1.,1.),(1.,1.),(1.,1.),(1.,1.),(1.,1.),(1.,1.),(1.,
1.),(1.,1.),(1.,1.),(1.,1.),(1.,1.),(1.,1.),(1.,1.),(1.,1.),(1.,1.),(1.,
1.),(1.,1.),(1.,1.),(1.,1.),(1.,1.),(1.,1.),(1.,1.),(1.,1.),(1.,1.),(1.,
1.),(1.,1.),(1.,1.),(1.,1.),(1.,1.),(1.,1.),(1.,1.),(1.,1.),(1.,1.),(1.,
1.),(1.,1.),(1.,1.),(1.,1.),(1.,1.),(1.,1.),(1.,1.),(1.,1.),(1.,1.),(1.,
1.),(1.,1.),(1.,1.),(1.,1.),(1.,1.),(1.,1.),(1.,1.),(1.,1.),(1.,1.),(1.,
1.),(1.,1.),(1.,1.),(1.,1.),(1.,1.),(1.,1.),(1.,1.),(1.,1.),(1.,1.),(1.,
1.),(1.,1.),(1.,1.),(1.,1.),(1.,1.),(1.,1.),(1.,1.),(1.,1.),(1.,1.),(1.,
1.),(1.,1.),(1.,1.),(1.,1.),(1.,1.),(1.,1.),(1.,1.),(1.,1.),(1.,1.),(1.,
1.),(1.,1.),(1.,1.),(1.,1.),(1.,1.),(1.,1.),(1.,1.),(1.,1.),(1.,1.),(1.,
1.),(1.,1.),(1.,1.),(1.,1.),(1.,1.),(1.,1.),(1.,1.),(1.,1.),(1.,1.),(1.,
1.),(1.,1.),(1.,1.),(1.,1.),(1.,1.),(1.,1.),(1.,1.),(1.,1.),(1.,1.),(1.,
1.),(1.,1.),(1.,1.),(1.,1.),(1.,1.),(1.,1.),(1.,1.),(1.,1.),(1.,1.),(1.,
1.),(1.,1.),(1.,1.),(1.,1.),(1.,1.),(1.,1.),(1.,1.),(1.,1.),(1.,1.),(1.,
1.),(1.,1.),(1.,1.),(1.,1.),(1.,1.),(1.,1.),(1.,1.),(1.,1.),(1.,1.),(1.,
1.),(1.,1.),(1.,1.),(1.,1.),(1.,1.),(1.,1.),(1.,1.),(1.,1.),(1.,1.),(1.,
1.),(1.,1.),(1.,1.),(1.,1.),(1.,1.),(1.,1.),(1.,1.),(1.,1.),(1.,1.),(1.,
1.),(1.,1.),(1.,1.),(1.,1.),(1.,1.),(1.,1.),(1.,1.),(1.,1.),(1.,1.),(1.,
1.),(1.,1.),(1.,1.),(1.,1.),(1.,1.),(1.,1.),(1.,1.),(1.,1.),(1.,1.),(1.,
1.),(1.,1.),(1.,1.),(1.,1.),(1.,1.),(1.,1.),(1.,1.),(1.,1.),(1.,1.),(1.,
1.),(1.,1.),(1.,1.),(1.,1.),(1.,1.),(1.,1.),(1.,1.),(1.,1.),(1.,1.),(1.,
1.),(1.,1.),(1.,1.),(1.,1.),(1.,1.),(1.,1.),(1.,1.),(1.,1.),(1.,1.),(1.,
1.),(1.,1.),(1.,1.),(1.,1.),(1.,1.),(1.,1.),(1.,1.),(1.,1.),(1.,1.),(1.,
1.),(1.,1.),(1.,1.),(1.,1.),(1.,1.),(1.,1.),(1.,1.),(1.,1.),(1.,1.),(1.,
1.),(1.,1.),(1.,1.),(1.,1.),(1.,1.),(1.,1.),(1.,1.),(1.,1.),(1.,1.),(1.,
1.),(1.,1.),(1.,1.),(1.,1.),(1.,1.),(1.,1.),(1.,1.),(1.,1.),(1.,1.),(1.,
1.),(1.,1.),(1.,1.),(1.,1.),(1.,1.),(1.,1.),(1.,1.),(1.,1.),(1.,1.),(1.,
1.),(1.,1.),(1.,1.),(1.,1.),(1.,1.),(1.,1.),(1.,1.),(1.,1.),(1.,1.),(1.,
1.),(1.,1.),(1.,1.),(1.,1.),(1.,1.),(1.,1.),(1.,1.),(1.,1.),(1.,1.),(1.,
1.),(1.,1.),(1.,1.),(1.,1.),(1.,1.),(1.,1.),(1.,1.),(1.,1.),(1.,1.),(1.,
1.),(1.,1.),(1.,1.),(1.,1.),(1.,1.),(1.,1.),(1.,1.),(1.,1.),(1.,1.),(1.,
1.),(1.,1.),(1.,1.),(1.,1.),(1.,1.),(1.,1.),(1.,1.),(1.,1.),(1.,1.),(1.,
1.),(1.,1.),(1.,1.),(1.,1.),(1.,1.),(1.,1.),(1.,1.),(1.,1.),(1.,1.),(1.,
1.),(1.,1.),(1.,1.),(1.,1.),(1.,1.),(1.,1.),(1.,1.),(1.,1.),(1.,1.),(1.,
1.),(1.,1.),(1.,1.),(1.,1.),(1.,1.),(1.,1.),(1.,1.),(1.,1.),(1.,1.),(1.,
1.),(1.,1.),(1.,1.),(1.,1.),(1.,1.),(1.,1.),(1.,1.),(1.,1.),(1.,1.),(1.,
1.),(1.,1.),(1.,1.),(1.,1.),(1.,1.),(1.,1.),(1.,1.),(1.,1.),(1.,1.),(1.,
1.),(1.,1.),(1.,1.),(1.,1.),(1.,1.),(1.,1.),(1.,1.),(1.,1.),(1.,1.),(1.,
1.),(1.,1.),(1.,1.),(1.,1.),(1.,1.),(1.,1.),(1.,1.),(1.,1.),(1.,1.),(1.,
1.),(1.,1.),(1.,1.),(1.,1.),(1.,1.),(1.,1.),(1.,1.),(1.,1.),(1.,1.),(1.,
1.),(1.,1.),(1.,1.),(1.,1.),(1.,1.),(1.,1.),(1.,1.),(1.,1.),(1.,1.),(1.,
1.),(1.,1.),(1.,1.),(1.,1.),(1.,1.),(1.,1.),(1.,1.),(1.,1.),(1.,1.),(1.,
1.),(1.,1.),(1.,1.),(1.,1.),(1.,1.),(1.,1.),(1.,1.),(1.,1.),(1.,1.),(1.,
1.),(1.,1.),(1.,1.),(1.,1.),(1.,1.),(1.,1.),(1.,1.),(1.,1.),(1.,1.),(1.,
1.),(1.,1.),(1.,1.),(1.,1.),(1.,1.),(1.,1.),(1.,1.),(1.,1.),(1.,1.),(1.,
1.),(1.,1.),(1.,1.),(1.,1.),(1.,1.),(1.,1.),(1.,1.),(1.,1.),(1.,1.),(1.,
1.),(1.,1.),(1.,1.),(1.,1.),(1.,1.),(1.,1.),(1.,1.),(1.,1.),(1.,1.),(1.,
1.),(1.,1.),(1.,1.),(1.,1.),(1.,1.),(1.,1.),(1.,1.),(1.,1.),(1.,1.),(1.,
1.)))
REPRESENTATION_ITEM('')
SURFACE()
);
#269=SHAPE_REPRESENTATION_RELATIONSHIP('SRR','None',#99626,#285);
#285=ADVANCED_BREP_SHAPE_REPRESENTATION('',(#317),#99511);
#301=STYLED_ITEM('',(#99715),#317);
#317=MANIFOLD_SOLID_BREP('Gear blank',#18271);
#350=FACE_BOUND('',#2346,.T.);
#351=FACE_BOUND('',#2347,.T.);
#352=FACE_BOUND('',#2348,.T.);
#353=FACE_BOUND('',#2349,.T.);
#354=FACE_BOUND('',#2350,.T.);
#355=FACE_BOUND('',#2351,.T.);
#356=FACE_BOUND('',#2352,.T.);
#357=FACE_BOUND('',#2439,.T.);
#358=FACE_BOUND('',#2441,.T.);
#359=FACE_BOUND('',#2444,.T.);
#360=FACE_BOUND('',#2446,.T.);
#361=FACE_BOUND('',#2449,.T.);
#362=FACE_BOUND('',#2451,.T.);
#363=FACE_BOUND('',#2454,.T.);
#364=FACE_BOUND('',#2456,.T.);
#365=FACE_BOUND('',#2459,.T.);
#366=FACE_BOUND('',#2461,.T.);
#367=FACE_BOUND('',#2464,.T.);
#368=FACE_BOUND('',#2466,.T.);
#369=FACE_BOUND('',#2469,.T.);
#370=FACE_BOUND('',#2472,.T.);
#371=FACE_BOUND('',#2474,.T.);
#372=FACE_BOUND('',#2477,.T.);
#373=FACE_BOUND('',#2480,.T.);
#374=FACE_BOUND('',#2483,.T.);
#375=FACE_BOUND('',#2486,.T.);
#376=FACE_BOUND('',#2489,.T.);
#377=FACE_BOUND('',#2493,.T.);
#378=FACE_BOUND('',#2496,.T.);
#379=FACE_BOUND('',#2507,.T.);
#380=FACE_BOUND('',#2510,.T.);
#381=FACE_BOUND('',#2522,.T.);
#382=FACE_BOUND('',#2523,.T.);
#383=FACE_BOUND('',#2524,.T.);
#384=FACE_BOUND('',#2525,.T.);
#385=FACE_BOUND('',#2526,.T.);
#386=FACE_BOUND('',#2527,.T.);
#387=FACE_BOUND('',#2528,.T.);
#470=PLANE('',#19254);
#471=PLANE('',#19255);
#472=PLANE('',#19256);
#473=PLANE('',#19257);
#474=PLANE('',#19271);
#475=PLANE('',#19274);
#476=PLANE('',#19277);
#477=PLANE('',#19280);
#478=PLANE('',#19283);
#479=PLANE('',#19286);
#480=PLANE('',#19287);
#481=PLANE('',#19288);
#482=PLANE('',#19289);
#483=PLANE('',#19290);
#484=PLANE('',#19291);
#485=PLANE('',#19292);
#486=PLANE('',#19293);
#487=PLANE('',#19294);
#488=PLANE('',#19295);
#489=PLANE('',#19296);
#490=PLANE('',#19299);
#491=PLANE('',#19302);
#492=PLANE('',#19305);
#493=PLANE('',#19308);
#494=PLANE('',#19311);
#495=PLANE('',#19312);
#496=PLANE('',#19313);
#497=PLANE('',#19314);
#498=PLANE('',#19315);
#499=PLANE('',#19316);
#500=PLANE('',#19317);
#501=PLANE('',#19318);
#502=PLANE('',#19319);
#503=PLANE('',#19320);
#504=PLANE('',#19321);
#505=PLANE('',#19324);
#506=PLANE('',#19325);
#507=PLANE('',#19326);
#508=PLANE('',#19329);
#509=PLANE('',#19330);
#510=PLANE('',#19337);
#511=PLANE('',#19344);
#512=PLANE('',#19351);
#513=PLANE('',#19358);
#514=PLANE('',#19365);
#515=PLANE('',#19372);
#516=PLANE('',#19373);
#517=PLANE('',#19374);
#518=PLANE('',#19375);
#519=PLANE('',#19376);
#520=PLANE('',#19377);
#521=PLANE('',#19378);
#522=PLANE('',#19379);
#523=PLANE('',#19380);
#524=PLANE('',#19381);
#525=PLANE('',#19382);
#526=PLANE('',#19383);
#527=PLANE('',#19384);
#528=PLANE('',#19385);
#529=PLANE('',#19386);
#530=PLANE('',#19387);
#531=PLANE('',#19388);
#532=PLANE('',#19389);
#533=PLANE('',#19390);
#534=PLANE('',#19391);
#535=PLANE('',#19392);
#536=PLANE('',#19393);
#537=PLANE('',#19394);
#538=PLANE('',#19395);
#539=PLANE('',#19396);
#540=PLANE('',#19401);
#541=PLANE('',#19406);
#542=PLANE('',#19411);
#543=PLANE('',#19412);
#544=PLANE('',#19420);
#545=PLANE('',#19423);
#546=PLANE('',#19426);
#646=B_SPLINE_SURFACE_WITH_KNOTS('',3,3,((#60804,#60805,#60806,#60807,#60808,
#60809,#60810,#60811,#60812,#60813,#60814,#60815,#60816,#60817,#60818,#60819,
#60820,#60821,#60822,#60823,#60824,#60825,#60826,#60827,#60828,#60829,#60830,
#60831,#60832,#60833,#60834,#60835,#60836,#60837,#60838,#60839,#60840,#60841,
#60842,#60843,#60844,#60845,#60846,#60847,#60848,#60849,#60850,#60851,#60852,
#60853,#60854,#60855,#60856,#60857,#60858,#60859),(#60860,#60861,#60862,
#60863,#60864,#60865,#60866,#60867,#60868,#60869,#60870,#60871,#60872,#60873,
#60874,#60875,#60876,#60877,#60878,#60879,#60880,#60881,#60882,#60883,#60884,
#60885,#60886,#60887,#60888,#60889,#60890,#60891,#60892,#60893,#60894,#60895,
#60896,#60897,#60898,#60899,#60900,#60901,#60902,#60903,#60904,#60905,#60906,
#60907,#60908,#60909,#60910,#60911,#60912,#60913,#60914,#60915),(#60916,
#60917,#60918,#60919,#60920,#60921,#60922,#60923,#60924,#60925,#60926,#60927,
#60928,#60929,#60930,#60931,#60932,#60933,#60934,#60935,#60936,#60937,#60938,
#60939,#60940,#60941,#60942,#60943,#60944,#60945,#60946,#60947,#60948,#60949,
#60950,#60951,#60952,#60953,#60954,#60955,#60956,#60957,#60958,#60959,#60960,
#60961,#60962,#60963,#60964,#60965,#60966,#60967,#60968,#60969,#60970,#60971),
(#60972,#60973,#60974,#60975,#60976,#60977,#60978,#60979,#60980,#60981,
#60982,#60983,#60984,#60985,#60986,#60987,#60988,#60989,#60990,#60991,#60992,
#60993,#60994,#60995,#60996,#60997,#60998,#60999,#61000,#61001,#61002,#61003,
#61004,#61005,#61006,#61007,#61008,#61009,#61010,#61011,#61012,#61013,#61014,
#61015,#61016,#61017,#61018,#61019,#61020,#61021,#61022,#61023,#61024,#61025,
#61026,#61027)),.UNSPECIFIED.,.F.,.F.,.F.,(4,4),(4,1,1,1,1,1,1,1,1,1,1,
1,1,1,1,1,1,1,1,1,1,1,1,1,1,1,1,1,1,1,1,1,1,1,1,1,1,1,1,1,1,1,1,1,1,1,1,
1,1,1,1,1,1,4),(0.,0.0321584099938623),(11.8553612635793,12.8418906022434,
13.8284199409074,14.8149492795714,15.8014786182354,16.7880079568995,17.7745372955635,
18.7610666342275,19.7475959728916,20.7341253115556,21.7206546502196,22.7071839888837,
23.6937133275477,24.6802426662117,25.6667720048757,26.6533013435398,27.6398306822038,
28.6263600208678,29.6128893595319,30.5994186981959,31.5859480368599,32.572477375524,
33.559006714188,34.545536052852,35.5320653915161,36.5185947301801,37.5051240688441,
38.4916534075081,39.4781827461722,40.4647120848362,41.4512414235002,42.4377707621643,
43.4243001008283,44.4108294394923,45.3973587781564,46.3838881168204,47.3704174554844,
48.3569467941485,49.3434761328125,50.3300054714765,51.3165348101405,52.3030641488046,
53.2895934874686,54.2761228261326,55.2626521647967,56.2491815034607,57.2357108421247,
58.2222401807888,59.2087695194528,60.1952988581168,61.1818281967808,62.1683575354449,
63.1548868741089,64.1414162127729),.UNSPECIFIED.);
#647=B_SPLINE_SURFACE_WITH_KNOTS('',3,3,((#61135,#61136,#61137,#61138,#61139,
#61140,#61141,#61142,#61143,#61144,#61145,#61146,#61147,#61148,#61149,#61150,
#61151,#61152,#61153,#61154,#61155,#61156,#61157,#61158,#61159,#61160,#61161,
#61162,#61163,#61164,#61165,#61166,#61167,#61168,#61169,#61170,#61171,#61172,
#61173,#61174,#61175,#61176,#61177,#61178,#61179,#61180,#61181,#61182,#61183,
#61184,#61185,#61186,#61187,#61188,#61189,#61190),(#61191,#61192,#61193,
#61194,#61195,#61196,#61197,#61198,#61199,#61200,#61201,#61202,#61203,#61204,
#61205,#61206,#61207,#61208,#61209,#61210,#61211,#61212,#61213,#61214,#61215,
#61216,#61217,#61218,#61219,#61220,#61221,#61222,#61223,#61224,#61225,#61226,
#61227,#61228,#61229,#61230,#61231,#61232,#61233,#61234,#61235,#61236,#61237,
#61238,#61239,#61240,#61241,#61242,#61243,#61244,#61245,#61246),(#61247,
#61248,#61249,#61250,#61251,#61252,#61253,#61254,#61255,#61256,#61257,#61258,
#61259,#61260,#61261,#61262,#61263,#61264,#61265,#61266,#61267,#61268,#61269,
#61270,#61271,#61272,#61273,#61274,#61275,#61276,#61277,#61278,#61279,#61280,
#61281,#61282,#61283,#61284,#61285,#61286,#61287,#61288,#61289,#61290,#61291,
#61292,#61293,#61294,#61295,#61296,#61297,#61298,#61299,#61300,#61301,#61302),
(#61303,#61304,#61305,#61306,#61307,#61308,#61309,#61310,#61311,#61312,
#61313,#61314,#61315,#61316,#61317,#61318,#61319,#61320,#61321,#61322,#61323,
#61324,#61325,#61326,#61327,#61328,#61329,#61330,#61331,#61332,#61333,#61334,
#61335,#61336,#61337,#61338,#61339,#61340,#61341,#61342,#61343,#61344,#61345,
#61346,#61347,#61348,#61349,#61350,#61351,#61352,#61353,#61354,#61355,#61356,
#61357,#61358)),.UNSPECIFIED.,.F.,.F.,.F.,(4,4),(4,1,1,1,1,1,1,1,1,1,1,
1,1,1,1,1,1,1,1,1,1,1,1,1,1,1,1,1,1,1,1,1,1,1,1,1,1,1,1,1,1,1,1,1,1,1,1,
1,1,1,1,1,1,4),(0.,0.0321584099938623),(14.3984001269718,15.3849294656359,
16.3714588042999,17.3579881429639,18.3445174816279,19.331046820292,20.317576158956,
21.30410549762,22.2906348362841,23.2771641749481,24.2636935136121,25.2502228522762,
26.2367521909402,27.2232815296042,28.2098108682683,29.1963402069323,30.1828695455963,
31.1693988842603,32.1559282229244,33.1424575615884,34.1289869002524,35.1155162389165,
36.1020455775805,37.0885749162445,38.0751042549086,39.0616335935726,40.0481629322366,
41.0346922709007,42.0212216095647,43.0077509482287,43.9942802868927,44.9808096255568,
45.9673389642208,46.9538683028848,47.9403976415489,48.9269269802129,49.9134563188769,
50.899985657541,51.886514996205,52.873044334869,53.8595736735331,54.8461030121971,
55.8326323508611,56.8191616895252,57.8056910281892,58.7922203668532,59.7787497055172,
60.7652790441813,61.7518083828453,62.7383377215093,63.7248670601734,64.7113963988374,
65.6979257375014,66.6844550761655),.UNSPECIFIED.);
#648=B_SPLINE_SURFACE_WITH_KNOTS('',3,3,((#61645,#61646,#61647,#61648,#61649,
#61650,#61651,#61652,#61653,#61654,#61655,#61656,#61657,#61658,#61659,#61660,
#61661,#61662,#61663,#61664,#61665,#61666,#61667,#61668,#61669,#61670,#61671,
#61672,#61673,#61674,#61675,#61676,#61677,#61678,#61679,#61680,#61681,#61682,
#61683,#61684,#61685,#61686,#61687,#61688,#61689,#61690,#61691,#61692,#61693,
#61694,#61695,#61696,#61697,#61698,#61699,#61700),(#61701,#61702,#61703,
#61704,#61705,#61706,#61707,#61708,#61709,#61710,#61711,#61712,#61713,#61714,
#61715,#61716,#61717,#61718,#61719,#61720,#61721,#61722,#61723,#61724,#61725,
#61726,#61727,#61728,#61729,#61730,#61731,#61732,#61733,#61734,#61735,#61736,
#61737,#61738,#61739,#61740,#61741,#61742,#61743,#61744,#61745,#61746,#61747,
#61748,#61749,#61750,#61751,#61752,#61753,#61754,#61755,#61756),(#61757,
#61758,#61759,#61760,#61761,#61762,#61763,#61764,#61765,#61766,#61767,#61768,
#61769,#61770,#61771,#61772,#61773,#61774,#61775,#61776,#61777,#61778,#61779,
#61780,#61781,#61782,#61783,#61784,#61785,#61786,#61787,#61788,#61789,#61790,
#61791,#61792,#61793,#61794,#61795,#61796,#61797,#61798,#61799,#61800,#61801,
#61802,#61803,#61804,#61805,#61806,#61807,#61808,#61809,#61810,#61811,#61812),
(#61813,#61814,#61815,#61816,#61817,#61818,#61819,#61820,#61821,#61822,
#61823,#61824,#61825,#61826,#61827,#61828,#61829,#61830,#61831,#61832,#61833,
#61834,#61835,#61836,#61837,#61838,#61839,#61840,#61841,#61842,#61843,#61844,
#61845,#61846,#61847,#61848,#61849,#61850,#61851,#61852,#61853,#61854,#61855,
#61856,#61857,#61858,#61859,#61860,#61861,#61862,#61863,#61864,#61865,#61866,
#61867,#61868)),.UNSPECIFIED.,.F.,.F.,.F.,(4,4),(4,1,1,1,1,1,1,1,1,1,1,
1,1,1,1,1,1,1,1,1,1,1,1,1,1,1,1,1,1,1,1,1,1,1,1,1,1,1,1,1,1,1,1,1,1,1,1,
1,1,1,1,1,1,4),(0.,0.0321584099938627),(11.8553612635793,12.8418906022434,
13.8284199409074,14.8149492795714,15.8014786182355,16.7880079568995,17.7745372955635,
18.7610666342275,19.7475959728916,20.7341253115556,21.7206546502196,22.7071839888837,
23.6937133275477,24.6802426662117,25.6667720048758,26.6533013435398,27.6398306822038,
28.6263600208679,29.6128893595319,30.5994186981959,31.5859480368599,32.572477375524,
33.559006714188,34.545536052852,35.5320653915161,36.5185947301801,37.5051240688441,
38.4916534075082,39.4781827461722,40.4647120848362,41.4512414235002,42.4377707621643,
43.4243001008283,44.4108294394923,45.3973587781564,46.3838881168204,47.3704174554844,
48.3569467941485,49.3434761328125,50.3300054714765,51.3165348101406,52.3030641488046,
53.2895934874686,54.2761228261326,55.2626521647967,56.2491815034607,57.2357108421247,
58.2222401807888,59.2087695194528,60.1952988581168,61.1818281967809,62.1683575354449,
63.1548868741089,64.141416212773),.UNSPECIFIED.);
#649=B_SPLINE_SURFACE_WITH_KNOTS('',3,3,((#61976,#61977,#61978,#61979,#61980,
#61981,#61982,#61983,#61984,#61985,#61986,#61987,#61988,#61989,#61990,#61991,
#61992,#61993,#61994,#61995,#61996,#61997,#61998,#61999,#62000,#62001,#62002,
#62003,#62004,#62005,#62006,#62007,#62008,#62009,#62010,#62011,#62012,#62013,
#62014,#62015,#62016,#62017,#62018,#62019,#62020,#62021,#62022,#62023,#62024,
#62025,#62026,#62027,#62028,#62029,#62030,#62031),(#62032,#62033,#62034,
#62035,#62036,#62037,#62038,#62039,#62040,#62041,#62042,#62043,#62044,#62045,
#62046,#62047,#62048,#62049,#62050,#62051,#62052,#62053,#62054,#62055,#62056,
#62057,#62058,#62059,#62060,#62061,#62062,#62063,#62064,#62065,#62066,#62067,
#62068,#62069,#62070,#62071,#62072,#62073,#62074,#62075,#62076,#62077,#62078,
#62079,#62080,#62081,#62082,#62083,#62084,#62085,#62086,#62087),(#62088,
#62089,#62090,#62091,#62092,#62093,#62094,#62095,#62096,#62097,#62098,#62099,
#62100,#62101,#62102,#62103,#62104,#62105,#62106,#62107,#62108,#62109,#62110,
#62111,#62112,#62113,#62114,#62115,#62116,#62117,#62118,#62119,#62120,#62121,
#62122,#62123,#62124,#62125,#62126,#62127,#62128,#62129,#62130,#62131,#62132,
#62133,#62134,#62135,#62136,#62137,#62138,#62139,#62140,#62141,#62142,#62143),
(#62144,#62145,#62146,#62147,#62148,#62149,#62150,#62151,#62152,#62153,
#62154,#62155,#62156,#62157,#62158,#62159,#62160,#62161,#62162,#62163,#62164,
#62165,#62166,#62167,#62168,#62169,#62170,#62171,#62172,#62173,#62174,#62175,
#62176,#62177,#62178,#62179,#62180,#62181,#62182,#62183,#62184,#62185,#62186,
#62187,#62188,#62189,#62190,#62191,#62192,#62193,#62194,#62195,#62196,#62197,
#62198,#62199)),.UNSPECIFIED.,.F.,.F.,.F.,(4,4),(4,1,1,1,1,1,1,1,1,1,1,
1,1,1,1,1,1,1,1,1,1,1,1,1,1,1,1,1,1,1,1,1,1,1,1,1,1,1,1,1,1,1,1,1,1,1,1,
1,1,1,1,1,1,4),(0.,0.0321584099938627),(14.3984001269718,15.3849294656359,
16.3714588042999,17.3579881429639,18.344517481628,19.331046820292,20.317576158956,
21.3041054976201,22.2906348362841,23.2771641749481,24.2636935136121,25.2502228522762,
26.2367521909402,27.2232815296042,28.2098108682683,29.1963402069323,30.1828695455963,
31.1693988842604,32.1559282229244,33.1424575615884,34.1289869002525,35.1155162389165,
36.1020455775805,37.0885749162445,38.0751042549086,39.0616335935726,40.0481629322366,
41.0346922709007,42.0212216095647,43.0077509482287,43.9942802868928,44.9808096255568,
45.9673389642208,46.9538683028849,47.9403976415489,48.9269269802129,49.9134563188769,
50.899985657541,51.886514996205,52.873044334869,53.8595736735331,54.8461030121971,
55.8326323508611,56.8191616895252,57.8056910281892,58.7922203668532,59.7787497055173,
60.7652790441813,61.7518083828453,62.7383377215094,63.7248670601734,64.7113963988374,
65.6979257375014,66.6844550761655),.UNSPECIFIED.);
#650=B_SPLINE_SURFACE_WITH_KNOTS('',3,3,((#62486,#62487,#62488,#62489,#62490,
#62491,#62492,#62493,#62494,#62495,#62496,#62497,#62498,#62499,#62500,#62501,
#62502,#62503,#62504,#62505,#62506,#62507,#62508,#62509,#62510,#62511,#62512,
#62513,#62514,#62515,#62516,#62517,#62518,#62519,#62520,#62521,#62522,#62523,
#62524,#62525,#62526,#62527,#62528,#62529,#62530,#62531,#62532,#62533,#62534,
#62535,#62536,#62537,#62538,#62539,#62540,#62541),(#62542,#62543,#62544,
#62545,#62546,#62547,#62548,#62549,#62550,#62551,#62552,#62553,#62554,#62555,
#62556,#62557,#62558,#62559,#62560,#62561,#62562,#62563,#62564,#62565,#62566,
#62567,#62568,#62569,#62570,#62571,#62572,#62573,#62574,#62575,#62576,#62577,
#62578,#62579,#62580,#62581,#62582,#62583,#62584,#62585,#62586,#62587,#62588,
#62589,#62590,#62591,#62592,#62593,#62594,#62595,#62596,#62597),(#62598,
#62599,#62600,#62601,#62602,#62603,#62604,#62605,#62606,#62607,#62608,#62609,
#62610,#62611,#62612,#62613,#62614,#62615,#62616,#62617,#62618,#62619,#62620,
#62621,#62622,#62623,#62624,#62625,#62626,#62627,#62628,#62629,#62630,#62631,
#62632,#62633,#62634,#62635,#62636,#62637,#62638,#62639,#62640,#62641,#62642,
#62643,#62644,#62645,#62646,#62647,#62648,#62649,#62650,#62651,#62652,#62653),
(#62654,#62655,#62656,#62657,#62658,#62659,#62660,#62661,#62662,#62663,
#62664,#62665,#62666,#62667,#62668,#62669,#62670,#62671,#62672,#62673,#62674,
#62675,#62676,#62677,#62678,#62679,#62680,#62681,#62682,#62683,#62684,#62685,
#62686,#62687,#62688,#62689,#62690,#62691,#62692,#62693,#62694,#62695,#62696,
#62697,#62698,#62699,#62700,#62701,#62702,#62703,#62704,#62705,#62706,#62707,
#62708,#62709)),.UNSPECIFIED.,.F.,.F.,.F.,(4,4),(4,1,1,1,1,1,1,1,1,1,1,
1,1,1,1,1,1,1,1,1,1,1,1,1,1,1,1,1,1,1,1,1,1,1,1,1,1,1,1,1,1,1,1,1,1,1,1,
1,1,1,1,1,1,4),(0.,0.0321584099938621),(11.8553612635793,12.8418906022434,
13.8284199409074,14.8149492795714,15.8014786182354,16.7880079568995,17.7745372955635,
18.7610666342275,19.7475959728916,20.7341253115556,21.7206546502196,22.7071839888837,
23.6937133275477,24.6802426662117,25.6667720048758,26.6533013435398,27.6398306822038,
28.6263600208678,29.6128893595319,30.5994186981959,31.5859480368599,32.572477375524,
33.559006714188,34.545536052852,35.5320653915161,36.5185947301801,37.5051240688441,
38.4916534075081,39.4781827461722,40.4647120848362,41.4512414235002,42.4377707621643,
43.4243001008283,44.4108294394923,45.3973587781564,46.3838881168204,47.3704174554844,
48.3569467941485,49.3434761328125,50.3300054714765,51.3165348101405,52.3030641488046,
53.2895934874686,54.2761228261326,55.2626521647967,56.2491815034607,57.2357108421247,
58.2222401807888,59.2087695194528,60.1952988581168,61.1818281967808,62.1683575354449,
63.1548868741089,64.1414162127729),.UNSPECIFIED.);
#651=B_SPLINE_SURFACE_WITH_KNOTS('',3,3,((#62817,#62818,#62819,#62820,#62821,
#62822,#62823,#62824,#62825,#62826,#62827,#62828,#62829,#62830,#62831,#62832,
#62833,#62834,#62835,#62836,#62837,#62838,#62839,#62840,#62841,#62842,#62843,
#62844,#62845,#62846,#62847,#62848,#62849,#62850,#62851,#62852,#62853,#62854,
#62855,#62856,#62857,#62858,#62859,#62860,#62861,#62862,#62863,#62864,#62865,
#62866,#62867,#62868,#62869,#62870,#62871,#62872),(#62873,#62874,#62875,
#62876,#62877,#62878,#62879,#62880,#62881,#62882,#62883,#62884,#62885,#62886,
#62887,#62888,#62889,#62890,#62891,#62892,#62893,#62894,#62895,#62896,#62897,
#62898,#62899,#62900,#62901,#62902,#62903,#62904,#62905,#62906,#62907,#62908,
#62909,#62910,#62911,#62912,#62913,#62914,#62915,#62916,#62917,#62918,#62919,
#62920,#62921,#62922,#62923,#62924,#62925,#62926,#62927,#62928),(#62929,
#62930,#62931,#62932,#62933,#62934,#62935,#62936,#62937,#62938,#62939,#62940,
#62941,#62942,#62943,#62944,#62945,#62946,#62947,#62948,#62949,#62950,#62951,
#62952,#62953,#62954,#62955,#62956,#62957,#62958,#62959,#62960,#62961,#62962,
#62963,#62964,#62965,#62966,#62967,#62968,#62969,#62970,#62971,#62972,#62973,
#62974,#62975,#62976,#62977,#62978,#62979,#62980,#62981,#62982,#62983,#62984),
(#62985,#62986,#62987,#62988,#62989,#62990,#62991,#62992,#62993,#62994,
#62995,#62996,#62997,#62998,#62999,#63000,#63001,#63002,#63003,#63004,#63005,
#63006,#63007,#63008,#63009,#63010,#63011,#63012,#63013,#63014,#63015,#63016,
#63017,#63018,#63019,#63020,#63021,#63022,#63023,#63024,#63025,#63026,#63027,
#63028,#63029,#63030,#63031,#63032,#63033,#63034,#63035,#63036,#63037,#63038,
#63039,#63040)),.UNSPECIFIED.,.F.,.F.,.F.,(4,4),(4,1,1,1,1,1,1,1,1,1,1,
1,1,1,1,1,1,1,1,1,1,1,1,1,1,1,1,1,1,1,1,1,1,1,1,1,1,1,1,1,1,1,1,1,1,1,1,
1,1,1,1,1,1,4),(0.,0.0321584099938621),(14.3984001269718,15.3849294656359,
16.3714588042999,17.3579881429639,18.3445174816279,19.331046820292,20.317576158956,
21.30410549762,22.2906348362841,23.2771641749481,24.2636935136121,25.2502228522762,
26.2367521909402,27.2232815296042,28.2098108682683,29.1963402069323,30.1828695455963,
31.1693988842603,32.1559282229244,33.1424575615884,34.1289869002524,35.1155162389165,
36.1020455775805,37.0885749162445,38.0751042549086,39.0616335935726,40.0481629322366,
41.0346922709007,42.0212216095647,43.0077509482287,43.9942802868928,44.9808096255568,
45.9673389642208,46.9538683028848,47.9403976415489,48.9269269802129,49.9134563188769,
50.899985657541,51.886514996205,52.873044334869,53.8595736735331,54.8461030121971,
55.8326323508611,56.8191616895252,57.8056910281892,58.7922203668532,59.7787497055172,
60.7652790441813,61.7518083828453,62.7383377215093,63.7248670601734,64.7113963988374,
65.6979257375014,66.6844550761655),.UNSPECIFIED.);
#652=B_SPLINE_SURFACE_WITH_KNOTS('',3,3,((#63327,#63328,#63329,#63330,#63331,
#63332,#63333,#63334,#63335,#63336,#63337,#63338,#63339,#63340,#63341,#63342,
#63343,#63344,#63345,#63346,#63347,#63348,#63349,#63350,#63351,#63352,#63353,
#63354,#63355,#63356,#63357,#63358,#63359,#63360,#63361,#63362,#63363,#63364,
#63365,#63366,#63367,#63368,#63369,#63370,#63371,#63372,#63373,#63374,#63375,
#63376,#63377,#63378,#63379,#63380,#63381,#63382),(#63383,#63384,#63385,
#63386,#63387,#63388,#63389,#63390,#63391,#63392,#63393,#63394,#63395,#63396,
#63397,#63398,#63399,#63400,#63401,#63402,#63403,#63404,#63405,#63406,#63407,
#63408,#63409,#63410,#63411,#63412,#63413,#63414,#63415,#63416,#63417,#63418,
#63419,#63420,#63421,#63422,#63423,#63424,#63425,#63426,#63427,#63428,#63429,
#63430,#63431,#63432,#63433,#63434,#63435,#63436,#63437,#63438),(#63439,
#63440,#63441,#63442,#63443,#63444,#63445,#63446,#63447,#63448,#63449,#63450,
#63451,#63452,#63453,#63454,#63455,#63456,#63457,#63458,#63459,#63460,#63461,
#63462,#63463,#63464,#63465,#63466,#63467,#63468,#63469,#63470,#63471,#63472,
#63473,#63474,#63475,#63476,#63477,#63478,#63479,#63480,#63481,#63482,#63483,
#63484,#63485,#63486,#63487,#63488,#63489,#63490,#63491,#63492,#63493,#63494),
(#63495,#63496,#63497,#63498,#63499,#63500,#63501,#63502,#63503,#63504,
#63505,#63506,#63507,#63508,#63509,#63510,#63511,#63512,#63513,#63514,#63515,
#63516,#63517,#63518,#63519,#63520,#63521,#63522,#63523,#63524,#63525,#63526,
#63527,#63528,#63529,#63530,#63531,#63532,#63533,#63534,#63535,#63536,#63537,
#63538,#63539,#63540,#63541,#63542,#63543,#63544,#63545,#63546,#63547,#63548,
#63549,#63550)),.UNSPECIFIED.,.F.,.F.,.F.,(4,4),(4,1,1,1,1,1,1,1,1,1,1,
1,1,1,1,1,1,1,1,1,1,1,1,1,1,1,1,1,1,1,1,1,1,1,1,1,1,1,1,1,1,1,1,1,1,1,1,
1,1,1,1,1,1,4),(0.,0.0321584099938623),(11.8553612635793,12.8418906022434,
13.8284199409074,14.8149492795714,15.8014786182354,16.7880079568995,17.7745372955635,
18.7610666342275,19.7475959728916,20.7341253115556,21.7206546502196,22.7071839888837,
23.6937133275477,24.6802426662117,25.6667720048757,26.6533013435398,27.6398306822038,
28.6263600208678,29.6128893595319,30.5994186981959,31.5859480368599,32.572477375524,
33.559006714188,34.545536052852,35.5320653915161,36.5185947301801,37.5051240688441,
38.4916534075081,39.4781827461722,40.4647120848362,41.4512414235002,42.4377707621643,
43.4243001008283,44.4108294394923,45.3973587781564,46.3838881168204,47.3704174554844,
48.3569467941485,49.3434761328125,50.3300054714765,51.3165348101405,52.3030641488046,
53.2895934874686,54.2761228261326,55.2626521647967,56.2491815034607,57.2357108421247,
58.2222401807888,59.2087695194528,60.1952988581168,61.1818281967808,62.1683575354449,
63.1548868741089,64.1414162127729),.UNSPECIFIED.);
#653=B_SPLINE_SURFACE_WITH_KNOTS('',3,3,((#63658,#63659,#63660,#63661,#63662,
#63663,#63664,#63665,#63666,#63667,#63668,#63669,#63670,#63671,#63672,#63673,
#63674,#63675,#63676,#63677,#63678,#63679,#63680,#63681,#63682,#63683,#63684,
#63685,#63686,#63687,#63688,#63689,#63690,#63691,#63692,#63693,#63694,#63695,
#63696,#63697,#63698,#63699,#63700,#63701,#63702,#63703,#63704,#63705,#63706,
#63707,#63708,#63709,#63710,#63711,#63712,#63713),(#63714,#63715,#63716,
#63717,#63718,#63719,#63720,#63721,#63722,#63723,#63724,#63725,#63726,#63727,
#63728,#63729,#63730,#63731,#63732,#63733,#63734,#63735,#63736,#63737,#63738,
#63739,#63740,#63741,#63742,#63743,#63744,#63745,#63746,#63747,#63748,#63749,
#63750,#63751,#63752,#63753,#63754,#63755,#63756,#63757,#63758,#63759,#63760,
#63761,#63762,#63763,#63764,#63765,#63766,#63767,#63768,#63769),(#63770,
#63771,#63772,#63773,#63774,#63775,#63776,#63777,#63778,#63779,#63780,#63781,
#63782,#63783,#63784,#63785,#63786,#63787,#63788,#63789,#63790,#63791,#63792,
#63793,#63794,#63795,#63796,#63797,#63798,#63799,#63800,#63801,#63802,#63803,
#63804,#63805,#63806,#63807,#63808,#63809,#63810,#63811,#63812,#63813,#63814,
#63815,#63816,#63817,#63818,#63819,#63820,#63821,#63822,#63823,#63824,#63825),
(#63826,#63827,#63828,#63829,#63830,#63831,#63832,#63833,#63834,#63835,
#63836,#63837,#63838,#63839,#63840,#63841,#63842,#63843,#63844,#63845,#63846,
#63847,#63848,#63849,#63850,#63851,#63852,#63853,#63854,#63855,#63856,#63857,
#63858,#63859,#63860,#63861,#63862,#63863,#63864,#63865,#63866,#63867,#63868,
#63869,#63870,#63871,#63872,#63873,#63874,#63875,#63876,#63877,#63878,#63879,
#63880,#63881)),.UNSPECIFIED.,.F.,.F.,.F.,(4,4),(4,1,1,1,1,1,1,1,1,1,1,
1,1,1,1,1,1,1,1,1,1,1,1,1,1,1,1,1,1,1,1,1,1,1,1,1,1,1,1,1,1,1,1,1,1,1,1,
1,1,1,1,1,1,4),(0.,0.0321584099938623),(14.3984001269718,15.3849294656359,
16.3714588042999,17.3579881429639,18.3445174816279,19.331046820292,20.317576158956,
21.30410549762,22.2906348362841,23.2771641749481,24.2636935136121,25.2502228522762,
26.2367521909402,27.2232815296042,28.2098108682683,29.1963402069323,30.1828695455963,
31.1693988842603,32.1559282229244,33.1424575615884,34.1289869002524,35.1155162389165,
36.1020455775805,37.0885749162445,38.0751042549086,39.0616335935726,40.0481629322366,
41.0346922709007,42.0212216095647,43.0077509482287,43.9942802868928,44.9808096255568,
45.9673389642208,46.9538683028848,47.9403976415489,48.9269269802129,49.9134563188769,
50.899985657541,51.886514996205,52.873044334869,53.8595736735331,54.8461030121971,
55.8326323508611,56.8191616895252,57.8056910281892,58.7922203668532,59.7787497055172,
60.7652790441813,61.7518083828453,62.7383377215093,63.7248670601734,64.7113963988374,
65.6979257375014,66.6844550761655),.UNSPECIFIED.);
#654=B_SPLINE_SURFACE_WITH_KNOTS('',3,3,((#64168,#64169,#64170,#64171,#64172,
#64173,#64174,#64175,#64176,#64177,#64178,#64179,#64180,#64181,#64182,#64183,
#64184,#64185,#64186,#64187,#64188,#64189,#64190,#64191,#64192,#64193,#64194,
#64195,#64196,#64197,#64198,#64199,#64200,#64201,#64202,#64203,#64204,#64205,
#64206,#64207,#64208,#64209,#64210,#64211,#64212,#64213,#64214,#64215,#64216,
#64217,#64218,#64219,#64220,#64221,#64222,#64223),(#64224,#64225,#64226,
#64227,#64228,#64229,#64230,#64231,#64232,#64233,#64234,#64235,#64236,#64237,
#64238,#64239,#64240,#64241,#64242,#64243,#64244,#64245,#64246,#64247,#64248,
#64249,#64250,#64251,#64252,#64253,#64254,#64255,#64256,#64257,#64258,#64259,
#64260,#64261,#64262,#64263,#64264,#64265,#64266,#64267,#64268,#64269,#64270,
#64271,#64272,#64273,#64274,#64275,#64276,#64277,#64278,#64279),(#64280,
#64281,#64282,#64283,#64284,#64285,#64286,#64287,#64288,#64289,#64290,#64291,
#64292,#64293,#64294,#64295,#64296,#64297,#64298,#64299,#64300,#64301,#64302,
#64303,#64304,#64305,#64306,#64307,#64308,#64309,#64310,#64311,#64312,#64313,
#64314,#64315,#64316,#64317,#64318,#64319,#64320,#64321,#64322,#64323,#64324,
#64325,#64326,#64327,#64328,#64329,#64330,#64331,#64332,#64333,#64334,#64335),
(#64336,#64337,#64338,#64339,#64340,#64341,#64342,#64343,#64344,#64345,
#64346,#64347,#64348,#64349,#64350,#64351,#64352,#64353,#64354,#64355,#64356,
#64357,#64358,#64359,#64360,#64361,#64362,#64363,#64364,#64365,#64366,#64367,
#64368,#64369,#64370,#64371,#64372,#64373,#64374,#64375,#64376,#64377,#64378,
#64379,#64380,#64381,#64382,#64383,#64384,#64385,#64386,#64387,#64388,#64389,
#64390,#64391)),.UNSPECIFIED.,.F.,.F.,.F.,(4,4),(4,1,1,1,1,1,1,1,1,1,1,
1,1,1,1,1,1,1,1,1,1,1,1,1,1,1,1,1,1,1,1,1,1,1,1,1,1,1,1,1,1,1,1,1,1,1,1,
1,1,1,1,1,1,4),(0.,0.0321584099938627),(11.8553612635793,12.8418906022434,
13.8284199409074,14.8149492795714,15.8014786182355,16.7880079568995,17.7745372955635,
18.7610666342275,19.7475959728916,20.7341253115556,21.7206546502196,22.7071839888837,
23.6937133275477,24.6802426662117,25.6667720048758,26.6533013435398,27.6398306822038,
28.6263600208678,29.6128893595319,30.5994186981959,31.5859480368599,32.572477375524,
33.559006714188,34.545536052852,35.5320653915161,36.5185947301801,37.5051240688441,
38.4916534075082,39.4781827461722,40.4647120848362,41.4512414235002,42.4377707621643,
43.4243001008283,44.4108294394923,45.3973587781564,46.3838881168204,47.3704174554844,
48.3569467941485,49.3434761328125,50.3300054714765,51.3165348101406,52.3030641488046,
53.2895934874686,54.2761228261326,55.2626521647967,56.2491815034607,57.2357108421247,
58.2222401807888,59.2087695194528,60.1952988581168,61.1818281967809,62.1683575354449,
63.1548868741089,64.1414162127729),.UNSPECIFIED.);
#655=B_SPLINE_SURFACE_WITH_KNOTS('',3,3,((#64499,#64500,#64501,#64502,#64503,
#64504,#64505,#64506,#64507,#64508,#64509,#64510,#64511,#64512,#64513,#64514,
#64515,#64516,#64517,#64518,#64519,#64520,#64521,#64522,#64523,#64524,#64525,
#64526,#64527,#64528,#64529,#64530,#64531,#64532,#64533,#64534,#64535,#64536,
#64537,#64538,#64539,#64540,#64541,#64542,#64543,#64544,#64545,#64546,#64547,
#64548,#64549,#64550,#64551,#64552,#64553,#64554),(#64555,#64556,#64557,
#64558,#64559,#64560,#64561,#64562,#64563,#64564,#64565,#64566,#64567,#64568,
#64569,#64570,#64571,#64572,#64573,#64574,#64575,#64576,#64577,#64578,#64579,
#64580,#64581,#64582,#64583,#64584,#64585,#64586,#64587,#64588,#64589,#64590,
#64591,#64592,#64593,#64594,#64595,#64596,#64597,#64598,#64599,#64600,#64601,
#64602,#64603,#64604,#64605,#64606,#64607,#64608,#64609,#64610),(#64611,
#64612,#64613,#64614,#64615,#64616,#64617,#64618,#64619,#64620,#64621,#64622,
#64623,#64624,#64625,#64626,#64627,#64628,#64629,#64630,#64631,#64632,#64633,
#64634,#64635,#64636,#64637,#64638,#64639,#64640,#64641,#64642,#64643,#64644,
#64645,#64646,#64647,#64648,#64649,#64650,#64651,#64652,#64653,#64654,#64655,
#64656,#64657,#64658,#64659,#64660,#64661,#64662,#64663,#64664,#64665,#64666),
(#64667,#64668,#64669,#64670,#64671,#64672,#64673,#64674,#64675,#64676,
#64677,#64678,#64679,#64680,#64681,#64682,#64683,#64684,#64685,#64686,#64687,
#64688,#64689,#64690,#64691,#64692,#64693,#64694,#64695,#64696,#64697,#64698,
#64699,#64700,#64701,#64702,#64703,#64704,#64705,#64706,#64707,#64708,#64709,
#64710,#64711,#64712,#64713,#64714,#64715,#64716,#64717,#64718,#64719,#64720,
#64721,#64722)),.UNSPECIFIED.,.F.,.F.,.F.,(4,4),(4,1,1,1,1,1,1,1,1,1,1,
1,1,1,1,1,1,1,1,1,1,1,1,1,1,1,1,1,1,1,1,1,1,1,1,1,1,1,1,1,1,1,1,1,1,1,1,
1,1,1,1,1,1,4),(0.,0.0321584099938627),(14.3984001269718,15.3849294656359,
16.3714588042999,17.3579881429639,18.344517481628,19.331046820292,20.317576158956,
21.30410549762,22.2906348362841,23.2771641749481,24.2636935136121,25.2502228522762,
26.2367521909402,27.2232815296042,28.2098108682683,29.1963402069323,30.1828695455963,
31.1693988842604,32.1559282229244,33.1424575615884,34.1289869002524,35.1155162389165,
36.1020455775805,37.0885749162445,38.0751042549086,39.0616335935726,40.0481629322366,
41.0346922709007,42.0212216095647,43.0077509482287,43.9942802868928,44.9808096255568,
45.9673389642208,46.9538683028848,47.9403976415489,48.9269269802129,49.9134563188769,
50.899985657541,51.886514996205,52.873044334869,53.8595736735331,54.8461030121971,
55.8326323508611,56.8191616895252,57.8056910281892,58.7922203668532,59.7787497055172,
60.7652790441813,61.7518083828453,62.7383377215093,63.7248670601734,64.7113963988374,
65.6979257375014,66.6844550761655),.UNSPECIFIED.);
#656=B_SPLINE_SURFACE_WITH_KNOTS('',3,3,((#65029,#65030,#65031,#65032,#65033,
#65034,#65035,#65036,#65037,#65038,#65039,#65040,#65041,#65042,#65043,#65044,
#65045,#65046,#65047,#65048,#65049,#65050,#65051,#65052,#65053,#65054,#65055,
#65056,#65057,#65058,#65059,#65060,#65061,#65062,#65063,#65064,#65065,#65066,
#65067,#65068,#65069,#65070,#65071,#65072,#65073,#65074,#65075,#65076,#65077,
#65078,#65079,#65080,#65081,#65082,#65083,#65084),(#65085,#65086,#65087,
#65088,#65089,#65090,#65091,#65092,#65093,#65094,#65095,#65096,#65097,#65098,
#65099,#65100,#65101,#65102,#65103,#65104,#65105,#65106,#65107,#65108,#65109,
#65110,#65111,#65112,#65113,#65114,#65115,#65116,#65117,#65118,#65119,#65120,
#65121,#65122,#65123,#65124,#65125,#65126,#65127,#65128,#65129,#65130,#65131,
#65132,#65133,#65134,#65135,#65136,#65137,#65138,#65139,#65140),(#65141,
#65142,#65143,#65144,#65145,#65146,#65147,#65148,#65149,#65150,#65151,#65152,
#65153,#65154,#65155,#65156,#65157,#65158,#65159,#65160,#65161,#65162,#65163,
#65164,#65165,#65166,#65167,#65168,#65169,#65170,#65171,#65172,#65173,#65174,
#65175,#65176,#65177,#65178,#65179,#65180,#65181,#65182,#65183,#65184,#65185,
#65186,#65187,#65188,#65189,#65190,#65191,#65192,#65193,#65194,#65195,#65196),
(#65197,#65198,#65199,#65200,#65201,#65202,#65203,#65204,#65205,#65206,
#65207,#65208,#65209,#65210,#65211,#65212,#65213,#65214,#65215,#65216,#65217,
#65218,#65219,#65220,#65221,#65222,#65223,#65224,#65225,#65226,#65227,#65228,
#65229,#65230,#65231,#65232,#65233,#65234,#65235,#65236,#65237,#65238,#65239,
#65240,#65241,#65242,#65243,#65244,#65245,#65246,#65247,#65248,#65249,#65250,
#65251,#65252)),.UNSPECIFIED.,.F.,.F.,.F.,(4,4),(4,1,1,1,1,1,1,1,1,1,1,
1,1,1,1,1,1,1,1,1,1,1,1,1,1,1,1,1,1,1,1,1,1,1,1,1,1,1,1,1,1,1,1,1,1,1,1,
1,1,1,1,1,1,4),(0.,0.032158409993862),(11.8553612635794,12.8418906022434,
13.8284199409074,14.8149492795714,15.8014786182355,16.7880079568995,17.7745372955635,
18.7610666342276,19.7475959728916,20.7341253115556,21.7206546502197,22.7071839888837,
23.6937133275477,24.6802426662118,25.6667720048758,26.6533013435398,27.6398306822038,
28.6263600208679,29.6128893595319,30.5994186981959,31.58594803686,32.572477375524,
33.559006714188,34.5455360528521,35.5320653915161,36.5185947301801,37.5051240688441,
38.4916534075082,39.4781827461722,40.4647120848362,41.4512414235003,42.4377707621643,
43.4243001008283,44.4108294394924,45.3973587781564,46.3838881168204,47.3704174554844,
48.3569467941485,49.3434761328125,50.3300054714765,51.3165348101406,52.3030641488046,
53.2895934874686,54.2761228261327,55.2626521647967,56.2491815034607,57.2357108421248,
58.2222401807888,59.2087695194528,60.1952988581168,61.1818281967809,62.1683575354449,
63.1548868741089,64.141416212773),.UNSPECIFIED.);
#657=B_SPLINE_SURFACE_WITH_KNOTS('',3,3,((#65278,#65279,#65280,#65281,#65282,
#65283,#65284,#65285,#65286,#65287,#65288,#65289,#65290,#65291,#65292,#65293,
#65294,#65295,#65296,#65297,#65298,#65299,#65300,#65301,#65302,#65303,#65304,
#65305,#65306,#65307,#65308,#65309,#65310,#65311,#65312,#65313,#65314,#65315,
#65316,#65317,#65318,#65319,#65320,#65321,#65322,#65323,#65324,#65325,#65326,
#65327,#65328,#65329,#65330,#65331,#65332,#65333),(#65334,#65335,#65336,
#65337,#65338,#65339,#65340,#65341,#65342,#65343,#65344,#65345,#65346,#65347,
#65348,#65349,#65350,#65351,#65352,#65353,#65354,#65355,#65356,#65357,#65358,
#65359,#65360,#65361,#65362,#65363,#65364,#65365,#65366,#65367,#65368,#65369,
#65370,#65371,#65372,#65373,#65374,#65375,#65376,#65377,#65378,#65379,#65380,
#65381,#65382,#65383,#65384,#65385,#65386,#65387,#65388,#65389),(#65390,
#65391,#65392,#65393,#65394,#65395,#65396,#65397,#65398,#65399,#65400,#65401,
#65402,#65403,#65404,#65405,#65406,#65407,#65408,#65409,#65410,#65411,#65412,
#65413,#65414,#65415,#65416,#65417,#65418,#65419,#65420,#65421,#65422,#65423,
#65424,#65425,#65426,#65427,#65428,#65429,#65430,#65431,#65432,#65433,#65434,
#65435,#65436,#65437,#65438,#65439,#65440,#65441,#65442,#65443,#65444,#65445),
(#65446,#65447,#65448,#65449,#65450,#65451,#65452,#65453,#65454,#65455,
#65456,#65457,#65458,#65459,#65460,#65461,#65462,#65463,#65464,#65465,#65466,
#65467,#65468,#65469,#65470,#65471,#65472,#65473,#65474,#65475,#65476,#65477,
#65478,#65479,#65480,#65481,#65482,#65483,#65484,#65485,#65486,#65487,#65488,
#65489,#65490,#65491,#65492,#65493,#65494,#65495,#65496,#65497,#65498,#65499,
#65500,#65501)),.UNSPECIFIED.,.F.,.F.,.F.,(4,4),(4,1,1,1,1,1,1,1,1,1,1,
1,1,1,1,1,1,1,1,1,1,1,1,1,1,1,1,1,1,1,1,1,1,1,1,1,1,1,1,1,1,1,1,1,1,1,1,
1,1,1,1,1,1,4),(0.,0.032158409993862),(14.3984001269719,15.3849294656359,
16.3714588042999,17.357988142964,18.344517481628,19.331046820292,20.317576158956,
21.3041054976201,22.2906348362841,23.2771641749481,24.2636935136122,25.2502228522762,
26.2367521909402,27.2232815296043,28.2098108682683,29.1963402069323,30.1828695455963,
31.1693988842604,32.1559282229244,33.1424575615884,34.1289869002525,35.1155162389165,
36.1020455775805,37.0885749162446,38.0751042549086,39.0616335935726,40.0481629322367,
41.0346922709007,42.0212216095647,43.0077509482287,43.9942802868928,44.9808096255568,
45.9673389642208,46.9538683028849,47.9403976415489,48.9269269802129,49.913456318877,
50.899985657541,51.886514996205,52.873044334869,53.8595736735331,54.8461030121971,
55.8326323508611,56.8191616895252,57.8056910281892,58.7922203668532,59.7787497055173,
60.7652790441813,61.7518083828453,62.7383377215094,63.7248670601734,64.7113963988374,
65.6979257375014,66.6844550761655),.UNSPECIFIED.);
#658=B_SPLINE_SURFACE_WITH_KNOTS('',3,3,((#65709,#65710,#65711,#65712,#65713,
#65714,#65715,#65716,#65717,#65718,#65719,#65720,#65721,#65722,#65723,#65724,
#65725,#65726,#65727,#65728,#65729,#65730,#65731,#65732,#65733,#65734,#65735,
#65736,#65737,#65738,#65739,#65740,#65741,#65742,#65743,#65744,#65745,#65746,
#65747,#65748,#65749,#65750,#65751,#65752,#65753,#65754,#65755,#65756,#65757,
#65758,#65759,#65760,#65761,#65762,#65763,#65764),(#65765,#65766,#65767,
#65768,#65769,#65770,#65771,#65772,#65773,#65774,#65775,#65776,#65777,#65778,
#65779,#65780,#65781,#65782,#65783,#65784,#65785,#65786,#65787,#65788,#65789,
#65790,#65791,#65792,#65793,#65794,#65795,#65796,#65797,#65798,#65799,#65800,
#65801,#65802,#65803,#65804,#65805,#65806,#65807,#65808,#65809,#65810,#65811,
#65812,#65813,#65814,#65815,#65816,#65817,#65818,#65819,#65820),(#65821,
#65822,#65823,#65824,#65825,#65826,#65827,#65828,#65829,#65830,#65831,#65832,
#65833,#65834,#65835,#65836,#65837,#65838,#65839,#65840,#65841,#65842,#65843,
#65844,#65845,#65846,#65847,#65848,#65849,#65850,#65851,#65852,#65853,#65854,
#65855,#65856,#65857,#65858,#65859,#65860,#65861,#65862,#65863,#65864,#65865,
#65866,#65867,#65868,#65869,#65870,#65871,#65872,#65873,#65874,#65875,#65876),
(#65877,#65878,#65879,#65880,#65881,#65882,#65883,#65884,#65885,#65886,
#65887,#65888,#65889,#65890,#65891,#65892,#65893,#65894,#65895,#65896,#65897,
#65898,#65899,#65900,#65901,#65902,#65903,#65904,#65905,#65906,#65907,#65908,
#65909,#65910,#65911,#65912,#65913,#65914,#65915,#65916,#65917,#65918,#65919,
#65920,#65921,#65922,#65923,#65924,#65925,#65926,#65927,#65928,#65929,#65930,
#65931,#65932)),.UNSPECIFIED.,.F.,.F.,.F.,(4,4),(4,1,1,1,1,1,1,1,1,1,1,
1,1,1,1,1,1,1,1,1,1,1,1,1,1,1,1,1,1,1,1,1,1,1,1,1,1,1,1,1,1,1,1,1,1,1,1,
1,1,1,1,1,1,4),(0.,0.0321584099938627),(11.8553612635794,12.8418906022434,
13.8284199409074,14.8149492795714,15.8014786182355,16.7880079568995,17.7745372955635,
18.7610666342276,19.7475959728916,20.7341253115556,21.7206546502197,22.7071839888837,
23.6937133275477,24.6802426662118,25.6667720048758,26.6533013435398,27.6398306822038,
28.6263600208679,29.6128893595319,30.5994186981959,31.58594803686,32.572477375524,
33.559006714188,34.5455360528521,35.5320653915161,36.5185947301801,37.5051240688441,
38.4916534075082,39.4781827461722,40.4647120848362,41.4512414235003,42.4377707621643,
43.4243001008283,44.4108294394924,45.3973587781564,46.3838881168204,47.3704174554844,
48.3569467941485,49.3434761328125,50.3300054714765,51.3165348101406,52.3030641488046,
53.2895934874686,54.2761228261327,55.2626521647967,56.2491815034607,57.2357108421248,
58.2222401807888,59.2087695194528,60.1952988581168,61.1818281967809,62.1683575354449,
63.1548868741089,64.141416212773),.UNSPECIFIED.);
#659=B_SPLINE_SURFACE_WITH_KNOTS('',3,3,((#65958,#65959,#65960,#65961,#65962,
#65963,#65964,#65965,#65966,#65967,#65968,#65969,#65970,#65971,#65972,#65973,
#65974,#65975,#65976,#65977,#65978,#65979,#65980,#65981,#65982,#65983,#65984,
#65985,#65986,#65987,#65988,#65989,#65990,#65991,#65992,#65993,#65994,#65995,
#65996,#65997,#65998,#65999,#66000,#66001,#66002,#66003,#66004,#66005,#66006,
#66007,#66008,#66009,#66010,#66011,#66012,#66013),(#66014,#66015,#66016,
#66017,#66018,#66019,#66020,#66021,#66022,#66023,#66024,#66025,#66026,#66027,
#66028,#66029,#66030,#66031,#66032,#66033,#66034,#66035,#66036,#66037,#66038,
#66039,#66040,#66041,#66042,#66043,#66044,#66045,#66046,#66047,#66048,#66049,
#66050,#66051,#66052,#66053,#66054,#66055,#66056,#66057,#66058,#66059,#66060,
#66061,#66062,#66063,#66064,#66065,#66066,#66067,#66068,#66069),(#66070,
#66071,#66072,#66073,#66074,#66075,#66076,#66077,#66078,#66079,#66080,#66081,
#66082,#66083,#66084,#66085,#66086,#66087,#66088,#66089,#66090,#66091,#66092,
#66093,#66094,#66095,#66096,#66097,#66098,#66099,#66100,#66101,#66102,#66103,
#66104,#66105,#66106,#66107,#66108,#66109,#66110,#66111,#66112,#66113,#66114,
#66115,#66116,#66117,#66118,#66119,#66120,#66121,#66122,#66123,#66124,#66125),
(#66126,#66127,#66128,#66129,#66130,#66131,#66132,#66133,#66134,#66135,
#66136,#66137,#66138,#66139,#66140,#66141,#66142,#66143,#66144,#66145,#66146,
#66147,#66148,#66149,#66150,#66151,#66152,#66153,#66154,#66155,#66156,#66157,
#66158,#66159,#66160,#66161,#66162,#66163,#66164,#66165,#66166,#66167,#66168,
#66169,#66170,#66171,#66172,#66173,#66174,#66175,#66176,#66177,#66178,#66179,
#66180,#66181)),.UNSPECIFIED.,.F.,.F.,.F.,(4,4),(4,1,1,1,1,1,1,1,1,1,1,
1,1,1,1,1,1,1,1,1,1,1,1,1,1,1,1,1,1,1,1,1,1,1,1,1,1,1,1,1,1,1,1,1,1,1,1,
1,1,1,1,1,1,4),(0.,0.0321584099938627),(14.3984001269719,15.3849294656359,
16.3714588042999,17.357988142964,18.344517481628,19.331046820292,20.317576158956,
21.3041054976201,22.2906348362841,23.2771641749481,24.2636935136122,25.2502228522762,
26.2367521909402,27.2232815296043,28.2098108682683,29.1963402069323,30.1828695455963,
31.1693988842604,32.1559282229244,33.1424575615884,34.1289869002525,35.1155162389165,
36.1020455775805,37.0885749162446,38.0751042549086,39.0616335935726,40.0481629322367,
41.0346922709007,42.0212216095647,43.0077509482287,43.9942802868928,44.9808096255568,
45.9673389642208,46.9538683028849,47.9403976415489,48.9269269802129,49.913456318877,
50.899985657541,51.886514996205,52.873044334869,53.8595736735331,54.8461030121971,
55.8326323508611,56.8191616895252,57.8056910281892,58.7922203668532,59.7787497055173,
60.7652790441813,61.7518083828453,62.7383377215094,63.7248670601734,64.7113963988374,
65.6979257375014,66.6844550761655),.UNSPECIFIED.);
#660=B_SPLINE_SURFACE_WITH_KNOTS('',3,3,((#66389,#66390,#66391,#66392,#66393,
#66394,#66395,#66396,#66397,#66398,#66399,#66400,#66401,#66402,#66403,#66404,
#66405,#66406,#66407,#66408,#66409,#66410,#66411,#66412,#66413,#66414,#66415,
#66416,#66417,#66418,#66419,#66420,#66421,#66422,#66423,#66424,#66425,#66426,
#66427,#66428,#66429,#66430,#66431,#66432,#66433,#66434,#66435,#66436,#66437,
#66438,#66439,#66440,#66441,#66442,#66443,#66444),(#66445,#66446,#66447,
#66448,#66449,#66450,#66451,#66452,#66453,#66454,#66455,#66456,#66457,#66458,
#66459,#66460,#66461,#66462,#66463,#66464,#66465,#66466,#66467,#66468,#66469,
#66470,#66471,#66472,#66473,#66474,#66475,#66476,#66477,#66478,#66479,#66480,
#66481,#66482,#66483,#66484,#66485,#66486,#66487,#66488,#66489,#66490,#66491,
#66492,#66493,#66494,#66495,#66496,#66497,#66498,#66499,#66500),(#66501,
#66502,#66503,#66504,#66505,#66506,#66507,#66508,#66509,#66510,#66511,#66512,
#66513,#66514,#66515,#66516,#66517,#66518,#66519,#66520,#66521,#66522,#66523,
#66524,#66525,#66526,#66527,#66528,#66529,#66530,#66531,#66532,#66533,#66534,
#66535,#66536,#66537,#66538,#66539,#66540,#66541,#66542,#66543,#66544,#66545,
#66546,#66547,#66548,#66549,#66550,#66551,#66552,#66553,#66554,#66555,#66556),
(#66557,#66558,#66559,#66560,#66561,#66562,#66563,#66564,#66565,#66566,
#66567,#66568,#66569,#66570,#66571,#66572,#66573,#66574,#66575,#66576,#66577,
#66578,#66579,#66580,#66581,#66582,#66583,#66584,#66585,#66586,#66587,#66588,
#66589,#66590,#66591,#66592,#66593,#66594,#66595,#66596,#66597,#66598,#66599,
#66600,#66601,#66602,#66603,#66604,#66605,#66606,#66607,#66608,#66609,#66610,
#66611,#66612)),.UNSPECIFIED.,.F.,.F.,.F.,(4,4),(4,1,1,1,1,1,1,1,1,1,1,
1,1,1,1,1,1,1,1,1,1,1,1,1,1,1,1,1,1,1,1,1,1,1,1,1,1,1,1,1,1,1,1,1,1,1,1,
1,1,1,1,1,1,4),(0.,0.0321584099938621),(11.8553612635794,12.8418906022434,
13.8284199409074,14.8149492795714,15.8014786182355,16.7880079568995,17.7745372955635,
18.7610666342276,19.7475959728916,20.7341253115556,21.7206546502197,22.7071839888837,
23.6937133275477,24.6802426662117,25.6667720048758,26.6533013435398,27.6398306822038,
28.6263600208679,29.6128893595319,30.5994186981959,31.58594803686,32.572477375524,
33.559006714188,34.5455360528521,35.5320653915161,36.5185947301801,37.5051240688441,
38.4916534075082,39.4781827461722,40.4647120848362,41.4512414235003,42.4377707621643,
43.4243001008283,44.4108294394924,45.3973587781564,46.3838881168204,47.3704174554844,
48.3569467941485,49.3434761328125,50.3300054714765,51.3165348101406,52.3030641488046,
53.2895934874686,54.2761228261327,55.2626521647967,56.2491815034607,57.2357108421247,
58.2222401807888,59.2087695194528,60.1952988581168,61.1818281967809,62.1683575354449,
63.1548868741089,64.141416212773),.UNSPECIFIED.);
#661=B_SPLINE_SURFACE_WITH_KNOTS('',3,3,((#66638,#66639,#66640,#66641,#66642,
#66643,#66644,#66645,#66646,#66647,#66648,#66649,#66650,#66651,#66652,#66653,
#66654,#66655,#66656,#66657,#66658,#66659,#66660,#66661,#66662,#66663,#66664,
#66665,#66666,#66667,#66668,#66669,#66670,#66671,#66672,#66673,#66674,#66675,
#66676,#66677,#66678,#66679,#66680,#66681,#66682,#66683,#66684,#66685,#66686,
#66687,#66688,#66689,#66690,#66691,#66692,#66693),(#66694,#66695,#66696,
#66697,#66698,#66699,#66700,#66701,#66702,#66703,#66704,#66705,#66706,#66707,
#66708,#66709,#66710,#66711,#66712,#66713,#66714,#66715,#66716,#66717,#66718,
#66719,#66720,#66721,#66722,#66723,#66724,#66725,#66726,#66727,#66728,#66729,
#66730,#66731,#66732,#66733,#66734,#66735,#66736,#66737,#66738,#66739,#66740,
#66741,#66742,#66743,#66744,#66745,#66746,#66747,#66748,#66749),(#66750,
#66751,#66752,#66753,#66754,#66755,#66756,#66757,#66758,#66759,#66760,#66761,
#66762,#66763,#66764,#66765,#66766,#66767,#66768,#66769,#66770,#66771,#66772,
#66773,#66774,#66775,#66776,#66777,#66778,#66779,#66780,#66781,#66782,#66783,
#66784,#66785,#66786,#66787,#66788,#66789,#66790,#66791,#66792,#66793,#66794,
#66795,#66796,#66797,#66798,#66799,#66800,#66801,#66802,#66803,#66804,#66805),
(#66806,#66807,#66808,#66809,#66810,#66811,#66812,#66813,#66814,#66815,
#66816,#66817,#66818,#66819,#66820,#66821,#66822,#66823,#66824,#66825,#66826,
#66827,#66828,#66829,#66830,#66831,#66832,#66833,#66834,#66835,#66836,#66837,
#66838,#66839,#66840,#66841,#66842,#66843,#66844,#66845,#66846,#66847,#66848,
#66849,#66850,#66851,#66852,#66853,#66854,#66855,#66856,#66857,#66858,#66859,
#66860,#66861)),.UNSPECIFIED.,.F.,.F.,.F.,(4,4),(4,1,1,1,1,1,1,1,1,1,1,
1,1,1,1,1,1,1,1,1,1,1,1,1,1,1,1,1,1,1,1,1,1,1,1,1,1,1,1,1,1,1,1,1,1,1,1,
1,1,1,1,1,1,4),(0.,0.0321584099938621),(14.3984001269719,15.3849294656359,
16.3714588042999,17.357988142964,18.344517481628,19.331046820292,20.317576158956,
21.3041054976201,22.2906348362841,23.2771641749481,24.2636935136122,25.2502228522762,
26.2367521909402,27.2232815296043,28.2098108682683,29.1963402069323,30.1828695455963,
31.1693988842604,32.1559282229244,33.1424575615884,34.1289869002525,35.1155162389165,
36.1020455775805,37.0885749162446,38.0751042549086,39.0616335935726,40.0481629322367,
41.0346922709007,42.0212216095647,43.0077509482287,43.9942802868928,44.9808096255568,
45.9673389642208,46.9538683028849,47.9403976415489,48.9269269802129,49.913456318877,
50.899985657541,51.886514996205,52.873044334869,53.8595736735331,54.8461030121971,
55.8326323508611,56.8191616895252,57.8056910281892,58.7922203668532,59.7787497055173,
60.7652790441813,61.7518083828453,62.7383377215094,63.7248670601734,64.7113963988374,
65.6979257375014,66.6844550761655),.UNSPECIFIED.);
#662=B_SPLINE_SURFACE_WITH_KNOTS('',3,3,((#67069,#67070,#67071,#67072,#67073,
#67074,#67075,#67076,#67077,#67078,#67079,#67080,#67081,#67082,#67083,#67084,
#67085,#67086,#67087,#67088,#67089,#67090,#67091,#67092,#67093,#67094,#67095,
#67096,#67097,#67098,#67099,#67100,#67101,#67102,#67103,#67104,#67105,#67106,
#67107,#67108,#67109,#67110,#67111,#67112,#67113,#67114,#67115,#67116,#67117,
#67118,#67119,#67120,#67121,#67122,#67123,#67124),(#67125,#67126,#67127,
#67128,#67129,#67130,#67131,#67132,#67133,#67134,#67135,#67136,#67137,#67138,
#67139,#67140,#67141,#67142,#67143,#67144,#67145,#67146,#67147,#67148,#67149,
#67150,#67151,#67152,#67153,#67154,#67155,#67156,#67157,#67158,#67159,#67160,
#67161,#67162,#67163,#67164,#67165,#67166,#67167,#67168,#67169,#67170,#67171,
#67172,#67173,#67174,#67175,#67176,#67177,#67178,#67179,#67180),(#67181,
#67182,#67183,#67184,#67185,#67186,#67187,#67188,#67189,#67190,#67191,#67192,
#67193,#67194,#67195,#67196,#67197,#67198,#67199,#67200,#67201,#67202,#67203,
#67204,#67205,#67206,#67207,#67208,#67209,#67210,#67211,#67212,#67213,#67214,
#67215,#67216,#67217,#67218,#67219,#67220,#67221,#67222,#67223,#67224,#67225,
#67226,#67227,#67228,#67229,#67230,#67231,#67232,#67233,#67234,#67235,#67236),
(#67237,#67238,#67239,#67240,#67241,#67242,#67243,#67244,#67245,#67246,
#67247,#67248,#67249,#67250,#67251,#67252,#67253,#67254,#67255,#67256,#67257,
#67258,#67259,#67260,#67261,#67262,#67263,#67264,#67265,#67266,#67267,#67268,
#67269,#67270,#67271,#67272,#67273,#67274,#67275,#67276,#67277,#67278,#67279,
#67280,#67281,#67282,#67283,#67284,#67285,#67286,#67287,#67288,#67289,#67290,
#67291,#67292)),.UNSPECIFIED.,.F.,.F.,.F.,(4,4),(4,1,1,1,1,1,1,1,1,1,1,
1,1,1,1,1,1,1,1,1,1,1,1,1,1,1,1,1,1,1,1,1,1,1,1,1,1,1,1,1,1,1,1,1,1,1,1,
1,1,1,1,1,1,4),(0.,0.032158409993862),(11.8553612635794,12.8418906022434,
13.8284199409074,14.8149492795714,15.8014786182355,16.7880079568995,17.7745372955635,
18.7610666342276,19.7475959728916,20.7341253115556,21.7206546502197,22.7071839888837,
23.6937133275477,24.6802426662118,25.6667720048758,26.6533013435398,27.6398306822039,
28.6263600208679,29.6128893595319,30.5994186981959,31.58594803686,32.572477375524,
33.559006714188,34.5455360528521,35.5320653915161,36.5185947301801,37.5051240688442,
38.4916534075082,39.4781827461722,40.4647120848363,41.4512414235003,42.4377707621643,
43.4243001008283,44.4108294394924,45.3973587781564,46.3838881168204,47.3704174554845,
48.3569467941485,49.3434761328125,50.3300054714766,51.3165348101406,52.3030641488046,
53.2895934874687,54.2761228261327,55.2626521647967,56.2491815034607,57.2357108421248,
58.2222401807888,59.2087695194528,60.1952988581169,61.1818281967809,62.1683575354449,
63.154886874109,64.141416212773),.UNSPECIFIED.);
#663=B_SPLINE_SURFACE_WITH_KNOTS('',3,3,((#67318,#67319,#67320,#67321,#67322,
#67323,#67324,#67325,#67326,#67327,#67328,#67329,#67330,#67331,#67332,#67333,
#67334,#67335,#67336,#67337,#67338,#67339,#67340,#67341,#67342,#67343,#67344,
#67345,#67346,#67347,#67348,#67349,#67350,#67351,#67352,#67353,#67354,#67355,
#67356,#67357,#67358,#67359,#67360,#67361,#67362,#67363,#67364,#67365,#67366,
#67367,#67368,#67369,#67370,#67371,#67372,#67373),(#67374,#67375,#67376,
#67377,#67378,#67379,#67380,#67381,#67382,#67383,#67384,#67385,#67386,#67387,
#67388,#67389,#67390,#67391,#67392,#67393,#67394,#67395,#67396,#67397,#67398,
#67399,#67400,#67401,#67402,#67403,#67404,#67405,#67406,#67407,#67408,#67409,
#67410,#67411,#67412,#67413,#67414,#67415,#67416,#67417,#67418,#67419,#67420,
#67421,#67422,#67423,#67424,#67425,#67426,#67427,#67428,#67429),(#67430,
#67431,#67432,#67433,#67434,#67435,#67436,#67437,#67438,#67439,#67440,#67441,
#67442,#67443,#67444,#67445,#67446,#67447,#67448,#67449,#67450,#67451,#67452,
#67453,#67454,#67455,#67456,#67457,#67458,#67459,#67460,#67461,#67462,#67463,
#67464,#67465,#67466,#67467,#67468,#67469,#67470,#67471,#67472,#67473,#67474,
#67475,#67476,#67477,#67478,#67479,#67480,#67481,#67482,#67483,#67484,#67485),
(#67486,#67487,#67488,#67489,#67490,#67491,#67492,#67493,#67494,#67495,
#67496,#67497,#67498,#67499,#67500,#67501,#67502,#67503,#67504,#67505,#67506,
#67507,#67508,#67509,#67510,#67511,#67512,#67513,#67514,#67515,#67516,#67517,
#67518,#67519,#67520,#67521,#67522,#67523,#67524,#67525,#67526,#67527,#67528,
#67529,#67530,#67531,#67532,#67533,#67534,#67535,#67536,#67537,#67538,#67539,
#67540,#67541)),.UNSPECIFIED.,.F.,.F.,.F.,(4,4),(4,1,1,1,1,1,1,1,1,1,1,
1,1,1,1,1,1,1,1,1,1,1,1,1,1,1,1,1,1,1,1,1,1,1,1,1,1,1,1,1,1,1,1,1,1,1,1,
1,1,1,1,1,1,4),(0.,0.032158409993862),(14.3984001269719,15.3849294656359,
16.3714588042999,17.357988142964,18.344517481628,19.331046820292,20.317576158956,
21.3041054976201,22.2906348362841,23.2771641749481,24.2636935136122,25.2502228522762,
26.2367521909402,27.2232815296043,28.2098108682683,29.1963402069323,30.1828695455964,
31.1693988842604,32.1559282229244,33.1424575615884,34.1289869002525,35.1155162389165,
36.1020455775805,37.0885749162446,38.0751042549086,39.0616335935726,40.0481629322367,
41.0346922709007,42.0212216095647,43.0077509482288,43.9942802868928,44.9808096255568,
45.9673389642208,46.9538683028849,47.9403976415489,48.9269269802129,49.913456318877,
50.899985657541,51.886514996205,52.8730443348691,53.8595736735331,54.8461030121971,
55.8326323508612,56.8191616895252,57.8056910281892,58.7922203668532,59.7787497055173,
60.7652790441813,61.7518083828453,62.7383377215094,63.7248670601734,64.7113963988374,
65.6979257375015,66.6844550761655),.UNSPECIFIED.);
#664=B_SPLINE_SURFACE_WITH_KNOTS('',3,3,((#67749,#67750,#67751,#67752,#67753,
#67754,#67755,#67756,#67757,#67758,#67759,#67760,#67761,#67762,#67763,#67764,
#67765,#67766,#67767,#67768,#67769,#67770,#67771,#67772,#67773,#67774,#67775,
#67776,#67777,#67778,#67779,#67780,#67781,#67782,#67783,#67784,#67785,#67786,
#67787,#67788,#67789,#67790,#67791,#67792,#67793,#67794,#67795,#67796,#67797,
#67798,#67799,#67800,#67801,#67802,#67803,#67804),(#67805,#67806,#67807,
#67808,#67809,#67810,#67811,#67812,#67813,#67814,#67815,#67816,#67817,#67818,
#67819,#67820,#67821,#67822,#67823,#67824,#67825,#67826,#67827,#67828,#67829,
#67830,#67831,#67832,#67833,#67834,#67835,#67836,#67837,#67838,#67839,#67840,
#67841,#67842,#67843,#67844,#67845,#67846,#67847,#67848,#67849,#67850,#67851,
#67852,#67853,#67854,#67855,#67856,#67857,#67858,#67859,#67860),(#67861,
#67862,#67863,#67864,#67865,#67866,#67867,#67868,#67869,#67870,#67871,#67872,
#67873,#67874,#67875,#67876,#67877,#67878,#67879,#67880,#67881,#67882,#67883,
#67884,#67885,#67886,#67887,#67888,#67889,#67890,#67891,#67892,#67893,#67894,
#67895,#67896,#67897,#67898,#67899,#67900,#67901,#67902,#67903,#67904,#67905,
#67906,#67907,#67908,#67909,#67910,#67911,#67912,#67913,#67914,#67915,#67916),
(#67917,#67918,#67919,#67920,#67921,#67922,#67923,#67924,#67925,#67926,
#67927,#67928,#67929,#67930,#67931,#67932,#67933,#67934,#67935,#67936,#67937,
#67938,#67939,#67940,#67941,#67942,#67943,#67944,#67945,#67946,#67947,#67948,
#67949,#67950,#67951,#67952,#67953,#67954,#67955,#67956,#67957,#67958,#67959,
#67960,#67961,#67962,#67963,#67964,#67965,#67966,#67967,#67968,#67969,#67970,
#67971,#67972)),.UNSPECIFIED.,.F.,.F.,.F.,(4,4),(4,1,1,1,1,1,1,1,1,1,1,
1,1,1,1,1,1,1,1,1,1,1,1,1,1,1,1,1,1,1,1,1,1,1,1,1,1,1,1,1,1,1,1,1,1,1,1,
1,1,1,1,1,1,4),(0.,0.0321584099938627),(11.8553612635793,12.8418906022434,
13.8284199409074,14.8149492795714,15.8014786182354,16.7880079568995,17.7745372955635,
18.7610666342275,19.7475959728916,20.7341253115556,21.7206546502196,22.7071839888837,
23.6937133275477,24.6802426662117,25.6667720048758,26.6533013435398,27.6398306822038,
28.6263600208678,29.6128893595319,30.5994186981959,31.5859480368599,32.572477375524,
33.559006714188,34.545536052852,35.5320653915161,36.5185947301801,37.5051240688441,
38.4916534075082,39.4781827461722,40.4647120848362,41.4512414235002,42.4377707621643,
43.4243001008283,44.4108294394923,45.3973587781564,46.3838881168204,47.3704174554844,
48.3569467941485,49.3434761328125,50.3300054714765,51.3165348101405,52.3030641488046,
53.2895934874686,54.2761228261326,55.2626521647967,56.2491815034607,57.2357108421247,
58.2222401807888,59.2087695194528,60.1952988581168,61.1818281967808,62.1683575354449,
63.1548868741089,64.1414162127729),.UNSPECIFIED.);
#665=B_SPLINE_SURFACE_WITH_KNOTS('',3,3,((#67998,#67999,#68000,#68001,#68002,
#68003,#68004,#68005,#68006,#68007,#68008,#68009,#68010,#68011,#68012,#68013,
#68014,#68015,#68016,#68017,#68018,#68019,#68020,#68021,#68022,#68023,#68024,
#68025,#68026,#68027,#68028,#68029,#68030,#68031,#68032,#68033,#68034,#68035,
#68036,#68037,#68038,#68039,#68040,#68041,#68042,#68043,#68044,#68045,#68046,
#68047,#68048,#68049,#68050,#68051,#68052,#68053),(#68054,#68055,#68056,
#68057,#68058,#68059,#68060,#68061,#68062,#68063,#68064,#68065,#68066,#68067,
#68068,#68069,#68070,#68071,#68072,#68073,#68074,#68075,#68076,#68077,#68078,
#68079,#68080,#68081,#68082,#68083,#68084,#68085,#68086,#68087,#68088,#68089,
#68090,#68091,#68092,#68093,#68094,#68095,#68096,#68097,#68098,#68099,#68100,
#68101,#68102,#68103,#68104,#68105,#68106,#68107,#68108,#68109),(#68110,
#68111,#68112,#68113,#68114,#68115,#68116,#68117,#68118,#68119,#68120,#68121,
#68122,#68123,#68124,#68125,#68126,#68127,#68128,#68129,#68130,#68131,#68132,
#68133,#68134,#68135,#68136,#68137,#68138,#68139,#68140,#68141,#68142,#68143,
#68144,#68145,#68146,#68147,#68148,#68149,#68150,#68151,#68152,#68153,#68154,
#68155,#68156,#68157,#68158,#68159,#68160,#68161,#68162,#68163,#68164,#68165),
(#68166,#68167,#68168,#68169,#68170,#68171,#68172,#68173,#68174,#68175,
#68176,#68177,#68178,#68179,#68180,#68181,#68182,#68183,#68184,#68185,#68186,
#68187,#68188,#68189,#68190,#68191,#68192,#68193,#68194,#68195,#68196,#68197,
#68198,#68199,#68200,#68201,#68202,#68203,#68204,#68205,#68206,#68207,#68208,
#68209,#68210,#68211,#68212,#68213,#68214,#68215,#68216,#68217,#68218,#68219,
#68220,#68221)),.UNSPECIFIED.,.F.,.F.,.F.,(4,4),(4,1,1,1,1,1,1,1,1,1,1,
1,1,1,1,1,1,1,1,1,1,1,1,1,1,1,1,1,1,1,1,1,1,1,1,1,1,1,1,1,1,1,1,1,1,1,1,
1,1,1,1,1,1,4),(0.,0.0321584099938627),(14.3984001269718,15.3849294656359,
16.3714588042999,17.3579881429639,18.344517481628,19.331046820292,20.317576158956,
21.30410549762,22.2906348362841,23.2771641749481,24.2636935136121,25.2502228522762,
26.2367521909402,27.2232815296042,28.2098108682683,29.1963402069323,30.1828695455963,
31.1693988842603,32.1559282229244,33.1424575615884,34.1289869002524,35.1155162389165,
36.1020455775805,37.0885749162445,38.0751042549086,39.0616335935726,40.0481629322366,
41.0346922709006,42.0212216095647,43.0077509482287,43.9942802868927,44.9808096255568,
45.9673389642208,46.9538683028848,47.9403976415489,48.9269269802129,49.9134563188769,
50.899985657541,51.886514996205,52.873044334869,53.859573673533,54.8461030121971,
55.8326323508611,56.8191616895251,57.8056910281892,58.7922203668532,59.7787497055172,
60.7652790441813,61.7518083828453,62.7383377215093,63.7248670601733,64.7113963988374,
65.6979257375014,66.6844550761654),.UNSPECIFIED.);
#666=B_SPLINE_SURFACE_WITH_KNOTS('',3,3,((#68449,#68450,#68451,#68452,#68453,
#68454,#68455,#68456,#68457,#68458,#68459,#68460,#68461,#68462,#68463,#68464,
#68465,#68466,#68467,#68468,#68469,#68470,#68471,#68472,#68473,#68474,#68475,
#68476,#68477,#68478,#68479,#68480,#68481,#68482,#68483,#68484,#68485,#68486,
#68487,#68488,#68489,#68490,#68491,#68492,#68493,#68494,#68495,#68496,#68497,
#68498,#68499,#68500,#68501,#68502,#68503,#68504),(#68505,#68506,#68507,
#68508,#68509,#68510,#68511,#68512,#68513,#68514,#68515,#68516,#68517,#68518,
#68519,#68520,#68521,#68522,#68523,#68524,#68525,#68526,#68527,#68528,#68529,
#68530,#68531,#68532,#68533,#68534,#68535,#68536,#68537,#68538,#68539,#68540,
#68541,#68542,#68543,#68544,#68545,#68546,#68547,#68548,#68549,#68550,#68551,
#68552,#68553,#68554,#68555,#68556,#68557,#68558,#68559,#68560),(#68561,
#68562,#68563,#68564,#68565,#68566,#68567,#68568,#68569,#68570,#68571,#68572,
#68573,#68574,#68575,#68576,#68577,#68578,#68579,#68580,#68581,#68582,#68583,
#68584,#68585,#68586,#68587,#68588,#68589,#68590,#68591,#68592,#68593,#68594,
#68595,#68596,#68597,#68598,#68599,#68600,#68601,#68602,#68603,#68604,#68605,
#68606,#68607,#68608,#68609,#68610,#68611,#68612,#68613,#68614,#68615,#68616),
(#68617,#68618,#68619,#68620,#68621,#68622,#68623,#68624,#68625,#68626,
#68627,#68628,#68629,#68630,#68631,#68632,#68633,#68634,#68635,#68636,#68637,
#68638,#68639,#68640,#68641,#68642,#68643,#68644,#68645,#68646,#68647,#68648,
#68649,#68650,#68651,#68652,#68653,#68654,#68655,#68656,#68657,#68658,#68659,
#68660,#68661,#68662,#68663,#68664,#68665,#68666,#68667,#68668,#68669,#68670,
#68671,#68672)),.UNSPECIFIED.,.F.,.F.,.F.,(4,4),(4,1,1,1,1,1,1,1,1,1,1,
1,1,1,1,1,1,1,1,1,1,1,1,1,1,1,1,1,1,1,1,1,1,1,1,1,1,1,1,1,1,1,1,1,1,1,1,
1,1,1,1,1,1,4),(0.,0.0321584099938621),(11.8553612635793,12.8418906022434,
13.8284199409074,14.8149492795714,15.8014786182355,16.7880079568995,17.7745372955635,
18.7610666342275,19.7475959728916,20.7341253115556,21.7206546502196,22.7071839888837,
23.6937133275477,24.6802426662117,25.6667720048758,26.6533013435398,27.6398306822038,
28.6263600208679,29.6128893595319,30.5994186981959,31.5859480368599,32.572477375524,
33.559006714188,34.545536052852,35.5320653915161,36.5185947301801,37.5051240688441,
38.4916534075082,39.4781827461722,40.4647120848362,41.4512414235002,42.4377707621643,
43.4243001008283,44.4108294394923,45.3973587781564,46.3838881168204,47.3704174554844,
48.3569467941485,49.3434761328125,50.3300054714765,51.3165348101406,52.3030641488046,
53.2895934874686,54.2761228261326,55.2626521647967,56.2491815034607,57.2357108421247,
58.2222401807888,59.2087695194528,60.1952988581168,61.1818281967809,62.1683575354449,
63.1548868741089,64.141416212773),.UNSPECIFIED.);
#667=B_SPLINE_SURFACE_WITH_KNOTS('',3,3,((#68780,#68781,#68782,#68783,#68784,
#68785,#68786,#68787,#68788,#68789,#68790,#68791,#68792,#68793,#68794,#68795,
#68796,#68797,#68798,#68799,#68800,#68801,#68802,#68803,#68804,#68805,#68806,
#68807,#68808,#68809,#68810,#68811,#68812,#68813,#68814,#68815,#68816,#68817,
#68818,#68819,#68820,#68821,#68822,#68823,#68824,#68825,#68826,#68827,#68828,
#68829,#68830,#68831,#68832,#68833,#68834,#68835),(#68836,#68837,#68838,
#68839,#68840,#68841,#68842,#68843,#68844,#68845,#68846,#68847,#68848,#68849,
#68850,#68851,#68852,#68853,#68854,#68855,#68856,#68857,#68858,#68859,#68860,
#68861,#68862,#68863,#68864,#68865,#68866,#68867,#68868,#68869,#68870,#68871,
#68872,#68873,#68874,#68875,#68876,#68877,#68878,#68879,#68880,#68881,#68882,
#68883,#68884,#68885,#68886,#68887,#68888,#68889,#68890,#68891),(#68892,
#68893,#68894,#68895,#68896,#68897,#68898,#68899,#68900,#68901,#68902,#68903,
#68904,#68905,#68906,#68907,#68908,#68909,#68910,#68911,#68912,#68913,#68914,
#68915,#68916,#68917,#68918,#68919,#68920,#68921,#68922,#68923,#68924,#68925,
#68926,#68927,#68928,#68929,#68930,#68931,#68932,#68933,#68934,#68935,#68936,
#68937,#68938,#68939,#68940,#68941,#68942,#68943,#68944,#68945,#68946,#68947),
(#68948,#68949,#68950,#68951,#68952,#68953,#68954,#68955,#68956,#68957,
#68958,#68959,#68960,#68961,#68962,#68963,#68964,#68965,#68966,#68967,#68968,
#68969,#68970,#68971,#68972,#68973,#68974,#68975,#68976,#68977,#68978,#68979,
#68980,#68981,#68982,#68983,#68984,#68985,#68986,#68987,#68988,#68989,#68990,
#68991,#68992,#68993,#68994,#68995,#68996,#68997,#68998,#68999,#69000,#69001,
#69002,#69003)),.UNSPECIFIED.,.F.,.F.,.F.,(4,4),(4,1,1,1,1,1,1,1,1,1,1,
1,1,1,1,1,1,1,1,1,1,1,1,1,1,1,1,1,1,1,1,1,1,1,1,1,1,1,1,1,1,1,1,1,1,1,1,
1,1,1,1,1,1,4),(0.,0.0321584099938621),(14.3984001269718,15.3849294656359,
16.3714588042999,17.3579881429639,18.344517481628,19.331046820292,20.317576158956,
21.3041054976201,22.2906348362841,23.2771641749481,24.2636935136121,25.2502228522762,
26.2367521909402,27.2232815296042,28.2098108682683,29.1963402069323,30.1828695455963,
31.1693988842604,32.1559282229244,33.1424575615884,34.1289869002525,35.1155162389165,
36.1020455775805,37.0885749162445,38.0751042549086,39.0616335935726,40.0481629322366,
41.0346922709007,42.0212216095647,43.0077509482287,43.9942802868928,44.9808096255568,
45.9673389642208,46.9538683028849,47.9403976415489,48.9269269802129,49.9134563188769,
50.899985657541,51.886514996205,52.873044334869,53.8595736735331,54.8461030121971,
55.8326323508611,56.8191616895252,57.8056910281892,58.7922203668532,59.7787497055173,
60.7652790441813,61.7518083828453,62.7383377215094,63.7248670601734,64.7113963988374,
65.6979257375014,66.6844550761655),.UNSPECIFIED.);
#668=B_SPLINE_SURFACE_WITH_KNOTS('',3,3,((#69294,#69295,#69296,#69297,#69298,
#69299,#69300,#69301,#69302,#69303,#69304,#69305,#69306,#69307,#69308,#69309,
#69310,#69311,#69312,#69313,#69314,#69315,#69316,#69317,#69318,#69319,#69320,
#69321,#69322,#69323,#69324,#69325,#69326,#69327,#69328,#69329,#69330,#69331,
#69332,#69333,#69334,#69335,#69336,#69337,#69338,#69339,#69340,#69341,#69342,
#69343,#69344,#69345,#69346,#69347,#69348,#69349),(#69350,#69351,#69352,
#69353,#69354,#69355,#69356,#69357,#69358,#69359,#69360,#69361,#69362,#69363,
#69364,#69365,#69366,#69367,#69368,#69369,#69370,#69371,#69372,#69373,#69374,
#69375,#69376,#69377,#69378,#69379,#69380,#69381,#69382,#69383,#69384,#69385,
#69386,#69387,#69388,#69389,#69390,#69391,#69392,#69393,#69394,#69395,#69396,
#69397,#69398,#69399,#69400,#69401,#69402,#69403,#69404,#69405),(#69406,
#69407,#69408,#69409,#69410,#69411,#69412,#69413,#69414,#69415,#69416,#69417,
#69418,#69419,#69420,#69421,#69422,#69423,#69424,#69425,#69426,#69427,#69428,
#69429,#69430,#69431,#69432,#69433,#69434,#69435,#69436,#69437,#69438,#69439,
#69440,#69441,#69442,#69443,#69444,#69445,#69446,#69447,#69448,#69449,#69450,
#69451,#69452,#69453,#69454,#69455,#69456,#69457,#69458,#69459,#69460,#69461),
(#69462,#69463,#69464,#69465,#69466,#69467,#69468,#69469,#69470,#69471,
#69472,#69473,#69474,#69475,#69476,#69477,#69478,#69479,#69480,#69481,#69482,
#69483,#69484,#69485,#69486,#69487,#69488,#69489,#69490,#69491,#69492,#69493,
#69494,#69495,#69496,#69497,#69498,#69499,#69500,#69501,#69502,#69503,#69504,
#69505,#69506,#69507,#69508,#69509,#69510,#69511,#69512,#69513,#69514,#69515,
#69516,#69517)),.UNSPECIFIED.,.F.,.F.,.F.,(4,4),(4,1,1,1,1,1,1,1,1,1,1,
1,1,1,1,1,1,1,1,1,1,1,1,1,1,1,1,1,1,1,1,1,1,1,1,1,1,1,1,1,1,1,1,1,1,1,1,
1,1,1,1,1,1,4),(0.,0.0321584099938621),(11.8553612635794,12.8418906022434,
13.8284199409074,14.8149492795714,15.8014786182355,16.7880079568995,17.7745372955635,
18.7610666342276,19.7475959728916,20.7341253115556,21.7206546502197,22.7071839888837,
23.6937133275477,24.6802426662117,25.6667720048758,26.6533013435398,27.6398306822038,
28.6263600208679,29.6128893595319,30.5994186981959,31.58594803686,32.572477375524,
33.559006714188,34.5455360528521,35.5320653915161,36.5185947301801,37.5051240688441,
38.4916534075082,39.4781827461722,40.4647120848362,41.4512414235003,42.4377707621643,
43.4243001008283,44.4108294394924,45.3973587781564,46.3838881168204,47.3704174554844,
48.3569467941485,49.3434761328125,50.3300054714765,51.3165348101406,52.3030641488046,
53.2895934874686,54.2761228261327,55.2626521647967,56.2491815034607,57.2357108421248,
58.2222401807888,59.2087695194528,60.1952988581168,61.1818281967809,62.1683575354449,
63.1548868741089,64.141416212773),.UNSPECIFIED.);
#669=B_SPLINE_SURFACE_WITH_KNOTS('',3,3,((#69543,#69544,#69545,#69546,#69547,
#69548,#69549,#69550,#69551,#69552,#69553,#69554,#69555,#69556,#69557,#69558,
#69559,#69560,#69561,#69562,#69563,#69564,#69565,#69566,#69567,#69568,#69569,
#69570,#69571,#69572,#69573,#69574,#69575,#69576,#69577,#69578,#69579,#69580,
#69581,#69582,#69583,#69584,#69585,#69586,#69587,#69588,#69589,#69590,#69591,
#69592,#69593,#69594,#69595,#69596,#69597,#69598),(#69599,#69600,#69601,
#69602,#69603,#69604,#69605,#69606,#69607,#69608,#69609,#69610,#69611,#69612,
#69613,#69614,#69615,#69616,#69617,#69618,#69619,#69620,#69621,#69622,#69623,
#69624,#69625,#69626,#69627,#69628,#69629,#69630,#69631,#69632,#69633,#69634,
#69635,#69636,#69637,#69638,#69639,#69640,#69641,#69642,#69643,#69644,#69645,
#69646,#69647,#69648,#69649,#69650,#69651,#69652,#69653,#69654),(#69655,
#69656,#69657,#69658,#69659,#69660,#69661,#69662,#69663,#69664,#69665,#69666,
#69667,#69668,#69669,#69670,#69671,#69672,#69673,#69674,#69675,#69676,#69677,
#69678,#69679,#69680,#69681,#69682,#69683,#69684,#69685,#69686,#69687,#69688,
#69689,#69690,#69691,#69692,#69693,#69694,#69695,#69696,#69697,#69698,#69699,
#69700,#69701,#69702,#69703,#69704,#69705,#69706,#69707,#69708,#69709,#69710),
(#69711,#69712,#69713,#69714,#69715,#69716,#69717,#69718,#69719,#69720,
#69721,#69722,#69723,#69724,#69725,#69726,#69727,#69728,#69729,#69730,#69731,
#69732,#69733,#69734,#69735,#69736,#69737,#69738,#69739,#69740,#69741,#69742,
#69743,#69744,#69745,#69746,#69747,#69748,#69749,#69750,#69751,#69752,#69753,
#69754,#69755,#69756,#69757,#69758,#69759,#69760,#69761,#69762,#69763,#69764,
#69765,#69766)),.UNSPECIFIED.,.F.,.F.,.F.,(4,4),(4,1,1,1,1,1,1,1,1,1,1,
1,1,1,1,1,1,1,1,1,1,1,1,1,1,1,1,1,1,1,1,1,1,1,1,1,1,1,1,1,1,1,1,1,1,1,1,
1,1,1,1,1,1,4),(0.,0.0321584099938621),(14.3984001269719,15.3849294656359,
16.3714588042999,17.357988142964,18.344517481628,19.331046820292,20.317576158956,
21.3041054976201,22.2906348362841,23.2771641749481,24.2636935136122,25.2502228522762,
26.2367521909402,27.2232815296043,28.2098108682683,29.1963402069323,30.1828695455963,
31.1693988842604,32.1559282229244,33.1424575615884,34.1289869002525,35.1155162389165,
36.1020455775805,37.0885749162446,38.0751042549086,39.0616335935726,40.0481629322367,
41.0346922709007,42.0212216095647,43.0077509482287,43.9942802868928,44.9808096255568,
45.9673389642208,46.9538683028849,47.9403976415489,48.9269269802129,49.913456318877,
50.899985657541,51.886514996205,52.873044334869,53.8595736735331,54.8461030121971,
55.8326323508611,56.8191616895252,57.8056910281892,58.7922203668532,59.7787497055172,
60.7652790441813,61.7518083828453,62.7383377215093,63.7248670601734,64.7113963988374,
65.6979257375014,66.6844550761655),.UNSPECIFIED.);
#1135=FACE_OUTER_BOUND('',#2150,.T.);
#1136=FACE_OUTER_BOUND('',#2151,.T.);
#1137=FACE_OUTER_BOUND('',#2152,.T.);
#1138=FACE_OUTER_BOUND('',#2153,.T.);
#1139=FACE_OUTER_BOUND('',#2154,.T.);
#1140=FACE_OUTER_BOUND('',#2155,.T.);
#1141=FACE_OUTER_BOUND('',#2156,.T.);
#1142=FACE_OUTER_BOUND('',#2157,.T.);
#1143=FACE_OUTER_BOUND('',#2158,.T.);
#1144=FACE_OUTER_BOUND('',#2159,.T.);
#1145=FACE_OUTER_BOUND('',#2160,.T.);
#1146=FACE_OUTER_BOUND('',#2161,.T.);
#1147=FACE_OUTER_BOUND('',#2162,.T.);
#1148=FACE_OUTER_BOUND('',#2163,.T.);
#1149=FACE_OUTER_BOUND('',#2164,.T.);
#1150=FACE_OUTER_BOUND('',#2165,.T.);
#1151=FACE_OUTER_BOUND('',#2166,.T.);
#1152=FACE_OUTER_BOUND('',#2167,.T.);
#1153=FACE_OUTER_BOUND('',#2168,.T.);
#1154=FACE_OUTER_BOUND('',#2169,.T.);
#1155=FACE_OUTER_BOUND('',#2170,.T.);
#1156=FACE_OUTER_BOUND('',#2171,.T.);
#1157=FACE_OUTER_BOUND('',#2172,.T.);
#1158=FACE_OUTER_BOUND('',#2173,.T.);
#1159=FACE_OUTER_BOUND('',#2174,.T.);
#1160=FACE_OUTER_BOUND('',#2175,.T.);
#1161=FACE_OUTER_BOUND('',#2176,.T.);
#1162=FACE_OUTER_BOUND('',#2177,.T.);
#1163=FACE_OUTER_BOUND('',#2178,.T.);
#1164=FACE_OUTER_BOUND('',#2179,.T.);
#1165=FACE_OUTER_BOUND('',#2180,.T.);
#1166=FACE_OUTER_BOUND('',#2181,.T.);
#1167=FACE_OUTER_BOUND('',#2182,.T.);
#1168=FACE_OUTER_BOUND('',#2183,.T.);
#1169=FACE_OUTER_BOUND('',#2184,.T.);
#1170=FACE_OUTER_BOUND('',#2185,.T.);
#1171=FACE_OUTER_BOUND('',#2186,.T.);
#1172=FACE_OUTER_BOUND('',#2187,.T.);
#1173=FACE_OUTER_BOUND('',#2188,.T.);
#1174=FACE_OUTER_BOUND('',#2189,.T.);
#1175=FACE_OUTER_BOUND('',#2190,.T.);
#1176=FACE_OUTER_BOUND('',#2191,.T.);
#1177=FACE_OUTER_BOUND('',#2192,.T.);
#1178=FACE_OUTER_BOUND('',#2193,.T.);
#1179=FACE_OUTER_BOUND('',#2194,.T.);
#1180=FACE_OUTER_BOUND('',#2195,.T.);
#1181=FACE_OUTER_BOUND('',#2196,.T.);
#1182=FACE_OUTER_BOUND('',#2197,.T.);
#1183=FACE_OUTER_BOUND('',#2198,.T.);
#1184=FACE_OUTER_BOUND('',#2199,.T.);
#1185=FACE_OUTER_BOUND('',#2200,.T.);
#1186=FACE_OUTER_BOUND('',#2201,.T.);
#1187=FACE_OUTER_BOUND('',#2202,.T.);
#1188=FACE_OUTER_BOUND('',#2203,.T.);
#1189=FACE_OUTER_BOUND('',#2204,.T.);
#1190=FACE_OUTER_BOUND('',#2205,.T.);
#1191=FACE_OUTER_BOUND('',#2206,.T.);
#1192=FACE_OUTER_BOUND('',#2207,.T.);
#1193=FACE_OUTER_BOUND('',#2208,.T.);
#1194=FACE_OUTER_BOUND('',#2209,.T.);
#1195=FACE_OUTER_BOUND('',#2210,.T.);
#1196=FACE_OUTER_BOUND('',#2211,.T.);
#1197=FACE_OUTER_BOUND('',#2212,.T.);
#1198=FACE_OUTER_BOUND('',#2213,.T.);
#1199=FACE_OUTER_BOUND('',#2214,.T.);
#1200=FACE_OUTER_BOUND('',#2215,.T.);
#1201=FACE_OUTER_BOUND('',#2216,.T.);
#1202=FACE_OUTER_BOUND('',#2217,.T.);
#1203=FACE_OUTER_BOUND('',#2218,.T.);
#1204=FACE_OUTER_BOUND('',#2219,.T.);
#1205=FACE_OUTER_BOUND('',#2220,.T.);
#1206=FACE_OUTER_BOUND('',#2221,.T.);
#1207=FACE_OUTER_BOUND('',#2222,.T.);
#1208=FACE_OUTER_BOUND('',#2223,.T.);
#1209=FACE_OUTER_BOUND('',#2224,.T.);
#1210=FACE_OUTER_BOUND('',#2225,.T.);
#1211=FACE_OUTER_BOUND('',#2226,.T.);
#1212=FACE_OUTER_BOUND('',#2227,.T.);
#1213=FACE_OUTER_BOUND('',#2228,.T.);
#1214=FACE_OUTER_BOUND('',#2229,.T.);
#1215=FACE_OUTER_BOUND('',#2230,.T.);
#1216=FACE_OUTER_BOUND('',#2231,.T.);
#1217=FACE_OUTER_BOUND('',#2232,.T.);
#1218=FACE_OUTER_BOUND('',#2233,.T.);
#1219=FACE_OUTER_BOUND('',#2234,.T.);
#1220=FACE_OUTER_BOUND('',#2235,.T.);
#1221=FACE_OUTER_BOUND('',#2236,.T.);
#1222=FACE_OUTER_BOUND('',#2237,.T.);
#1223=FACE_OUTER_BOUND('',#2238,.T.);
#1224=FACE_OUTER_BOUND('',#2239,.T.);
#1225=FACE_OUTER_BOUND('',#2240,.T.);
#1226=FACE_OUTER_BOUND('',#2241,.T.);
#1227=FACE_OUTER_BOUND('',#2242,.T.);
#1228=FACE_OUTER_BOUND('',#2243,.T.);
#1229=FACE_OUTER_BOUND('',#2244,.T.);
#1230=FACE_OUTER_BOUND('',#2245,.T.);
#1231=FACE_OUTER_BOUND('',#2246,.T.);
#1232=FACE_OUTER_BOUND('',#2247,.T.);
#1233=FACE_OUTER_BOUND('',#2248,.T.);
#1234=FACE_OUTER_BOUND('',#2249,.T.);
#1235=FACE_OUTER_BOUND('',#2250,.T.);
#1236=FACE_OUTER_BOUND('',#2251,.T.);
#1237=FACE_OUTER_BOUND('',#2252,.T.);
#1238=FACE_OUTER_BOUND('',#2253,.T.);
#1239=FACE_OUTER_BOUND('',#2254,.T.);
#1240=FACE_OUTER_BOUND('',#2255,.T.);
#1241=FACE_OUTER_BOUND('',#2256,.T.);
#1242=FACE_OUTER_BOUND('',#2257,.T.);
#1243=FACE_OUTER_BOUND('',#2258,.T.);
#1244=FACE_OUTER_BOUND('',#2259,.T.);
#1245=FACE_OUTER_BOUND('',#2260,.T.);
#1246=FACE_OUTER_BOUND('',#2261,.T.);
#1247=FACE_OUTER_BOUND('',#2262,.T.);
#1248=FACE_OUTER_BOUND('',#2263,.T.);
#1249=FACE_OUTER_BOUND('',#2264,.T.);
#1250=FACE_OUTER_BOUND('',#2265,.T.);
#1251=FACE_OUTER_BOUND('',#2266,.T.);
#1252=FACE_OUTER_BOUND('',#2267,.T.);
#1253=FACE_OUTER_BOUND('',#2268,.T.);
#1254=FACE_OUTER_BOUND('',#2269,.T.);
#1255=FACE_OUTER_BOUND('',#2270,.T.);
#1256=FACE_OUTER_BOUND('',#2271,.T.);
#1257=FACE_OUTER_BOUND('',#2272,.T.);
#1258=FACE_OUTER_BOUND('',#2273,.T.);
#1259=FACE_OUTER_BOUND('',#2274,.T.);
#1260=FACE_OUTER_BOUND('',#2275,.T.);
#1261=FACE_OUTER_BOUND('',#2276,.T.);
#1262=FACE_OUTER_BOUND('',#2277,.T.);
#1263=FACE_OUTER_BOUND('',#2278,.T.);
#1264=FACE_OUTER_BOUND('',#2279,.T.);
#1265=FACE_OUTER_BOUND('',#2280,.T.);
#1266=FACE_OUTER_BOUND('',#2281,.T.);
#1267=FACE_OUTER_BOUND('',#2282,.T.);
#1268=FACE_OUTER_BOUND('',#2283,.T.);
#1269=FACE_OUTER_BOUND('',#2284,.T.);
#1270=FACE_OUTER_BOUND('',#2285,.T.);
#1271=FACE_OUTER_BOUND('',#2286,.T.);
#1272=FACE_OUTER_BOUND('',#2287,.T.);
#1273=FACE_OUTER_BOUND('',#2288,.T.);
#1274=FACE_OUTER_BOUND('',#2289,.T.);
#1275=FACE_OUTER_BOUND('',#2290,.T.);
#1276=FACE_OUTER_BOUND('',#2291,.T.);
#1277=FACE_OUTER_BOUND('',#2292,.T.);
#1278=FACE_OUTER_BOUND('',#2293,.T.);
#1279=FACE_OUTER_BOUND('',#2294,.T.);
#1280=FACE_OUTER_BOUND('',#2295,.T.);
#1281=FACE_OUTER_BOUND('',#2296,.T.);
#1282=FACE_OUTER_BOUND('',#2297,.T.);
#1283=FACE_OUTER_BOUND('',#2298,.T.);
#1284=FACE_OUTER_BOUND('',#2299,.T.);
#1285=FACE_OUTER_BOUND('',#2300,.T.);
#1286=FACE_OUTER_BOUND('',#2301,.T.);
#1287=FACE_OUTER_BOUND('',#2302,.T.);
#1288=FACE_OUTER_BOUND('',#2303,.T.);
#1289=FACE_OUTER_BOUND('',#2304,.T.);
#1290=FACE_OUTER_BOUND('',#2305,.T.);
#1291=FACE_OUTER_BOUND('',#2306,.T.);
#1292=FACE_OUTER_BOUND('',#2307,.T.);
#1293=FACE_OUTER_BOUND('',#2308,.T.);
#1294=FACE_OUTER_BOUND('',#2309,.T.);
#1295=FACE_OUTER_BOUND('',#2310,.T.);
#1296=FACE_OUTER_BOUND('',#2311,.T.);
#1297=FACE_OUTER_BOUND('',#2312,.T.);
#1298=FACE_OUTER_BOUND('',#2313,.T.);
#1299=FACE_OUTER_BOUND('',#2314,.T.);
#1300=FACE_OUTER_BOUND('',#2315,.T.);
#1301=FACE_OUTER_BOUND('',#2316,.T.);
#1302=FACE_OUTER_BOUND('',#2317,.T.);
#1303=FACE_OUTER_BOUND('',#2318,.T.);
#1304=FACE_OUTER_BOUND('',#2319,.T.);
#1305=FACE_OUTER_BOUND('',#2320,.T.);
#1306=FACE_OUTER_BOUND('',#2321,.T.);
#1307=FACE_OUTER_BOUND('',#2322,.T.);
#1308=FACE_OUTER_BOUND('',#2323,.T.);
#1309=FACE_OUTER_BOUND('',#2324,.T.);
#1310=FACE_OUTER_BOUND('',#2325,.T.);
#1311=FACE_OUTER_BOUND('',#2326,.T.);
#1312=FACE_OUTER_BOUND('',#2327,.T.);
#1313=FACE_OUTER_BOUND('',#2328,.T.);
#1314=FACE_OUTER_BOUND('',#2329,.T.);
#1315=FACE_OUTER_BOUND('',#2330,.T.);
#1316=FACE_OUTER_BOUND('',#2331,.T.);
#1317=FACE_OUTER_BOUND('',#2332,.T.);
#1318=FACE_OUTER_BOUND('',#2333,.T.);
#1319=FACE_OUTER_BOUND('',#2334,.T.);
#1320=FACE_OUTER_BOUND('',#2335,.T.);
#1321=FACE_OUTER_BOUND('',#2336,.T.);
#1322=FACE_OUTER_BOUND('',#2337,.T.);
#1323=FACE_OUTER_BOUND('',#2338,.T.);
#1324=FACE_OUTER_BOUND('',#2339,.T.);
#1325=FACE_OUTER_BOUND('',#2340,.T.);
#1326=FACE_OUTER_BOUND('',#2341,.T.);
#1327=FACE_OUTER_BOUND('',#2342,.T.);
#1328=FACE_OUTER_BOUND('',#2343,.T.);
#1329=FACE_OUTER_BOUND('',#2344,.T.);
#1330=FACE_OUTER_BOUND('',#2345,.T.);
#1331=FACE_OUTER_BOUND('',#2353,.T.);
#1332=FACE_OUTER_BOUND('',#2354,.T.);
#1333=FACE_OUTER_BOUND('',#2355,.T.);
#1334=FACE_OUTER_BOUND('',#2356,.T.);
#1335=FACE_OUTER_BOUND('',#2357,.T.);
#1336=FACE_OUTER_BOUND('',#2358,.T.);
#1337=FACE_OUTER_BOUND('',#2359,.T.);
#1338=FACE_OUTER_BOUND('',#2360,.T.);
#1339=FACE_OUTER_BOUND('',#2361,.T.);
#1340=FACE_OUTER_BOUND('',#2362,.T.);
#1341=FACE_OUTER_BOUND('',#2363,.T.);
#1342=FACE_OUTER_BOUND('',#2364,.T.);
#1343=FACE_OUTER_BOUND('',#2365,.T.);
#1344=FACE_OUTER_BOUND('',#2366,.T.);
#1345=FACE_OUTER_BOUND('',#2367,.T.);
#1346=FACE_OUTER_BOUND('',#2368,.T.);
#1347=FACE_OUTER_BOUND('',#2369,.T.);
#1348=FACE_OUTER_BOUND('',#2370,.T.);
#1349=FACE_OUTER_BOUND('',#2371,.T.);
#1350=FACE_OUTER_BOUND('',#2372,.T.);
#1351=FACE_OUTER_BOUND('',#2373,.T.);
#1352=FACE_OUTER_BOUND('',#2374,.T.);
#1353=FACE_OUTER_BOUND('',#2375,.T.);
#1354=FACE_OUTER_BOUND('',#2376,.T.);
#1355=FACE_OUTER_BOUND('',#2377,.T.);
#1356=FACE_OUTER_BOUND('',#2378,.T.);
#1357=FACE_OUTER_BOUND('',#2379,.T.);
#1358=FACE_OUTER_BOUND('',#2380,.T.);
#1359=FACE_OUTER_BOUND('',#2381,.T.);
#1360=FACE_OUTER_BOUND('',#2382,.T.);
#1361=FACE_OUTER_BOUND('',#2383,.T.);
#1362=FACE_OUTER_BOUND('',#2384,.T.);
#1363=FACE_OUTER_BOUND('',#2385,.T.);
#1364=FACE_OUTER_BOUND('',#2386,.T.);
#1365=FACE_OUTER_BOUND('',#2387,.T.);
#1366=FACE_OUTER_BOUND('',#2388,.T.);
#1367=FACE_OUTER_BOUND('',#2389,.T.);
#1368=FACE_OUTER_BOUND('',#2390,.T.);
#1369=FACE_OUTER_BOUND('',#2391,.T.);
#1370=FACE_OUTER_BOUND('',#2392,.T.);
#1371=FACE_OUTER_BOUND('',#2393,.T.);
#1372=FACE_OUTER_BOUND('',#2394,.T.);
#1373=FACE_OUTER_BOUND('',#2395,.T.);
#1374=FACE_OUTER_BOUND('',#2396,.T.);
#1375=FACE_OUTER_BOUND('',#2397,.T.);
#1376=FACE_OUTER_BOUND('',#2398,.T.);
#1377=FACE_OUTER_BOUND('',#2399,.T.);
#1378=FACE_OUTER_BOUND('',#2400,.T.);
#1379=FACE_OUTER_BOUND('',#2401,.T.);
#1380=FACE_OUTER_BOUND('',#2402,.T.);
#1381=FACE_OUTER_BOUND('',#2403,.T.);
#1382=FACE_OUTER_BOUND('',#2404,.T.);
#1383=FACE_OUTER_BOUND('',#2405,.T.);
#1384=FACE_OUTER_BOUND('',#2406,.T.);
#1385=FACE_OUTER_BOUND('',#2407,.T.);
#1386=FACE_OUTER_BOUND('',#2408,.T.);
#1387=FACE_OUTER_BOUND('',#2409,.T.);
#1388=FACE_OUTER_BOUND('',#2410,.T.);
#1389=FACE_OUTER_BOUND('',#2411,.T.);
#1390=FACE_OUTER_BOUND('',#2412,.T.);
#1391=FACE_OUTER_BOUND('',#2413,.T.);
#1392=FACE_OUTER_BOUND('',#2414,.T.);
#1393=FACE_OUTER_BOUND('',#2415,.T.);
#1394=FACE_OUTER_BOUND('',#2416,.T.);
#1395=FACE_OUTER_BOUND('',#2417,.T.);
#1396=FACE_OUTER_BOUND('',#2418,.T.);
#1397=FACE_OUTER_BOUND('',#2419,.T.);
#1398=FACE_OUTER_BOUND('',#2420,.T.);
#1399=FACE_OUTER_BOUND('',#2421,.T.);
#1400=FACE_OUTER_BOUND('',#2422,.T.);
#1401=FACE_OUTER_BOUND('',#2423,.T.);
#1402=FACE_OUTER_BOUND('',#2424,.T.);
#1403=FACE_OUTER_BOUND('',#2425,.T.);
#1404=FACE_OUTER_BOUND('',#2426,.T.);
#1405=FACE_OUTER_BOUND('',#2427,.T.);
#1406=FACE_OUTER_BOUND('',#2428,.T.);
#1407=FACE_OUTER_BOUND('',#2429,.T.);
#1408=FACE_OUTER_BOUND('',#2430,.T.);
#1409=FACE_OUTER_BOUND('',#2431,.T.);
#1410=FACE_OUTER_BOUND('',#2432,.T.);
#1411=FACE_OUTER_BOUND('',#2433,.T.);
#1412=FACE_OUTER_BOUND('',#2434,.T.);
#1413=FACE_OUTER_BOUND('',#2435,.T.);
#1414=FACE_OUTER_BOUND('',#2436,.T.);
#1415=FACE_OUTER_BOUND('',#2437,.T.);
#1416=FACE_OUTER_BOUND('',#2438,.T.);
#1417=FACE_OUTER_BOUND('',#2440,.T.);
#1418=FACE_OUTER_BOUND('',#2442,.T.);
#1419=FACE_OUTER_BOUND('',#2443,.T.);
#1420=FACE_OUTER_BOUND('',#2445,.T.);
#1421=FACE_OUTER_BOUND('',#2447,.T.);
#1422=FACE_OUTER_BOUND('',#2448,.T.);
#1423=FACE_OUTER_BOUND('',#2450,.T.);
#1424=FACE_OUTER_BOUND('',#2452,.T.);
#1425=FACE_OUTER_BOUND('',#2453,.T.);
#1426=FACE_OUTER_BOUND('',#2455,.T.);
#1427=FACE_OUTER_BOUND('',#2457,.T.);
#1428=FACE_OUTER_BOUND('',#2458,.T.);
#1429=FACE_OUTER_BOUND('',#2460,.T.);
#1430=FACE_OUTER_BOUND('',#2462,.T.);
#1431=FACE_OUTER_BOUND('',#2463,.T.);
#1432=FACE_OUTER_BOUND('',#2465,.T.);
#1433=FACE_OUTER_BOUND('',#2467,.T.);
#1434=FACE_OUTER_BOUND('',#2468,.T.);
#1435=FACE_OUTER_BOUND('',#2470,.T.);
#1436=FACE_OUTER_BOUND('',#2471,.T.);
#1437=FACE_OUTER_BOUND('',#2473,.T.);
#1438=FACE_OUTER_BOUND('',#2475,.T.);
#1439=FACE_OUTER_BOUND('',#2476,.T.);
#1440=FACE_OUTER_BOUND('',#2478,.T.);
#1441=FACE_OUTER_BOUND('',#2479,.T.);
#1442=FACE_OUTER_BOUND('',#2481,.T.);
#1443=FACE_OUTER_BOUND('',#2482,.T.);
#1444=FACE_OUTER_BOUND('',#2484,.T.);
#1445=FACE_OUTER_BOUND('',#2485,.T.);
#1446=FACE_OUTER_BOUND('',#2487,.T.);
#1447=FACE_OUTER_BOUND('',#2488,.T.);
#1448=FACE_OUTER_BOUND('',#2490,.T.);
#1449=FACE_OUTER_BOUND('',#2491,.T.);
#1450=FACE_OUTER_BOUND('',#2492,.T.);
#1451=FACE_OUTER_BOUND('',#2494,.T.);
#1452=FACE_OUTER_BOUND('',#2495,.T.);
#1453=FACE_OUTER_BOUND('',#2497,.T.);
#1454=FACE_OUTER_BOUND('',#2498,.T.);
#1455=FACE_OUTER_BOUND('',#2499,.T.);
#1456=FACE_OUTER_BOUND('',#2500,.T.);
#1457=FACE_OUTER_BOUND('',#2501,.T.);
#1458=FACE_OUTER_BOUND('',#2502,.T.);
#1459=FACE_OUTER_BOUND('',#2503,.T.);
#1460=FACE_OUTER_BOUND('',#2504,.T.);
#1461=FACE_OUTER_BOUND('',#2505,.T.);
#1462=FACE_OUTER_BOUND('',#2506,.T.);
#1463=FACE_OUTER_BOUND('',#2508,.T.);
#1464=FACE_OUTER_BOUND('',#2509,.T.);
#1465=FACE_OUTER_BOUND('',#2511,.T.);
#1466=FACE_OUTER_BOUND('',#2512,.T.);
#1467=FACE_OUTER_BOUND('',#2513,.T.);
#1468=FACE_OUTER_BOUND('',#2514,.T.);
#1469=FACE_OUTER_BOUND('',#2515,.T.);
#1470=FACE_OUTER_BOUND('',#2516,.T.);
#1471=FACE_OUTER_BOUND('',#2517,.T.);
#1472=FACE_OUTER_BOUND('',#2518,.T.);
#1473=FACE_OUTER_BOUND('',#2519,.T.);
#1474=FACE_OUTER_BOUND('',#2520,.T.);
#1475=FACE_OUTER_BOUND('',#2521,.T.);
#1476=FACE_OUTER_BOUND('',#2529,.T.);
#1477=FACE_OUTER_BOUND('',#2530,.T.);
#1478=FACE_OUTER_BOUND('',#2531,.T.);
#1479=FACE_OUTER_BOUND('',#2532,.T.);
#1480=FACE_OUTER_BOUND('',#2533,.T.);
#1481=FACE_OUTER_BOUND('',#2534,.T.);
#1482=FACE_OUTER_BOUND('',#2535,.T.);
#1483=FACE_OUTER_BOUND('',#2536,.T.);
#1484=FACE_OUTER_BOUND('',#2537,.T.);
#1485=FACE_OUTER_BOUND('',#2538,.T.);
#1486=FACE_OUTER_BOUND('',#2539,.T.);
#1487=FACE_OUTER_BOUND('',#2540,.T.);
#1488=FACE_OUTER_BOUND('',#2541,.T.);
#2150=EDGE_LOOP('',(#13678,#13679,#13680,#13681,#13682,#13683,#13684,#13685,
#13686,#13687));
#2151=EDGE_LOOP('',(#13688,#13689,#13690,#13691));
#2152=EDGE_LOOP('',(#13692,#13693,#13694,#13695));
#2153=EDGE_LOOP('',(#13696,#13697,#13698,#13699));
#2154=EDGE_LOOP('',(#13700,#13701,#13702,#13703));
#2155=EDGE_LOOP('',(#13704,#13705,#13706,#13707));
#2156=EDGE_LOOP('',(#13708,#13709,#13710,#13711));
#2157=EDGE_LOOP('',(#13712,#13713,#13714,#13715));
#2158=EDGE_LOOP('',(#13716,#13717,#13718,#13719));
#2159=EDGE_LOOP('',(#13720,#13721,#13722,#13723));
#2160=EDGE_LOOP('',(#13724,#13725,#13726,#13727));
#2161=EDGE_LOOP('',(#13728,#13729,#13730,#13731));
#2162=EDGE_LOOP('',(#13732,#13733,#13734,#13735));
#2163=EDGE_LOOP('',(#13736,#13737,#13738,#13739));
#2164=EDGE_LOOP('',(#13740,#13741,#13742,#13743));
#2165=EDGE_LOOP('',(#13744,#13745,#13746,#13747));
#2166=EDGE_LOOP('',(#13748,#13749,#13750,#13751,#13752,#13753,#13754,#13755,
#13756,#13757));
#2167=EDGE_LOOP('',(#13758,#13759,#13760,#13761));
#2168=EDGE_LOOP('',(#13762,#13763,#13764,#13765));
#2169=EDGE_LOOP('',(#13766,#13767,#13768,#13769));
#2170=EDGE_LOOP('',(#13770,#13771,#13772,#13773));
#2171=EDGE_LOOP('',(#13774,#13775,#13776,#13777));
#2172=EDGE_LOOP('',(#13778,#13779,#13780,#13781));
#2173=EDGE_LOOP('',(#13782,#13783,#13784,#13785));
#2174=EDGE_LOOP('',(#13786,#13787,#13788,#13789));
#2175=EDGE_LOOP('',(#13790,#13791,#13792,#13793));
#2176=EDGE_LOOP('',(#13794,#13795,#13796,#13797));
#2177=EDGE_LOOP('',(#13798,#13799,#13800,#13801));
#2178=EDGE_LOOP('',(#13802,#13803,#13804,#13805));
#2179=EDGE_LOOP('',(#13806,#13807,#13808,#13809));
#2180=EDGE_LOOP('',(#13810,#13811,#13812,#13813));
#2181=EDGE_LOOP('',(#13814,#13815,#13816,#13817));
#2182=EDGE_LOOP('',(#13818,#13819,#13820,#13821,#13822,#13823,#13824,#13825,
#13826,#13827));
#2183=EDGE_LOOP('',(#13828,#13829,#13830,#13831));
#2184=EDGE_LOOP('',(#13832,#13833,#13834,#13835));
#2185=EDGE_LOOP('',(#13836,#13837,#13838,#13839));
#2186=EDGE_LOOP('',(#13840,#13841,#13842,#13843));
#2187=EDGE_LOOP('',(#13844,#13845,#13846,#13847));
#2188=EDGE_LOOP('',(#13848,#13849,#13850,#13851));
#2189=EDGE_LOOP('',(#13852,#13853,#13854,#13855));
#2190=EDGE_LOOP('',(#13856,#13857,#13858,#13859));
#2191=EDGE_LOOP('',(#13860,#13861,#13862,#13863));
#2192=EDGE_LOOP('',(#13864,#13865,#13866,#13867));
#2193=EDGE_LOOP('',(#13868,#13869,#13870,#13871));
#2194=EDGE_LOOP('',(#13872,#13873,#13874,#13875));
#2195=EDGE_LOOP('',(#13876,#13877,#13878,#13879));
#2196=EDGE_LOOP('',(#13880,#13881,#13882,#13883));
#2197=EDGE_LOOP('',(#13884,#13885,#13886,#13887));
#2198=EDGE_LOOP('',(#13888,#13889,#13890,#13891,#13892,#13893,#13894,#13895,
#13896,#13897));
#2199=EDGE_LOOP('',(#13898,#13899,#13900,#13901));
#2200=EDGE_LOOP('',(#13902,#13903,#13904,#13905));
#2201=EDGE_LOOP('',(#13906,#13907,#13908,#13909));
#2202=EDGE_LOOP('',(#13910,#13911,#13912,#13913));
#2203=EDGE_LOOP('',(#13914,#13915,#13916,#13917));
#2204=EDGE_LOOP('',(#13918,#13919,#13920,#13921));
#2205=EDGE_LOOP('',(#13922,#13923,#13924,#13925));
#2206=EDGE_LOOP('',(#13926,#13927,#13928,#13929));
#2207=EDGE_LOOP('',(#13930,#13931,#13932,#13933));
#2208=EDGE_LOOP('',(#13934,#13935,#13936,#13937));
#2209=EDGE_LOOP('',(#13938,#13939,#13940,#13941));
#2210=EDGE_LOOP('',(#13942,#13943,#13944,#13945));
#2211=EDGE_LOOP('',(#13946,#13947,#13948,#13949));
#2212=EDGE_LOOP('',(#13950,#13951,#13952,#13953));
#2213=EDGE_LOOP('',(#13954,#13955,#13956,#13957));
#2214=EDGE_LOOP('',(#13958,#13959,#13960,#13961,#13962,#13963,#13964,#13965,
#13966,#13967));
#2215=EDGE_LOOP('',(#13968,#13969,#13970,#13971));
#2216=EDGE_LOOP('',(#13972,#13973,#13974,#13975));
#2217=EDGE_LOOP('',(#13976,#13977,#13978,#13979));
#2218=EDGE_LOOP('',(#13980,#13981,#13982,#13983));
#2219=EDGE_LOOP('',(#13984,#13985,#13986,#13987));
#2220=EDGE_LOOP('',(#13988,#13989,#13990,#13991));
#2221=EDGE_LOOP('',(#13992,#13993,#13994,#13995));
#2222=EDGE_LOOP('',(#13996,#13997,#13998,#13999));
#2223=EDGE_LOOP('',(#14000,#14001,#14002,#14003));
#2224=EDGE_LOOP('',(#14004,#14005,#14006,#14007));
#2225=EDGE_LOOP('',(#14008,#14009,#14010,#14011));
#2226=EDGE_LOOP('',(#14012,#14013,#14014,#14015));
#2227=EDGE_LOOP('',(#14016,#14017,#14018,#14019));
#2228=EDGE_LOOP('',(#14020,#14021,#14022,#14023));
#2229=EDGE_LOOP('',(#14024,#14025,#14026,#14027));
#2230=EDGE_LOOP('',(#14028,#14029,#14030,#14031,#14032,#14033,#14034,#14035,
#14036,#14037));
#2231=EDGE_LOOP('',(#14038,#14039,#14040,#14041));
#2232=EDGE_LOOP('',(#14042,#14043,#14044,#14045));
#2233=EDGE_LOOP('',(#14046,#14047,#14048,#14049));
#2234=EDGE_LOOP('',(#14050,#14051,#14052,#14053));
#2235=EDGE_LOOP('',(#14054,#14055,#14056,#14057));
#2236=EDGE_LOOP('',(#14058,#14059,#14060,#14061));
#2237=EDGE_LOOP('',(#14062,#14063,#14064,#14065));
#2238=EDGE_LOOP('',(#14066,#14067,#14068,#14069));
#2239=EDGE_LOOP('',(#14070,#14071,#14072,#14073));
#2240=EDGE_LOOP('',(#14074,#14075,#14076,#14077));
#2241=EDGE_LOOP('',(#14078,#14079,#14080,#14081));
#2242=EDGE_LOOP('',(#14082,#14083,#14084,#14085));
#2243=EDGE_LOOP('',(#14086,#14087,#14088,#14089));
#2244=EDGE_LOOP('',(#14090,#14091,#14092,#14093));
#2245=EDGE_LOOP('',(#14094,#14095,#14096,#14097));
#2246=EDGE_LOOP('',(#14098,#14099,#14100,#14101,#14102,#14103,#14104,#14105,
#14106,#14107));
#2247=EDGE_LOOP('',(#14108,#14109,#14110,#14111));
#2248=EDGE_LOOP('',(#14112,#14113,#14114,#14115));
#2249=EDGE_LOOP('',(#14116,#14117,#14118,#14119));
#2250=EDGE_LOOP('',(#14120,#14121,#14122,#14123));
#2251=EDGE_LOOP('',(#14124,#14125,#14126,#14127));
#2252=EDGE_LOOP('',(#14128,#14129,#14130,#14131));
#2253=EDGE_LOOP('',(#14132,#14133,#14134,#14135));
#2254=EDGE_LOOP('',(#14136,#14137,#14138,#14139));
#2255=EDGE_LOOP('',(#14140,#14141,#14142,#14143));
#2256=EDGE_LOOP('',(#14144,#14145,#14146,#14147));
#2257=EDGE_LOOP('',(#14148,#14149,#14150,#14151));
#2258=EDGE_LOOP('',(#14152,#14153,#14154,#14155));
#2259=EDGE_LOOP('',(#14156,#14157,#14158,#14159));
#2260=EDGE_LOOP('',(#14160,#14161,#14162,#14163));
#2261=EDGE_LOOP('',(#14164,#14165,#14166,#14167));
#2262=EDGE_LOOP('',(#14168,#14169,#14170,#14171,#14172,#14173,#14174,#14175,
#14176,#14177));
#2263=EDGE_LOOP('',(#14178,#14179,#14180,#14181));
#2264=EDGE_LOOP('',(#14182,#14183,#14184,#14185));
#2265=EDGE_LOOP('',(#14186,#14187,#14188,#14189));
#2266=EDGE_LOOP('',(#14190,#14191,#14192,#14193));
#2267=EDGE_LOOP('',(#14194,#14195,#14196,#14197));
#2268=EDGE_LOOP('',(#14198,#14199,#14200,#14201));
#2269=EDGE_LOOP('',(#14202,#14203,#14204,#14205));
#2270=EDGE_LOOP('',(#14206,#14207,#14208,#14209));
#2271=EDGE_LOOP('',(#14210,#14211,#14212,#14213));
#2272=EDGE_LOOP('',(#14214,#14215,#14216,#14217));
#2273=EDGE_LOOP('',(#14218,#14219,#14220,#14221));
#2274=EDGE_LOOP('',(#14222,#14223,#14224,#14225));
#2275=EDGE_LOOP('',(#14226,#14227,#14228,#14229));
#2276=EDGE_LOOP('',(#14230,#14231,#14232,#14233));
#2277=EDGE_LOOP('',(#14234,#14235,#14236,#14237));
#2278=EDGE_LOOP('',(#14238,#14239,#14240,#14241,#14242,#14243,#14244,#14245,
#14246,#14247));
#2279=EDGE_LOOP('',(#14248,#14249,#14250,#14251));
#2280=EDGE_LOOP('',(#14252,#14253,#14254,#14255));
#2281=EDGE_LOOP('',(#14256,#14257,#14258,#14259));
#2282=EDGE_LOOP('',(#14260,#14261,#14262,#14263));
#2283=EDGE_LOOP('',(#14264,#14265,#14266,#14267));
#2284=EDGE_LOOP('',(#14268,#14269,#14270,#14271));
#2285=EDGE_LOOP('',(#14272,#14273,#14274,#14275));
#2286=EDGE_LOOP('',(#14276,#14277,#14278,#14279));
#2287=EDGE_LOOP('',(#14280,#14281,#14282,#14283));
#2288=EDGE_LOOP('',(#14284,#14285,#14286,#14287));
#2289=EDGE_LOOP('',(#14288,#14289,#14290,#14291));
#2290=EDGE_LOOP('',(#14292,#14293,#14294,#14295));
#2291=EDGE_LOOP('',(#14296,#14297,#14298,#14299));
#2292=EDGE_LOOP('',(#14300,#14301,#14302,#14303));
#2293=EDGE_LOOP('',(#14304,#14305,#14306,#14307));
#2294=EDGE_LOOP('',(#14308,#14309,#14310,#14311,#14312,#14313,#14314,#14315,
#14316,#14317));
#2295=EDGE_LOOP('',(#14318,#14319,#14320,#14321));
#2296=EDGE_LOOP('',(#14322,#14323,#14324,#14325));
#2297=EDGE_LOOP('',(#14326,#14327,#14328,#14329));
#2298=EDGE_LOOP('',(#14330,#14331,#14332,#14333));
#2299=EDGE_LOOP('',(#14334,#14335,#14336,#14337));
#2300=EDGE_LOOP('',(#14338,#14339,#14340,#14341));
#2301=EDGE_LOOP('',(#14342,#14343,#14344,#14345));
#2302=EDGE_LOOP('',(#14346,#14347,#14348,#14349));
#2303=EDGE_LOOP('',(#14350,#14351,#14352,#14353));
#2304=EDGE_LOOP('',(#14354,#14355,#14356,#14357));
#2305=EDGE_LOOP('',(#14358,#14359,#14360,#14361));
#2306=EDGE_LOOP('',(#14362,#14363,#14364,#14365));
#2307=EDGE_LOOP('',(#14366,#14367,#14368,#14369));
#2308=EDGE_LOOP('',(#14370,#14371,#14372,#14373));
#2309=EDGE_LOOP('',(#14374,#14375,#14376,#14377));
#2310=EDGE_LOOP('',(#14378,#14379,#14380,#14381,#14382,#14383,#14384,#14385,
#14386,#14387));
#2311=EDGE_LOOP('',(#14388,#14389,#14390,#14391));
#2312=EDGE_LOOP('',(#14392,#14393,#14394,#14395));
#2313=EDGE_LOOP('',(#14396,#14397,#14398,#14399));
#2314=EDGE_LOOP('',(#14400,#14401,#14402,#14403));
#2315=EDGE_LOOP('',(#14404,#14405,#14406,#14407));
#2316=EDGE_LOOP('',(#14408,#14409,#14410,#14411));
#2317=EDGE_LOOP('',(#14412,#14413,#14414,#14415));
#2318=EDGE_LOOP('',(#14416,#14417,#14418,#14419));
#2319=EDGE_LOOP('',(#14420,#14421,#14422,#14423));
#2320=EDGE_LOOP('',(#14424,#14425,#14426,#14427));
#2321=EDGE_LOOP('',(#14428,#14429,#14430,#14431));
#2322=EDGE_LOOP('',(#14432,#14433,#14434,#14435));
#2323=EDGE_LOOP('',(#14436,#14437,#14438,#14439));
#2324=EDGE_LOOP('',(#14440,#14441,#14442,#14443));
#2325=EDGE_LOOP('',(#14444,#14445,#14446,#14447));
#2326=EDGE_LOOP('',(#14448,#14449,#14450,#14451,#14452,#14453,#14454,#14455,
#14456,#14457));
#2327=EDGE_LOOP('',(#14458,#14459,#14460,#14461));
#2328=EDGE_LOOP('',(#14462,#14463,#14464,#14465));
#2329=EDGE_LOOP('',(#14466,#14467,#14468,#14469));
#2330=EDGE_LOOP('',(#14470,#14471,#14472,#14473));
#2331=EDGE_LOOP('',(#14474,#14475,#14476,#14477));
#2332=EDGE_LOOP('',(#14478,#14479,#14480,#14481));
#2333=EDGE_LOOP('',(#14482,#14483,#14484,#14485));
#2334=EDGE_LOOP('',(#14486,#14487,#14488,#14489));
#2335=EDGE_LOOP('',(#14490,#14491,#14492,#14493));
#2336=EDGE_LOOP('',(#14494,#14495,#14496,#14497));
#2337=EDGE_LOOP('',(#14498,#14499,#14500,#14501));
#2338=EDGE_LOOP('',(#14502,#14503,#14504,#14505));
#2339=EDGE_LOOP('',(#14506,#14507,#14508,#14509));
#2340=EDGE_LOOP('',(#14510,#14511,#14512,#14513));
#2341=EDGE_LOOP('',(#14514,#14515,#14516,#14517));
#2342=EDGE_LOOP('',(#14518,#14519,#14520,#14521));
#2343=EDGE_LOOP('',(#14522,#14523,#14524,#14525));
#2344=EDGE_LOOP('',(#14526,#14527,#14528,#14529));
#2345=EDGE_LOOP('',(#14530,#14531,#14532,#14533,#14534,#14535,#14536,#14537,
#14538,#14539,#14540,#14541,#14542,#14543,#14544,#14545,#14546,#14547,#14548,
#14549,#14550,#14551,#14552,#14553,#14554,#14555,#14556,#14557,#14558,#14559,
#14560,#14561,#14562,#14563,#14564,#14565,#14566,#14567,#14568,#14569,#14570,
#14571,#14572,#14573,#14574,#14575,#14576,#14577,#14578,#14579,#14580,#14581,
#14582,#14583));
#2346=EDGE_LOOP('',(#14584,#14585,#14586,#14587));
#2347=EDGE_LOOP('',(#14588,#14589,#14590,#14591));
#2348=EDGE_LOOP('',(#14592,#14593,#14594,#14595));
#2349=EDGE_LOOP('',(#14596,#14597,#14598,#14599));
#2350=EDGE_LOOP('',(#14600,#14601,#14602,#14603));
#2351=EDGE_LOOP('',(#14604,#14605,#14606,#14607));
#2352=EDGE_LOOP('',(#14608,#14609,#14610,#14611));
#2353=EDGE_LOOP('',(#14612,#14613,#14614,#14615,#14616));
#2354=EDGE_LOOP('',(#14617,#14618,#14619,#14620));
#2355=EDGE_LOOP('',(#14621,#14622,#14623,#14624,#14625,#14626,#14627,#14628,
#14629,#14630,#14631,#14632,#14633,#14634,#14635,#14636,#14637,#14638,#14639,
#14640));
#2356=EDGE_LOOP('',(#14641,#14642,#14643,#14644,#14645,#14646,#14647,#14648,
#14649,#14650,#14651,#14652,#14653,#14654,#14655,#14656,#14657,#14658,#14659,
#14660));
#2357=EDGE_LOOP('',(#14661,#14662,#14663,#14664));
#2358=EDGE_LOOP('',(#14665,#14666,#14667,#14668,#14669));
#2359=EDGE_LOOP('',(#14670,#14671,#14672,#14673));
#2360=EDGE_LOOP('',(#14674,#14675,#14676,#14677,#14678,#14679,#14680,#14681,
#14682,#14683,#14684,#14685,#14686,#14687,#14688,#14689,#14690,#14691,#14692,
#14693));
#2361=EDGE_LOOP('',(#14694,#14695,#14696,#14697,#14698,#14699,#14700,#14701,
#14702,#14703,#14704,#14705,#14706,#14707,#14708,#14709,#14710,#14711,#14712,
#14713));
#2362=EDGE_LOOP('',(#14714,#14715,#14716,#14717));
#2363=EDGE_LOOP('',(#14718,#14719,#14720,#14721,#14722));
#2364=EDGE_LOOP('',(#14723,#14724,#14725,#14726));
#2365=EDGE_LOOP('',(#14727,#14728,#14729,#14730,#14731,#14732,#14733,#14734,
#14735,#14736,#14737,#14738,#14739,#14740,#14741,#14742,#14743,#14744,#14745,
#14746));
#2366=EDGE_LOOP('',(#14747,#14748,#14749,#14750,#14751,#14752,#14753,#14754,
#14755,#14756,#14757,#14758,#14759,#14760,#14761,#14762,#14763,#14764,#14765,
#14766));
#2367=EDGE_LOOP('',(#14767,#14768,#14769,#14770));
#2368=EDGE_LOOP('',(#14771,#14772,#14773,#14774,#14775));
#2369=EDGE_LOOP('',(#14776,#14777,#14778,#14779));
#2370=EDGE_LOOP('',(#14780,#14781,#14782,#14783,#14784,#14785,#14786,#14787,
#14788,#14789,#14790,#14791,#14792,#14793,#14794,#14795,#14796,#14797,#14798,
#14799));
#2371=EDGE_LOOP('',(#14800,#14801,#14802,#14803,#14804,#14805,#14806,#14807,
#14808,#14809,#14810,#14811,#14812,#14813,#14814,#14815,#14816,#14817,#14818,
#14819));
#2372=EDGE_LOOP('',(#14820,#14821,#14822,#14823));
#2373=EDGE_LOOP('',(#14824,#14825,#14826,#14827,#14828));
#2374=EDGE_LOOP('',(#14829,#14830,#14831,#14832));
#2375=EDGE_LOOP('',(#14833,#14834,#14835,#14836,#14837,#14838,#14839,#14840,
#14841,#14842,#14843,#14844,#14845,#14846,#14847,#14848,#14849,#14850,#14851,
#14852));
#2376=EDGE_LOOP('',(#14853,#14854,#14855,#14856,#14857,#14858,#14859,#14860,
#14861,#14862,#14863,#14864,#14865,#14866,#14867,#14868,#14869,#14870,#14871,
#14872));
#2377=EDGE_LOOP('',(#14873,#14874,#14875,#14876));
#2378=EDGE_LOOP('',(#14877,#14878,#14879));
#2379=EDGE_LOOP('',(#14880,#14881));
#2380=EDGE_LOOP('',(#14882,#14883,#14884));
#2381=EDGE_LOOP('',(#14885,#14886));
#2382=EDGE_LOOP('',(#14887,#14888,#14889));
#2383=EDGE_LOOP('',(#14890,#14891));
#2384=EDGE_LOOP('',(#14892,#14893,#14894));
#2385=EDGE_LOOP('',(#14895,#14896));
#2386=EDGE_LOOP('',(#14897,#14898,#14899));
#2387=EDGE_LOOP('',(#14900,#14901));
#2388=EDGE_LOOP('',(#14902,#14903,#14904,#14905,#14906));
#2389=EDGE_LOOP('',(#14907,#14908,#14909,#14910));
#2390=EDGE_LOOP('',(#14911,#14912,#14913,#14914,#14915,#14916,#14917,#14918,
#14919,#14920,#14921,#14922,#14923,#14924,#14925,#14926,#14927,#14928,#14929,
#14930));
#2391=EDGE_LOOP('',(#14931,#14932,#14933,#14934,#14935,#14936,#14937,#14938,
#14939,#14940,#14941,#14942,#14943,#14944,#14945,#14946,#14947,#14948,#14949,
#14950));
#2392=EDGE_LOOP('',(#14951,#14952,#14953,#14954));
#2393=EDGE_LOOP('',(#14955,#14956,#14957,#14958,#14959));
#2394=EDGE_LOOP('',(#14960,#14961,#14962,#14963));
#2395=EDGE_LOOP('',(#14964,#14965,#14966,#14967,#14968,#14969,#14970,#14971,
#14972,#14973,#14974,#14975,#14976,#14977,#14978,#14979,#14980,#14981,#14982,
#14983));
#2396=EDGE_LOOP('',(#14984,#14985,#14986,#14987,#14988,#14989,#14990,#14991,
#14992,#14993,#14994,#14995,#14996,#14997,#14998,#14999,#15000,#15001,#15002,
#15003));
#2397=EDGE_LOOP('',(#15004,#15005,#15006,#15007));
#2398=EDGE_LOOP('',(#15008,#15009,#15010,#15011,#15012));
#2399=EDGE_LOOP('',(#15013,#15014,#15015,#15016));
#2400=EDGE_LOOP('',(#15017,#15018,#15019,#15020,#15021,#15022,#15023,#15024,
#15025,#15026,#15027,#15028,#15029,#15030,#15031,#15032,#15033,#15034,#15035,
#15036));
#2401=EDGE_LOOP('',(#15037,#15038,#15039,#15040,#15041,#15042,#15043,#15044,
#15045,#15046,#15047,#15048,#15049,#15050,#15051,#15052,#15053,#15054,#15055,
#15056));
#2402=EDGE_LOOP('',(#15057,#15058,#15059,#15060));
#2403=EDGE_LOOP('',(#15061,#15062,#15063,#15064,#15065));
#2404=EDGE_LOOP('',(#15066,#15067,#15068,#15069));
#2405=EDGE_LOOP('',(#15070,#15071,#15072,#15073,#15074,#15075,#15076,#15077,
#15078,#15079,#15080,#15081,#15082,#15083,#15084,#15085,#15086,#15087,#15088,
#15089));
#2406=EDGE_LOOP('',(#15090,#15091,#15092,#15093,#15094,#15095,#15096,#15097,
#15098,#15099,#15100,#15101,#15102,#15103,#15104,#15105,#15106,#15107,#15108,
#15109));
#2407=EDGE_LOOP('',(#15110,#15111,#15112,#15113));
#2408=EDGE_LOOP('',(#15114,#15115,#15116,#15117,#15118));
#2409=EDGE_LOOP('',(#15119,#15120,#15121,#15122));
#2410=EDGE_LOOP('',(#15123,#15124,#15125,#15126,#15127,#15128,#15129,#15130,
#15131,#15132,#15133,#15134,#15135,#15136,#15137,#15138,#15139,#15140,#15141,
#15142));
#2411=EDGE_LOOP('',(#15143,#15144,#15145,#15146,#15147,#15148,#15149,#15150,
#15151,#15152,#15153,#15154,#15155,#15156,#15157,#15158,#15159,#15160,#15161,
#15162));
#2412=EDGE_LOOP('',(#15163,#15164,#15165,#15166));
#2413=EDGE_LOOP('',(#15167,#15168,#15169));
#2414=EDGE_LOOP('',(#15170,#15171));
#2415=EDGE_LOOP('',(#15172,#15173,#15174));
#2416=EDGE_LOOP('',(#15175,#15176));
#2417=EDGE_LOOP('',(#15177,#15178,#15179));
#2418=EDGE_LOOP('',(#15180,#15181));
#2419=EDGE_LOOP('',(#15182,#15183,#15184));
#2420=EDGE_LOOP('',(#15185,#15186));
#2421=EDGE_LOOP('',(#15187,#15188,#15189));
#2422=EDGE_LOOP('',(#15190,#15191));
#2423=EDGE_LOOP('',(#15192,#15193,#15194,#15195,#15196));
#2424=EDGE_LOOP('',(#15197,#15198,#15199,#15200));
#2425=EDGE_LOOP('',(#15201,#15202,#15203,#15204,#15205,#15206,#15207,#15208,
#15209,#15210,#15211,#15212,#15213,#15214,#15215,#15216,#15217,#15218,#15219,
#15220));
#2426=EDGE_LOOP('',(#15221,#15222,#15223,#15224,#15225,#15226,#15227,#15228,
#15229,#15230,#15231,#15232,#15233,#15234,#15235,#15236,#15237,#15238,#15239,
#15240));
#2427=EDGE_LOOP('',(#15241,#15242,#15243,#15244));
#2428=EDGE_LOOP('',(#15245,#15246,#15247));
#2429=EDGE_LOOP('',(#15248,#15249));
#2430=EDGE_LOOP('',(#15250,#15251,#15252,#15253,#15254));
#2431=EDGE_LOOP('',(#15255,#15256,#15257,#15258));
#2432=EDGE_LOOP('',(#15259,#15260,#15261,#15262,#15263,#15264,#15265,#15266,
#15267,#15268,#15269,#15270,#15271,#15272,#15273,#15274,#15275,#15276,#15277,
#15278));
#2433=EDGE_LOOP('',(#15279,#15280,#15281,#15282,#15283,#15284,#15285,#15286,
#15287,#15288,#15289,#15290,#15291,#15292,#15293,#15294,#15295,#15296,#15297,
#15298));
#2434=EDGE_LOOP('',(#15299,#15300,#15301,#15302));
#2435=EDGE_LOOP('',(#15303,#15304,#15305));
#2436=EDGE_LOOP('',(#15306,#15307));
#2437=EDGE_LOOP('',(#15308,#15309,#15310,#15311));
#2438=EDGE_LOOP('',(#15312,#15313,#15314,#15315,#15316,#15317,#15318,#15319));
#2439=EDGE_LOOP('',(#15320,#15321));
#2440=EDGE_LOOP('',(#15322));
#2441=EDGE_LOOP('',(#15323));
#2442=EDGE_LOOP('',(#15324,#15325,#15326,#15327));
#2443=EDGE_LOOP('',(#15328,#15329,#15330,#15331,#15332,#15333,#15334,#15335));
#2444=EDGE_LOOP('',(#15336,#15337));
#2445=EDGE_LOOP('',(#15338));
#2446=EDGE_LOOP('',(#15339));
#2447=EDGE_LOOP('',(#15340,#15341,#15342,#15343));
#2448=EDGE_LOOP('',(#15344,#15345,#15346,#15347,#15348,#15349,#15350,#15351));
#2449=EDGE_LOOP('',(#15352,#15353));
#2450=EDGE_LOOP('',(#15354));
#2451=EDGE_LOOP('',(#15355));
#2452=EDGE_LOOP('',(#15356,#15357,#15358,#15359));
#2453=EDGE_LOOP('',(#15360,#15361,#15362,#15363,#15364,#15365,#15366,#15367));
#2454=EDGE_LOOP('',(#15368,#15369));
#2455=EDGE_LOOP('',(#15370));
#2456=EDGE_LOOP('',(#15371));
#2457=EDGE_LOOP('',(#15372,#15373,#15374,#15375));
#2458=EDGE_LOOP('',(#15376,#15377,#15378,#15379,#15380,#15381,#15382,#15383));
#2459=EDGE_LOOP('',(#15384,#15385));
#2460=EDGE_LOOP('',(#15386));
#2461=EDGE_LOOP('',(#15387));
#2462=EDGE_LOOP('',(#15388,#15389,#15390,#15391));
#2463=EDGE_LOOP('',(#15392,#15393,#15394,#15395,#15396,#15397,#15398,#15399));
#2464=EDGE_LOOP('',(#15400,#15401));
#2465=EDGE_LOOP('',(#15402));
#2466=EDGE_LOOP('',(#15403));
#2467=EDGE_LOOP('',(#15404,#15405,#15406,#15407));
#2468=EDGE_LOOP('',(#15408,#15409,#15410,#15411));
#2469=EDGE_LOOP('',(#15412));
#2470=EDGE_LOOP('',(#15413,#15414,#15415,#15416));
#2471=EDGE_LOOP('',(#15417,#15418,#15419,#15420));
#2472=EDGE_LOOP('',(#15421));
#2473=EDGE_LOOP('',(#15422,#15423,#15424,#15425));
#2474=EDGE_LOOP('',(#15426));
#2475=EDGE_LOOP('',(#15427,#15428,#15429,#15430));
#2476=EDGE_LOOP('',(#15431,#15432,#15433,#15434));
#2477=EDGE_LOOP('',(#15435));
#2478=EDGE_LOOP('',(#15436,#15437,#15438,#15439));
#2479=EDGE_LOOP('',(#15440,#15441,#15442,#15443));
#2480=EDGE_LOOP('',(#15444));
#2481=EDGE_LOOP('',(#15445,#15446,#15447,#15448));
#2482=EDGE_LOOP('',(#15449,#15450,#15451,#15452));
#2483=EDGE_LOOP('',(#15453));
#2484=EDGE_LOOP('',(#15454,#15455,#15456,#15457));
#2485=EDGE_LOOP('',(#15458,#15459,#15460,#15461));
#2486=EDGE_LOOP('',(#15462));
#2487=EDGE_LOOP('',(#15463,#15464,#15465,#15466));
#2488=EDGE_LOOP('',(#15467,#15468,#15469,#15470));
#2489=EDGE_LOOP('',(#15471));
#2490=EDGE_LOOP('',(#15472,#15473,#15474,#15475));
#2491=EDGE_LOOP('',(#15476,#15477,#15478,#15479));
#2492=EDGE_LOOP('',(#15480,#15481,#15482,#15483));
#2493=EDGE_LOOP('',(#15484));
#2494=EDGE_LOOP('',(#15485,#15486,#15487,#15488));
#2495=EDGE_LOOP('',(#15489,#15490,#15491,#15492));
#2496=EDGE_LOOP('',(#15493));
#2497=EDGE_LOOP('',(#15494,#15495,#15496,#15497));
#2498=EDGE_LOOP('',(#15498,#15499,#15500,#15501));
#2499=EDGE_LOOP('',(#15502,#15503,#15504,#15505));
#2500=EDGE_LOOP('',(#15506,#15507,#15508,#15509));
#2501=EDGE_LOOP('',(#15510,#15511,#15512,#15513));
#2502=EDGE_LOOP('',(#15514,#15515,#15516,#15517));
#2503=EDGE_LOOP('',(#15518,#15519,#15520,#15521));
#2504=EDGE_LOOP('',(#15522,#15523,#15524,#15525));
#2505=EDGE_LOOP('',(#15526,#15527,#15528,#15529));
#2506=EDGE_LOOP('',(#15530,#15531,#15532,#15533));
#2507=EDGE_LOOP('',(#15534));
#2508=EDGE_LOOP('',(#15535,#15536,#15537,#15538));
#2509=EDGE_LOOP('',(#15539,#15540,#15541,#15542));
#2510=EDGE_LOOP('',(#15543));
#2511=EDGE_LOOP('',(#15544,#15545,#15546,#15547));
#2512=EDGE_LOOP('',(#15548,#15549,#15550,#15551));
#2513=EDGE_LOOP('',(#15552,#15553,#15554,#15555));
#2514=EDGE_LOOP('',(#15556,#15557,#15558,#15559));
#2515=EDGE_LOOP('',(#15560,#15561,#15562,#15563));
#2516=EDGE_LOOP('',(#15564,#15565,#15566,#15567));
#2517=EDGE_LOOP('',(#15568,#15569,#15570,#15571));
#2518=EDGE_LOOP('',(#15572,#15573,#15574,#15575));
#2519=EDGE_LOOP('',(#15576,#15577,#15578,#15579));
#2520=EDGE_LOOP('',(#15580,#15581,#15582,#15583));
#2521=EDGE_LOOP('',(#15584,#15585,#15586,#15587,#15588,#15589,#15590,#15591,
#15592,#15593,#15594,#15595,#15596,#15597,#15598,#15599,#15600,#15601,#15602,
#15603,#15604,#15605,#15606,#15607,#15608,#15609,#15610,#15611,#15612,#15613,
#15614,#15615,#15616,#15617,#15618,#15619,#15620,#15621,#15622,#15623,#15624,
#15625,#15626,#15627,#15628,#15629,#15630,#15631,#15632,#15633,#15634,#15635,
#15636,#15637));
#2522=EDGE_LOOP('',(#15638,#15639,#15640,#15641));
#2523=EDGE_LOOP('',(#15642,#15643,#15644,#15645));
#2524=EDGE_LOOP('',(#15646,#15647,#15648,#15649));
#2525=EDGE_LOOP('',(#15650,#15651,#15652,#15653));
#2526=EDGE_LOOP('',(#15654,#15655,#15656,#15657));
#2527=EDGE_LOOP('',(#15658,#15659,#15660,#15661));
#2528=EDGE_LOOP('',(#15662,#15663,#15664,#15665));
#2529=EDGE_LOOP('',(#15666,#15667,#15668,#15669));
#2530=EDGE_LOOP('',(#15670,#15671,#15672,#15673));
#2531=EDGE_LOOP('',(#15674,#15675,#15676,#15677));
#2532=EDGE_LOOP('',(#15678,#15679,#15680,#15681));
#2533=EDGE_LOOP('',(#15682,#15683,#15684,#15685));
#2534=EDGE_LOOP('',(#15686,#15687,#15688,#15689));
#2535=EDGE_LOOP('',(#15690,#15691,#15692,#15693));
#2536=EDGE_LOOP('',(#15694,#15695,#15696,#15697));
#2537=EDGE_LOOP('',(#15698,#15699,#15700,#15701));
#2538=EDGE_LOOP('',(#15702,#15703,#15704,#15705));
#2539=EDGE_LOOP('',(#15706,#15707,#15708,#15709));
#2540=EDGE_LOOP('',(#15710,#15711,#15712,#15713));
#2541=EDGE_LOOP('',(#15714,#15715,#15716,#15717));
#2849=CIRCLE('',#18967,1.2645);
#2850=CIRCLE('',#18968,1.2645);
#2851=CIRCLE('',#18969,1.2645);
#2852=CIRCLE('',#18970,1.2645);
#2853=CIRCLE('',#18971,1.2645);
#2854=CIRCLE('',#18979,1.2645);
#2855=CIRCLE('',#18981,1.543);
#2856=CIRCLE('',#18989,1.543);
#2857=CIRCLE('',#18991,1.2645);
#2858=CIRCLE('',#18992,1.2645);
#2859=CIRCLE('',#18993,1.2645);
#2860=CIRCLE('',#18994,1.2645);
#2861=CIRCLE('',#18995,1.2645);
#2862=CIRCLE('',#19003,1.2645);
#2863=CIRCLE('',#19005,1.54299999999999);
#2864=CIRCLE('',#19013,1.54299999999999);
#2865=CIRCLE('',#19015,1.2645);
#2866=CIRCLE('',#19016,1.2645);
#2867=CIRCLE('',#19017,1.2645);
#2868=CIRCLE('',#19018,1.2645);
#2869=CIRCLE('',#19019,1.2645);
#2870=CIRCLE('',#19027,1.2645);
#2871=CIRCLE('',#19029,1.543);
#2872=CIRCLE('',#19037,1.543);
#2873=CIRCLE('',#19039,1.2645);
#2874=CIRCLE('',#19040,1.2645);
#2875=CIRCLE('',#19041,1.2645);
#2876=CIRCLE('',#19042,1.2645);
#2877=CIRCLE('',#19043,1.2645);
#2878=CIRCLE('',#19051,1.2645);
#2879=CIRCLE('',#19053,1.543);
#2880=CIRCLE('',#19061,1.543);
#2881=CIRCLE('',#19063,1.2645);
#2882=CIRCLE('',#19064,1.2645);
#2883=CIRCLE('',#19065,1.2645);
#2884=CIRCLE('',#19066,1.2645);
#2885=CIRCLE('',#19067,1.2645);
#2886=CIRCLE('',#19075,1.2645);
#2887=CIRCLE('',#19077,1.54300000000001);
#2888=CIRCLE('',#19085,1.54300000000001);
#2889=CIRCLE('',#19087,1.2645);
#2890=CIRCLE('',#19088,1.2645);
#2891=CIRCLE('',#19089,1.2645);
#2892=CIRCLE('',#19090,1.2645);
#2893=CIRCLE('',#19091,1.2645);
#2894=CIRCLE('',#19099,1.2645);
#2895=CIRCLE('',#19101,1.54300000000001);
#2896=CIRCLE('',#19109,1.54300000000001);
#2897=CIRCLE('',#19111,1.2645);
#2898=CIRCLE('',#19112,1.2645);
#2899=CIRCLE('',#19113,1.2645);
#2900=CIRCLE('',#19114,1.2645);
#2901=CIRCLE('',#19115,1.2645);
#2902=CIRCLE('',#19123,1.2645);
#2903=CIRCLE('',#19125,1.543);
#2904=CIRCLE('',#19133,1.543);
#2905=CIRCLE('',#19135,1.2645);
#2906=CIRCLE('',#19136,1.2645);
#2907=CIRCLE('',#19137,1.2645);
#2908=CIRCLE('',#19138,1.2645);
#2909=CIRCLE('',#19139,1.2645);
#2910=CIRCLE('',#19147,1.2645);
#2911=CIRCLE('',#19149,1.54300000000001);
#2912=CIRCLE('',#19157,1.54300000000001);
#2913=CIRCLE('',#19159,1.2645);
#2914=CIRCLE('',#19160,1.2645);
#2915=CIRCLE('',#19161,1.2645);
#2916=CIRCLE('',#19162,1.2645);
#2917=CIRCLE('',#19163,1.2645);
#2918=CIRCLE('',#19171,1.2645);
#2919=CIRCLE('',#19173,1.54300000000001);
#2920=CIRCLE('',#19181,1.54300000000001);
#2921=CIRCLE('',#19183,1.2645);
#2922=CIRCLE('',#19184,1.2645);
#2923=CIRCLE('',#19185,1.2645);
#2924=CIRCLE('',#19186,1.2645);
#2925=CIRCLE('',#19187,1.2645);
#2926=CIRCLE('',#19195,1.2645);
#2927=CIRCLE('',#19197,1.543);
#2928=CIRCLE('',#19205,1.543);
#2929=CIRCLE('',#19207,1.2645);
#2930=CIRCLE('',#19208,1.2645);
#2931=CIRCLE('',#19209,1.2645);
#2932=CIRCLE('',#19210,1.2645);
#2933=CIRCLE('',#19211,1.2645);
#2934=CIRCLE('',#19219,1.2645);
#2935=CIRCLE('',#19221,1.54299999999999);
#2936=CIRCLE('',#19229,1.54299999999999);
#2937=CIRCLE('',#19231,1.2645);
#2938=CIRCLE('',#19232,1.2645);
#2939=CIRCLE('',#19233,1.2645);
#2940=CIRCLE('',#19234,1.2645);
#2941=CIRCLE('',#19235,1.2645);
#2942=CIRCLE('',#19243,1.2645);
#2943=CIRCLE('',#19245,1.543);
#2944=CIRCLE('',#19253,1.543);
#2945=CIRCLE('',#19258,1.);
#2946=CIRCLE('',#19259,45.9999999999998);
#2947=CIRCLE('',#19260,1.);
#2948=CIRCLE('',#19261,45.9999999999998);
#2949=CIRCLE('',#19262,1.);
#2950=CIRCLE('',#19263,45.9999999999998);
#2951=CIRCLE('',#19264,1.);
#2952=CIRCLE('',#19265,45.9999999999998);
#2953=CIRCLE('',#19266,1.);
#2954=CIRCLE('',#19267,45.9999999999998);
#2955=CIRCLE('',#19268,1.);
#2956=CIRCLE('',#19269,45.9999999999998);
#2957=CIRCLE('',#19270,10.);
#2958=CIRCLE('',#19332,1.5);
#2959=CIRCLE('',#19333,1.5);
#2960=CIRCLE('',#19335,3.);
#2961=CIRCLE('',#19336,3.);
#2962=CIRCLE('',#19339,1.5);
#2963=CIRCLE('',#19340,1.5);
#2964=CIRCLE('',#19342,3.);
#2965=CIRCLE('',#19343,3.);
#2966=CIRCLE('',#19346,1.5);
#2967=CIRCLE('',#19347,1.5);
#2968=CIRCLE('',#19349,3.);
#2969=CIRCLE('',#19350,3.);
#2970=CIRCLE('',#19353,1.5);
#2971=CIRCLE('',#19354,1.5);
#2972=CIRCLE('',#19356,3.);
#2973=CIRCLE('',#19357,3.);
#2974=CIRCLE('',#19360,1.5);
#2975=CIRCLE('',#19361,1.5);
#2976=CIRCLE('',#19363,3.);
#2977=CIRCLE('',#19364,3.);
#2978=CIRCLE('',#19367,1.5);
#2979=CIRCLE('',#19368,1.5);
#2980=CIRCLE('',#19370,3.);
#2981=CIRCLE('',#19371,3.);
#2982=CIRCLE('',#19398,45.9999999999998);
#2983=CIRCLE('',#19400,1.);
#2984=CIRCLE('',#19403,45.9999999999998);
#2985=CIRCLE('',#19405,1.);
#2986=CIRCLE('',#19408,45.9999999999998);
#2987=CIRCLE('',#19410,1.);
#2988=CIRCLE('',#19413,45.9999999999998);
#2989=CIRCLE('',#19414,1.);
#2990=CIRCLE('',#19415,45.9999999999998);
#2991=CIRCLE('',#19416,1.);
#2992=CIRCLE('',#19417,45.9999999999998);
#2993=CIRCLE('',#19418,1.);
#2994=CIRCLE('',#19419,10.);
#3993=B_SPLINE_CURVE_WITH_KNOTS('',3,(#52677,#52678,#52679,#52680),
 .UNSPECIFIED.,.F.,.F.,(4,4),(51.5750455984138,52.2860549491936),
 .UNSPECIFIED.);
#3994=B_SPLINE_CURVE_WITH_KNOTS('',3,(#52692,#52693,#52694,#52695,#52696,
#52697,#52698,#52699,#52700,#52701),.UNSPECIFIED.,.F.,.F.,(4,3,3,4),(-50.2654824574367,
-49.3264669332015,-48.3399375945375,-47.8348991546267),.UNSPECIFIED.);
#3995=B_SPLINE_CURVE_WITH_KNOTS('',3,(#52706,#52707,#52708,#52709,#52710,
#52711,#52712,#52713,#52714,#52715,#52716,#52717,#52718,#52719,#52720,#52721,
#52722,#52723,#52724,#52725,#52726,#52727,#52728,#52729,#52730),
 .UNSPECIFIED.,.F.,.F.,(4,3,3,3,3,3,3,3,4),(45.2918602912342,45.3803495785454,
46.3668789172094,47.3534082558734,48.3399375945375,49.3264669332015,50.3129962718655,
51.2995256105296,51.5750455984138),.UNSPECIFIED.);
#3996=B_SPLINE_CURVE_WITH_KNOTS('',3,(#52731,#52732,#52733,#52734,#52735,
#52736,#52737,#52738,#52739,#52740,#52741,#52742,#52743,#52744,#52745,#52746,
#52747,#52748,#52749,#52750,#52751,#52752),.UNSPECIFIED.,.F.,.F.,(4,3,3,
3,3,3,3,4),(-47.8348991546267,-47.3534082558735,-46.3668789172094,-45.3803495785454,
-44.3938202398814,-43.4072909012173,-42.4207615625533,-41.5517138474471),
 .UNSPECIFIED.);
#3997=B_SPLINE_CURVE_WITH_KNOTS('',3,(#52757,#52758,#52759,#52760,#52761,
#52762,#52763,#52764,#52765,#52766,#52767,#52768,#52769,#52770,#52771,#52772,
#52773,#52774,#52775,#52776,#52777,#52778),.UNSPECIFIED.,.F.,.F.,(4,3,3,
3,3,3,3,4),(39.0086749840546,39.4611735465612,40.4477028852252,41.4342322238893,
42.4207615625533,43.4072909012173,44.3938202398814,45.2918602912342),
 .UNSPECIFIED.);
#3998=B_SPLINE_CURVE_WITH_KNOTS('',3,(#52779,#52780,#52781,#52782,#52783,
#52784,#52785,#52786,#52787,#52788,#52789,#52790,#52791,#52792,#52793,#52794,
#52795,#52796,#52797,#52798,#52799,#52800,#52801,#52802,#52803),
 .UNSPECIFIED.,.F.,.F.,(4,3,3,3,3,3,3,3,4),(-41.5517138474471,-41.4342322238893,
-40.4477028852252,-39.4611735465612,-38.4746442078972,-37.4881148692332,
-36.5015855305691,-35.5150561919051,-35.2685285402675),.UNSPECIFIED.);
#3999=B_SPLINE_CURVE_WITH_KNOTS('',3,(#52808,#52809,#52810,#52811,#52812,
#52813,#52814,#52815,#52816,#52817,#52818,#52819,#52820,#52821,#52822,#52823,
#52824,#52825,#52826,#52827,#52828,#52829),.UNSPECIFIED.,.F.,.F.,(4,3,3,
3,3,3,3,4),(32.725489676875,33.541997514577,34.5285268532411,35.5150561919051,
36.5015855305691,37.4881148692331,38.4746442078972,39.0086749840546),
 .UNSPECIFIED.);
#4000=B_SPLINE_CURVE_WITH_KNOTS('',3,(#52830,#52831,#52832,#52833,#52834,
#52835,#52836,#52837,#52838,#52839,#52840,#52841,#52842,#52843,#52844,#52845,
#52846,#52847,#52848,#52849,#52850,#52851),.UNSPECIFIED.,.F.,.F.,(4,3,3,
3,3,3,3,4),(-35.2685285402675,-34.5285268532411,-33.541997514577,-32.555468175913,
-31.568938837249,-30.5824094985849,-29.5958801599209,-28.9853432330879),
 .UNSPECIFIED.);
#4001=B_SPLINE_CURVE_WITH_KNOTS('',3,(#52856,#52857,#52858,#52859,#52860,
#52861,#52862,#52863,#52864,#52865,#52866,#52867,#52868,#52869,#52870,#52871,
#52872,#52873,#52874,#52875,#52876,#52877,#52878,#52879,#52880),
 .UNSPECIFIED.,.F.,.F.,(4,3,3,3,3,3,3,3,4),(26.4423043696954,26.6362921439288,
27.6228214825928,28.6093508212569,29.5958801599209,30.5824094985849,31.568938837249,
32.555468175913,32.725489676875),.UNSPECIFIED.);
#4002=B_SPLINE_CURVE_WITH_KNOTS('',3,(#52881,#52882,#52883,#52884,#52885,
#52886,#52887,#52888,#52889,#52890,#52891,#52892,#52893,#52894,#52895,#52896,
#52897,#52898,#52899,#52900,#52901,#52902),.UNSPECIFIED.,.F.,.F.,(4,3,3,
3,3,3,3,4),(-28.9853432330879,-28.6093508212569,-27.6228214825929,-26.6362921439288,
-25.6497628052648,-24.6632334666008,-23.6767041279367,-22.7021579259083),
 .UNSPECIFIED.);
#4003=B_SPLINE_CURVE_WITH_KNOTS('',3,(#52907,#52908,#52909,#52910,#52911,
#52912,#52913,#52914,#52915,#52916,#52917,#52918,#52919,#52920,#52921,#52922,
#52923,#52924,#52925,#52926,#52927,#52928),.UNSPECIFIED.,.F.,.F.,(4,3,3,
3,3,3,3,4),(20.1591190625158,20.7171161119446,21.7036454506087,22.6901747892727,
23.6767041279367,24.6632334666008,25.6497628052648,26.4423043696954),
 .UNSPECIFIED.);
#4004=B_SPLINE_CURVE_WITH_KNOTS('',3,(#52929,#52930,#52931,#52932,#52933,
#52934,#52935,#52936,#52937,#52938,#52939,#52940,#52941,#52942,#52943,#52944,
#52945,#52946,#52947,#52948,#52949,#52950,#52951,#52952,#52953),
 .UNSPECIFIED.,.F.,.F.,(4,3,3,3,3,3,3,3,4),(-22.7021579259083,-22.6901747892727,
-21.7036454506087,-20.7171161119446,-19.7305867732806,-18.7440574346166,
-17.7575280959525,-16.7709987572885,-16.4189726187288),.UNSPECIFIED.);
#4005=B_SPLINE_CURVE_WITH_KNOTS('',3,(#52958,#52959,#52960,#52961,#52962,
#52963,#52964,#52965,#52966,#52967,#52968,#52969,#52970,#52971,#52972,#52973,
#52974,#52975,#52976,#52977,#52978,#52979),.UNSPECIFIED.,.F.,.F.,(4,3,3,
3,3,3,3,4),(13.8759337553362,14.7979400799604,15.7844694186245,16.7709987572885,
17.7575280959525,18.7440574346166,19.7305867732806,20.1591190625158),
 .UNSPECIFIED.);
#4006=B_SPLINE_CURVE_WITH_KNOTS('',3,(#52980,#52981,#52982,#52983,#52984,
#52985,#52986,#52987,#52988,#52989,#52990,#52991,#52992,#52993,#52994,#52995,
#52996,#52997,#52998,#52999,#53000,#53001),.UNSPECIFIED.,.F.,.F.,(4,3,3,
3,3,3,3,4),(-16.4189726187288,-15.7844694186245,-14.7979400799605,-13.8114107412964,
-12.8248814026324,-11.8383520639684,-10.8518227253043,-10.1357873115492),
 .UNSPECIFIED.);
#4007=B_SPLINE_CURVE_WITH_KNOTS('',3,(#53007,#53008,#53009,#53010,#53011,
#53012,#53013,#53014,#53015,#53016,#53017,#53018,#53019),.UNSPECIFIED.,
 .F.,.F.,(4,3,3,3,4),(-3.85260200436958,-2.95958801599209,-1.97305867732806,
-0.986529338664031,0.),.UNSPECIFIED.);
#4008=B_SPLINE_CURVE_WITH_KNOTS('',3,(#53022,#53023,#53024,#53025,#53026,
#53027,#53028,#53029,#53030,#53031,#53032,#53033,#53034,#53035,#53036,#53037,
#53038,#53039,#53040),.UNSPECIFIED.,.F.,.F.,(4,3,3,3,3,3,4),(2.02057249175696,
2.95958801599209,3.94611735465612,4.93264669332015,5.91917603198418,6.90570537064821,
7.59274844815664),.UNSPECIFIED.);
#4009=B_SPLINE_CURVE_WITH_KNOTS('',3,(#53046,#53047,#53048,#53049,#53050,
#53051,#53052,#53053),.UNSPECIFIED.,.F.,.F.,(4,1,1,1,1,4),(59.6902604182061,
60.1952988581168,61.1818281967809,62.1683575354449,63.1548868741089,64.141416212773),
 .UNSPECIFIED.);
#4010=B_SPLINE_CURVE_WITH_KNOTS('',3,(#53056,#53057,#53058,#53059,#53060,
#53061,#53062,#53063,#53064),.UNSPECIFIED.,.F.,.F.,(4,1,1,1,1,1,4),(59.6902604182061,
59.7787497055172,60.7652790441813,61.7518083828453,62.7383377215093,63.7248670601734,
64.6638825844085),.UNSPECIFIED.);
#4011=B_SPLINE_CURVE_WITH_KNOTS('',3,(#53069,#53070,#53071,#53072,#53073,
#53074,#53075,#53076,#53077,#53078),.UNSPECIFIED.,.F.,.F.,(4,1,1,1,1,1,
1,4),(53.4070751110265,54.2761228261327,55.2626521647967,56.2491815034607,
57.2357108421248,58.2222401807888,59.2087695194528,59.6902604182061),
 .UNSPECIFIED.);
#4012=B_SPLINE_CURVE_WITH_KNOTS('',3,(#53079,#53080,#53081,#53082,#53083,
#53084,#53085,#53086,#53087,#53088),.UNSPECIFIED.,.F.,.F.,(4,1,1,1,1,1,
1,4),(53.4070751110265,53.8595736735331,54.8461030121971,55.8326323508611,
56.8191616895252,57.8056910281892,58.7922203668532,59.6902604182061),
 .UNSPECIFIED.);
#4013=B_SPLINE_CURVE_WITH_KNOTS('',3,(#53093,#53094,#53095,#53096,#53097,
#53098,#53099,#53100,#53101,#53102,#53103),.UNSPECIFIED.,.F.,.F.,(4,1,1,
1,1,1,1,1,4),(47.1238898038469,47.3704174554844,48.3569467941485,49.3434761328125,
50.3300054714765,51.3165348101406,52.3030641488046,53.2895934874686,53.4070751110265),
 .UNSPECIFIED.);
#4014=B_SPLINE_CURVE_WITH_KNOTS('',3,(#53104,#53105,#53106,#53107,#53108,
#53109,#53110,#53111,#53112,#53113),.UNSPECIFIED.,.F.,.F.,(4,1,1,1,1,1,
1,4),(47.1238898038469,47.9403976415489,48.9269269802129,49.913456318877,
50.899985657541,51.886514996205,52.873044334869,53.4070751110265),
 .UNSPECIFIED.);
#4015=B_SPLINE_CURVE_WITH_KNOTS('',3,(#53118,#53119,#53120,#53121,#53122,
#53123,#53124,#53125,#53126,#53127),.UNSPECIFIED.,.F.,.F.,(4,1,1,1,1,1,
1,4),(40.8407044966673,41.4512414235003,42.4377707621643,43.4243001008283,
44.4108294394924,45.3973587781564,46.3838881168204,47.1238898038469),
 .UNSPECIFIED.);
#4016=B_SPLINE_CURVE_WITH_KNOTS('',3,(#53128,#53129,#53130,#53131,#53132,
#53133,#53134,#53135,#53136,#53137,#53138),.UNSPECIFIED.,.F.,.F.,(4,1,1,
1,1,1,1,1,4),(40.8407044966673,41.0346922709007,42.0212216095647,43.0077509482287,
43.9942802868928,44.9808096255568,45.9673389642208,46.9538683028849,47.1238898038469),
 .UNSPECIFIED.);
#4017=B_SPLINE_CURVE_WITH_KNOTS('',3,(#53143,#53144,#53145,#53146,#53147,
#53148,#53149,#53150,#53151,#53152),.UNSPECIFIED.,.F.,.F.,(4,1,1,1,1,1,
1,4),(34.5575191894877,35.5320653915161,36.5185947301801,37.5051240688441,
38.4916534075082,39.4781827461722,40.4647120848362,40.8407044966673),
 .UNSPECIFIED.);
#4018=B_SPLINE_CURVE_WITH_KNOTS('',3,(#53153,#53154,#53155,#53156,#53157,
#53158,#53159,#53160,#53161,#53162),.UNSPECIFIED.,.F.,.F.,(4,1,1,1,1,1,
1,4),(34.5575191894877,35.1155162389165,36.1020455775805,37.0885749162446,
38.0751042549086,39.0616335935726,40.0481629322367,40.8407044966673),
 .UNSPECIFIED.);
#4019=B_SPLINE_CURVE_WITH_KNOTS('',3,(#53167,#53168,#53169,#53170,#53171,
#53172,#53173,#53174,#53175,#53176,#53177),.UNSPECIFIED.,.F.,.F.,(4,1,1,
1,1,1,1,1,4),(28.2743338823081,28.6263600208679,29.6128893595319,30.5994186981959,
31.58594803686,32.572477375524,33.559006714188,34.5455360528521,34.5575191894877),
 .UNSPECIFIED.);
#4020=B_SPLINE_CURVE_WITH_KNOTS('',3,(#53178,#53179,#53180,#53181,#53182,
#53183,#53184,#53185,#53186,#53187),.UNSPECIFIED.,.F.,.F.,(4,1,1,1,1,1,
1,4),(28.2743338823081,29.1963402069323,30.1828695455963,31.1693988842604,
32.1559282229244,33.1424575615884,34.1289869002525,34.5575191894877),
 .UNSPECIFIED.);
#4021=B_SPLINE_CURVE_WITH_KNOTS('',3,(#53192,#53193,#53194,#53195,#53196,
#53197,#53198,#53199,#53200,#53201),.UNSPECIFIED.,.F.,.F.,(4,1,1,1,1,1,
1,4),(21.9911485751285,22.7071839888837,23.6937133275477,24.6802426662117,
25.6667720048758,26.6533013435398,27.6398306822038,28.2743338823081),
 .UNSPECIFIED.);
#4022=B_SPLINE_CURVE_WITH_KNOTS('',3,(#53202,#53203,#53204,#53205,#53206,
#53207,#53208,#53209,#53210,#53211,#53212),.UNSPECIFIED.,.F.,.F.,(4,1,1,
1,1,1,1,1,4),(21.9911485751285,22.2906348362841,23.2771641749481,24.2636935136122,
25.2502228522762,26.2367521909402,27.2232815296043,28.2098108682683,28.2743338823081),
 .UNSPECIFIED.);
#4023=B_SPLINE_CURVE_WITH_KNOTS('',3,(#53218,#53219,#53220,#53221,#53222),
 .UNSPECIFIED.,.F.,.F.,(4,1,4),(14.3984001269719,15.3849294656359,15.7079632679489),
 .UNSPECIFIED.);
#4024=B_SPLINE_CURVE_WITH_KNOTS('',3,(#53225,#53226,#53227,#53228,#53229),
 .UNSPECIFIED.,.F.,.F.,(4,1,4),(13.8759337553363,14.8149492795714,15.7079632679489),
 .UNSPECIFIED.);
#4025=B_SPLINE_CURVE_WITH_KNOTS('',3,(#53235,#53236,#53237,#53238),
 .UNSPECIFIED.,.F.,.F.,(4,4),(51.5750455984138,52.2860549491937),
 .UNSPECIFIED.);
#4026=B_SPLINE_CURVE_WITH_KNOTS('',3,(#53250,#53251,#53252,#53253,#53254,
#53255,#53256,#53257,#53258,#53259),.UNSPECIFIED.,.F.,.F.,(4,3,3,4),(-50.2654824574367,
-49.3264669332015,-48.3399375945375,-47.8348991546267),.UNSPECIFIED.);
#4027=B_SPLINE_CURVE_WITH_KNOTS('',3,(#53264,#53265,#53266,#53267,#53268,
#53269,#53270,#53271,#53272,#53273,#53274,#53275,#53276,#53277,#53278,#53279,
#53280,#53281,#53282,#53283,#53284,#53285,#53286,#53287,#53288),
 .UNSPECIFIED.,.F.,.F.,(4,3,3,3,3,3,3,3,4),(45.2918602912342,45.3803495785454,
46.3668789172095,47.3534082558735,48.3399375945375,49.3264669332015,50.3129962718656,
51.2995256105296,51.5750455984138),.UNSPECIFIED.);
#4028=B_SPLINE_CURVE_WITH_KNOTS('',3,(#53289,#53290,#53291,#53292,#53293,
#53294,#53295,#53296,#53297,#53298,#53299,#53300,#53301,#53302,#53303,#53304,
#53305,#53306,#53307,#53308,#53309,#53310),.UNSPECIFIED.,.F.,.F.,(4,3,3,
3,3,3,3,4),(-47.8348991546267,-47.3534082558735,-46.3668789172094,-45.3803495785454,
-44.3938202398814,-43.4072909012173,-42.4207615625533,-41.5517138474471),
 .UNSPECIFIED.);
#4029=B_SPLINE_CURVE_WITH_KNOTS('',3,(#53315,#53316,#53317,#53318,#53319,
#53320,#53321,#53322,#53323,#53324,#53325,#53326,#53327,#53328,#53329,#53330,
#53331,#53332,#53333,#53334,#53335,#53336),.UNSPECIFIED.,.F.,.F.,(4,3,3,
3,3,3,3,4),(39.0086749840546,39.4611735465612,40.4477028852253,41.4342322238893,
42.4207615625533,43.4072909012174,44.3938202398814,45.2918602912342),
 .UNSPECIFIED.);
#4030=B_SPLINE_CURVE_WITH_KNOTS('',3,(#53337,#53338,#53339,#53340,#53341,
#53342,#53343,#53344,#53345,#53346,#53347,#53348,#53349,#53350,#53351,#53352,
#53353,#53354,#53355,#53356,#53357,#53358,#53359,#53360,#53361),
 .UNSPECIFIED.,.F.,.F.,(4,3,3,3,3,3,3,3,4),(-41.5517138474471,-41.4342322238893,
-40.4477028852253,-39.4611735465612,-38.4746442078972,-37.4881148692332,
-36.5015855305691,-35.5150561919051,-35.2685285402676),.UNSPECIFIED.);
#4031=B_SPLINE_CURVE_WITH_KNOTS('',3,(#53366,#53367,#53368,#53369,#53370,
#53371,#53372,#53373,#53374,#53375,#53376,#53377,#53378,#53379,#53380,#53381,
#53382,#53383,#53384,#53385,#53386,#53387),.UNSPECIFIED.,.F.,.F.,(4,3,3,
3,3,3,3,4),(32.725489676875,33.541997514577,34.5285268532411,35.5150561919051,
36.5015855305691,37.4881148692332,38.4746442078972,39.0086749840546),
 .UNSPECIFIED.);
#4032=B_SPLINE_CURVE_WITH_KNOTS('',3,(#53388,#53389,#53390,#53391,#53392,
#53393,#53394,#53395,#53396,#53397,#53398,#53399,#53400,#53401,#53402,#53403,
#53404,#53405,#53406,#53407,#53408,#53409),.UNSPECIFIED.,.F.,.F.,(4,3,3,
3,3,3,3,4),(-35.2685285402676,-34.5285268532411,-33.541997514577,-32.555468175913,
-31.568938837249,-30.5824094985849,-29.5958801599209,-28.985343233088),
 .UNSPECIFIED.);
#4033=B_SPLINE_CURVE_WITH_KNOTS('',3,(#53414,#53415,#53416,#53417,#53418,
#53419,#53420,#53421,#53422,#53423,#53424,#53425,#53426,#53427,#53428,#53429,
#53430,#53431,#53432,#53433,#53434,#53435,#53436,#53437,#53438),
 .UNSPECIFIED.,.F.,.F.,(4,3,3,3,3,3,3,3,4),(26.4423043696954,26.6362921439288,
27.6228214825929,28.6093508212569,29.5958801599209,30.582409498585,31.568938837249,
32.555468175913,32.725489676875),.UNSPECIFIED.);
#4034=B_SPLINE_CURVE_WITH_KNOTS('',3,(#53439,#53440,#53441,#53442,#53443,
#53444,#53445,#53446,#53447,#53448,#53449,#53450,#53451,#53452,#53453,#53454,
#53455,#53456,#53457,#53458,#53459,#53460),.UNSPECIFIED.,.F.,.F.,(4,3,3,
3,3,3,3,4),(-28.985343233088,-28.6093508212569,-27.6228214825929,-26.6362921439288,
-25.6497628052648,-24.6632334666008,-23.6767041279367,-22.7021579259084),
 .UNSPECIFIED.);
#4035=B_SPLINE_CURVE_WITH_KNOTS('',3,(#53465,#53466,#53467,#53468,#53469,
#53470,#53471,#53472,#53473,#53474,#53475,#53476,#53477,#53478,#53479,#53480,
#53481,#53482,#53483,#53484,#53485,#53486),.UNSPECIFIED.,.F.,.F.,(4,3,3,
3,3,3,3,4),(20.1591190625159,20.7171161119446,21.7036454506087,22.6901747892727,
23.6767041279367,24.6632334666008,25.6497628052648,26.4423043696954),
 .UNSPECIFIED.);
#4036=B_SPLINE_CURVE_WITH_KNOTS('',3,(#53487,#53488,#53489,#53490,#53491,
#53492,#53493,#53494,#53495,#53496,#53497,#53498,#53499,#53500,#53501,#53502,
#53503,#53504,#53505,#53506,#53507,#53508,#53509,#53510,#53511),
 .UNSPECIFIED.,.F.,.F.,(4,3,3,3,3,3,3,3,4),(-22.7021579259084,-22.6901747892727,
-21.7036454506087,-20.7171161119446,-19.7305867732806,-18.7440574346166,
-17.7575280959526,-16.7709987572885,-16.4189726187288),.UNSPECIFIED.);
#4037=B_SPLINE_CURVE_WITH_KNOTS('',3,(#53516,#53517,#53518,#53519,#53520,
#53521,#53522,#53523,#53524,#53525,#53526,#53527,#53528,#53529,#53530,#53531,
#53532,#53533,#53534,#53535,#53536,#53537),.UNSPECIFIED.,.F.,.F.,(4,3,3,
3,3,3,3,4),(13.8759337553363,14.7979400799605,15.7844694186245,16.7709987572885,
17.7575280959526,18.7440574346166,19.7305867732806,20.1591190625159),
 .UNSPECIFIED.);
#4038=B_SPLINE_CURVE_WITH_KNOTS('',3,(#53538,#53539,#53540,#53541,#53542,
#53543,#53544,#53545,#53546,#53547,#53548,#53549,#53550,#53551,#53552,#53553,
#53554,#53555,#53556,#53557,#53558,#53559),.UNSPECIFIED.,.F.,.F.,(4,3,3,
3,3,3,3,4),(-16.4189726187288,-15.7844694186245,-14.7979400799605,-13.8114107412964,
-12.8248814026324,-11.8383520639684,-10.8518227253043,-10.1357873115492),
 .UNSPECIFIED.);
#4039=B_SPLINE_CURVE_WITH_KNOTS('',3,(#53565,#53566,#53567,#53568,#53569,
#53570,#53571,#53572,#53573,#53574,#53575,#53576,#53577),.UNSPECIFIED.,
 .F.,.F.,(4,3,3,3,4),(-3.85260200436962,-2.9595880159921,-1.97305867732806,
-0.986529338664032,0.),.UNSPECIFIED.);
#4040=B_SPLINE_CURVE_WITH_KNOTS('',3,(#53580,#53581,#53582,#53583,#53584,
#53585,#53586,#53587,#53588,#53589,#53590,#53591,#53592,#53593,#53594,#53595,
#53596,#53597,#53598),.UNSPECIFIED.,.F.,.F.,(4,3,3,3,3,3,4),(2.02057249175687,
2.95958801599209,3.94611735465612,4.93264669332016,5.91917603198419,6.90570537064822,
7.59274844815668),.UNSPECIFIED.);
#4041=B_SPLINE_CURVE_WITH_KNOTS('',3,(#53604,#53605,#53606,#53607,#53608,
#53609,#53610,#53611),.UNSPECIFIED.,.F.,.F.,(4,1,1,1,1,4),(59.6902604182061,
60.1952988581168,61.1818281967809,62.1683575354449,63.1548868741089,64.141416212773),
 .UNSPECIFIED.);
#4042=B_SPLINE_CURVE_WITH_KNOTS('',3,(#53614,#53615,#53616,#53617,#53618,
#53619,#53620,#53621,#53622),.UNSPECIFIED.,.F.,.F.,(4,1,1,1,1,1,4),(59.6902604182061,
59.7787497055173,60.7652790441813,61.7518083828453,62.7383377215094,63.7248670601734,
64.6638825844085),.UNSPECIFIED.);
#4043=B_SPLINE_CURVE_WITH_KNOTS('',3,(#53627,#53628,#53629,#53630,#53631,
#53632,#53633,#53634,#53635,#53636),.UNSPECIFIED.,.F.,.F.,(4,1,1,1,1,1,
1,4),(53.4070751110265,54.2761228261326,55.2626521647967,56.2491815034607,
57.2357108421247,58.2222401807888,59.2087695194528,59.6902604182061),
 .UNSPECIFIED.);
#4044=B_SPLINE_CURVE_WITH_KNOTS('',3,(#53637,#53638,#53639,#53640,#53641,
#53642,#53643,#53644,#53645,#53646),.UNSPECIFIED.,.F.,.F.,(4,1,1,1,1,1,
1,4),(53.4070751110265,53.8595736735331,54.8461030121971,55.8326323508611,
56.8191616895252,57.8056910281892,58.7922203668532,59.6902604182061),
 .UNSPECIFIED.);
#4045=B_SPLINE_CURVE_WITH_KNOTS('',3,(#53651,#53652,#53653,#53654,#53655,
#53656,#53657,#53658,#53659,#53660,#53661),.UNSPECIFIED.,.F.,.F.,(4,1,1,
1,1,1,1,1,4),(47.1238898038469,47.3704174554844,48.3569467941485,49.3434761328125,
50.3300054714765,51.3165348101406,52.3030641488046,53.2895934874686,53.4070751110265),
 .UNSPECIFIED.);
#4046=B_SPLINE_CURVE_WITH_KNOTS('',3,(#53662,#53663,#53664,#53665,#53666,
#53667,#53668,#53669,#53670,#53671),.UNSPECIFIED.,.F.,.F.,(4,1,1,1,1,1,
1,4),(47.1238898038469,47.9403976415489,48.9269269802129,49.9134563188769,
50.899985657541,51.886514996205,52.873044334869,53.4070751110265),
 .UNSPECIFIED.);
#4047=B_SPLINE_CURVE_WITH_KNOTS('',3,(#53676,#53677,#53678,#53679,#53680,
#53681,#53682,#53683,#53684,#53685),.UNSPECIFIED.,.F.,.F.,(4,1,1,1,1,1,
1,4),(40.8407044966673,41.4512414235002,42.4377707621643,43.4243001008283,
44.4108294394923,45.3973587781564,46.3838881168204,47.1238898038469),
 .UNSPECIFIED.);
#4048=B_SPLINE_CURVE_WITH_KNOTS('',3,(#53686,#53687,#53688,#53689,#53690,
#53691,#53692,#53693,#53694,#53695,#53696),.UNSPECIFIED.,.F.,.F.,(4,1,1,
1,1,1,1,1,4),(40.8407044966673,41.0346922709007,42.0212216095647,43.0077509482287,
43.9942802868928,44.9808096255568,45.9673389642208,46.9538683028849,47.1238898038469),
 .UNSPECIFIED.);
#4049=B_SPLINE_CURVE_WITH_KNOTS('',3,(#53701,#53702,#53703,#53704,#53705,
#53706,#53707,#53708,#53709,#53710),.UNSPECIFIED.,.F.,.F.,(4,1,1,1,1,1,
1,4),(34.5575191894877,35.5320653915161,36.5185947301801,37.5051240688441,
38.4916534075082,39.4781827461722,40.4647120848362,40.8407044966673),
 .UNSPECIFIED.);
#4050=B_SPLINE_CURVE_WITH_KNOTS('',3,(#53711,#53712,#53713,#53714,#53715,
#53716,#53717,#53718,#53719,#53720),.UNSPECIFIED.,.F.,.F.,(4,1,1,1,1,1,
1,4),(34.5575191894877,35.1155162389165,36.1020455775805,37.0885749162445,
38.0751042549086,39.0616335935726,40.0481629322366,40.8407044966673),
 .UNSPECIFIED.);
#4051=B_SPLINE_CURVE_WITH_KNOTS('',3,(#53725,#53726,#53727,#53728,#53729,
#53730,#53731,#53732,#53733,#53734,#53735),.UNSPECIFIED.,.F.,.F.,(4,1,1,
1,1,1,1,1,4),(28.2743338823081,28.6263600208679,29.6128893595319,30.5994186981959,
31.5859480368599,32.572477375524,33.559006714188,34.545536052852,34.5575191894877),
 .UNSPECIFIED.);
#4052=B_SPLINE_CURVE_WITH_KNOTS('',3,(#53736,#53737,#53738,#53739,#53740,
#53741,#53742,#53743,#53744,#53745),.UNSPECIFIED.,.F.,.F.,(4,1,1,1,1,1,
1,4),(28.2743338823081,29.1963402069323,30.1828695455963,31.1693988842604,
32.1559282229244,33.1424575615884,34.1289869002525,34.5575191894877),
 .UNSPECIFIED.);
#4053=B_SPLINE_CURVE_WITH_KNOTS('',3,(#53750,#53751,#53752,#53753,#53754,
#53755,#53756,#53757,#53758,#53759),.UNSPECIFIED.,.F.,.F.,(4,1,1,1,1,1,
1,4),(21.9911485751285,22.7071839888837,23.6937133275477,24.6802426662117,
25.6667720048758,26.6533013435398,27.6398306822038,28.2743338823081),
 .UNSPECIFIED.);
#4054=B_SPLINE_CURVE_WITH_KNOTS('',3,(#53760,#53761,#53762,#53763,#53764,
#53765,#53766,#53767,#53768,#53769,#53770),.UNSPECIFIED.,.F.,.F.,(4,1,1,
1,1,1,1,1,4),(21.9911485751285,22.2906348362841,23.2771641749481,24.2636935136121,
25.2502228522762,26.2367521909402,27.2232815296042,28.2098108682683,28.2743338823081),
 .UNSPECIFIED.);
#4055=B_SPLINE_CURVE_WITH_KNOTS('',3,(#53776,#53777,#53778,#53779,#53780),
 .UNSPECIFIED.,.F.,.F.,(4,1,4),(14.3984001269718,15.3849294656359,15.7079632679489),
 .UNSPECIFIED.);
#4056=B_SPLINE_CURVE_WITH_KNOTS('',3,(#53783,#53784,#53785,#53786,#53787),
 .UNSPECIFIED.,.F.,.F.,(4,1,4),(13.8759337553363,14.8149492795714,15.7079632679489),
 .UNSPECIFIED.);
#4057=B_SPLINE_CURVE_WITH_KNOTS('',3,(#53793,#53794,#53795,#53796),
 .UNSPECIFIED.,.F.,.F.,(4,4),(51.5750455984138,52.2860549491936),
 .UNSPECIFIED.);
#4058=B_SPLINE_CURVE_WITH_KNOTS('',3,(#53808,#53809,#53810,#53811,#53812,
#53813,#53814,#53815,#53816,#53817),.UNSPECIFIED.,.F.,.F.,(4,3,3,4),(-50.2654824574367,
-49.3264669332015,-48.3399375945375,-47.8348991546267),.UNSPECIFIED.);
#4059=B_SPLINE_CURVE_WITH_KNOTS('',3,(#53822,#53823,#53824,#53825,#53826,
#53827,#53828,#53829,#53830,#53831,#53832,#53833,#53834,#53835,#53836,#53837,
#53838,#53839,#53840,#53841,#53842,#53843,#53844,#53845,#53846),
 .UNSPECIFIED.,.F.,.F.,(4,3,3,3,3,3,3,3,4),(45.2918602912342,45.3803495785454,
46.3668789172094,47.3534082558735,48.3399375945375,49.3264669332015,50.3129962718655,
51.2995256105296,51.5750455984138),.UNSPECIFIED.);
#4060=B_SPLINE_CURVE_WITH_KNOTS('',3,(#53847,#53848,#53849,#53850,#53851,
#53852,#53853,#53854,#53855,#53856,#53857,#53858,#53859,#53860,#53861,#53862,
#53863,#53864,#53865,#53866,#53867,#53868),.UNSPECIFIED.,.F.,.F.,(4,3,3,
3,3,3,3,4),(-47.8348991546267,-47.3534082558735,-46.3668789172094,-45.3803495785454,
-44.3938202398814,-43.4072909012173,-42.4207615625533,-41.5517138474471),
 .UNSPECIFIED.);
#4061=B_SPLINE_CURVE_WITH_KNOTS('',3,(#53873,#53874,#53875,#53876,#53877,
#53878,#53879,#53880,#53881,#53882,#53883,#53884,#53885,#53886,#53887,#53888,
#53889,#53890,#53891,#53892,#53893,#53894),.UNSPECIFIED.,.F.,.F.,(4,3,3,
3,3,3,3,4),(39.0086749840546,39.4611735465612,40.4477028852252,41.4342322238893,
42.4207615625533,43.4072909012173,44.3938202398814,45.2918602912342),
 .UNSPECIFIED.);
#4062=B_SPLINE_CURVE_WITH_KNOTS('',3,(#53895,#53896,#53897,#53898,#53899,
#53900,#53901,#53902,#53903,#53904,#53905,#53906,#53907,#53908,#53909,#53910,
#53911,#53912,#53913,#53914,#53915,#53916,#53917,#53918,#53919),
 .UNSPECIFIED.,.F.,.F.,(4,3,3,3,3,3,3,3,4),(-41.5517138474471,-41.4342322238893,
-40.4477028852252,-39.4611735465612,-38.4746442078972,-37.4881148692332,
-36.5015855305691,-35.5150561919051,-35.2685285402675),.UNSPECIFIED.);
#4063=B_SPLINE_CURVE_WITH_KNOTS('',3,(#53924,#53925,#53926,#53927,#53928,
#53929,#53930,#53931,#53932,#53933,#53934,#53935,#53936,#53937,#53938,#53939,
#53940,#53941,#53942,#53943,#53944,#53945),.UNSPECIFIED.,.F.,.F.,(4,3,3,
3,3,3,3,4),(32.725489676875,33.541997514577,34.5285268532411,35.5150561919051,
36.5015855305691,37.4881148692332,38.4746442078972,39.0086749840546),
 .UNSPECIFIED.);
#4064=B_SPLINE_CURVE_WITH_KNOTS('',3,(#53946,#53947,#53948,#53949,#53950,
#53951,#53952,#53953,#53954,#53955,#53956,#53957,#53958,#53959,#53960,#53961,
#53962,#53963,#53964,#53965,#53966,#53967),.UNSPECIFIED.,.F.,.F.,(4,3,3,
3,3,3,3,4),(-35.2685285402675,-34.5285268532411,-33.541997514577,-32.555468175913,
-31.568938837249,-30.582409498585,-29.5958801599209,-28.9853432330879),
 .UNSPECIFIED.);
#4065=B_SPLINE_CURVE_WITH_KNOTS('',3,(#53972,#53973,#53974,#53975,#53976,
#53977,#53978,#53979,#53980,#53981,#53982,#53983,#53984,#53985,#53986,#53987,
#53988,#53989,#53990,#53991,#53992,#53993,#53994,#53995,#53996),
 .UNSPECIFIED.,.F.,.F.,(4,3,3,3,3,3,3,3,4),(26.4423043696954,26.6362921439288,
27.6228214825928,28.6093508212569,29.5958801599209,30.5824094985849,31.568938837249,
32.555468175913,32.725489676875),.UNSPECIFIED.);
#4066=B_SPLINE_CURVE_WITH_KNOTS('',3,(#53997,#53998,#53999,#54000,#54001,
#54002,#54003,#54004,#54005,#54006,#54007,#54008,#54009,#54010,#54011,#54012,
#54013,#54014,#54015,#54016,#54017,#54018),.UNSPECIFIED.,.F.,.F.,(4,3,3,
3,3,3,3,4),(-28.9853432330879,-28.6093508212569,-27.6228214825929,-26.6362921439288,
-25.6497628052648,-24.6632334666008,-23.6767041279367,-22.7021579259084),
 .UNSPECIFIED.);
#4067=B_SPLINE_CURVE_WITH_KNOTS('',3,(#54023,#54024,#54025,#54026,#54027,
#54028,#54029,#54030,#54031,#54032,#54033,#54034,#54035,#54036,#54037,#54038,
#54039,#54040,#54041,#54042,#54043,#54044),.UNSPECIFIED.,.F.,.F.,(4,3,3,
3,3,3,3,4),(20.1591190625158,20.7171161119446,21.7036454506087,22.6901747892727,
23.6767041279367,24.6632334666008,25.6497628052648,26.4423043696954),
 .UNSPECIFIED.);
#4068=B_SPLINE_CURVE_WITH_KNOTS('',3,(#54045,#54046,#54047,#54048,#54049,
#54050,#54051,#54052,#54053,#54054,#54055,#54056,#54057,#54058,#54059,#54060,
#54061,#54062,#54063,#54064,#54065,#54066,#54067,#54068,#54069),
 .UNSPECIFIED.,.F.,.F.,(4,3,3,3,3,3,3,3,4),(-22.7021579259084,-22.6901747892727,
-21.7036454506087,-20.7171161119446,-19.7305867732806,-18.7440574346166,
-17.7575280959525,-16.7709987572885,-16.4189726187288),.UNSPECIFIED.);
#4069=B_SPLINE_CURVE_WITH_KNOTS('',3,(#54074,#54075,#54076,#54077,#54078,
#54079,#54080,#54081,#54082,#54083,#54084,#54085,#54086,#54087,#54088,#54089,
#54090,#54091,#54092,#54093,#54094,#54095),.UNSPECIFIED.,.F.,.F.,(4,3,3,
3,3,3,3,4),(13.8759337553362,14.7979400799604,15.7844694186245,16.7709987572885,
17.7575280959525,18.7440574346166,19.7305867732806,20.1591190625158),
 .UNSPECIFIED.);
#4070=B_SPLINE_CURVE_WITH_KNOTS('',3,(#54096,#54097,#54098,#54099,#54100,
#54101,#54102,#54103,#54104,#54105,#54106,#54107,#54108,#54109,#54110,#54111,
#54112,#54113,#54114,#54115,#54116,#54117),.UNSPECIFIED.,.F.,.F.,(4,3,3,
3,3,3,3,4),(-16.4189726187288,-15.7844694186245,-14.7979400799605,-13.8114107412964,
-12.8248814026324,-11.8383520639684,-10.8518227253043,-10.1357873115492),
 .UNSPECIFIED.);
#4071=B_SPLINE_CURVE_WITH_KNOTS('',3,(#54123,#54124,#54125,#54126,#54127,
#54128,#54129,#54130,#54131,#54132,#54133,#54134,#54135),.UNSPECIFIED.,
 .F.,.F.,(4,3,3,3,4),(-3.85260200436958,-2.95958801599209,-1.97305867732806,
-0.986529338664032,0.),.UNSPECIFIED.);
#4072=B_SPLINE_CURVE_WITH_KNOTS('',3,(#54138,#54139,#54140,#54141,#54142,
#54143,#54144,#54145,#54146,#54147,#54148,#54149,#54150,#54151,#54152,#54153,
#54154,#54155,#54156),.UNSPECIFIED.,.F.,.F.,(4,3,3,3,3,3,4),(2.02057249175685,
2.95958801599209,3.94611735465612,4.93264669332016,5.91917603198418,6.90570537064822,
7.59274844815664),.UNSPECIFIED.);
#4073=B_SPLINE_CURVE_WITH_KNOTS('',3,(#54162,#54163,#54164,#54165,#54166,
#54167,#54168,#54169),.UNSPECIFIED.,.F.,.F.,(4,1,1,1,1,4),(59.6902604182061,
60.1952988581168,61.1818281967808,62.1683575354449,63.1548868741089,64.1414162127729),
 .UNSPECIFIED.);
#4074=B_SPLINE_CURVE_WITH_KNOTS('',3,(#54172,#54173,#54174,#54175,#54176,
#54177,#54178,#54179,#54180),.UNSPECIFIED.,.F.,.F.,(4,1,1,1,1,1,4),(59.6902604182061,
59.7787497055172,60.7652790441813,61.7518083828453,62.7383377215093,63.7248670601733,
64.6638825844085),.UNSPECIFIED.);
#4075=B_SPLINE_CURVE_WITH_KNOTS('',3,(#54185,#54186,#54187,#54188,#54189,
#54190,#54191,#54192,#54193,#54194),.UNSPECIFIED.,.F.,.F.,(4,1,1,1,1,1,
1,4),(53.4070751110265,54.2761228261326,55.2626521647967,56.2491815034607,
57.2357108421247,58.2222401807888,59.2087695194528,59.6902604182061),
 .UNSPECIFIED.);
#4076=B_SPLINE_CURVE_WITH_KNOTS('',3,(#54195,#54196,#54197,#54198,#54199,
#54200,#54201,#54202,#54203,#54204),.UNSPECIFIED.,.F.,.F.,(4,1,1,1,1,1,
1,4),(53.4070751110265,53.859573673533,54.8461030121971,55.8326323508611,
56.8191616895251,57.8056910281892,58.7922203668532,59.6902604182061),
 .UNSPECIFIED.);
#4077=B_SPLINE_CURVE_WITH_KNOTS('',3,(#54209,#54210,#54211,#54212,#54213,
#54214,#54215,#54216,#54217,#54218,#54219),.UNSPECIFIED.,.F.,.F.,(4,1,1,
1,1,1,1,1,4),(47.1238898038469,47.3704174554844,48.3569467941485,49.3434761328125,
50.3300054714765,51.3165348101405,52.3030641488046,53.2895934874686,53.4070751110265),
 .UNSPECIFIED.);
#4078=B_SPLINE_CURVE_WITH_KNOTS('',3,(#54220,#54221,#54222,#54223,#54224,
#54225,#54226,#54227,#54228,#54229),.UNSPECIFIED.,.F.,.F.,(4,1,1,1,1,1,
1,4),(47.1238898038469,47.9403976415489,48.9269269802129,49.9134563188769,
50.899985657541,51.886514996205,52.873044334869,53.4070751110265),
 .UNSPECIFIED.);
#4079=B_SPLINE_CURVE_WITH_KNOTS('',3,(#54234,#54235,#54236,#54237,#54238,
#54239,#54240,#54241,#54242,#54243),.UNSPECIFIED.,.F.,.F.,(4,1,1,1,1,1,
1,4),(40.8407044966673,41.4512414235002,42.4377707621643,43.4243001008283,
44.4108294394923,45.3973587781564,46.3838881168204,47.1238898038469),
 .UNSPECIFIED.);
#4080=B_SPLINE_CURVE_WITH_KNOTS('',3,(#54244,#54245,#54246,#54247,#54248,
#54249,#54250,#54251,#54252,#54253,#54254),.UNSPECIFIED.,.F.,.F.,(4,1,1,
1,1,1,1,1,4),(40.8407044966673,41.0346922709006,42.0212216095647,43.0077509482287,
43.9942802868927,44.9808096255568,45.9673389642208,46.9538683028848,47.1238898038469),
 .UNSPECIFIED.);
#4081=B_SPLINE_CURVE_WITH_KNOTS('',3,(#54259,#54260,#54261,#54262,#54263,
#54264,#54265,#54266,#54267,#54268),.UNSPECIFIED.,.F.,.F.,(4,1,1,1,1,1,
1,4),(34.5575191894877,35.5320653915161,36.5185947301801,37.5051240688441,
38.4916534075082,39.4781827461722,40.4647120848362,40.8407044966673),
 .UNSPECIFIED.);
#4082=B_SPLINE_CURVE_WITH_KNOTS('',3,(#54269,#54270,#54271,#54272,#54273,
#54274,#54275,#54276,#54277,#54278),.UNSPECIFIED.,.F.,.F.,(4,1,1,1,1,1,
1,4),(34.5575191894877,35.1155162389165,36.1020455775805,37.0885749162445,
38.0751042549086,39.0616335935726,40.0481629322366,40.8407044966673),
 .UNSPECIFIED.);
#4083=B_SPLINE_CURVE_WITH_KNOTS('',3,(#54283,#54284,#54285,#54286,#54287,
#54288,#54289,#54290,#54291,#54292,#54293),.UNSPECIFIED.,.F.,.F.,(4,1,1,
1,1,1,1,1,4),(28.2743338823081,28.6263600208678,29.6128893595319,30.5994186981959,
31.5859480368599,32.572477375524,33.559006714188,34.545536052852,34.5575191894877),
 .UNSPECIFIED.);
#4084=B_SPLINE_CURVE_WITH_KNOTS('',3,(#54294,#54295,#54296,#54297,#54298,
#54299,#54300,#54301,#54302,#54303),.UNSPECIFIED.,.F.,.F.,(4,1,1,1,1,1,
1,4),(28.2743338823081,29.1963402069323,30.1828695455963,31.1693988842603,
32.1559282229244,33.1424575615884,34.1289869002524,34.5575191894877),
 .UNSPECIFIED.);
#4085=B_SPLINE_CURVE_WITH_KNOTS('',3,(#54308,#54309,#54310,#54311,#54312,
#54313,#54314,#54315,#54316,#54317),.UNSPECIFIED.,.F.,.F.,(4,1,1,1,1,1,
1,4),(21.9911485751285,22.7071839888837,23.6937133275477,24.6802426662117,
25.6667720048758,26.6533013435398,27.6398306822038,28.2743338823081),
 .UNSPECIFIED.);
#4086=B_SPLINE_CURVE_WITH_KNOTS('',3,(#54318,#54319,#54320,#54321,#54322,
#54323,#54324,#54325,#54326,#54327,#54328),.UNSPECIFIED.,.F.,.F.,(4,1,1,
1,1,1,1,1,4),(21.9911485751285,22.2906348362841,23.2771641749481,24.2636935136121,
25.2502228522762,26.2367521909402,27.2232815296042,28.2098108682683,28.2743338823081),
 .UNSPECIFIED.);
#4087=B_SPLINE_CURVE_WITH_KNOTS('',3,(#54334,#54335,#54336,#54337,#54338),
 .UNSPECIFIED.,.F.,.F.,(4,1,4),(14.3984001269718,15.3849294656359,15.7079632679489),
 .UNSPECIFIED.);
#4088=B_SPLINE_CURVE_WITH_KNOTS('',3,(#54341,#54342,#54343,#54344,#54345),
 .UNSPECIFIED.,.F.,.F.,(4,1,4),(13.8759337553363,14.8149492795714,15.7079632679489),
 .UNSPECIFIED.);
#4089=B_SPLINE_CURVE_WITH_KNOTS('',3,(#54351,#54352,#54353,#54354),
 .UNSPECIFIED.,.F.,.F.,(4,4),(51.5750455984138,52.2860549491936),
 .UNSPECIFIED.);
#4090=B_SPLINE_CURVE_WITH_KNOTS('',3,(#54366,#54367,#54368,#54369,#54370,
#54371,#54372,#54373,#54374,#54375),.UNSPECIFIED.,.F.,.F.,(4,3,3,4),(-50.2654824574367,
-49.3264669332015,-48.3399375945375,-47.8348991546267),.UNSPECIFIED.);
#4091=B_SPLINE_CURVE_WITH_KNOTS('',3,(#54380,#54381,#54382,#54383,#54384,
#54385,#54386,#54387,#54388,#54389,#54390,#54391,#54392,#54393,#54394,#54395,
#54396,#54397,#54398,#54399,#54400,#54401,#54402,#54403,#54404),
 .UNSPECIFIED.,.F.,.F.,(4,3,3,3,3,3,3,3,4),(45.2918602912342,45.3803495785454,
46.3668789172094,47.3534082558735,48.3399375945375,49.3264669332015,50.3129962718656,
51.2995256105296,51.5750455984138),.UNSPECIFIED.);
#4092=B_SPLINE_CURVE_WITH_KNOTS('',3,(#54405,#54406,#54407,#54408,#54409,
#54410,#54411,#54412,#54413,#54414,#54415,#54416,#54417,#54418,#54419,#54420,
#54421,#54422,#54423,#54424,#54425,#54426),.UNSPECIFIED.,.F.,.F.,(4,3,3,
3,3,3,3,4),(-47.8348991546267,-47.3534082558735,-46.3668789172095,-45.3803495785454,
-44.3938202398814,-43.4072909012174,-42.4207615625533,-41.5517138474471),
 .UNSPECIFIED.);
#4093=B_SPLINE_CURVE_WITH_KNOTS('',3,(#54431,#54432,#54433,#54434,#54435,
#54436,#54437,#54438,#54439,#54440,#54441,#54442,#54443,#54444,#54445,#54446,
#54447,#54448,#54449,#54450,#54451,#54452),.UNSPECIFIED.,.F.,.F.,(4,3,3,
3,3,3,3,4),(39.0086749840546,39.4611735465612,40.4477028852253,41.4342322238893,
42.4207615625533,43.4072909012174,44.3938202398814,45.2918602912342),
 .UNSPECIFIED.);
#4094=B_SPLINE_CURVE_WITH_KNOTS('',3,(#54453,#54454,#54455,#54456,#54457,
#54458,#54459,#54460,#54461,#54462,#54463,#54464,#54465,#54466,#54467,#54468,
#54469,#54470,#54471,#54472,#54473,#54474,#54475,#54476,#54477),
 .UNSPECIFIED.,.F.,.F.,(4,3,3,3,3,3,3,3,4),(-41.5517138474471,-41.4342322238893,
-40.4477028852253,-39.4611735465612,-38.4746442078972,-37.4881148692332,
-36.5015855305691,-35.5150561919051,-35.2685285402675),.UNSPECIFIED.);
#4095=B_SPLINE_CURVE_WITH_KNOTS('',3,(#54482,#54483,#54484,#54485,#54486,
#54487,#54488,#54489,#54490,#54491,#54492,#54493,#54494,#54495,#54496,#54497,
#54498,#54499,#54500,#54501,#54502,#54503),.UNSPECIFIED.,.F.,.F.,(4,3,3,
3,3,3,3,4),(32.725489676875,33.541997514577,34.5285268532411,35.5150561919051,
36.5015855305691,37.4881148692332,38.4746442078972,39.0086749840546),
 .UNSPECIFIED.);
#4096=B_SPLINE_CURVE_WITH_KNOTS('',3,(#54504,#54505,#54506,#54507,#54508,
#54509,#54510,#54511,#54512,#54513,#54514,#54515,#54516,#54517,#54518,#54519,
#54520,#54521,#54522,#54523,#54524,#54525),.UNSPECIFIED.,.F.,.F.,(4,3,3,
3,3,3,3,4),(-35.2685285402675,-34.5285268532411,-33.541997514577,-32.555468175913,
-31.568938837249,-30.582409498585,-29.5958801599209,-28.9853432330879),
 .UNSPECIFIED.);
#4097=B_SPLINE_CURVE_WITH_KNOTS('',3,(#54530,#54531,#54532,#54533,#54534,
#54535,#54536,#54537,#54538,#54539,#54540,#54541,#54542,#54543,#54544,#54545,
#54546,#54547,#54548,#54549,#54550,#54551,#54552,#54553,#54554),
 .UNSPECIFIED.,.F.,.F.,(4,3,3,3,3,3,3,3,4),(26.4423043696954,26.6362921439288,
27.6228214825929,28.6093508212569,29.5958801599209,30.582409498585,31.568938837249,
32.555468175913,32.725489676875),.UNSPECIFIED.);
#4098=B_SPLINE_CURVE_WITH_KNOTS('',3,(#54555,#54556,#54557,#54558,#54559,
#54560,#54561,#54562,#54563,#54564,#54565,#54566,#54567,#54568,#54569,#54570,
#54571,#54572,#54573,#54574,#54575,#54576),.UNSPECIFIED.,.F.,.F.,(4,3,3,
3,3,3,3,4),(-28.9853432330879,-28.6093508212569,-27.6228214825929,-26.6362921439288,
-25.6497628052648,-24.6632334666008,-23.6767041279367,-22.7021579259083),
 .UNSPECIFIED.);
#4099=B_SPLINE_CURVE_WITH_KNOTS('',3,(#54581,#54582,#54583,#54584,#54585,
#54586,#54587,#54588,#54589,#54590,#54591,#54592,#54593,#54594,#54595,#54596,
#54597,#54598,#54599,#54600,#54601,#54602),.UNSPECIFIED.,.F.,.F.,(4,3,3,
3,3,3,3,4),(20.1591190625158,20.7171161119446,21.7036454506087,22.6901747892727,
23.6767041279367,24.6632334666008,25.6497628052648,26.4423043696954),
 .UNSPECIFIED.);
#4100=B_SPLINE_CURVE_WITH_KNOTS('',3,(#54603,#54604,#54605,#54606,#54607,
#54608,#54609,#54610,#54611,#54612,#54613,#54614,#54615,#54616,#54617,#54618,
#54619,#54620,#54621,#54622,#54623,#54624,#54625,#54626,#54627),
 .UNSPECIFIED.,.F.,.F.,(4,3,3,3,3,3,3,3,4),(-22.7021579259083,-22.6901747892727,
-21.7036454506087,-20.7171161119447,-19.7305867732806,-18.7440574346166,
-17.7575280959526,-16.7709987572885,-16.4189726187287),.UNSPECIFIED.);
#4101=B_SPLINE_CURVE_WITH_KNOTS('',3,(#54632,#54633,#54634,#54635,#54636,
#54637,#54638,#54639,#54640,#54641,#54642,#54643,#54644,#54645,#54646,#54647,
#54648,#54649,#54650,#54651,#54652,#54653),.UNSPECIFIED.,.F.,.F.,(4,3,3,
3,3,3,3,4),(13.8759337553362,14.7979400799605,15.7844694186245,16.7709987572885,
17.7575280959526,18.7440574346166,19.7305867732806,20.1591190625158),
 .UNSPECIFIED.);
#4102=B_SPLINE_CURVE_WITH_KNOTS('',3,(#54654,#54655,#54656,#54657,#54658,
#54659,#54660,#54661,#54662,#54663,#54664,#54665,#54666,#54667,#54668,#54669,
#54670,#54671,#54672,#54673,#54674,#54675),.UNSPECIFIED.,.F.,.F.,(4,3,3,
3,3,3,3,4),(-16.4189726187287,-15.7844694186245,-14.7979400799605,-13.8114107412964,
-12.8248814026324,-11.8383520639684,-10.8518227253043,-10.1357873115491),
 .UNSPECIFIED.);
#4103=B_SPLINE_CURVE_WITH_KNOTS('',3,(#54681,#54682,#54683,#54684,#54685,
#54686,#54687,#54688,#54689,#54690,#54691,#54692,#54693),.UNSPECIFIED.,
 .F.,.F.,(4,3,3,3,4),(-3.85260200436958,-2.95958801599209,-1.97305867732806,
-0.986529338664031,0.),.UNSPECIFIED.);
#4104=B_SPLINE_CURVE_WITH_KNOTS('',3,(#54696,#54697,#54698,#54699,#54700,
#54701,#54702,#54703,#54704,#54705,#54706,#54707,#54708,#54709,#54710,#54711,
#54712,#54713,#54714),.UNSPECIFIED.,.F.,.F.,(4,3,3,3,3,3,4),(2.02057249175696,
2.95958801599209,3.94611735465612,4.93264669332015,5.91917603198418,6.90570537064821,
7.59274844815661),.UNSPECIFIED.);
#4105=B_SPLINE_CURVE_WITH_KNOTS('',3,(#54720,#54721,#54722,#54723,#54724,
#54725,#54726,#54727),.UNSPECIFIED.,.F.,.F.,(4,1,1,1,1,4),(59.6902604182061,
60.1952988581169,61.1818281967809,62.1683575354449,63.154886874109,64.141416212773),
 .UNSPECIFIED.);
#4106=B_SPLINE_CURVE_WITH_KNOTS('',3,(#54730,#54731,#54732,#54733,#54734,
#54735,#54736,#54737,#54738),.UNSPECIFIED.,.F.,.F.,(4,1,1,1,1,1,4),(59.6902604182061,
59.7787497055173,60.7652790441813,61.7518083828453,62.7383377215094,63.7248670601734,
64.6638825844086),.UNSPECIFIED.);
#4107=B_SPLINE_CURVE_WITH_KNOTS('',3,(#54743,#54744,#54745,#54746,#54747,
#54748,#54749,#54750,#54751,#54752),.UNSPECIFIED.,.F.,.F.,(4,1,1,1,1,1,
1,4),(53.4070751110265,54.2761228261327,55.2626521647967,56.2491815034607,
57.2357108421248,58.2222401807888,59.2087695194528,59.6902604182061),
 .UNSPECIFIED.);
#4108=B_SPLINE_CURVE_WITH_KNOTS('',3,(#54753,#54754,#54755,#54756,#54757,
#54758,#54759,#54760,#54761,#54762),.UNSPECIFIED.,.F.,.F.,(4,1,1,1,1,1,
1,4),(53.4070751110265,53.8595736735331,54.8461030121971,55.8326323508612,
56.8191616895252,57.8056910281892,58.7922203668532,59.6902604182061),
 .UNSPECIFIED.);
#4109=B_SPLINE_CURVE_WITH_KNOTS('',3,(#54767,#54768,#54769,#54770,#54771,
#54772,#54773,#54774,#54775,#54776,#54777),.UNSPECIFIED.,.F.,.F.,(4,1,1,
1,1,1,1,1,4),(47.1238898038469,47.3704174554845,48.3569467941485,49.3434761328125,
50.3300054714766,51.3165348101406,52.3030641488046,53.2895934874687,53.4070751110265),
 .UNSPECIFIED.);
#4110=B_SPLINE_CURVE_WITH_KNOTS('',3,(#54778,#54779,#54780,#54781,#54782,
#54783,#54784,#54785,#54786,#54787),.UNSPECIFIED.,.F.,.F.,(4,1,1,1,1,1,
1,4),(47.1238898038469,47.9403976415489,48.9269269802129,49.913456318877,
50.899985657541,51.886514996205,52.8730443348691,53.4070751110265),
 .UNSPECIFIED.);
#4111=B_SPLINE_CURVE_WITH_KNOTS('',3,(#54792,#54793,#54794,#54795,#54796,
#54797,#54798,#54799,#54800,#54801),.UNSPECIFIED.,.F.,.F.,(4,1,1,1,1,1,
1,4),(40.8407044966673,41.4512414235003,42.4377707621643,43.4243001008283,
44.4108294394924,45.3973587781564,46.3838881168204,47.1238898038469),
 .UNSPECIFIED.);
#4112=B_SPLINE_CURVE_WITH_KNOTS('',3,(#54802,#54803,#54804,#54805,#54806,
#54807,#54808,#54809,#54810,#54811,#54812),.UNSPECIFIED.,.F.,.F.,(4,1,1,
1,1,1,1,1,4),(40.8407044966673,41.0346922709007,42.0212216095647,43.0077509482288,
43.9942802868928,44.9808096255568,45.9673389642208,46.9538683028849,47.1238898038469),
 .UNSPECIFIED.);
#4113=B_SPLINE_CURVE_WITH_KNOTS('',3,(#54817,#54818,#54819,#54820,#54821,
#54822,#54823,#54824,#54825,#54826),.UNSPECIFIED.,.F.,.F.,(4,1,1,1,1,1,
1,4),(34.5575191894877,35.5320653915161,36.5185947301801,37.5051240688442,
38.4916534075082,39.4781827461722,40.4647120848363,40.8407044966673),
 .UNSPECIFIED.);
#4114=B_SPLINE_CURVE_WITH_KNOTS('',3,(#54827,#54828,#54829,#54830,#54831,
#54832,#54833,#54834,#54835,#54836),.UNSPECIFIED.,.F.,.F.,(4,1,1,1,1,1,
1,4),(34.5575191894877,35.1155162389165,36.1020455775805,37.0885749162446,
38.0751042549086,39.0616335935726,40.0481629322367,40.8407044966673),
 .UNSPECIFIED.);
#4115=B_SPLINE_CURVE_WITH_KNOTS('',3,(#54841,#54842,#54843,#54844,#54845,
#54846,#54847,#54848,#54849,#54850,#54851),.UNSPECIFIED.,.F.,.F.,(4,1,1,
1,1,1,1,1,4),(28.2743338823081,28.6263600208679,29.6128893595319,30.5994186981959,
31.58594803686,32.572477375524,33.559006714188,34.5455360528521,34.5575191894877),
 .UNSPECIFIED.);
#4116=B_SPLINE_CURVE_WITH_KNOTS('',3,(#54852,#54853,#54854,#54855,#54856,
#54857,#54858,#54859,#54860,#54861),.UNSPECIFIED.,.F.,.F.,(4,1,1,1,1,1,
1,4),(28.2743338823081,29.1963402069323,30.1828695455964,31.1693988842604,
32.1559282229244,33.1424575615884,34.1289869002525,34.5575191894877),
 .UNSPECIFIED.);
#4117=B_SPLINE_CURVE_WITH_KNOTS('',3,(#54866,#54867,#54868,#54869,#54870,
#54871,#54872,#54873,#54874,#54875),.UNSPECIFIED.,.F.,.F.,(4,1,1,1,1,1,
1,4),(21.9911485751285,22.7071839888837,23.6937133275477,24.6802426662118,
25.6667720048758,26.6533013435398,27.6398306822039,28.2743338823081),
 .UNSPECIFIED.);
#4118=B_SPLINE_CURVE_WITH_KNOTS('',3,(#54876,#54877,#54878,#54879,#54880,
#54881,#54882,#54883,#54884,#54885,#54886),.UNSPECIFIED.,.F.,.F.,(4,1,1,
1,1,1,1,1,4),(21.9911485751285,22.2906348362841,23.2771641749481,24.2636935136122,
25.2502228522762,26.2367521909402,27.2232815296043,28.2098108682683,28.2743338823081),
 .UNSPECIFIED.);
#4119=B_SPLINE_CURVE_WITH_KNOTS('',3,(#54892,#54893,#54894,#54895,#54896),
 .UNSPECIFIED.,.F.,.F.,(4,1,4),(14.3984001269719,15.3849294656359,15.7079632679489),
 .UNSPECIFIED.);
#4120=B_SPLINE_CURVE_WITH_KNOTS('',3,(#54899,#54900,#54901,#54902,#54903),
 .UNSPECIFIED.,.F.,.F.,(4,1,4),(13.8759337553363,14.8149492795714,15.7079632679489),
 .UNSPECIFIED.);
#4121=B_SPLINE_CURVE_WITH_KNOTS('',3,(#54909,#54910,#54911,#54912),
 .UNSPECIFIED.,.F.,.F.,(4,4),(51.5750455984138,52.2860549491936),
 .UNSPECIFIED.);
#4122=B_SPLINE_CURVE_WITH_KNOTS('',3,(#54924,#54925,#54926,#54927,#54928,
#54929,#54930,#54931,#54932,#54933),.UNSPECIFIED.,.F.,.F.,(4,3,3,4),(-50.2654824574366,
-49.3264669332015,-48.3399375945375,-47.8348991546267),.UNSPECIFIED.);
#4123=B_SPLINE_CURVE_WITH_KNOTS('',3,(#54938,#54939,#54940,#54941,#54942,
#54943,#54944,#54945,#54946,#54947,#54948,#54949,#54950,#54951,#54952,#54953,
#54954,#54955,#54956,#54957,#54958,#54959,#54960,#54961,#54962),
 .UNSPECIFIED.,.F.,.F.,(4,3,3,3,3,3,3,3,4),(45.2918602912342,45.3803495785454,
46.3668789172094,47.3534082558735,48.3399375945375,49.3264669332015,50.3129962718656,
51.2995256105296,51.5750455984138),.UNSPECIFIED.);
#4124=B_SPLINE_CURVE_WITH_KNOTS('',3,(#54963,#54964,#54965,#54966,#54967,
#54968,#54969,#54970,#54971,#54972,#54973,#54974,#54975,#54976,#54977,#54978,
#54979,#54980,#54981,#54982,#54983,#54984),.UNSPECIFIED.,.F.,.F.,(4,3,3,
3,3,3,3,4),(-47.8348991546267,-47.3534082558735,-46.3668789172094,-45.3803495785454,
-44.3938202398814,-43.4072909012173,-42.4207615625533,-41.5517138474471),
 .UNSPECIFIED.);
#4125=B_SPLINE_CURVE_WITH_KNOTS('',3,(#54989,#54990,#54991,#54992,#54993,
#54994,#54995,#54996,#54997,#54998,#54999,#55000,#55001,#55002,#55003,#55004,
#55005,#55006,#55007,#55008,#55009,#55010),.UNSPECIFIED.,.F.,.F.,(4,3,3,
3,3,3,3,4),(39.0086749840546,39.4611735465612,40.4477028852253,41.4342322238893,
42.4207615625533,43.4072909012173,44.3938202398814,45.2918602912342),
 .UNSPECIFIED.);
#4126=B_SPLINE_CURVE_WITH_KNOTS('',3,(#55011,#55012,#55013,#55014,#55015,
#55016,#55017,#55018,#55019,#55020,#55021,#55022,#55023,#55024,#55025,#55026,
#55027,#55028,#55029,#55030,#55031,#55032,#55033,#55034,#55035),
 .UNSPECIFIED.,.F.,.F.,(4,3,3,3,3,3,3,3,4),(-41.5517138474471,-41.4342322238893,
-40.4477028852253,-39.4611735465612,-38.4746442078972,-37.4881148692332,
-36.5015855305691,-35.5150561919051,-35.2685285402675),.UNSPECIFIED.);
#4127=B_SPLINE_CURVE_WITH_KNOTS('',3,(#55040,#55041,#55042,#55043,#55044,
#55045,#55046,#55047,#55048,#55049,#55050,#55051,#55052,#55053,#55054,#55055,
#55056,#55057,#55058,#55059,#55060,#55061),.UNSPECIFIED.,.F.,.F.,(4,3,3,
3,3,3,3,4),(32.725489676875,33.541997514577,34.5285268532411,35.5150561919051,
36.5015855305691,37.4881148692332,38.4746442078972,39.0086749840546),
 .UNSPECIFIED.);
#4128=B_SPLINE_CURVE_WITH_KNOTS('',3,(#55062,#55063,#55064,#55065,#55066,
#55067,#55068,#55069,#55070,#55071,#55072,#55073,#55074,#55075,#55076,#55077,
#55078,#55079,#55080,#55081,#55082,#55083),.UNSPECIFIED.,.F.,.F.,(4,3,3,
3,3,3,3,4),(-35.2685285402675,-34.5285268532411,-33.541997514577,-32.555468175913,
-31.568938837249,-30.5824094985849,-29.5958801599209,-28.9853432330879),
 .UNSPECIFIED.);
#4129=B_SPLINE_CURVE_WITH_KNOTS('',3,(#55088,#55089,#55090,#55091,#55092,
#55093,#55094,#55095,#55096,#55097,#55098,#55099,#55100,#55101,#55102,#55103,
#55104,#55105,#55106,#55107,#55108,#55109,#55110,#55111,#55112),
 .UNSPECIFIED.,.F.,.F.,(4,3,3,3,3,3,3,3,4),(26.4423043696954,26.6362921439288,
27.6228214825929,28.6093508212569,29.5958801599209,30.5824094985849,31.568938837249,
32.555468175913,32.725489676875),.UNSPECIFIED.);
#4130=B_SPLINE_CURVE_WITH_KNOTS('',3,(#55113,#55114,#55115,#55116,#55117,
#55118,#55119,#55120,#55121,#55122,#55123,#55124,#55125,#55126,#55127,#55128,
#55129,#55130,#55131,#55132,#55133,#55134),.UNSPECIFIED.,.F.,.F.,(4,3,3,
3,3,3,3,4),(-28.9853432330879,-28.6093508212569,-27.6228214825929,-26.6362921439288,
-25.6497628052648,-24.6632334666008,-23.6767041279367,-22.7021579259084),
 .UNSPECIFIED.);
#4131=B_SPLINE_CURVE_WITH_KNOTS('',3,(#55139,#55140,#55141,#55142,#55143,
#55144,#55145,#55146,#55147,#55148,#55149,#55150,#55151,#55152,#55153,#55154,
#55155,#55156,#55157,#55158,#55159,#55160),.UNSPECIFIED.,.F.,.F.,(4,3,3,
3,3,3,3,4),(20.1591190625158,20.7171161119446,21.7036454506087,22.6901747892727,
23.6767041279367,24.6632334666008,25.6497628052648,26.4423043696954),
 .UNSPECIFIED.);
#4132=B_SPLINE_CURVE_WITH_KNOTS('',3,(#55161,#55162,#55163,#55164,#55165,
#55166,#55167,#55168,#55169,#55170,#55171,#55172,#55173,#55174,#55175,#55176,
#55177,#55178,#55179,#55180,#55181,#55182,#55183,#55184,#55185),
 .UNSPECIFIED.,.F.,.F.,(4,3,3,3,3,3,3,3,4),(-22.7021579259084,-22.6901747892727,
-21.7036454506087,-20.7171161119446,-19.7305867732806,-18.7440574346166,
-17.7575280959525,-16.7709987572885,-16.4189726187288),.UNSPECIFIED.);
#4133=B_SPLINE_CURVE_WITH_KNOTS('',3,(#55190,#55191,#55192,#55193,#55194,
#55195,#55196,#55197,#55198,#55199,#55200,#55201,#55202,#55203,#55204,#55205,
#55206,#55207,#55208,#55209,#55210,#55211),.UNSPECIFIED.,.F.,.F.,(4,3,3,
3,3,3,3,4),(13.8759337553362,14.7979400799605,15.7844694186245,16.7709987572885,
17.7575280959526,18.7440574346166,19.7305867732806,20.1591190625158),
 .UNSPECIFIED.);
#4134=B_SPLINE_CURVE_WITH_KNOTS('',3,(#55212,#55213,#55214,#55215,#55216,
#55217,#55218,#55219,#55220,#55221,#55222,#55223,#55224,#55225,#55226,#55227,
#55228,#55229,#55230,#55231,#55232,#55233),.UNSPECIFIED.,.F.,.F.,(4,3,3,
3,3,3,3,4),(-16.4189726187288,-15.7844694186245,-14.7979400799605,-13.8114107412964,
-12.8248814026324,-11.8383520639684,-10.8518227253043,-10.1357873115492),
 .UNSPECIFIED.);
#4135=B_SPLINE_CURVE_WITH_KNOTS('',3,(#55239,#55240,#55241,#55242,#55243,
#55244,#55245,#55246,#55247,#55248,#55249,#55250,#55251),.UNSPECIFIED.,
 .F.,.F.,(4,3,3,3,4),(-3.85260200436961,-2.95958801599209,-1.97305867732806,
-0.986529338664032,0.),.UNSPECIFIED.);
#4136=B_SPLINE_CURVE_WITH_KNOTS('',3,(#55254,#55255,#55256,#55257,#55258,
#55259,#55260,#55261,#55262,#55263,#55264,#55265,#55266,#55267,#55268,#55269,
#55270,#55271,#55272),.UNSPECIFIED.,.F.,.F.,(4,3,3,3,3,3,4),(2.02057249175701,
2.9595880159921,3.94611735465613,4.93264669332016,5.91917603198419,6.90570537064822,
7.59274844815664),.UNSPECIFIED.);
#4137=B_SPLINE_CURVE_WITH_KNOTS('',3,(#55278,#55279,#55280,#55281,#55282,
#55283,#55284,#55285),.UNSPECIFIED.,.F.,.F.,(4,1,1,1,1,4),(59.6902604182061,
60.1952988581168,61.1818281967809,62.1683575354449,63.1548868741089,64.141416212773),
 .UNSPECIFIED.);
#4138=B_SPLINE_CURVE_WITH_KNOTS('',3,(#55288,#55289,#55290,#55291,#55292,
#55293,#55294,#55295,#55296),.UNSPECIFIED.,.F.,.F.,(4,1,1,1,1,1,4),(59.6902604182061,
59.7787497055173,60.7652790441813,61.7518083828453,62.7383377215094,63.7248670601734,
64.6638825844085),.UNSPECIFIED.);
#4139=B_SPLINE_CURVE_WITH_KNOTS('',3,(#55301,#55302,#55303,#55304,#55305,
#55306,#55307,#55308,#55309,#55310),.UNSPECIFIED.,.F.,.F.,(4,1,1,1,1,1,
1,4),(53.4070751110265,54.2761228261327,55.2626521647967,56.2491815034607,
57.2357108421247,58.2222401807888,59.2087695194528,59.6902604182061),
 .UNSPECIFIED.);
#4140=B_SPLINE_CURVE_WITH_KNOTS('',3,(#55311,#55312,#55313,#55314,#55315,
#55316,#55317,#55318,#55319,#55320),.UNSPECIFIED.,.F.,.F.,(4,1,1,1,1,1,
1,4),(53.4070751110265,53.8595736735331,54.8461030121971,55.8326323508611,
56.8191616895252,57.8056910281892,58.7922203668532,59.6902604182061),
 .UNSPECIFIED.);
#4141=B_SPLINE_CURVE_WITH_KNOTS('',3,(#55325,#55326,#55327,#55328,#55329,
#55330,#55331,#55332,#55333,#55334,#55335),.UNSPECIFIED.,.F.,.F.,(4,1,1,
1,1,1,1,1,4),(47.1238898038469,47.3704174554844,48.3569467941485,49.3434761328125,
50.3300054714765,51.3165348101406,52.3030641488046,53.2895934874686,53.4070751110265),
 .UNSPECIFIED.);
#4142=B_SPLINE_CURVE_WITH_KNOTS('',3,(#55336,#55337,#55338,#55339,#55340,
#55341,#55342,#55343,#55344,#55345),.UNSPECIFIED.,.F.,.F.,(4,1,1,1,1,1,
1,4),(47.1238898038469,47.9403976415489,48.9269269802129,49.913456318877,
50.899985657541,51.886514996205,52.873044334869,53.4070751110265),
 .UNSPECIFIED.);
#4143=B_SPLINE_CURVE_WITH_KNOTS('',3,(#55350,#55351,#55352,#55353,#55354,
#55355,#55356,#55357,#55358,#55359),.UNSPECIFIED.,.F.,.F.,(4,1,1,1,1,1,
1,4),(40.8407044966673,41.4512414235003,42.4377707621643,43.4243001008283,
44.4108294394924,45.3973587781564,46.3838881168204,47.1238898038469),
 .UNSPECIFIED.);
#4144=B_SPLINE_CURVE_WITH_KNOTS('',3,(#55360,#55361,#55362,#55363,#55364,
#55365,#55366,#55367,#55368,#55369,#55370),.UNSPECIFIED.,.F.,.F.,(4,1,1,
1,1,1,1,1,4),(40.8407044966673,41.0346922709007,42.0212216095647,43.0077509482287,
43.9942802868928,44.9808096255568,45.9673389642208,46.9538683028849,47.1238898038469),
 .UNSPECIFIED.);
#4145=B_SPLINE_CURVE_WITH_KNOTS('',3,(#55375,#55376,#55377,#55378,#55379,
#55380,#55381,#55382,#55383,#55384),.UNSPECIFIED.,.F.,.F.,(4,1,1,1,1,1,
1,4),(34.5575191894877,35.5320653915161,36.5185947301801,37.5051240688441,
38.4916534075082,39.4781827461722,40.4647120848362,40.8407044966673),
 .UNSPECIFIED.);
#4146=B_SPLINE_CURVE_WITH_KNOTS('',3,(#55385,#55386,#55387,#55388,#55389,
#55390,#55391,#55392,#55393,#55394),.UNSPECIFIED.,.F.,.F.,(4,1,1,1,1,1,
1,4),(34.5575191894877,35.1155162389165,36.1020455775805,37.0885749162446,
38.0751042549086,39.0616335935726,40.0481629322367,40.8407044966673),
 .UNSPECIFIED.);
#4147=B_SPLINE_CURVE_WITH_KNOTS('',3,(#55399,#55400,#55401,#55402,#55403,
#55404,#55405,#55406,#55407,#55408,#55409),.UNSPECIFIED.,.F.,.F.,(4,1,1,
1,1,1,1,1,4),(28.2743338823081,28.6263600208679,29.6128893595319,30.5994186981959,
31.58594803686,32.572477375524,33.559006714188,34.5455360528521,34.5575191894877),
 .UNSPECIFIED.);
#4148=B_SPLINE_CURVE_WITH_KNOTS('',3,(#55410,#55411,#55412,#55413,#55414,
#55415,#55416,#55417,#55418,#55419),.UNSPECIFIED.,.F.,.F.,(4,1,1,1,1,1,
1,4),(28.2743338823081,29.1963402069323,30.1828695455963,31.1693988842604,
32.1559282229244,33.1424575615884,34.1289869002525,34.5575191894877),
 .UNSPECIFIED.);
#4149=B_SPLINE_CURVE_WITH_KNOTS('',3,(#55424,#55425,#55426,#55427,#55428,
#55429,#55430,#55431,#55432,#55433),.UNSPECIFIED.,.F.,.F.,(4,1,1,1,1,1,
1,4),(21.9911485751285,22.7071839888837,23.6937133275477,24.6802426662117,
25.6667720048758,26.6533013435398,27.6398306822038,28.2743338823081),
 .UNSPECIFIED.);
#4150=B_SPLINE_CURVE_WITH_KNOTS('',3,(#55434,#55435,#55436,#55437,#55438,
#55439,#55440,#55441,#55442,#55443,#55444),.UNSPECIFIED.,.F.,.F.,(4,1,1,
1,1,1,1,1,4),(21.9911485751285,22.2906348362841,23.2771641749481,24.2636935136122,
25.2502228522762,26.2367521909402,27.2232815296043,28.2098108682683,28.2743338823081),
 .UNSPECIFIED.);
#4151=B_SPLINE_CURVE_WITH_KNOTS('',3,(#55450,#55451,#55452,#55453,#55454),
 .UNSPECIFIED.,.F.,.F.,(4,1,4),(14.3984001269719,15.3849294656359,15.7079632679489),
 .UNSPECIFIED.);
#4152=B_SPLINE_CURVE_WITH_KNOTS('',3,(#55457,#55458,#55459,#55460,#55461),
 .UNSPECIFIED.,.F.,.F.,(4,1,4),(13.8759337553363,14.8149492795714,15.7079632679489),
 .UNSPECIFIED.);
#4153=B_SPLINE_CURVE_WITH_KNOTS('',3,(#55467,#55468,#55469,#55470),
 .UNSPECIFIED.,.F.,.F.,(4,4),(51.5750455984138,52.2860549491936),
 .UNSPECIFIED.);
#4154=B_SPLINE_CURVE_WITH_KNOTS('',3,(#55482,#55483,#55484,#55485,#55486,
#55487,#55488,#55489,#55490,#55491),.UNSPECIFIED.,.F.,.F.,(4,3,3,4),(-50.2654824574366,
-49.3264669332015,-48.3399375945375,-47.8348991546267),.UNSPECIFIED.);
#4155=B_SPLINE_CURVE_WITH_KNOTS('',3,(#55496,#55497,#55498,#55499,#55500,
#55501,#55502,#55503,#55504,#55505,#55506,#55507,#55508,#55509,#55510,#55511,
#55512,#55513,#55514,#55515,#55516,#55517,#55518,#55519,#55520),
 .UNSPECIFIED.,.F.,.F.,(4,3,3,3,3,3,3,3,4),(45.2918602912342,45.3803495785454,
46.3668789172094,47.3534082558735,48.3399375945375,49.3264669332015,50.3129962718656,
51.2995256105296,51.5750455984138),.UNSPECIFIED.);
#4156=B_SPLINE_CURVE_WITH_KNOTS('',3,(#55521,#55522,#55523,#55524,#55525,
#55526,#55527,#55528,#55529,#55530,#55531,#55532,#55533,#55534,#55535,#55536,
#55537,#55538,#55539,#55540,#55541,#55542),.UNSPECIFIED.,.F.,.F.,(4,3,3,
3,3,3,3,4),(-47.8348991546267,-47.3534082558735,-46.3668789172094,-45.3803495785454,
-44.3938202398814,-43.4072909012173,-42.4207615625533,-41.5517138474471),
 .UNSPECIFIED.);
#4157=B_SPLINE_CURVE_WITH_KNOTS('',3,(#55547,#55548,#55549,#55550,#55551,
#55552,#55553,#55554,#55555,#55556,#55557,#55558,#55559,#55560,#55561,#55562,
#55563,#55564,#55565,#55566,#55567,#55568),.UNSPECIFIED.,.F.,.F.,(4,3,3,
3,3,3,3,4),(39.0086749840546,39.4611735465612,40.4477028852253,41.4342322238893,
42.4207615625533,43.4072909012173,44.3938202398814,45.2918602912342),
 .UNSPECIFIED.);
#4158=B_SPLINE_CURVE_WITH_KNOTS('',3,(#55569,#55570,#55571,#55572,#55573,
#55574,#55575,#55576,#55577,#55578,#55579,#55580,#55581,#55582,#55583,#55584,
#55585,#55586,#55587,#55588,#55589,#55590,#55591,#55592,#55593),
 .UNSPECIFIED.,.F.,.F.,(4,3,3,3,3,3,3,3,4),(-41.5517138474471,-41.4342322238893,
-40.4477028852252,-39.4611735465612,-38.4746442078972,-37.4881148692332,
-36.5015855305691,-35.5150561919051,-35.2685285402675),.UNSPECIFIED.);
#4159=B_SPLINE_CURVE_WITH_KNOTS('',3,(#55598,#55599,#55600,#55601,#55602,
#55603,#55604,#55605,#55606,#55607,#55608,#55609,#55610,#55611,#55612,#55613,
#55614,#55615,#55616,#55617,#55618,#55619),.UNSPECIFIED.,.F.,.F.,(4,3,3,
3,3,3,3,4),(32.725489676875,33.541997514577,34.5285268532411,35.5150561919051,
36.5015855305691,37.4881148692332,38.4746442078972,39.0086749840546),
 .UNSPECIFIED.);
#4160=B_SPLINE_CURVE_WITH_KNOTS('',3,(#55620,#55621,#55622,#55623,#55624,
#55625,#55626,#55627,#55628,#55629,#55630,#55631,#55632,#55633,#55634,#55635,
#55636,#55637,#55638,#55639,#55640,#55641),.UNSPECIFIED.,.F.,.F.,(4,3,3,
3,3,3,3,4),(-35.2685285402675,-34.5285268532411,-33.541997514577,-32.555468175913,
-31.568938837249,-30.5824094985849,-29.5958801599209,-28.9853432330879),
 .UNSPECIFIED.);
#4161=B_SPLINE_CURVE_WITH_KNOTS('',3,(#55646,#55647,#55648,#55649,#55650,
#55651,#55652,#55653,#55654,#55655,#55656,#55657,#55658,#55659,#55660,#55661,
#55662,#55663,#55664,#55665,#55666,#55667,#55668,#55669,#55670),
 .UNSPECIFIED.,.F.,.F.,(4,3,3,3,3,3,3,3,4),(26.4423043696954,26.6362921439288,
27.6228214825929,28.6093508212569,29.5958801599209,30.582409498585,31.568938837249,
32.555468175913,32.725489676875),.UNSPECIFIED.);
#4162=B_SPLINE_CURVE_WITH_KNOTS('',3,(#55671,#55672,#55673,#55674,#55675,
#55676,#55677,#55678,#55679,#55680,#55681,#55682,#55683,#55684,#55685,#55686,
#55687,#55688,#55689,#55690,#55691,#55692),.UNSPECIFIED.,.F.,.F.,(4,3,3,
3,3,3,3,4),(-28.9853432330879,-28.6093508212569,-27.6228214825929,-26.6362921439288,
-25.6497628052648,-24.6632334666008,-23.6767041279367,-22.7021579259083),
 .UNSPECIFIED.);
#4163=B_SPLINE_CURVE_WITH_KNOTS('',3,(#55697,#55698,#55699,#55700,#55701,
#55702,#55703,#55704,#55705,#55706,#55707,#55708,#55709,#55710,#55711,#55712,
#55713,#55714,#55715,#55716,#55717,#55718),.UNSPECIFIED.,.F.,.F.,(4,3,3,
3,3,3,3,4),(20.1591190625158,20.7171161119446,21.7036454506087,22.6901747892727,
23.6767041279367,24.6632334666008,25.6497628052648,26.4423043696954),
 .UNSPECIFIED.);
#4164=B_SPLINE_CURVE_WITH_KNOTS('',3,(#55719,#55720,#55721,#55722,#55723,
#55724,#55725,#55726,#55727,#55728,#55729,#55730,#55731,#55732,#55733,#55734,
#55735,#55736,#55737,#55738,#55739,#55740,#55741,#55742,#55743),
 .UNSPECIFIED.,.F.,.F.,(4,3,3,3,3,3,3,3,4),(-22.7021579259083,-22.6901747892727,
-21.7036454506087,-20.7171161119446,-19.7305867732806,-18.7440574346166,
-17.7575280959526,-16.7709987572885,-16.4189726187288),.UNSPECIFIED.);
#4165=B_SPLINE_CURVE_WITH_KNOTS('',3,(#55748,#55749,#55750,#55751,#55752,
#55753,#55754,#55755,#55756,#55757,#55758,#55759,#55760,#55761,#55762,#55763,
#55764,#55765,#55766,#55767,#55768,#55769),.UNSPECIFIED.,.F.,.F.,(4,3,3,
3,3,3,3,4),(13.8759337553362,14.7979400799605,15.7844694186245,16.7709987572885,
17.7575280959525,18.7440574346166,19.7305867732806,20.1591190625158),
 .UNSPECIFIED.);
#4166=B_SPLINE_CURVE_WITH_KNOTS('',3,(#55770,#55771,#55772,#55773,#55774,
#55775,#55776,#55777,#55778,#55779,#55780,#55781,#55782,#55783,#55784,#55785,
#55786,#55787,#55788,#55789,#55790,#55791),.UNSPECIFIED.,.F.,.F.,(4,3,3,
3,3,3,3,4),(-16.4189726187288,-15.7844694186245,-14.7979400799605,-13.8114107412964,
-12.8248814026324,-11.8383520639684,-10.8518227253043,-10.1357873115492),
 .UNSPECIFIED.);
#4167=B_SPLINE_CURVE_WITH_KNOTS('',3,(#55797,#55798,#55799,#55800,#55801,
#55802,#55803,#55804,#55805,#55806,#55807,#55808,#55809),.UNSPECIFIED.,
 .F.,.F.,(4,3,3,3,4),(-3.85260200436958,-2.95958801599209,-1.97305867732806,
-0.986529338664032,0.),.UNSPECIFIED.);
#4168=B_SPLINE_CURVE_WITH_KNOTS('',3,(#55812,#55813,#55814,#55815,#55816,
#55817,#55818,#55819,#55820,#55821,#55822,#55823,#55824,#55825,#55826,#55827,
#55828,#55829,#55830),.UNSPECIFIED.,.F.,.F.,(4,3,3,3,3,3,4),(2.02057249175696,
2.95958801599209,3.94611735465612,4.93264669332015,5.91917603198418,6.90570537064821,
7.59274844815664),.UNSPECIFIED.);
#4169=B_SPLINE_CURVE_WITH_KNOTS('',3,(#55836,#55837,#55838,#55839,#55840,
#55841,#55842,#55843),.UNSPECIFIED.,.F.,.F.,(4,1,1,1,1,4),(59.6902604182061,
60.1952988581168,61.1818281967809,62.1683575354449,63.1548868741089,64.141416212773),
 .UNSPECIFIED.);
#4170=B_SPLINE_CURVE_WITH_KNOTS('',3,(#55846,#55847,#55848,#55849,#55850,
#55851,#55852,#55853,#55854),.UNSPECIFIED.,.F.,.F.,(4,1,1,1,1,1,4),(59.6902604182061,
59.7787497055173,60.7652790441813,61.7518083828453,62.7383377215094,63.7248670601734,
64.6638825844085),.UNSPECIFIED.);
#4171=B_SPLINE_CURVE_WITH_KNOTS('',3,(#55859,#55860,#55861,#55862,#55863,
#55864,#55865,#55866,#55867,#55868),.UNSPECIFIED.,.F.,.F.,(4,1,1,1,1,1,
1,4),(53.4070751110265,54.2761228261327,55.2626521647967,56.2491815034607,
57.2357108421248,58.2222401807888,59.2087695194528,59.6902604182061),
 .UNSPECIFIED.);
#4172=B_SPLINE_CURVE_WITH_KNOTS('',3,(#55869,#55870,#55871,#55872,#55873,
#55874,#55875,#55876,#55877,#55878),.UNSPECIFIED.,.F.,.F.,(4,1,1,1,1,1,
1,4),(53.4070751110265,53.8595736735331,54.8461030121971,55.8326323508611,
56.8191616895252,57.8056910281892,58.7922203668532,59.6902604182061),
 .UNSPECIFIED.);
#4173=B_SPLINE_CURVE_WITH_KNOTS('',3,(#55883,#55884,#55885,#55886,#55887,
#55888,#55889,#55890,#55891,#55892,#55893),.UNSPECIFIED.,.F.,.F.,(4,1,1,
1,1,1,1,1,4),(47.1238898038469,47.3704174554844,48.3569467941485,49.3434761328125,
50.3300054714765,51.3165348101406,52.3030641488046,53.2895934874686,53.4070751110265),
 .UNSPECIFIED.);
#4174=B_SPLINE_CURVE_WITH_KNOTS('',3,(#55894,#55895,#55896,#55897,#55898,
#55899,#55900,#55901,#55902,#55903),.UNSPECIFIED.,.F.,.F.,(4,1,1,1,1,1,
1,4),(47.1238898038469,47.9403976415489,48.9269269802129,49.913456318877,
50.899985657541,51.886514996205,52.873044334869,53.4070751110265),
 .UNSPECIFIED.);
#4175=B_SPLINE_CURVE_WITH_KNOTS('',3,(#55908,#55909,#55910,#55911,#55912,
#55913,#55914,#55915,#55916,#55917),.UNSPECIFIED.,.F.,.F.,(4,1,1,1,1,1,
1,4),(40.8407044966673,41.4512414235003,42.4377707621643,43.4243001008283,
44.4108294394924,45.3973587781564,46.3838881168204,47.1238898038469),
 .UNSPECIFIED.);
#4176=B_SPLINE_CURVE_WITH_KNOTS('',3,(#55918,#55919,#55920,#55921,#55922,
#55923,#55924,#55925,#55926,#55927,#55928),.UNSPECIFIED.,.F.,.F.,(4,1,1,
1,1,1,1,1,4),(40.8407044966673,41.0346922709007,42.0212216095647,43.0077509482287,
43.9942802868928,44.9808096255568,45.9673389642208,46.9538683028849,47.1238898038469),
 .UNSPECIFIED.);
#4177=B_SPLINE_CURVE_WITH_KNOTS('',3,(#55933,#55934,#55935,#55936,#55937,
#55938,#55939,#55940,#55941,#55942),.UNSPECIFIED.,.F.,.F.,(4,1,1,1,1,1,
1,4),(34.5575191894877,35.5320653915161,36.5185947301801,37.5051240688441,
38.4916534075082,39.4781827461722,40.4647120848362,40.8407044966673),
 .UNSPECIFIED.);
#4178=B_SPLINE_CURVE_WITH_KNOTS('',3,(#55943,#55944,#55945,#55946,#55947,
#55948,#55949,#55950,#55951,#55952),.UNSPECIFIED.,.F.,.F.,(4,1,1,1,1,1,
1,4),(34.5575191894877,35.1155162389165,36.1020455775805,37.0885749162446,
38.0751042549086,39.0616335935726,40.0481629322367,40.8407044966673),
 .UNSPECIFIED.);
#4179=B_SPLINE_CURVE_WITH_KNOTS('',3,(#55957,#55958,#55959,#55960,#55961,
#55962,#55963,#55964,#55965,#55966,#55967),.UNSPECIFIED.,.F.,.F.,(4,1,1,
1,1,1,1,1,4),(28.2743338823081,28.6263600208679,29.6128893595319,30.5994186981959,
31.58594803686,32.572477375524,33.559006714188,34.5455360528521,34.5575191894877),
 .UNSPECIFIED.);
#4180=B_SPLINE_CURVE_WITH_KNOTS('',3,(#55968,#55969,#55970,#55971,#55972,
#55973,#55974,#55975,#55976,#55977),.UNSPECIFIED.,.F.,.F.,(4,1,1,1,1,1,
1,4),(28.2743338823081,29.1963402069323,30.1828695455963,31.1693988842604,
32.1559282229244,33.1424575615884,34.1289869002525,34.5575191894877),
 .UNSPECIFIED.);
#4181=B_SPLINE_CURVE_WITH_KNOTS('',3,(#55982,#55983,#55984,#55985,#55986,
#55987,#55988,#55989,#55990,#55991),.UNSPECIFIED.,.F.,.F.,(4,1,1,1,1,1,
1,4),(21.9911485751285,22.7071839888837,23.6937133275477,24.6802426662118,
25.6667720048758,26.6533013435398,27.6398306822038,28.2743338823081),
 .UNSPECIFIED.);
#4182=B_SPLINE_CURVE_WITH_KNOTS('',3,(#55992,#55993,#55994,#55995,#55996,
#55997,#55998,#55999,#56000,#56001,#56002),.UNSPECIFIED.,.F.,.F.,(4,1,1,
1,1,1,1,1,4),(21.9911485751285,22.2906348362841,23.2771641749481,24.2636935136122,
25.2502228522762,26.2367521909402,27.2232815296043,28.2098108682683,28.2743338823081),
 .UNSPECIFIED.);
#4183=B_SPLINE_CURVE_WITH_KNOTS('',3,(#56008,#56009,#56010,#56011,#56012),
 .UNSPECIFIED.,.F.,.F.,(4,1,4),(14.3984001269719,15.3849294656359,15.7079632679489),
 .UNSPECIFIED.);
#4184=B_SPLINE_CURVE_WITH_KNOTS('',3,(#56015,#56016,#56017,#56018,#56019),
 .UNSPECIFIED.,.F.,.F.,(4,1,4),(13.8759337553363,14.8149492795714,15.7079632679489),
 .UNSPECIFIED.);
#4185=B_SPLINE_CURVE_WITH_KNOTS('',3,(#56025,#56026,#56027,#56028),
 .UNSPECIFIED.,.F.,.F.,(4,4),(51.5750455984138,52.2860549491936),
 .UNSPECIFIED.);
#4186=B_SPLINE_CURVE_WITH_KNOTS('',3,(#56040,#56041,#56042,#56043,#56044,
#56045,#56046,#56047,#56048,#56049),.UNSPECIFIED.,.F.,.F.,(4,3,3,4),(-50.2654824574367,
-49.3264669332015,-48.3399375945375,-47.8348991546267),.UNSPECIFIED.);
#4187=B_SPLINE_CURVE_WITH_KNOTS('',3,(#56054,#56055,#56056,#56057,#56058,
#56059,#56060,#56061,#56062,#56063,#56064,#56065,#56066,#56067,#56068,#56069,
#56070,#56071,#56072,#56073,#56074,#56075,#56076,#56077,#56078),
 .UNSPECIFIED.,.F.,.F.,(4,3,3,3,3,3,3,3,4),(45.2918602912342,45.3803495785454,
46.3668789172094,47.3534082558735,48.3399375945375,49.3264669332015,50.3129962718656,
51.2995256105296,51.5750455984138),.UNSPECIFIED.);
#4188=B_SPLINE_CURVE_WITH_KNOTS('',3,(#56079,#56080,#56081,#56082,#56083,
#56084,#56085,#56086,#56087,#56088,#56089,#56090,#56091,#56092,#56093,#56094,
#56095,#56096,#56097,#56098,#56099,#56100),.UNSPECIFIED.,.F.,.F.,(4,3,3,
3,3,3,3,4),(-47.8348991546267,-47.3534082558735,-46.3668789172094,-45.3803495785454,
-44.3938202398814,-43.4072909012173,-42.4207615625533,-41.5517138474471),
 .UNSPECIFIED.);
#4189=B_SPLINE_CURVE_WITH_KNOTS('',3,(#56105,#56106,#56107,#56108,#56109,
#56110,#56111,#56112,#56113,#56114,#56115,#56116,#56117,#56118,#56119,#56120,
#56121,#56122,#56123,#56124,#56125,#56126),.UNSPECIFIED.,.F.,.F.,(4,3,3,
3,3,3,3,4),(39.0086749840546,39.4611735465612,40.4477028852253,41.4342322238893,
42.4207615625533,43.4072909012173,44.3938202398814,45.2918602912342),
 .UNSPECIFIED.);
#4190=B_SPLINE_CURVE_WITH_KNOTS('',3,(#56127,#56128,#56129,#56130,#56131,
#56132,#56133,#56134,#56135,#56136,#56137,#56138,#56139,#56140,#56141,#56142,
#56143,#56144,#56145,#56146,#56147,#56148,#56149,#56150,#56151),
 .UNSPECIFIED.,.F.,.F.,(4,3,3,3,3,3,3,3,4),(-41.5517138474471,-41.4342322238893,
-40.4477028852252,-39.4611735465612,-38.4746442078972,-37.4881148692332,
-36.5015855305691,-35.5150561919051,-35.2685285402675),.UNSPECIFIED.);
#4191=B_SPLINE_CURVE_WITH_KNOTS('',3,(#56156,#56157,#56158,#56159,#56160,
#56161,#56162,#56163,#56164,#56165,#56166,#56167,#56168,#56169,#56170,#56171,
#56172,#56173,#56174,#56175,#56176,#56177),.UNSPECIFIED.,.F.,.F.,(4,3,3,
3,3,3,3,4),(32.725489676875,33.541997514577,34.5285268532411,35.5150561919051,
36.5015855305691,37.4881148692332,38.4746442078972,39.0086749840546),
 .UNSPECIFIED.);
#4192=B_SPLINE_CURVE_WITH_KNOTS('',3,(#56178,#56179,#56180,#56181,#56182,
#56183,#56184,#56185,#56186,#56187,#56188,#56189,#56190,#56191,#56192,#56193,
#56194,#56195,#56196,#56197,#56198,#56199),.UNSPECIFIED.,.F.,.F.,(4,3,3,
3,3,3,3,4),(-35.2685285402675,-34.5285268532411,-33.541997514577,-32.555468175913,
-31.568938837249,-30.5824094985849,-29.5958801599209,-28.9853432330879),
 .UNSPECIFIED.);
#4193=B_SPLINE_CURVE_WITH_KNOTS('',3,(#56204,#56205,#56206,#56207,#56208,
#56209,#56210,#56211,#56212,#56213,#56214,#56215,#56216,#56217,#56218,#56219,
#56220,#56221,#56222,#56223,#56224,#56225,#56226,#56227,#56228),
 .UNSPECIFIED.,.F.,.F.,(4,3,3,3,3,3,3,3,4),(26.4423043696954,26.6362921439288,
27.6228214825929,28.6093508212569,29.5958801599209,30.582409498585,31.568938837249,
32.555468175913,32.725489676875),.UNSPECIFIED.);
#4194=B_SPLINE_CURVE_WITH_KNOTS('',3,(#56229,#56230,#56231,#56232,#56233,
#56234,#56235,#56236,#56237,#56238,#56239,#56240,#56241,#56242,#56243,#56244,
#56245,#56246,#56247,#56248,#56249,#56250),.UNSPECIFIED.,.F.,.F.,(4,3,3,
3,3,3,3,4),(-28.9853432330879,-28.6093508212569,-27.6228214825929,-26.6362921439288,
-25.6497628052648,-24.6632334666008,-23.6767041279367,-22.7021579259083),
 .UNSPECIFIED.);
#4195=B_SPLINE_CURVE_WITH_KNOTS('',3,(#56255,#56256,#56257,#56258,#56259,
#56260,#56261,#56262,#56263,#56264,#56265,#56266,#56267,#56268,#56269,#56270,
#56271,#56272,#56273,#56274,#56275,#56276),.UNSPECIFIED.,.F.,.F.,(4,3,3,
3,3,3,3,4),(20.1591190625158,20.7171161119446,21.7036454506087,22.6901747892727,
23.6767041279367,24.6632334666008,25.6497628052648,26.4423043696954),
 .UNSPECIFIED.);
#4196=B_SPLINE_CURVE_WITH_KNOTS('',3,(#56277,#56278,#56279,#56280,#56281,
#56282,#56283,#56284,#56285,#56286,#56287,#56288,#56289,#56290,#56291,#56292,
#56293,#56294,#56295,#56296,#56297,#56298,#56299,#56300,#56301),
 .UNSPECIFIED.,.F.,.F.,(4,3,3,3,3,3,3,3,4),(-22.7021579259083,-22.6901747892727,
-21.7036454506087,-20.7171161119446,-19.7305867732806,-18.7440574346166,
-17.7575280959525,-16.7709987572885,-16.4189726187287),.UNSPECIFIED.);
#4197=B_SPLINE_CURVE_WITH_KNOTS('',3,(#56306,#56307,#56308,#56309,#56310,
#56311,#56312,#56313,#56314,#56315,#56316,#56317,#56318,#56319,#56320,#56321,
#56322,#56323,#56324,#56325,#56326,#56327),.UNSPECIFIED.,.F.,.F.,(4,3,3,
3,3,3,3,4),(13.8759337553362,14.7979400799605,15.7844694186245,16.7709987572885,
17.7575280959525,18.7440574346166,19.7305867732806,20.1591190625158),
 .UNSPECIFIED.);
#4198=B_SPLINE_CURVE_WITH_KNOTS('',3,(#56328,#56329,#56330,#56331,#56332,
#56333,#56334,#56335,#56336,#56337,#56338,#56339,#56340,#56341,#56342,#56343,
#56344,#56345,#56346,#56347,#56348,#56349),.UNSPECIFIED.,.F.,.F.,(4,3,3,
3,3,3,3,4),(-16.4189726187287,-15.7844694186245,-14.7979400799605,-13.8114107412964,
-12.8248814026324,-11.8383520639684,-10.8518227253043,-10.1357873115492),
 .UNSPECIFIED.);
#4199=B_SPLINE_CURVE_WITH_KNOTS('',3,(#56355,#56356,#56357,#56358,#56359,
#56360,#56361,#56362,#56363,#56364,#56365,#56366,#56367),.UNSPECIFIED.,
 .F.,.F.,(4,3,3,3,4),(-3.85260200436958,-2.95958801599209,-1.97305867732806,
-0.986529338664031,0.),.UNSPECIFIED.);
#4200=B_SPLINE_CURVE_WITH_KNOTS('',3,(#56370,#56371,#56372,#56373,#56374,
#56375,#56376,#56377,#56378,#56379,#56380,#56381,#56382,#56383,#56384,#56385,
#56386,#56387,#56388),.UNSPECIFIED.,.F.,.F.,(4,3,3,3,3,3,4),(2.02057249175696,
2.95958801599209,3.94611735465612,4.93264669332015,5.91917603198419,6.90570537064821,
7.59274844815664),.UNSPECIFIED.);
#4201=B_SPLINE_CURVE_WITH_KNOTS('',3,(#56394,#56395,#56396,#56397,#56398,
#56399,#56400,#56401),.UNSPECIFIED.,.F.,.F.,(4,1,1,1,1,4),(59.6902604182061,
60.1952988581168,61.1818281967809,62.1683575354449,63.1548868741089,64.141416212773),
 .UNSPECIFIED.);
#4202=B_SPLINE_CURVE_WITH_KNOTS('',3,(#56404,#56405,#56406,#56407,#56408,
#56409,#56410,#56411,#56412),.UNSPECIFIED.,.F.,.F.,(4,1,1,1,1,1,4),(59.6902604182061,
59.7787497055173,60.7652790441813,61.7518083828453,62.7383377215094,63.7248670601734,
64.6638825844085),.UNSPECIFIED.);
#4203=B_SPLINE_CURVE_WITH_KNOTS('',3,(#56417,#56418,#56419,#56420,#56421,
#56422,#56423,#56424,#56425,#56426),.UNSPECIFIED.,.F.,.F.,(4,1,1,1,1,1,
1,4),(53.4070751110265,54.2761228261327,55.2626521647967,56.2491815034607,
57.2357108421248,58.2222401807888,59.2087695194528,59.6902604182061),
 .UNSPECIFIED.);
#4204=B_SPLINE_CURVE_WITH_KNOTS('',3,(#56427,#56428,#56429,#56430,#56431,
#56432,#56433,#56434,#56435,#56436),.UNSPECIFIED.,.F.,.F.,(4,1,1,1,1,1,
1,4),(53.4070751110265,53.8595736735331,54.8461030121971,55.8326323508611,
56.8191616895252,57.8056910281892,58.7922203668532,59.6902604182061),
 .UNSPECIFIED.);
#4205=B_SPLINE_CURVE_WITH_KNOTS('',3,(#56441,#56442,#56443,#56444,#56445,
#56446,#56447,#56448,#56449,#56450,#56451),.UNSPECIFIED.,.F.,.F.,(4,1,1,
1,1,1,1,1,4),(47.1238898038469,47.3704174554844,48.3569467941485,49.3434761328125,
50.3300054714765,51.3165348101406,52.3030641488046,53.2895934874686,53.4070751110265),
 .UNSPECIFIED.);
#4206=B_SPLINE_CURVE_WITH_KNOTS('',3,(#56452,#56453,#56454,#56455,#56456,
#56457,#56458,#56459,#56460,#56461),.UNSPECIFIED.,.F.,.F.,(4,1,1,1,1,1,
1,4),(47.1238898038469,47.9403976415489,48.9269269802129,49.913456318877,
50.899985657541,51.886514996205,52.873044334869,53.4070751110265),
 .UNSPECIFIED.);
#4207=B_SPLINE_CURVE_WITH_KNOTS('',3,(#56466,#56467,#56468,#56469,#56470,
#56471,#56472,#56473,#56474,#56475),.UNSPECIFIED.,.F.,.F.,(4,1,1,1,1,1,
1,4),(40.8407044966673,41.4512414235003,42.4377707621643,43.4243001008283,
44.4108294394924,45.3973587781564,46.3838881168204,47.1238898038469),
 .UNSPECIFIED.);
#4208=B_SPLINE_CURVE_WITH_KNOTS('',3,(#56476,#56477,#56478,#56479,#56480,
#56481,#56482,#56483,#56484,#56485,#56486),.UNSPECIFIED.,.F.,.F.,(4,1,1,
1,1,1,1,1,4),(40.8407044966673,41.0346922709007,42.0212216095647,43.0077509482287,
43.9942802868928,44.9808096255568,45.9673389642208,46.9538683028849,47.1238898038469),
 .UNSPECIFIED.);
#4209=B_SPLINE_CURVE_WITH_KNOTS('',3,(#56491,#56492,#56493,#56494,#56495,
#56496,#56497,#56498,#56499,#56500),.UNSPECIFIED.,.F.,.F.,(4,1,1,1,1,1,
1,4),(34.5575191894877,35.5320653915161,36.5185947301801,37.5051240688441,
38.4916534075082,39.4781827461722,40.4647120848362,40.8407044966673),
 .UNSPECIFIED.);
#4210=B_SPLINE_CURVE_WITH_KNOTS('',3,(#56501,#56502,#56503,#56504,#56505,
#56506,#56507,#56508,#56509,#56510),.UNSPECIFIED.,.F.,.F.,(4,1,1,1,1,1,
1,4),(34.5575191894877,35.1155162389165,36.1020455775805,37.0885749162446,
38.0751042549086,39.0616335935726,40.0481629322367,40.8407044966673),
 .UNSPECIFIED.);
#4211=B_SPLINE_CURVE_WITH_KNOTS('',3,(#56515,#56516,#56517,#56518,#56519,
#56520,#56521,#56522,#56523,#56524,#56525),.UNSPECIFIED.,.F.,.F.,(4,1,1,
1,1,1,1,1,4),(28.2743338823081,28.6263600208679,29.6128893595319,30.5994186981959,
31.58594803686,32.572477375524,33.559006714188,34.5455360528521,34.5575191894877),
 .UNSPECIFIED.);
#4212=B_SPLINE_CURVE_WITH_KNOTS('',3,(#56526,#56527,#56528,#56529,#56530,
#56531,#56532,#56533,#56534,#56535),.UNSPECIFIED.,.F.,.F.,(4,1,1,1,1,1,
1,4),(28.2743338823081,29.1963402069323,30.1828695455963,31.1693988842604,
32.1559282229244,33.1424575615884,34.1289869002525,34.5575191894877),
 .UNSPECIFIED.);
#4213=B_SPLINE_CURVE_WITH_KNOTS('',3,(#56540,#56541,#56542,#56543,#56544,
#56545,#56546,#56547,#56548,#56549),.UNSPECIFIED.,.F.,.F.,(4,1,1,1,1,1,
1,4),(21.9911485751285,22.7071839888837,23.6937133275477,24.6802426662118,
25.6667720048758,26.6533013435398,27.6398306822038,28.2743338823081),
 .UNSPECIFIED.);
#4214=B_SPLINE_CURVE_WITH_KNOTS('',3,(#56550,#56551,#56552,#56553,#56554,
#56555,#56556,#56557,#56558,#56559,#56560),.UNSPECIFIED.,.F.,.F.,(4,1,1,
1,1,1,1,1,4),(21.9911485751285,22.2906348362841,23.2771641749481,24.2636935136122,
25.2502228522762,26.2367521909402,27.2232815296043,28.2098108682683,28.2743338823081),
 .UNSPECIFIED.);
#4215=B_SPLINE_CURVE_WITH_KNOTS('',3,(#56566,#56567,#56568,#56569,#56570),
 .UNSPECIFIED.,.F.,.F.,(4,1,4),(14.3984001269719,15.3849294656359,15.7079632679489),
 .UNSPECIFIED.);
#4216=B_SPLINE_CURVE_WITH_KNOTS('',3,(#56573,#56574,#56575,#56576,#56577),
 .UNSPECIFIED.,.F.,.F.,(4,1,4),(13.8759337553363,14.8149492795714,15.7079632679489),
 .UNSPECIFIED.);
#4217=B_SPLINE_CURVE_WITH_KNOTS('',3,(#56583,#56584,#56585,#56586),
 .UNSPECIFIED.,.F.,.F.,(4,4),(51.5750455984138,52.2860549491936),
 .UNSPECIFIED.);
#4218=B_SPLINE_CURVE_WITH_KNOTS('',3,(#56598,#56599,#56600,#56601,#56602,
#56603,#56604,#56605,#56606,#56607),.UNSPECIFIED.,.F.,.F.,(4,3,3,4),(-50.2654824574367,
-49.3264669332015,-48.3399375945375,-47.8348991546267),.UNSPECIFIED.);
#4219=B_SPLINE_CURVE_WITH_KNOTS('',3,(#56612,#56613,#56614,#56615,#56616,
#56617,#56618,#56619,#56620,#56621,#56622,#56623,#56624,#56625,#56626,#56627,
#56628,#56629,#56630,#56631,#56632,#56633,#56634,#56635,#56636),
 .UNSPECIFIED.,.F.,.F.,(4,3,3,3,3,3,3,3,4),(45.2918602912342,45.3803495785454,
46.3668789172094,47.3534082558735,48.3399375945375,49.3264669332015,50.3129962718656,
51.2995256105296,51.5750455984138),.UNSPECIFIED.);
#4220=B_SPLINE_CURVE_WITH_KNOTS('',3,(#56637,#56638,#56639,#56640,#56641,
#56642,#56643,#56644,#56645,#56646,#56647,#56648,#56649,#56650,#56651,#56652,
#56653,#56654,#56655,#56656,#56657,#56658),.UNSPECIFIED.,.F.,.F.,(4,3,3,
3,3,3,3,4),(-47.8348991546267,-47.3534082558735,-46.3668789172094,-45.3803495785454,
-44.3938202398814,-43.4072909012174,-42.4207615625533,-41.5517138474471),
 .UNSPECIFIED.);
#4221=B_SPLINE_CURVE_WITH_KNOTS('',3,(#56663,#56664,#56665,#56666,#56667,
#56668,#56669,#56670,#56671,#56672,#56673,#56674,#56675,#56676,#56677,#56678,
#56679,#56680,#56681,#56682,#56683,#56684),.UNSPECIFIED.,.F.,.F.,(4,3,3,
3,3,3,3,4),(39.0086749840546,39.4611735465612,40.4477028852253,41.4342322238893,
42.4207615625533,43.4072909012174,44.3938202398814,45.2918602912342),
 .UNSPECIFIED.);
#4222=B_SPLINE_CURVE_WITH_KNOTS('',3,(#56685,#56686,#56687,#56688,#56689,
#56690,#56691,#56692,#56693,#56694,#56695,#56696,#56697,#56698,#56699,#56700,
#56701,#56702,#56703,#56704,#56705,#56706,#56707,#56708,#56709),
 .UNSPECIFIED.,.F.,.F.,(4,3,3,3,3,3,3,3,4),(-41.5517138474471,-41.4342322238893,
-40.4477028852253,-39.4611735465612,-38.4746442078972,-37.4881148692332,
-36.5015855305691,-35.5150561919051,-35.2685285402676),.UNSPECIFIED.);
#4223=B_SPLINE_CURVE_WITH_KNOTS('',3,(#56714,#56715,#56716,#56717,#56718,
#56719,#56720,#56721,#56722,#56723,#56724,#56725,#56726,#56727,#56728,#56729,
#56730,#56731,#56732,#56733,#56734,#56735),.UNSPECIFIED.,.F.,.F.,(4,3,3,
3,3,3,3,4),(32.725489676875,33.541997514577,34.5285268532411,35.5150561919051,
36.5015855305691,37.4881148692332,38.4746442078972,39.0086749840546),
 .UNSPECIFIED.);
#4224=B_SPLINE_CURVE_WITH_KNOTS('',3,(#56736,#56737,#56738,#56739,#56740,
#56741,#56742,#56743,#56744,#56745,#56746,#56747,#56748,#56749,#56750,#56751,
#56752,#56753,#56754,#56755,#56756,#56757),.UNSPECIFIED.,.F.,.F.,(4,3,3,
3,3,3,3,4),(-35.2685285402676,-34.5285268532411,-33.541997514577,-32.555468175913,
-31.568938837249,-30.5824094985849,-29.5958801599209,-28.985343233088),
 .UNSPECIFIED.);
#4225=B_SPLINE_CURVE_WITH_KNOTS('',3,(#56762,#56763,#56764,#56765,#56766,
#56767,#56768,#56769,#56770,#56771,#56772,#56773,#56774,#56775,#56776,#56777,
#56778,#56779,#56780,#56781,#56782,#56783,#56784,#56785,#56786),
 .UNSPECIFIED.,.F.,.F.,(4,3,3,3,3,3,3,3,4),(26.4423043696954,26.6362921439288,
27.6228214825929,28.6093508212569,29.5958801599209,30.582409498585,31.568938837249,
32.555468175913,32.725489676875),.UNSPECIFIED.);
#4226=B_SPLINE_CURVE_WITH_KNOTS('',3,(#56787,#56788,#56789,#56790,#56791,
#56792,#56793,#56794,#56795,#56796,#56797,#56798,#56799,#56800,#56801,#56802,
#56803,#56804,#56805,#56806,#56807,#56808),.UNSPECIFIED.,.F.,.F.,(4,3,3,
3,3,3,3,4),(-28.985343233088,-28.6093508212569,-27.6228214825929,-26.6362921439288,
-25.6497628052648,-24.6632334666008,-23.6767041279367,-22.7021579259084),
 .UNSPECIFIED.);
#4227=B_SPLINE_CURVE_WITH_KNOTS('',3,(#56813,#56814,#56815,#56816,#56817,
#56818,#56819,#56820,#56821,#56822,#56823,#56824,#56825,#56826,#56827,#56828,
#56829,#56830,#56831,#56832,#56833,#56834),.UNSPECIFIED.,.F.,.F.,(4,3,3,
3,3,3,3,4),(20.1591190625159,20.7171161119446,21.7036454506087,22.6901747892727,
23.6767041279367,24.6632334666008,25.6497628052648,26.4423043696954),
 .UNSPECIFIED.);
#4228=B_SPLINE_CURVE_WITH_KNOTS('',3,(#56835,#56836,#56837,#56838,#56839,
#56840,#56841,#56842,#56843,#56844,#56845,#56846,#56847,#56848,#56849,#56850,
#56851,#56852,#56853,#56854,#56855,#56856,#56857,#56858,#56859),
 .UNSPECIFIED.,.F.,.F.,(4,3,3,3,3,3,3,3,4),(-22.7021579259084,-22.6901747892727,
-21.7036454506087,-20.7171161119446,-19.7305867732806,-18.7440574346166,
-17.7575280959526,-16.7709987572885,-16.4189726187288),.UNSPECIFIED.);
#4229=B_SPLINE_CURVE_WITH_KNOTS('',3,(#56864,#56865,#56866,#56867,#56868,
#56869,#56870,#56871,#56872,#56873,#56874,#56875,#56876,#56877,#56878,#56879,
#56880,#56881,#56882,#56883,#56884,#56885),.UNSPECIFIED.,.F.,.F.,(4,3,3,
3,3,3,3,4),(13.8759337553363,14.7979400799605,15.7844694186245,16.7709987572885,
17.7575280959526,18.7440574346166,19.7305867732806,20.1591190625159),
 .UNSPECIFIED.);
#4230=B_SPLINE_CURVE_WITH_KNOTS('',3,(#56886,#56887,#56888,#56889,#56890,
#56891,#56892,#56893,#56894,#56895,#56896,#56897,#56898,#56899,#56900,#56901,
#56902,#56903,#56904,#56905,#56906,#56907),.UNSPECIFIED.,.F.,.F.,(4,3,3,
3,3,3,3,4),(-16.4189726187288,-15.7844694186245,-14.7979400799605,-13.8114107412964,
-12.8248814026324,-11.8383520639684,-10.8518227253043,-10.1357873115492),
 .UNSPECIFIED.);
#4231=B_SPLINE_CURVE_WITH_KNOTS('',3,(#56913,#56914,#56915,#56916,#56917,
#56918,#56919,#56920,#56921,#56922,#56923,#56924,#56925),.UNSPECIFIED.,
 .F.,.F.,(4,3,3,3,4),(-3.85260200436962,-2.95958801599209,-1.97305867732806,
-0.986529338664032,0.),.UNSPECIFIED.);
#4232=B_SPLINE_CURVE_WITH_KNOTS('',3,(#56928,#56929,#56930,#56931,#56932,
#56933,#56934,#56935,#56936,#56937,#56938,#56939,#56940,#56941,#56942,#56943,
#56944,#56945,#56946),.UNSPECIFIED.,.F.,.F.,(4,3,3,3,3,3,4),(2.02057249175696,
2.95958801599209,3.94611735465612,4.93264669332015,5.91917603198418,6.90570537064821,
7.59274844815668),.UNSPECIFIED.);
#4233=B_SPLINE_CURVE_WITH_KNOTS('',3,(#56952,#56953,#56954,#56955,#56956,
#56957,#56958,#56959),.UNSPECIFIED.,.F.,.F.,(4,1,1,1,1,4),(59.6902604182061,
60.1952988581168,61.1818281967809,62.1683575354449,63.1548868741089,64.1414162127729),
 .UNSPECIFIED.);
#4234=B_SPLINE_CURVE_WITH_KNOTS('',3,(#56962,#56963,#56964,#56965,#56966,
#56967,#56968,#56969,#56970),.UNSPECIFIED.,.F.,.F.,(4,1,1,1,1,1,4),(59.6902604182061,
59.7787497055172,60.7652790441813,61.7518083828453,62.7383377215093,63.7248670601734,
64.6638825844085),.UNSPECIFIED.);
#4235=B_SPLINE_CURVE_WITH_KNOTS('',3,(#56975,#56976,#56977,#56978,#56979,
#56980,#56981,#56982,#56983,#56984),.UNSPECIFIED.,.F.,.F.,(4,1,1,1,1,1,
1,4),(53.4070751110265,54.2761228261326,55.2626521647967,56.2491815034607,
57.2357108421247,58.2222401807888,59.2087695194528,59.6902604182061),
 .UNSPECIFIED.);
#4236=B_SPLINE_CURVE_WITH_KNOTS('',3,(#56985,#56986,#56987,#56988,#56989,
#56990,#56991,#56992,#56993,#56994),.UNSPECIFIED.,.F.,.F.,(4,1,1,1,1,1,
1,4),(53.4070751110265,53.8595736735331,54.8461030121971,55.8326323508611,
56.8191616895252,57.8056910281892,58.7922203668532,59.6902604182061),
 .UNSPECIFIED.);
#4237=B_SPLINE_CURVE_WITH_KNOTS('',3,(#56999,#57000,#57001,#57002,#57003,
#57004,#57005,#57006,#57007,#57008,#57009),.UNSPECIFIED.,.F.,.F.,(4,1,1,
1,1,1,1,1,4),(47.1238898038469,47.3704174554844,48.3569467941485,49.3434761328125,
50.3300054714765,51.3165348101406,52.3030641488046,53.2895934874686,53.4070751110265),
 .UNSPECIFIED.);
#4238=B_SPLINE_CURVE_WITH_KNOTS('',3,(#57010,#57011,#57012,#57013,#57014,
#57015,#57016,#57017,#57018,#57019),.UNSPECIFIED.,.F.,.F.,(4,1,1,1,1,1,
1,4),(47.1238898038469,47.9403976415489,48.9269269802129,49.9134563188769,
50.899985657541,51.886514996205,52.873044334869,53.4070751110265),
 .UNSPECIFIED.);
#4239=B_SPLINE_CURVE_WITH_KNOTS('',3,(#57024,#57025,#57026,#57027,#57028,
#57029,#57030,#57031,#57032,#57033),.UNSPECIFIED.,.F.,.F.,(4,1,1,1,1,1,
1,4),(40.8407044966673,41.4512414235002,42.4377707621643,43.4243001008283,
44.4108294394923,45.3973587781564,46.3838881168204,47.1238898038469),
 .UNSPECIFIED.);
#4240=B_SPLINE_CURVE_WITH_KNOTS('',3,(#57034,#57035,#57036,#57037,#57038,
#57039,#57040,#57041,#57042,#57043,#57044),.UNSPECIFIED.,.F.,.F.,(4,1,1,
1,1,1,1,1,4),(40.8407044966673,41.0346922709007,42.0212216095647,43.0077509482287,
43.9942802868928,44.9808096255568,45.9673389642208,46.9538683028848,47.1238898038469),
 .UNSPECIFIED.);
#4241=B_SPLINE_CURVE_WITH_KNOTS('',3,(#57049,#57050,#57051,#57052,#57053,
#57054,#57055,#57056,#57057,#57058),.UNSPECIFIED.,.F.,.F.,(4,1,1,1,1,1,
1,4),(34.5575191894877,35.5320653915161,36.5185947301801,37.5051240688441,
38.4916534075082,39.4781827461722,40.4647120848362,40.8407044966673),
 .UNSPECIFIED.);
#4242=B_SPLINE_CURVE_WITH_KNOTS('',3,(#57059,#57060,#57061,#57062,#57063,
#57064,#57065,#57066,#57067,#57068),.UNSPECIFIED.,.F.,.F.,(4,1,1,1,1,1,
1,4),(34.5575191894877,35.1155162389165,36.1020455775805,37.0885749162445,
38.0751042549086,39.0616335935726,40.0481629322366,40.8407044966673),
 .UNSPECIFIED.);
#4243=B_SPLINE_CURVE_WITH_KNOTS('',3,(#57073,#57074,#57075,#57076,#57077,
#57078,#57079,#57080,#57081,#57082,#57083),.UNSPECIFIED.,.F.,.F.,(4,1,1,
1,1,1,1,1,4),(28.2743338823081,28.6263600208678,29.6128893595319,30.5994186981959,
31.5859480368599,32.572477375524,33.559006714188,34.545536052852,34.5575191894877),
 .UNSPECIFIED.);
#4244=B_SPLINE_CURVE_WITH_KNOTS('',3,(#57084,#57085,#57086,#57087,#57088,
#57089,#57090,#57091,#57092,#57093),.UNSPECIFIED.,.F.,.F.,(4,1,1,1,1,1,
1,4),(28.2743338823081,29.1963402069323,30.1828695455963,31.1693988842604,
32.1559282229244,33.1424575615884,34.1289869002524,34.5575191894877),
 .UNSPECIFIED.);
#4245=B_SPLINE_CURVE_WITH_KNOTS('',3,(#57098,#57099,#57100,#57101,#57102,
#57103,#57104,#57105,#57106,#57107),.UNSPECIFIED.,.F.,.F.,(4,1,1,1,1,1,
1,4),(21.9911485751285,22.7071839888837,23.6937133275477,24.6802426662117,
25.6667720048758,26.6533013435398,27.6398306822038,28.2743338823081),
 .UNSPECIFIED.);
#4246=B_SPLINE_CURVE_WITH_KNOTS('',3,(#57108,#57109,#57110,#57111,#57112,
#57113,#57114,#57115,#57116,#57117,#57118),.UNSPECIFIED.,.F.,.F.,(4,1,1,
1,1,1,1,1,4),(21.9911485751285,22.2906348362841,23.2771641749481,24.2636935136121,
25.2502228522762,26.2367521909402,27.2232815296042,28.2098108682683,28.2743338823081),
 .UNSPECIFIED.);
#4247=B_SPLINE_CURVE_WITH_KNOTS('',3,(#57124,#57125,#57126,#57127,#57128),
 .UNSPECIFIED.,.F.,.F.,(4,1,4),(14.3984001269718,15.3849294656359,15.7079632679489),
 .UNSPECIFIED.);
#4248=B_SPLINE_CURVE_WITH_KNOTS('',3,(#57131,#57132,#57133,#57134,#57135),
 .UNSPECIFIED.,.F.,.F.,(4,1,4),(13.8759337553363,14.8149492795714,15.7079632679489),
 .UNSPECIFIED.);
#4249=B_SPLINE_CURVE_WITH_KNOTS('',3,(#57141,#57142,#57143,#57144),
 .UNSPECIFIED.,.F.,.F.,(4,4),(51.5750455984138,52.2860549491936),
 .UNSPECIFIED.);
#4250=B_SPLINE_CURVE_WITH_KNOTS('',3,(#57156,#57157,#57158,#57159,#57160,
#57161,#57162,#57163,#57164,#57165),.UNSPECIFIED.,.F.,.F.,(4,3,3,4),(-50.2654824574366,
-49.3264669332015,-48.3399375945375,-47.8348991546267),.UNSPECIFIED.);
#4251=B_SPLINE_CURVE_WITH_KNOTS('',3,(#57170,#57171,#57172,#57173,#57174,
#57175,#57176,#57177,#57178,#57179,#57180,#57181,#57182,#57183,#57184,#57185,
#57186,#57187,#57188,#57189,#57190,#57191,#57192,#57193,#57194),
 .UNSPECIFIED.,.F.,.F.,(4,3,3,3,3,3,3,3,4),(45.2918602912342,45.3803495785454,
46.3668789172095,47.3534082558735,48.3399375945375,49.3264669332015,50.3129962718656,
51.2995256105296,51.5750455984138),.UNSPECIFIED.);
#4252=B_SPLINE_CURVE_WITH_KNOTS('',3,(#57195,#57196,#57197,#57198,#57199,
#57200,#57201,#57202,#57203,#57204,#57205,#57206,#57207,#57208,#57209,#57210,
#57211,#57212,#57213,#57214,#57215,#57216),.UNSPECIFIED.,.F.,.F.,(4,3,3,
3,3,3,3,4),(-47.8348991546267,-47.3534082558735,-46.3668789172094,-45.3803495785454,
-44.3938202398814,-43.4072909012173,-42.4207615625533,-41.5517138474471),
 .UNSPECIFIED.);
#4253=B_SPLINE_CURVE_WITH_KNOTS('',3,(#57221,#57222,#57223,#57224,#57225,
#57226,#57227,#57228,#57229,#57230,#57231,#57232,#57233,#57234,#57235,#57236,
#57237,#57238,#57239,#57240,#57241,#57242),.UNSPECIFIED.,.F.,.F.,(4,3,3,
3,3,3,3,4),(39.0086749840546,39.4611735465612,40.4477028852253,41.4342322238893,
42.4207615625533,43.4072909012174,44.3938202398814,45.2918602912342),
 .UNSPECIFIED.);
#4254=B_SPLINE_CURVE_WITH_KNOTS('',3,(#57243,#57244,#57245,#57246,#57247,
#57248,#57249,#57250,#57251,#57252,#57253,#57254,#57255,#57256,#57257,#57258,
#57259,#57260,#57261,#57262,#57263,#57264,#57265,#57266,#57267),
 .UNSPECIFIED.,.F.,.F.,(4,3,3,3,3,3,3,3,4),(-41.5517138474471,-41.4342322238893,
-40.4477028852252,-39.4611735465612,-38.4746442078972,-37.4881148692332,
-36.5015855305691,-35.5150561919051,-35.2685285402676),.UNSPECIFIED.);
#4255=B_SPLINE_CURVE_WITH_KNOTS('',3,(#57272,#57273,#57274,#57275,#57276,
#57277,#57278,#57279,#57280,#57281,#57282,#57283,#57284,#57285,#57286,#57287,
#57288,#57289,#57290,#57291,#57292,#57293),.UNSPECIFIED.,.F.,.F.,(4,3,3,
3,3,3,3,4),(32.725489676875,33.541997514577,34.5285268532411,35.5150561919051,
36.5015855305691,37.4881148692332,38.4746442078972,39.0086749840546),
 .UNSPECIFIED.);
#4256=B_SPLINE_CURVE_WITH_KNOTS('',3,(#57294,#57295,#57296,#57297,#57298,
#57299,#57300,#57301,#57302,#57303,#57304,#57305,#57306,#57307,#57308,#57309,
#57310,#57311,#57312,#57313,#57314,#57315),.UNSPECIFIED.,.F.,.F.,(4,3,3,
3,3,3,3,4),(-35.2685285402676,-34.5285268532411,-33.541997514577,-32.555468175913,
-31.568938837249,-30.5824094985849,-29.5958801599209,-28.985343233088),
 .UNSPECIFIED.);
#4257=B_SPLINE_CURVE_WITH_KNOTS('',3,(#57320,#57321,#57322,#57323,#57324,
#57325,#57326,#57327,#57328,#57329,#57330,#57331,#57332,#57333,#57334,#57335,
#57336,#57337,#57338,#57339,#57340,#57341,#57342,#57343,#57344),
 .UNSPECIFIED.,.F.,.F.,(4,3,3,3,3,3,3,3,4),(26.4423043696954,26.6362921439288,
27.6228214825929,28.6093508212569,29.5958801599209,30.582409498585,31.568938837249,
32.555468175913,32.725489676875),.UNSPECIFIED.);
#4258=B_SPLINE_CURVE_WITH_KNOTS('',3,(#57345,#57346,#57347,#57348,#57349,
#57350,#57351,#57352,#57353,#57354,#57355,#57356,#57357,#57358,#57359,#57360,
#57361,#57362,#57363,#57364,#57365,#57366),.UNSPECIFIED.,.F.,.F.,(4,3,3,
3,3,3,3,4),(-28.985343233088,-28.6093508212569,-27.6228214825929,-26.6362921439288,
-25.6497628052648,-24.6632334666008,-23.6767041279367,-22.7021579259084),
 .UNSPECIFIED.);
#4259=B_SPLINE_CURVE_WITH_KNOTS('',3,(#57371,#57372,#57373,#57374,#57375,
#57376,#57377,#57378,#57379,#57380,#57381,#57382,#57383,#57384,#57385,#57386,
#57387,#57388,#57389,#57390,#57391,#57392),.UNSPECIFIED.,.F.,.F.,(4,3,3,
3,3,3,3,4),(20.1591190625158,20.7171161119446,21.7036454506087,22.6901747892727,
23.6767041279367,24.6632334666008,25.6497628052648,26.4423043696954),
 .UNSPECIFIED.);
#4260=B_SPLINE_CURVE_WITH_KNOTS('',3,(#57393,#57394,#57395,#57396,#57397,
#57398,#57399,#57400,#57401,#57402,#57403,#57404,#57405,#57406,#57407,#57408,
#57409,#57410,#57411,#57412,#57413,#57414,#57415,#57416,#57417),
 .UNSPECIFIED.,.F.,.F.,(4,3,3,3,3,3,3,3,4),(-22.7021579259084,-22.6901747892727,
-21.7036454506087,-20.7171161119446,-19.7305867732806,-18.7440574346166,
-17.7575280959526,-16.7709987572885,-16.4189726187288),.UNSPECIFIED.);
#4261=B_SPLINE_CURVE_WITH_KNOTS('',3,(#57422,#57423,#57424,#57425,#57426,
#57427,#57428,#57429,#57430,#57431,#57432,#57433,#57434,#57435,#57436,#57437,
#57438,#57439,#57440,#57441,#57442,#57443),.UNSPECIFIED.,.F.,.F.,(4,3,3,
3,3,3,3,4),(13.8759337553363,14.7979400799605,15.7844694186245,16.7709987572885,
17.7575280959526,18.7440574346166,19.7305867732806,20.1591190625158),
 .UNSPECIFIED.);
#4262=B_SPLINE_CURVE_WITH_KNOTS('',3,(#57444,#57445,#57446,#57447,#57448,
#57449,#57450,#57451,#57452,#57453,#57454,#57455,#57456,#57457,#57458,#57459,
#57460,#57461,#57462,#57463,#57464,#57465),.UNSPECIFIED.,.F.,.F.,(4,3,3,
3,3,3,3,4),(-16.4189726187288,-15.7844694186245,-14.7979400799605,-13.8114107412964,
-12.8248814026324,-11.8383520639684,-10.8518227253043,-10.1357873115492),
 .UNSPECIFIED.);
#4263=B_SPLINE_CURVE_WITH_KNOTS('',3,(#57471,#57472,#57473,#57474,#57475,
#57476,#57477,#57478,#57479,#57480,#57481,#57482,#57483),.UNSPECIFIED.,
 .F.,.F.,(4,3,3,3,4),(-3.85260200436961,-2.95958801599209,-1.97305867732806,
-0.98652933866403,0.),.UNSPECIFIED.);
#4264=B_SPLINE_CURVE_WITH_KNOTS('',3,(#57486,#57487,#57488,#57489,#57490,
#57491,#57492,#57493,#57494,#57495,#57496,#57497,#57498,#57499,#57500,#57501,
#57502,#57503,#57504),.UNSPECIFIED.,.F.,.F.,(4,3,3,3,3,3,4),(2.020572491757,
2.95958801599209,3.94611735465612,4.93264669332015,5.91917603198419,6.90570537064822,
7.59274844815667),.UNSPECIFIED.);
#4265=B_SPLINE_CURVE_WITH_KNOTS('',3,(#57510,#57511,#57512,#57513,#57514,
#57515,#57516,#57517),.UNSPECIFIED.,.F.,.F.,(4,1,1,1,1,4),(59.6902604182061,
60.1952988581168,61.1818281967808,62.1683575354449,63.1548868741089,64.1414162127729),
 .UNSPECIFIED.);
#4266=B_SPLINE_CURVE_WITH_KNOTS('',3,(#57520,#57521,#57522,#57523,#57524,
#57525,#57526,#57527,#57528),.UNSPECIFIED.,.F.,.F.,(4,1,1,1,1,1,4),(59.6902604182061,
59.7787497055172,60.7652790441813,61.7518083828453,62.7383377215093,63.7248670601734,
64.6638825844085),.UNSPECIFIED.);
#4267=B_SPLINE_CURVE_WITH_KNOTS('',3,(#57533,#57534,#57535,#57536,#57537,
#57538,#57539,#57540,#57541,#57542),.UNSPECIFIED.,.F.,.F.,(4,1,1,1,1,1,
1,4),(53.4070751110265,54.2761228261326,55.2626521647967,56.2491815034607,
57.2357108421247,58.2222401807888,59.2087695194528,59.6902604182061),
 .UNSPECIFIED.);
#4268=B_SPLINE_CURVE_WITH_KNOTS('',3,(#57543,#57544,#57545,#57546,#57547,
#57548,#57549,#57550,#57551,#57552),.UNSPECIFIED.,.F.,.F.,(4,1,1,1,1,1,
1,4),(53.4070751110265,53.8595736735331,54.8461030121971,55.8326323508611,
56.8191616895252,57.8056910281892,58.7922203668532,59.6902604182061),
 .UNSPECIFIED.);
#4269=B_SPLINE_CURVE_WITH_KNOTS('',3,(#57557,#57558,#57559,#57560,#57561,
#57562,#57563,#57564,#57565,#57566,#57567),.UNSPECIFIED.,.F.,.F.,(4,1,1,
1,1,1,1,1,4),(47.1238898038469,47.3704174554844,48.3569467941485,49.3434761328125,
50.3300054714765,51.3165348101405,52.3030641488046,53.2895934874686,53.4070751110265),
 .UNSPECIFIED.);
#4270=B_SPLINE_CURVE_WITH_KNOTS('',3,(#57568,#57569,#57570,#57571,#57572,
#57573,#57574,#57575,#57576,#57577),.UNSPECIFIED.,.F.,.F.,(4,1,1,1,1,1,
1,4),(47.1238898038469,47.9403976415489,48.9269269802129,49.9134563188769,
50.899985657541,51.886514996205,52.873044334869,53.4070751110265),
 .UNSPECIFIED.);
#4271=B_SPLINE_CURVE_WITH_KNOTS('',3,(#57582,#57583,#57584,#57585,#57586,
#57587,#57588,#57589,#57590,#57591),.UNSPECIFIED.,.F.,.F.,(4,1,1,1,1,1,
1,4),(40.8407044966673,41.4512414235002,42.4377707621643,43.4243001008283,
44.4108294394923,45.3973587781564,46.3838881168204,47.1238898038469),
 .UNSPECIFIED.);
#4272=B_SPLINE_CURVE_WITH_KNOTS('',3,(#57592,#57593,#57594,#57595,#57596,
#57597,#57598,#57599,#57600,#57601,#57602),.UNSPECIFIED.,.F.,.F.,(4,1,1,
1,1,1,1,1,4),(40.8407044966673,41.0346922709007,42.0212216095647,43.0077509482287,
43.9942802868928,44.9808096255568,45.9673389642208,46.9538683028848,47.1238898038469),
 .UNSPECIFIED.);
#4273=B_SPLINE_CURVE_WITH_KNOTS('',3,(#57607,#57608,#57609,#57610,#57611,
#57612,#57613,#57614,#57615,#57616),.UNSPECIFIED.,.F.,.F.,(4,1,1,1,1,1,
1,4),(34.5575191894877,35.5320653915161,36.5185947301801,37.5051240688441,
38.4916534075081,39.4781827461722,40.4647120848362,40.8407044966673),
 .UNSPECIFIED.);
#4274=B_SPLINE_CURVE_WITH_KNOTS('',3,(#57617,#57618,#57619,#57620,#57621,
#57622,#57623,#57624,#57625,#57626),.UNSPECIFIED.,.F.,.F.,(4,1,1,1,1,1,
1,4),(34.5575191894877,35.1155162389165,36.1020455775805,37.0885749162445,
38.0751042549086,39.0616335935726,40.0481629322366,40.8407044966673),
 .UNSPECIFIED.);
#4275=B_SPLINE_CURVE_WITH_KNOTS('',3,(#57631,#57632,#57633,#57634,#57635,
#57636,#57637,#57638,#57639,#57640,#57641),.UNSPECIFIED.,.F.,.F.,(4,1,1,
1,1,1,1,1,4),(28.2743338823081,28.6263600208678,29.6128893595319,30.5994186981959,
31.5859480368599,32.572477375524,33.559006714188,34.545536052852,34.5575191894877),
 .UNSPECIFIED.);
#4276=B_SPLINE_CURVE_WITH_KNOTS('',3,(#57642,#57643,#57644,#57645,#57646,
#57647,#57648,#57649,#57650,#57651),.UNSPECIFIED.,.F.,.F.,(4,1,1,1,1,1,
1,4),(28.2743338823081,29.1963402069323,30.1828695455963,31.1693988842603,
32.1559282229244,33.1424575615884,34.1289869002524,34.5575191894877),
 .UNSPECIFIED.);
#4277=B_SPLINE_CURVE_WITH_KNOTS('',3,(#57656,#57657,#57658,#57659,#57660,
#57661,#57662,#57663,#57664,#57665),.UNSPECIFIED.,.F.,.F.,(4,1,1,1,1,1,
1,4),(21.9911485751285,22.7071839888837,23.6937133275477,24.6802426662117,
25.6667720048757,26.6533013435398,27.6398306822038,28.2743338823081),
 .UNSPECIFIED.);
#4278=B_SPLINE_CURVE_WITH_KNOTS('',3,(#57666,#57667,#57668,#57669,#57670,
#57671,#57672,#57673,#57674,#57675,#57676),.UNSPECIFIED.,.F.,.F.,(4,1,1,
1,1,1,1,1,4),(21.9911485751285,22.2906348362841,23.2771641749481,24.2636935136121,
25.2502228522762,26.2367521909402,27.2232815296042,28.2098108682683,28.2743338823081),
 .UNSPECIFIED.);
#4279=B_SPLINE_CURVE_WITH_KNOTS('',3,(#57682,#57683,#57684,#57685,#57686),
 .UNSPECIFIED.,.F.,.F.,(4,1,4),(14.3984001269718,15.3849294656359,15.7079632679489),
 .UNSPECIFIED.);
#4280=B_SPLINE_CURVE_WITH_KNOTS('',3,(#57689,#57690,#57691,#57692,#57693),
 .UNSPECIFIED.,.F.,.F.,(4,1,4),(13.8759337553362,14.8149492795714,15.7079632679489),
 .UNSPECIFIED.);
#4281=B_SPLINE_CURVE_WITH_KNOTS('',3,(#57699,#57700,#57701,#57702),
 .UNSPECIFIED.,.F.,.F.,(4,4),(51.5750455984138,52.2860549491937),
 .UNSPECIFIED.);
#4282=B_SPLINE_CURVE_WITH_KNOTS('',3,(#57714,#57715,#57716,#57717,#57718,
#57719,#57720,#57721,#57722,#57723),.UNSPECIFIED.,.F.,.F.,(4,3,3,4),(-50.2654824574367,
-49.3264669332015,-48.3399375945375,-47.8348991546267),.UNSPECIFIED.);
#4283=B_SPLINE_CURVE_WITH_KNOTS('',3,(#57728,#57729,#57730,#57731,#57732,
#57733,#57734,#57735,#57736,#57737,#57738,#57739,#57740,#57741,#57742,#57743,
#57744,#57745,#57746,#57747,#57748,#57749,#57750,#57751,#57752),
 .UNSPECIFIED.,.F.,.F.,(4,3,3,3,3,3,3,3,4),(45.2918602912342,45.3803495785454,
46.3668789172095,47.3534082558735,48.3399375945375,49.3264669332015,50.3129962718656,
51.2995256105296,51.5750455984138),.UNSPECIFIED.);
#4284=B_SPLINE_CURVE_WITH_KNOTS('',3,(#57753,#57754,#57755,#57756,#57757,
#57758,#57759,#57760,#57761,#57762,#57763,#57764,#57765,#57766,#57767,#57768,
#57769,#57770,#57771,#57772,#57773,#57774),.UNSPECIFIED.,.F.,.F.,(4,3,3,
3,3,3,3,4),(-47.8348991546267,-47.3534082558735,-46.3668789172094,-45.3803495785454,
-44.3938202398814,-43.4072909012173,-42.4207615625533,-41.5517138474471),
 .UNSPECIFIED.);
#4285=B_SPLINE_CURVE_WITH_KNOTS('',3,(#57779,#57780,#57781,#57782,#57783,
#57784,#57785,#57786,#57787,#57788,#57789,#57790,#57791,#57792,#57793,#57794,
#57795,#57796,#57797,#57798,#57799,#57800),.UNSPECIFIED.,.F.,.F.,(4,3,3,
3,3,3,3,4),(39.0086749840546,39.4611735465612,40.4477028852253,41.4342322238893,
42.4207615625533,43.4072909012174,44.3938202398814,45.2918602912342),
 .UNSPECIFIED.);
#4286=B_SPLINE_CURVE_WITH_KNOTS('',3,(#57801,#57802,#57803,#57804,#57805,
#57806,#57807,#57808,#57809,#57810,#57811,#57812,#57813,#57814,#57815,#57816,
#57817,#57818,#57819,#57820,#57821,#57822,#57823,#57824,#57825),
 .UNSPECIFIED.,.F.,.F.,(4,3,3,3,3,3,3,3,4),(-41.5517138474471,-41.4342322238893,
-40.4477028852252,-39.4611735465612,-38.4746442078972,-37.4881148692332,
-36.5015855305691,-35.5150561919051,-35.2685285402675),.UNSPECIFIED.);
#4287=B_SPLINE_CURVE_WITH_KNOTS('',3,(#57830,#57831,#57832,#57833,#57834,
#57835,#57836,#57837,#57838,#57839,#57840,#57841,#57842,#57843,#57844,#57845,
#57846,#57847,#57848,#57849,#57850,#57851),.UNSPECIFIED.,.F.,.F.,(4,3,3,
3,3,3,3,4),(32.725489676875,33.541997514577,34.5285268532411,35.5150561919051,
36.5015855305691,37.4881148692332,38.4746442078972,39.0086749840546),
 .UNSPECIFIED.);
#4288=B_SPLINE_CURVE_WITH_KNOTS('',3,(#57852,#57853,#57854,#57855,#57856,
#57857,#57858,#57859,#57860,#57861,#57862,#57863,#57864,#57865,#57866,#57867,
#57868,#57869,#57870,#57871,#57872,#57873),.UNSPECIFIED.,.F.,.F.,(4,3,3,
3,3,3,3,4),(-35.2685285402675,-34.5285268532411,-33.541997514577,-32.555468175913,
-31.568938837249,-30.5824094985849,-29.5958801599209,-28.985343233088),
 .UNSPECIFIED.);
#4289=B_SPLINE_CURVE_WITH_KNOTS('',3,(#57878,#57879,#57880,#57881,#57882,
#57883,#57884,#57885,#57886,#57887,#57888,#57889,#57890,#57891,#57892,#57893,
#57894,#57895,#57896,#57897,#57898,#57899,#57900,#57901,#57902),
 .UNSPECIFIED.,.F.,.F.,(4,3,3,3,3,3,3,3,4),(26.4423043696954,26.6362921439288,
27.6228214825929,28.6093508212569,29.5958801599209,30.582409498585,31.568938837249,
32.555468175913,32.725489676875),.UNSPECIFIED.);
#4290=B_SPLINE_CURVE_WITH_KNOTS('',3,(#57903,#57904,#57905,#57906,#57907,
#57908,#57909,#57910,#57911,#57912,#57913,#57914,#57915,#57916,#57917,#57918,
#57919,#57920,#57921,#57922,#57923,#57924),.UNSPECIFIED.,.F.,.F.,(4,3,3,
3,3,3,3,4),(-28.985343233088,-28.6093508212569,-27.6228214825929,-26.6362921439288,
-25.6497628052648,-24.6632334666008,-23.6767041279367,-22.7021579259084),
 .UNSPECIFIED.);
#4291=B_SPLINE_CURVE_WITH_KNOTS('',3,(#57929,#57930,#57931,#57932,#57933,
#57934,#57935,#57936,#57937,#57938,#57939,#57940,#57941,#57942,#57943,#57944,
#57945,#57946,#57947,#57948,#57949,#57950),.UNSPECIFIED.,.F.,.F.,(4,3,3,
3,3,3,3,4),(20.1591190625159,20.7171161119446,21.7036454506087,22.6901747892727,
23.6767041279367,24.6632334666008,25.6497628052648,26.4423043696954),
 .UNSPECIFIED.);
#4292=B_SPLINE_CURVE_WITH_KNOTS('',3,(#57951,#57952,#57953,#57954,#57955,
#57956,#57957,#57958,#57959,#57960,#57961,#57962,#57963,#57964,#57965,#57966,
#57967,#57968,#57969,#57970,#57971,#57972,#57973,#57974,#57975),
 .UNSPECIFIED.,.F.,.F.,(4,3,3,3,3,3,3,3,4),(-22.7021579259084,-22.6901747892727,
-21.7036454506087,-20.7171161119446,-19.7305867732806,-18.7440574346166,
-17.7575280959525,-16.7709987572885,-16.4189726187288),.UNSPECIFIED.);
#4293=B_SPLINE_CURVE_WITH_KNOTS('',3,(#57980,#57981,#57982,#57983,#57984,
#57985,#57986,#57987,#57988,#57989,#57990,#57991,#57992,#57993,#57994,#57995,
#57996,#57997,#57998,#57999,#58000,#58001),.UNSPECIFIED.,.F.,.F.,(4,3,3,
3,3,3,3,4),(13.8759337553363,14.7979400799605,15.7844694186245,16.7709987572885,
17.7575280959526,18.7440574346166,19.7305867732806,20.1591190625159),
 .UNSPECIFIED.);
#4294=B_SPLINE_CURVE_WITH_KNOTS('',3,(#58002,#58003,#58004,#58005,#58006,
#58007,#58008,#58009,#58010,#58011,#58012,#58013,#58014,#58015,#58016,#58017,
#58018,#58019,#58020,#58021,#58022,#58023),.UNSPECIFIED.,.F.,.F.,(4,3,3,
3,3,3,3,4),(-16.4189726187288,-15.7844694186245,-14.7979400799605,-13.8114107412964,
-12.8248814026324,-11.8383520639684,-10.8518227253043,-10.1357873115492),
 .UNSPECIFIED.);
#4295=B_SPLINE_CURVE_WITH_KNOTS('',3,(#58029,#58030,#58031,#58032,#58033,
#58034,#58035,#58036,#58037,#58038,#58039,#58040,#58041),.UNSPECIFIED.,
 .F.,.F.,(4,3,3,3,4),(-3.85260200436961,-2.95958801599209,-1.97305867732806,
-0.986529338664033,0.),.UNSPECIFIED.);
#4296=B_SPLINE_CURVE_WITH_KNOTS('',3,(#58044,#58045,#58046,#58047,#58048,
#58049,#58050,#58051,#58052,#58053,#58054,#58055,#58056,#58057,#58058,#58059,
#58060,#58061,#58062),.UNSPECIFIED.,.F.,.F.,(4,3,3,3,3,3,4),(2.02057249175696,
2.95958801599209,3.94611735465612,4.93264669332015,5.91917603198419,6.90570537064821,
7.59274844815668),.UNSPECIFIED.);
#4297=B_SPLINE_CURVE_WITH_KNOTS('',3,(#58068,#58069,#58070,#58071,#58072,
#58073,#58074,#58075),.UNSPECIFIED.,.F.,.F.,(4,1,1,1,1,4),(59.6902604182061,
60.1952988581168,61.1818281967808,62.1683575354449,63.1548868741089,64.1414162127729),
 .UNSPECIFIED.);
#4298=B_SPLINE_CURVE_WITH_KNOTS('',3,(#58078,#58079,#58080,#58081,#58082,
#58083,#58084,#58085,#58086),.UNSPECIFIED.,.F.,.F.,(4,1,1,1,1,1,4),(59.6902604182061,
59.7787497055172,60.7652790441813,61.7518083828453,62.7383377215093,63.7248670601734,
64.6638825844085),.UNSPECIFIED.);
#4299=B_SPLINE_CURVE_WITH_KNOTS('',3,(#58091,#58092,#58093,#58094,#58095,
#58096,#58097,#58098,#58099,#58100),.UNSPECIFIED.,.F.,.F.,(4,1,1,1,1,1,
1,4),(53.4070751110265,54.2761228261326,55.2626521647967,56.2491815034607,
57.2357108421247,58.2222401807888,59.2087695194528,59.6902604182061),
 .UNSPECIFIED.);
#4300=B_SPLINE_CURVE_WITH_KNOTS('',3,(#58101,#58102,#58103,#58104,#58105,
#58106,#58107,#58108,#58109,#58110),.UNSPECIFIED.,.F.,.F.,(4,1,1,1,1,1,
1,4),(53.4070751110265,53.8595736735331,54.8461030121971,55.8326323508611,
56.8191616895252,57.8056910281892,58.7922203668532,59.6902604182061),
 .UNSPECIFIED.);
#4301=B_SPLINE_CURVE_WITH_KNOTS('',3,(#58115,#58116,#58117,#58118,#58119,
#58120,#58121,#58122,#58123,#58124,#58125),.UNSPECIFIED.,.F.,.F.,(4,1,1,
1,1,1,1,1,4),(47.1238898038469,47.3704174554844,48.3569467941485,49.3434761328125,
50.3300054714765,51.3165348101405,52.3030641488046,53.2895934874686,53.4070751110265),
 .UNSPECIFIED.);
#4302=B_SPLINE_CURVE_WITH_KNOTS('',3,(#58126,#58127,#58128,#58129,#58130,
#58131,#58132,#58133,#58134,#58135),.UNSPECIFIED.,.F.,.F.,(4,1,1,1,1,1,
1,4),(47.1238898038469,47.9403976415489,48.9269269802129,49.9134563188769,
50.899985657541,51.886514996205,52.873044334869,53.4070751110265),
 .UNSPECIFIED.);
#4303=B_SPLINE_CURVE_WITH_KNOTS('',3,(#58140,#58141,#58142,#58143,#58144,
#58145,#58146,#58147,#58148,#58149),.UNSPECIFIED.,.F.,.F.,(4,1,1,1,1,1,
1,4),(40.8407044966673,41.4512414235002,42.4377707621643,43.4243001008283,
44.4108294394923,45.3973587781564,46.3838881168204,47.1238898038469),
 .UNSPECIFIED.);
#4304=B_SPLINE_CURVE_WITH_KNOTS('',3,(#58150,#58151,#58152,#58153,#58154,
#58155,#58156,#58157,#58158,#58159,#58160),.UNSPECIFIED.,.F.,.F.,(4,1,1,
1,1,1,1,1,4),(40.8407044966673,41.0346922709007,42.0212216095647,43.0077509482287,
43.9942802868928,44.9808096255568,45.9673389642208,46.9538683028848,47.1238898038469),
 .UNSPECIFIED.);
#4305=B_SPLINE_CURVE_WITH_KNOTS('',3,(#58165,#58166,#58167,#58168,#58169,
#58170,#58171,#58172,#58173,#58174),.UNSPECIFIED.,.F.,.F.,(4,1,1,1,1,1,
1,4),(34.5575191894877,35.5320653915161,36.5185947301801,37.5051240688441,
38.4916534075081,39.4781827461722,40.4647120848362,40.8407044966673),
 .UNSPECIFIED.);
#4306=B_SPLINE_CURVE_WITH_KNOTS('',3,(#58175,#58176,#58177,#58178,#58179,
#58180,#58181,#58182,#58183,#58184),.UNSPECIFIED.,.F.,.F.,(4,1,1,1,1,1,
1,4),(34.5575191894877,35.1155162389165,36.1020455775805,37.0885749162445,
38.0751042549086,39.0616335935726,40.0481629322366,40.8407044966673),
 .UNSPECIFIED.);
#4307=B_SPLINE_CURVE_WITH_KNOTS('',3,(#58189,#58190,#58191,#58192,#58193,
#58194,#58195,#58196,#58197,#58198,#58199),.UNSPECIFIED.,.F.,.F.,(4,1,1,
1,1,1,1,1,4),(28.2743338823081,28.6263600208678,29.6128893595319,30.5994186981959,
31.5859480368599,32.572477375524,33.559006714188,34.545536052852,34.5575191894877),
 .UNSPECIFIED.);
#4308=B_SPLINE_CURVE_WITH_KNOTS('',3,(#58200,#58201,#58202,#58203,#58204,
#58205,#58206,#58207,#58208,#58209),.UNSPECIFIED.,.F.,.F.,(4,1,1,1,1,1,
1,4),(28.2743338823081,29.1963402069323,30.1828695455963,31.1693988842603,
32.1559282229244,33.1424575615884,34.1289869002524,34.5575191894877),
 .UNSPECIFIED.);
#4309=B_SPLINE_CURVE_WITH_KNOTS('',3,(#58214,#58215,#58216,#58217,#58218,
#58219,#58220,#58221,#58222,#58223),.UNSPECIFIED.,.F.,.F.,(4,1,1,1,1,1,
1,4),(21.9911485751285,22.7071839888837,23.6937133275477,24.6802426662117,
25.6667720048758,26.6533013435398,27.6398306822038,28.2743338823081),
 .UNSPECIFIED.);
#4310=B_SPLINE_CURVE_WITH_KNOTS('',3,(#58224,#58225,#58226,#58227,#58228,
#58229,#58230,#58231,#58232,#58233,#58234),.UNSPECIFIED.,.F.,.F.,(4,1,1,
1,1,1,1,1,4),(21.9911485751285,22.2906348362841,23.2771641749481,24.2636935136121,
25.2502228522762,26.2367521909402,27.2232815296042,28.2098108682683,28.2743338823081),
 .UNSPECIFIED.);
#4311=B_SPLINE_CURVE_WITH_KNOTS('',3,(#58240,#58241,#58242,#58243,#58244),
 .UNSPECIFIED.,.F.,.F.,(4,1,4),(14.3984001269718,15.3849294656359,15.7079632679489),
 .UNSPECIFIED.);
#4312=B_SPLINE_CURVE_WITH_KNOTS('',3,(#58247,#58248,#58249,#58250,#58251),
 .UNSPECIFIED.,.F.,.F.,(4,1,4),(13.8759337553362,14.8149492795714,15.7079632679489),
 .UNSPECIFIED.);
#4313=B_SPLINE_CURVE_WITH_KNOTS('',3,(#58257,#58258,#58259,#58260),
 .UNSPECIFIED.,.F.,.F.,(4,4),(51.5750455984138,52.2860549491937),
 .UNSPECIFIED.);
#4314=B_SPLINE_CURVE_WITH_KNOTS('',3,(#58272,#58273,#58274,#58275,#58276,
#58277,#58278,#58279,#58280,#58281),.UNSPECIFIED.,.F.,.F.,(4,3,3,4),(-50.2654824574368,
-49.3264669332015,-48.3399375945375,-47.8348991546267),.UNSPECIFIED.);
#4315=B_SPLINE_CURVE_WITH_KNOTS('',3,(#58286,#58287,#58288,#58289,#58290,
#58291,#58292,#58293,#58294,#58295,#58296,#58297,#58298,#58299,#58300,#58301,
#58302,#58303,#58304,#58305,#58306,#58307,#58308,#58309,#58310),
 .UNSPECIFIED.,.F.,.F.,(4,3,3,3,3,3,3,3,4),(45.2918602912342,45.3803495785454,
46.3668789172095,47.3534082558735,48.3399375945375,49.3264669332015,50.3129962718656,
51.2995256105296,51.5750455984138),.UNSPECIFIED.);
#4316=B_SPLINE_CURVE_WITH_KNOTS('',3,(#58311,#58312,#58313,#58314,#58315,
#58316,#58317,#58318,#58319,#58320,#58321,#58322,#58323,#58324,#58325,#58326,
#58327,#58328,#58329,#58330,#58331,#58332),.UNSPECIFIED.,.F.,.F.,(4,3,3,
3,3,3,3,4),(-47.8348991546267,-47.3534082558735,-46.3668789172094,-45.3803495785454,
-44.3938202398814,-43.4072909012173,-42.4207615625533,-41.5517138474471),
 .UNSPECIFIED.);
#4317=B_SPLINE_CURVE_WITH_KNOTS('',3,(#58337,#58338,#58339,#58340,#58341,
#58342,#58343,#58344,#58345,#58346,#58347,#58348,#58349,#58350,#58351,#58352,
#58353,#58354,#58355,#58356,#58357,#58358),.UNSPECIFIED.,.F.,.F.,(4,3,3,
3,3,3,3,4),(39.0086749840546,39.4611735465612,40.4477028852253,41.4342322238893,
42.4207615625533,43.4072909012174,44.3938202398814,45.2918602912342),
 .UNSPECIFIED.);
#4318=B_SPLINE_CURVE_WITH_KNOTS('',3,(#58359,#58360,#58361,#58362,#58363,
#58364,#58365,#58366,#58367,#58368,#58369,#58370,#58371,#58372,#58373,#58374,
#58375,#58376,#58377,#58378,#58379,#58380,#58381,#58382,#58383),
 .UNSPECIFIED.,.F.,.F.,(4,3,3,3,3,3,3,3,4),(-41.5517138474471,-41.4342322238893,
-40.4477028852253,-39.4611735465612,-38.4746442078972,-37.4881148692332,
-36.5015855305691,-35.5150561919051,-35.2685285402676),.UNSPECIFIED.);
#4319=B_SPLINE_CURVE_WITH_KNOTS('',3,(#58388,#58389,#58390,#58391,#58392,
#58393,#58394,#58395,#58396,#58397,#58398,#58399,#58400,#58401,#58402,#58403,
#58404,#58405,#58406,#58407,#58408,#58409),.UNSPECIFIED.,.F.,.F.,(4,3,3,
3,3,3,3,4),(32.725489676875,33.541997514577,34.5285268532411,35.5150561919051,
36.5015855305691,37.4881148692332,38.4746442078972,39.0086749840546),
 .UNSPECIFIED.);
#4320=B_SPLINE_CURVE_WITH_KNOTS('',3,(#58410,#58411,#58412,#58413,#58414,
#58415,#58416,#58417,#58418,#58419,#58420,#58421,#58422,#58423,#58424,#58425,
#58426,#58427,#58428,#58429,#58430,#58431),.UNSPECIFIED.,.F.,.F.,(4,3,3,
3,3,3,3,4),(-35.2685285402676,-34.5285268532411,-33.541997514577,-32.555468175913,
-31.568938837249,-30.5824094985849,-29.5958801599209,-28.985343233088),
 .UNSPECIFIED.);
#4321=B_SPLINE_CURVE_WITH_KNOTS('',3,(#58436,#58437,#58438,#58439,#58440,
#58441,#58442,#58443,#58444,#58445,#58446,#58447,#58448,#58449,#58450,#58451,
#58452,#58453,#58454,#58455,#58456,#58457,#58458,#58459,#58460),
 .UNSPECIFIED.,.F.,.F.,(4,3,3,3,3,3,3,3,4),(26.4423043696954,26.6362921439288,
27.6228214825929,28.6093508212569,29.5958801599209,30.582409498585,31.568938837249,
32.555468175913,32.725489676875),.UNSPECIFIED.);
#4322=B_SPLINE_CURVE_WITH_KNOTS('',3,(#58461,#58462,#58463,#58464,#58465,
#58466,#58467,#58468,#58469,#58470,#58471,#58472,#58473,#58474,#58475,#58476,
#58477,#58478,#58479,#58480,#58481,#58482),.UNSPECIFIED.,.F.,.F.,(4,3,3,
3,3,3,3,4),(-28.985343233088,-28.6093508212569,-27.6228214825929,-26.6362921439288,
-25.6497628052648,-24.6632334666008,-23.6767041279367,-22.7021579259084),
 .UNSPECIFIED.);
#4323=B_SPLINE_CURVE_WITH_KNOTS('',3,(#58487,#58488,#58489,#58490,#58491,
#58492,#58493,#58494,#58495,#58496,#58497,#58498,#58499,#58500,#58501,#58502,
#58503,#58504,#58505,#58506,#58507,#58508),.UNSPECIFIED.,.F.,.F.,(4,3,3,
3,3,3,3,4),(20.1591190625159,20.7171161119446,21.7036454506087,22.6901747892727,
23.6767041279367,24.6632334666008,25.6497628052648,26.4423043696954),
 .UNSPECIFIED.);
#4324=B_SPLINE_CURVE_WITH_KNOTS('',3,(#58509,#58510,#58511,#58512,#58513,
#58514,#58515,#58516,#58517,#58518,#58519,#58520,#58521,#58522,#58523,#58524,
#58525,#58526,#58527,#58528,#58529,#58530,#58531,#58532,#58533),
 .UNSPECIFIED.,.F.,.F.,(4,3,3,3,3,3,3,3,4),(-22.7021579259084,-22.6901747892727,
-21.7036454506087,-20.7171161119446,-19.7305867732806,-18.7440574346166,
-17.7575280959526,-16.7709987572885,-16.4189726187288),.UNSPECIFIED.);
#4325=B_SPLINE_CURVE_WITH_KNOTS('',3,(#58538,#58539,#58540,#58541,#58542,
#58543,#58544,#58545,#58546,#58547,#58548,#58549,#58550,#58551,#58552,#58553,
#58554,#58555,#58556,#58557,#58558,#58559),.UNSPECIFIED.,.F.,.F.,(4,3,3,
3,3,3,3,4),(13.8759337553363,14.7979400799605,15.7844694186245,16.7709987572885,
17.7575280959526,18.7440574346166,19.7305867732806,20.1591190625159),
 .UNSPECIFIED.);
#4326=B_SPLINE_CURVE_WITH_KNOTS('',3,(#58560,#58561,#58562,#58563,#58564,
#58565,#58566,#58567,#58568,#58569,#58570,#58571,#58572,#58573,#58574,#58575,
#58576,#58577,#58578,#58579,#58580,#58581),.UNSPECIFIED.,.F.,.F.,(4,3,3,
3,3,3,3,4),(-16.4189726187288,-15.7844694186245,-14.7979400799605,-13.8114107412964,
-12.8248814026324,-11.8383520639684,-10.8518227253043,-10.1357873115492),
 .UNSPECIFIED.);
#4327=B_SPLINE_CURVE_WITH_KNOTS('',3,(#58587,#58588,#58589,#58590,#58591,
#58592,#58593,#58594,#58595,#58596,#58597,#58598,#58599),.UNSPECIFIED.,
 .F.,.F.,(4,3,3,3,4),(-3.85260200436962,-2.95958801599209,-1.97305867732806,
-0.986529338664033,0.),.UNSPECIFIED.);
#4328=B_SPLINE_CURVE_WITH_KNOTS('',3,(#58602,#58603,#58604,#58605,#58606,
#58607,#58608,#58609,#58610,#58611,#58612,#58613,#58614,#58615,#58616,#58617,
#58618,#58619,#58620),.UNSPECIFIED.,.F.,.F.,(4,3,3,3,3,3,4),(2.02057249175683,
2.95958801599209,3.94611735465612,4.93264669332015,5.91917603198419,6.90570537064822,
7.59274844815668),.UNSPECIFIED.);
#4329=B_SPLINE_CURVE_WITH_KNOTS('',3,(#58626,#58627,#58628,#58629,#58630,
#58631,#58632,#58633),.UNSPECIFIED.,.F.,.F.,(4,1,1,1,1,4),(59.6902604182061,
60.1952988581168,61.1818281967809,62.1683575354449,63.1548868741089,64.141416212773),
 .UNSPECIFIED.);
#4330=B_SPLINE_CURVE_WITH_KNOTS('',3,(#58636,#58637,#58638,#58639,#58640,
#58641,#58642,#58643,#58644),.UNSPECIFIED.,.F.,.F.,(4,1,1,1,1,1,4),(59.6902604182061,
59.7787497055173,60.7652790441813,61.7518083828453,62.7383377215094,63.7248670601734,
64.6638825844085),.UNSPECIFIED.);
#4331=B_SPLINE_CURVE_WITH_KNOTS('',3,(#58649,#58650,#58651,#58652,#58653,
#58654,#58655,#58656,#58657,#58658),.UNSPECIFIED.,.F.,.F.,(4,1,1,1,1,1,
1,4),(53.4070751110265,54.2761228261326,55.2626521647967,56.2491815034607,
57.2357108421247,58.2222401807888,59.2087695194528,59.6902604182061),
 .UNSPECIFIED.);
#4332=B_SPLINE_CURVE_WITH_KNOTS('',3,(#58659,#58660,#58661,#58662,#58663,
#58664,#58665,#58666,#58667,#58668),.UNSPECIFIED.,.F.,.F.,(4,1,1,1,1,1,
1,4),(53.4070751110265,53.8595736735331,54.8461030121971,55.8326323508611,
56.8191616895252,57.8056910281892,58.7922203668532,59.6902604182061),
 .UNSPECIFIED.);
#4333=B_SPLINE_CURVE_WITH_KNOTS('',3,(#58673,#58674,#58675,#58676,#58677,
#58678,#58679,#58680,#58681,#58682,#58683),.UNSPECIFIED.,.F.,.F.,(4,1,1,
1,1,1,1,1,4),(47.1238898038469,47.3704174554844,48.3569467941485,49.3434761328125,
50.3300054714765,51.3165348101406,52.3030641488046,53.2895934874686,53.4070751110265),
 .UNSPECIFIED.);
#4334=B_SPLINE_CURVE_WITH_KNOTS('',3,(#58684,#58685,#58686,#58687,#58688,
#58689,#58690,#58691,#58692,#58693),.UNSPECIFIED.,.F.,.F.,(4,1,1,1,1,1,
1,4),(47.1238898038469,47.9403976415489,48.9269269802129,49.9134563188769,
50.899985657541,51.886514996205,52.873044334869,53.4070751110265),
 .UNSPECIFIED.);
#4335=B_SPLINE_CURVE_WITH_KNOTS('',3,(#58698,#58699,#58700,#58701,#58702,
#58703,#58704,#58705,#58706,#58707),.UNSPECIFIED.,.F.,.F.,(4,1,1,1,1,1,
1,4),(40.8407044966673,41.4512414235002,42.4377707621643,43.4243001008283,
44.4108294394923,45.3973587781564,46.3838881168204,47.1238898038469),
 .UNSPECIFIED.);
#4336=B_SPLINE_CURVE_WITH_KNOTS('',3,(#58708,#58709,#58710,#58711,#58712,
#58713,#58714,#58715,#58716,#58717,#58718),.UNSPECIFIED.,.F.,.F.,(4,1,1,
1,1,1,1,1,4),(40.8407044966673,41.0346922709007,42.0212216095647,43.0077509482287,
43.9942802868928,44.9808096255568,45.9673389642208,46.9538683028849,47.1238898038469),
 .UNSPECIFIED.);
#4337=B_SPLINE_CURVE_WITH_KNOTS('',3,(#58723,#58724,#58725,#58726,#58727,
#58728,#58729,#58730,#58731,#58732),.UNSPECIFIED.,.F.,.F.,(4,1,1,1,1,1,
1,4),(34.5575191894877,35.5320653915161,36.5185947301801,37.5051240688441,
38.4916534075082,39.4781827461722,40.4647120848362,40.8407044966673),
 .UNSPECIFIED.);
#4338=B_SPLINE_CURVE_WITH_KNOTS('',3,(#58733,#58734,#58735,#58736,#58737,
#58738,#58739,#58740,#58741,#58742),.UNSPECIFIED.,.F.,.F.,(4,1,1,1,1,1,
1,4),(34.5575191894877,35.1155162389165,36.1020455775805,37.0885749162445,
38.0751042549086,39.0616335935726,40.0481629322366,40.8407044966673),
 .UNSPECIFIED.);
#4339=B_SPLINE_CURVE_WITH_KNOTS('',3,(#58747,#58748,#58749,#58750,#58751,
#58752,#58753,#58754,#58755,#58756,#58757),.UNSPECIFIED.,.F.,.F.,(4,1,1,
1,1,1,1,1,4),(28.2743338823081,28.6263600208679,29.6128893595319,30.5994186981959,
31.5859480368599,32.572477375524,33.559006714188,34.545536052852,34.5575191894877),
 .UNSPECIFIED.);
#4340=B_SPLINE_CURVE_WITH_KNOTS('',3,(#58758,#58759,#58760,#58761,#58762,
#58763,#58764,#58765,#58766,#58767),.UNSPECIFIED.,.F.,.F.,(4,1,1,1,1,1,
1,4),(28.2743338823081,29.1963402069323,30.1828695455963,31.1693988842604,
32.1559282229244,33.1424575615884,34.1289869002525,34.5575191894877),
 .UNSPECIFIED.);
#4341=B_SPLINE_CURVE_WITH_KNOTS('',3,(#58772,#58773,#58774,#58775,#58776,
#58777,#58778,#58779,#58780,#58781),.UNSPECIFIED.,.F.,.F.,(4,1,1,1,1,1,
1,4),(21.9911485751285,22.7071839888837,23.6937133275477,24.6802426662117,
25.6667720048758,26.6533013435398,27.6398306822038,28.2743338823081),
 .UNSPECIFIED.);
#4342=B_SPLINE_CURVE_WITH_KNOTS('',3,(#58782,#58783,#58784,#58785,#58786,
#58787,#58788,#58789,#58790,#58791,#58792),.UNSPECIFIED.,.F.,.F.,(4,1,1,
1,1,1,1,1,4),(21.9911485751285,22.2906348362841,23.2771641749481,24.2636935136121,
25.2502228522762,26.2367521909402,27.2232815296042,28.2098108682683,28.2743338823081),
 .UNSPECIFIED.);
#4343=B_SPLINE_CURVE_WITH_KNOTS('',3,(#58798,#58799,#58800,#58801,#58802),
 .UNSPECIFIED.,.F.,.F.,(4,1,4),(14.3984001269718,15.3849294656359,15.7079632679489),
 .UNSPECIFIED.);
#4344=B_SPLINE_CURVE_WITH_KNOTS('',3,(#58805,#58806,#58807,#58808,#58809),
 .UNSPECIFIED.,.F.,.F.,(4,1,4),(13.8759337553363,14.8149492795714,15.7079632679489),
 .UNSPECIFIED.);
#4345=B_SPLINE_CURVE_WITH_KNOTS('',3,(#58815,#58816,#58817,#58818),
 .UNSPECIFIED.,.F.,.F.,(4,4),(51.5750455984138,52.2860549491937),
 .UNSPECIFIED.);
#4346=B_SPLINE_CURVE_WITH_KNOTS('',3,(#58830,#58831,#58832,#58833,#58834,
#58835,#58836,#58837,#58838,#58839),.UNSPECIFIED.,.F.,.F.,(4,3,3,4),(-50.2654824574367,
-49.3264669332015,-48.3399375945375,-47.8348991546267),.UNSPECIFIED.);
#4347=B_SPLINE_CURVE_WITH_KNOTS('',3,(#58844,#58845,#58846,#58847,#58848,
#58849,#58850,#58851,#58852,#58853,#58854,#58855,#58856,#58857,#58858,#58859,
#58860,#58861,#58862,#58863,#58864,#58865,#58866,#58867,#58868),
 .UNSPECIFIED.,.F.,.F.,(4,3,3,3,3,3,3,3,4),(45.2918602912342,45.3803495785454,
46.3668789172095,47.3534082558735,48.3399375945375,49.3264669332015,50.3129962718656,
51.2995256105296,51.5750455984138),.UNSPECIFIED.);
#4348=B_SPLINE_CURVE_WITH_KNOTS('',3,(#58869,#58870,#58871,#58872,#58873,
#58874,#58875,#58876,#58877,#58878,#58879,#58880,#58881,#58882,#58883,#58884,
#58885,#58886,#58887,#58888,#58889,#58890),.UNSPECIFIED.,.F.,.F.,(4,3,3,
3,3,3,3,4),(-47.8348991546267,-47.3534082558735,-46.3668789172094,-45.3803495785454,
-44.3938202398814,-43.4072909012173,-42.4207615625533,-41.5517138474471),
 .UNSPECIFIED.);
#4349=B_SPLINE_CURVE_WITH_KNOTS('',3,(#58895,#58896,#58897,#58898,#58899,
#58900,#58901,#58902,#58903,#58904,#58905,#58906,#58907,#58908,#58909,#58910,
#58911,#58912,#58913,#58914,#58915,#58916),.UNSPECIFIED.,.F.,.F.,(4,3,3,
3,3,3,3,4),(39.0086749840546,39.4611735465612,40.4477028852253,41.4342322238893,
42.4207615625533,43.4072909012174,44.3938202398814,45.2918602912342),
 .UNSPECIFIED.);
#4350=B_SPLINE_CURVE_WITH_KNOTS('',3,(#58917,#58918,#58919,#58920,#58921,
#58922,#58923,#58924,#58925,#58926,#58927,#58928,#58929,#58930,#58931,#58932,
#58933,#58934,#58935,#58936,#58937,#58938,#58939,#58940,#58941),
 .UNSPECIFIED.,.F.,.F.,(4,3,3,3,3,3,3,3,4),(-41.5517138474471,-41.4342322238893,
-40.4477028852252,-39.4611735465612,-38.4746442078972,-37.4881148692332,
-36.5015855305691,-35.5150561919051,-35.2685285402676),.UNSPECIFIED.);
#4351=B_SPLINE_CURVE_WITH_KNOTS('',3,(#58946,#58947,#58948,#58949,#58950,
#58951,#58952,#58953,#58954,#58955,#58956,#58957,#58958,#58959,#58960,#58961,
#58962,#58963,#58964,#58965,#58966,#58967),.UNSPECIFIED.,.F.,.F.,(4,3,3,
3,3,3,3,4),(32.725489676875,33.5419975145771,34.5285268532411,35.5150561919051,
36.5015855305692,37.4881148692332,38.4746442078972,39.0086749840546),
 .UNSPECIFIED.);
#4352=B_SPLINE_CURVE_WITH_KNOTS('',3,(#58968,#58969,#58970,#58971,#58972,
#58973,#58974,#58975,#58976,#58977,#58978,#58979,#58980,#58981,#58982,#58983,
#58984,#58985,#58986,#58987,#58988,#58989),.UNSPECIFIED.,.F.,.F.,(4,3,3,
3,3,3,3,4),(-35.2685285402676,-34.5285268532411,-33.541997514577,-32.555468175913,
-31.568938837249,-30.5824094985849,-29.5958801599209,-28.985343233088),
 .UNSPECIFIED.);
#4353=B_SPLINE_CURVE_WITH_KNOTS('',3,(#58994,#58995,#58996,#58997,#58998,
#58999,#59000,#59001,#59002,#59003,#59004,#59005,#59006,#59007,#59008,#59009,
#59010,#59011,#59012,#59013,#59014,#59015,#59016,#59017,#59018),
 .UNSPECIFIED.,.F.,.F.,(4,3,3,3,3,3,3,3,4),(26.4423043696954,26.6362921439288,
27.6228214825929,28.6093508212569,29.5958801599209,30.582409498585,31.568938837249,
32.555468175913,32.725489676875),.UNSPECIFIED.);
#4354=B_SPLINE_CURVE_WITH_KNOTS('',3,(#59019,#59020,#59021,#59022,#59023,
#59024,#59025,#59026,#59027,#59028,#59029,#59030,#59031,#59032,#59033,#59034,
#59035,#59036,#59037,#59038,#59039,#59040),.UNSPECIFIED.,.F.,.F.,(4,3,3,
3,3,3,3,4),(-28.985343233088,-28.6093508212569,-27.6228214825929,-26.6362921439288,
-25.6497628052648,-24.6632334666008,-23.6767041279367,-22.7021579259084),
 .UNSPECIFIED.);
#4355=B_SPLINE_CURVE_WITH_KNOTS('',3,(#59045,#59046,#59047,#59048,#59049,
#59050,#59051,#59052,#59053,#59054,#59055,#59056,#59057,#59058,#59059,#59060,
#59061,#59062,#59063,#59064,#59065,#59066),.UNSPECIFIED.,.F.,.F.,(4,3,3,
3,3,3,3,4),(20.1591190625159,20.7171161119447,21.7036454506087,22.6901747892727,
23.6767041279367,24.6632334666008,25.6497628052648,26.4423043696954),
 .UNSPECIFIED.);
#4356=B_SPLINE_CURVE_WITH_KNOTS('',3,(#59067,#59068,#59069,#59070,#59071,
#59072,#59073,#59074,#59075,#59076,#59077,#59078,#59079,#59080,#59081,#59082,
#59083,#59084,#59085,#59086,#59087,#59088,#59089,#59090,#59091),
 .UNSPECIFIED.,.F.,.F.,(4,3,3,3,3,3,3,3,4),(-22.7021579259084,-22.6901747892727,
-21.7036454506087,-20.7171161119446,-19.7305867732806,-18.7440574346166,
-17.7575280959525,-16.7709987572885,-16.4189726187288),.UNSPECIFIED.);
#4357=B_SPLINE_CURVE_WITH_KNOTS('',3,(#59096,#59097,#59098,#59099,#59100,
#59101,#59102,#59103,#59104,#59105,#59106,#59107,#59108,#59109,#59110,#59111,
#59112,#59113,#59114,#59115,#59116,#59117),.UNSPECIFIED.,.F.,.F.,(4,3,3,
3,3,3,3,4),(13.8759337553363,14.7979400799605,15.7844694186245,16.7709987572885,
17.7575280959526,18.7440574346166,19.7305867732806,20.1591190625159),
 .UNSPECIFIED.);
#4358=B_SPLINE_CURVE_WITH_KNOTS('',3,(#59118,#59119,#59120,#59121,#59122,
#59123,#59124,#59125,#59126,#59127,#59128,#59129,#59130,#59131,#59132,#59133,
#59134,#59135,#59136,#59137,#59138,#59139),.UNSPECIFIED.,.F.,.F.,(4,3,3,
3,3,3,3,4),(-16.4189726187288,-15.7844694186245,-14.7979400799605,-13.8114107412964,
-12.8248814026324,-11.8383520639684,-10.8518227253043,-10.1357873115492),
 .UNSPECIFIED.);
#4359=B_SPLINE_CURVE_WITH_KNOTS('',3,(#59145,#59146,#59147,#59148,#59149,
#59150,#59151,#59152,#59153,#59154,#59155,#59156,#59157),.UNSPECIFIED.,
 .F.,.F.,(4,3,3,3,4),(-3.85260200436961,-2.95958801599209,-1.97305867732806,
-0.986529338664031,0.),.UNSPECIFIED.);
#4360=B_SPLINE_CURVE_WITH_KNOTS('',3,(#59160,#59161,#59162,#59163,#59164,
#59165,#59166,#59167,#59168,#59169,#59170,#59171,#59172,#59173,#59174,#59175,
#59176,#59177,#59178),.UNSPECIFIED.,.F.,.F.,(4,3,3,3,3,3,4),(2.02057249175691,
2.95958801599209,3.94611735465613,4.93264669332016,5.91917603198419,6.90570537064822,
7.59274844815668),.UNSPECIFIED.);
#4361=B_SPLINE_CURVE_WITH_KNOTS('',3,(#59184,#59185,#59186,#59187,#59188,
#59189,#59190,#59191),.UNSPECIFIED.,.F.,.F.,(4,1,1,1,1,4),(59.6902604182061,
60.1952988581168,61.1818281967808,62.1683575354449,63.1548868741089,64.1414162127729),
 .UNSPECIFIED.);
#4362=B_SPLINE_CURVE_WITH_KNOTS('',3,(#59194,#59195,#59196,#59197,#59198,
#59199,#59200,#59201,#59202),.UNSPECIFIED.,.F.,.F.,(4,1,1,1,1,1,4),(59.6902604182061,
59.7787497055172,60.7652790441813,61.7518083828453,62.7383377215093,63.7248670601734,
64.6638825844085),.UNSPECIFIED.);
#4363=B_SPLINE_CURVE_WITH_KNOTS('',3,(#59207,#59208,#59209,#59210,#59211,
#59212,#59213,#59214,#59215,#59216),.UNSPECIFIED.,.F.,.F.,(4,1,1,1,1,1,
1,4),(53.4070751110265,54.2761228261326,55.2626521647967,56.2491815034607,
57.2357108421247,58.2222401807888,59.2087695194528,59.6902604182061),
 .UNSPECIFIED.);
#4364=B_SPLINE_CURVE_WITH_KNOTS('',3,(#59217,#59218,#59219,#59220,#59221,
#59222,#59223,#59224,#59225,#59226),.UNSPECIFIED.,.F.,.F.,(4,1,1,1,1,1,
1,4),(53.4070751110265,53.8595736735331,54.8461030121971,55.8326323508611,
56.8191616895252,57.8056910281892,58.7922203668532,59.6902604182061),
 .UNSPECIFIED.);
#4365=B_SPLINE_CURVE_WITH_KNOTS('',3,(#59231,#59232,#59233,#59234,#59235,
#59236,#59237,#59238,#59239,#59240,#59241),.UNSPECIFIED.,.F.,.F.,(4,1,1,
1,1,1,1,1,4),(47.1238898038469,47.3704174554844,48.3569467941485,49.3434761328125,
50.3300054714765,51.3165348101405,52.3030641488046,53.2895934874686,53.4070751110265),
 .UNSPECIFIED.);
#4366=B_SPLINE_CURVE_WITH_KNOTS('',3,(#59242,#59243,#59244,#59245,#59246,
#59247,#59248,#59249,#59250,#59251),.UNSPECIFIED.,.F.,.F.,(4,1,1,1,1,1,
1,4),(47.1238898038469,47.9403976415489,48.9269269802129,49.9134563188769,
50.899985657541,51.886514996205,52.873044334869,53.4070751110265),
 .UNSPECIFIED.);
#4367=B_SPLINE_CURVE_WITH_KNOTS('',3,(#59256,#59257,#59258,#59259,#59260,
#59261,#59262,#59263,#59264,#59265),.UNSPECIFIED.,.F.,.F.,(4,1,1,1,1,1,
1,4),(40.8407044966673,41.4512414235002,42.4377707621643,43.4243001008283,
44.4108294394923,45.3973587781564,46.3838881168204,47.1238898038469),
 .UNSPECIFIED.);
#4368=B_SPLINE_CURVE_WITH_KNOTS('',3,(#59266,#59267,#59268,#59269,#59270,
#59271,#59272,#59273,#59274,#59275,#59276),.UNSPECIFIED.,.F.,.F.,(4,1,1,
1,1,1,1,1,4),(40.8407044966673,41.0346922709007,42.0212216095647,43.0077509482287,
43.9942802868927,44.9808096255568,45.9673389642208,46.9538683028848,47.1238898038469),
 .UNSPECIFIED.);
#4369=B_SPLINE_CURVE_WITH_KNOTS('',3,(#59281,#59282,#59283,#59284,#59285,
#59286,#59287,#59288,#59289,#59290),.UNSPECIFIED.,.F.,.F.,(4,1,1,1,1,1,
1,4),(34.5575191894877,35.5320653915161,36.5185947301801,37.5051240688441,
38.4916534075081,39.4781827461722,40.4647120848362,40.8407044966673),
 .UNSPECIFIED.);
#4370=B_SPLINE_CURVE_WITH_KNOTS('',3,(#59291,#59292,#59293,#59294,#59295,
#59296,#59297,#59298,#59299,#59300),.UNSPECIFIED.,.F.,.F.,(4,1,1,1,1,1,
1,4),(34.5575191894877,35.1155162389165,36.1020455775805,37.0885749162445,
38.0751042549086,39.0616335935726,40.0481629322366,40.8407044966673),
 .UNSPECIFIED.);
#4371=B_SPLINE_CURVE_WITH_KNOTS('',3,(#59305,#59306,#59307,#59308,#59309,
#59310,#59311,#59312,#59313,#59314,#59315),.UNSPECIFIED.,.F.,.F.,(4,1,1,
1,1,1,1,1,4),(28.2743338823081,28.6263600208678,29.6128893595319,30.5994186981959,
31.5859480368599,32.572477375524,33.559006714188,34.545536052852,34.5575191894877),
 .UNSPECIFIED.);
#4372=B_SPLINE_CURVE_WITH_KNOTS('',3,(#59316,#59317,#59318,#59319,#59320,
#59321,#59322,#59323,#59324,#59325),.UNSPECIFIED.,.F.,.F.,(4,1,1,1,1,1,
1,4),(28.2743338823081,29.1963402069323,30.1828695455963,31.1693988842603,
32.1559282229244,33.1424575615884,34.1289869002524,34.5575191894877),
 .UNSPECIFIED.);
#4373=B_SPLINE_CURVE_WITH_KNOTS('',3,(#59330,#59331,#59332,#59333,#59334,
#59335,#59336,#59337,#59338,#59339),.UNSPECIFIED.,.F.,.F.,(4,1,1,1,1,1,
1,4),(21.9911485751285,22.7071839888837,23.6937133275477,24.6802426662117,
25.6667720048757,26.6533013435398,27.6398306822038,28.2743338823081),
 .UNSPECIFIED.);
#4374=B_SPLINE_CURVE_WITH_KNOTS('',3,(#59340,#59341,#59342,#59343,#59344,
#59345,#59346,#59347,#59348,#59349,#59350),.UNSPECIFIED.,.F.,.F.,(4,1,1,
1,1,1,1,1,4),(21.9911485751285,22.2906348362841,23.2771641749481,24.2636935136121,
25.2502228522762,26.2367521909402,27.2232815296042,28.2098108682683,28.2743338823081),
 .UNSPECIFIED.);
#4375=B_SPLINE_CURVE_WITH_KNOTS('',3,(#59356,#59357,#59358,#59359,#59360),
 .UNSPECIFIED.,.F.,.F.,(4,1,4),(14.3984001269718,15.3849294656359,15.7079632679489),
 .UNSPECIFIED.);
#4376=B_SPLINE_CURVE_WITH_KNOTS('',3,(#59363,#59364,#59365,#59366,#59367),
 .UNSPECIFIED.,.F.,.F.,(4,1,4),(13.8759337553362,14.8149492795714,15.7079632679489),
 .UNSPECIFIED.);
#4377=B_SPLINE_CURVE_WITH_KNOTS('',3,(#59392,#59393,#59394,#59395,#59396,
#59397,#59398,#59399,#59400,#59401,#59402,#59403,#59404,#59405,#59406,#59407,
#59408,#59409,#59410,#59411,#59412,#59413,#59414,#59415,#59416,#59417,#59418,
#59419),.UNSPECIFIED.,.F.,.F.,(4,3,3,3,3,3,3,3,3,4),(-3.3351277338005,-3.21581204732697,
-2.97127448377657,-2.7269541692994,-2.48284991968139,-2.23896215435049,
-1.99538742760096,-1.75200286037067,-1.50889051064716,-1.38513595606351),
 .UNSPECIFIED.);
#4378=B_SPLINE_CURVE_WITH_KNOTS('',3,(#59427,#59428,#59429,#59430),
 .UNSPECIFIED.,.F.,.F.,(4,4),(-0.742759490140667,0.),.UNSPECIFIED.);
#4379=B_SPLINE_CURVE_WITH_KNOTS('',3,(#59440,#59441,#59442,#59443,#59444,
#59445,#59446,#59447,#59448,#59449,#59450,#59451,#59452,#59453,#59454,#59455,
#59456,#59457,#59458,#59459,#59460,#59461,#59462,#59463,#59464,#59465,#59466,
#59467),.UNSPECIFIED.,.F.,.F.,(4,3,3,3,3,3,3,3,3,4),(-3.33512774168352,
-3.21581203937105,-2.9712743901168,-2.72695409823512,-2.48284967780954,
-2.23896138594529,-1.99538662077021,-1.75200218102298,-1.50888981531756,
-1.38513595694967),.UNSPECIFIED.);
#4380=B_SPLINE_CURVE_WITH_KNOTS('',3,(#59475,#59476,#59477,#59478),
 .UNSPECIFIED.,.F.,.F.,(4,4),(-0.742759490382603,0.),.UNSPECIFIED.);
#4381=B_SPLINE_CURVE_WITH_KNOTS('',3,(#59488,#59489,#59490,#59491,#59492,
#59493,#59494,#59495,#59496,#59497,#59498,#59499,#59500,#59501,#59502,#59503,
#59504,#59505,#59506,#59507,#59508,#59509,#59510,#59511,#59512,#59513,#59514,
#59515),.UNSPECIFIED.,.F.,.F.,(4,3,3,3,3,3,3,3,3,4),(-3.33512773971227,
-3.21581201970404,-2.97127437729292,-2.72695395668863,-2.48284982134185,
-2.23896171731076,-1.99538699487002,-1.75200192521914,-1.50888988861517,
-1.38513595702442),.UNSPECIFIED.);
#4382=B_SPLINE_CURVE_WITH_KNOTS('',3,(#59523,#59524,#59525,#59526),
 .UNSPECIFIED.,.F.,.F.,(4,4),(-0.742759490770743,0.),.UNSPECIFIED.);
#4383=B_SPLINE_CURVE_WITH_KNOTS('',3,(#59536,#59537,#59538,#59539,#59540,
#59541),.UNSPECIFIED.,.F.,.F.,(4,2,4),(-3.33512774197138,-1.65413782257416,
-1.38513595763138),.UNSPECIFIED.);
#4384=B_SPLINE_CURVE_WITH_KNOTS('',3,(#59549,#59550,#59551,#59552),
 .UNSPECIFIED.,.F.,.F.,(4,4),(-0.742759491009937,0.),.UNSPECIFIED.);
#4385=B_SPLINE_CURVE_WITH_KNOTS('',3,(#59562,#59563,#59564,#59565,#59566,
#59567,#59568,#59569,#59570,#59571,#59572,#59573,#59574,#59575,#59576,#59577,
#59578,#59579,#59580,#59581,#59582,#59583,#59584,#59585,#59586,#59587,#59588,
#59589),.UNSPECIFIED.,.F.,.F.,(4,3,3,3,3,3,3,3,3,4),(-3.33512774327252,
-3.21581188244371,-2.97127402802938,-2.72695367771143,-2.48284924184614,
-2.23896121967729,-1.99538649326093,-1.75200210679088,-1.50888993573079,
-1.38513595840749),.UNSPECIFIED.);
#4386=B_SPLINE_CURVE_WITH_KNOTS('',3,(#59597,#59598,#59599,#59600),
 .UNSPECIFIED.,.F.,.F.,(4,4),(-0.742759490516493,0.),.UNSPECIFIED.);
#4387=B_SPLINE_CURVE_WITH_KNOTS('',3,(#59610,#59611,#59612,#59613,#59614,
#59615,#59616,#59617,#59618,#59619,#59620,#59621,#59622,#59623,#59624,#59625,
#59626,#59627,#59628,#59629,#59630,#59631,#59632,#59633,#59634,#59635,#59636,
#59637),.UNSPECIFIED.,.F.,.F.,(4,3,3,3,3,3,3,3,3,4),(-3.33512774337593,
-3.21581201730802,-2.97127431262814,-2.72695414046584,-2.48285027782337,
-2.2389618830467,-1.99538715953051,-1.7520020612767,-1.5088900089662,-1.38513595750991),
 .UNSPECIFIED.);
#4388=B_SPLINE_CURVE_WITH_KNOTS('',3,(#59645,#59646,#59647,#59648),
 .UNSPECIFIED.,.F.,.F.,(4,4),(-0.742759490399252,0.),.UNSPECIFIED.);
#4389=B_SPLINE_CURVE_WITH_KNOTS('',3,(#59656,#59657,#59658,#59659,#59660,
#59661,#59662,#59663,#59664,#59665,#59666,#59667,#59668,#59669,#59670,#59671,
#59672,#59673,#59674,#59675,#59676,#59677,#59678,#59679,#59680,#59681,#59682,
#59683,#59684,#59685,#59686,#59687,#59688,#59689,#59690,#59691,#59692,#59693,
#59694,#59695,#59696,#59697,#59698,#59699,#59700,#59701,#59702,#59703,#59704,
#59705,#59706,#59707,#59708,#59709,#59710,#59711,#59712,#59713,#59714,#59715,
#59716,#59717,#59718,#59719,#59720,#59721,#59722,#59723,#59724,#59725,#59726,
#59727,#59728,#59729,#59730,#59731,#59732,#59733,#59734),.UNSPECIFIED.,
 .F.,.F.,(4,3,3,3,3,3,3,3,3,3,3,3,3,3,3,3,3,3,3,3,3,3,3,3,3,3,4),(0.,0.0183455177171488,
0.0365842194687939,0.0503567097523435,0.0575063938651825,0.0612717135192181,
0.0790233191281566,0.096412403715043,0.10900033822058,0.115579427932303,
0.11863915864875,0.13548956751629,0.14676414173719,0.163451454243383,0.168605352621408,
0.173128046239674,0.189898672554047,0.206649133260606,0.217355581880073,
0.222872485157851,0.226199941445228,0.2422909706325,0.252395568311884,0.256090122700147,
0.271598926188493,0.280262641786736,0.286347380332249),.UNSPECIFIED.);
#4390=B_SPLINE_CURVE_WITH_KNOTS('',3,(#59735,#59736,#59737,#59738,#59739,
#59740,#59741,#59742,#59743,#59744,#59745,#59746,#59747,#59748,#59749,#59750,
#59751,#59752,#59753,#59754,#59755,#59756,#59757,#59758,#59759,#59760,#59761,
#59762,#59763,#59764,#59765,#59766,#59767,#59768,#59769,#59770,#59771,#59772,
#59773,#59774,#59775,#59776,#59777,#59778,#59779,#59780,#59781,#59782,#59783,
#59784,#59785,#59786,#59787,#59788,#59789,#59790,#59791,#59792,#59793,#59794,
#59795,#59796,#59797,#59798,#59799,#59800,#59801,#59802,#59803,#59804,#59805,
#59806,#59807,#59808,#59809,#59810,#59811,#59812,#59813,#59814,#59815,#59816),
 .UNSPECIFIED.,.F.,.F.,(4,3,3,3,3,3,3,3,3,3,3,3,3,3,3,3,3,3,3,3,3,3,3,3,
3,3,3,4),(0.,0.0151376945523622,0.0309539555233482,0.0436386424985849,0.049000547090806,
0.0520439606424598,0.0683447111906178,0.0849441791722525,0.0968159972104999,
0.101863070537586,0.10487005785608,0.121945783028775,0.132431451325242,
0.149057557666816,0.154031803331322,0.158630806444058,0.175669023659517,
0.193110008838669,0.203698775422856,0.209528903797298,0.213039490372793,
0.231030287351627,0.242727750891762,0.247562329943512,0.251101657049746,
0.269297746623456,0.277820141512166,0.285142803995177),.UNSPECIFIED.);
#4391=B_SPLINE_CURVE_WITH_KNOTS('',3,(#59818,#59819,#59820,#59821,#59822,
#59823,#59824,#59825,#59826,#59827,#59828,#59829,#59830,#59831,#59832,#59833,
#59834,#59835,#59836,#59837,#59838,#59839,#59840,#59841,#59842,#59843,#59844,
#59845,#59846,#59847,#59848,#59849,#59850,#59851,#59852,#59853,#59854,#59855,
#59856,#59857,#59858,#59859,#59860,#59861,#59862,#59863,#59864,#59865,#59866,
#59867,#59868,#59869,#59870,#59871,#59872,#59873,#59874,#59875,#59876,#59877,
#59878,#59879,#59880,#59881,#59882,#59883,#59884,#59885,#59886,#59887,#59888,
#59889,#59890,#59891,#59892,#59893,#59894,#59895,#59896),.UNSPECIFIED.,
 .F.,.F.,(4,3,3,3,3,3,3,3,3,3,3,3,3,3,3,3,3,3,3,3,3,3,3,3,3,3,4),(0.,0.0183455177171464,
0.0365842202218134,0.0503567104112331,0.0575063958814502,0.0612717147976262,
0.0790233202990436,0.096412400821268,0.109000336050244,0.115579427690159,
0.11863915902179,0.135489564068242,0.146764141737171,0.163451454243363,
0.168605347203144,0.173128047807504,0.189898674519216,0.206649134734921,
0.217355586796981,0.222872485969177,0.226199940772131,0.24229096629471,
0.252395560905716,0.256090108931784,0.271598906474471,0.280262641786705,
0.286347380332217),.UNSPECIFIED.);
#4392=B_SPLINE_CURVE_WITH_KNOTS('',3,(#59897,#59898,#59899,#59900,#59901,
#59902,#59903,#59904,#59905,#59906,#59907,#59908,#59909,#59910,#59911,#59912,
#59913,#59914,#59915,#59916,#59917,#59918,#59919,#59920,#59921,#59922,#59923,
#59924,#59925,#59926,#59927,#59928,#59929,#59930,#59931,#59932,#59933,#59934,
#59935,#59936,#59937,#59938,#59939,#59940,#59941,#59942,#59943,#59944,#59945,
#59946,#59947,#59948,#59949,#59950,#59951,#59952,#59953,#59954,#59955,#59956,
#59957,#59958,#59959,#59960,#59961,#59962,#59963,#59964,#59965,#59966,#59967,
#59968,#59969,#59970,#59971,#59972,#59973,#59974,#59975,#59976,#59977,#59978),
 .UNSPECIFIED.,.F.,.F.,(4,3,3,3,3,3,3,3,3,3,3,3,3,3,3,3,3,3,3,3,3,3,3,3,
3,3,3,4),(0.,0.0151377073331275,0.0309539773939491,0.0436386616353583,0.049000603702908,
0.0520439678481244,0.068344727340715,0.0849441979341871,0.0968160112819461,
0.101863110224252,0.104870125248596,0.121945848980836,0.132431451325223,
0.149057551294161,0.154031802130475,0.158630806791255,0.175669017059408,
0.193109999022821,0.203698766833983,0.209528894188178,0.213039481192876,
0.231030277572612,0.242727743557488,0.24756230355572,0.251101629527168,
0.26929771945885,0.277820141512119,0.285142803995128),.UNSPECIFIED.);
#4393=B_SPLINE_CURVE_WITH_KNOTS('',3,(#59979,#59980,#59981,#59982,#59983,
#59984,#59985,#59986,#59987,#59988,#59989,#59990,#59991,#59992,#59993,#59994,
#59995,#59996,#59997,#59998,#59999,#60000,#60001,#60002,#60003,#60004,#60005,
#60006,#60007,#60008,#60009,#60010,#60011,#60012,#60013,#60014,#60015,#60016,
#60017,#60018,#60019,#60020,#60021,#60022,#60023,#60024,#60025,#60026,#60027,
#60028,#60029,#60030,#60031,#60032,#60033,#60034,#60035,#60036,#60037,#60038,
#60039,#60040,#60041,#60042,#60043,#60044,#60045,#60046,#60047,#60048,#60049,
#60050,#60051,#60052,#60053,#60054,#60055,#60056,#60057),.UNSPECIFIED.,
 .F.,.F.,(4,3,3,3,3,3,3,3,3,3,3,3,3,3,3,3,3,3,3,3,3,3,3,3,3,3,4),(0.,0.0183455177171491,
0.0365841943725053,0.0503566877930912,0.0575063272586958,0.0612716713524759,
0.0790232799247667,0.0964124964716688,0.10900040778805,0.115579434178192,
0.118639143887527,0.135489676819533,0.146764141737193,0.163451454243384,
0.168605528191993,0.173127995302464,0.189898608413707,0.206649084167343,
0.217355422796664,0.222872458887097,0.226199963177961,0.24229110995885,
0.252395806920558,0.256090567682751,0.27159956261746,0.280262641786727,
0.28634738033224),.UNSPECIFIED.);
#4394=B_SPLINE_CURVE_WITH_KNOTS('',3,(#60058,#60059,#60060,#60061,#60062,
#60063,#60064,#60065,#60066,#60067,#60068,#60069,#60070,#60071,#60072,#60073,
#60074,#60075,#60076,#60077,#60078,#60079,#60080,#60081,#60082,#60083,#60084,
#60085,#60086,#60087,#60088,#60089,#60090,#60091,#60092,#60093,#60094,#60095,
#60096,#60097,#60098,#60099,#60100,#60101,#60102,#60103,#60104,#60105,#60106,
#60107,#60108,#60109,#60110,#60111,#60112,#60113,#60114,#60115,#60116,#60117,
#60118,#60119,#60120,#60121,#60122,#60123,#60124,#60125,#60126,#60127,#60128,
#60129,#60130,#60131,#60132,#60133,#60134,#60135,#60136,#60137,#60138,#60139),
 .UNSPECIFIED.,.F.,.F.,(4,3,3,3,3,3,3,3,3,3,3,3,3,3,3,3,3,3,3,3,3,3,3,3,
3,3,3,4),(0.,0.0151372184044385,0.0309531403735887,0.043637929242543,0.0489984376247301,
0.0520436975026237,0.0683441145647309,0.0849434845410623,0.0968154762371025,
0.10186160092259,0.10486756751019,0.121943345305763,0.132431451325223,0.149057794056237,
0.154031847028422,0.158630793802344,0.175669268709996,0.193110373371059,
0.203699094388695,0.209529259612817,0.213039830397245,0.231030649717207,
0.242728022665942,0.247563307937232,0.251102678589767,0.269298754560415,
0.277820141512145,0.285142803995156),.UNSPECIFIED.);
#4395=B_SPLINE_CURVE_WITH_KNOTS('',3,(#60140,#60141,#60142,#60143,#60144,
#60145,#60146,#60147,#60148,#60149,#60150,#60151,#60152,#60153,#60154,#60155,
#60156,#60157,#60158,#60159,#60160,#60161,#60162,#60163,#60164,#60165,#60166,
#60167,#60168,#60169,#60170,#60171,#60172,#60173,#60174,#60175,#60176,#60177,
#60178,#60179,#60180,#60181,#60182,#60183,#60184,#60185,#60186,#60187,#60188,
#60189,#60190,#60191,#60192,#60193,#60194,#60195,#60196,#60197,#60198,#60199,
#60200,#60201,#60202,#60203,#60204,#60205,#60206,#60207,#60208,#60209,#60210,
#60211,#60212,#60213,#60214,#60215,#60216,#60217,#60218),.UNSPECIFIED.,
 .F.,.F.,(4,3,3,3,3,3,3,3,3,3,3,3,3,3,3,3,3,3,3,3,3,3,3,3,3,3,4),(0.,0.0183455177171496,
0.0365842194687423,0.0503567097522991,0.0575063938651049,0.0612717135166192,
0.0790233191256915,0.0964124037125833,0.109000338218737,0.115579427930349,
0.118639158644869,0.13548956751248,0.146764141737196,0.163451454243393,
0.16860535262136,0.173128046238754,0.189898672553141,0.206649133259799,
0.21735558187922,0.222872485156807,0.226199941447941,0.242290970635022,
0.252395568315028,0.256090122699954,0.271598926188319,0.280262641786767,
0.286347380332284),.UNSPECIFIED.);
#4396=B_SPLINE_CURVE_WITH_KNOTS('',3,(#60219,#60220,#60221,#60222,#60223,
#60224,#60225,#60226,#60227,#60228,#60229,#60230,#60231,#60232,#60233,#60234,
#60235,#60236,#60237,#60238,#60239,#60240,#60241,#60242,#60243,#60244,#60245,
#60246,#60247,#60248,#60249,#60250,#60251,#60252,#60253,#60254,#60255,#60256,
#60257,#60258,#60259,#60260,#60261,#60262,#60263,#60264,#60265,#60266,#60267,
#60268,#60269,#60270,#60271,#60272,#60273,#60274,#60275,#60276,#60277,#60278,
#60279,#60280,#60281,#60282,#60283,#60284,#60285,#60286,#60287,#60288,#60289,
#60290,#60291,#60292,#60293,#60294,#60295,#60296,#60297,#60298,#60299,#60300),
 .UNSPECIFIED.,.F.,.F.,(4,3,3,3,3,3,3,3,3,3,3,3,3,3,3,3,3,3,3,3,3,3,3,3,
3,3,3,4),(0.,0.015137694552346,0.0309539555233422,0.0436386424985786,0.0490005470908032,
0.052043960644431,0.068344711192548,0.0849441791741085,0.0968159972118898,
0.101863070541411,0.104870057863348,0.121945783035943,0.132431451325233,
0.149057557666585,0.154031803331171,0.158630806444046,0.175669023659537,
0.193110008838639,0.203698775422825,0.209528903797183,0.213039490371705,
0.231030287350353,0.242727750890797,0.24756232993717,0.251101657039408,
0.26929774661335,0.277820141512129,0.285142803995137),.UNSPECIFIED.);
#4397=B_SPLINE_CURVE_WITH_KNOTS('',3,(#60301,#60302,#60303,#60304,#60305,
#60306,#60307,#60308,#60309,#60310,#60311,#60312,#60313,#60314,#60315,#60316,
#60317,#60318,#60319,#60320,#60321,#60322,#60323,#60324,#60325,#60326,#60327,
#60328,#60329,#60330,#60331,#60332,#60333,#60334,#60335,#60336,#60337,#60338,
#60339,#60340,#60341,#60342,#60343,#60344,#60345,#60346,#60347,#60348,#60349,
#60350,#60351,#60352,#60353,#60354,#60355,#60356,#60357,#60358,#60359,#60360,
#60361,#60362,#60363,#60364,#60365,#60366,#60367,#60368,#60369,#60370,#60371,
#60372,#60373,#60374,#60375,#60376,#60377,#60378,#60379),.UNSPECIFIED.,
 .F.,.F.,(4,3,3,3,3,3,3,3,3,3,3,3,3,3,3,3,3,3,3,3,3,3,3,3,3,3,4),(0.,0.0183455177171492,
0.0365842202217887,0.0503567104112144,0.0575063958813968,0.0612717147969415,
0.0790233202984323,0.0964124008207027,0.109000336049826,0.115579427689752,
0.118639159024108,0.135489564070542,0.146764141737194,0.163451454243389,
0.168605347203302,0.173128047809237,0.189898674521018,0.206649134736986,
0.217355586794765,0.222872485965579,0.226199940772176,0.242290966294427,
0.252395560905467,0.256090108929053,0.271598906471585,0.280262641786756,
0.286347380332274),.UNSPECIFIED.);
#4398=B_SPLINE_CURVE_WITH_KNOTS('',3,(#60380,#60381,#60382,#60383,#60384,
#60385,#60386,#60387,#60388,#60389,#60390,#60391,#60392,#60393,#60394,#60395,
#60396,#60397,#60398,#60399,#60400,#60401,#60402,#60403,#60404,#60405,#60406,
#60407,#60408,#60409,#60410,#60411,#60412,#60413,#60414,#60415,#60416,#60417,
#60418,#60419,#60420,#60421,#60422,#60423,#60424,#60425,#60426,#60427,#60428,
#60429,#60430,#60431,#60432,#60433,#60434,#60435,#60436,#60437,#60438,#60439,
#60440,#60441,#60442,#60443,#60444,#60445,#60446,#60447,#60448,#60449,#60450,
#60451,#60452,#60453,#60454,#60455,#60456,#60457,#60458,#60459,#60460,#60461),
 .UNSPECIFIED.,.F.,.F.,(4,3,3,3,3,3,3,3,3,3,3,3,3,3,3,3,3,3,3,3,3,3,3,3,
3,3,3,4),(0.,0.0151377073334981,0.0309539773942999,0.0436386616356645,0.0490006037038296,
0.0520439678487852,0.0683447273416009,0.0849441979349755,0.0968160112825359,
0.101863110225754,0.104870125256082,0.121945848988211,0.132431451325217,
0.149057551294131,0.154031802130417,0.158630806785895,0.1756690170539,0.193109999017219,
0.203698766829082,0.209528894184026,0.213039481197191,0.231030277576794,
0.242727743560627,0.247562303564317,0.251101629536978,0.269297719468806,
0.277820141512128,0.285142803995138),.UNSPECIFIED.);
#4399=B_SPLINE_CURVE_WITH_KNOTS('',3,(#60462,#60463,#60464,#60465,#60466,
#60467,#60468,#60469,#60470,#60471,#60472,#60473,#60474,#60475,#60476,#60477,
#60478,#60479,#60480,#60481,#60482,#60483,#60484,#60485,#60486,#60487,#60488,
#60489,#60490,#60491,#60492,#60493,#60494,#60495,#60496,#60497,#60498,#60499,
#60500,#60501,#60502,#60503,#60504,#60505,#60506,#60507,#60508,#60509,#60510,
#60511,#60512,#60513,#60514,#60515,#60516,#60517,#60518,#60519,#60520,#60521,
#60522,#60523,#60524,#60525,#60526,#60527,#60528,#60529,#60530,#60531,#60532,
#60533,#60534,#60535,#60536,#60537,#60538,#60539,#60540),.UNSPECIFIED.,
 .F.,.F.,(4,3,3,3,3,3,3,3,3,3,3,3,3,3,3,3,3,3,3,3,3,3,3,3,3,3,4),(0.,0.018345517717149,
0.0365841943724813,0.0503566877930701,0.057506327258564,0.0612716713518624,
0.079023279923942,0.0964124964708253,0.109000407787417,0.115579434177528,
0.118639143891469,0.135489676823446,0.146764141737192,0.163451454243385,
0.168605528191884,0.173127995305518,0.189898608416791,0.206649084170442,
0.21735542279444,0.222872458884167,0.226199963170307,0.242291109951151,
0.252395806910312,0.256090567650659,0.271599562585826,0.280262641786738,
0.286347380332254),.UNSPECIFIED.);
#4400=B_SPLINE_CURVE_WITH_KNOTS('',3,(#60541,#60542,#60543,#60544,#60545,
#60546,#60547,#60548,#60549,#60550,#60551,#60552,#60553,#60554,#60555,#60556,
#60557,#60558,#60559,#60560,#60561,#60562,#60563,#60564,#60565,#60566,#60567,
#60568,#60569,#60570,#60571,#60572,#60573,#60574,#60575,#60576,#60577,#60578,
#60579,#60580,#60581,#60582,#60583,#60584,#60585,#60586,#60587,#60588,#60589,
#60590,#60591,#60592,#60593,#60594,#60595,#60596,#60597,#60598,#60599,#60600,
#60601,#60602,#60603,#60604,#60605,#60606,#60607,#60608,#60609,#60610,#60611,
#60612,#60613,#60614,#60615,#60616,#60617,#60618,#60619,#60620,#60621,#60622),
 .UNSPECIFIED.,.F.,.F.,(4,3,3,3,3,3,3,3,3,3,3,3,3,3,3,3,3,3,3,3,3,3,3,3,
3,3,3,4),(0.,0.0151372184042629,0.0309531403734452,0.0436379292424174,0.0489984376244327,
0.0520436974965136,0.068344114558214,0.0849434845342685,0.0968154762320069,
0.101861600908548,0.104867567483352,0.121943345279016,0.132431451325222,
0.149057794056487,0.15403184702849,0.158630793803121,0.175669268710828,
0.193110373371818,0.203699094389356,0.209529259613411,0.213039830390277,
0.23103064971016,0.242728022660651,0.247563307922767,0.251102678572032,
0.26929875454266,0.277820141512126,0.285142803995136),.UNSPECIFIED.);
#4401=B_SPLINE_CURVE_WITH_KNOTS('',3,(#60624,#60625,#60626,#60627,#60628,
#60629,#60630,#60631,#60632,#60633,#60634,#60635,#60636,#60637,#60638,#60639,
#60640,#60641,#60642,#60643,#60644,#60645,#60646,#60647,#60648,#60649,#60650,
#60651,#60652,#60653,#60654,#60655,#60656,#60657,#60658,#60659,#60660,#60661,
#60662,#60663,#60664,#60665,#60666,#60667,#60668,#60669,#60670,#60671,#60672,
#60673,#60674,#60675,#60676,#60677,#60678,#60679,#60680,#60681,#60682,#60683,
#60684,#60685,#60686,#60687,#60688,#60689,#60690,#60691,#60692,#60693,#60694,
#60695,#60696,#60697,#60698,#60699,#60700,#60701,#60702,#60703,#60704,#60705),
 .UNSPECIFIED.,.F.,.F.,(4,3,3,3,3,3,3,3,3,3,3,3,3,3,3,3,3,3,3,3,3,3,3,3,
3,3,3,4),(-0.286347380332265,-0.271025621689181,-0.2607001267017,-0.255933999919549,
-0.251928786217061,-0.235739770681133,-0.229543552625755,-0.225090694889911,
-0.221644284966547,-0.204610638152085,-0.187823738644011,-0.179057759822907,
-0.17435510384889,-0.171011960015997,-0.168068908456346,-0.153509697708698,
-0.136938545278062,-0.120740430888098,-0.116772838424861,-0.113777170632241,
-0.0964534278367324,-0.0787580645164197,-0.0609069559269026,-0.0568632900112524,
-0.0386443178831796,-0.0205854755521028,-0.00735363015835137,0.),
 .UNSPECIFIED.);
#4402=B_SPLINE_CURVE_WITH_KNOTS('',3,(#60706,#60707,#60708,#60709,#60710,
#60711,#60712,#60713,#60714,#60715,#60716,#60717,#60718,#60719,#60720,#60721,
#60722,#60723,#60724,#60725,#60726,#60727,#60728,#60729,#60730,#60731,#60732,
#60733,#60734,#60735,#60736,#60737,#60738,#60739,#60740,#60741,#60742,#60743,
#60744,#60745,#60746,#60747,#60748,#60749,#60750,#60751,#60752,#60753,#60754,
#60755,#60756,#60757,#60758,#60759,#60760,#60761,#60762,#60763,#60764,#60765,
#60766,#60767,#60768,#60769,#60770,#60771,#60772,#60773,#60774,#60775,#60776,
#60777,#60778,#60779,#60780,#60781),.UNSPECIFIED.,.F.,.F.,(4,3,3,3,3,3,
3,3,3,3,3,3,3,3,3,3,3,3,3,3,3,3,3,3,3,4),(-0.285142803995153,-0.266893522635859,
-0.249971640311975,-0.245887155067402,-0.227911309461469,-0.216815964918886,
-0.213019369676792,-0.209467693445812,-0.19188790836456,-0.174756961586316,
-0.165469070515125,-0.157741742341544,-0.154438844453031,-0.139148553120806,
-0.122062040548429,-0.107562425207839,-0.103576093458224,-0.100472602942305,
-0.0838658643924183,-0.067352053952836,-0.0520303199205553,-0.0480946799675465,
-0.0321859944606069,-0.0168167950639115,-0.00606511782371307,0.),
 .UNSPECIFIED.);
#4403=B_SPLINE_CURVE_WITH_KNOTS('',3,(#60783,#60784,#60785,#60786,#60787,
#60788,#60789,#60790,#60791,#60792,#60793),.UNSPECIFIED.,.F.,.F.,(4,1,1,
1,1,1,1,1,4),(15.7079632679489,15.8014786182354,16.7880079568995,17.7745372955635,
18.7610666342275,19.7475959728916,20.7341253115556,21.7206546502196,21.9911485751285),
 .UNSPECIFIED.);
#4404=B_SPLINE_CURVE_WITH_KNOTS('',3,(#60794,#60795,#60796,#60797,#60798,
#60799,#60800,#60801,#60802,#60803),.UNSPECIFIED.,.F.,.F.,(4,1,1,1,1,1,
1,4),(15.7079632679489,16.3714588042999,17.3579881429639,18.3445174816279,
19.331046820292,20.317576158956,21.30410549762,21.9911485751285),
 .UNSPECIFIED.);
#4405=B_SPLINE_CURVE_WITH_KNOTS('',3,(#61028,#61029,#61030,#61031,#61032,
#61033,#61034,#61035,#61036,#61037,#61038,#61039,#61040,#61041,#61042,#61043,
#61044,#61045,#61046,#61047,#61048,#61049,#61050,#61051,#61052,#61053,#61054,
#61055,#61056,#61057,#61058,#61059,#61060,#61061,#61062,#61063,#61064,#61065,
#61066,#61067,#61068,#61069,#61070,#61071,#61072,#61073,#61074,#61075,#61076,
#61077,#61078,#61079,#61080,#61081,#61082,#61083,#61084,#61085,#61086,#61087,
#61088,#61089,#61090,#61091,#61092,#61093,#61094,#61095,#61096,#61097,#61098,
#61099,#61100,#61101,#61102,#61103,#61104,#61105,#61106,#61107,#61108,#61109),
 .UNSPECIFIED.,.F.,.F.,(4,3,3,3,3,3,3,3,3,3,3,3,3,3,3,3,3,3,3,3,3,3,3,3,
3,3,3,4),(0.,0.015137799248671,0.0309541346648961,0.0436387992474388,0.0490010108224065,
0.0520440199058781,0.0683448437142619,0.0849443330626919,0.0968161126283283,
0.101863396045917,0.104870610850094,0.121946324179646,0.132431451325237,
0.149057505425983,0.154031793452878,0.158630809285983,0.175668969545569,
0.193109928370158,0.203698705012908,0.209528824985022,0.213039415113619,
0.231030207185071,0.242727690766841,0.247562113630917,0.251101431476904,
0.269297523974363,0.277820141512152,0.285142803995165),.UNSPECIFIED.);
#4406=B_SPLINE_CURVE_WITH_KNOTS('',3,(#61110,#61111,#61112,#61113,#61114,
#61115,#61116,#61117,#61118,#61119,#61120,#61121,#61122,#61123,#61124,#61125,
#61126,#61127,#61128,#61129,#61130,#61131,#61132,#61133,#61134),
 .UNSPECIFIED.,.F.,.F.,(4,3,3,3,3,3,3,3,4),(-10.1357873115492,-9.86529338664031,
-8.87876404797627,-7.89223470931224,-6.90570537064822,-5.91917603198418,
-4.93264669332015,-3.94611735465612,-3.85260200436961),.UNSPECIFIED.);
#4407=B_SPLINE_CURVE_WITH_KNOTS('',3,(#61359,#61360,#61361,#61362,#61363,
#61364,#61365,#61366,#61367,#61368,#61369,#61370,#61371,#61372,#61373,#61374,
#61375,#61376,#61377,#61378,#61379,#61380,#61381,#61382,#61383),
 .UNSPECIFIED.,.F.,.F.,(4,3,3,3,3,3,3,3,4),(7.59274844815668,7.89223470931225,
8.87876404797628,9.86529338664031,10.8518227253043,11.8383520639684,12.8248814026324,
13.8114107412964,13.8759337553363),.UNSPECIFIED.);
#4408=B_SPLINE_CURVE_WITH_KNOTS('',3,(#61384,#61385,#61386,#61387,#61388,
#61389,#61390,#61391,#61392,#61393,#61394,#61395,#61396,#61397,#61398,#61399,
#61400,#61401,#61402,#61403,#61404,#61405,#61406,#61407,#61408,#61409,#61410,
#61411,#61412,#61413,#61414,#61415,#61416,#61417,#61418,#61419,#61420,#61421,
#61422,#61423,#61424,#61425,#61426,#61427,#61428,#61429,#61430,#61431,#61432,
#61433,#61434,#61435,#61436,#61437,#61438,#61439,#61440,#61441,#61442,#61443,
#61444,#61445,#61446,#61447,#61448,#61449,#61450,#61451,#61452,#61453,#61454,
#61455,#61456,#61457,#61458,#61459,#61460,#61461,#61462),.UNSPECIFIED.,
 .F.,.F.,(4,3,3,3,3,3,3,3,3,3,3,3,3,3,3,3,3,3,3,3,3,3,3,3,3,3,4),(0.,0.0183455177171469,
0.0365842224515149,0.0503567123622224,0.0575064018579709,0.0612717186027069,
0.0790233237781577,0.0964123922275627,0.109000329604966,0.115579426964778,
0.118639160106121,0.135489553802985,0.146764141737175,0.16345145424337,
0.16860533110635,0.173128052468331,0.189898680357127,0.206649139105657,
0.217355601404692,0.2228724883745,0.226199938776673,0.242290953398615,0.252395538894453,
0.256090068020206,0.271598847885511,0.280262641786736,0.286347380332253),
 .UNSPECIFIED.);
#4409=B_SPLINE_CURVE_WITH_KNOTS('',3,(#61465,#61466,#61467,#61468,#61469,
#61470,#61471,#61472,#61473,#61474,#61475,#61476,#61477,#61478,#61479,#61480,
#61481,#61482,#61483,#61484,#61485,#61486,#61487,#61488,#61489,#61490,#61491,
#61492,#61493,#61494,#61495,#61496,#61497,#61498,#61499,#61500,#61501,#61502,
#61503,#61504,#61505,#61506,#61507,#61508,#61509,#61510,#61511,#61512,#61513,
#61514,#61515,#61516,#61517,#61518,#61519,#61520,#61521,#61522,#61523,#61524,
#61525,#61526,#61527,#61528,#61529,#61530,#61531,#61532,#61533,#61534,#61535,
#61536,#61537,#61538,#61539,#61540,#61541,#61542,#61543,#61544,#61545,#61546),
 .UNSPECIFIED.,.F.,.F.,(4,3,3,3,3,3,3,3,3,3,3,3,3,3,3,3,3,3,3,3,3,3,3,3,
3,3,3,4),(-0.286347380332235,-0.271025121721878,-0.260698471407634,-0.255927424635191,
-0.251928101931866,-0.235738748722702,-0.229541533305995,-0.225083562731207,
-0.221641685050275,-0.204608688214882,-0.187821861453013,-0.179056467789758,
-0.17435297386637,-0.171008268443927,-0.168068104867454,-0.153509697708701,
-0.136938887237132,-0.120740730102284,-0.116774494101265,-0.113778981555512,
-0.0964555421171121,-0.0787603000996159,-0.0609086326142997,-0.0568635712073007,
-0.0386446475024485,-0.0205858121909903,-0.00735363015835102,0.),
 .UNSPECIFIED.);
#4410=B_SPLINE_CURVE_WITH_KNOTS('',3,(#61547,#61548,#61549,#61550,#61551,
#61552,#61553,#61554,#61555,#61556,#61557,#61558,#61559,#61560,#61561,#61562,
#61563,#61564,#61565,#61566,#61567,#61568,#61569,#61570,#61571,#61572,#61573,
#61574,#61575,#61576,#61577,#61578,#61579,#61580,#61581,#61582,#61583,#61584,
#61585,#61586,#61587,#61588,#61589,#61590,#61591,#61592,#61593,#61594,#61595,
#61596,#61597,#61598,#61599,#61600,#61601,#61602,#61603,#61604,#61605,#61606,
#61607,#61608,#61609,#61610,#61611,#61612,#61613,#61614,#61615,#61616,#61617,
#61618,#61619,#61620,#61621,#61622),.UNSPECIFIED.,.F.,.F.,(4,3,3,3,3,3,
3,3,3,3,3,3,3,3,3,3,3,3,3,3,3,3,3,3,3,4),(-0.285142803995111,-0.266893522635822,
-0.249971476962298,-0.24588710473722,-0.22791128063125,-0.216815939692444,
-0.213019163167601,-0.209467643672605,-0.191887871034653,-0.174757065702234,
-0.165469235776541,-0.157741962735036,-0.154438808545209,-0.139148553120797,
-0.122062022789849,-0.107562409669082,-0.103576180068673,-0.100472613982929,
-0.0838658564336281,-0.0673520878880563,-0.0520303453719698,-0.0480947095105707,
-0.0321861105599142,-0.0168171759222756,-0.0060651178237103,0.),
 .UNSPECIFIED.);
#4411=B_SPLINE_CURVE_WITH_KNOTS('',3,(#61624,#61625,#61626,#61627,#61628,
#61629,#61630,#61631,#61632,#61633,#61634),.UNSPECIFIED.,.F.,.F.,(4,1,1,
1,1,1,1,1,4),(15.7079632679489,15.8014786182355,16.7880079568995,17.7745372955635,
18.7610666342275,19.7475959728916,20.7341253115556,21.7206546502196,21.9911485751285),
 .UNSPECIFIED.);
#4412=B_SPLINE_CURVE_WITH_KNOTS('',3,(#61635,#61636,#61637,#61638,#61639,
#61640,#61641,#61642,#61643,#61644),.UNSPECIFIED.,.F.,.F.,(4,1,1,1,1,1,
1,4),(15.7079632679489,16.3714588042999,17.3579881429639,18.344517481628,
19.331046820292,20.317576158956,21.3041054976201,21.9911485751285),
 .UNSPECIFIED.);
#4413=B_SPLINE_CURVE_WITH_KNOTS('',3,(#61869,#61870,#61871,#61872,#61873,
#61874,#61875,#61876,#61877,#61878,#61879,#61880,#61881,#61882,#61883,#61884,
#61885,#61886,#61887,#61888,#61889,#61890,#61891,#61892,#61893,#61894,#61895,
#61896,#61897,#61898,#61899,#61900,#61901,#61902,#61903,#61904,#61905,#61906,
#61907,#61908,#61909,#61910,#61911,#61912,#61913,#61914,#61915,#61916,#61917,
#61918,#61919,#61920,#61921,#61922,#61923,#61924,#61925,#61926,#61927,#61928,
#61929,#61930,#61931,#61932,#61933,#61934,#61935,#61936,#61937,#61938,#61939,
#61940,#61941,#61942,#61943,#61944,#61945,#61946,#61947,#61948,#61949,#61950),
 .UNSPECIFIED.,.F.,.F.,(4,3,3,3,3,3,3,3,3,3,3,3,3,3,3,3,3,3,3,3,3,3,3,3,
3,3,3,4),(0.,0.0151383248854633,0.0309550335466972,0.0436395857690147,0.0490033384906151,
0.0520443250916062,0.0683455163450802,0.084945111984634,0.0968166968197849,
0.101865043241974,0.10487341705618,0.121949069466398,0.132431451325238,
0.14905724175649,0.154031742415311,0.158630823850449,0.17566869659654,0.193109522683113,
0.203698350036742,0.209528426219277,0.213039034676904,0.231029802154963,
0.242727386994258,0.247561020935096,0.251100294233131,0.269296401038409,
0.277820141512142,0.285142803995154),.UNSPECIFIED.);
#4414=B_SPLINE_CURVE_WITH_KNOTS('',3,(#61951,#61952,#61953,#61954,#61955,
#61956,#61957,#61958,#61959,#61960,#61961,#61962,#61963,#61964,#61965,#61966,
#61967,#61968,#61969,#61970,#61971,#61972,#61973,#61974,#61975),
 .UNSPECIFIED.,.F.,.F.,(4,3,3,3,3,3,3,3,4),(-10.1357873115492,-9.86529338664031,
-8.87876404797628,-7.89223470931225,-6.90570537064822,-5.91917603198419,
-4.93264669332016,-3.94611735465612,-3.85260200436962),.UNSPECIFIED.);
#4415=B_SPLINE_CURVE_WITH_KNOTS('',3,(#62200,#62201,#62202,#62203,#62204,
#62205,#62206,#62207,#62208,#62209,#62210,#62211,#62212,#62213,#62214,#62215,
#62216,#62217,#62218,#62219,#62220,#62221,#62222,#62223,#62224),
 .UNSPECIFIED.,.F.,.F.,(4,3,3,3,3,3,3,3,4),(7.59274844815668,7.89223470931225,
8.87876404797628,9.86529338664031,10.8518227253043,11.8383520639684,12.8248814026324,
13.8114107412964,13.8759337553363),.UNSPECIFIED.);
#4416=B_SPLINE_CURVE_WITH_KNOTS('',3,(#62225,#62226,#62227,#62228,#62229,
#62230,#62231,#62232,#62233,#62234,#62235,#62236,#62237,#62238,#62239,#62240,
#62241,#62242,#62243,#62244,#62245,#62246,#62247,#62248,#62249,#62250,#62251,
#62252,#62253,#62254,#62255,#62256,#62257,#62258,#62259,#62260,#62261,#62262,
#62263,#62264,#62265,#62266,#62267,#62268,#62269,#62270,#62271,#62272,#62273,
#62274,#62275,#62276,#62277,#62278,#62279,#62280,#62281,#62282,#62283,#62284,
#62285,#62286,#62287,#62288,#62289,#62290,#62291,#62292,#62293,#62294,#62295,
#62296,#62297,#62298,#62299,#62300,#62301,#62302,#62303),.UNSPECIFIED.,
 .F.,.F.,(4,3,3,3,3,3,3,3,3,3,3,3,3,3,3,3,3,3,3,3,3,3,3,3,3,3,4),(0.,0.0183455177171484,
0.0365842486584377,0.0503567352932813,0.057506472843321,0.0612717639518736,
0.0790233645150093,0.096412286696173,0.109000250456427,0.115579416228416,
0.118639170027439,0.135489426230602,0.146764141737187,0.163451454243377,
0.16860513566105,0.173128108917708,0.189898750695883,0.20664919054828,0.217355779107483,
0.22287251764273,0.226199914557468,0.242290795343361,0.252395270027202,
0.256089569829458,0.271598133490708,0.280262641786704,0.28634738033222),
 .UNSPECIFIED.);
#4417=B_SPLINE_CURVE_WITH_KNOTS('',3,(#62306,#62307,#62308,#62309,#62310,
#62311,#62312,#62313,#62314,#62315,#62316,#62317,#62318,#62319,#62320,#62321,
#62322,#62323,#62324,#62325,#62326,#62327,#62328,#62329,#62330,#62331,#62332,
#62333,#62334,#62335,#62336,#62337,#62338,#62339,#62340,#62341,#62342,#62343,
#62344,#62345,#62346,#62347,#62348,#62349,#62350,#62351,#62352,#62353,#62354,
#62355,#62356,#62357,#62358,#62359,#62360,#62361,#62362,#62363,#62364,#62365,
#62366,#62367,#62368,#62369,#62370,#62371,#62372,#62373,#62374,#62375,#62376,
#62377,#62378,#62379,#62380,#62381,#62382,#62383,#62384,#62385,#62386,#62387),
 .UNSPECIFIED.,.F.,.F.,(4,3,3,3,3,3,3,3,3,3,3,3,3,3,3,3,3,3,3,3,3,3,3,3,
3,3,3,4),(-0.28634738033221,-0.271025134810133,-0.260698514729526,-0.255927597095004,
-0.251928120084434,-0.235738775707159,-0.229541586612368,-0.225083751275628,
-0.221641755210153,-0.204608740834787,-0.187821912129427,-0.179056502768601,
-0.174353031512105,-0.17100836839964,-0.168068126672392,-0.153509697708691,
-0.136938878241907,-0.120740722231463,-0.116774450513702,-0.113778933952734,
-0.0964554865389578,-0.078760241337473,-0.0609085885426931,-0.0568635638370591,
-0.0386446388676857,-0.0205858033551501,-0.00735363015835327,0.),
 .UNSPECIFIED.);
#4418=B_SPLINE_CURVE_WITH_KNOTS('',3,(#62388,#62389,#62390,#62391,#62392,
#62393,#62394,#62395,#62396,#62397,#62398,#62399,#62400,#62401,#62402,#62403,
#62404,#62405,#62406,#62407,#62408,#62409,#62410,#62411,#62412,#62413,#62414,
#62415,#62416,#62417,#62418,#62419,#62420,#62421,#62422,#62423,#62424,#62425,
#62426,#62427,#62428,#62429,#62430,#62431,#62432,#62433,#62434,#62435,#62436,
#62437,#62438,#62439,#62440,#62441,#62442,#62443,#62444,#62445,#62446,#62447,
#62448,#62449,#62450,#62451,#62452,#62453,#62454,#62455,#62456,#62457,#62458,
#62459,#62460,#62461,#62462,#62463),.UNSPECIFIED.,.F.,.F.,(4,3,3,3,3,3,
3,3,3,3,3,3,3,3,3,3,3,3,3,3,3,3,3,3,3,4),(-0.285142803995119,-0.266893522635827,
-0.249971481821918,-0.245887106233145,-0.227911281467346,-0.216815940424025,
-0.213019169001087,-0.209467645119212,-0.191887872119604,-0.174757062554003,
-0.165469230791568,-0.157741956071688,-0.154438809614972,-0.139148553120781,
-0.122062023309062,-0.107562410123394,-0.10357617742568,-0.100472613627008,
-0.0838658566323333,-0.0673520867984852,-0.0520303445547921,-0.048094708626416,
-0.0321861070442482,-0.0168171644241619,-0.00606511782371298,0.),
 .UNSPECIFIED.);
#4419=B_SPLINE_CURVE_WITH_KNOTS('',3,(#62465,#62466,#62467,#62468,#62469,
#62470,#62471,#62472,#62473,#62474,#62475),.UNSPECIFIED.,.F.,.F.,(4,1,1,
1,1,1,1,1,4),(15.7079632679489,15.8014786182354,16.7880079568995,17.7745372955635,
18.7610666342275,19.7475959728916,20.7341253115556,21.7206546502196,21.9911485751285),
 .UNSPECIFIED.);
#4420=B_SPLINE_CURVE_WITH_KNOTS('',3,(#62476,#62477,#62478,#62479,#62480,
#62481,#62482,#62483,#62484,#62485),.UNSPECIFIED.,.F.,.F.,(4,1,1,1,1,1,
1,4),(15.7079632679489,16.3714588042999,17.3579881429639,18.3445174816279,
19.331046820292,20.317576158956,21.30410549762,21.9911485751285),
 .UNSPECIFIED.);
#4421=B_SPLINE_CURVE_WITH_KNOTS('',3,(#62710,#62711,#62712,#62713,#62714,
#62715,#62716,#62717,#62718,#62719,#62720,#62721,#62722,#62723,#62724,#62725,
#62726,#62727,#62728,#62729,#62730,#62731,#62732,#62733,#62734,#62735,#62736,
#62737,#62738,#62739,#62740,#62741,#62742,#62743,#62744,#62745,#62746,#62747,
#62748,#62749,#62750,#62751,#62752,#62753,#62754,#62755,#62756,#62757,#62758,
#62759,#62760,#62761,#62762,#62763,#62764,#62765,#62766,#62767,#62768,#62769,
#62770,#62771,#62772,#62773,#62774,#62775,#62776,#62777,#62778,#62779,#62780,
#62781,#62782,#62783,#62784,#62785,#62786,#62787,#62788,#62789,#62790,#62791),
 .UNSPECIFIED.,.F.,.F.,(4,3,3,3,3,3,3,3,3,3,3,3,3,3,3,3,3,3,3,3,3,3,3,3,
3,3,3,4),(0.,0.0151383092199202,0.030955006769346,0.0436395623388301,0.0490032691308595,
0.0520443158127519,0.0683454961235161,0.0849450886188161,0.0968166792954167,
0.101864993838732,0.104873332695592,0.121948986956247,0.132431451325219,
0.149057249647569,0.154031743970792,0.15863082340794,0.17566870475993,0.193109534812356,
0.203698360649826,0.209528438175835,0.213039046070598,0.231029814280384,
0.242727396088317,0.247561053645041,0.251100328226373,0.269296434614431,
0.277820141512116,0.285142803995131),.UNSPECIFIED.);
#4422=B_SPLINE_CURVE_WITH_KNOTS('',3,(#62792,#62793,#62794,#62795,#62796,
#62797,#62798,#62799,#62800,#62801,#62802,#62803,#62804,#62805,#62806,#62807,
#62808,#62809,#62810,#62811,#62812,#62813,#62814,#62815,#62816),
 .UNSPECIFIED.,.F.,.F.,(4,3,3,3,3,3,3,3,4),(-10.1357873115492,-9.8652933866403,
-8.87876404797628,-7.89223470931224,-6.90570537064822,-5.91917603198418,
-4.93264669332016,-3.94611735465612,-3.85260200436961),.UNSPECIFIED.);
#4423=B_SPLINE_CURVE_WITH_KNOTS('',3,(#63041,#63042,#63043,#63044,#63045,
#63046,#63047,#63048,#63049,#63050,#63051,#63052,#63053,#63054,#63055,#63056,
#63057,#63058,#63059,#63060,#63061,#63062,#63063,#63064,#63065),
 .UNSPECIFIED.,.F.,.F.,(4,3,3,3,3,3,3,3,4),(7.59274844815668,7.89223470931225,
8.87876404797628,9.86529338664031,10.8518227253043,11.8383520639684,12.8248814026324,
13.8114107412964,13.8759337553363),.UNSPECIFIED.);
#4424=B_SPLINE_CURVE_WITH_KNOTS('',3,(#63066,#63067,#63068,#63069,#63070,
#63071,#63072,#63073,#63074,#63075,#63076,#63077,#63078,#63079,#63080,#63081,
#63082,#63083,#63084,#63085,#63086,#63087,#63088,#63089,#63090,#63091,#63092,
#63093,#63094,#63095,#63096,#63097,#63098,#63099,#63100,#63101,#63102,#63103,
#63104,#63105,#63106,#63107,#63108,#63109,#63110,#63111,#63112,#63113,#63114,
#63115,#63116,#63117,#63118,#63119,#63120,#63121,#63122,#63123,#63124,#63125,
#63126,#63127,#63128,#63129,#63130,#63131,#63132,#63133,#63134,#63135,#63136,
#63137,#63138,#63139,#63140,#63141,#63142,#63143,#63144),.UNSPECIFIED.,
 .F.,.F.,(4,3,3,3,3,3,3,3,3,3,3,3,3,3,3,3,3,3,3,3,3,3,3,3,3,3,4),(0.,0.0183455177171501,
0.0365842479880188,0.0503567347066666,0.0575064710097809,0.06127176277414,
0.0790233634744086,0.096412289501403,0.109000252560352,0.115579416554078,
0.118639169840573,0.135489429658593,0.146764141737201,0.163451454243393,
0.168605140810027,0.173128107436249,0.189898748857662,0.2066491892331,0.217355774416626,
0.222872516868838,0.226199915188627,0.242290799535295,0.25239527713926,
0.25608958297081,0.27159815236556,0.280262641786741,0.286347380332253),
 .UNSPECIFIED.);
#4425=B_SPLINE_CURVE_WITH_KNOTS('',3,(#63147,#63148,#63149,#63150,#63151,
#63152,#63153,#63154,#63155,#63156,#63157,#63158,#63159,#63160,#63161,#63162,
#63163,#63164,#63165,#63166,#63167,#63168,#63169,#63170,#63171,#63172,#63173,
#63174,#63175,#63176,#63177,#63178,#63179,#63180,#63181,#63182,#63183,#63184,
#63185,#63186,#63187,#63188,#63189,#63190,#63191,#63192,#63193,#63194,#63195,
#63196,#63197,#63198,#63199,#63200,#63201,#63202,#63203,#63204,#63205,#63206,
#63207,#63208,#63209,#63210,#63211,#63212,#63213,#63214,#63215,#63216,#63217,
#63218,#63219,#63220,#63221,#63222,#63223,#63224,#63225,#63226,#63227,#63228),
 .UNSPECIFIED.,.F.,.F.,(4,3,3,3,3,3,3,3,3,3,3,3,3,3,3,3,3,3,3,3,3,3,3,3,
3,3,3,4),(-0.286347380332241,-0.271025621689686,-0.260700126708286,-0.255933999923882,
-0.251928786217571,-0.235739770682513,-0.229543552627355,-0.225090694895415,
-0.221644284962138,-0.204610638148777,-0.187823738640676,-0.179057759820386,
-0.174355103845197,-0.171011959994442,-0.168068908451443,-0.153509697708694,
-0.136938545278193,-0.120740430888213,-0.116772838423195,-0.113777170653691,
-0.0964534278594871,-0.0787580645389843,-0.0609069559438266,-0.0568632900412494,
-0.0386443179131428,-0.0205854755819572,-0.00735363015835342,0.),
 .UNSPECIFIED.);
#4426=B_SPLINE_CURVE_WITH_KNOTS('',3,(#63229,#63230,#63231,#63232,#63233,
#63234,#63235,#63236,#63237,#63238,#63239,#63240,#63241,#63242,#63243,#63244,
#63245,#63246,#63247,#63248,#63249,#63250,#63251,#63252,#63253,#63254,#63255,
#63256,#63257,#63258,#63259,#63260,#63261,#63262,#63263,#63264,#63265,#63266,
#63267,#63268,#63269,#63270,#63271,#63272,#63273,#63274,#63275,#63276,#63277,
#63278,#63279,#63280,#63281,#63282,#63283,#63284,#63285,#63286,#63287,#63288,
#63289,#63290,#63291,#63292,#63293,#63294,#63295,#63296,#63297,#63298,#63299,
#63300,#63301,#63302,#63303,#63304),.UNSPECIFIED.,.F.,.F.,(4,3,3,3,3,3,
3,3,3,3,3,3,3,3,3,3,3,3,3,3,3,3,3,3,3,4),(-0.285142803995115,-0.266893522635823,
-0.249971640312005,-0.245887155062476,-0.227911309456783,-0.216815964914783,
-0.213019369681369,-0.209467693446233,-0.191887908364871,-0.174756961587167,
-0.165469070516051,-0.157741742342989,-0.15443884445219,-0.139148553120784,
-0.122062040548301,-0.107562425207727,-0.103576093457847,-0.100472602972665,
-0.0838658644229591,-0.0673520539817759,-0.0520303199422602,-0.0480946799671829,
-0.0321859944606137,-0.0168167950638599,-0.00606511782371299,0.),
 .UNSPECIFIED.);
#4427=B_SPLINE_CURVE_WITH_KNOTS('',3,(#63306,#63307,#63308,#63309,#63310,
#63311,#63312,#63313,#63314,#63315,#63316),.UNSPECIFIED.,.F.,.F.,(4,1,1,
1,1,1,1,1,4),(15.7079632679489,15.8014786182354,16.7880079568995,17.7745372955635,
18.7610666342275,19.7475959728916,20.7341253115556,21.7206546502196,21.9911485751285),
 .UNSPECIFIED.);
#4428=B_SPLINE_CURVE_WITH_KNOTS('',3,(#63317,#63318,#63319,#63320,#63321,
#63322,#63323,#63324,#63325,#63326),.UNSPECIFIED.,.F.,.F.,(4,1,1,1,1,1,
1,4),(15.7079632679489,16.3714588042999,17.3579881429639,18.3445174816279,
19.331046820292,20.317576158956,21.30410549762,21.9911485751285),
 .UNSPECIFIED.);
#4429=B_SPLINE_CURVE_WITH_KNOTS('',3,(#63551,#63552,#63553,#63554,#63555,
#63556,#63557,#63558,#63559,#63560,#63561,#63562,#63563,#63564,#63565,#63566,
#63567,#63568,#63569,#63570,#63571,#63572,#63573,#63574,#63575,#63576,#63577,
#63578,#63579,#63580,#63581,#63582,#63583,#63584,#63585,#63586,#63587,#63588,
#63589,#63590,#63591,#63592,#63593,#63594,#63595,#63596,#63597,#63598,#63599,
#63600,#63601,#63602,#63603,#63604,#63605,#63606,#63607,#63608,#63609,#63610,
#63611,#63612,#63613,#63614,#63615,#63616,#63617,#63618,#63619,#63620,#63621,
#63622,#63623,#63624,#63625,#63626,#63627,#63628,#63629,#63630,#63631,#63632),
 .UNSPECIFIED.,.F.,.F.,(4,3,3,3,3,3,3,3,3,3,3,3,3,3,3,3,3,3,3,3,3,3,3,3,
3,3,3,4),(0.,0.0151377992486527,0.0309541346648382,0.0436387992473864,0.049001010822214,
0.0520440199057219,0.0683448437138882,0.084944333062083,0.0968161126278682,
0.101863396044648,0.104870610854465,0.121946324184151,0.132431451325224,
0.149057505426147,0.154031793452874,0.158630809283319,0.175668969542699,
0.193109928367254,0.203698705010364,0.209528824983296,0.213039415112694,
0.231030207184506,0.242727690766411,0.247562113622632,0.251101431476124,
0.269297523973198,0.277820141512129,0.28514280399514),.UNSPECIFIED.);
#4430=B_SPLINE_CURVE_WITH_KNOTS('',3,(#63633,#63634,#63635,#63636,#63637,
#63638,#63639,#63640,#63641,#63642,#63643,#63644,#63645,#63646,#63647,#63648,
#63649,#63650,#63651,#63652,#63653,#63654,#63655,#63656,#63657),
 .UNSPECIFIED.,.F.,.F.,(4,3,3,3,3,3,3,3,4),(-10.1357873115492,-9.86529338664031,
-8.87876404797628,-7.89223470931225,-6.90570537064822,-5.91917603198419,
-4.93264669332015,-3.94611735465612,-3.85260200436961),.UNSPECIFIED.);
#4431=B_SPLINE_CURVE_WITH_KNOTS('',3,(#63882,#63883,#63884,#63885,#63886,
#63887,#63888,#63889,#63890,#63891,#63892,#63893,#63894,#63895,#63896,#63897,
#63898,#63899,#63900,#63901,#63902,#63903,#63904,#63905,#63906),
 .UNSPECIFIED.,.F.,.F.,(4,3,3,3,3,3,3,3,4),(7.59274844815667,7.89223470931225,
8.87876404797628,9.86529338664031,10.8518227253043,11.8383520639684,12.8248814026324,
13.8114107412964,13.8759337553363),.UNSPECIFIED.);
#4432=B_SPLINE_CURVE_WITH_KNOTS('',3,(#63907,#63908,#63909,#63910,#63911,
#63912,#63913,#63914,#63915,#63916,#63917,#63918,#63919,#63920,#63921,#63922,
#63923,#63924,#63925,#63926,#63927,#63928,#63929,#63930,#63931,#63932,#63933,
#63934,#63935,#63936,#63937,#63938,#63939,#63940,#63941,#63942,#63943,#63944,
#63945,#63946,#63947,#63948,#63949,#63950,#63951,#63952,#63953,#63954,#63955,
#63956,#63957,#63958,#63959,#63960,#63961,#63962,#63963,#63964,#63965,#63966,
#63967,#63968,#63969,#63970,#63971,#63972,#63973,#63974,#63975,#63976,#63977,
#63978,#63979,#63980,#63981,#63982,#63983,#63984,#63985),.UNSPECIFIED.,
 .F.,.F.,(4,3,3,3,3,3,3,3,3,3,3,3,3,3,3,3,3,3,3,3,3,3,3,3,3,3,4),(0.,0.0183455177171494,
0.0365842224514134,0.0503567123621361,0.0575064018577643,0.0612717186008677,
0.0790233237763444,0.096412392225862,0.109000329603695,0.115579426963446,
0.118639160101204,0.135489553798197,0.146764141737195,0.163451454243386,
0.168605331106135,0.173128052469876,0.189898680358684,0.206649139107136,
0.217355601404959,0.222872488375841,0.22619993877691,0.242290953399338,
0.252395538895798,0.256090068005537,0.271598847870641,0.280262641786722,
0.286347380332235),.UNSPECIFIED.);
#4433=B_SPLINE_CURVE_WITH_KNOTS('',3,(#63988,#63989,#63990,#63991,#63992,
#63993,#63994,#63995,#63996,#63997,#63998,#63999,#64000,#64001,#64002,#64003,
#64004,#64005,#64006,#64007,#64008,#64009,#64010,#64011,#64012,#64013,#64014,
#64015,#64016,#64017,#64018,#64019,#64020,#64021,#64022,#64023,#64024,#64025,
#64026,#64027,#64028,#64029,#64030,#64031,#64032,#64033,#64034,#64035,#64036,
#64037,#64038,#64039,#64040,#64041,#64042,#64043,#64044,#64045,#64046,#64047,
#64048,#64049,#64050,#64051,#64052,#64053,#64054,#64055,#64056,#64057,#64058,
#64059,#64060,#64061,#64062,#64063,#64064,#64065,#64066,#64067,#64068,#64069),
 .UNSPECIFIED.,.F.,.F.,(4,3,3,3,3,3,3,3,3,3,3,3,3,3,3,3,3,3,3,3,3,3,3,3,
3,3,3,4),(-0.286347380332241,-0.271025121721634,-0.260698471406766,-0.255927424639791,
-0.251928101932755,-0.235738748723829,-0.229541533307826,-0.225083562737093,
-0.22164168507229,-0.20460868823139,-0.187821861469231,-0.179056467802176,
-0.174352973887146,-0.171008268495978,-0.168068104878629,-0.153509697708687,
-0.136938887238054,-0.120740730103091,-0.116774494105204,-0.113778981547202,
-0.0964555421096816,-0.0787603000911127,-0.0609086326079217,-0.0568635712110021,
-0.0386446475073598,-0.0205858121953219,-0.00735363015834877,0.),
 .UNSPECIFIED.);
#4434=B_SPLINE_CURVE_WITH_KNOTS('',3,(#64070,#64071,#64072,#64073,#64074,
#64075,#64076,#64077,#64078,#64079,#64080,#64081,#64082,#64083,#64084,#64085,
#64086,#64087,#64088,#64089,#64090,#64091,#64092,#64093,#64094,#64095,#64096,
#64097,#64098,#64099,#64100,#64101,#64102,#64103,#64104,#64105,#64106,#64107,
#64108,#64109,#64110,#64111,#64112,#64113,#64114,#64115,#64116,#64117,#64118,
#64119,#64120,#64121,#64122,#64123,#64124,#64125,#64126,#64127,#64128,#64129,
#64130,#64131,#64132,#64133,#64134,#64135,#64136,#64137,#64138,#64139,#64140,
#64141,#64142,#64143,#64144,#64145),.UNSPECIFIED.,.F.,.F.,(4,3,3,3,3,3,
3,3,3,3,3,3,3,3,3,3,3,3,3,3,3,3,3,3,3,4),(-0.285142803995177,-0.266893522635881,
-0.24997147696309,-0.245887104754832,-0.227911280648222,-0.216815939707296,
-0.213019163245401,-0.209467643680815,-0.191887871040814,-0.174757065708801,
-0.16546923578312,-0.157741962744139,-0.154438808517409,-0.13914855312081,
-0.122062022789569,-0.107562409668837,-0.103576180068357,-0.100472613959823,
-0.0838658564094648,-0.0673520878642787,-0.0520303453541372,-0.0480947095174562,
-0.0321861105661567,-0.0168171759288923,-0.00606511782371295,0.),
 .UNSPECIFIED.);
#4435=B_SPLINE_CURVE_WITH_KNOTS('',3,(#64147,#64148,#64149,#64150,#64151,
#64152,#64153,#64154,#64155,#64156,#64157),.UNSPECIFIED.,.F.,.F.,(4,1,1,
1,1,1,1,1,4),(15.7079632679489,15.8014786182355,16.7880079568995,17.7745372955635,
18.7610666342275,19.7475959728916,20.7341253115556,21.7206546502196,21.9911485751285),
 .UNSPECIFIED.);
#4436=B_SPLINE_CURVE_WITH_KNOTS('',3,(#64158,#64159,#64160,#64161,#64162,
#64163,#64164,#64165,#64166,#64167),.UNSPECIFIED.,.F.,.F.,(4,1,1,1,1,1,
1,4),(15.7079632679489,16.3714588042999,17.3579881429639,18.344517481628,
19.331046820292,20.317576158956,21.30410549762,21.9911485751285),
 .UNSPECIFIED.);
#4437=B_SPLINE_CURVE_WITH_KNOTS('',3,(#64392,#64393,#64394,#64395,#64396,
#64397,#64398,#64399,#64400,#64401,#64402,#64403,#64404,#64405,#64406,#64407,
#64408,#64409,#64410,#64411,#64412,#64413,#64414,#64415,#64416,#64417,#64418,
#64419,#64420,#64421,#64422,#64423,#64424,#64425,#64426,#64427,#64428,#64429,
#64430,#64431,#64432,#64433,#64434,#64435,#64436,#64437,#64438,#64439,#64440,
#64441,#64442,#64443,#64444,#64445,#64446,#64447,#64448,#64449,#64450,#64451,
#64452,#64453,#64454,#64455,#64456,#64457,#64458,#64459,#64460,#64461,#64462,
#64463,#64464,#64465,#64466,#64467,#64468,#64469,#64470,#64471,#64472,#64473),
 .UNSPECIFIED.,.F.,.F.,(4,3,3,3,3,3,3,3,3,3,3,3,3,3,3,3,3,3,3,3,3,3,3,3,
3,3,3,4),(0.,0.0151383248856871,0.0309550335469064,0.0436395857691952,0.0490033384910799,
0.0520443250910099,0.0683455163444214,0.0849451119840661,0.0968166968193539,
0.101865043240895,0.104873417046857,0.121949069457094,0.132431451325217,
0.149057241756068,0.154031742415278,0.15863082385134,0.175668696597353,
0.193109522683886,0.203698350037412,0.209528426219566,0.213039034673188,
0.231029802151329,0.24272738699152,0.247561020928704,0.251100294224577,
0.269296401030219,0.277820141512092,0.285142803995105),.UNSPECIFIED.);
#4438=B_SPLINE_CURVE_WITH_KNOTS('',3,(#64474,#64475,#64476,#64477,#64478,
#64479,#64480,#64481,#64482,#64483,#64484,#64485,#64486,#64487,#64488,#64489,
#64490,#64491,#64492,#64493,#64494,#64495,#64496,#64497,#64498),
 .UNSPECIFIED.,.F.,.F.,(4,3,3,3,3,3,3,3,4),(-10.1357873115492,-9.86529338664031,
-8.87876404797628,-7.89223470931225,-6.90570537064822,-5.91917603198419,
-4.93264669332015,-3.94611735465612,-3.85260200436962),.UNSPECIFIED.);
#4439=B_SPLINE_CURVE_WITH_KNOTS('',3,(#64723,#64724,#64725,#64726,#64727,
#64728,#64729,#64730,#64731,#64732,#64733,#64734,#64735,#64736,#64737,#64738,
#64739,#64740,#64741,#64742,#64743,#64744,#64745,#64746,#64747),
 .UNSPECIFIED.,.F.,.F.,(4,3,3,3,3,3,3,3,4),(7.59274844815668,7.89223470931224,
8.87876404797627,9.8652933866403,10.8518227253043,11.8383520639684,12.8248814026324,
13.8114107412964,13.8759337553363),.UNSPECIFIED.);
#4440=B_SPLINE_CURVE_WITH_KNOTS('',3,(#64748,#64749,#64750,#64751,#64752,
#64753,#64754,#64755,#64756,#64757,#64758,#64759,#64760,#64761,#64762,#64763,
#64764,#64765,#64766,#64767,#64768,#64769,#64770,#64771,#64772,#64773,#64774,
#64775,#64776,#64777,#64778,#64779,#64780,#64781,#64782,#64783,#64784,#64785,
#64786,#64787,#64788,#64789,#64790,#64791,#64792,#64793,#64794,#64795,#64796,
#64797,#64798,#64799,#64800,#64801,#64802,#64803,#64804,#64805,#64806,#64807,
#64808,#64809,#64810,#64811,#64812,#64813,#64814,#64815,#64816,#64817,#64818,
#64819,#64820,#64821,#64822,#64823,#64824,#64825,#64826),.UNSPECIFIED.,
 .F.,.F.,(4,3,3,3,3,3,3,3,3,3,3,3,3,3,3,3,3,3,3,3,3,3,3,3,3,3,4),(0.,0.0183455177171494,
0.0365842486584371,0.0503567352932819,0.0575064728432776,0.0612717639547951,
0.0790233645178617,0.0964122866988397,0.109000250458429,0.115579416230427,
0.118639170032811,0.135489426235933,0.146764141737196,0.163451454243387,
0.168605135661181,0.173128108919256,0.189898750697359,0.206649190549959,
0.217355779106873,0.222872517642441,0.22619991455212,0.242290795338002,
0.2523952700195,0.256089569811339,0.271598133473104,0.280262641786723,0.286347380332239),
 .UNSPECIFIED.);
#4441=B_SPLINE_CURVE_WITH_KNOTS('',3,(#64849,#64850,#64851,#64852,#64853,
#64854,#64855,#64856,#64857,#64858,#64859,#64860,#64861,#64862,#64863,#64864,
#64865,#64866,#64867,#64868,#64869,#64870,#64871,#64872,#64873,#64874,#64875,
#64876,#64877,#64878,#64879,#64880,#64881,#64882,#64883,#64884,#64885,#64886,
#64887,#64888,#64889,#64890,#64891,#64892,#64893,#64894,#64895,#64896,#64897,
#64898,#64899,#64900,#64901,#64902,#64903,#64904,#64905,#64906,#64907,#64908,
#64909,#64910,#64911,#64912,#64913,#64914,#64915,#64916,#64917,#64918,#64919,
#64920,#64921,#64922,#64923,#64924,#64925,#64926,#64927,#64928,#64929,#64930),
 .UNSPECIFIED.,.F.,.F.,(4,3,3,3,3,3,3,3,3,3,3,3,3,3,3,3,3,3,3,3,3,3,3,3,
3,3,3,4),(-0.286347380332242,-0.271026132708159,-0.26070181912171,-0.255940688203078,
-0.251929465810934,-0.235740795969021,-0.229545579465539,-0.225097832776575,
-0.221646776596611,-0.204612506874632,-0.187825536148012,-0.179058989177513,
-0.17435713213233,-0.17101547339657,-0.168069670163224,-0.153509697708693,
-0.136938199431907,-0.120740128272712,-0.116771166875623,-0.113775334580713,
-0.096451284491223,-0.0787557978507567,-0.0609052559276548,-0.0568630026035331,
-0.0386439810009667,-0.0205851328894473,-0.00735363015834924,0.),
 .UNSPECIFIED.);
#4442=B_SPLINE_CURVE_WITH_KNOTS('',3,(#64931,#64932,#64933,#64934,#64935,
#64936,#64937,#64938,#64939,#64940,#64941,#64942,#64943,#64944,#64945,#64946,
#64947,#64948,#64949,#64950,#64951,#64952,#64953,#64954,#64955,#64956,#64957,
#64958,#64959,#64960,#64961,#64962,#64963,#64964,#64965,#64966,#64967,#64968,
#64969,#64970,#64971,#64972,#64973,#64974,#64975,#64976,#64977,#64978,#64979,
#64980,#64981,#64982,#64983,#64984,#64985,#64986,#64987,#64988,#64989,#64990,
#64991,#64992,#64993,#64994,#64995,#64996,#64997,#64998,#64999,#65000,#65001,
#65002,#65003,#65004,#65005,#65006),.UNSPECIFIED.,.F.,.F.,(4,3,3,3,3,3,
3,3,3,3,3,3,3,3,3,3,3,3,3,3,3,3,3,3,3,4),(-0.285142803995146,-0.266893522635853,
-0.249971821339198,-0.245887210812531,-0.227911342993235,-0.216815994259181,
-0.21301961305492,-0.209467750298075,-0.191887951003757,-0.174756849434581,
-0.165468891951558,-0.157741505410476,-0.1544388836839,-0.139148553120802,
-0.122062060978925,-0.107562443084524,-0.103576002803389,-0.10047259097034,
-0.0838658743207705,-0.0673520207865497,-0.0520302950458412,-0.0480946476761015,
-0.0321858707120756,-0.0168163861623916,-0.00606511782371579,0.),
 .UNSPECIFIED.);
#4443=B_SPLINE_CURVE_WITH_KNOTS('',3,(#65008,#65009,#65010,#65011,#65012,
#65013,#65014,#65015,#65016,#65017,#65018),.UNSPECIFIED.,.F.,.F.,(4,1,1,
1,1,1,1,1,4),(15.7079632679489,15.8014786182355,16.7880079568995,17.7745372955635,
18.7610666342276,19.7475959728916,20.7341253115556,21.7206546502197,21.9911485751285),
 .UNSPECIFIED.);
#4444=B_SPLINE_CURVE_WITH_KNOTS('',3,(#65019,#65020,#65021,#65022,#65023,
#65024,#65025,#65026,#65027,#65028),.UNSPECIFIED.,.F.,.F.,(4,1,1,1,1,1,
1,4),(15.7079632679489,16.3714588042999,17.357988142964,18.344517481628,
19.331046820292,20.317576158956,21.3041054976201,21.9911485751285),
 .UNSPECIFIED.);
#4445=B_SPLINE_CURVE_WITH_KNOTS('',3,(#65253,#65254,#65255,#65256,#65257,
#65258,#65259,#65260,#65261,#65262,#65263,#65264,#65265,#65266,#65267,#65268,
#65269,#65270,#65271,#65272,#65273,#65274,#65275,#65276,#65277),
 .UNSPECIFIED.,.F.,.F.,(4,3,3,3,3,3,3,3,4),(-10.1357873115492,-9.8652933866403,
-8.87876404797628,-7.89223470931225,-6.90570537064821,-5.91917603198418,
-4.93264669332015,-3.94611735465612,-3.85260200436958),.UNSPECIFIED.);
#4446=B_SPLINE_CURVE_WITH_KNOTS('',3,(#65502,#65503,#65504,#65505,#65506,
#65507,#65508,#65509,#65510,#65511,#65512,#65513,#65514,#65515,#65516,#65517,
#65518,#65519,#65520,#65521,#65522,#65523,#65524,#65525,#65526),
 .UNSPECIFIED.,.F.,.F.,(4,3,3,3,3,3,3,3,4),(7.59274844815664,7.89223470931225,
8.87876404797627,9.86529338664031,10.8518227253043,11.8383520639684,12.8248814026324,
13.8114107412964,13.8759337553362),.UNSPECIFIED.);
#4447=B_SPLINE_CURVE_WITH_KNOTS('',3,(#65529,#65530,#65531,#65532,#65533,
#65534,#65535,#65536,#65537,#65538,#65539,#65540,#65541,#65542,#65543,#65544,
#65545,#65546,#65547,#65548,#65549,#65550,#65551,#65552,#65553,#65554,#65555,
#65556,#65557,#65558,#65559,#65560,#65561,#65562,#65563,#65564,#65565,#65566,
#65567,#65568,#65569,#65570,#65571,#65572,#65573,#65574,#65575,#65576,#65577,
#65578,#65579,#65580,#65581,#65582,#65583,#65584,#65585,#65586,#65587,#65588,
#65589,#65590,#65591,#65592,#65593,#65594,#65595,#65596,#65597,#65598,#65599,
#65600,#65601,#65602,#65603,#65604,#65605,#65606,#65607,#65608,#65609,#65610),
 .UNSPECIFIED.,.F.,.F.,(4,3,3,3,3,3,3,3,3,3,3,3,3,3,3,3,3,3,3,3,3,3,3,3,
3,3,3,4),(-0.286347380332275,-0.27102566316108,-0.260700264038628,-0.255934543840492,
-0.251928842105127,-0.235739854602674,-0.229543718486113,-0.225091279778216,
-0.221644493299042,-0.204610794401459,-0.187823888995587,-0.179057862959692,
-0.174355273945332,-0.171012254723885,-0.168068972461,-0.153509697708709,
-0.136938517071018,-0.120740406206935,-0.116772701979239,-0.113777021075996,
-0.0964532532380554,-0.0787578798842962,-0.0609068174528094,-0.056863266677987,
-0.0386442905322982,-0.0205854476800074,-0.00735363015834906,0.),
 .UNSPECIFIED.);
#4448=B_SPLINE_CURVE_WITH_KNOTS('',3,(#65611,#65612,#65613,#65614,#65615,
#65616,#65617,#65618,#65619,#65620,#65621,#65622,#65623,#65624,#65625,#65626,
#65627,#65628,#65629,#65630,#65631,#65632,#65633,#65634,#65635,#65636,#65637,
#65638,#65639,#65640,#65641,#65642,#65643,#65644,#65645,#65646,#65647,#65648,
#65649,#65650,#65651,#65652,#65653,#65654,#65655,#65656,#65657,#65658,#65659,
#65660,#65661,#65662,#65663,#65664,#65665,#65666,#65667,#65668,#65669,#65670,
#65671,#65672,#65673,#65674,#65675,#65676,#65677,#65678,#65679,#65680,#65681,
#65682,#65683,#65684,#65685,#65686),.UNSPECIFIED.,.F.,.F.,(4,3,3,3,3,3,
3,3,3,3,3,3,3,3,3,3,3,3,3,3,3,3,3,3,3,4),(-0.285142803995182,-0.266893522635886,
-0.249971668921242,-0.245887163875788,-0.227911314645579,-0.216815969454983,
-0.213019407143944,-0.209467702314156,-0.19188791501582,-0.174756943635084,
-0.165469041972909,-0.157741704382841,-0.154438850672044,-0.139148553120812,
-0.122062043724214,-0.107562427986652,-0.103576078755324,-0.100472601057323,
-0.0838658659084289,-0.0673520484249552,-0.0520303157746454,-0.0480946748254668,
-0.0321859745524222,-0.0168167295122947,-0.00606511782371583,0.),
 .UNSPECIFIED.);
#4449=B_SPLINE_CURVE_WITH_KNOTS('',3,(#65688,#65689,#65690,#65691,#65692,
#65693,#65694,#65695,#65696,#65697,#65698),.UNSPECIFIED.,.F.,.F.,(4,1,1,
1,1,1,1,1,4),(15.7079632679489,15.8014786182355,16.7880079568995,17.7745372955635,
18.7610666342276,19.7475959728916,20.7341253115556,21.7206546502197,21.9911485751285),
 .UNSPECIFIED.);
#4450=B_SPLINE_CURVE_WITH_KNOTS('',3,(#65699,#65700,#65701,#65702,#65703,
#65704,#65705,#65706,#65707,#65708),.UNSPECIFIED.,.F.,.F.,(4,1,1,1,1,1,
1,4),(15.7079632679489,16.3714588042999,17.357988142964,18.344517481628,
19.331046820292,20.317576158956,21.3041054976201,21.9911485751285),
 .UNSPECIFIED.);
#4451=B_SPLINE_CURVE_WITH_KNOTS('',3,(#65933,#65934,#65935,#65936,#65937,
#65938,#65939,#65940,#65941,#65942,#65943,#65944,#65945,#65946,#65947,#65948,
#65949,#65950,#65951,#65952,#65953,#65954,#65955,#65956,#65957),
 .UNSPECIFIED.,.F.,.F.,(4,3,3,3,3,3,3,3,4),(-10.1357873115492,-9.86529338664031,
-8.87876404797628,-7.89223470931225,-6.90570537064822,-5.91917603198419,
-4.93264669332016,-3.94611735465613,-3.85260200436958),.UNSPECIFIED.);
#4452=B_SPLINE_CURVE_WITH_KNOTS('',3,(#66182,#66183,#66184,#66185,#66186,
#66187,#66188,#66189,#66190,#66191,#66192,#66193,#66194,#66195,#66196,#66197,
#66198,#66199,#66200,#66201,#66202,#66203,#66204,#66205,#66206),
 .UNSPECIFIED.,.F.,.F.,(4,3,3,3,3,3,3,3,4),(7.59274844815664,7.89223470931224,
8.87876404797627,9.86529338664031,10.8518227253043,11.8383520639684,12.8248814026324,
13.8114107412964,13.8759337553362),.UNSPECIFIED.);
#4453=B_SPLINE_CURVE_WITH_KNOTS('',3,(#66209,#66210,#66211,#66212,#66213,
#66214,#66215,#66216,#66217,#66218,#66219,#66220,#66221,#66222,#66223,#66224,
#66225,#66226,#66227,#66228,#66229,#66230,#66231,#66232,#66233,#66234,#66235,
#66236,#66237,#66238,#66239,#66240,#66241,#66242,#66243,#66244,#66245,#66246,
#66247,#66248,#66249,#66250,#66251,#66252,#66253,#66254,#66255,#66256,#66257,
#66258,#66259,#66260,#66261,#66262,#66263,#66264,#66265,#66266,#66267,#66268,
#66269,#66270,#66271,#66272,#66273,#66274,#66275,#66276,#66277,#66278,#66279,
#66280,#66281,#66282,#66283,#66284,#66285,#66286,#66287,#66288,#66289,#66290),
 .UNSPECIFIED.,.F.,.F.,(4,3,3,3,3,3,3,3,3,3,3,3,3,3,3,3,3,3,3,3,3,3,3,3,
3,3,3,4),(-0.286347380332252,-0.271025677132851,-0.260700310300518,-0.25593472713892,
-0.251928860913337,-0.235739882855375,-0.229543774327833,-0.225091476664371,
-0.221644563262721,-0.204610846874213,-0.18782393948616,-0.179057897584765,
-0.174355331052151,-0.171012353638296,-0.168068993938383,-0.15350969770869,
-0.136938507575371,-0.120740397898244,-0.116772656051337,-0.113776970697825,
-0.0964531944270655,-0.0787578176938258,-0.0609067708099572,-0.0568632588365736,
-0.0386442813392898,-0.020585438313091,-0.0073536301583514,0.),
 .UNSPECIFIED.);
#4454=B_SPLINE_CURVE_WITH_KNOTS('',3,(#66291,#66292,#66293,#66294,#66295,
#66296,#66297,#66298,#66299,#66300,#66301,#66302,#66303,#66304,#66305,#66306,
#66307,#66308,#66309,#66310,#66311,#66312,#66313,#66314,#66315,#66316,#66317,
#66318,#66319,#66320,#66321,#66322,#66323,#66324,#66325,#66326,#66327,#66328,
#66329,#66330,#66331,#66332,#66333,#66334,#66335,#66336,#66337,#66338,#66339,
#66340,#66341,#66342,#66343,#66344,#66345,#66346,#66347,#66348,#66349,#66350,
#66351,#66352,#66353,#66354,#66355,#66356,#66357,#66358,#66359,#66360,#66361,
#66362,#66363,#66364,#66365,#66366),.UNSPECIFIED.,.F.,.F.,(4,3,3,3,3,3,
3,3,3,3,3,3,3,3,3,3,3,3,3,3,3,3,3,3,3,4),(-0.285142803995135,-0.266893522635843,
-0.24997167290136,-0.245887165108436,-0.227911315377379,-0.216815970095306,
-0.213019412325979,-0.20946770354527,-0.191887915939152,-0.174756941140708,
-0.165469038008051,-0.157741699112297,-0.154438851562339,-0.139148553120795,
-0.122062044167205,-0.107562428374269,-0.10357607672048,-0.100472600788513,
-0.083865866115183,-0.0673520476568359,-0.0520303151985547,-0.0480946741162576,
-0.0321859717979194,-0.0168167204262572,-0.00606511782371128,0.),
 .UNSPECIFIED.);
#4455=B_SPLINE_CURVE_WITH_KNOTS('',3,(#66368,#66369,#66370,#66371,#66372,
#66373,#66374,#66375,#66376,#66377,#66378),.UNSPECIFIED.,.F.,.F.,(4,1,1,
1,1,1,1,1,4),(15.7079632679489,15.8014786182355,16.7880079568995,17.7745372955635,
18.7610666342276,19.7475959728916,20.7341253115556,21.7206546502197,21.9911485751285),
 .UNSPECIFIED.);
#4456=B_SPLINE_CURVE_WITH_KNOTS('',3,(#66379,#66380,#66381,#66382,#66383,
#66384,#66385,#66386,#66387,#66388),.UNSPECIFIED.,.F.,.F.,(4,1,1,1,1,1,
1,4),(15.7079632679489,16.3714588042999,17.357988142964,18.344517481628,
19.331046820292,20.317576158956,21.3041054976201,21.9911485751285),
 .UNSPECIFIED.);
#4457=B_SPLINE_CURVE_WITH_KNOTS('',3,(#66613,#66614,#66615,#66616,#66617,
#66618,#66619,#66620,#66621,#66622,#66623,#66624,#66625,#66626,#66627,#66628,
#66629,#66630,#66631,#66632,#66633,#66634,#66635,#66636,#66637),
 .UNSPECIFIED.,.F.,.F.,(4,3,3,3,3,3,3,3,4),(-10.1357873115492,-9.86529338664031,
-8.87876404797628,-7.89223470931225,-6.90570537064822,-5.91917603198419,
-4.93264669332016,-3.94611735465613,-3.85260200436961),.UNSPECIFIED.);
#4458=B_SPLINE_CURVE_WITH_KNOTS('',3,(#66862,#66863,#66864,#66865,#66866,
#66867,#66868,#66869,#66870,#66871,#66872,#66873,#66874,#66875,#66876,#66877,
#66878,#66879,#66880,#66881,#66882,#66883,#66884,#66885,#66886),
 .UNSPECIFIED.,.F.,.F.,(4,3,3,3,3,3,3,3,4),(7.59274844815664,7.89223470931225,
8.87876404797628,9.86529338664032,10.8518227253043,11.8383520639684,12.8248814026324,
13.8114107412964,13.8759337553362),.UNSPECIFIED.);
#4459=B_SPLINE_CURVE_WITH_KNOTS('',3,(#66889,#66890,#66891,#66892,#66893,
#66894,#66895,#66896,#66897,#66898,#66899,#66900,#66901,#66902,#66903,#66904,
#66905,#66906,#66907,#66908,#66909,#66910,#66911,#66912,#66913,#66914,#66915,
#66916,#66917,#66918,#66919,#66920,#66921,#66922,#66923,#66924,#66925,#66926,
#66927,#66928,#66929,#66930,#66931,#66932,#66933,#66934,#66935,#66936,#66937,
#66938,#66939,#66940,#66941,#66942,#66943,#66944,#66945,#66946,#66947,#66948,
#66949,#66950,#66951,#66952,#66953,#66954,#66955,#66956,#66957,#66958,#66959,
#66960,#66961,#66962,#66963,#66964,#66965,#66966,#66967,#66968,#66969,#66970),
 .UNSPECIFIED.,.F.,.F.,(4,3,3,3,3,3,3,3,3,3,3,3,3,3,3,3,3,3,3,3,3,3,3,3,
3,3,3,4),(-0.286347380332231,-0.271026132710428,-0.260701819128595,-0.255940688215407,
-0.251929465812578,-0.235740795970596,-0.229545579468544,-0.225097832787767,
-0.221646776634828,-0.204612506903293,-0.187825536176126,-0.179058989199214,
-0.174357132167787,-0.171015473459643,-0.168069670176233,-0.153509697708689,
-0.136938199431204,-0.120740128272097,-0.116771166870588,-0.11377533457899,
-0.0964512844881509,-0.0787557978480441,-0.0609052559256208,-0.0568630026064093,
-0.0386439810009145,-0.0205851328893904,-0.00735363015835105,0.),
 .UNSPECIFIED.);
#4460=B_SPLINE_CURVE_WITH_KNOTS('',3,(#66971,#66972,#66973,#66974,#66975,
#66976,#66977,#66978,#66979,#66980,#66981,#66982,#66983,#66984,#66985,#66986,
#66987,#66988,#66989,#66990,#66991,#66992,#66993,#66994,#66995,#66996,#66997,
#66998,#66999,#67000,#67001,#67002,#67003,#67004,#67005,#67006,#67007,#67008,
#67009,#67010,#67011,#67012,#67013,#67014,#67015,#67016,#67017,#67018,#67019,
#67020,#67021,#67022,#67023,#67024,#67025,#67026,#67027,#67028,#67029,#67030,
#67031,#67032,#67033,#67034,#67035,#67036,#67037,#67038,#67039,#67040,#67041,
#67042,#67043,#67044,#67045,#67046),.UNSPECIFIED.,.F.,.F.,(4,3,3,3,3,3,
3,3,3,3,3,3,3,3,3,3,3,3,3,3,3,3,3,3,3,4),(-0.285142803995179,-0.266893522635882,
-0.249971821340761,-0.245887210846563,-0.227911343027248,-0.216815994288942,
-0.213019613595473,-0.209467750355521,-0.191887951046842,-0.174756849476473,
-0.165468891994637,-0.157741505469733,-0.154438883651103,-0.139148553120804,
-0.122062060979163,-0.107562443084732,-0.103576002803925,-0.100472590970432,
-0.0838658743199319,-0.0673520207859246,-0.0520302950453719,-0.0480946476698915,
-0.0321858707070638,-0.0168163861575255,-0.00606511782371399,0.),
 .UNSPECIFIED.);
#4461=B_SPLINE_CURVE_WITH_KNOTS('',3,(#67048,#67049,#67050,#67051,#67052,
#67053,#67054,#67055,#67056,#67057,#67058),.UNSPECIFIED.,.F.,.F.,(4,1,1,
1,1,1,1,1,4),(15.7079632679489,15.8014786182355,16.7880079568995,17.7745372955635,
18.7610666342276,19.7475959728916,20.7341253115556,21.7206546502197,21.9911485751285),
 .UNSPECIFIED.);
#4462=B_SPLINE_CURVE_WITH_KNOTS('',3,(#67059,#67060,#67061,#67062,#67063,
#67064,#67065,#67066,#67067,#67068),.UNSPECIFIED.,.F.,.F.,(4,1,1,1,1,1,
1,4),(15.7079632679489,16.3714588042999,17.357988142964,18.344517481628,
19.331046820292,20.317576158956,21.3041054976201,21.9911485751285),
 .UNSPECIFIED.);
#4463=B_SPLINE_CURVE_WITH_KNOTS('',3,(#67293,#67294,#67295,#67296,#67297,
#67298,#67299,#67300,#67301,#67302,#67303,#67304,#67305,#67306,#67307,#67308,
#67309,#67310,#67311,#67312,#67313,#67314,#67315,#67316,#67317),
 .UNSPECIFIED.,.F.,.F.,(4,3,3,3,3,3,3,3,4),(-10.1357873115491,-9.86529338664031,
-8.87876404797628,-7.89223470931225,-6.90570537064822,-5.91917603198419,
-4.93264669332015,-3.94611735465612,-3.85260200436958),.UNSPECIFIED.);
#4464=B_SPLINE_CURVE_WITH_KNOTS('',3,(#67542,#67543,#67544,#67545,#67546,
#67547,#67548,#67549,#67550,#67551,#67552,#67553,#67554,#67555,#67556,#67557,
#67558,#67559,#67560,#67561,#67562,#67563,#67564,#67565,#67566),
 .UNSPECIFIED.,.F.,.F.,(4,3,3,3,3,3,3,3,4),(7.59274844815661,7.89223470931225,
8.87876404797628,9.86529338664031,10.8518227253043,11.8383520639684,12.8248814026324,
13.8114107412964,13.8759337553362),.UNSPECIFIED.);
#4465=B_SPLINE_CURVE_WITH_KNOTS('',3,(#67569,#67570,#67571,#67572,#67573,
#67574,#67575,#67576,#67577,#67578,#67579,#67580,#67581,#67582,#67583,#67584,
#67585,#67586,#67587,#67588,#67589,#67590,#67591,#67592,#67593,#67594,#67595,
#67596,#67597,#67598,#67599,#67600,#67601,#67602,#67603,#67604,#67605,#67606,
#67607,#67608,#67609,#67610,#67611,#67612,#67613,#67614,#67615,#67616,#67617,
#67618,#67619,#67620,#67621,#67622,#67623,#67624,#67625,#67626,#67627,#67628,
#67629,#67630,#67631,#67632,#67633,#67634,#67635,#67636,#67637,#67638,#67639,
#67640,#67641,#67642,#67643,#67644,#67645,#67646,#67647,#67648,#67649,#67650),
 .UNSPECIFIED.,.F.,.F.,(4,3,3,3,3,3,3,3,3,3,3,3,3,3,3,3,3,3,3,3,3,3,3,3,
3,3,3,4),(-0.28634738033223,-0.271025663162511,-0.260700264029441,-0.25593454384516,
-0.251928842104989,-0.235739854602305,-0.229543718489692,-0.225091279789565,
-0.22164449331224,-0.204610794411351,-0.187823889005095,-0.17905786296708,
-0.174355273957306,-0.171012254735667,-0.168068972463406,-0.153509697708683,
-0.136938517070056,-0.120740406206092,-0.116772701974538,-0.113777021063045,
-0.0964532532245246,-0.0787578798704614,-0.0609068174424322,-0.0568632666880998,
-0.0386442905433222,-0.020585447690582,-0.00735363015834469,0.),
 .UNSPECIFIED.);
#4466=B_SPLINE_CURVE_WITH_KNOTS('',3,(#67651,#67652,#67653,#67654,#67655,
#67656,#67657,#67658,#67659,#67660,#67661,#67662,#67663,#67664,#67665,#67666,
#67667,#67668,#67669,#67670,#67671,#67672,#67673,#67674,#67675,#67676,#67677,
#67678,#67679,#67680,#67681,#67682,#67683,#67684,#67685,#67686,#67687,#67688,
#67689,#67690,#67691,#67692,#67693,#67694,#67695,#67696,#67697,#67698,#67699,
#67700,#67701,#67702,#67703,#67704,#67705,#67706,#67707,#67708,#67709,#67710,
#67711,#67712,#67713,#67714,#67715,#67716,#67717,#67718,#67719,#67720,#67721,
#67722,#67723,#67724,#67725,#67726),.UNSPECIFIED.,.F.,.F.,(4,3,3,3,3,3,
3,3,3,3,3,3,3,3,3,3,3,3,3,3,3,3,3,3,3,4),(-0.285142803995139,-0.266893522635845,
-0.24997166892056,-0.245887163874206,-0.227911314643986,-0.216815969453587,
-0.213019407093492,-0.209467702309002,-0.191887915011948,-0.174756943631577,
-0.165469041969139,-0.157741704377863,-0.154438850709308,-0.139148553120788,
-0.122062043723843,-0.107562427986327,-0.103576078754398,-0.100472601051161,
-0.0838658659032878,-0.0673520484187001,-0.0520303157699535,-0.0480946748290876,
-0.0321859745551226,-0.0168167295145933,-0.00606511782371382,0.),
 .UNSPECIFIED.);
#4467=B_SPLINE_CURVE_WITH_KNOTS('',3,(#67728,#67729,#67730,#67731,#67732,
#67733,#67734,#67735,#67736,#67737,#67738),.UNSPECIFIED.,.F.,.F.,(4,1,1,
1,1,1,1,1,4),(15.7079632679489,15.8014786182354,16.7880079568995,17.7745372955635,
18.7610666342275,19.7475959728916,20.7341253115556,21.7206546502196,21.9911485751285),
 .UNSPECIFIED.);
#4468=B_SPLINE_CURVE_WITH_KNOTS('',3,(#67739,#67740,#67741,#67742,#67743,
#67744,#67745,#67746,#67747,#67748),.UNSPECIFIED.,.F.,.F.,(4,1,1,1,1,1,
1,4),(15.7079632679489,16.3714588042999,17.3579881429639,18.344517481628,
19.331046820292,20.317576158956,21.30410549762,21.9911485751285),
 .UNSPECIFIED.);
#4469=B_SPLINE_CURVE_WITH_KNOTS('',3,(#67973,#67974,#67975,#67976,#67977,
#67978,#67979,#67980,#67981,#67982,#67983,#67984,#67985,#67986,#67987,#67988,
#67989,#67990,#67991,#67992,#67993,#67994,#67995,#67996,#67997),
 .UNSPECIFIED.,.F.,.F.,(4,3,3,3,3,3,3,3,4),(-10.1357873115492,-9.86529338664031,
-8.87876404797628,-7.89223470931225,-6.90570537064822,-5.91917603198418,
-4.93264669332015,-3.94611735465612,-3.85260200436958),.UNSPECIFIED.);
#4470=B_SPLINE_CURVE_WITH_KNOTS('',3,(#68222,#68223,#68224,#68225,#68226,
#68227,#68228,#68229,#68230,#68231,#68232,#68233,#68234,#68235,#68236,#68237,
#68238,#68239,#68240,#68241,#68242,#68243,#68244,#68245,#68246),
 .UNSPECIFIED.,.F.,.F.,(4,3,3,3,3,3,3,3,4),(7.59274844815664,7.89223470931224,
8.87876404797627,9.86529338664031,10.8518227253043,11.8383520639684,12.8248814026324,
13.8114107412964,13.8759337553362),.UNSPECIFIED.);
#4471=B_SPLINE_CURVE_WITH_KNOTS('',3,(#68269,#68270,#68271,#68272,#68273,
#68274,#68275,#68276,#68277,#68278,#68279,#68280,#68281,#68282,#68283,#68284,
#68285,#68286,#68287,#68288,#68289,#68290,#68291,#68292,#68293,#68294,#68295,
#68296,#68297,#68298,#68299,#68300,#68301,#68302,#68303,#68304,#68305,#68306,
#68307,#68308,#68309,#68310,#68311,#68312,#68313,#68314,#68315,#68316,#68317,
#68318,#68319,#68320,#68321,#68322,#68323,#68324,#68325,#68326,#68327,#68328,
#68329,#68330,#68331,#68332,#68333,#68334,#68335,#68336,#68337,#68338,#68339,
#68340,#68341,#68342,#68343,#68344,#68345,#68346,#68347,#68348,#68349,#68350),
 .UNSPECIFIED.,.F.,.F.,(4,3,3,3,3,3,3,3,3,3,3,3,3,3,3,3,3,3,3,3,3,3,3,3,
3,3,3,4),(-0.286347380332213,-0.271025134809031,-0.260698514723011,-0.255927597151592,
-0.251928120089878,-0.23573877571394,-0.229541586624538,-0.225083751316981,
-0.22164175520813,-0.204608740833268,-0.18782191212788,-0.179056502767314,
-0.17435303150997,-0.171008368415998,-0.168068126675904,-0.153509697708681,
-0.136938878241049,-0.120740722230713,-0.116774450511282,-0.113778933942795,
-0.0964554865286861,-0.0787602413272305,-0.0609085885350118,-0.0568635638522563,
-0.0386446388833524,-0.0205858033701879,-0.00735363015835568,0.),
 .UNSPECIFIED.);
#4472=B_SPLINE_CURVE_WITH_KNOTS('',3,(#68351,#68352,#68353,#68354,#68355,
#68356,#68357,#68358,#68359,#68360,#68361,#68362,#68363,#68364,#68365,#68366,
#68367,#68368,#68369,#68370,#68371,#68372,#68373,#68374,#68375,#68376,#68377,
#68378,#68379,#68380,#68381,#68382,#68383,#68384,#68385,#68386,#68387,#68388,
#68389,#68390,#68391,#68392,#68393,#68394,#68395,#68396,#68397,#68398,#68399,
#68400,#68401,#68402,#68403,#68404,#68405,#68406,#68407,#68408,#68409,#68410,
#68411,#68412,#68413,#68414,#68415,#68416,#68417,#68418,#68419,#68420,#68421,
#68422,#68423,#68424,#68425,#68426),.UNSPECIFIED.,.F.,.F.,(4,3,3,3,3,3,
3,3,3,3,3,3,3,3,3,3,3,3,3,3,3,3,3,3,3,4),(-0.285142803995108,-0.266893522635817,
-0.24997148182261,-0.245887106228687,-0.227911281463377,-0.216815940420553,
-0.21301916907798,-0.209467645127105,-0.191887872125524,-0.174757062559625,
-0.165469230797229,-0.157741956079593,-0.154438809603899,-0.13914855312078,
-0.122062023308955,-0.107562410123299,-0.103576177425209,-0.100472613628106,
-0.0838658566327193,-0.0673520867998959,-0.0520303445558493,-0.0480947086188938,
-0.0321861070361084,-0.016817164416105,-0.00606511782370935,0.),
 .UNSPECIFIED.);
#4473=B_SPLINE_CURVE_WITH_KNOTS('',3,(#68428,#68429,#68430,#68431,#68432,
#68433,#68434,#68435,#68436,#68437,#68438),.UNSPECIFIED.,.F.,.F.,(4,1,1,
1,1,1,1,1,4),(15.7079632679489,15.8014786182355,16.7880079568995,17.7745372955635,
18.7610666342275,19.7475959728916,20.7341253115556,21.7206546502196,21.9911485751285),
 .UNSPECIFIED.);
#4474=B_SPLINE_CURVE_WITH_KNOTS('',3,(#68439,#68440,#68441,#68442,#68443,
#68444,#68445,#68446,#68447,#68448),.UNSPECIFIED.,.F.,.F.,(4,1,1,1,1,1,
1,4),(15.7079632679489,16.3714588042999,17.3579881429639,18.344517481628,
19.331046820292,20.317576158956,21.3041054976201,21.9911485751285),
 .UNSPECIFIED.);
#4475=B_SPLINE_CURVE_WITH_KNOTS('',3,(#68673,#68674,#68675,#68676,#68677,
#68678,#68679,#68680,#68681,#68682,#68683,#68684,#68685,#68686,#68687,#68688,
#68689,#68690,#68691,#68692,#68693,#68694,#68695,#68696,#68697,#68698,#68699,
#68700,#68701,#68702,#68703,#68704,#68705,#68706,#68707,#68708,#68709,#68710,
#68711,#68712,#68713,#68714,#68715,#68716,#68717,#68718,#68719,#68720,#68721,
#68722,#68723,#68724,#68725,#68726,#68727,#68728,#68729,#68730,#68731,#68732,
#68733,#68734,#68735,#68736,#68737,#68738,#68739,#68740,#68741,#68742,#68743,
#68744,#68745,#68746,#68747,#68748,#68749,#68750,#68751,#68752,#68753,#68754),
 .UNSPECIFIED.,.F.,.F.,(4,3,3,3,3,3,3,3,3,3,3,3,3,3,3,3,3,3,3,3,3,3,3,3,
3,3,3,4),(0.,0.0151383092197915,0.0309550067692597,0.043639562338757,0.0490032691307438,
0.0520443158185715,0.0683454961299883,0.0849450886251988,0.0968166793002086,
0.101864993851806,0.10487333271342,0.121948986974184,0.132431451325238,
0.149057249647502,0.154031743970893,0.158630823409783,0.175668704761865,
0.193109534814407,0.203698360651626,0.209528438177436,0.213039046077353,
0.231029814287289,0.242727396093505,0.247561053661448,0.251100328242942,
0.269296434630926,0.277820141512155,0.285142803995171),.UNSPECIFIED.);
#4476=B_SPLINE_CURVE_WITH_KNOTS('',3,(#68755,#68756,#68757,#68758,#68759,
#68760,#68761,#68762,#68763,#68764,#68765,#68766,#68767,#68768,#68769,#68770,
#68771,#68772,#68773,#68774,#68775,#68776,#68777,#68778,#68779),
 .UNSPECIFIED.,.F.,.F.,(4,3,3,3,3,3,3,3,4),(-10.1357873115492,-9.86529338664031,
-8.87876404797628,-7.89223470931225,-6.90570537064822,-5.91917603198418,
-4.93264669332016,-3.94611735465613,-3.85260200436962),.UNSPECIFIED.);
#4477=B_SPLINE_CURVE_WITH_KNOTS('',3,(#69004,#69005,#69006,#69007,#69008,
#69009,#69010,#69011,#69012,#69013,#69014,#69015,#69016,#69017,#69018,#69019,
#69020,#69021,#69022,#69023,#69024,#69025,#69026,#69027,#69028),
 .UNSPECIFIED.,.F.,.F.,(4,3,3,3,3,3,3,3,4),(7.59274844815668,7.89223470931225,
8.87876404797628,9.86529338664031,10.8518227253043,11.8383520639684,12.8248814026324,
13.8114107412964,13.8759337553363),.UNSPECIFIED.);
#4478=B_SPLINE_CURVE_WITH_KNOTS('',3,(#69029,#69030,#69031,#69032,#69033,
#69034,#69035,#69036,#69037,#69038,#69039,#69040,#69041,#69042,#69043,#69044,
#69045,#69046,#69047,#69048,#69049,#69050,#69051,#69052,#69053,#69054,#69055,
#69056,#69057,#69058,#69059,#69060,#69061,#69062,#69063,#69064,#69065,#69066,
#69067,#69068,#69069,#69070,#69071,#69072,#69073,#69074,#69075,#69076,#69077,
#69078,#69079,#69080,#69081,#69082,#69083,#69084,#69085,#69086,#69087,#69088,
#69089,#69090,#69091,#69092,#69093,#69094,#69095,#69096,#69097,#69098,#69099,
#69100,#69101,#69102,#69103,#69104,#69105,#69106,#69107),.UNSPECIFIED.,
 .F.,.F.,(4,3,3,3,3,3,3,3,3,3,3,3,3,3,3,3,3,3,3,3,3,3,3,3,3,3,4),(0.,0.0183455177171492,
0.0365842479880597,0.0503567347067014,0.0575064710097589,0.0612717627824107,
0.0790233634825616,0.09641228950938,0.109000252566333,0.115579416560097,
0.118639169849882,0.13548942966781,0.146764141737194,0.163451454243388,
0.168605140809902,0.173128107433064,0.189898748854532,0.206649189230336,
0.217355774416694,0.222872516867536,0.226199915190878,0.242290799536828,
0.252395277141555,0.256089582974829,0.271598152369448,0.280262641786752,
0.286347380332268),.UNSPECIFIED.);
#4479=B_SPLINE_CURVE_WITH_KNOTS('',3,(#69114,#69115,#69116,#69117,#69118,
#69119,#69120,#69121,#69122,#69123,#69124,#69125,#69126,#69127,#69128,#69129,
#69130,#69131,#69132,#69133,#69134,#69135,#69136,#69137,#69138,#69139,#69140,
#69141,#69142,#69143,#69144,#69145,#69146,#69147,#69148,#69149,#69150,#69151,
#69152,#69153,#69154,#69155,#69156,#69157,#69158,#69159,#69160,#69161,#69162,
#69163,#69164,#69165,#69166,#69167,#69168,#69169,#69170,#69171,#69172,#69173,
#69174,#69175,#69176,#69177,#69178,#69179,#69180,#69181,#69182,#69183,#69184,
#69185,#69186,#69187,#69188,#69189,#69190,#69191,#69192,#69193,#69194,#69195),
 .UNSPECIFIED.,.F.,.F.,(4,3,3,3,3,3,3,3,3,3,3,3,3,3,3,3,3,3,3,3,3,3,3,3,
3,3,3,4),(-0.286347380332246,-0.271025677130926,-0.260700310292963,-0.255934727086495,
-0.25192886090893,-0.235739882849757,-0.229543774316331,-0.225091476626096,
-0.221644563245787,-0.204610846861512,-0.187823939473357,-0.179057897575031,
-0.174355331036021,-0.171012353628943,-0.168068993936419,-0.153509697708686,
-0.136938507575535,-0.120740397898387,-0.116772656048653,-0.113776970694075,
-0.0964531944223393,-0.0787578176889207,-0.0609067708062778,-0.0568632588541979,
-0.0386442813548163,-0.0205854383279417,-0.00735363015834907,0.),
 .UNSPECIFIED.);
#4480=B_SPLINE_CURVE_WITH_KNOTS('',3,(#69196,#69197,#69198,#69199,#69200,
#69201,#69202,#69203,#69204,#69205,#69206,#69207,#69208,#69209,#69210,#69211,
#69212,#69213,#69214,#69215,#69216,#69217,#69218,#69219,#69220,#69221,#69222,
#69223,#69224,#69225,#69226,#69227,#69228,#69229,#69230,#69231,#69232,#69233,
#69234,#69235,#69236,#69237,#69238,#69239,#69240,#69241,#69242,#69243,#69244,
#69245,#69246,#69247,#69248,#69249,#69250,#69251,#69252,#69253,#69254,#69255,
#69256,#69257,#69258,#69259,#69260,#69261,#69262,#69263,#69264,#69265,#69266,
#69267,#69268,#69269,#69270,#69271),.UNSPECIFIED.,.F.,.F.,(4,3,3,3,3,3,
3,3,3,3,3,3,3,3,3,3,3,3,3,3,3,3,3,3,3,4),(-0.285142803995095,-0.266893522635806,
-0.24997167290184,-0.245887165090684,-0.227911315359866,-0.21681597007998,
-0.213019412352564,-0.209467703547662,-0.191887915940942,-0.174756941142404,
-0.165469038009959,-0.157741699115177,-0.15443885155403,-0.139148553120782,
-0.122062044167413,-0.10756242837445,-0.103576076720583,-0.100472600797313,
-0.0838658661242367,-0.0673520476672987,-0.0520303152064016,-0.0480946741240866,
-0.0321859718066127,-0.016816720434557,-0.00606511782371032,0.),
 .UNSPECIFIED.);
#4481=B_SPLINE_CURVE_WITH_KNOTS('',3,(#69273,#69274,#69275,#69276,#69277,
#69278,#69279,#69280,#69281,#69282,#69283),.UNSPECIFIED.,.F.,.F.,(4,1,1,
1,1,1,1,1,4),(15.7079632679489,15.8014786182355,16.7880079568995,17.7745372955635,
18.7610666342276,19.7475959728916,20.7341253115556,21.7206546502197,21.9911485751285),
 .UNSPECIFIED.);
#4482=B_SPLINE_CURVE_WITH_KNOTS('',3,(#69284,#69285,#69286,#69287,#69288,
#69289,#69290,#69291,#69292,#69293),.UNSPECIFIED.,.F.,.F.,(4,1,1,1,1,1,
1,4),(15.7079632679489,16.3714588042999,17.357988142964,18.344517481628,
19.331046820292,20.317576158956,21.3041054976201,21.9911485751285),
 .UNSPECIFIED.);
#4483=B_SPLINE_CURVE_WITH_KNOTS('',3,(#69518,#69519,#69520,#69521,#69522,
#69523,#69524,#69525,#69526,#69527,#69528,#69529,#69530,#69531,#69532,#69533,
#69534,#69535,#69536,#69537,#69538,#69539,#69540,#69541,#69542),
 .UNSPECIFIED.,.F.,.F.,(4,3,3,3,3,3,3,3,4),(-10.1357873115492,-9.8652933866403,
-8.87876404797628,-7.89223470931224,-6.90570537064821,-5.91917603198418,
-4.93264669332015,-3.94611735465612,-3.85260200436958),.UNSPECIFIED.);
#4484=B_SPLINE_CURVE_WITH_KNOTS('',3,(#69767,#69768,#69769,#69770,#69771,
#69772,#69773,#69774,#69775,#69776,#69777,#69778,#69779,#69780,#69781,#69782,
#69783,#69784,#69785,#69786,#69787,#69788,#69789,#69790,#69791),
 .UNSPECIFIED.,.F.,.F.,(4,3,3,3,3,3,3,3,4),(7.59274844815664,7.89223470931223,
8.87876404797627,9.8652933866403,10.8518227253043,11.8383520639684,12.8248814026324,
13.8114107412964,13.8759337553362),.UNSPECIFIED.);
#4485=B_SPLINE_CURVE_WITH_KNOTS('',3,(#69883,#69884,#69885,#69886,#69887,
#69888),.UNSPECIFIED.,.F.,.F.,(4,2,4),(-1.6,-0.8,0.),.UNSPECIFIED.);
#4486=B_SPLINE_CURVE_WITH_KNOTS('',3,(#69894,#69895,#69896,#69897,#69898,
#69899),.UNSPECIFIED.,.F.,.F.,(4,2,4),(-1.6,-0.8,0.),.UNSPECIFIED.);
#4487=B_SPLINE_CURVE_WITH_KNOTS('',3,(#69911,#69912,#69913,#69914,#69915,
#69916),.UNSPECIFIED.,.F.,.F.,(4,2,4),(-1.6,-0.8,0.),.UNSPECIFIED.);
#4488=B_SPLINE_CURVE_WITH_KNOTS('',3,(#69930,#69931,#69932,#69933,#69934,
#69935),.UNSPECIFIED.,.F.,.F.,(4,2,4),(-1.6,-0.8,0.),.UNSPECIFIED.);
#4489=B_SPLINE_CURVE_WITH_KNOTS('',3,(#69939,#69940,#69941,#69942,#69943,
#69944),.UNSPECIFIED.,.F.,.F.,(4,2,4),(-1.6,-0.8,0.),.UNSPECIFIED.);
#4490=B_SPLINE_CURVE_WITH_KNOTS('',3,(#69958,#69959,#69960,#69961,#69962,
#69963),.UNSPECIFIED.,.F.,.F.,(4,2,4),(-1.6,-0.8,0.),.UNSPECIFIED.);
#4491=B_SPLINE_CURVE_WITH_KNOTS('',3,(#69967,#69968,#69969,#69970,#69971,
#69972),.UNSPECIFIED.,.F.,.F.,(4,2,4),(-1.6,-0.8,0.),.UNSPECIFIED.);
#4492=B_SPLINE_CURVE_WITH_KNOTS('',3,(#69986,#69987,#69988,#69989,#69990,
#69991),.UNSPECIFIED.,.F.,.F.,(4,2,4),(-1.6,-0.8,0.),.UNSPECIFIED.);
#4493=B_SPLINE_CURVE_WITH_KNOTS('',3,(#69995,#69996,#69997,#69998,#69999,
#70000),.UNSPECIFIED.,.F.,.F.,(4,2,4),(-1.6,-0.8,0.),.UNSPECIFIED.);
#4494=B_SPLINE_CURVE_WITH_KNOTS('',3,(#70006,#70007,#70008,#70009,#70010,
#70011),.UNSPECIFIED.,.F.,.F.,(4,2,4),(-1.6,-0.8,0.),.UNSPECIFIED.);
#4495=B_SPLINE_CURVE_WITH_KNOTS('',3,(#72032,#72033,#72034,#72035,#72036,
#72037,#72038,#72039,#72040,#72041,#72042,#72043,#72044,#72045,#72046,#72047,
#72048,#72049,#72050,#72051,#72052,#72053,#72054,#72055,#72056,#72057,#72058,
#72059),.UNSPECIFIED.,.F.,.F.,(4,3,3,3,3,3,3,3,3,4),(-1.95245002670228,
-1.7083937733645,-1.4646957205336,-1.22078701844286,-0.97666712493882,-0.732202856815818,
-0.487562123458939,-0.24378106172947,-0.0832160650278452,0.),
 .UNSPECIFIED.);
#4496=B_SPLINE_CURVE_WITH_KNOTS('',3,(#74072,#74073,#74074,#74075,#74076,
#74077,#74078,#74079,#74080,#74081,#74082,#74083,#74084,#74085,#74086,#74087,
#74088,#74089,#74090,#74091,#74092,#74093,#74094,#74095,#74096,#74097,#74098,
#74099),.UNSPECIFIED.,.F.,.F.,(4,3,3,3,3,3,3,3,3,4),(-1.95245002774481,
-1.70839377427671,-1.46469569943071,-1.22078743097454,-0.976667451078158,
-0.732203245920036,-0.487562280383025,-0.243781140191512,-0.0832160609216453,
0.),.UNSPECIFIED.);
#4497=B_SPLINE_CURVE_WITH_KNOTS('',3,(#76113,#76114,#76115,#76116),
 .UNSPECIFIED.,.F.,.F.,(4,4),(-3.33933214605564,-2.59563630155322),
 .UNSPECIFIED.);
#4498=B_SPLINE_CURVE_WITH_KNOTS('',3,(#78128,#78129,#78130,#78131,#78132,
#78133,#78134,#78135,#78136,#78137,#78138,#78139,#78140,#78141,#78142,#78143,
#78144,#78145,#78146,#78147,#78148,#78149,#78150,#78151,#78152,#78153,#78154,
#78155),.UNSPECIFIED.,.F.,.F.,(4,3,3,3,3,3,3,3,3,4),(-1.95245003576054,
-1.70839378129047,-1.46469576962979,-1.22078693523904,-0.976667204248944,
-0.732202830545938,-0.487562139320946,-0.243781069660473,-0.0832159489912239,
0.),.UNSPECIFIED.);
#4499=B_SPLINE_CURVE_WITH_KNOTS('',3,(#80169,#80170,#80171,#80172),
 .UNSPECIFIED.,.F.,.F.,(4,4),(-3.3393321613758,-2.59563631294433),
 .UNSPECIFIED.);
#4500=B_SPLINE_CURVE_WITH_KNOTS('',3,(#82184,#82185,#82186,#82187,#82188,
#82189,#82190,#82191,#82192,#82193,#82194,#82195,#82196,#82197,#82198,#82199,
#82200,#82201,#82202,#82203,#82204,#82205,#82206,#82207,#82208,#82209,#82210,
#82211),.UNSPECIFIED.,.F.,.F.,(4,3,3,3,3,3,3,3,3,4),(-1.95245002395252,
-1.70839377095845,-1.46469574316389,-1.22078724480627,-0.97666698126864,
-0.732202626712538,-0.487561565272828,-0.243780782636414,-0.083215645232922,
0.),.UNSPECIFIED.);
#4501=B_SPLINE_CURVE_WITH_KNOTS('',3,(#84225,#84226,#84227,#84228),
 .UNSPECIFIED.,.F.,.F.,(4,4),(-3.33933214077653,-2.59563629688202),
 .UNSPECIFIED.);
#4502=B_SPLINE_CURVE_WITH_KNOTS('',3,(#86240,#86241,#86242,#86243,#86244,
#86245,#86246,#86247,#86248,#86249,#86250,#86251,#86252,#86253,#86254,#86255,
#86256,#86257,#86258,#86259,#86260,#86261,#86262,#86263,#86264,#86265,#86266,
#86267),.UNSPECIFIED.,.F.,.F.,(4,3,3,3,3,3,3,3,3,4),(-1.95245003704233,
-1.70839378241204,-1.46469565989463,-1.22078739198828,-0.97666741362503,
-0.732203206774895,-0.487562540884707,-0.243781270442354,-0.0832161724652675,
0.),.UNSPECIFIED.);
#4503=B_SPLINE_CURVE_WITH_KNOTS('',3,(#86271,#86272,#86273,#86274,#86275,
#86276),.UNSPECIFIED.,.F.,.F.,(4,2,4),(-1.6,-0.8,0.),.UNSPECIFIED.);
#4504=B_SPLINE_CURVE_WITH_KNOTS('',3,(#86282,#86283,#86284,#86285,#86286,
#86287),.UNSPECIFIED.,.F.,.F.,(4,2,4),(-1.6,-0.8,0.),.UNSPECIFIED.);
#4505=B_SPLINE_CURVE_WITH_KNOTS('',3,(#88308,#88309,#88310,#88311,#88312,
#88313,#88314,#88315,#88316,#88317,#88318,#88319,#88320,#88321,#88322,#88323,
#88324,#88325,#88326,#88327,#88328,#88329,#88330,#88331,#88332,#88333,#88334,
#88335),.UNSPECIFIED.,.F.,.F.,(4,3,3,3,3,3,3,3,3,4),(-1.95245003867437,
-1.70839378384007,-1.46469580928766,-1.22078735724755,-0.976667179798372,
-0.732202890769605,-0.487561952370783,-0.243780976185391,-0.0832159842231958,
0.),.UNSPECIFIED.);
#4506=B_SPLINE_CURVE_WITH_KNOTS('',3,(#88369,#88370,#88371,#88372),
 .UNSPECIFIED.,.F.,.F.,(4,4),(-3.3393321486059,-2.59563630156681),
 .UNSPECIFIED.);
#4507=B_SPLINE_CURVE_WITH_KNOTS('',3,(#88379,#88380,#88381,#88382),
 .UNSPECIFIED.,.F.,.F.,(4,4),(-3.33933216373174,-2.59563631465892),
 .UNSPECIFIED.);
#4508=B_SPLINE_CURVE_WITH_KNOTS('',3,(#88389,#88390,#88391,#88392),
 .UNSPECIFIED.,.F.,.F.,(4,4),(-3.33933216499304,-2.59563631632113),
 .UNSPECIFIED.);
#5008=LINE('',#52675,#5912);
#5009=LINE('',#52684,#5913);
#5010=LINE('',#52705,#5914);
#5011=LINE('',#52756,#5915);
#5012=LINE('',#52807,#5916);
#5013=LINE('',#52855,#5917);
#5014=LINE('',#52906,#5918);
#5015=LINE('',#52957,#5919);
#5016=LINE('',#53005,#5920);
#5017=LINE('',#53044,#5921);
#5018=LINE('',#53068,#5922);
#5019=LINE('',#53092,#5923);
#5020=LINE('',#53117,#5924);
#5021=LINE('',#53142,#5925);
#5022=LINE('',#53166,#5926);
#5023=LINE('',#53191,#5927);
#5024=LINE('',#53216,#5928);
#5025=LINE('',#53233,#5929);
#5026=LINE('',#53242,#5930);
#5027=LINE('',#53263,#5931);
#5028=LINE('',#53314,#5932);
#5029=LINE('',#53365,#5933);
#5030=LINE('',#53413,#5934);
#5031=LINE('',#53464,#5935);
#5032=LINE('',#53515,#5936);
#5033=LINE('',#53563,#5937);
#5034=LINE('',#53602,#5938);
#5035=LINE('',#53626,#5939);
#5036=LINE('',#53650,#5940);
#5037=LINE('',#53675,#5941);
#5038=LINE('',#53700,#5942);
#5039=LINE('',#53724,#5943);
#5040=LINE('',#53749,#5944);
#5041=LINE('',#53774,#5945);
#5042=LINE('',#53791,#5946);
#5043=LINE('',#53800,#5947);
#5044=LINE('',#53821,#5948);
#5045=LINE('',#53872,#5949);
#5046=LINE('',#53923,#5950);
#5047=LINE('',#53971,#5951);
#5048=LINE('',#54022,#5952);
#5049=LINE('',#54073,#5953);
#5050=LINE('',#54121,#5954);
#5051=LINE('',#54160,#5955);
#5052=LINE('',#54184,#5956);
#5053=LINE('',#54208,#5957);
#5054=LINE('',#54233,#5958);
#5055=LINE('',#54258,#5959);
#5056=LINE('',#54282,#5960);
#5057=LINE('',#54307,#5961);
#5058=LINE('',#54332,#5962);
#5059=LINE('',#54349,#5963);
#5060=LINE('',#54358,#5964);
#5061=LINE('',#54379,#5965);
#5062=LINE('',#54430,#5966);
#5063=LINE('',#54481,#5967);
#5064=LINE('',#54529,#5968);
#5065=LINE('',#54580,#5969);
#5066=LINE('',#54631,#5970);
#5067=LINE('',#54679,#5971);
#5068=LINE('',#54718,#5972);
#5069=LINE('',#54742,#5973);
#5070=LINE('',#54766,#5974);
#5071=LINE('',#54791,#5975);
#5072=LINE('',#54816,#5976);
#5073=LINE('',#54840,#5977);
#5074=LINE('',#54865,#5978);
#5075=LINE('',#54890,#5979);
#5076=LINE('',#54907,#5980);
#5077=LINE('',#54916,#5981);
#5078=LINE('',#54937,#5982);
#5079=LINE('',#54988,#5983);
#5080=LINE('',#55039,#5984);
#5081=LINE('',#55087,#5985);
#5082=LINE('',#55138,#5986);
#5083=LINE('',#55189,#5987);
#5084=LINE('',#55237,#5988);
#5085=LINE('',#55276,#5989);
#5086=LINE('',#55300,#5990);
#5087=LINE('',#55324,#5991);
#5088=LINE('',#55349,#5992);
#5089=LINE('',#55374,#5993);
#5090=LINE('',#55398,#5994);
#5091=LINE('',#55423,#5995);
#5092=LINE('',#55448,#5996);
#5093=LINE('',#55465,#5997);
#5094=LINE('',#55474,#5998);
#5095=LINE('',#55495,#5999);
#5096=LINE('',#55546,#6000);
#5097=LINE('',#55597,#6001);
#5098=LINE('',#55645,#6002);
#5099=LINE('',#55696,#6003);
#5100=LINE('',#55747,#6004);
#5101=LINE('',#55795,#6005);
#5102=LINE('',#55834,#6006);
#5103=LINE('',#55858,#6007);
#5104=LINE('',#55882,#6008);
#5105=LINE('',#55907,#6009);
#5106=LINE('',#55932,#6010);
#5107=LINE('',#55956,#6011);
#5108=LINE('',#55981,#6012);
#5109=LINE('',#56006,#6013);
#5110=LINE('',#56023,#6014);
#5111=LINE('',#56032,#6015);
#5112=LINE('',#56053,#6016);
#5113=LINE('',#56104,#6017);
#5114=LINE('',#56155,#6018);
#5115=LINE('',#56203,#6019);
#5116=LINE('',#56254,#6020);
#5117=LINE('',#56305,#6021);
#5118=LINE('',#56353,#6022);
#5119=LINE('',#56392,#6023);
#5120=LINE('',#56416,#6024);
#5121=LINE('',#56440,#6025);
#5122=LINE('',#56465,#6026);
#5123=LINE('',#56490,#6027);
#5124=LINE('',#56514,#6028);
#5125=LINE('',#56539,#6029);
#5126=LINE('',#56564,#6030);
#5127=LINE('',#56581,#6031);
#5128=LINE('',#56590,#6032);
#5129=LINE('',#56611,#6033);
#5130=LINE('',#56662,#6034);
#5131=LINE('',#56713,#6035);
#5132=LINE('',#56761,#6036);
#5133=LINE('',#56812,#6037);
#5134=LINE('',#56863,#6038);
#5135=LINE('',#56911,#6039);
#5136=LINE('',#56950,#6040);
#5137=LINE('',#56974,#6041);
#5138=LINE('',#56998,#6042);
#5139=LINE('',#57023,#6043);
#5140=LINE('',#57048,#6044);
#5141=LINE('',#57072,#6045);
#5142=LINE('',#57097,#6046);
#5143=LINE('',#57122,#6047);
#5144=LINE('',#57139,#6048);
#5145=LINE('',#57148,#6049);
#5146=LINE('',#57169,#6050);
#5147=LINE('',#57220,#6051);
#5148=LINE('',#57271,#6052);
#5149=LINE('',#57319,#6053);
#5150=LINE('',#57370,#6054);
#5151=LINE('',#57421,#6055);
#5152=LINE('',#57469,#6056);
#5153=LINE('',#57508,#6057);
#5154=LINE('',#57532,#6058);
#5155=LINE('',#57556,#6059);
#5156=LINE('',#57581,#6060);
#5157=LINE('',#57606,#6061);
#5158=LINE('',#57630,#6062);
#5159=LINE('',#57655,#6063);
#5160=LINE('',#57680,#6064);
#5161=LINE('',#57697,#6065);
#5162=LINE('',#57706,#6066);
#5163=LINE('',#57727,#6067);
#5164=LINE('',#57778,#6068);
#5165=LINE('',#57829,#6069);
#5166=LINE('',#57877,#6070);
#5167=LINE('',#57928,#6071);
#5168=LINE('',#57979,#6072);
#5169=LINE('',#58027,#6073);
#5170=LINE('',#58066,#6074);
#5171=LINE('',#58090,#6075);
#5172=LINE('',#58114,#6076);
#5173=LINE('',#58139,#6077);
#5174=LINE('',#58164,#6078);
#5175=LINE('',#58188,#6079);
#5176=LINE('',#58213,#6080);
#5177=LINE('',#58238,#6081);
#5178=LINE('',#58255,#6082);
#5179=LINE('',#58264,#6083);
#5180=LINE('',#58285,#6084);
#5181=LINE('',#58336,#6085);
#5182=LINE('',#58387,#6086);
#5183=LINE('',#58435,#6087);
#5184=LINE('',#58486,#6088);
#5185=LINE('',#58537,#6089);
#5186=LINE('',#58585,#6090);
#5187=LINE('',#58624,#6091);
#5188=LINE('',#58648,#6092);
#5189=LINE('',#58672,#6093);
#5190=LINE('',#58697,#6094);
#5191=LINE('',#58722,#6095);
#5192=LINE('',#58746,#6096);
#5193=LINE('',#58771,#6097);
#5194=LINE('',#58796,#6098);
#5195=LINE('',#58813,#6099);
#5196=LINE('',#58822,#6100);
#5197=LINE('',#58843,#6101);
#5198=LINE('',#58894,#6102);
#5199=LINE('',#58945,#6103);
#5200=LINE('',#58993,#6104);
#5201=LINE('',#59044,#6105);
#5202=LINE('',#59095,#6106);
#5203=LINE('',#59143,#6107);
#5204=LINE('',#59182,#6108);
#5205=LINE('',#59206,#6109);
#5206=LINE('',#59230,#6110);
#5207=LINE('',#59255,#6111);
#5208=LINE('',#59280,#6112);
#5209=LINE('',#59304,#6113);
#5210=LINE('',#59329,#6114);
#5211=LINE('',#59354,#6115);
#5212=LINE('',#59371,#6116);
#5213=LINE('',#59373,#6117);
#5214=LINE('',#59375,#6118);
#5215=LINE('',#59376,#6119);
#5216=LINE('',#59379,#6120);
#5217=LINE('',#59381,#6121);
#5218=LINE('',#59382,#6122);
#5219=LINE('',#59386,#6123);
#5220=LINE('',#59387,#6124);
#5221=LINE('',#59388,#6125);
#5222=LINE('',#59421,#6126);
#5223=LINE('',#59432,#6127);
#5224=LINE('',#59434,#6128);
#5225=LINE('',#59436,#6129);
#5226=LINE('',#59438,#6130);
#5227=LINE('',#59469,#6131);
#5228=LINE('',#59480,#6132);
#5229=LINE('',#59482,#6133);
#5230=LINE('',#59484,#6134);
#5231=LINE('',#59486,#6135);
#5232=LINE('',#59517,#6136);
#5233=LINE('',#59528,#6137);
#5234=LINE('',#59530,#6138);
#5235=LINE('',#59532,#6139);
#5236=LINE('',#59534,#6140);
#5237=LINE('',#59543,#6141);
#5238=LINE('',#59554,#6142);
#5239=LINE('',#59556,#6143);
#5240=LINE('',#59558,#6144);
#5241=LINE('',#59560,#6145);
#5242=LINE('',#59591,#6146);
#5243=LINE('',#59602,#6147);
#5244=LINE('',#59604,#6148);
#5245=LINE('',#59606,#6149);
#5246=LINE('',#59608,#6150);
#5247=LINE('',#59639,#6151);
#5248=LINE('',#59650,#6152);
#5249=LINE('',#59652,#6153);
#5250=LINE('',#59654,#6154);
#5251=LINE('',#59655,#6155);
#5252=LINE('',#64829,#6156);
#5253=LINE('',#64831,#6157);
#5254=LINE('',#64833,#6158);
#5255=LINE('',#64835,#6159);
#5256=LINE('',#64837,#6160);
#5257=LINE('',#64839,#6161);
#5258=LINE('',#64841,#6162);
#5259=LINE('',#64843,#6163);
#5260=LINE('',#64845,#6164);
#5261=LINE('',#64847,#6165);
#5262=LINE('',#68249,#6166);
#5263=LINE('',#68251,#6167);
#5264=LINE('',#68253,#6168);
#5265=LINE('',#68255,#6169);
#5266=LINE('',#68257,#6170);
#5267=LINE('',#68259,#6171);
#5268=LINE('',#68261,#6172);
#5269=LINE('',#68263,#6173);
#5270=LINE('',#68265,#6174);
#5271=LINE('',#68267,#6175);
#5272=LINE('',#69110,#6176);
#5273=LINE('',#69112,#6177);
#5274=LINE('',#69794,#6178);
#5275=LINE('',#69796,#6179);
#5276=LINE('',#69801,#6180);
#5277=LINE('',#69806,#6181);
#5278=LINE('',#69808,#6182);
#5279=LINE('',#69815,#6183);
#5280=LINE('',#69820,#6184);
#5281=LINE('',#69822,#6185);
#5282=LINE('',#69829,#6186);
#5283=LINE('',#69834,#6187);
#5284=LINE('',#69836,#6188);
#5285=LINE('',#69843,#6189);
#5286=LINE('',#69848,#6190);
#5287=LINE('',#69850,#6191);
#5288=LINE('',#69857,#6192);
#5289=LINE('',#69862,#6193);
#5290=LINE('',#69864,#6194);
#5291=LINE('',#69871,#6195);
#5292=LINE('',#69876,#6196);
#5293=LINE('',#69878,#6197);
#5294=LINE('',#69890,#6198);
#5295=LINE('',#69891,#6199);
#5296=LINE('',#69901,#6200);
#5297=LINE('',#69902,#6201);
#5298=LINE('',#69905,#6202);
#5299=LINE('',#69906,#6203);
#5300=LINE('',#69908,#6204);
#5301=LINE('',#69918,#6205);
#5302=LINE('',#69919,#6206);
#5303=LINE('',#69922,#6207);
#5304=LINE('',#69923,#6208);
#5305=LINE('',#69926,#6209);
#5306=LINE('',#69927,#6210);
#5307=LINE('',#69936,#6211);
#5308=LINE('',#69946,#6212);
#5309=LINE('',#69947,#6213);
#5310=LINE('',#69950,#6214);
#5311=LINE('',#69951,#6215);
#5312=LINE('',#69954,#6216);
#5313=LINE('',#69955,#6217);
#5314=LINE('',#69964,#6218);
#5315=LINE('',#69974,#6219);
#5316=LINE('',#69975,#6220);
#5317=LINE('',#69978,#6221);
#5318=LINE('',#69979,#6222);
#5319=LINE('',#69982,#6223);
#5320=LINE('',#69983,#6224);
#5321=LINE('',#69992,#6225);
#5322=LINE('',#70002,#6226);
#5323=LINE('',#70003,#6227);
#5324=LINE('',#70013,#6228);
#5325=LINE('',#70014,#6229);
#5326=LINE('',#70017,#6230);
#5327=LINE('',#70018,#6231);
#5328=LINE('',#70020,#6232);
#5329=LINE('',#72060,#6233);
#5330=LINE('',#74100,#6234);
#5331=LINE('',#76112,#6235);
#5332=LINE('',#78156,#6236);
#5333=LINE('',#80168,#6237);
#5334=LINE('',#82212,#6238);
#5335=LINE('',#84224,#6239);
#5336=LINE('',#86268,#6240);
#5337=LINE('',#86278,#6241);
#5338=LINE('',#86279,#6242);
#5339=LINE('',#86289,#6243);
#5340=LINE('',#86290,#6244);
#5341=LINE('',#86293,#6245);
#5342=LINE('',#86294,#6246);
#5343=LINE('',#86296,#6247);
#5344=LINE('',#88336,#6248);
#5345=LINE('',#88339,#6249);
#5346=LINE('',#88343,#6250);
#5347=LINE('',#88346,#6251);
#5348=LINE('',#88349,#6252);
#5349=LINE('',#88353,#6253);
#5350=LINE('',#88356,#6254);
#5351=LINE('',#88359,#6255);
#5352=LINE('',#88363,#6256);
#5353=LINE('',#88366,#6257);
#5354=LINE('',#88377,#6258);
#5355=LINE('',#88387,#6259);
#5356=LINE('',#88397,#6260);
#5357=LINE('',#88400,#6261);
#5358=LINE('',#88402,#6262);
#5359=LINE('',#88404,#6263);
#5360=LINE('',#90416,#6264);
#5361=LINE('',#90418,#6265);
#5362=LINE('',#90420,#6266);
#5363=LINE('',#92432,#6267);
#5364=LINE('',#94443,#6268);
#5365=LINE('',#94445,#6269);
#5912=VECTOR('',#21185,1.5);
#5913=VECTOR('',#21188,1.5);
#5914=VECTOR('',#21199,1.5);
#5915=VECTOR('',#21202,1.5);
#5916=VECTOR('',#21205,1.5);
#5917=VECTOR('',#21208,1.5);
#5918=VECTOR('',#21211,1.5);
#5919=VECTOR('',#21214,1.5);
#5920=VECTOR('',#21217,1.5);
#5921=VECTOR('',#21222,1.543);
#5922=VECTOR('',#21227,1.543);
#5923=VECTOR('',#21230,1.543);
#5924=VECTOR('',#21233,1.543);
#5925=VECTOR('',#21236,1.543);
#5926=VECTOR('',#21239,1.543);
#5927=VECTOR('',#21242,1.543);
#5928=VECTOR('',#21245,1.543);
#5929=VECTOR('',#21250,1.5);
#5930=VECTOR('',#21253,1.5);
#5931=VECTOR('',#21264,1.5);
#5932=VECTOR('',#21267,1.5);
#5933=VECTOR('',#21270,1.5);
#5934=VECTOR('',#21273,1.5);
#5935=VECTOR('',#21276,1.5);
#5936=VECTOR('',#21279,1.5);
#5937=VECTOR('',#21282,1.5);
#5938=VECTOR('',#21287,1.54299999999999);
#5939=VECTOR('',#21292,1.54299999999999);
#5940=VECTOR('',#21295,1.54299999999999);
#5941=VECTOR('',#21298,1.54299999999999);
#5942=VECTOR('',#21301,1.54299999999999);
#5943=VECTOR('',#21304,1.54299999999999);
#5944=VECTOR('',#21307,1.54299999999999);
#5945=VECTOR('',#21310,1.54299999999999);
#5946=VECTOR('',#21315,1.5);
#5947=VECTOR('',#21318,1.5);
#5948=VECTOR('',#21329,1.5);
#5949=VECTOR('',#21332,1.5);
#5950=VECTOR('',#21335,1.5);
#5951=VECTOR('',#21338,1.5);
#5952=VECTOR('',#21341,1.5);
#5953=VECTOR('',#21344,1.5);
#5954=VECTOR('',#21347,1.5);
#5955=VECTOR('',#21352,1.543);
#5956=VECTOR('',#21357,1.543);
#5957=VECTOR('',#21360,1.543);
#5958=VECTOR('',#21363,1.543);
#5959=VECTOR('',#21366,1.543);
#5960=VECTOR('',#21369,1.543);
#5961=VECTOR('',#21372,1.543);
#5962=VECTOR('',#21375,1.543);
#5963=VECTOR('',#21380,1.5);
#5964=VECTOR('',#21383,1.5);
#5965=VECTOR('',#21394,1.5);
#5966=VECTOR('',#21397,1.5);
#5967=VECTOR('',#21400,1.5);
#5968=VECTOR('',#21403,1.5);
#5969=VECTOR('',#21406,1.5);
#5970=VECTOR('',#21409,1.5);
#5971=VECTOR('',#21412,1.5);
#5972=VECTOR('',#21417,1.543);
#5973=VECTOR('',#21422,1.543);
#5974=VECTOR('',#21425,1.543);
#5975=VECTOR('',#21428,1.543);
#5976=VECTOR('',#21431,1.543);
#5977=VECTOR('',#21434,1.543);
#5978=VECTOR('',#21437,1.543);
#5979=VECTOR('',#21440,1.543);
#5980=VECTOR('',#21445,1.5);
#5981=VECTOR('',#21448,1.5);
#5982=VECTOR('',#21459,1.5);
#5983=VECTOR('',#21462,1.5);
#5984=VECTOR('',#21465,1.5);
#5985=VECTOR('',#21468,1.5);
#5986=VECTOR('',#21471,1.5);
#5987=VECTOR('',#21474,1.5);
#5988=VECTOR('',#21477,1.5);
#5989=VECTOR('',#21482,1.54300000000001);
#5990=VECTOR('',#21487,1.54300000000001);
#5991=VECTOR('',#21490,1.54300000000001);
#5992=VECTOR('',#21493,1.54300000000001);
#5993=VECTOR('',#21496,1.54300000000001);
#5994=VECTOR('',#21499,1.54300000000001);
#5995=VECTOR('',#21502,1.54300000000001);
#5996=VECTOR('',#21505,1.54300000000001);
#5997=VECTOR('',#21510,1.5);
#5998=VECTOR('',#21513,1.5);
#5999=VECTOR('',#21524,1.5);
#6000=VECTOR('',#21527,1.5);
#6001=VECTOR('',#21530,1.5);
#6002=VECTOR('',#21533,1.5);
#6003=VECTOR('',#21536,1.5);
#6004=VECTOR('',#21539,1.5);
#6005=VECTOR('',#21542,1.5);
#6006=VECTOR('',#21547,1.54300000000001);
#6007=VECTOR('',#21552,1.54300000000001);
#6008=VECTOR('',#21555,1.54300000000001);
#6009=VECTOR('',#21558,1.54300000000001);
#6010=VECTOR('',#21561,1.54300000000001);
#6011=VECTOR('',#21564,1.54300000000001);
#6012=VECTOR('',#21567,1.54300000000001);
#6013=VECTOR('',#21570,1.54300000000001);
#6014=VECTOR('',#21575,1.5);
#6015=VECTOR('',#21578,1.5);
#6016=VECTOR('',#21589,1.5);
#6017=VECTOR('',#21592,1.5);
#6018=VECTOR('',#21595,1.5);
#6019=VECTOR('',#21598,1.5);
#6020=VECTOR('',#21601,1.5);
#6021=VECTOR('',#21604,1.5);
#6022=VECTOR('',#21607,1.5);
#6023=VECTOR('',#21612,1.543);
#6024=VECTOR('',#21617,1.543);
#6025=VECTOR('',#21620,1.543);
#6026=VECTOR('',#21623,1.543);
#6027=VECTOR('',#21626,1.543);
#6028=VECTOR('',#21629,1.543);
#6029=VECTOR('',#21632,1.543);
#6030=VECTOR('',#21635,1.543);
#6031=VECTOR('',#21640,1.5);
#6032=VECTOR('',#21643,1.5);
#6033=VECTOR('',#21654,1.5);
#6034=VECTOR('',#21657,1.5);
#6035=VECTOR('',#21660,1.5);
#6036=VECTOR('',#21663,1.5);
#6037=VECTOR('',#21666,1.5);
#6038=VECTOR('',#21669,1.5);
#6039=VECTOR('',#21672,1.5);
#6040=VECTOR('',#21677,1.54300000000001);
#6041=VECTOR('',#21682,1.54300000000001);
#6042=VECTOR('',#21685,1.54300000000001);
#6043=VECTOR('',#21688,1.54300000000001);
#6044=VECTOR('',#21691,1.54300000000001);
#6045=VECTOR('',#21694,1.54300000000001);
#6046=VECTOR('',#21697,1.54300000000001);
#6047=VECTOR('',#21700,1.54300000000001);
#6048=VECTOR('',#21705,1.5);
#6049=VECTOR('',#21708,1.5);
#6050=VECTOR('',#21719,1.5);
#6051=VECTOR('',#21722,1.5);
#6052=VECTOR('',#21725,1.5);
#6053=VECTOR('',#21728,1.5);
#6054=VECTOR('',#21731,1.5);
#6055=VECTOR('',#21734,1.5);
#6056=VECTOR('',#21737,1.5);
#6057=VECTOR('',#21742,1.54300000000001);
#6058=VECTOR('',#21747,1.54300000000001);
#6059=VECTOR('',#21750,1.54300000000001);
#6060=VECTOR('',#21753,1.54300000000001);
#6061=VECTOR('',#21756,1.54300000000001);
#6062=VECTOR('',#21759,1.54300000000001);
#6063=VECTOR('',#21762,1.54300000000001);
#6064=VECTOR('',#21765,1.54300000000001);
#6065=VECTOR('',#21770,1.5);
#6066=VECTOR('',#21773,1.5);
#6067=VECTOR('',#21784,1.5);
#6068=VECTOR('',#21787,1.5);
#6069=VECTOR('',#21790,1.5);
#6070=VECTOR('',#21793,1.5);
#6071=VECTOR('',#21796,1.5);
#6072=VECTOR('',#21799,1.5);
#6073=VECTOR('',#21802,1.5);
#6074=VECTOR('',#21807,1.543);
#6075=VECTOR('',#21812,1.543);
#6076=VECTOR('',#21815,1.543);
#6077=VECTOR('',#21818,1.543);
#6078=VECTOR('',#21821,1.543);
#6079=VECTOR('',#21824,1.543);
#6080=VECTOR('',#21827,1.543);
#6081=VECTOR('',#21830,1.543);
#6082=VECTOR('',#21835,1.5);
#6083=VECTOR('',#21838,1.5);
#6084=VECTOR('',#21849,1.5);
#6085=VECTOR('',#21852,1.5);
#6086=VECTOR('',#21855,1.5);
#6087=VECTOR('',#21858,1.5);
#6088=VECTOR('',#21861,1.5);
#6089=VECTOR('',#21864,1.5);
#6090=VECTOR('',#21867,1.5);
#6091=VECTOR('',#21872,1.54299999999999);
#6092=VECTOR('',#21877,1.54299999999999);
#6093=VECTOR('',#21880,1.54299999999999);
#6094=VECTOR('',#21883,1.54299999999999);
#6095=VECTOR('',#21886,1.54299999999999);
#6096=VECTOR('',#21889,1.54299999999999);
#6097=VECTOR('',#21892,1.54299999999999);
#6098=VECTOR('',#21895,1.54299999999999);
#6099=VECTOR('',#21900,1.5);
#6100=VECTOR('',#21903,1.5);
#6101=VECTOR('',#21914,1.5);
#6102=VECTOR('',#21917,1.5);
#6103=VECTOR('',#21920,1.5);
#6104=VECTOR('',#21923,1.5);
#6105=VECTOR('',#21926,1.5);
#6106=VECTOR('',#21929,1.5);
#6107=VECTOR('',#21932,1.5);
#6108=VECTOR('',#21937,1.543);
#6109=VECTOR('',#21942,1.543);
#6110=VECTOR('',#21945,1.543);
#6111=VECTOR('',#21948,1.543);
#6112=VECTOR('',#21951,1.543);
#6113=VECTOR('',#21954,1.543);
#6114=VECTOR('',#21957,1.543);
#6115=VECTOR('',#21960,1.543);
#6116=VECTOR('',#21965,10.);
#6117=VECTOR('',#21966,10.);
#6118=VECTOR('',#21967,10.);
#6119=VECTOR('',#21968,10.);
#6120=VECTOR('',#21971,10.);
#6121=VECTOR('',#21972,10.);
#6122=VECTOR('',#21973,10.);
#6123=VECTOR('',#21976,10.);
#6124=VECTOR('',#21977,10.);
#6125=VECTOR('',#21978,10.);
#6126=VECTOR('',#21981,10.);
#6127=VECTOR('',#21986,10.);
#6128=VECTOR('',#21987,10.);
#6129=VECTOR('',#21988,10.);
#6130=VECTOR('',#21989,10.);
#6131=VECTOR('',#21990,10.);
#6132=VECTOR('',#21995,10.);
#6133=VECTOR('',#21996,10.);
#6134=VECTOR('',#21997,10.);
#6135=VECTOR('',#21998,10.);
#6136=VECTOR('',#21999,10.);
#6137=VECTOR('',#22004,10.);
#6138=VECTOR('',#22005,10.);
#6139=VECTOR('',#22006,10.);
#6140=VECTOR('',#22007,10.);
#6141=VECTOR('',#22008,10.);
#6142=VECTOR('',#22013,10.);
#6143=VECTOR('',#22014,10.);
#6144=VECTOR('',#22015,10.);
#6145=VECTOR('',#22016,10.);
#6146=VECTOR('',#22017,10.);
#6147=VECTOR('',#22022,10.);
#6148=VECTOR('',#22023,10.);
#6149=VECTOR('',#22024,10.);
#6150=VECTOR('',#22025,10.);
#6151=VECTOR('',#22026,10.);
#6152=VECTOR('',#22031,10.);
#6153=VECTOR('',#22032,10.);
#6154=VECTOR('',#22033,10.);
#6155=VECTOR('',#22034,10.);
#6156=VECTOR('',#22069,10.);
#6157=VECTOR('',#22072,10.);
#6158=VECTOR('',#22075,10.);
#6159=VECTOR('',#22078,10.);
#6160=VECTOR('',#22081,10.);
#6161=VECTOR('',#22084,10.);
#6162=VECTOR('',#22087,10.);
#6163=VECTOR('',#22090,10.);
#6164=VECTOR('',#22093,10.);
#6165=VECTOR('',#22096,10.);
#6166=VECTOR('',#22129,10.);
#6167=VECTOR('',#22132,10.);
#6168=VECTOR('',#22135,10.);
#6169=VECTOR('',#22138,10.);
#6170=VECTOR('',#22141,10.);
#6171=VECTOR('',#22144,10.);
#6172=VECTOR('',#22147,10.);
#6173=VECTOR('',#22150,10.);
#6174=VECTOR('',#22153,10.);
#6175=VECTOR('',#22156,10.);
#6176=VECTOR('',#22165,10.);
#6177=VECTOR('',#22168,10.);
#6178=VECTOR('',#22177,10.);
#6179=VECTOR('',#22180,10.);
#6180=VECTOR('',#22185,1.5);
#6181=VECTOR('',#22192,3.);
#6182=VECTOR('',#22193,3.);
#6183=VECTOR('',#22202,1.5);
#6184=VECTOR('',#22209,3.);
#6185=VECTOR('',#22210,3.);
#6186=VECTOR('',#22219,1.5);
#6187=VECTOR('',#22226,3.);
#6188=VECTOR('',#22227,3.);
#6189=VECTOR('',#22236,1.5);
#6190=VECTOR('',#22243,3.);
#6191=VECTOR('',#22244,3.);
#6192=VECTOR('',#22253,1.5);
#6193=VECTOR('',#22260,3.);
#6194=VECTOR('',#22261,3.);
#6195=VECTOR('',#22270,1.5);
#6196=VECTOR('',#22277,3.);
#6197=VECTOR('',#22278,3.);
#6198=VECTOR('',#22285,10.);
#6199=VECTOR('',#22286,10.);
#6200=VECTOR('',#22289,10.);
#6201=VECTOR('',#22290,10.);
#6202=VECTOR('',#22293,10.);
#6203=VECTOR('',#22294,10.);
#6204=VECTOR('',#22297,10.);
#6205=VECTOR('',#22300,10.);
#6206=VECTOR('',#22301,10.);
#6207=VECTOR('',#22304,10.);
#6208=VECTOR('',#22305,10.);
#6209=VECTOR('',#22308,10.);
#6210=VECTOR('',#22309,10.);
#6211=VECTOR('',#22312,10.);
#6212=VECTOR('',#22315,10.);
#6213=VECTOR('',#22316,10.);
#6214=VECTOR('',#22319,10.);
#6215=VECTOR('',#22320,10.);
#6216=VECTOR('',#22323,10.);
#6217=VECTOR('',#22324,10.);
#6218=VECTOR('',#22327,10.);
#6219=VECTOR('',#22330,10.);
#6220=VECTOR('',#22331,10.);
#6221=VECTOR('',#22334,10.);
#6222=VECTOR('',#22335,10.);
#6223=VECTOR('',#22338,10.);
#6224=VECTOR('',#22339,10.);
#6225=VECTOR('',#22342,10.);
#6226=VECTOR('',#22345,10.);
#6227=VECTOR('',#22346,10.);
#6228=VECTOR('',#22349,10.);
#6229=VECTOR('',#22350,10.);
#6230=VECTOR('',#22353,10.);
#6231=VECTOR('',#22354,10.);
#6232=VECTOR('',#22357,10.);
#6233=VECTOR('',#22358,10.);
#6234=VECTOR('',#22359,10.);
#6235=VECTOR('',#22360,10.);
#6236=VECTOR('',#22361,10.);
#6237=VECTOR('',#22362,10.);
#6238=VECTOR('',#22363,10.);
#6239=VECTOR('',#22364,10.);
#6240=VECTOR('',#22365,10.);
#6241=VECTOR('',#22368,10.);
#6242=VECTOR('',#22369,10.);
#6243=VECTOR('',#22372,10.);
#6244=VECTOR('',#22373,10.);
#6245=VECTOR('',#22376,10.);
#6246=VECTOR('',#22377,10.);
#6247=VECTOR('',#22380,10.);
#6248=VECTOR('',#22381,10.);
#6249=VECTOR('',#22384,10.);
#6250=VECTOR('',#22389,10.);
#6251=VECTOR('',#22394,10.);
#6252=VECTOR('',#22397,10.);
#6253=VECTOR('',#22402,10.);
#6254=VECTOR('',#22407,10.);
#6255=VECTOR('',#22410,10.);
#6256=VECTOR('',#22415,10.);
#6257=VECTOR('',#22420,10.);
#6258=VECTOR('',#22427,10.);
#6259=VECTOR('',#22432,10.);
#6260=VECTOR('',#22437,10.);
#6261=VECTOR('',#22442,10.);
#6262=VECTOR('',#22445,10.);
#6263=VECTOR('',#22448,10.);
#6264=VECTOR('',#22451,10.);
#6265=VECTOR('',#22454,10.);
#6266=VECTOR('',#22457,10.);
#6267=VECTOR('',#22460,10.);
#6268=VECTOR('',#22461,10.);
#6269=VECTOR('',#22464,10.);
#7326=VERTEX_POINT('',#52673);
#7327=VERTEX_POINT('',#52674);
#7328=VERTEX_POINT('',#52676);
#7329=VERTEX_POINT('',#52681);
#7330=VERTEX_POINT('',#52683);
#7331=VERTEX_POINT('',#52685);
#7332=VERTEX_POINT('',#52687);
#7333=VERTEX_POINT('',#52690);
#7334=VERTEX_POINT('',#52703);
#7335=VERTEX_POINT('',#52704);
#7336=VERTEX_POINT('',#52754);
#7337=VERTEX_POINT('',#52755);
#7338=VERTEX_POINT('',#52805);
#7339=VERTEX_POINT('',#52806);
#7340=VERTEX_POINT('',#52853);
#7341=VERTEX_POINT('',#52854);
#7342=VERTEX_POINT('',#52904);
#7343=VERTEX_POINT('',#52905);
#7344=VERTEX_POINT('',#52955);
#7345=VERTEX_POINT('',#52956);
#7346=VERTEX_POINT('',#53003);
#7347=VERTEX_POINT('',#53004);
#7348=VERTEX_POINT('',#53006);
#7349=VERTEX_POINT('',#53020);
#7350=VERTEX_POINT('',#53042);
#7351=VERTEX_POINT('',#53043);
#7352=VERTEX_POINT('',#53045);
#7353=VERTEX_POINT('',#53054);
#7354=VERTEX_POINT('',#53066);
#7355=VERTEX_POINT('',#53067);
#7356=VERTEX_POINT('',#53090);
#7357=VERTEX_POINT('',#53091);
#7358=VERTEX_POINT('',#53115);
#7359=VERTEX_POINT('',#53116);
#7360=VERTEX_POINT('',#53140);
#7361=VERTEX_POINT('',#53141);
#7362=VERTEX_POINT('',#53164);
#7363=VERTEX_POINT('',#53165);
#7364=VERTEX_POINT('',#53189);
#7365=VERTEX_POINT('',#53190);
#7366=VERTEX_POINT('',#53214);
#7367=VERTEX_POINT('',#53215);
#7368=VERTEX_POINT('',#53217);
#7369=VERTEX_POINT('',#53223);
#7370=VERTEX_POINT('',#53231);
#7371=VERTEX_POINT('',#53232);
#7372=VERTEX_POINT('',#53234);
#7373=VERTEX_POINT('',#53239);
#7374=VERTEX_POINT('',#53241);
#7375=VERTEX_POINT('',#53243);
#7376=VERTEX_POINT('',#53245);
#7377=VERTEX_POINT('',#53248);
#7378=VERTEX_POINT('',#53261);
#7379=VERTEX_POINT('',#53262);
#7380=VERTEX_POINT('',#53312);
#7381=VERTEX_POINT('',#53313);
#7382=VERTEX_POINT('',#53363);
#7383=VERTEX_POINT('',#53364);
#7384=VERTEX_POINT('',#53411);
#7385=VERTEX_POINT('',#53412);
#7386=VERTEX_POINT('',#53462);
#7387=VERTEX_POINT('',#53463);
#7388=VERTEX_POINT('',#53513);
#7389=VERTEX_POINT('',#53514);
#7390=VERTEX_POINT('',#53561);
#7391=VERTEX_POINT('',#53562);
#7392=VERTEX_POINT('',#53564);
#7393=VERTEX_POINT('',#53578);
#7394=VERTEX_POINT('',#53600);
#7395=VERTEX_POINT('',#53601);
#7396=VERTEX_POINT('',#53603);
#7397=VERTEX_POINT('',#53612);
#7398=VERTEX_POINT('',#53624);
#7399=VERTEX_POINT('',#53625);
#7400=VERTEX_POINT('',#53648);
#7401=VERTEX_POINT('',#53649);
#7402=VERTEX_POINT('',#53673);
#7403=VERTEX_POINT('',#53674);
#7404=VERTEX_POINT('',#53698);
#7405=VERTEX_POINT('',#53699);
#7406=VERTEX_POINT('',#53722);
#7407=VERTEX_POINT('',#53723);
#7408=VERTEX_POINT('',#53747);
#7409=VERTEX_POINT('',#53748);
#7410=VERTEX_POINT('',#53772);
#7411=VERTEX_POINT('',#53773);
#7412=VERTEX_POINT('',#53775);
#7413=VERTEX_POINT('',#53781);
#7414=VERTEX_POINT('',#53789);
#7415=VERTEX_POINT('',#53790);
#7416=VERTEX_POINT('',#53792);
#7417=VERTEX_POINT('',#53797);
#7418=VERTEX_POINT('',#53799);
#7419=VERTEX_POINT('',#53801);
#7420=VERTEX_POINT('',#53803);
#7421=VERTEX_POINT('',#53806);
#7422=VERTEX_POINT('',#53819);
#7423=VERTEX_POINT('',#53820);
#7424=VERTEX_POINT('',#53870);
#7425=VERTEX_POINT('',#53871);
#7426=VERTEX_POINT('',#53921);
#7427=VERTEX_POINT('',#53922);
#7428=VERTEX_POINT('',#53969);
#7429=VERTEX_POINT('',#53970);
#7430=VERTEX_POINT('',#54020);
#7431=VERTEX_POINT('',#54021);
#7432=VERTEX_POINT('',#54071);
#7433=VERTEX_POINT('',#54072);
#7434=VERTEX_POINT('',#54119);
#7435=VERTEX_POINT('',#54120);
#7436=VERTEX_POINT('',#54122);
#7437=VERTEX_POINT('',#54136);
#7438=VERTEX_POINT('',#54158);
#7439=VERTEX_POINT('',#54159);
#7440=VERTEX_POINT('',#54161);
#7441=VERTEX_POINT('',#54170);
#7442=VERTEX_POINT('',#54182);
#7443=VERTEX_POINT('',#54183);
#7444=VERTEX_POINT('',#54206);
#7445=VERTEX_POINT('',#54207);
#7446=VERTEX_POINT('',#54231);
#7447=VERTEX_POINT('',#54232);
#7448=VERTEX_POINT('',#54256);
#7449=VERTEX_POINT('',#54257);
#7450=VERTEX_POINT('',#54280);
#7451=VERTEX_POINT('',#54281);
#7452=VERTEX_POINT('',#54305);
#7453=VERTEX_POINT('',#54306);
#7454=VERTEX_POINT('',#54330);
#7455=VERTEX_POINT('',#54331);
#7456=VERTEX_POINT('',#54333);
#7457=VERTEX_POINT('',#54339);
#7458=VERTEX_POINT('',#54347);
#7459=VERTEX_POINT('',#54348);
#7460=VERTEX_POINT('',#54350);
#7461=VERTEX_POINT('',#54355);
#7462=VERTEX_POINT('',#54357);
#7463=VERTEX_POINT('',#54359);
#7464=VERTEX_POINT('',#54361);
#7465=VERTEX_POINT('',#54364);
#7466=VERTEX_POINT('',#54377);
#7467=VERTEX_POINT('',#54378);
#7468=VERTEX_POINT('',#54428);
#7469=VERTEX_POINT('',#54429);
#7470=VERTEX_POINT('',#54479);
#7471=VERTEX_POINT('',#54480);
#7472=VERTEX_POINT('',#54527);
#7473=VERTEX_POINT('',#54528);
#7474=VERTEX_POINT('',#54578);
#7475=VERTEX_POINT('',#54579);
#7476=VERTEX_POINT('',#54629);
#7477=VERTEX_POINT('',#54630);
#7478=VERTEX_POINT('',#54677);
#7479=VERTEX_POINT('',#54678);
#7480=VERTEX_POINT('',#54680);
#7481=VERTEX_POINT('',#54694);
#7482=VERTEX_POINT('',#54716);
#7483=VERTEX_POINT('',#54717);
#7484=VERTEX_POINT('',#54719);
#7485=VERTEX_POINT('',#54728);
#7486=VERTEX_POINT('',#54740);
#7487=VERTEX_POINT('',#54741);
#7488=VERTEX_POINT('',#54764);
#7489=VERTEX_POINT('',#54765);
#7490=VERTEX_POINT('',#54789);
#7491=VERTEX_POINT('',#54790);
#7492=VERTEX_POINT('',#54814);
#7493=VERTEX_POINT('',#54815);
#7494=VERTEX_POINT('',#54838);
#7495=VERTEX_POINT('',#54839);
#7496=VERTEX_POINT('',#54863);
#7497=VERTEX_POINT('',#54864);
#7498=VERTEX_POINT('',#54888);
#7499=VERTEX_POINT('',#54889);
#7500=VERTEX_POINT('',#54891);
#7501=VERTEX_POINT('',#54897);
#7502=VERTEX_POINT('',#54905);
#7503=VERTEX_POINT('',#54906);
#7504=VERTEX_POINT('',#54908);
#7505=VERTEX_POINT('',#54913);
#7506=VERTEX_POINT('',#54915);
#7507=VERTEX_POINT('',#54917);
#7508=VERTEX_POINT('',#54919);
#7509=VERTEX_POINT('',#54922);
#7510=VERTEX_POINT('',#54935);
#7511=VERTEX_POINT('',#54936);
#7512=VERTEX_POINT('',#54986);
#7513=VERTEX_POINT('',#54987);
#7514=VERTEX_POINT('',#55037);
#7515=VERTEX_POINT('',#55038);
#7516=VERTEX_POINT('',#55085);
#7517=VERTEX_POINT('',#55086);
#7518=VERTEX_POINT('',#55136);
#7519=VERTEX_POINT('',#55137);
#7520=VERTEX_POINT('',#55187);
#7521=VERTEX_POINT('',#55188);
#7522=VERTEX_POINT('',#55235);
#7523=VERTEX_POINT('',#55236);
#7524=VERTEX_POINT('',#55238);
#7525=VERTEX_POINT('',#55252);
#7526=VERTEX_POINT('',#55274);
#7527=VERTEX_POINT('',#55275);
#7528=VERTEX_POINT('',#55277);
#7529=VERTEX_POINT('',#55286);
#7530=VERTEX_POINT('',#55298);
#7531=VERTEX_POINT('',#55299);
#7532=VERTEX_POINT('',#55322);
#7533=VERTEX_POINT('',#55323);
#7534=VERTEX_POINT('',#55347);
#7535=VERTEX_POINT('',#55348);
#7536=VERTEX_POINT('',#55372);
#7537=VERTEX_POINT('',#55373);
#7538=VERTEX_POINT('',#55396);
#7539=VERTEX_POINT('',#55397);
#7540=VERTEX_POINT('',#55421);
#7541=VERTEX_POINT('',#55422);
#7542=VERTEX_POINT('',#55446);
#7543=VERTEX_POINT('',#55447);
#7544=VERTEX_POINT('',#55449);
#7545=VERTEX_POINT('',#55455);
#7546=VERTEX_POINT('',#55463);
#7547=VERTEX_POINT('',#55464);
#7548=VERTEX_POINT('',#55466);
#7549=VERTEX_POINT('',#55471);
#7550=VERTEX_POINT('',#55473);
#7551=VERTEX_POINT('',#55475);
#7552=VERTEX_POINT('',#55477);
#7553=VERTEX_POINT('',#55480);
#7554=VERTEX_POINT('',#55493);
#7555=VERTEX_POINT('',#55494);
#7556=VERTEX_POINT('',#55544);
#7557=VERTEX_POINT('',#55545);
#7558=VERTEX_POINT('',#55595);
#7559=VERTEX_POINT('',#55596);
#7560=VERTEX_POINT('',#55643);
#7561=VERTEX_POINT('',#55644);
#7562=VERTEX_POINT('',#55694);
#7563=VERTEX_POINT('',#55695);
#7564=VERTEX_POINT('',#55745);
#7565=VERTEX_POINT('',#55746);
#7566=VERTEX_POINT('',#55793);
#7567=VERTEX_POINT('',#55794);
#7568=VERTEX_POINT('',#55796);
#7569=VERTEX_POINT('',#55810);
#7570=VERTEX_POINT('',#55832);
#7571=VERTEX_POINT('',#55833);
#7572=VERTEX_POINT('',#55835);
#7573=VERTEX_POINT('',#55844);
#7574=VERTEX_POINT('',#55856);
#7575=VERTEX_POINT('',#55857);
#7576=VERTEX_POINT('',#55880);
#7577=VERTEX_POINT('',#55881);
#7578=VERTEX_POINT('',#55905);
#7579=VERTEX_POINT('',#55906);
#7580=VERTEX_POINT('',#55930);
#7581=VERTEX_POINT('',#55931);
#7582=VERTEX_POINT('',#55954);
#7583=VERTEX_POINT('',#55955);
#7584=VERTEX_POINT('',#55979);
#7585=VERTEX_POINT('',#55980);
#7586=VERTEX_POINT('',#56004);
#7587=VERTEX_POINT('',#56005);
#7588=VERTEX_POINT('',#56007);
#7589=VERTEX_POINT('',#56013);
#7590=VERTEX_POINT('',#56021);
#7591=VERTEX_POINT('',#56022);
#7592=VERTEX_POINT('',#56024);
#7593=VERTEX_POINT('',#56029);
#7594=VERTEX_POINT('',#56031);
#7595=VERTEX_POINT('',#56033);
#7596=VERTEX_POINT('',#56035);
#7597=VERTEX_POINT('',#56038);
#7598=VERTEX_POINT('',#56051);
#7599=VERTEX_POINT('',#56052);
#7600=VERTEX_POINT('',#56102);
#7601=VERTEX_POINT('',#56103);
#7602=VERTEX_POINT('',#56153);
#7603=VERTEX_POINT('',#56154);
#7604=VERTEX_POINT('',#56201);
#7605=VERTEX_POINT('',#56202);
#7606=VERTEX_POINT('',#56252);
#7607=VERTEX_POINT('',#56253);
#7608=VERTEX_POINT('',#56303);
#7609=VERTEX_POINT('',#56304);
#7610=VERTEX_POINT('',#56351);
#7611=VERTEX_POINT('',#56352);
#7612=VERTEX_POINT('',#56354);
#7613=VERTEX_POINT('',#56368);
#7614=VERTEX_POINT('',#56390);
#7615=VERTEX_POINT('',#56391);
#7616=VERTEX_POINT('',#56393);
#7617=VERTEX_POINT('',#56402);
#7618=VERTEX_POINT('',#56414);
#7619=VERTEX_POINT('',#56415);
#7620=VERTEX_POINT('',#56438);
#7621=VERTEX_POINT('',#56439);
#7622=VERTEX_POINT('',#56463);
#7623=VERTEX_POINT('',#56464);
#7624=VERTEX_POINT('',#56488);
#7625=VERTEX_POINT('',#56489);
#7626=VERTEX_POINT('',#56512);
#7627=VERTEX_POINT('',#56513);
#7628=VERTEX_POINT('',#56537);
#7629=VERTEX_POINT('',#56538);
#7630=VERTEX_POINT('',#56562);
#7631=VERTEX_POINT('',#56563);
#7632=VERTEX_POINT('',#56565);
#7633=VERTEX_POINT('',#56571);
#7634=VERTEX_POINT('',#56579);
#7635=VERTEX_POINT('',#56580);
#7636=VERTEX_POINT('',#56582);
#7637=VERTEX_POINT('',#56587);
#7638=VERTEX_POINT('',#56589);
#7639=VERTEX_POINT('',#56591);
#7640=VERTEX_POINT('',#56593);
#7641=VERTEX_POINT('',#56596);
#7642=VERTEX_POINT('',#56609);
#7643=VERTEX_POINT('',#56610);
#7644=VERTEX_POINT('',#56660);
#7645=VERTEX_POINT('',#56661);
#7646=VERTEX_POINT('',#56711);
#7647=VERTEX_POINT('',#56712);
#7648=VERTEX_POINT('',#56759);
#7649=VERTEX_POINT('',#56760);
#7650=VERTEX_POINT('',#56810);
#7651=VERTEX_POINT('',#56811);
#7652=VERTEX_POINT('',#56861);
#7653=VERTEX_POINT('',#56862);
#7654=VERTEX_POINT('',#56909);
#7655=VERTEX_POINT('',#56910);
#7656=VERTEX_POINT('',#56912);
#7657=VERTEX_POINT('',#56926);
#7658=VERTEX_POINT('',#56948);
#7659=VERTEX_POINT('',#56949);
#7660=VERTEX_POINT('',#56951);
#7661=VERTEX_POINT('',#56960);
#7662=VERTEX_POINT('',#56972);
#7663=VERTEX_POINT('',#56973);
#7664=VERTEX_POINT('',#56996);
#7665=VERTEX_POINT('',#56997);
#7666=VERTEX_POINT('',#57021);
#7667=VERTEX_POINT('',#57022);
#7668=VERTEX_POINT('',#57046);
#7669=VERTEX_POINT('',#57047);
#7670=VERTEX_POINT('',#57070);
#7671=VERTEX_POINT('',#57071);
#7672=VERTEX_POINT('',#57095);
#7673=VERTEX_POINT('',#57096);
#7674=VERTEX_POINT('',#57120);
#7675=VERTEX_POINT('',#57121);
#7676=VERTEX_POINT('',#57123);
#7677=VERTEX_POINT('',#57129);
#7678=VERTEX_POINT('',#57137);
#7679=VERTEX_POINT('',#57138);
#7680=VERTEX_POINT('',#57140);
#7681=VERTEX_POINT('',#57145);
#7682=VERTEX_POINT('',#57147);
#7683=VERTEX_POINT('',#57149);
#7684=VERTEX_POINT('',#57151);
#7685=VERTEX_POINT('',#57154);
#7686=VERTEX_POINT('',#57167);
#7687=VERTEX_POINT('',#57168);
#7688=VERTEX_POINT('',#57218);
#7689=VERTEX_POINT('',#57219);
#7690=VERTEX_POINT('',#57269);
#7691=VERTEX_POINT('',#57270);
#7692=VERTEX_POINT('',#57317);
#7693=VERTEX_POINT('',#57318);
#7694=VERTEX_POINT('',#57368);
#7695=VERTEX_POINT('',#57369);
#7696=VERTEX_POINT('',#57419);
#7697=VERTEX_POINT('',#57420);
#7698=VERTEX_POINT('',#57467);
#7699=VERTEX_POINT('',#57468);
#7700=VERTEX_POINT('',#57470);
#7701=VERTEX_POINT('',#57484);
#7702=VERTEX_POINT('',#57506);
#7703=VERTEX_POINT('',#57507);
#7704=VERTEX_POINT('',#57509);
#7705=VERTEX_POINT('',#57518);
#7706=VERTEX_POINT('',#57530);
#7707=VERTEX_POINT('',#57531);
#7708=VERTEX_POINT('',#57554);
#7709=VERTEX_POINT('',#57555);
#7710=VERTEX_POINT('',#57579);
#7711=VERTEX_POINT('',#57580);
#7712=VERTEX_POINT('',#57604);
#7713=VERTEX_POINT('',#57605);
#7714=VERTEX_POINT('',#57628);
#7715=VERTEX_POINT('',#57629);
#7716=VERTEX_POINT('',#57653);
#7717=VERTEX_POINT('',#57654);
#7718=VERTEX_POINT('',#57678);
#7719=VERTEX_POINT('',#57679);
#7720=VERTEX_POINT('',#57681);
#7721=VERTEX_POINT('',#57687);
#7722=VERTEX_POINT('',#57695);
#7723=VERTEX_POINT('',#57696);
#7724=VERTEX_POINT('',#57698);
#7725=VERTEX_POINT('',#57703);
#7726=VERTEX_POINT('',#57705);
#7727=VERTEX_POINT('',#57707);
#7728=VERTEX_POINT('',#57709);
#7729=VERTEX_POINT('',#57712);
#7730=VERTEX_POINT('',#57725);
#7731=VERTEX_POINT('',#57726);
#7732=VERTEX_POINT('',#57776);
#7733=VERTEX_POINT('',#57777);
#7734=VERTEX_POINT('',#57827);
#7735=VERTEX_POINT('',#57828);
#7736=VERTEX_POINT('',#57875);
#7737=VERTEX_POINT('',#57876);
#7738=VERTEX_POINT('',#57926);
#7739=VERTEX_POINT('',#57927);
#7740=VERTEX_POINT('',#57977);
#7741=VERTEX_POINT('',#57978);
#7742=VERTEX_POINT('',#58025);
#7743=VERTEX_POINT('',#58026);
#7744=VERTEX_POINT('',#58028);
#7745=VERTEX_POINT('',#58042);
#7746=VERTEX_POINT('',#58064);
#7747=VERTEX_POINT('',#58065);
#7748=VERTEX_POINT('',#58067);
#7749=VERTEX_POINT('',#58076);
#7750=VERTEX_POINT('',#58088);
#7751=VERTEX_POINT('',#58089);
#7752=VERTEX_POINT('',#58112);
#7753=VERTEX_POINT('',#58113);
#7754=VERTEX_POINT('',#58137);
#7755=VERTEX_POINT('',#58138);
#7756=VERTEX_POINT('',#58162);
#7757=VERTEX_POINT('',#58163);
#7758=VERTEX_POINT('',#58186);
#7759=VERTEX_POINT('',#58187);
#7760=VERTEX_POINT('',#58211);
#7761=VERTEX_POINT('',#58212);
#7762=VERTEX_POINT('',#58236);
#7763=VERTEX_POINT('',#58237);
#7764=VERTEX_POINT('',#58239);
#7765=VERTEX_POINT('',#58245);
#7766=VERTEX_POINT('',#58253);
#7767=VERTEX_POINT('',#58254);
#7768=VERTEX_POINT('',#58256);
#7769=VERTEX_POINT('',#58261);
#7770=VERTEX_POINT('',#58263);
#7771=VERTEX_POINT('',#58265);
#7772=VERTEX_POINT('',#58267);
#7773=VERTEX_POINT('',#58270);
#7774=VERTEX_POINT('',#58283);
#7775=VERTEX_POINT('',#58284);
#7776=VERTEX_POINT('',#58334);
#7777=VERTEX_POINT('',#58335);
#7778=VERTEX_POINT('',#58385);
#7779=VERTEX_POINT('',#58386);
#7780=VERTEX_POINT('',#58433);
#7781=VERTEX_POINT('',#58434);
#7782=VERTEX_POINT('',#58484);
#7783=VERTEX_POINT('',#58485);
#7784=VERTEX_POINT('',#58535);
#7785=VERTEX_POINT('',#58536);
#7786=VERTEX_POINT('',#58583);
#7787=VERTEX_POINT('',#58584);
#7788=VERTEX_POINT('',#58586);
#7789=VERTEX_POINT('',#58600);
#7790=VERTEX_POINT('',#58622);
#7791=VERTEX_POINT('',#58623);
#7792=VERTEX_POINT('',#58625);
#7793=VERTEX_POINT('',#58634);
#7794=VERTEX_POINT('',#58646);
#7795=VERTEX_POINT('',#58647);
#7796=VERTEX_POINT('',#58670);
#7797=VERTEX_POINT('',#58671);
#7798=VERTEX_POINT('',#58695);
#7799=VERTEX_POINT('',#58696);
#7800=VERTEX_POINT('',#58720);
#7801=VERTEX_POINT('',#58721);
#7802=VERTEX_POINT('',#58744);
#7803=VERTEX_POINT('',#58745);
#7804=VERTEX_POINT('',#58769);
#7805=VERTEX_POINT('',#58770);
#7806=VERTEX_POINT('',#58794);
#7807=VERTEX_POINT('',#58795);
#7808=VERTEX_POINT('',#58797);
#7809=VERTEX_POINT('',#58803);
#7810=VERTEX_POINT('',#58811);
#7811=VERTEX_POINT('',#58812);
#7812=VERTEX_POINT('',#58814);
#7813=VERTEX_POINT('',#58819);
#7814=VERTEX_POINT('',#58821);
#7815=VERTEX_POINT('',#58823);
#7816=VERTEX_POINT('',#58825);
#7817=VERTEX_POINT('',#58828);
#7818=VERTEX_POINT('',#58841);
#7819=VERTEX_POINT('',#58842);
#7820=VERTEX_POINT('',#58892);
#7821=VERTEX_POINT('',#58893);
#7822=VERTEX_POINT('',#58943);
#7823=VERTEX_POINT('',#58944);
#7824=VERTEX_POINT('',#58991);
#7825=VERTEX_POINT('',#58992);
#7826=VERTEX_POINT('',#59042);
#7827=VERTEX_POINT('',#59043);
#7828=VERTEX_POINT('',#59093);
#7829=VERTEX_POINT('',#59094);
#7830=VERTEX_POINT('',#59141);
#7831=VERTEX_POINT('',#59142);
#7832=VERTEX_POINT('',#59144);
#7833=VERTEX_POINT('',#59158);
#7834=VERTEX_POINT('',#59180);
#7835=VERTEX_POINT('',#59181);
#7836=VERTEX_POINT('',#59183);
#7837=VERTEX_POINT('',#59192);
#7838=VERTEX_POINT('',#59204);
#7839=VERTEX_POINT('',#59205);
#7840=VERTEX_POINT('',#59228);
#7841=VERTEX_POINT('',#59229);
#7842=VERTEX_POINT('',#59253);
#7843=VERTEX_POINT('',#59254);
#7844=VERTEX_POINT('',#59278);
#7845=VERTEX_POINT('',#59279);
#7846=VERTEX_POINT('',#59302);
#7847=VERTEX_POINT('',#59303);
#7848=VERTEX_POINT('',#59327);
#7849=VERTEX_POINT('',#59328);
#7850=VERTEX_POINT('',#59352);
#7851=VERTEX_POINT('',#59353);
#7852=VERTEX_POINT('',#59355);
#7853=VERTEX_POINT('',#59361);
#7854=VERTEX_POINT('',#59369);
#7855=VERTEX_POINT('',#59370);
#7856=VERTEX_POINT('',#59372);
#7857=VERTEX_POINT('',#59374);
#7858=VERTEX_POINT('',#59378);
#7859=VERTEX_POINT('',#59380);
#7860=VERTEX_POINT('',#59384);
#7861=VERTEX_POINT('',#59385);
#7862=VERTEX_POINT('',#59390);
#7863=VERTEX_POINT('',#59391);
#7864=VERTEX_POINT('',#59420);
#7865=VERTEX_POINT('',#59422);
#7866=VERTEX_POINT('',#59424);
#7867=VERTEX_POINT('',#59426);
#7868=VERTEX_POINT('',#59431);
#7869=VERTEX_POINT('',#59433);
#7870=VERTEX_POINT('',#59435);
#7871=VERTEX_POINT('',#59437);
#7872=VERTEX_POINT('',#59439);
#7873=VERTEX_POINT('',#59468);
#7874=VERTEX_POINT('',#59470);
#7875=VERTEX_POINT('',#59472);
#7876=VERTEX_POINT('',#59474);
#7877=VERTEX_POINT('',#59479);
#7878=VERTEX_POINT('',#59481);
#7879=VERTEX_POINT('',#59483);
#7880=VERTEX_POINT('',#59485);
#7881=VERTEX_POINT('',#59487);
#7882=VERTEX_POINT('',#59516);
#7883=VERTEX_POINT('',#59518);
#7884=VERTEX_POINT('',#59520);
#7885=VERTEX_POINT('',#59522);
#7886=VERTEX_POINT('',#59527);
#7887=VERTEX_POINT('',#59529);
#7888=VERTEX_POINT('',#59531);
#7889=VERTEX_POINT('',#59533);
#7890=VERTEX_POINT('',#59535);
#7891=VERTEX_POINT('',#59542);
#7892=VERTEX_POINT('',#59544);
#7893=VERTEX_POINT('',#59546);
#7894=VERTEX_POINT('',#59548);
#7895=VERTEX_POINT('',#59553);
#7896=VERTEX_POINT('',#59555);
#7897=VERTEX_POINT('',#59557);
#7898=VERTEX_POINT('',#59559);
#7899=VERTEX_POINT('',#59561);
#7900=VERTEX_POINT('',#59590);
#7901=VERTEX_POINT('',#59592);
#7902=VERTEX_POINT('',#59594);
#7903=VERTEX_POINT('',#59596);
#7904=VERTEX_POINT('',#59601);
#7905=VERTEX_POINT('',#59603);
#7906=VERTEX_POINT('',#59605);
#7907=VERTEX_POINT('',#59607);
#7908=VERTEX_POINT('',#59609);
#7909=VERTEX_POINT('',#59638);
#7910=VERTEX_POINT('',#59640);
#7911=VERTEX_POINT('',#59642);
#7912=VERTEX_POINT('',#59644);
#7913=VERTEX_POINT('',#59649);
#7914=VERTEX_POINT('',#59651);
#7915=VERTEX_POINT('',#59653);
#7916=VERTEX_POINT('',#69798);
#7917=VERTEX_POINT('',#69800);
#7918=VERTEX_POINT('',#69804);
#7919=VERTEX_POINT('',#69807);
#7920=VERTEX_POINT('',#69812);
#7921=VERTEX_POINT('',#69814);
#7922=VERTEX_POINT('',#69818);
#7923=VERTEX_POINT('',#69821);
#7924=VERTEX_POINT('',#69826);
#7925=VERTEX_POINT('',#69828);
#7926=VERTEX_POINT('',#69832);
#7927=VERTEX_POINT('',#69835);
#7928=VERTEX_POINT('',#69840);
#7929=VERTEX_POINT('',#69842);
#7930=VERTEX_POINT('',#69846);
#7931=VERTEX_POINT('',#69849);
#7932=VERTEX_POINT('',#69854);
#7933=VERTEX_POINT('',#69856);
#7934=VERTEX_POINT('',#69860);
#7935=VERTEX_POINT('',#69863);
#7936=VERTEX_POINT('',#69868);
#7937=VERTEX_POINT('',#69870);
#7938=VERTEX_POINT('',#69874);
#7939=VERTEX_POINT('',#69877);
#7940=VERTEX_POINT('',#69882);
#7941=VERTEX_POINT('',#69889);
#7942=VERTEX_POINT('',#69893);
#7943=VERTEX_POINT('',#69900);
#7944=VERTEX_POINT('',#69904);
#7945=VERTEX_POINT('',#69910);
#7946=VERTEX_POINT('',#69917);
#7947=VERTEX_POINT('',#69921);
#7948=VERTEX_POINT('',#69925);
#7949=VERTEX_POINT('',#69929);
#7950=VERTEX_POINT('',#69938);
#7951=VERTEX_POINT('',#69945);
#7952=VERTEX_POINT('',#69949);
#7953=VERTEX_POINT('',#69953);
#7954=VERTEX_POINT('',#69957);
#7955=VERTEX_POINT('',#69966);
#7956=VERTEX_POINT('',#69973);
#7957=VERTEX_POINT('',#69977);
#7958=VERTEX_POINT('',#69981);
#7959=VERTEX_POINT('',#69985);
#7960=VERTEX_POINT('',#69994);
#7961=VERTEX_POINT('',#70001);
#7962=VERTEX_POINT('',#70005);
#7963=VERTEX_POINT('',#70012);
#7964=VERTEX_POINT('',#70016);
#7965=VERTEX_POINT('',#72031);
#7966=VERTEX_POINT('',#74071);
#7967=VERTEX_POINT('',#76111);
#7968=VERTEX_POINT('',#78127);
#7969=VERTEX_POINT('',#80167);
#7970=VERTEX_POINT('',#82183);
#7971=VERTEX_POINT('',#84223);
#7972=VERTEX_POINT('',#86239);
#7973=VERTEX_POINT('',#86270);
#7974=VERTEX_POINT('',#86277);
#7975=VERTEX_POINT('',#86281);
#7976=VERTEX_POINT('',#86288);
#7977=VERTEX_POINT('',#86292);
#7978=VERTEX_POINT('',#88307);
#7979=VERTEX_POINT('',#88338);
#7980=VERTEX_POINT('',#88342);
#7981=VERTEX_POINT('',#88348);
#7982=VERTEX_POINT('',#88352);
#7983=VERTEX_POINT('',#88358);
#7984=VERTEX_POINT('',#88362);
#7985=VERTEX_POINT('',#88368);
#7986=VERTEX_POINT('',#88373);
#7987=VERTEX_POINT('',#88375);
#7988=VERTEX_POINT('',#88378);
#7989=VERTEX_POINT('',#88383);
#7990=VERTEX_POINT('',#88385);
#7991=VERTEX_POINT('',#88388);
#7992=VERTEX_POINT('',#88393);
#7993=VERTEX_POINT('',#88395);
#9591=EDGE_CURVE('',#7326,#7327,#5008,.T.);
#9592=EDGE_CURVE('',#7327,#7328,#3993,.T.);
#9593=EDGE_CURVE('',#7328,#7329,#2849,.T.);
#9594=EDGE_CURVE('',#7329,#7330,#5009,.T.);
#9595=EDGE_CURVE('',#7330,#7331,#2850,.F.);
#9596=EDGE_CURVE('',#7331,#7332,#2851,.F.);
#9597=EDGE_CURVE('',#7332,#7330,#2852,.F.);
#9598=EDGE_CURVE('',#7329,#7333,#2853,.T.);
#9599=EDGE_CURVE('',#7333,#7326,#3994,.T.);
#9600=EDGE_CURVE('',#7334,#7335,#5010,.T.);
#9601=EDGE_CURVE('',#7335,#7327,#3995,.T.);
#9602=EDGE_CURVE('',#7326,#7334,#3996,.T.);
#9603=EDGE_CURVE('',#7336,#7337,#5011,.T.);
#9604=EDGE_CURVE('',#7337,#7335,#3997,.T.);
#9605=EDGE_CURVE('',#7334,#7336,#3998,.T.);
#9606=EDGE_CURVE('',#7338,#7339,#5012,.T.);
#9607=EDGE_CURVE('',#7339,#7337,#3999,.T.);
#9608=EDGE_CURVE('',#7336,#7338,#4000,.T.);
#9609=EDGE_CURVE('',#7340,#7341,#5013,.T.);
#9610=EDGE_CURVE('',#7341,#7339,#4001,.T.);
#9611=EDGE_CURVE('',#7338,#7340,#4002,.T.);
#9612=EDGE_CURVE('',#7342,#7343,#5014,.T.);
#9613=EDGE_CURVE('',#7343,#7341,#4003,.T.);
#9614=EDGE_CURVE('',#7340,#7342,#4004,.T.);
#9615=EDGE_CURVE('',#7344,#7345,#5015,.T.);
#9616=EDGE_CURVE('',#7345,#7343,#4005,.T.);
#9617=EDGE_CURVE('',#7342,#7344,#4006,.T.);
#9618=EDGE_CURVE('',#7346,#7347,#5016,.T.);
#9619=EDGE_CURVE('',#7346,#7348,#4007,.T.);
#9620=EDGE_CURVE('',#7349,#7348,#2854,.F.);
#9621=EDGE_CURVE('',#7349,#7347,#4008,.T.);
#9622=EDGE_CURVE('',#7350,#7351,#5017,.T.);
#9623=EDGE_CURVE('',#7351,#7352,#4009,.T.);
#9624=EDGE_CURVE('',#7353,#7352,#2855,.T.);
#9625=EDGE_CURVE('',#7350,#7353,#4010,.T.);
#9626=EDGE_CURVE('',#7354,#7355,#5018,.T.);
#9627=EDGE_CURVE('',#7355,#7351,#4011,.T.);
#9628=EDGE_CURVE('',#7354,#7350,#4012,.T.);
#9629=EDGE_CURVE('',#7356,#7357,#5019,.T.);
#9630=EDGE_CURVE('',#7357,#7355,#4013,.T.);
#9631=EDGE_CURVE('',#7356,#7354,#4014,.T.);
#9632=EDGE_CURVE('',#7358,#7359,#5020,.T.);
#9633=EDGE_CURVE('',#7359,#7357,#4015,.T.);
#9634=EDGE_CURVE('',#7358,#7356,#4016,.T.);
#9635=EDGE_CURVE('',#7360,#7361,#5021,.T.);
#9636=EDGE_CURVE('',#7361,#7359,#4017,.T.);
#9637=EDGE_CURVE('',#7360,#7358,#4018,.T.);
#9638=EDGE_CURVE('',#7362,#7363,#5022,.T.);
#9639=EDGE_CURVE('',#7363,#7361,#4019,.T.);
#9640=EDGE_CURVE('',#7362,#7360,#4020,.T.);
#9641=EDGE_CURVE('',#7364,#7365,#5023,.T.);
#9642=EDGE_CURVE('',#7365,#7363,#4021,.T.);
#9643=EDGE_CURVE('',#7364,#7362,#4022,.T.);
#9644=EDGE_CURVE('',#7366,#7367,#5024,.T.);
#9645=EDGE_CURVE('',#7368,#7366,#4023,.T.);
#9646=EDGE_CURVE('',#7369,#7368,#2856,.T.);
#9647=EDGE_CURVE('',#7369,#7367,#4024,.T.);
#9648=EDGE_CURVE('',#7370,#7371,#5025,.T.);
#9649=EDGE_CURVE('',#7371,#7372,#4025,.T.);
#9650=EDGE_CURVE('',#7372,#7373,#2857,.T.);
#9651=EDGE_CURVE('',#7373,#7374,#5026,.T.);
#9652=EDGE_CURVE('',#7374,#7375,#2858,.F.);
#9653=EDGE_CURVE('',#7375,#7376,#2859,.F.);
#9654=EDGE_CURVE('',#7376,#7374,#2860,.F.);
#9655=EDGE_CURVE('',#7373,#7377,#2861,.T.);
#9656=EDGE_CURVE('',#7377,#7370,#4026,.T.);
#9657=EDGE_CURVE('',#7378,#7379,#5027,.T.);
#9658=EDGE_CURVE('',#7379,#7371,#4027,.T.);
#9659=EDGE_CURVE('',#7370,#7378,#4028,.T.);
#9660=EDGE_CURVE('',#7380,#7381,#5028,.T.);
#9661=EDGE_CURVE('',#7381,#7379,#4029,.T.);
#9662=EDGE_CURVE('',#7378,#7380,#4030,.T.);
#9663=EDGE_CURVE('',#7382,#7383,#5029,.T.);
#9664=EDGE_CURVE('',#7383,#7381,#4031,.T.);
#9665=EDGE_CURVE('',#7380,#7382,#4032,.T.);
#9666=EDGE_CURVE('',#7384,#7385,#5030,.T.);
#9667=EDGE_CURVE('',#7385,#7383,#4033,.T.);
#9668=EDGE_CURVE('',#7382,#7384,#4034,.T.);
#9669=EDGE_CURVE('',#7386,#7387,#5031,.T.);
#9670=EDGE_CURVE('',#7387,#7385,#4035,.T.);
#9671=EDGE_CURVE('',#7384,#7386,#4036,.T.);
#9672=EDGE_CURVE('',#7388,#7389,#5032,.T.);
#9673=EDGE_CURVE('',#7389,#7387,#4037,.T.);
#9674=EDGE_CURVE('',#7386,#7388,#4038,.T.);
#9675=EDGE_CURVE('',#7390,#7391,#5033,.T.);
#9676=EDGE_CURVE('',#7390,#7392,#4039,.T.);
#9677=EDGE_CURVE('',#7393,#7392,#2862,.F.);
#9678=EDGE_CURVE('',#7393,#7391,#4040,.T.);
#9679=EDGE_CURVE('',#7394,#7395,#5034,.T.);
#9680=EDGE_CURVE('',#7395,#7396,#4041,.T.);
#9681=EDGE_CURVE('',#7397,#7396,#2863,.T.);
#9682=EDGE_CURVE('',#7394,#7397,#4042,.T.);
#9683=EDGE_CURVE('',#7398,#7399,#5035,.T.);
#9684=EDGE_CURVE('',#7399,#7395,#4043,.T.);
#9685=EDGE_CURVE('',#7398,#7394,#4044,.T.);
#9686=EDGE_CURVE('',#7400,#7401,#5036,.T.);
#9687=EDGE_CURVE('',#7401,#7399,#4045,.T.);
#9688=EDGE_CURVE('',#7400,#7398,#4046,.T.);
#9689=EDGE_CURVE('',#7402,#7403,#5037,.T.);
#9690=EDGE_CURVE('',#7403,#7401,#4047,.T.);
#9691=EDGE_CURVE('',#7402,#7400,#4048,.T.);
#9692=EDGE_CURVE('',#7404,#7405,#5038,.T.);
#9693=EDGE_CURVE('',#7405,#7403,#4049,.T.);
#9694=EDGE_CURVE('',#7404,#7402,#4050,.T.);
#9695=EDGE_CURVE('',#7406,#7407,#5039,.T.);
#9696=EDGE_CURVE('',#7407,#7405,#4051,.T.);
#9697=EDGE_CURVE('',#7406,#7404,#4052,.T.);
#9698=EDGE_CURVE('',#7408,#7409,#5040,.T.);
#9699=EDGE_CURVE('',#7409,#7407,#4053,.T.);
#9700=EDGE_CURVE('',#7408,#7406,#4054,.T.);
#9701=EDGE_CURVE('',#7410,#7411,#5041,.T.);
#9702=EDGE_CURVE('',#7412,#7410,#4055,.T.);
#9703=EDGE_CURVE('',#7413,#7412,#2864,.T.);
#9704=EDGE_CURVE('',#7413,#7411,#4056,.T.);
#9705=EDGE_CURVE('',#7414,#7415,#5042,.T.);
#9706=EDGE_CURVE('',#7415,#7416,#4057,.T.);
#9707=EDGE_CURVE('',#7416,#7417,#2865,.T.);
#9708=EDGE_CURVE('',#7417,#7418,#5043,.T.);
#9709=EDGE_CURVE('',#7418,#7419,#2866,.F.);
#9710=EDGE_CURVE('',#7419,#7420,#2867,.F.);
#9711=EDGE_CURVE('',#7420,#7418,#2868,.F.);
#9712=EDGE_CURVE('',#7417,#7421,#2869,.T.);
#9713=EDGE_CURVE('',#7421,#7414,#4058,.T.);
#9714=EDGE_CURVE('',#7422,#7423,#5044,.T.);
#9715=EDGE_CURVE('',#7423,#7415,#4059,.T.);
#9716=EDGE_CURVE('',#7414,#7422,#4060,.T.);
#9717=EDGE_CURVE('',#7424,#7425,#5045,.T.);
#9718=EDGE_CURVE('',#7425,#7423,#4061,.T.);
#9719=EDGE_CURVE('',#7422,#7424,#4062,.T.);
#9720=EDGE_CURVE('',#7426,#7427,#5046,.T.);
#9721=EDGE_CURVE('',#7427,#7425,#4063,.T.);
#9722=EDGE_CURVE('',#7424,#7426,#4064,.T.);
#9723=EDGE_CURVE('',#7428,#7429,#5047,.T.);
#9724=EDGE_CURVE('',#7429,#7427,#4065,.T.);
#9725=EDGE_CURVE('',#7426,#7428,#4066,.T.);
#9726=EDGE_CURVE('',#7430,#7431,#5048,.T.);
#9727=EDGE_CURVE('',#7431,#7429,#4067,.T.);
#9728=EDGE_CURVE('',#7428,#7430,#4068,.T.);
#9729=EDGE_CURVE('',#7432,#7433,#5049,.T.);
#9730=EDGE_CURVE('',#7433,#7431,#4069,.T.);
#9731=EDGE_CURVE('',#7430,#7432,#4070,.T.);
#9732=EDGE_CURVE('',#7434,#7435,#5050,.T.);
#9733=EDGE_CURVE('',#7434,#7436,#4071,.T.);
#9734=EDGE_CURVE('',#7437,#7436,#2870,.F.);
#9735=EDGE_CURVE('',#7437,#7435,#4072,.T.);
#9736=EDGE_CURVE('',#7438,#7439,#5051,.T.);
#9737=EDGE_CURVE('',#7439,#7440,#4073,.T.);
#9738=EDGE_CURVE('',#7441,#7440,#2871,.T.);
#9739=EDGE_CURVE('',#7438,#7441,#4074,.T.);
#9740=EDGE_CURVE('',#7442,#7443,#5052,.T.);
#9741=EDGE_CURVE('',#7443,#7439,#4075,.T.);
#9742=EDGE_CURVE('',#7442,#7438,#4076,.T.);
#9743=EDGE_CURVE('',#7444,#7445,#5053,.T.);
#9744=EDGE_CURVE('',#7445,#7443,#4077,.T.);
#9745=EDGE_CURVE('',#7444,#7442,#4078,.T.);
#9746=EDGE_CURVE('',#7446,#7447,#5054,.T.);
#9747=EDGE_CURVE('',#7447,#7445,#4079,.T.);
#9748=EDGE_CURVE('',#7446,#7444,#4080,.T.);
#9749=EDGE_CURVE('',#7448,#7449,#5055,.T.);
#9750=EDGE_CURVE('',#7449,#7447,#4081,.T.);
#9751=EDGE_CURVE('',#7448,#7446,#4082,.T.);
#9752=EDGE_CURVE('',#7450,#7451,#5056,.T.);
#9753=EDGE_CURVE('',#7451,#7449,#4083,.T.);
#9754=EDGE_CURVE('',#7450,#7448,#4084,.T.);
#9755=EDGE_CURVE('',#7452,#7453,#5057,.T.);
#9756=EDGE_CURVE('',#7453,#7451,#4085,.T.);
#9757=EDGE_CURVE('',#7452,#7450,#4086,.T.);
#9758=EDGE_CURVE('',#7454,#7455,#5058,.T.);
#9759=EDGE_CURVE('',#7456,#7454,#4087,.T.);
#9760=EDGE_CURVE('',#7457,#7456,#2872,.T.);
#9761=EDGE_CURVE('',#7457,#7455,#4088,.T.);
#9762=EDGE_CURVE('',#7458,#7459,#5059,.T.);
#9763=EDGE_CURVE('',#7459,#7460,#4089,.T.);
#9764=EDGE_CURVE('',#7460,#7461,#2873,.T.);
#9765=EDGE_CURVE('',#7461,#7462,#5060,.T.);
#9766=EDGE_CURVE('',#7462,#7463,#2874,.F.);
#9767=EDGE_CURVE('',#7463,#7464,#2875,.F.);
#9768=EDGE_CURVE('',#7464,#7462,#2876,.F.);
#9769=EDGE_CURVE('',#7461,#7465,#2877,.T.);
#9770=EDGE_CURVE('',#7465,#7458,#4090,.T.);
#9771=EDGE_CURVE('',#7466,#7467,#5061,.T.);
#9772=EDGE_CURVE('',#7467,#7459,#4091,.T.);
#9773=EDGE_CURVE('',#7458,#7466,#4092,.T.);
#9774=EDGE_CURVE('',#7468,#7469,#5062,.T.);
#9775=EDGE_CURVE('',#7469,#7467,#4093,.T.);
#9776=EDGE_CURVE('',#7466,#7468,#4094,.T.);
#9777=EDGE_CURVE('',#7470,#7471,#5063,.T.);
#9778=EDGE_CURVE('',#7471,#7469,#4095,.T.);
#9779=EDGE_CURVE('',#7468,#7470,#4096,.T.);
#9780=EDGE_CURVE('',#7472,#7473,#5064,.T.);
#9781=EDGE_CURVE('',#7473,#7471,#4097,.T.);
#9782=EDGE_CURVE('',#7470,#7472,#4098,.T.);
#9783=EDGE_CURVE('',#7474,#7475,#5065,.T.);
#9784=EDGE_CURVE('',#7475,#7473,#4099,.T.);
#9785=EDGE_CURVE('',#7472,#7474,#4100,.T.);
#9786=EDGE_CURVE('',#7476,#7477,#5066,.T.);
#9787=EDGE_CURVE('',#7477,#7475,#4101,.T.);
#9788=EDGE_CURVE('',#7474,#7476,#4102,.T.);
#9789=EDGE_CURVE('',#7478,#7479,#5067,.T.);
#9790=EDGE_CURVE('',#7478,#7480,#4103,.T.);
#9791=EDGE_CURVE('',#7481,#7480,#2878,.F.);
#9792=EDGE_CURVE('',#7481,#7479,#4104,.T.);
#9793=EDGE_CURVE('',#7482,#7483,#5068,.T.);
#9794=EDGE_CURVE('',#7483,#7484,#4105,.T.);
#9795=EDGE_CURVE('',#7485,#7484,#2879,.T.);
#9796=EDGE_CURVE('',#7482,#7485,#4106,.T.);
#9797=EDGE_CURVE('',#7486,#7487,#5069,.T.);
#9798=EDGE_CURVE('',#7487,#7483,#4107,.T.);
#9799=EDGE_CURVE('',#7486,#7482,#4108,.T.);
#9800=EDGE_CURVE('',#7488,#7489,#5070,.T.);
#9801=EDGE_CURVE('',#7489,#7487,#4109,.T.);
#9802=EDGE_CURVE('',#7488,#7486,#4110,.T.);
#9803=EDGE_CURVE('',#7490,#7491,#5071,.T.);
#9804=EDGE_CURVE('',#7491,#7489,#4111,.T.);
#9805=EDGE_CURVE('',#7490,#7488,#4112,.T.);
#9806=EDGE_CURVE('',#7492,#7493,#5072,.T.);
#9807=EDGE_CURVE('',#7493,#7491,#4113,.T.);
#9808=EDGE_CURVE('',#7492,#7490,#4114,.T.);
#9809=EDGE_CURVE('',#7494,#7495,#5073,.T.);
#9810=EDGE_CURVE('',#7495,#7493,#4115,.T.);
#9811=EDGE_CURVE('',#7494,#7492,#4116,.T.);
#9812=EDGE_CURVE('',#7496,#7497,#5074,.T.);
#9813=EDGE_CURVE('',#7497,#7495,#4117,.T.);
#9814=EDGE_CURVE('',#7496,#7494,#4118,.T.);
#9815=EDGE_CURVE('',#7498,#7499,#5075,.T.);
#9816=EDGE_CURVE('',#7500,#7498,#4119,.T.);
#9817=EDGE_CURVE('',#7501,#7500,#2880,.T.);
#9818=EDGE_CURVE('',#7501,#7499,#4120,.T.);
#9819=EDGE_CURVE('',#7502,#7503,#5076,.T.);
#9820=EDGE_CURVE('',#7503,#7504,#4121,.T.);
#9821=EDGE_CURVE('',#7504,#7505,#2881,.T.);
#9822=EDGE_CURVE('',#7505,#7506,#5077,.T.);
#9823=EDGE_CURVE('',#7506,#7507,#2882,.F.);
#9824=EDGE_CURVE('',#7507,#7508,#2883,.F.);
#9825=EDGE_CURVE('',#7508,#7506,#2884,.F.);
#9826=EDGE_CURVE('',#7505,#7509,#2885,.T.);
#9827=EDGE_CURVE('',#7509,#7502,#4122,.T.);
#9828=EDGE_CURVE('',#7510,#7511,#5078,.T.);
#9829=EDGE_CURVE('',#7511,#7503,#4123,.T.);
#9830=EDGE_CURVE('',#7502,#7510,#4124,.T.);
#9831=EDGE_CURVE('',#7512,#7513,#5079,.T.);
#9832=EDGE_CURVE('',#7513,#7511,#4125,.T.);
#9833=EDGE_CURVE('',#7510,#7512,#4126,.T.);
#9834=EDGE_CURVE('',#7514,#7515,#5080,.T.);
#9835=EDGE_CURVE('',#7515,#7513,#4127,.T.);
#9836=EDGE_CURVE('',#7512,#7514,#4128,.T.);
#9837=EDGE_CURVE('',#7516,#7517,#5081,.T.);
#9838=EDGE_CURVE('',#7517,#7515,#4129,.T.);
#9839=EDGE_CURVE('',#7514,#7516,#4130,.T.);
#9840=EDGE_CURVE('',#7518,#7519,#5082,.T.);
#9841=EDGE_CURVE('',#7519,#7517,#4131,.T.);
#9842=EDGE_CURVE('',#7516,#7518,#4132,.T.);
#9843=EDGE_CURVE('',#7520,#7521,#5083,.T.);
#9844=EDGE_CURVE('',#7521,#7519,#4133,.T.);
#9845=EDGE_CURVE('',#7518,#7520,#4134,.T.);
#9846=EDGE_CURVE('',#7522,#7523,#5084,.T.);
#9847=EDGE_CURVE('',#7522,#7524,#4135,.T.);
#9848=EDGE_CURVE('',#7525,#7524,#2886,.F.);
#9849=EDGE_CURVE('',#7525,#7523,#4136,.T.);
#9850=EDGE_CURVE('',#7526,#7527,#5085,.T.);
#9851=EDGE_CURVE('',#7527,#7528,#4137,.T.);
#9852=EDGE_CURVE('',#7529,#7528,#2887,.T.);
#9853=EDGE_CURVE('',#7526,#7529,#4138,.T.);
#9854=EDGE_CURVE('',#7530,#7531,#5086,.T.);
#9855=EDGE_CURVE('',#7531,#7527,#4139,.T.);
#9856=EDGE_CURVE('',#7530,#7526,#4140,.T.);
#9857=EDGE_CURVE('',#7532,#7533,#5087,.T.);
#9858=EDGE_CURVE('',#7533,#7531,#4141,.T.);
#9859=EDGE_CURVE('',#7532,#7530,#4142,.T.);
#9860=EDGE_CURVE('',#7534,#7535,#5088,.T.);
#9861=EDGE_CURVE('',#7535,#7533,#4143,.T.);
#9862=EDGE_CURVE('',#7534,#7532,#4144,.T.);
#9863=EDGE_CURVE('',#7536,#7537,#5089,.T.);
#9864=EDGE_CURVE('',#7537,#7535,#4145,.T.);
#9865=EDGE_CURVE('',#7536,#7534,#4146,.T.);
#9866=EDGE_CURVE('',#7538,#7539,#5090,.T.);
#9867=EDGE_CURVE('',#7539,#7537,#4147,.T.);
#9868=EDGE_CURVE('',#7538,#7536,#4148,.T.);
#9869=EDGE_CURVE('',#7540,#7541,#5091,.T.);
#9870=EDGE_CURVE('',#7541,#7539,#4149,.T.);
#9871=EDGE_CURVE('',#7540,#7538,#4150,.T.);
#9872=EDGE_CURVE('',#7542,#7543,#5092,.T.);
#9873=EDGE_CURVE('',#7544,#7542,#4151,.T.);
#9874=EDGE_CURVE('',#7545,#7544,#2888,.T.);
#9875=EDGE_CURVE('',#7545,#7543,#4152,.T.);
#9876=EDGE_CURVE('',#7546,#7547,#5093,.T.);
#9877=EDGE_CURVE('',#7547,#7548,#4153,.T.);
#9878=EDGE_CURVE('',#7548,#7549,#2889,.T.);
#9879=EDGE_CURVE('',#7549,#7550,#5094,.T.);
#9880=EDGE_CURVE('',#7550,#7551,#2890,.F.);
#9881=EDGE_CURVE('',#7551,#7552,#2891,.F.);
#9882=EDGE_CURVE('',#7552,#7550,#2892,.F.);
#9883=EDGE_CURVE('',#7549,#7553,#2893,.T.);
#9884=EDGE_CURVE('',#7553,#7546,#4154,.T.);
#9885=EDGE_CURVE('',#7554,#7555,#5095,.T.);
#9886=EDGE_CURVE('',#7555,#7547,#4155,.T.);
#9887=EDGE_CURVE('',#7546,#7554,#4156,.T.);
#9888=EDGE_CURVE('',#7556,#7557,#5096,.T.);
#9889=EDGE_CURVE('',#7557,#7555,#4157,.T.);
#9890=EDGE_CURVE('',#7554,#7556,#4158,.T.);
#9891=EDGE_CURVE('',#7558,#7559,#5097,.T.);
#9892=EDGE_CURVE('',#7559,#7557,#4159,.T.);
#9893=EDGE_CURVE('',#7556,#7558,#4160,.T.);
#9894=EDGE_CURVE('',#7560,#7561,#5098,.T.);
#9895=EDGE_CURVE('',#7561,#7559,#4161,.T.);
#9896=EDGE_CURVE('',#7558,#7560,#4162,.T.);
#9897=EDGE_CURVE('',#7562,#7563,#5099,.T.);
#9898=EDGE_CURVE('',#7563,#7561,#4163,.T.);
#9899=EDGE_CURVE('',#7560,#7562,#4164,.T.);
#9900=EDGE_CURVE('',#7564,#7565,#5100,.T.);
#9901=EDGE_CURVE('',#7565,#7563,#4165,.T.);
#9902=EDGE_CURVE('',#7562,#7564,#4166,.T.);
#9903=EDGE_CURVE('',#7566,#7567,#5101,.T.);
#9904=EDGE_CURVE('',#7566,#7568,#4167,.T.);
#9905=EDGE_CURVE('',#7569,#7568,#2894,.F.);
#9906=EDGE_CURVE('',#7569,#7567,#4168,.T.);
#9907=EDGE_CURVE('',#7570,#7571,#5102,.T.);
#9908=EDGE_CURVE('',#7571,#7572,#4169,.T.);
#9909=EDGE_CURVE('',#7573,#7572,#2895,.T.);
#9910=EDGE_CURVE('',#7570,#7573,#4170,.T.);
#9911=EDGE_CURVE('',#7574,#7575,#5103,.T.);
#9912=EDGE_CURVE('',#7575,#7571,#4171,.T.);
#9913=EDGE_CURVE('',#7574,#7570,#4172,.T.);
#9914=EDGE_CURVE('',#7576,#7577,#5104,.T.);
#9915=EDGE_CURVE('',#7577,#7575,#4173,.T.);
#9916=EDGE_CURVE('',#7576,#7574,#4174,.T.);
#9917=EDGE_CURVE('',#7578,#7579,#5105,.T.);
#9918=EDGE_CURVE('',#7579,#7577,#4175,.T.);
#9919=EDGE_CURVE('',#7578,#7576,#4176,.T.);
#9920=EDGE_CURVE('',#7580,#7581,#5106,.T.);
#9921=EDGE_CURVE('',#7581,#7579,#4177,.T.);
#9922=EDGE_CURVE('',#7580,#7578,#4178,.T.);
#9923=EDGE_CURVE('',#7582,#7583,#5107,.T.);
#9924=EDGE_CURVE('',#7583,#7581,#4179,.T.);
#9925=EDGE_CURVE('',#7582,#7580,#4180,.T.);
#9926=EDGE_CURVE('',#7584,#7585,#5108,.T.);
#9927=EDGE_CURVE('',#7585,#7583,#4181,.T.);
#9928=EDGE_CURVE('',#7584,#7582,#4182,.T.);
#9929=EDGE_CURVE('',#7586,#7587,#5109,.T.);
#9930=EDGE_CURVE('',#7588,#7586,#4183,.T.);
#9931=EDGE_CURVE('',#7589,#7588,#2896,.T.);
#9932=EDGE_CURVE('',#7589,#7587,#4184,.T.);
#9933=EDGE_CURVE('',#7590,#7591,#5110,.T.);
#9934=EDGE_CURVE('',#7591,#7592,#4185,.T.);
#9935=EDGE_CURVE('',#7592,#7593,#2897,.T.);
#9936=EDGE_CURVE('',#7593,#7594,#5111,.T.);
#9937=EDGE_CURVE('',#7594,#7595,#2898,.F.);
#9938=EDGE_CURVE('',#7595,#7596,#2899,.F.);
#9939=EDGE_CURVE('',#7596,#7594,#2900,.F.);
#9940=EDGE_CURVE('',#7593,#7597,#2901,.T.);
#9941=EDGE_CURVE('',#7597,#7590,#4186,.T.);
#9942=EDGE_CURVE('',#7598,#7599,#5112,.T.);
#9943=EDGE_CURVE('',#7599,#7591,#4187,.T.);
#9944=EDGE_CURVE('',#7590,#7598,#4188,.T.);
#9945=EDGE_CURVE('',#7600,#7601,#5113,.T.);
#9946=EDGE_CURVE('',#7601,#7599,#4189,.T.);
#9947=EDGE_CURVE('',#7598,#7600,#4190,.T.);
#9948=EDGE_CURVE('',#7602,#7603,#5114,.T.);
#9949=EDGE_CURVE('',#7603,#7601,#4191,.T.);
#9950=EDGE_CURVE('',#7600,#7602,#4192,.T.);
#9951=EDGE_CURVE('',#7604,#7605,#5115,.T.);
#9952=EDGE_CURVE('',#7605,#7603,#4193,.T.);
#9953=EDGE_CURVE('',#7602,#7604,#4194,.T.);
#9954=EDGE_CURVE('',#7606,#7607,#5116,.T.);
#9955=EDGE_CURVE('',#7607,#7605,#4195,.T.);
#9956=EDGE_CURVE('',#7604,#7606,#4196,.T.);
#9957=EDGE_CURVE('',#7608,#7609,#5117,.T.);
#9958=EDGE_CURVE('',#7609,#7607,#4197,.T.);
#9959=EDGE_CURVE('',#7606,#7608,#4198,.T.);
#9960=EDGE_CURVE('',#7610,#7611,#5118,.T.);
#9961=EDGE_CURVE('',#7610,#7612,#4199,.T.);
#9962=EDGE_CURVE('',#7613,#7612,#2902,.F.);
#9963=EDGE_CURVE('',#7613,#7611,#4200,.T.);
#9964=EDGE_CURVE('',#7614,#7615,#5119,.T.);
#9965=EDGE_CURVE('',#7615,#7616,#4201,.T.);
#9966=EDGE_CURVE('',#7617,#7616,#2903,.T.);
#9967=EDGE_CURVE('',#7614,#7617,#4202,.T.);
#9968=EDGE_CURVE('',#7618,#7619,#5120,.T.);
#9969=EDGE_CURVE('',#7619,#7615,#4203,.T.);
#9970=EDGE_CURVE('',#7618,#7614,#4204,.T.);
#9971=EDGE_CURVE('',#7620,#7621,#5121,.T.);
#9972=EDGE_CURVE('',#7621,#7619,#4205,.T.);
#9973=EDGE_CURVE('',#7620,#7618,#4206,.T.);
#9974=EDGE_CURVE('',#7622,#7623,#5122,.T.);
#9975=EDGE_CURVE('',#7623,#7621,#4207,.T.);
#9976=EDGE_CURVE('',#7622,#7620,#4208,.T.);
#9977=EDGE_CURVE('',#7624,#7625,#5123,.T.);
#9978=EDGE_CURVE('',#7625,#7623,#4209,.T.);
#9979=EDGE_CURVE('',#7624,#7622,#4210,.T.);
#9980=EDGE_CURVE('',#7626,#7627,#5124,.T.);
#9981=EDGE_CURVE('',#7627,#7625,#4211,.T.);
#9982=EDGE_CURVE('',#7626,#7624,#4212,.T.);
#9983=EDGE_CURVE('',#7628,#7629,#5125,.T.);
#9984=EDGE_CURVE('',#7629,#7627,#4213,.T.);
#9985=EDGE_CURVE('',#7628,#7626,#4214,.T.);
#9986=EDGE_CURVE('',#7630,#7631,#5126,.T.);
#9987=EDGE_CURVE('',#7632,#7630,#4215,.T.);
#9988=EDGE_CURVE('',#7633,#7632,#2904,.T.);
#9989=EDGE_CURVE('',#7633,#7631,#4216,.T.);
#9990=EDGE_CURVE('',#7634,#7635,#5127,.T.);
#9991=EDGE_CURVE('',#7635,#7636,#4217,.T.);
#9992=EDGE_CURVE('',#7636,#7637,#2905,.T.);
#9993=EDGE_CURVE('',#7637,#7638,#5128,.T.);
#9994=EDGE_CURVE('',#7638,#7639,#2906,.F.);
#9995=EDGE_CURVE('',#7639,#7640,#2907,.F.);
#9996=EDGE_CURVE('',#7640,#7638,#2908,.F.);
#9997=EDGE_CURVE('',#7637,#7641,#2909,.T.);
#9998=EDGE_CURVE('',#7641,#7634,#4218,.T.);
#9999=EDGE_CURVE('',#7642,#7643,#5129,.T.);
#10000=EDGE_CURVE('',#7643,#7635,#4219,.T.);
#10001=EDGE_CURVE('',#7634,#7642,#4220,.T.);
#10002=EDGE_CURVE('',#7644,#7645,#5130,.T.);
#10003=EDGE_CURVE('',#7645,#7643,#4221,.T.);
#10004=EDGE_CURVE('',#7642,#7644,#4222,.T.);
#10005=EDGE_CURVE('',#7646,#7647,#5131,.T.);
#10006=EDGE_CURVE('',#7647,#7645,#4223,.T.);
#10007=EDGE_CURVE('',#7644,#7646,#4224,.T.);
#10008=EDGE_CURVE('',#7648,#7649,#5132,.T.);
#10009=EDGE_CURVE('',#7649,#7647,#4225,.T.);
#10010=EDGE_CURVE('',#7646,#7648,#4226,.T.);
#10011=EDGE_CURVE('',#7650,#7651,#5133,.T.);
#10012=EDGE_CURVE('',#7651,#7649,#4227,.T.);
#10013=EDGE_CURVE('',#7648,#7650,#4228,.T.);
#10014=EDGE_CURVE('',#7652,#7653,#5134,.T.);
#10015=EDGE_CURVE('',#7653,#7651,#4229,.T.);
#10016=EDGE_CURVE('',#7650,#7652,#4230,.T.);
#10017=EDGE_CURVE('',#7654,#7655,#5135,.T.);
#10018=EDGE_CURVE('',#7654,#7656,#4231,.T.);
#10019=EDGE_CURVE('',#7657,#7656,#2910,.F.);
#10020=EDGE_CURVE('',#7657,#7655,#4232,.T.);
#10021=EDGE_CURVE('',#7658,#7659,#5136,.T.);
#10022=EDGE_CURVE('',#7659,#7660,#4233,.T.);
#10023=EDGE_CURVE('',#7661,#7660,#2911,.T.);
#10024=EDGE_CURVE('',#7658,#7661,#4234,.T.);
#10025=EDGE_CURVE('',#7662,#7663,#5137,.T.);
#10026=EDGE_CURVE('',#7663,#7659,#4235,.T.);
#10027=EDGE_CURVE('',#7662,#7658,#4236,.T.);
#10028=EDGE_CURVE('',#7664,#7665,#5138,.T.);
#10029=EDGE_CURVE('',#7665,#7663,#4237,.T.);
#10030=EDGE_CURVE('',#7664,#7662,#4238,.T.);
#10031=EDGE_CURVE('',#7666,#7667,#5139,.T.);
#10032=EDGE_CURVE('',#7667,#7665,#4239,.T.);
#10033=EDGE_CURVE('',#7666,#7664,#4240,.T.);
#10034=EDGE_CURVE('',#7668,#7669,#5140,.T.);
#10035=EDGE_CURVE('',#7669,#7667,#4241,.T.);
#10036=EDGE_CURVE('',#7668,#7666,#4242,.T.);
#10037=EDGE_CURVE('',#7670,#7671,#5141,.T.);
#10038=EDGE_CURVE('',#7671,#7669,#4243,.T.);
#10039=EDGE_CURVE('',#7670,#7668,#4244,.T.);
#10040=EDGE_CURVE('',#7672,#7673,#5142,.T.);
#10041=EDGE_CURVE('',#7673,#7671,#4245,.T.);
#10042=EDGE_CURVE('',#7672,#7670,#4246,.T.);
#10043=EDGE_CURVE('',#7674,#7675,#5143,.T.);
#10044=EDGE_CURVE('',#7676,#7674,#4247,.T.);
#10045=EDGE_CURVE('',#7677,#7676,#2912,.T.);
#10046=EDGE_CURVE('',#7677,#7675,#4248,.T.);
#10047=EDGE_CURVE('',#7678,#7679,#5144,.T.);
#10048=EDGE_CURVE('',#7679,#7680,#4249,.T.);
#10049=EDGE_CURVE('',#7680,#7681,#2913,.T.);
#10050=EDGE_CURVE('',#7681,#7682,#5145,.T.);
#10051=EDGE_CURVE('',#7682,#7683,#2914,.F.);
#10052=EDGE_CURVE('',#7683,#7684,#2915,.F.);
#10053=EDGE_CURVE('',#7684,#7682,#2916,.F.);
#10054=EDGE_CURVE('',#7681,#7685,#2917,.T.);
#10055=EDGE_CURVE('',#7685,#7678,#4250,.T.);
#10056=EDGE_CURVE('',#7686,#7687,#5146,.T.);
#10057=EDGE_CURVE('',#7687,#7679,#4251,.T.);
#10058=EDGE_CURVE('',#7678,#7686,#4252,.T.);
#10059=EDGE_CURVE('',#7688,#7689,#5147,.T.);
#10060=EDGE_CURVE('',#7689,#7687,#4253,.T.);
#10061=EDGE_CURVE('',#7686,#7688,#4254,.T.);
#10062=EDGE_CURVE('',#7690,#7691,#5148,.T.);
#10063=EDGE_CURVE('',#7691,#7689,#4255,.T.);
#10064=EDGE_CURVE('',#7688,#7690,#4256,.T.);
#10065=EDGE_CURVE('',#7692,#7693,#5149,.T.);
#10066=EDGE_CURVE('',#7693,#7691,#4257,.T.);
#10067=EDGE_CURVE('',#7690,#7692,#4258,.T.);
#10068=EDGE_CURVE('',#7694,#7695,#5150,.T.);
#10069=EDGE_CURVE('',#7695,#7693,#4259,.T.);
#10070=EDGE_CURVE('',#7692,#7694,#4260,.T.);
#10071=EDGE_CURVE('',#7696,#7697,#5151,.T.);
#10072=EDGE_CURVE('',#7697,#7695,#4261,.T.);
#10073=EDGE_CURVE('',#7694,#7696,#4262,.T.);
#10074=EDGE_CURVE('',#7698,#7699,#5152,.T.);
#10075=EDGE_CURVE('',#7698,#7700,#4263,.T.);
#10076=EDGE_CURVE('',#7701,#7700,#2918,.F.);
#10077=EDGE_CURVE('',#7701,#7699,#4264,.T.);
#10078=EDGE_CURVE('',#7702,#7703,#5153,.T.);
#10079=EDGE_CURVE('',#7703,#7704,#4265,.T.);
#10080=EDGE_CURVE('',#7705,#7704,#2919,.T.);
#10081=EDGE_CURVE('',#7702,#7705,#4266,.T.);
#10082=EDGE_CURVE('',#7706,#7707,#5154,.T.);
#10083=EDGE_CURVE('',#7707,#7703,#4267,.T.);
#10084=EDGE_CURVE('',#7706,#7702,#4268,.T.);
#10085=EDGE_CURVE('',#7708,#7709,#5155,.T.);
#10086=EDGE_CURVE('',#7709,#7707,#4269,.T.);
#10087=EDGE_CURVE('',#7708,#7706,#4270,.T.);
#10088=EDGE_CURVE('',#7710,#7711,#5156,.T.);
#10089=EDGE_CURVE('',#7711,#7709,#4271,.T.);
#10090=EDGE_CURVE('',#7710,#7708,#4272,.T.);
#10091=EDGE_CURVE('',#7712,#7713,#5157,.T.);
#10092=EDGE_CURVE('',#7713,#7711,#4273,.T.);
#10093=EDGE_CURVE('',#7712,#7710,#4274,.T.);
#10094=EDGE_CURVE('',#7714,#7715,#5158,.T.);
#10095=EDGE_CURVE('',#7715,#7713,#4275,.T.);
#10096=EDGE_CURVE('',#7714,#7712,#4276,.T.);
#10097=EDGE_CURVE('',#7716,#7717,#5159,.T.);
#10098=EDGE_CURVE('',#7717,#7715,#4277,.T.);
#10099=EDGE_CURVE('',#7716,#7714,#4278,.T.);
#10100=EDGE_CURVE('',#7718,#7719,#5160,.T.);
#10101=EDGE_CURVE('',#7720,#7718,#4279,.T.);
#10102=EDGE_CURVE('',#7721,#7720,#2920,.T.);
#10103=EDGE_CURVE('',#7721,#7719,#4280,.T.);
#10104=EDGE_CURVE('',#7722,#7723,#5161,.T.);
#10105=EDGE_CURVE('',#7723,#7724,#4281,.T.);
#10106=EDGE_CURVE('',#7724,#7725,#2921,.T.);
#10107=EDGE_CURVE('',#7725,#7726,#5162,.T.);
#10108=EDGE_CURVE('',#7726,#7727,#2922,.F.);
#10109=EDGE_CURVE('',#7727,#7728,#2923,.F.);
#10110=EDGE_CURVE('',#7728,#7726,#2924,.F.);
#10111=EDGE_CURVE('',#7725,#7729,#2925,.T.);
#10112=EDGE_CURVE('',#7729,#7722,#4282,.T.);
#10113=EDGE_CURVE('',#7730,#7731,#5163,.T.);
#10114=EDGE_CURVE('',#7731,#7723,#4283,.T.);
#10115=EDGE_CURVE('',#7722,#7730,#4284,.T.);
#10116=EDGE_CURVE('',#7732,#7733,#5164,.T.);
#10117=EDGE_CURVE('',#7733,#7731,#4285,.T.);
#10118=EDGE_CURVE('',#7730,#7732,#4286,.T.);
#10119=EDGE_CURVE('',#7734,#7735,#5165,.T.);
#10120=EDGE_CURVE('',#7735,#7733,#4287,.T.);
#10121=EDGE_CURVE('',#7732,#7734,#4288,.T.);
#10122=EDGE_CURVE('',#7736,#7737,#5166,.T.);
#10123=EDGE_CURVE('',#7737,#7735,#4289,.T.);
#10124=EDGE_CURVE('',#7734,#7736,#4290,.T.);
#10125=EDGE_CURVE('',#7738,#7739,#5167,.T.);
#10126=EDGE_CURVE('',#7739,#7737,#4291,.T.);
#10127=EDGE_CURVE('',#7736,#7738,#4292,.T.);
#10128=EDGE_CURVE('',#7740,#7741,#5168,.T.);
#10129=EDGE_CURVE('',#7741,#7739,#4293,.T.);
#10130=EDGE_CURVE('',#7738,#7740,#4294,.T.);
#10131=EDGE_CURVE('',#7742,#7743,#5169,.T.);
#10132=EDGE_CURVE('',#7742,#7744,#4295,.T.);
#10133=EDGE_CURVE('',#7745,#7744,#2926,.F.);
#10134=EDGE_CURVE('',#7745,#7743,#4296,.T.);
#10135=EDGE_CURVE('',#7746,#7747,#5170,.T.);
#10136=EDGE_CURVE('',#7747,#7748,#4297,.T.);
#10137=EDGE_CURVE('',#7749,#7748,#2927,.T.);
#10138=EDGE_CURVE('',#7746,#7749,#4298,.T.);
#10139=EDGE_CURVE('',#7750,#7751,#5171,.T.);
#10140=EDGE_CURVE('',#7751,#7747,#4299,.T.);
#10141=EDGE_CURVE('',#7750,#7746,#4300,.T.);
#10142=EDGE_CURVE('',#7752,#7753,#5172,.T.);
#10143=EDGE_CURVE('',#7753,#7751,#4301,.T.);
#10144=EDGE_CURVE('',#7752,#7750,#4302,.T.);
#10145=EDGE_CURVE('',#7754,#7755,#5173,.T.);
#10146=EDGE_CURVE('',#7755,#7753,#4303,.T.);
#10147=EDGE_CURVE('',#7754,#7752,#4304,.T.);
#10148=EDGE_CURVE('',#7756,#7757,#5174,.T.);
#10149=EDGE_CURVE('',#7757,#7755,#4305,.T.);
#10150=EDGE_CURVE('',#7756,#7754,#4306,.T.);
#10151=EDGE_CURVE('',#7758,#7759,#5175,.T.);
#10152=EDGE_CURVE('',#7759,#7757,#4307,.T.);
#10153=EDGE_CURVE('',#7758,#7756,#4308,.T.);
#10154=EDGE_CURVE('',#7760,#7761,#5176,.T.);
#10155=EDGE_CURVE('',#7761,#7759,#4309,.T.);
#10156=EDGE_CURVE('',#7760,#7758,#4310,.T.);
#10157=EDGE_CURVE('',#7762,#7763,#5177,.T.);
#10158=EDGE_CURVE('',#7764,#7762,#4311,.T.);
#10159=EDGE_CURVE('',#7765,#7764,#2928,.T.);
#10160=EDGE_CURVE('',#7765,#7763,#4312,.T.);
#10161=EDGE_CURVE('',#7766,#7767,#5178,.T.);
#10162=EDGE_CURVE('',#7767,#7768,#4313,.T.);
#10163=EDGE_CURVE('',#7768,#7769,#2929,.T.);
#10164=EDGE_CURVE('',#7769,#7770,#5179,.T.);
#10165=EDGE_CURVE('',#7770,#7771,#2930,.F.);
#10166=EDGE_CURVE('',#7771,#7772,#2931,.F.);
#10167=EDGE_CURVE('',#7772,#7770,#2932,.F.);
#10168=EDGE_CURVE('',#7769,#7773,#2933,.T.);
#10169=EDGE_CURVE('',#7773,#7766,#4314,.T.);
#10170=EDGE_CURVE('',#7774,#7775,#5180,.T.);
#10171=EDGE_CURVE('',#7775,#7767,#4315,.T.);
#10172=EDGE_CURVE('',#7766,#7774,#4316,.T.);
#10173=EDGE_CURVE('',#7776,#7777,#5181,.T.);
#10174=EDGE_CURVE('',#7777,#7775,#4317,.T.);
#10175=EDGE_CURVE('',#7774,#7776,#4318,.T.);
#10176=EDGE_CURVE('',#7778,#7779,#5182,.T.);
#10177=EDGE_CURVE('',#7779,#7777,#4319,.T.);
#10178=EDGE_CURVE('',#7776,#7778,#4320,.T.);
#10179=EDGE_CURVE('',#7780,#7781,#5183,.T.);
#10180=EDGE_CURVE('',#7781,#7779,#4321,.T.);
#10181=EDGE_CURVE('',#7778,#7780,#4322,.T.);
#10182=EDGE_CURVE('',#7782,#7783,#5184,.T.);
#10183=EDGE_CURVE('',#7783,#7781,#4323,.T.);
#10184=EDGE_CURVE('',#7780,#7782,#4324,.T.);
#10185=EDGE_CURVE('',#7784,#7785,#5185,.T.);
#10186=EDGE_CURVE('',#7785,#7783,#4325,.T.);
#10187=EDGE_CURVE('',#7782,#7784,#4326,.T.);
#10188=EDGE_CURVE('',#7786,#7787,#5186,.T.);
#10189=EDGE_CURVE('',#7786,#7788,#4327,.T.);
#10190=EDGE_CURVE('',#7789,#7788,#2934,.F.);
#10191=EDGE_CURVE('',#7789,#7787,#4328,.T.);
#10192=EDGE_CURVE('',#7790,#7791,#5187,.T.);
#10193=EDGE_CURVE('',#7791,#7792,#4329,.T.);
#10194=EDGE_CURVE('',#7793,#7792,#2935,.T.);
#10195=EDGE_CURVE('',#7790,#7793,#4330,.T.);
#10196=EDGE_CURVE('',#7794,#7795,#5188,.T.);
#10197=EDGE_CURVE('',#7795,#7791,#4331,.T.);
#10198=EDGE_CURVE('',#7794,#7790,#4332,.T.);
#10199=EDGE_CURVE('',#7796,#7797,#5189,.T.);
#10200=EDGE_CURVE('',#7797,#7795,#4333,.T.);
#10201=EDGE_CURVE('',#7796,#7794,#4334,.T.);
#10202=EDGE_CURVE('',#7798,#7799,#5190,.T.);
#10203=EDGE_CURVE('',#7799,#7797,#4335,.T.);
#10204=EDGE_CURVE('',#7798,#7796,#4336,.T.);
#10205=EDGE_CURVE('',#7800,#7801,#5191,.T.);
#10206=EDGE_CURVE('',#7801,#7799,#4337,.T.);
#10207=EDGE_CURVE('',#7800,#7798,#4338,.T.);
#10208=EDGE_CURVE('',#7802,#7803,#5192,.T.);
#10209=EDGE_CURVE('',#7803,#7801,#4339,.T.);
#10210=EDGE_CURVE('',#7802,#7800,#4340,.T.);
#10211=EDGE_CURVE('',#7804,#7805,#5193,.T.);
#10212=EDGE_CURVE('',#7805,#7803,#4341,.T.);
#10213=EDGE_CURVE('',#7804,#7802,#4342,.T.);
#10214=EDGE_CURVE('',#7806,#7807,#5194,.T.);
#10215=EDGE_CURVE('',#7808,#7806,#4343,.T.);
#10216=EDGE_CURVE('',#7809,#7808,#2936,.T.);
#10217=EDGE_CURVE('',#7809,#7807,#4344,.T.);
#10218=EDGE_CURVE('',#7810,#7811,#5195,.T.);
#10219=EDGE_CURVE('',#7811,#7812,#4345,.T.);
#10220=EDGE_CURVE('',#7812,#7813,#2937,.T.);
#10221=EDGE_CURVE('',#7813,#7814,#5196,.T.);
#10222=EDGE_CURVE('',#7814,#7815,#2938,.F.);
#10223=EDGE_CURVE('',#7815,#7816,#2939,.F.);
#10224=EDGE_CURVE('',#7816,#7814,#2940,.F.);
#10225=EDGE_CURVE('',#7813,#7817,#2941,.T.);
#10226=EDGE_CURVE('',#7817,#7810,#4346,.T.);
#10227=EDGE_CURVE('',#7818,#7819,#5197,.T.);
#10228=EDGE_CURVE('',#7819,#7811,#4347,.T.);
#10229=EDGE_CURVE('',#7810,#7818,#4348,.T.);
#10230=EDGE_CURVE('',#7820,#7821,#5198,.T.);
#10231=EDGE_CURVE('',#7821,#7819,#4349,.T.);
#10232=EDGE_CURVE('',#7818,#7820,#4350,.T.);
#10233=EDGE_CURVE('',#7822,#7823,#5199,.T.);
#10234=EDGE_CURVE('',#7823,#7821,#4351,.T.);
#10235=EDGE_CURVE('',#7820,#7822,#4352,.T.);
#10236=EDGE_CURVE('',#7824,#7825,#5200,.T.);
#10237=EDGE_CURVE('',#7825,#7823,#4353,.T.);
#10238=EDGE_CURVE('',#7822,#7824,#4354,.T.);
#10239=EDGE_CURVE('',#7826,#7827,#5201,.T.);
#10240=EDGE_CURVE('',#7827,#7825,#4355,.T.);
#10241=EDGE_CURVE('',#7824,#7826,#4356,.T.);
#10242=EDGE_CURVE('',#7828,#7829,#5202,.T.);
#10243=EDGE_CURVE('',#7829,#7827,#4357,.T.);
#10244=EDGE_CURVE('',#7826,#7828,#4358,.T.);
#10245=EDGE_CURVE('',#7830,#7831,#5203,.T.);
#10246=EDGE_CURVE('',#7830,#7832,#4359,.T.);
#10247=EDGE_CURVE('',#7833,#7832,#2942,.F.);
#10248=EDGE_CURVE('',#7833,#7831,#4360,.T.);
#10249=EDGE_CURVE('',#7834,#7835,#5204,.T.);
#10250=EDGE_CURVE('',#7835,#7836,#4361,.T.);
#10251=EDGE_CURVE('',#7837,#7836,#2943,.T.);
#10252=EDGE_CURVE('',#7834,#7837,#4362,.T.);
#10253=EDGE_CURVE('',#7838,#7839,#5205,.T.);
#10254=EDGE_CURVE('',#7839,#7835,#4363,.T.);
#10255=EDGE_CURVE('',#7838,#7834,#4364,.T.);
#10256=EDGE_CURVE('',#7840,#7841,#5206,.T.);
#10257=EDGE_CURVE('',#7841,#7839,#4365,.T.);
#10258=EDGE_CURVE('',#7840,#7838,#4366,.T.);
#10259=EDGE_CURVE('',#7842,#7843,#5207,.T.);
#10260=EDGE_CURVE('',#7843,#7841,#4367,.T.);
#10261=EDGE_CURVE('',#7842,#7840,#4368,.T.);
#10262=EDGE_CURVE('',#7844,#7845,#5208,.T.);
#10263=EDGE_CURVE('',#7845,#7843,#4369,.T.);
#10264=EDGE_CURVE('',#7844,#7842,#4370,.T.);
#10265=EDGE_CURVE('',#7846,#7847,#5209,.T.);
#10266=EDGE_CURVE('',#7847,#7845,#4371,.T.);
#10267=EDGE_CURVE('',#7846,#7844,#4372,.T.);
#10268=EDGE_CURVE('',#7848,#7849,#5210,.T.);
#10269=EDGE_CURVE('',#7849,#7847,#4373,.T.);
#10270=EDGE_CURVE('',#7848,#7846,#4374,.T.);
#10271=EDGE_CURVE('',#7850,#7851,#5211,.T.);
#10272=EDGE_CURVE('',#7852,#7850,#4375,.T.);
#10273=EDGE_CURVE('',#7853,#7852,#2944,.T.);
#10274=EDGE_CURVE('',#7853,#7851,#4376,.T.);
#10275=EDGE_CURVE('',#7854,#7855,#5212,.T.);
#10276=EDGE_CURVE('',#7856,#7854,#5213,.T.);
#10277=EDGE_CURVE('',#7856,#7857,#5214,.T.);
#10278=EDGE_CURVE('',#7855,#7857,#5215,.T.);
#10279=EDGE_CURVE('',#7858,#7856,#5216,.T.);
#10280=EDGE_CURVE('',#7858,#7859,#5217,.T.);
#10281=EDGE_CURVE('',#7857,#7859,#5218,.T.);
#10282=EDGE_CURVE('',#7860,#7861,#5219,.T.);
#10283=EDGE_CURVE('',#7859,#7860,#5220,.T.);
#10284=EDGE_CURVE('',#7861,#7858,#5221,.T.);
#10285=EDGE_CURVE('',#7862,#7863,#4377,.T.);
#10286=EDGE_CURVE('',#7864,#7862,#5222,.T.);
#10287=EDGE_CURVE('',#7865,#7864,#2945,.T.);
#10288=EDGE_CURVE('',#7866,#7865,#2946,.T.);
#10289=EDGE_CURVE('',#7867,#7866,#4378,.T.);
#10290=EDGE_CURVE('',#7867,#7868,#5223,.T.);
#10291=EDGE_CURVE('',#7868,#7869,#5224,.T.);
#10292=EDGE_CURVE('',#7869,#7870,#5225,.T.);
#10293=EDGE_CURVE('',#7870,#7871,#5226,.T.);
#10294=EDGE_CURVE('',#7872,#7871,#4379,.T.);
#10295=EDGE_CURVE('',#7873,#7872,#5227,.T.);
#10296=EDGE_CURVE('',#7874,#7873,#2947,.T.);
#10297=EDGE_CURVE('',#7875,#7874,#2948,.T.);
#10298=EDGE_CURVE('',#7876,#7875,#4380,.T.);
#10299=EDGE_CURVE('',#7876,#7877,#5228,.T.);
#10300=EDGE_CURVE('',#7877,#7878,#5229,.T.);
#10301=EDGE_CURVE('',#7878,#7879,#5230,.T.);
#10302=EDGE_CURVE('',#7879,#7880,#5231,.T.);
#10303=EDGE_CURVE('',#7881,#7880,#4381,.T.);
#10304=EDGE_CURVE('',#7882,#7881,#5232,.T.);
#10305=EDGE_CURVE('',#7883,#7882,#2949,.T.);
#10306=EDGE_CURVE('',#7884,#7883,#2950,.T.);
#10307=EDGE_CURVE('',#7885,#7884,#4382,.T.);
#10308=EDGE_CURVE('',#7885,#7886,#5233,.T.);
#10309=EDGE_CURVE('',#7886,#7887,#5234,.T.);
#10310=EDGE_CURVE('',#7887,#7888,#5235,.T.);
#10311=EDGE_CURVE('',#7888,#7889,#5236,.T.);
#10312=EDGE_CURVE('',#7890,#7889,#4383,.T.);
#10313=EDGE_CURVE('',#7891,#7890,#5237,.T.);
#10314=EDGE_CURVE('',#7892,#7891,#2951,.T.);
#10315=EDGE_CURVE('',#7893,#7892,#2952,.T.);
#10316=EDGE_CURVE('',#7894,#7893,#4384,.T.);
#10317=EDGE_CURVE('',#7894,#7895,#5238,.T.);
#10318=EDGE_CURVE('',#7895,#7896,#5239,.T.);
#10319=EDGE_CURVE('',#7896,#7897,#5240,.T.);
#10320=EDGE_CURVE('',#7897,#7898,#5241,.T.);
#10321=EDGE_CURVE('',#7899,#7898,#4385,.T.);
#10322=EDGE_CURVE('',#7900,#7899,#5242,.T.);
#10323=EDGE_CURVE('',#7901,#7900,#2953,.T.);
#10324=EDGE_CURVE('',#7902,#7901,#2954,.T.);
#10325=EDGE_CURVE('',#7903,#7902,#4386,.T.);
#10326=EDGE_CURVE('',#7903,#7904,#5243,.T.);
#10327=EDGE_CURVE('',#7904,#7905,#5244,.T.);
#10328=EDGE_CURVE('',#7905,#7906,#5245,.T.);
#10329=EDGE_CURVE('',#7906,#7907,#5246,.T.);
#10330=EDGE_CURVE('',#7908,#7907,#4387,.T.);
#10331=EDGE_CURVE('',#7909,#7908,#5247,.T.);
#10332=EDGE_CURVE('',#7910,#7909,#2955,.T.);
#10333=EDGE_CURVE('',#7911,#7910,#2956,.T.);
#10334=EDGE_CURVE('',#7912,#7911,#4388,.T.);
#10335=EDGE_CURVE('',#7912,#7913,#5248,.T.);
#10336=EDGE_CURVE('',#7913,#7914,#5249,.T.);
#10337=EDGE_CURVE('',#7914,#7915,#5250,.T.);
#10338=EDGE_CURVE('',#7915,#7863,#5251,.T.);
#10339=EDGE_CURVE('',#7368,#7349,#4389,.T.);
#10340=EDGE_CURVE('',#7348,#7369,#4390,.T.);
#10341=EDGE_CURVE('',#7861,#7854,#2957,.T.);
#10342=EDGE_CURVE('',#7456,#7437,#4391,.T.);
#10343=EDGE_CURVE('',#7436,#7457,#4392,.T.);
#10344=EDGE_CURVE('',#7500,#7481,#4393,.T.);
#10345=EDGE_CURVE('',#7480,#7501,#4394,.T.);
#10346=EDGE_CURVE('',#7544,#7525,#4395,.T.);
#10347=EDGE_CURVE('',#7524,#7545,#4396,.T.);
#10348=EDGE_CURVE('',#7588,#7569,#4397,.T.);
#10349=EDGE_CURVE('',#7568,#7589,#4398,.T.);
#10350=EDGE_CURVE('',#7632,#7613,#4399,.T.);
#10351=EDGE_CURVE('',#7612,#7633,#4400,.T.);
#10352=EDGE_CURVE('',#7812,#7837,#4401,.T.);
#10353=EDGE_CURVE('',#7836,#7817,#4402,.T.);
#10354=EDGE_CURVE('',#7851,#7849,#4403,.T.);
#10355=EDGE_CURVE('',#7850,#7848,#4404,.T.);
#10356=EDGE_CURVE('',#7832,#7853,#4405,.T.);
#10357=EDGE_CURVE('',#7828,#7830,#4406,.T.);
#10358=EDGE_CURVE('',#7831,#7829,#4407,.T.);
#10359=EDGE_CURVE('',#7852,#7833,#4408,.T.);
#10360=EDGE_CURVE('',#7768,#7793,#4409,.T.);
#10361=EDGE_CURVE('',#7792,#7773,#4410,.T.);
#10362=EDGE_CURVE('',#7807,#7805,#4411,.T.);
#10363=EDGE_CURVE('',#7806,#7804,#4412,.T.);
#10364=EDGE_CURVE('',#7788,#7809,#4413,.T.);
#10365=EDGE_CURVE('',#7784,#7786,#4414,.T.);
#10366=EDGE_CURVE('',#7787,#7785,#4415,.T.);
#10367=EDGE_CURVE('',#7808,#7789,#4416,.T.);
#10368=EDGE_CURVE('',#7724,#7749,#4417,.T.);
#10369=EDGE_CURVE('',#7748,#7729,#4418,.T.);
#10370=EDGE_CURVE('',#7763,#7761,#4419,.T.);
#10371=EDGE_CURVE('',#7762,#7760,#4420,.T.);
#10372=EDGE_CURVE('',#7744,#7765,#4421,.T.);
#10373=EDGE_CURVE('',#7740,#7742,#4422,.T.);
#10374=EDGE_CURVE('',#7743,#7741,#4423,.T.);
#10375=EDGE_CURVE('',#7764,#7745,#4424,.T.);
#10376=EDGE_CURVE('',#7680,#7705,#4425,.T.);
#10377=EDGE_CURVE('',#7704,#7685,#4426,.T.);
#10378=EDGE_CURVE('',#7719,#7717,#4427,.T.);
#10379=EDGE_CURVE('',#7718,#7716,#4428,.T.);
#10380=EDGE_CURVE('',#7700,#7721,#4429,.T.);
#10381=EDGE_CURVE('',#7696,#7698,#4430,.T.);
#10382=EDGE_CURVE('',#7699,#7697,#4431,.T.);
#10383=EDGE_CURVE('',#7720,#7701,#4432,.T.);
#10384=EDGE_CURVE('',#7636,#7661,#4433,.T.);
#10385=EDGE_CURVE('',#7660,#7641,#4434,.T.);
#10386=EDGE_CURVE('',#7675,#7673,#4435,.T.);
#10387=EDGE_CURVE('',#7674,#7672,#4436,.T.);
#10388=EDGE_CURVE('',#7656,#7677,#4437,.T.);
#10389=EDGE_CURVE('',#7652,#7654,#4438,.T.);
#10390=EDGE_CURVE('',#7655,#7653,#4439,.T.);
#10391=EDGE_CURVE('',#7676,#7657,#4440,.T.);
#10392=EDGE_CURVE('',#7816,#7815,#5252,.T.);
#10393=EDGE_CURVE('',#7816,#7815,#5253,.T.);
#10394=EDGE_CURVE('',#7772,#7771,#5254,.T.);
#10395=EDGE_CURVE('',#7772,#7771,#5255,.T.);
#10396=EDGE_CURVE('',#7728,#7727,#5256,.T.);
#10397=EDGE_CURVE('',#7728,#7727,#5257,.T.);
#10398=EDGE_CURVE('',#7684,#7683,#5258,.T.);
#10399=EDGE_CURVE('',#7684,#7683,#5259,.T.);
#10400=EDGE_CURVE('',#7640,#7639,#5260,.T.);
#10401=EDGE_CURVE('',#7640,#7639,#5261,.T.);
#10402=EDGE_CURVE('',#7592,#7617,#4441,.T.);
#10403=EDGE_CURVE('',#7616,#7597,#4442,.T.);
#10404=EDGE_CURVE('',#7631,#7629,#4443,.T.);
#10405=EDGE_CURVE('',#7630,#7628,#4444,.T.);
#10406=EDGE_CURVE('',#7608,#7610,#4445,.T.);
#10407=EDGE_CURVE('',#7611,#7609,#4446,.T.);
#10408=EDGE_CURVE('',#7548,#7573,#4447,.T.);
#10409=EDGE_CURVE('',#7572,#7553,#4448,.T.);
#10410=EDGE_CURVE('',#7587,#7585,#4449,.T.);
#10411=EDGE_CURVE('',#7586,#7584,#4450,.T.);
#10412=EDGE_CURVE('',#7564,#7566,#4451,.T.);
#10413=EDGE_CURVE('',#7567,#7565,#4452,.T.);
#10414=EDGE_CURVE('',#7504,#7529,#4453,.T.);
#10415=EDGE_CURVE('',#7528,#7509,#4454,.T.);
#10416=EDGE_CURVE('',#7543,#7541,#4455,.T.);
#10417=EDGE_CURVE('',#7542,#7540,#4456,.T.);
#10418=EDGE_CURVE('',#7520,#7522,#4457,.T.);
#10419=EDGE_CURVE('',#7523,#7521,#4458,.T.);
#10420=EDGE_CURVE('',#7460,#7485,#4459,.T.);
#10421=EDGE_CURVE('',#7484,#7465,#4460,.T.);
#10422=EDGE_CURVE('',#7499,#7497,#4461,.T.);
#10423=EDGE_CURVE('',#7498,#7496,#4462,.T.);
#10424=EDGE_CURVE('',#7476,#7478,#4463,.T.);
#10425=EDGE_CURVE('',#7479,#7477,#4464,.T.);
#10426=EDGE_CURVE('',#7416,#7441,#4465,.T.);
#10427=EDGE_CURVE('',#7440,#7421,#4466,.T.);
#10428=EDGE_CURVE('',#7455,#7453,#4467,.T.);
#10429=EDGE_CURVE('',#7454,#7452,#4468,.T.);
#10430=EDGE_CURVE('',#7432,#7434,#4469,.T.);
#10431=EDGE_CURVE('',#7435,#7433,#4470,.T.);
#10432=EDGE_CURVE('',#7596,#7595,#5262,.T.);
#10433=EDGE_CURVE('',#7596,#7595,#5263,.T.);
#10434=EDGE_CURVE('',#7552,#7551,#5264,.T.);
#10435=EDGE_CURVE('',#7552,#7551,#5265,.T.);
#10436=EDGE_CURVE('',#7508,#7507,#5266,.T.);
#10437=EDGE_CURVE('',#7508,#7507,#5267,.T.);
#10438=EDGE_CURVE('',#7464,#7463,#5268,.T.);
#10439=EDGE_CURVE('',#7464,#7463,#5269,.T.);
#10440=EDGE_CURVE('',#7420,#7419,#5270,.T.);
#10441=EDGE_CURVE('',#7420,#7419,#5271,.T.);
#10442=EDGE_CURVE('',#7372,#7397,#4471,.T.);
#10443=EDGE_CURVE('',#7396,#7377,#4472,.T.);
#10444=EDGE_CURVE('',#7411,#7409,#4473,.T.);
#10445=EDGE_CURVE('',#7410,#7408,#4474,.T.);
#10446=EDGE_CURVE('',#7392,#7413,#4475,.T.);
#10447=EDGE_CURVE('',#7388,#7390,#4476,.T.);
#10448=EDGE_CURVE('',#7391,#7389,#4477,.T.);
#10449=EDGE_CURVE('',#7412,#7393,#4478,.T.);
#10450=EDGE_CURVE('',#7376,#7375,#5272,.T.);
#10451=EDGE_CURVE('',#7376,#7375,#5273,.T.);
#10452=EDGE_CURVE('',#7328,#7353,#4479,.T.);
#10453=EDGE_CURVE('',#7352,#7333,#4480,.T.);
#10454=EDGE_CURVE('',#7367,#7365,#4481,.T.);
#10455=EDGE_CURVE('',#7366,#7364,#4482,.T.);
#10456=EDGE_CURVE('',#7344,#7346,#4483,.T.);
#10457=EDGE_CURVE('',#7347,#7345,#4484,.T.);
#10458=EDGE_CURVE('',#7332,#7331,#5274,.T.);
#10459=EDGE_CURVE('',#7332,#7331,#5275,.T.);
#10460=EDGE_CURVE('',#7916,#7916,#2958,.T.);
#10461=EDGE_CURVE('',#7916,#7917,#5276,.T.);
#10462=EDGE_CURVE('',#7917,#7917,#2959,.T.);
#10463=EDGE_CURVE('',#7918,#7918,#2960,.T.);
#10464=EDGE_CURVE('',#7918,#7815,#5277,.T.);
#10465=EDGE_CURVE('',#7816,#7919,#5278,.T.);
#10466=EDGE_CURVE('',#7919,#7919,#2961,.T.);
#10467=EDGE_CURVE('',#7920,#7920,#2962,.T.);
#10468=EDGE_CURVE('',#7920,#7921,#5279,.T.);
#10469=EDGE_CURVE('',#7921,#7921,#2963,.T.);
#10470=EDGE_CURVE('',#7922,#7922,#2964,.T.);
#10471=EDGE_CURVE('',#7922,#7771,#5280,.T.);
#10472=EDGE_CURVE('',#7772,#7923,#5281,.T.);
#10473=EDGE_CURVE('',#7923,#7923,#2965,.T.);
#10474=EDGE_CURVE('',#7924,#7924,#2966,.T.);
#10475=EDGE_CURVE('',#7924,#7925,#5282,.T.);
#10476=EDGE_CURVE('',#7925,#7925,#2967,.T.);
#10477=EDGE_CURVE('',#7926,#7926,#2968,.T.);
#10478=EDGE_CURVE('',#7926,#7727,#5283,.T.);
#10479=EDGE_CURVE('',#7728,#7927,#5284,.T.);
#10480=EDGE_CURVE('',#7927,#7927,#2969,.T.);
#10481=EDGE_CURVE('',#7928,#7928,#2970,.T.);
#10482=EDGE_CURVE('',#7928,#7929,#5285,.T.);
#10483=EDGE_CURVE('',#7929,#7929,#2971,.T.);
#10484=EDGE_CURVE('',#7930,#7930,#2972,.T.);
#10485=EDGE_CURVE('',#7930,#7683,#5286,.T.);
#10486=EDGE_CURVE('',#7684,#7931,#5287,.T.);
#10487=EDGE_CURVE('',#7931,#7931,#2973,.T.);
#10488=EDGE_CURVE('',#7932,#7932,#2974,.T.);
#10489=EDGE_CURVE('',#7932,#7933,#5288,.T.);
#10490=EDGE_CURVE('',#7933,#7933,#2975,.T.);
#10491=EDGE_CURVE('',#7934,#7934,#2976,.T.);
#10492=EDGE_CURVE('',#7934,#7639,#5289,.T.);
#10493=EDGE_CURVE('',#7640,#7935,#5290,.T.);
#10494=EDGE_CURVE('',#7935,#7935,#2977,.T.);
#10495=EDGE_CURVE('',#7936,#7936,#2978,.T.);
#10496=EDGE_CURVE('',#7936,#7937,#5291,.T.);
#10497=EDGE_CURVE('',#7937,#7937,#2979,.T.);
#10498=EDGE_CURVE('',#7938,#7938,#2980,.T.);
#10499=EDGE_CURVE('',#7938,#7375,#5292,.T.);
#10500=EDGE_CURVE('',#7376,#7939,#5293,.T.);
#10501=EDGE_CURVE('',#7939,#7939,#2981,.T.);
#10502=EDGE_CURVE('',#7940,#7912,#4485,.T.);
#10503=EDGE_CURVE('',#7940,#7941,#5294,.T.);
#10504=EDGE_CURVE('',#7941,#7913,#5295,.T.);
#10505=EDGE_CURVE('',#7863,#7942,#4486,.T.);
#10506=EDGE_CURVE('',#7943,#7915,#5296,.T.);
#10507=EDGE_CURVE('',#7943,#7942,#5297,.T.);
#10508=EDGE_CURVE('',#7944,#7943,#5298,.T.);
#10509=EDGE_CURVE('',#7944,#7914,#5299,.T.);
#10510=EDGE_CURVE('',#7941,#7944,#5300,.T.);
#10511=EDGE_CURVE('',#7907,#7945,#4487,.T.);
#10512=EDGE_CURVE('',#7946,#7906,#5301,.T.);
#10513=EDGE_CURVE('',#7946,#7945,#5302,.T.);
#10514=EDGE_CURVE('',#7947,#7946,#5303,.T.);
#10515=EDGE_CURVE('',#7947,#7905,#5304,.T.);
#10516=EDGE_CURVE('',#7948,#7947,#5305,.T.);
#10517=EDGE_CURVE('',#7948,#7904,#5306,.T.);
#10518=EDGE_CURVE('',#7949,#7903,#4488,.T.);
#10519=EDGE_CURVE('',#7949,#7948,#5307,.T.);
#10520=EDGE_CURVE('',#7898,#7950,#4489,.T.);
#10521=EDGE_CURVE('',#7951,#7897,#5308,.T.);
#10522=EDGE_CURVE('',#7951,#7950,#5309,.T.);
#10523=EDGE_CURVE('',#7952,#7951,#5310,.T.);
#10524=EDGE_CURVE('',#7952,#7896,#5311,.T.);
#10525=EDGE_CURVE('',#7953,#7952,#5312,.T.);
#10526=EDGE_CURVE('',#7953,#7895,#5313,.T.);
#10527=EDGE_CURVE('',#7954,#7894,#4490,.T.);
#10528=EDGE_CURVE('',#7954,#7953,#5314,.T.);
#10529=EDGE_CURVE('',#7889,#7955,#4491,.T.);
#10530=EDGE_CURVE('',#7956,#7888,#5315,.T.);
#10531=EDGE_CURVE('',#7956,#7955,#5316,.T.);
#10532=EDGE_CURVE('',#7957,#7956,#5317,.T.);
#10533=EDGE_CURVE('',#7957,#7887,#5318,.T.);
#10534=EDGE_CURVE('',#7958,#7957,#5319,.T.);
#10535=EDGE_CURVE('',#7958,#7886,#5320,.T.);
#10536=EDGE_CURVE('',#7959,#7885,#4492,.T.);
#10537=EDGE_CURVE('',#7959,#7958,#5321,.T.);
#10538=EDGE_CURVE('',#7960,#7876,#4493,.T.);
#10539=EDGE_CURVE('',#7960,#7961,#5322,.T.);
#10540=EDGE_CURVE('',#7961,#7877,#5323,.T.);
#10541=EDGE_CURVE('',#7880,#7962,#4494,.T.);
#10542=EDGE_CURVE('',#7963,#7879,#5324,.T.);
#10543=EDGE_CURVE('',#7963,#7962,#5325,.T.);
#10544=EDGE_CURVE('',#7964,#7963,#5326,.T.);
#10545=EDGE_CURVE('',#7964,#7878,#5327,.T.);
#10546=EDGE_CURVE('',#7961,#7964,#5328,.T.);
#10547=EDGE_CURVE('',#7942,#7965,#4495,.T.);
#10548=EDGE_CURVE('',#7862,#7965,#5329,.T.);
#10549=EDGE_CURVE('',#7945,#7966,#4496,.T.);
#10550=EDGE_CURVE('',#7908,#7966,#5330,.T.);
#10551=EDGE_CURVE('',#7967,#7902,#5331,.T.);
#10552=EDGE_CURVE('',#7967,#7949,#4497,.T.);
#10553=EDGE_CURVE('',#7950,#7968,#4498,.T.);
#10554=EDGE_CURVE('',#7899,#7968,#5332,.T.);
#10555=EDGE_CURVE('',#7969,#7893,#5333,.T.);
#10556=EDGE_CURVE('',#7969,#7954,#4499,.T.);
#10557=EDGE_CURVE('',#7955,#7970,#4500,.T.);
#10558=EDGE_CURVE('',#7890,#7970,#5334,.T.);
#10559=EDGE_CURVE('',#7971,#7884,#5335,.T.);
#10560=EDGE_CURVE('',#7971,#7959,#4501,.T.);
#10561=EDGE_CURVE('',#7962,#7972,#4502,.T.);
#10562=EDGE_CURVE('',#7881,#7972,#5336,.T.);
#10563=EDGE_CURVE('',#7973,#7867,#4503,.T.);
#10564=EDGE_CURVE('',#7973,#7974,#5337,.T.);
#10565=EDGE_CURVE('',#7974,#7868,#5338,.T.);
#10566=EDGE_CURVE('',#7871,#7975,#4504,.T.);
#10567=EDGE_CURVE('',#7976,#7870,#5339,.T.);
#10568=EDGE_CURVE('',#7976,#7975,#5340,.T.);
#10569=EDGE_CURVE('',#7977,#7976,#5341,.T.);
#10570=EDGE_CURVE('',#7977,#7869,#5342,.T.);
#10571=EDGE_CURVE('',#7974,#7977,#5343,.T.);
#10572=EDGE_CURVE('',#7975,#7978,#4505,.T.);
#10573=EDGE_CURVE('',#7872,#7978,#5344,.T.);
#10574=EDGE_CURVE('',#7979,#7901,#5345,.T.);
#10575=EDGE_CURVE('',#7979,#7967,#2982,.T.);
#10576=EDGE_CURVE('',#7900,#7980,#5346,.T.);
#10577=EDGE_CURVE('',#7980,#7979,#2983,.T.);
#10578=EDGE_CURVE('',#7968,#7980,#5347,.T.);
#10579=EDGE_CURVE('',#7981,#7892,#5348,.T.);
#10580=EDGE_CURVE('',#7981,#7969,#2984,.T.);
#10581=EDGE_CURVE('',#7891,#7982,#5349,.T.);
#10582=EDGE_CURVE('',#7982,#7981,#2985,.T.);
#10583=EDGE_CURVE('',#7970,#7982,#5350,.T.);
#10584=EDGE_CURVE('',#7983,#7883,#5351,.T.);
#10585=EDGE_CURVE('',#7983,#7971,#2986,.T.);
#10586=EDGE_CURVE('',#7882,#7984,#5352,.T.);
#10587=EDGE_CURVE('',#7984,#7983,#2987,.T.);
#10588=EDGE_CURVE('',#7972,#7984,#5353,.T.);
#10589=EDGE_CURVE('',#7985,#7940,#4506,.T.);
#10590=EDGE_CURVE('',#7986,#7985,#2988,.T.);
#10591=EDGE_CURVE('',#7987,#7986,#2989,.T.);
#10592=EDGE_CURVE('',#7966,#7987,#5354,.T.);
#10593=EDGE_CURVE('',#7988,#7960,#4507,.T.);
#10594=EDGE_CURVE('',#7989,#7988,#2990,.T.);
#10595=EDGE_CURVE('',#7990,#7989,#2991,.T.);
#10596=EDGE_CURVE('',#7978,#7990,#5355,.T.);
#10597=EDGE_CURVE('',#7991,#7973,#4508,.T.);
#10598=EDGE_CURVE('',#7992,#7991,#2992,.T.);
#10599=EDGE_CURVE('',#7993,#7992,#2993,.T.);
#10600=EDGE_CURVE('',#7965,#7993,#5356,.T.);
#10601=EDGE_CURVE('',#7855,#7860,#2994,.T.);
#10602=EDGE_CURVE('',#7909,#7987,#5357,.T.);
#10603=EDGE_CURVE('',#7986,#7910,#5358,.T.);
#10604=EDGE_CURVE('',#7985,#7911,#5359,.T.);
#10605=EDGE_CURVE('',#7864,#7993,#5360,.T.);
#10606=EDGE_CURVE('',#7992,#7865,#5361,.T.);
#10607=EDGE_CURVE('',#7991,#7866,#5362,.T.);
#10608=EDGE_CURVE('',#7873,#7990,#5363,.T.);
#10609=EDGE_CURVE('',#7988,#7875,#5364,.T.);
#10610=EDGE_CURVE('',#7989,#7874,#5365,.T.);
#13678=ORIENTED_EDGE('',*,*,#9591,.T.);
#13679=ORIENTED_EDGE('',*,*,#9592,.T.);
#13680=ORIENTED_EDGE('',*,*,#9593,.T.);
#13681=ORIENTED_EDGE('',*,*,#9594,.T.);
#13682=ORIENTED_EDGE('',*,*,#9595,.T.);
#13683=ORIENTED_EDGE('',*,*,#9596,.T.);
#13684=ORIENTED_EDGE('',*,*,#9597,.T.);
#13685=ORIENTED_EDGE('',*,*,#9594,.F.);
#13686=ORIENTED_EDGE('',*,*,#9598,.T.);
#13687=ORIENTED_EDGE('',*,*,#9599,.T.);
#13688=ORIENTED_EDGE('',*,*,#9600,.T.);
#13689=ORIENTED_EDGE('',*,*,#9601,.T.);
#13690=ORIENTED_EDGE('',*,*,#9591,.F.);
#13691=ORIENTED_EDGE('',*,*,#9602,.T.);
#13692=ORIENTED_EDGE('',*,*,#9603,.T.);
#13693=ORIENTED_EDGE('',*,*,#9604,.T.);
#13694=ORIENTED_EDGE('',*,*,#9600,.F.);
#13695=ORIENTED_EDGE('',*,*,#9605,.T.);
#13696=ORIENTED_EDGE('',*,*,#9606,.T.);
#13697=ORIENTED_EDGE('',*,*,#9607,.T.);
#13698=ORIENTED_EDGE('',*,*,#9603,.F.);
#13699=ORIENTED_EDGE('',*,*,#9608,.T.);
#13700=ORIENTED_EDGE('',*,*,#9609,.T.);
#13701=ORIENTED_EDGE('',*,*,#9610,.T.);
#13702=ORIENTED_EDGE('',*,*,#9606,.F.);
#13703=ORIENTED_EDGE('',*,*,#9611,.T.);
#13704=ORIENTED_EDGE('',*,*,#9612,.T.);
#13705=ORIENTED_EDGE('',*,*,#9613,.T.);
#13706=ORIENTED_EDGE('',*,*,#9609,.F.);
#13707=ORIENTED_EDGE('',*,*,#9614,.T.);
#13708=ORIENTED_EDGE('',*,*,#9615,.T.);
#13709=ORIENTED_EDGE('',*,*,#9616,.T.);
#13710=ORIENTED_EDGE('',*,*,#9612,.F.);
#13711=ORIENTED_EDGE('',*,*,#9617,.T.);
#13712=ORIENTED_EDGE('',*,*,#9618,.F.);
#13713=ORIENTED_EDGE('',*,*,#9619,.T.);
#13714=ORIENTED_EDGE('',*,*,#9620,.F.);
#13715=ORIENTED_EDGE('',*,*,#9621,.T.);
#13716=ORIENTED_EDGE('',*,*,#9622,.T.);
#13717=ORIENTED_EDGE('',*,*,#9623,.T.);
#13718=ORIENTED_EDGE('',*,*,#9624,.F.);
#13719=ORIENTED_EDGE('',*,*,#9625,.F.);
#13720=ORIENTED_EDGE('',*,*,#9626,.T.);
#13721=ORIENTED_EDGE('',*,*,#9627,.T.);
#13722=ORIENTED_EDGE('',*,*,#9622,.F.);
#13723=ORIENTED_EDGE('',*,*,#9628,.F.);
#13724=ORIENTED_EDGE('',*,*,#9629,.T.);
#13725=ORIENTED_EDGE('',*,*,#9630,.T.);
#13726=ORIENTED_EDGE('',*,*,#9626,.F.);
#13727=ORIENTED_EDGE('',*,*,#9631,.F.);
#13728=ORIENTED_EDGE('',*,*,#9632,.T.);
#13729=ORIENTED_EDGE('',*,*,#9633,.T.);
#13730=ORIENTED_EDGE('',*,*,#9629,.F.);
#13731=ORIENTED_EDGE('',*,*,#9634,.F.);
#13732=ORIENTED_EDGE('',*,*,#9635,.T.);
#13733=ORIENTED_EDGE('',*,*,#9636,.T.);
#13734=ORIENTED_EDGE('',*,*,#9632,.F.);
#13735=ORIENTED_EDGE('',*,*,#9637,.F.);
#13736=ORIENTED_EDGE('',*,*,#9638,.T.);
#13737=ORIENTED_EDGE('',*,*,#9639,.T.);
#13738=ORIENTED_EDGE('',*,*,#9635,.F.);
#13739=ORIENTED_EDGE('',*,*,#9640,.F.);
#13740=ORIENTED_EDGE('',*,*,#9641,.T.);
#13741=ORIENTED_EDGE('',*,*,#9642,.T.);
#13742=ORIENTED_EDGE('',*,*,#9638,.F.);
#13743=ORIENTED_EDGE('',*,*,#9643,.F.);
#13744=ORIENTED_EDGE('',*,*,#9644,.F.);
#13745=ORIENTED_EDGE('',*,*,#9645,.F.);
#13746=ORIENTED_EDGE('',*,*,#9646,.F.);
#13747=ORIENTED_EDGE('',*,*,#9647,.T.);
#13748=ORIENTED_EDGE('',*,*,#9648,.T.);
#13749=ORIENTED_EDGE('',*,*,#9649,.T.);
#13750=ORIENTED_EDGE('',*,*,#9650,.T.);
#13751=ORIENTED_EDGE('',*,*,#9651,.T.);
#13752=ORIENTED_EDGE('',*,*,#9652,.T.);
#13753=ORIENTED_EDGE('',*,*,#9653,.T.);
#13754=ORIENTED_EDGE('',*,*,#9654,.T.);
#13755=ORIENTED_EDGE('',*,*,#9651,.F.);
#13756=ORIENTED_EDGE('',*,*,#9655,.T.);
#13757=ORIENTED_EDGE('',*,*,#9656,.T.);
#13758=ORIENTED_EDGE('',*,*,#9657,.T.);
#13759=ORIENTED_EDGE('',*,*,#9658,.T.);
#13760=ORIENTED_EDGE('',*,*,#9648,.F.);
#13761=ORIENTED_EDGE('',*,*,#9659,.T.);
#13762=ORIENTED_EDGE('',*,*,#9660,.T.);
#13763=ORIENTED_EDGE('',*,*,#9661,.T.);
#13764=ORIENTED_EDGE('',*,*,#9657,.F.);
#13765=ORIENTED_EDGE('',*,*,#9662,.T.);
#13766=ORIENTED_EDGE('',*,*,#9663,.T.);
#13767=ORIENTED_EDGE('',*,*,#9664,.T.);
#13768=ORIENTED_EDGE('',*,*,#9660,.F.);
#13769=ORIENTED_EDGE('',*,*,#9665,.T.);
#13770=ORIENTED_EDGE('',*,*,#9666,.T.);
#13771=ORIENTED_EDGE('',*,*,#9667,.T.);
#13772=ORIENTED_EDGE('',*,*,#9663,.F.);
#13773=ORIENTED_EDGE('',*,*,#9668,.T.);
#13774=ORIENTED_EDGE('',*,*,#9669,.T.);
#13775=ORIENTED_EDGE('',*,*,#9670,.T.);
#13776=ORIENTED_EDGE('',*,*,#9666,.F.);
#13777=ORIENTED_EDGE('',*,*,#9671,.T.);
#13778=ORIENTED_EDGE('',*,*,#9672,.T.);
#13779=ORIENTED_EDGE('',*,*,#9673,.T.);
#13780=ORIENTED_EDGE('',*,*,#9669,.F.);
#13781=ORIENTED_EDGE('',*,*,#9674,.T.);
#13782=ORIENTED_EDGE('',*,*,#9675,.F.);
#13783=ORIENTED_EDGE('',*,*,#9676,.T.);
#13784=ORIENTED_EDGE('',*,*,#9677,.F.);
#13785=ORIENTED_EDGE('',*,*,#9678,.T.);
#13786=ORIENTED_EDGE('',*,*,#9679,.T.);
#13787=ORIENTED_EDGE('',*,*,#9680,.T.);
#13788=ORIENTED_EDGE('',*,*,#9681,.F.);
#13789=ORIENTED_EDGE('',*,*,#9682,.F.);
#13790=ORIENTED_EDGE('',*,*,#9683,.T.);
#13791=ORIENTED_EDGE('',*,*,#9684,.T.);
#13792=ORIENTED_EDGE('',*,*,#9679,.F.);
#13793=ORIENTED_EDGE('',*,*,#9685,.F.);
#13794=ORIENTED_EDGE('',*,*,#9686,.T.);
#13795=ORIENTED_EDGE('',*,*,#9687,.T.);
#13796=ORIENTED_EDGE('',*,*,#9683,.F.);
#13797=ORIENTED_EDGE('',*,*,#9688,.F.);
#13798=ORIENTED_EDGE('',*,*,#9689,.T.);
#13799=ORIENTED_EDGE('',*,*,#9690,.T.);
#13800=ORIENTED_EDGE('',*,*,#9686,.F.);
#13801=ORIENTED_EDGE('',*,*,#9691,.F.);
#13802=ORIENTED_EDGE('',*,*,#9692,.T.);
#13803=ORIENTED_EDGE('',*,*,#9693,.T.);
#13804=ORIENTED_EDGE('',*,*,#9689,.F.);
#13805=ORIENTED_EDGE('',*,*,#9694,.F.);
#13806=ORIENTED_EDGE('',*,*,#9695,.T.);
#13807=ORIENTED_EDGE('',*,*,#9696,.T.);
#13808=ORIENTED_EDGE('',*,*,#9692,.F.);
#13809=ORIENTED_EDGE('',*,*,#9697,.F.);
#13810=ORIENTED_EDGE('',*,*,#9698,.T.);
#13811=ORIENTED_EDGE('',*,*,#9699,.T.);
#13812=ORIENTED_EDGE('',*,*,#9695,.F.);
#13813=ORIENTED_EDGE('',*,*,#9700,.F.);
#13814=ORIENTED_EDGE('',*,*,#9701,.F.);
#13815=ORIENTED_EDGE('',*,*,#9702,.F.);
#13816=ORIENTED_EDGE('',*,*,#9703,.F.);
#13817=ORIENTED_EDGE('',*,*,#9704,.T.);
#13818=ORIENTED_EDGE('',*,*,#9705,.T.);
#13819=ORIENTED_EDGE('',*,*,#9706,.T.);
#13820=ORIENTED_EDGE('',*,*,#9707,.T.);
#13821=ORIENTED_EDGE('',*,*,#9708,.T.);
#13822=ORIENTED_EDGE('',*,*,#9709,.T.);
#13823=ORIENTED_EDGE('',*,*,#9710,.T.);
#13824=ORIENTED_EDGE('',*,*,#9711,.T.);
#13825=ORIENTED_EDGE('',*,*,#9708,.F.);
#13826=ORIENTED_EDGE('',*,*,#9712,.T.);
#13827=ORIENTED_EDGE('',*,*,#9713,.T.);
#13828=ORIENTED_EDGE('',*,*,#9714,.T.);
#13829=ORIENTED_EDGE('',*,*,#9715,.T.);
#13830=ORIENTED_EDGE('',*,*,#9705,.F.);
#13831=ORIENTED_EDGE('',*,*,#9716,.T.);
#13832=ORIENTED_EDGE('',*,*,#9717,.T.);
#13833=ORIENTED_EDGE('',*,*,#9718,.T.);
#13834=ORIENTED_EDGE('',*,*,#9714,.F.);
#13835=ORIENTED_EDGE('',*,*,#9719,.T.);
#13836=ORIENTED_EDGE('',*,*,#9720,.T.);
#13837=ORIENTED_EDGE('',*,*,#9721,.T.);
#13838=ORIENTED_EDGE('',*,*,#9717,.F.);
#13839=ORIENTED_EDGE('',*,*,#9722,.T.);
#13840=ORIENTED_EDGE('',*,*,#9723,.T.);
#13841=ORIENTED_EDGE('',*,*,#9724,.T.);
#13842=ORIENTED_EDGE('',*,*,#9720,.F.);
#13843=ORIENTED_EDGE('',*,*,#9725,.T.);
#13844=ORIENTED_EDGE('',*,*,#9726,.T.);
#13845=ORIENTED_EDGE('',*,*,#9727,.T.);
#13846=ORIENTED_EDGE('',*,*,#9723,.F.);
#13847=ORIENTED_EDGE('',*,*,#9728,.T.);
#13848=ORIENTED_EDGE('',*,*,#9729,.T.);
#13849=ORIENTED_EDGE('',*,*,#9730,.T.);
#13850=ORIENTED_EDGE('',*,*,#9726,.F.);
#13851=ORIENTED_EDGE('',*,*,#9731,.T.);
#13852=ORIENTED_EDGE('',*,*,#9732,.F.);
#13853=ORIENTED_EDGE('',*,*,#9733,.T.);
#13854=ORIENTED_EDGE('',*,*,#9734,.F.);
#13855=ORIENTED_EDGE('',*,*,#9735,.T.);
#13856=ORIENTED_EDGE('',*,*,#9736,.T.);
#13857=ORIENTED_EDGE('',*,*,#9737,.T.);
#13858=ORIENTED_EDGE('',*,*,#9738,.F.);
#13859=ORIENTED_EDGE('',*,*,#9739,.F.);
#13860=ORIENTED_EDGE('',*,*,#9740,.T.);
#13861=ORIENTED_EDGE('',*,*,#9741,.T.);
#13862=ORIENTED_EDGE('',*,*,#9736,.F.);
#13863=ORIENTED_EDGE('',*,*,#9742,.F.);
#13864=ORIENTED_EDGE('',*,*,#9743,.T.);
#13865=ORIENTED_EDGE('',*,*,#9744,.T.);
#13866=ORIENTED_EDGE('',*,*,#9740,.F.);
#13867=ORIENTED_EDGE('',*,*,#9745,.F.);
#13868=ORIENTED_EDGE('',*,*,#9746,.T.);
#13869=ORIENTED_EDGE('',*,*,#9747,.T.);
#13870=ORIENTED_EDGE('',*,*,#9743,.F.);
#13871=ORIENTED_EDGE('',*,*,#9748,.F.);
#13872=ORIENTED_EDGE('',*,*,#9749,.T.);
#13873=ORIENTED_EDGE('',*,*,#9750,.T.);
#13874=ORIENTED_EDGE('',*,*,#9746,.F.);
#13875=ORIENTED_EDGE('',*,*,#9751,.F.);
#13876=ORIENTED_EDGE('',*,*,#9752,.T.);
#13877=ORIENTED_EDGE('',*,*,#9753,.T.);
#13878=ORIENTED_EDGE('',*,*,#9749,.F.);
#13879=ORIENTED_EDGE('',*,*,#9754,.F.);
#13880=ORIENTED_EDGE('',*,*,#9755,.T.);
#13881=ORIENTED_EDGE('',*,*,#9756,.T.);
#13882=ORIENTED_EDGE('',*,*,#9752,.F.);
#13883=ORIENTED_EDGE('',*,*,#9757,.F.);
#13884=ORIENTED_EDGE('',*,*,#9758,.F.);
#13885=ORIENTED_EDGE('',*,*,#9759,.F.);
#13886=ORIENTED_EDGE('',*,*,#9760,.F.);
#13887=ORIENTED_EDGE('',*,*,#9761,.T.);
#13888=ORIENTED_EDGE('',*,*,#9762,.T.);
#13889=ORIENTED_EDGE('',*,*,#9763,.T.);
#13890=ORIENTED_EDGE('',*,*,#9764,.T.);
#13891=ORIENTED_EDGE('',*,*,#9765,.T.);
#13892=ORIENTED_EDGE('',*,*,#9766,.T.);
#13893=ORIENTED_EDGE('',*,*,#9767,.T.);
#13894=ORIENTED_EDGE('',*,*,#9768,.T.);
#13895=ORIENTED_EDGE('',*,*,#9765,.F.);
#13896=ORIENTED_EDGE('',*,*,#9769,.T.);
#13897=ORIENTED_EDGE('',*,*,#9770,.T.);
#13898=ORIENTED_EDGE('',*,*,#9771,.T.);
#13899=ORIENTED_EDGE('',*,*,#9772,.T.);
#13900=ORIENTED_EDGE('',*,*,#9762,.F.);
#13901=ORIENTED_EDGE('',*,*,#9773,.T.);
#13902=ORIENTED_EDGE('',*,*,#9774,.T.);
#13903=ORIENTED_EDGE('',*,*,#9775,.T.);
#13904=ORIENTED_EDGE('',*,*,#9771,.F.);
#13905=ORIENTED_EDGE('',*,*,#9776,.T.);
#13906=ORIENTED_EDGE('',*,*,#9777,.T.);
#13907=ORIENTED_EDGE('',*,*,#9778,.T.);
#13908=ORIENTED_EDGE('',*,*,#9774,.F.);
#13909=ORIENTED_EDGE('',*,*,#9779,.T.);
#13910=ORIENTED_EDGE('',*,*,#9780,.T.);
#13911=ORIENTED_EDGE('',*,*,#9781,.T.);
#13912=ORIENTED_EDGE('',*,*,#9777,.F.);
#13913=ORIENTED_EDGE('',*,*,#9782,.T.);
#13914=ORIENTED_EDGE('',*,*,#9783,.T.);
#13915=ORIENTED_EDGE('',*,*,#9784,.T.);
#13916=ORIENTED_EDGE('',*,*,#9780,.F.);
#13917=ORIENTED_EDGE('',*,*,#9785,.T.);
#13918=ORIENTED_EDGE('',*,*,#9786,.T.);
#13919=ORIENTED_EDGE('',*,*,#9787,.T.);
#13920=ORIENTED_EDGE('',*,*,#9783,.F.);
#13921=ORIENTED_EDGE('',*,*,#9788,.T.);
#13922=ORIENTED_EDGE('',*,*,#9789,.F.);
#13923=ORIENTED_EDGE('',*,*,#9790,.T.);
#13924=ORIENTED_EDGE('',*,*,#9791,.F.);
#13925=ORIENTED_EDGE('',*,*,#9792,.T.);
#13926=ORIENTED_EDGE('',*,*,#9793,.T.);
#13927=ORIENTED_EDGE('',*,*,#9794,.T.);
#13928=ORIENTED_EDGE('',*,*,#9795,.F.);
#13929=ORIENTED_EDGE('',*,*,#9796,.F.);
#13930=ORIENTED_EDGE('',*,*,#9797,.T.);
#13931=ORIENTED_EDGE('',*,*,#9798,.T.);
#13932=ORIENTED_EDGE('',*,*,#9793,.F.);
#13933=ORIENTED_EDGE('',*,*,#9799,.F.);
#13934=ORIENTED_EDGE('',*,*,#9800,.T.);
#13935=ORIENTED_EDGE('',*,*,#9801,.T.);
#13936=ORIENTED_EDGE('',*,*,#9797,.F.);
#13937=ORIENTED_EDGE('',*,*,#9802,.F.);
#13938=ORIENTED_EDGE('',*,*,#9803,.T.);
#13939=ORIENTED_EDGE('',*,*,#9804,.T.);
#13940=ORIENTED_EDGE('',*,*,#9800,.F.);
#13941=ORIENTED_EDGE('',*,*,#9805,.F.);
#13942=ORIENTED_EDGE('',*,*,#9806,.T.);
#13943=ORIENTED_EDGE('',*,*,#9807,.T.);
#13944=ORIENTED_EDGE('',*,*,#9803,.F.);
#13945=ORIENTED_EDGE('',*,*,#9808,.F.);
#13946=ORIENTED_EDGE('',*,*,#9809,.T.);
#13947=ORIENTED_EDGE('',*,*,#9810,.T.);
#13948=ORIENTED_EDGE('',*,*,#9806,.F.);
#13949=ORIENTED_EDGE('',*,*,#9811,.F.);
#13950=ORIENTED_EDGE('',*,*,#9812,.T.);
#13951=ORIENTED_EDGE('',*,*,#9813,.T.);
#13952=ORIENTED_EDGE('',*,*,#9809,.F.);
#13953=ORIENTED_EDGE('',*,*,#9814,.F.);
#13954=ORIENTED_EDGE('',*,*,#9815,.F.);
#13955=ORIENTED_EDGE('',*,*,#9816,.F.);
#13956=ORIENTED_EDGE('',*,*,#9817,.F.);
#13957=ORIENTED_EDGE('',*,*,#9818,.T.);
#13958=ORIENTED_EDGE('',*,*,#9819,.T.);
#13959=ORIENTED_EDGE('',*,*,#9820,.T.);
#13960=ORIENTED_EDGE('',*,*,#9821,.T.);
#13961=ORIENTED_EDGE('',*,*,#9822,.T.);
#13962=ORIENTED_EDGE('',*,*,#9823,.T.);
#13963=ORIENTED_EDGE('',*,*,#9824,.T.);
#13964=ORIENTED_EDGE('',*,*,#9825,.T.);
#13965=ORIENTED_EDGE('',*,*,#9822,.F.);
#13966=ORIENTED_EDGE('',*,*,#9826,.T.);
#13967=ORIENTED_EDGE('',*,*,#9827,.T.);
#13968=ORIENTED_EDGE('',*,*,#9828,.T.);
#13969=ORIENTED_EDGE('',*,*,#9829,.T.);
#13970=ORIENTED_EDGE('',*,*,#9819,.F.);
#13971=ORIENTED_EDGE('',*,*,#9830,.T.);
#13972=ORIENTED_EDGE('',*,*,#9831,.T.);
#13973=ORIENTED_EDGE('',*,*,#9832,.T.);
#13974=ORIENTED_EDGE('',*,*,#9828,.F.);
#13975=ORIENTED_EDGE('',*,*,#9833,.T.);
#13976=ORIENTED_EDGE('',*,*,#9834,.T.);
#13977=ORIENTED_EDGE('',*,*,#9835,.T.);
#13978=ORIENTED_EDGE('',*,*,#9831,.F.);
#13979=ORIENTED_EDGE('',*,*,#9836,.T.);
#13980=ORIENTED_EDGE('',*,*,#9837,.T.);
#13981=ORIENTED_EDGE('',*,*,#9838,.T.);
#13982=ORIENTED_EDGE('',*,*,#9834,.F.);
#13983=ORIENTED_EDGE('',*,*,#9839,.T.);
#13984=ORIENTED_EDGE('',*,*,#9840,.T.);
#13985=ORIENTED_EDGE('',*,*,#9841,.T.);
#13986=ORIENTED_EDGE('',*,*,#9837,.F.);
#13987=ORIENTED_EDGE('',*,*,#9842,.T.);
#13988=ORIENTED_EDGE('',*,*,#9843,.T.);
#13989=ORIENTED_EDGE('',*,*,#9844,.T.);
#13990=ORIENTED_EDGE('',*,*,#9840,.F.);
#13991=ORIENTED_EDGE('',*,*,#9845,.T.);
#13992=ORIENTED_EDGE('',*,*,#9846,.F.);
#13993=ORIENTED_EDGE('',*,*,#9847,.T.);
#13994=ORIENTED_EDGE('',*,*,#9848,.F.);
#13995=ORIENTED_EDGE('',*,*,#9849,.T.);
#13996=ORIENTED_EDGE('',*,*,#9850,.T.);
#13997=ORIENTED_EDGE('',*,*,#9851,.T.);
#13998=ORIENTED_EDGE('',*,*,#9852,.F.);
#13999=ORIENTED_EDGE('',*,*,#9853,.F.);
#14000=ORIENTED_EDGE('',*,*,#9854,.T.);
#14001=ORIENTED_EDGE('',*,*,#9855,.T.);
#14002=ORIENTED_EDGE('',*,*,#9850,.F.);
#14003=ORIENTED_EDGE('',*,*,#9856,.F.);
#14004=ORIENTED_EDGE('',*,*,#9857,.T.);
#14005=ORIENTED_EDGE('',*,*,#9858,.T.);
#14006=ORIENTED_EDGE('',*,*,#9854,.F.);
#14007=ORIENTED_EDGE('',*,*,#9859,.F.);
#14008=ORIENTED_EDGE('',*,*,#9860,.T.);
#14009=ORIENTED_EDGE('',*,*,#9861,.T.);
#14010=ORIENTED_EDGE('',*,*,#9857,.F.);
#14011=ORIENTED_EDGE('',*,*,#9862,.F.);
#14012=ORIENTED_EDGE('',*,*,#9863,.T.);
#14013=ORIENTED_EDGE('',*,*,#9864,.T.);
#14014=ORIENTED_EDGE('',*,*,#9860,.F.);
#14015=ORIENTED_EDGE('',*,*,#9865,.F.);
#14016=ORIENTED_EDGE('',*,*,#9866,.T.);
#14017=ORIENTED_EDGE('',*,*,#9867,.T.);
#14018=ORIENTED_EDGE('',*,*,#9863,.F.);
#14019=ORIENTED_EDGE('',*,*,#9868,.F.);
#14020=ORIENTED_EDGE('',*,*,#9869,.T.);
#14021=ORIENTED_EDGE('',*,*,#9870,.T.);
#14022=ORIENTED_EDGE('',*,*,#9866,.F.);
#14023=ORIENTED_EDGE('',*,*,#9871,.F.);
#14024=ORIENTED_EDGE('',*,*,#9872,.F.);
#14025=ORIENTED_EDGE('',*,*,#9873,.F.);
#14026=ORIENTED_EDGE('',*,*,#9874,.F.);
#14027=ORIENTED_EDGE('',*,*,#9875,.T.);
#14028=ORIENTED_EDGE('',*,*,#9876,.T.);
#14029=ORIENTED_EDGE('',*,*,#9877,.T.);
#14030=ORIENTED_EDGE('',*,*,#9878,.T.);
#14031=ORIENTED_EDGE('',*,*,#9879,.T.);
#14032=ORIENTED_EDGE('',*,*,#9880,.T.);
#14033=ORIENTED_EDGE('',*,*,#9881,.T.);
#14034=ORIENTED_EDGE('',*,*,#9882,.T.);
#14035=ORIENTED_EDGE('',*,*,#9879,.F.);
#14036=ORIENTED_EDGE('',*,*,#9883,.T.);
#14037=ORIENTED_EDGE('',*,*,#9884,.T.);
#14038=ORIENTED_EDGE('',*,*,#9885,.T.);
#14039=ORIENTED_EDGE('',*,*,#9886,.T.);
#14040=ORIENTED_EDGE('',*,*,#9876,.F.);
#14041=ORIENTED_EDGE('',*,*,#9887,.T.);
#14042=ORIENTED_EDGE('',*,*,#9888,.T.);
#14043=ORIENTED_EDGE('',*,*,#9889,.T.);
#14044=ORIENTED_EDGE('',*,*,#9885,.F.);
#14045=ORIENTED_EDGE('',*,*,#9890,.T.);
#14046=ORIENTED_EDGE('',*,*,#9891,.T.);
#14047=ORIENTED_EDGE('',*,*,#9892,.T.);
#14048=ORIENTED_EDGE('',*,*,#9888,.F.);
#14049=ORIENTED_EDGE('',*,*,#9893,.T.);
#14050=ORIENTED_EDGE('',*,*,#9894,.T.);
#14051=ORIENTED_EDGE('',*,*,#9895,.T.);
#14052=ORIENTED_EDGE('',*,*,#9891,.F.);
#14053=ORIENTED_EDGE('',*,*,#9896,.T.);
#14054=ORIENTED_EDGE('',*,*,#9897,.T.);
#14055=ORIENTED_EDGE('',*,*,#9898,.T.);
#14056=ORIENTED_EDGE('',*,*,#9894,.F.);
#14057=ORIENTED_EDGE('',*,*,#9899,.T.);
#14058=ORIENTED_EDGE('',*,*,#9900,.T.);
#14059=ORIENTED_EDGE('',*,*,#9901,.T.);
#14060=ORIENTED_EDGE('',*,*,#9897,.F.);
#14061=ORIENTED_EDGE('',*,*,#9902,.T.);
#14062=ORIENTED_EDGE('',*,*,#9903,.F.);
#14063=ORIENTED_EDGE('',*,*,#9904,.T.);
#14064=ORIENTED_EDGE('',*,*,#9905,.F.);
#14065=ORIENTED_EDGE('',*,*,#9906,.T.);
#14066=ORIENTED_EDGE('',*,*,#9907,.T.);
#14067=ORIENTED_EDGE('',*,*,#9908,.T.);
#14068=ORIENTED_EDGE('',*,*,#9909,.F.);
#14069=ORIENTED_EDGE('',*,*,#9910,.F.);
#14070=ORIENTED_EDGE('',*,*,#9911,.T.);
#14071=ORIENTED_EDGE('',*,*,#9912,.T.);
#14072=ORIENTED_EDGE('',*,*,#9907,.F.);
#14073=ORIENTED_EDGE('',*,*,#9913,.F.);
#14074=ORIENTED_EDGE('',*,*,#9914,.T.);
#14075=ORIENTED_EDGE('',*,*,#9915,.T.);
#14076=ORIENTED_EDGE('',*,*,#9911,.F.);
#14077=ORIENTED_EDGE('',*,*,#9916,.F.);
#14078=ORIENTED_EDGE('',*,*,#9917,.T.);
#14079=ORIENTED_EDGE('',*,*,#9918,.T.);
#14080=ORIENTED_EDGE('',*,*,#9914,.F.);
#14081=ORIENTED_EDGE('',*,*,#9919,.F.);
#14082=ORIENTED_EDGE('',*,*,#9920,.T.);
#14083=ORIENTED_EDGE('',*,*,#9921,.T.);
#14084=ORIENTED_EDGE('',*,*,#9917,.F.);
#14085=ORIENTED_EDGE('',*,*,#9922,.F.);
#14086=ORIENTED_EDGE('',*,*,#9923,.T.);
#14087=ORIENTED_EDGE('',*,*,#9924,.T.);
#14088=ORIENTED_EDGE('',*,*,#9920,.F.);
#14089=ORIENTED_EDGE('',*,*,#9925,.F.);
#14090=ORIENTED_EDGE('',*,*,#9926,.T.);
#14091=ORIENTED_EDGE('',*,*,#9927,.T.);
#14092=ORIENTED_EDGE('',*,*,#9923,.F.);
#14093=ORIENTED_EDGE('',*,*,#9928,.F.);
#14094=ORIENTED_EDGE('',*,*,#9929,.F.);
#14095=ORIENTED_EDGE('',*,*,#9930,.F.);
#14096=ORIENTED_EDGE('',*,*,#9931,.F.);
#14097=ORIENTED_EDGE('',*,*,#9932,.T.);
#14098=ORIENTED_EDGE('',*,*,#9933,.T.);
#14099=ORIENTED_EDGE('',*,*,#9934,.T.);
#14100=ORIENTED_EDGE('',*,*,#9935,.T.);
#14101=ORIENTED_EDGE('',*,*,#9936,.T.);
#14102=ORIENTED_EDGE('',*,*,#9937,.T.);
#14103=ORIENTED_EDGE('',*,*,#9938,.T.);
#14104=ORIENTED_EDGE('',*,*,#9939,.T.);
#14105=ORIENTED_EDGE('',*,*,#9936,.F.);
#14106=ORIENTED_EDGE('',*,*,#9940,.T.);
#14107=ORIENTED_EDGE('',*,*,#9941,.T.);
#14108=ORIENTED_EDGE('',*,*,#9942,.T.);
#14109=ORIENTED_EDGE('',*,*,#9943,.T.);
#14110=ORIENTED_EDGE('',*,*,#9933,.F.);
#14111=ORIENTED_EDGE('',*,*,#9944,.T.);
#14112=ORIENTED_EDGE('',*,*,#9945,.T.);
#14113=ORIENTED_EDGE('',*,*,#9946,.T.);
#14114=ORIENTED_EDGE('',*,*,#9942,.F.);
#14115=ORIENTED_EDGE('',*,*,#9947,.T.);
#14116=ORIENTED_EDGE('',*,*,#9948,.T.);
#14117=ORIENTED_EDGE('',*,*,#9949,.T.);
#14118=ORIENTED_EDGE('',*,*,#9945,.F.);
#14119=ORIENTED_EDGE('',*,*,#9950,.T.);
#14120=ORIENTED_EDGE('',*,*,#9951,.T.);
#14121=ORIENTED_EDGE('',*,*,#9952,.T.);
#14122=ORIENTED_EDGE('',*,*,#9948,.F.);
#14123=ORIENTED_EDGE('',*,*,#9953,.T.);
#14124=ORIENTED_EDGE('',*,*,#9954,.T.);
#14125=ORIENTED_EDGE('',*,*,#9955,.T.);
#14126=ORIENTED_EDGE('',*,*,#9951,.F.);
#14127=ORIENTED_EDGE('',*,*,#9956,.T.);
#14128=ORIENTED_EDGE('',*,*,#9957,.T.);
#14129=ORIENTED_EDGE('',*,*,#9958,.T.);
#14130=ORIENTED_EDGE('',*,*,#9954,.F.);
#14131=ORIENTED_EDGE('',*,*,#9959,.T.);
#14132=ORIENTED_EDGE('',*,*,#9960,.F.);
#14133=ORIENTED_EDGE('',*,*,#9961,.T.);
#14134=ORIENTED_EDGE('',*,*,#9962,.F.);
#14135=ORIENTED_EDGE('',*,*,#9963,.T.);
#14136=ORIENTED_EDGE('',*,*,#9964,.T.);
#14137=ORIENTED_EDGE('',*,*,#9965,.T.);
#14138=ORIENTED_EDGE('',*,*,#9966,.F.);
#14139=ORIENTED_EDGE('',*,*,#9967,.F.);
#14140=ORIENTED_EDGE('',*,*,#9968,.T.);
#14141=ORIENTED_EDGE('',*,*,#9969,.T.);
#14142=ORIENTED_EDGE('',*,*,#9964,.F.);
#14143=ORIENTED_EDGE('',*,*,#9970,.F.);
#14144=ORIENTED_EDGE('',*,*,#9971,.T.);
#14145=ORIENTED_EDGE('',*,*,#9972,.T.);
#14146=ORIENTED_EDGE('',*,*,#9968,.F.);
#14147=ORIENTED_EDGE('',*,*,#9973,.F.);
#14148=ORIENTED_EDGE('',*,*,#9974,.T.);
#14149=ORIENTED_EDGE('',*,*,#9975,.T.);
#14150=ORIENTED_EDGE('',*,*,#9971,.F.);
#14151=ORIENTED_EDGE('',*,*,#9976,.F.);
#14152=ORIENTED_EDGE('',*,*,#9977,.T.);
#14153=ORIENTED_EDGE('',*,*,#9978,.T.);
#14154=ORIENTED_EDGE('',*,*,#9974,.F.);
#14155=ORIENTED_EDGE('',*,*,#9979,.F.);
#14156=ORIENTED_EDGE('',*,*,#9980,.T.);
#14157=ORIENTED_EDGE('',*,*,#9981,.T.);
#14158=ORIENTED_EDGE('',*,*,#9977,.F.);
#14159=ORIENTED_EDGE('',*,*,#9982,.F.);
#14160=ORIENTED_EDGE('',*,*,#9983,.T.);
#14161=ORIENTED_EDGE('',*,*,#9984,.T.);
#14162=ORIENTED_EDGE('',*,*,#9980,.F.);
#14163=ORIENTED_EDGE('',*,*,#9985,.F.);
#14164=ORIENTED_EDGE('',*,*,#9986,.F.);
#14165=ORIENTED_EDGE('',*,*,#9987,.F.);
#14166=ORIENTED_EDGE('',*,*,#9988,.F.);
#14167=ORIENTED_EDGE('',*,*,#9989,.T.);
#14168=ORIENTED_EDGE('',*,*,#9990,.T.);
#14169=ORIENTED_EDGE('',*,*,#9991,.T.);
#14170=ORIENTED_EDGE('',*,*,#9992,.T.);
#14171=ORIENTED_EDGE('',*,*,#9993,.T.);
#14172=ORIENTED_EDGE('',*,*,#9994,.T.);
#14173=ORIENTED_EDGE('',*,*,#9995,.T.);
#14174=ORIENTED_EDGE('',*,*,#9996,.T.);
#14175=ORIENTED_EDGE('',*,*,#9993,.F.);
#14176=ORIENTED_EDGE('',*,*,#9997,.T.);
#14177=ORIENTED_EDGE('',*,*,#9998,.T.);
#14178=ORIENTED_EDGE('',*,*,#9999,.T.);
#14179=ORIENTED_EDGE('',*,*,#10000,.T.);
#14180=ORIENTED_EDGE('',*,*,#9990,.F.);
#14181=ORIENTED_EDGE('',*,*,#10001,.T.);
#14182=ORIENTED_EDGE('',*,*,#10002,.T.);
#14183=ORIENTED_EDGE('',*,*,#10003,.T.);
#14184=ORIENTED_EDGE('',*,*,#9999,.F.);
#14185=ORIENTED_EDGE('',*,*,#10004,.T.);
#14186=ORIENTED_EDGE('',*,*,#10005,.T.);
#14187=ORIENTED_EDGE('',*,*,#10006,.T.);
#14188=ORIENTED_EDGE('',*,*,#10002,.F.);
#14189=ORIENTED_EDGE('',*,*,#10007,.T.);
#14190=ORIENTED_EDGE('',*,*,#10008,.T.);
#14191=ORIENTED_EDGE('',*,*,#10009,.T.);
#14192=ORIENTED_EDGE('',*,*,#10005,.F.);
#14193=ORIENTED_EDGE('',*,*,#10010,.T.);
#14194=ORIENTED_EDGE('',*,*,#10011,.T.);
#14195=ORIENTED_EDGE('',*,*,#10012,.T.);
#14196=ORIENTED_EDGE('',*,*,#10008,.F.);
#14197=ORIENTED_EDGE('',*,*,#10013,.T.);
#14198=ORIENTED_EDGE('',*,*,#10014,.T.);
#14199=ORIENTED_EDGE('',*,*,#10015,.T.);
#14200=ORIENTED_EDGE('',*,*,#10011,.F.);
#14201=ORIENTED_EDGE('',*,*,#10016,.T.);
#14202=ORIENTED_EDGE('',*,*,#10017,.F.);
#14203=ORIENTED_EDGE('',*,*,#10018,.T.);
#14204=ORIENTED_EDGE('',*,*,#10019,.F.);
#14205=ORIENTED_EDGE('',*,*,#10020,.T.);
#14206=ORIENTED_EDGE('',*,*,#10021,.T.);
#14207=ORIENTED_EDGE('',*,*,#10022,.T.);
#14208=ORIENTED_EDGE('',*,*,#10023,.F.);
#14209=ORIENTED_EDGE('',*,*,#10024,.F.);
#14210=ORIENTED_EDGE('',*,*,#10025,.T.);
#14211=ORIENTED_EDGE('',*,*,#10026,.T.);
#14212=ORIENTED_EDGE('',*,*,#10021,.F.);
#14213=ORIENTED_EDGE('',*,*,#10027,.F.);
#14214=ORIENTED_EDGE('',*,*,#10028,.T.);
#14215=ORIENTED_EDGE('',*,*,#10029,.T.);
#14216=ORIENTED_EDGE('',*,*,#10025,.F.);
#14217=ORIENTED_EDGE('',*,*,#10030,.F.);
#14218=ORIENTED_EDGE('',*,*,#10031,.T.);
#14219=ORIENTED_EDGE('',*,*,#10032,.T.);
#14220=ORIENTED_EDGE('',*,*,#10028,.F.);
#14221=ORIENTED_EDGE('',*,*,#10033,.F.);
#14222=ORIENTED_EDGE('',*,*,#10034,.T.);
#14223=ORIENTED_EDGE('',*,*,#10035,.T.);
#14224=ORIENTED_EDGE('',*,*,#10031,.F.);
#14225=ORIENTED_EDGE('',*,*,#10036,.F.);
#14226=ORIENTED_EDGE('',*,*,#10037,.T.);
#14227=ORIENTED_EDGE('',*,*,#10038,.T.);
#14228=ORIENTED_EDGE('',*,*,#10034,.F.);
#14229=ORIENTED_EDGE('',*,*,#10039,.F.);
#14230=ORIENTED_EDGE('',*,*,#10040,.T.);
#14231=ORIENTED_EDGE('',*,*,#10041,.T.);
#14232=ORIENTED_EDGE('',*,*,#10037,.F.);
#14233=ORIENTED_EDGE('',*,*,#10042,.F.);
#14234=ORIENTED_EDGE('',*,*,#10043,.F.);
#14235=ORIENTED_EDGE('',*,*,#10044,.F.);
#14236=ORIENTED_EDGE('',*,*,#10045,.F.);
#14237=ORIENTED_EDGE('',*,*,#10046,.T.);
#14238=ORIENTED_EDGE('',*,*,#10047,.T.);
#14239=ORIENTED_EDGE('',*,*,#10048,.T.);
#14240=ORIENTED_EDGE('',*,*,#10049,.T.);
#14241=ORIENTED_EDGE('',*,*,#10050,.T.);
#14242=ORIENTED_EDGE('',*,*,#10051,.T.);
#14243=ORIENTED_EDGE('',*,*,#10052,.T.);
#14244=ORIENTED_EDGE('',*,*,#10053,.T.);
#14245=ORIENTED_EDGE('',*,*,#10050,.F.);
#14246=ORIENTED_EDGE('',*,*,#10054,.T.);
#14247=ORIENTED_EDGE('',*,*,#10055,.T.);
#14248=ORIENTED_EDGE('',*,*,#10056,.T.);
#14249=ORIENTED_EDGE('',*,*,#10057,.T.);
#14250=ORIENTED_EDGE('',*,*,#10047,.F.);
#14251=ORIENTED_EDGE('',*,*,#10058,.T.);
#14252=ORIENTED_EDGE('',*,*,#10059,.T.);
#14253=ORIENTED_EDGE('',*,*,#10060,.T.);
#14254=ORIENTED_EDGE('',*,*,#10056,.F.);
#14255=ORIENTED_EDGE('',*,*,#10061,.T.);
#14256=ORIENTED_EDGE('',*,*,#10062,.T.);
#14257=ORIENTED_EDGE('',*,*,#10063,.T.);
#14258=ORIENTED_EDGE('',*,*,#10059,.F.);
#14259=ORIENTED_EDGE('',*,*,#10064,.T.);
#14260=ORIENTED_EDGE('',*,*,#10065,.T.);
#14261=ORIENTED_EDGE('',*,*,#10066,.T.);
#14262=ORIENTED_EDGE('',*,*,#10062,.F.);
#14263=ORIENTED_EDGE('',*,*,#10067,.T.);
#14264=ORIENTED_EDGE('',*,*,#10068,.T.);
#14265=ORIENTED_EDGE('',*,*,#10069,.T.);
#14266=ORIENTED_EDGE('',*,*,#10065,.F.);
#14267=ORIENTED_EDGE('',*,*,#10070,.T.);
#14268=ORIENTED_EDGE('',*,*,#10071,.T.);
#14269=ORIENTED_EDGE('',*,*,#10072,.T.);
#14270=ORIENTED_EDGE('',*,*,#10068,.F.);
#14271=ORIENTED_EDGE('',*,*,#10073,.T.);
#14272=ORIENTED_EDGE('',*,*,#10074,.F.);
#14273=ORIENTED_EDGE('',*,*,#10075,.T.);
#14274=ORIENTED_EDGE('',*,*,#10076,.F.);
#14275=ORIENTED_EDGE('',*,*,#10077,.T.);
#14276=ORIENTED_EDGE('',*,*,#10078,.T.);
#14277=ORIENTED_EDGE('',*,*,#10079,.T.);
#14278=ORIENTED_EDGE('',*,*,#10080,.F.);
#14279=ORIENTED_EDGE('',*,*,#10081,.F.);
#14280=ORIENTED_EDGE('',*,*,#10082,.T.);
#14281=ORIENTED_EDGE('',*,*,#10083,.T.);
#14282=ORIENTED_EDGE('',*,*,#10078,.F.);
#14283=ORIENTED_EDGE('',*,*,#10084,.F.);
#14284=ORIENTED_EDGE('',*,*,#10085,.T.);
#14285=ORIENTED_EDGE('',*,*,#10086,.T.);
#14286=ORIENTED_EDGE('',*,*,#10082,.F.);
#14287=ORIENTED_EDGE('',*,*,#10087,.F.);
#14288=ORIENTED_EDGE('',*,*,#10088,.T.);
#14289=ORIENTED_EDGE('',*,*,#10089,.T.);
#14290=ORIENTED_EDGE('',*,*,#10085,.F.);
#14291=ORIENTED_EDGE('',*,*,#10090,.F.);
#14292=ORIENTED_EDGE('',*,*,#10091,.T.);
#14293=ORIENTED_EDGE('',*,*,#10092,.T.);
#14294=ORIENTED_EDGE('',*,*,#10088,.F.);
#14295=ORIENTED_EDGE('',*,*,#10093,.F.);
#14296=ORIENTED_EDGE('',*,*,#10094,.T.);
#14297=ORIENTED_EDGE('',*,*,#10095,.T.);
#14298=ORIENTED_EDGE('',*,*,#10091,.F.);
#14299=ORIENTED_EDGE('',*,*,#10096,.F.);
#14300=ORIENTED_EDGE('',*,*,#10097,.T.);
#14301=ORIENTED_EDGE('',*,*,#10098,.T.);
#14302=ORIENTED_EDGE('',*,*,#10094,.F.);
#14303=ORIENTED_EDGE('',*,*,#10099,.F.);
#14304=ORIENTED_EDGE('',*,*,#10100,.F.);
#14305=ORIENTED_EDGE('',*,*,#10101,.F.);
#14306=ORIENTED_EDGE('',*,*,#10102,.F.);
#14307=ORIENTED_EDGE('',*,*,#10103,.T.);
#14308=ORIENTED_EDGE('',*,*,#10104,.T.);
#14309=ORIENTED_EDGE('',*,*,#10105,.T.);
#14310=ORIENTED_EDGE('',*,*,#10106,.T.);
#14311=ORIENTED_EDGE('',*,*,#10107,.T.);
#14312=ORIENTED_EDGE('',*,*,#10108,.T.);
#14313=ORIENTED_EDGE('',*,*,#10109,.T.);
#14314=ORIENTED_EDGE('',*,*,#10110,.T.);
#14315=ORIENTED_EDGE('',*,*,#10107,.F.);
#14316=ORIENTED_EDGE('',*,*,#10111,.T.);
#14317=ORIENTED_EDGE('',*,*,#10112,.T.);
#14318=ORIENTED_EDGE('',*,*,#10113,.T.);
#14319=ORIENTED_EDGE('',*,*,#10114,.T.);
#14320=ORIENTED_EDGE('',*,*,#10104,.F.);
#14321=ORIENTED_EDGE('',*,*,#10115,.T.);
#14322=ORIENTED_EDGE('',*,*,#10116,.T.);
#14323=ORIENTED_EDGE('',*,*,#10117,.T.);
#14324=ORIENTED_EDGE('',*,*,#10113,.F.);
#14325=ORIENTED_EDGE('',*,*,#10118,.T.);
#14326=ORIENTED_EDGE('',*,*,#10119,.T.);
#14327=ORIENTED_EDGE('',*,*,#10120,.T.);
#14328=ORIENTED_EDGE('',*,*,#10116,.F.);
#14329=ORIENTED_EDGE('',*,*,#10121,.T.);
#14330=ORIENTED_EDGE('',*,*,#10122,.T.);
#14331=ORIENTED_EDGE('',*,*,#10123,.T.);
#14332=ORIENTED_EDGE('',*,*,#10119,.F.);
#14333=ORIENTED_EDGE('',*,*,#10124,.T.);
#14334=ORIENTED_EDGE('',*,*,#10125,.T.);
#14335=ORIENTED_EDGE('',*,*,#10126,.T.);
#14336=ORIENTED_EDGE('',*,*,#10122,.F.);
#14337=ORIENTED_EDGE('',*,*,#10127,.T.);
#14338=ORIENTED_EDGE('',*,*,#10128,.T.);
#14339=ORIENTED_EDGE('',*,*,#10129,.T.);
#14340=ORIENTED_EDGE('',*,*,#10125,.F.);
#14341=ORIENTED_EDGE('',*,*,#10130,.T.);
#14342=ORIENTED_EDGE('',*,*,#10131,.F.);
#14343=ORIENTED_EDGE('',*,*,#10132,.T.);
#14344=ORIENTED_EDGE('',*,*,#10133,.F.);
#14345=ORIENTED_EDGE('',*,*,#10134,.T.);
#14346=ORIENTED_EDGE('',*,*,#10135,.T.);
#14347=ORIENTED_EDGE('',*,*,#10136,.T.);
#14348=ORIENTED_EDGE('',*,*,#10137,.F.);
#14349=ORIENTED_EDGE('',*,*,#10138,.F.);
#14350=ORIENTED_EDGE('',*,*,#10139,.T.);
#14351=ORIENTED_EDGE('',*,*,#10140,.T.);
#14352=ORIENTED_EDGE('',*,*,#10135,.F.);
#14353=ORIENTED_EDGE('',*,*,#10141,.F.);
#14354=ORIENTED_EDGE('',*,*,#10142,.T.);
#14355=ORIENTED_EDGE('',*,*,#10143,.T.);
#14356=ORIENTED_EDGE('',*,*,#10139,.F.);
#14357=ORIENTED_EDGE('',*,*,#10144,.F.);
#14358=ORIENTED_EDGE('',*,*,#10145,.T.);
#14359=ORIENTED_EDGE('',*,*,#10146,.T.);
#14360=ORIENTED_EDGE('',*,*,#10142,.F.);
#14361=ORIENTED_EDGE('',*,*,#10147,.F.);
#14362=ORIENTED_EDGE('',*,*,#10148,.T.);
#14363=ORIENTED_EDGE('',*,*,#10149,.T.);
#14364=ORIENTED_EDGE('',*,*,#10145,.F.);
#14365=ORIENTED_EDGE('',*,*,#10150,.F.);
#14366=ORIENTED_EDGE('',*,*,#10151,.T.);
#14367=ORIENTED_EDGE('',*,*,#10152,.T.);
#14368=ORIENTED_EDGE('',*,*,#10148,.F.);
#14369=ORIENTED_EDGE('',*,*,#10153,.F.);
#14370=ORIENTED_EDGE('',*,*,#10154,.T.);
#14371=ORIENTED_EDGE('',*,*,#10155,.T.);
#14372=ORIENTED_EDGE('',*,*,#10151,.F.);
#14373=ORIENTED_EDGE('',*,*,#10156,.F.);
#14374=ORIENTED_EDGE('',*,*,#10157,.F.);
#14375=ORIENTED_EDGE('',*,*,#10158,.F.);
#14376=ORIENTED_EDGE('',*,*,#10159,.F.);
#14377=ORIENTED_EDGE('',*,*,#10160,.T.);
#14378=ORIENTED_EDGE('',*,*,#10161,.T.);
#14379=ORIENTED_EDGE('',*,*,#10162,.T.);
#14380=ORIENTED_EDGE('',*,*,#10163,.T.);
#14381=ORIENTED_EDGE('',*,*,#10164,.T.);
#14382=ORIENTED_EDGE('',*,*,#10165,.T.);
#14383=ORIENTED_EDGE('',*,*,#10166,.T.);
#14384=ORIENTED_EDGE('',*,*,#10167,.T.);
#14385=ORIENTED_EDGE('',*,*,#10164,.F.);
#14386=ORIENTED_EDGE('',*,*,#10168,.T.);
#14387=ORIENTED_EDGE('',*,*,#10169,.T.);
#14388=ORIENTED_EDGE('',*,*,#10170,.T.);
#14389=ORIENTED_EDGE('',*,*,#10171,.T.);
#14390=ORIENTED_EDGE('',*,*,#10161,.F.);
#14391=ORIENTED_EDGE('',*,*,#10172,.T.);
#14392=ORIENTED_EDGE('',*,*,#10173,.T.);
#14393=ORIENTED_EDGE('',*,*,#10174,.T.);
#14394=ORIENTED_EDGE('',*,*,#10170,.F.);
#14395=ORIENTED_EDGE('',*,*,#10175,.T.);
#14396=ORIENTED_EDGE('',*,*,#10176,.T.);
#14397=ORIENTED_EDGE('',*,*,#10177,.T.);
#14398=ORIENTED_EDGE('',*,*,#10173,.F.);
#14399=ORIENTED_EDGE('',*,*,#10178,.T.);
#14400=ORIENTED_EDGE('',*,*,#10179,.T.);
#14401=ORIENTED_EDGE('',*,*,#10180,.T.);
#14402=ORIENTED_EDGE('',*,*,#10176,.F.);
#14403=ORIENTED_EDGE('',*,*,#10181,.T.);
#14404=ORIENTED_EDGE('',*,*,#10182,.T.);
#14405=ORIENTED_EDGE('',*,*,#10183,.T.);
#14406=ORIENTED_EDGE('',*,*,#10179,.F.);
#14407=ORIENTED_EDGE('',*,*,#10184,.T.);
#14408=ORIENTED_EDGE('',*,*,#10185,.T.);
#14409=ORIENTED_EDGE('',*,*,#10186,.T.);
#14410=ORIENTED_EDGE('',*,*,#10182,.F.);
#14411=ORIENTED_EDGE('',*,*,#10187,.T.);
#14412=ORIENTED_EDGE('',*,*,#10188,.F.);
#14413=ORIENTED_EDGE('',*,*,#10189,.T.);
#14414=ORIENTED_EDGE('',*,*,#10190,.F.);
#14415=ORIENTED_EDGE('',*,*,#10191,.T.);
#14416=ORIENTED_EDGE('',*,*,#10192,.T.);
#14417=ORIENTED_EDGE('',*,*,#10193,.T.);
#14418=ORIENTED_EDGE('',*,*,#10194,.F.);
#14419=ORIENTED_EDGE('',*,*,#10195,.F.);
#14420=ORIENTED_EDGE('',*,*,#10196,.T.);
#14421=ORIENTED_EDGE('',*,*,#10197,.T.);
#14422=ORIENTED_EDGE('',*,*,#10192,.F.);
#14423=ORIENTED_EDGE('',*,*,#10198,.F.);
#14424=ORIENTED_EDGE('',*,*,#10199,.T.);
#14425=ORIENTED_EDGE('',*,*,#10200,.T.);
#14426=ORIENTED_EDGE('',*,*,#10196,.F.);
#14427=ORIENTED_EDGE('',*,*,#10201,.F.);
#14428=ORIENTED_EDGE('',*,*,#10202,.T.);
#14429=ORIENTED_EDGE('',*,*,#10203,.T.);
#14430=ORIENTED_EDGE('',*,*,#10199,.F.);
#14431=ORIENTED_EDGE('',*,*,#10204,.F.);
#14432=ORIENTED_EDGE('',*,*,#10205,.T.);
#14433=ORIENTED_EDGE('',*,*,#10206,.T.);
#14434=ORIENTED_EDGE('',*,*,#10202,.F.);
#14435=ORIENTED_EDGE('',*,*,#10207,.F.);
#14436=ORIENTED_EDGE('',*,*,#10208,.T.);
#14437=ORIENTED_EDGE('',*,*,#10209,.T.);
#14438=ORIENTED_EDGE('',*,*,#10205,.F.);
#14439=ORIENTED_EDGE('',*,*,#10210,.F.);
#14440=ORIENTED_EDGE('',*,*,#10211,.T.);
#14441=ORIENTED_EDGE('',*,*,#10212,.T.);
#14442=ORIENTED_EDGE('',*,*,#10208,.F.);
#14443=ORIENTED_EDGE('',*,*,#10213,.F.);
#14444=ORIENTED_EDGE('',*,*,#10214,.F.);
#14445=ORIENTED_EDGE('',*,*,#10215,.F.);
#14446=ORIENTED_EDGE('',*,*,#10216,.F.);
#14447=ORIENTED_EDGE('',*,*,#10217,.T.);
#14448=ORIENTED_EDGE('',*,*,#10218,.T.);
#14449=ORIENTED_EDGE('',*,*,#10219,.T.);
#14450=ORIENTED_EDGE('',*,*,#10220,.T.);
#14451=ORIENTED_EDGE('',*,*,#10221,.T.);
#14452=ORIENTED_EDGE('',*,*,#10222,.T.);
#14453=ORIENTED_EDGE('',*,*,#10223,.T.);
#14454=ORIENTED_EDGE('',*,*,#10224,.T.);
#14455=ORIENTED_EDGE('',*,*,#10221,.F.);
#14456=ORIENTED_EDGE('',*,*,#10225,.T.);
#14457=ORIENTED_EDGE('',*,*,#10226,.T.);
#14458=ORIENTED_EDGE('',*,*,#10227,.T.);
#14459=ORIENTED_EDGE('',*,*,#10228,.T.);
#14460=ORIENTED_EDGE('',*,*,#10218,.F.);
#14461=ORIENTED_EDGE('',*,*,#10229,.T.);
#14462=ORIENTED_EDGE('',*,*,#10230,.T.);
#14463=ORIENTED_EDGE('',*,*,#10231,.T.);
#14464=ORIENTED_EDGE('',*,*,#10227,.F.);
#14465=ORIENTED_EDGE('',*,*,#10232,.T.);
#14466=ORIENTED_EDGE('',*,*,#10233,.T.);
#14467=ORIENTED_EDGE('',*,*,#10234,.T.);
#14468=ORIENTED_EDGE('',*,*,#10230,.F.);
#14469=ORIENTED_EDGE('',*,*,#10235,.T.);
#14470=ORIENTED_EDGE('',*,*,#10236,.T.);
#14471=ORIENTED_EDGE('',*,*,#10237,.T.);
#14472=ORIENTED_EDGE('',*,*,#10233,.F.);
#14473=ORIENTED_EDGE('',*,*,#10238,.T.);
#14474=ORIENTED_EDGE('',*,*,#10239,.T.);
#14475=ORIENTED_EDGE('',*,*,#10240,.T.);
#14476=ORIENTED_EDGE('',*,*,#10236,.F.);
#14477=ORIENTED_EDGE('',*,*,#10241,.T.);
#14478=ORIENTED_EDGE('',*,*,#10242,.T.);
#14479=ORIENTED_EDGE('',*,*,#10243,.T.);
#14480=ORIENTED_EDGE('',*,*,#10239,.F.);
#14481=ORIENTED_EDGE('',*,*,#10244,.T.);
#14482=ORIENTED_EDGE('',*,*,#10245,.F.);
#14483=ORIENTED_EDGE('',*,*,#10246,.T.);
#14484=ORIENTED_EDGE('',*,*,#10247,.F.);
#14485=ORIENTED_EDGE('',*,*,#10248,.T.);
#14486=ORIENTED_EDGE('',*,*,#10249,.T.);
#14487=ORIENTED_EDGE('',*,*,#10250,.T.);
#14488=ORIENTED_EDGE('',*,*,#10251,.F.);
#14489=ORIENTED_EDGE('',*,*,#10252,.F.);
#14490=ORIENTED_EDGE('',*,*,#10253,.T.);
#14491=ORIENTED_EDGE('',*,*,#10254,.T.);
#14492=ORIENTED_EDGE('',*,*,#10249,.F.);
#14493=ORIENTED_EDGE('',*,*,#10255,.F.);
#14494=ORIENTED_EDGE('',*,*,#10256,.T.);
#14495=ORIENTED_EDGE('',*,*,#10257,.T.);
#14496=ORIENTED_EDGE('',*,*,#10253,.F.);
#14497=ORIENTED_EDGE('',*,*,#10258,.F.);
#14498=ORIENTED_EDGE('',*,*,#10259,.T.);
#14499=ORIENTED_EDGE('',*,*,#10260,.T.);
#14500=ORIENTED_EDGE('',*,*,#10256,.F.);
#14501=ORIENTED_EDGE('',*,*,#10261,.F.);
#14502=ORIENTED_EDGE('',*,*,#10262,.T.);
#14503=ORIENTED_EDGE('',*,*,#10263,.T.);
#14504=ORIENTED_EDGE('',*,*,#10259,.F.);
#14505=ORIENTED_EDGE('',*,*,#10264,.F.);
#14506=ORIENTED_EDGE('',*,*,#10265,.T.);
#14507=ORIENTED_EDGE('',*,*,#10266,.T.);
#14508=ORIENTED_EDGE('',*,*,#10262,.F.);
#14509=ORIENTED_EDGE('',*,*,#10267,.F.);
#14510=ORIENTED_EDGE('',*,*,#10268,.T.);
#14511=ORIENTED_EDGE('',*,*,#10269,.T.);
#14512=ORIENTED_EDGE('',*,*,#10265,.F.);
#14513=ORIENTED_EDGE('',*,*,#10270,.F.);
#14514=ORIENTED_EDGE('',*,*,#10271,.F.);
#14515=ORIENTED_EDGE('',*,*,#10272,.F.);
#14516=ORIENTED_EDGE('',*,*,#10273,.F.);
#14517=ORIENTED_EDGE('',*,*,#10274,.T.);
#14518=ORIENTED_EDGE('',*,*,#10275,.F.);
#14519=ORIENTED_EDGE('',*,*,#10276,.F.);
#14520=ORIENTED_EDGE('',*,*,#10277,.T.);
#14521=ORIENTED_EDGE('',*,*,#10278,.F.);
#14522=ORIENTED_EDGE('',*,*,#10279,.F.);
#14523=ORIENTED_EDGE('',*,*,#10280,.T.);
#14524=ORIENTED_EDGE('',*,*,#10281,.F.);
#14525=ORIENTED_EDGE('',*,*,#10277,.F.);
#14526=ORIENTED_EDGE('',*,*,#10282,.F.);
#14527=ORIENTED_EDGE('',*,*,#10283,.F.);
#14528=ORIENTED_EDGE('',*,*,#10280,.F.);
#14529=ORIENTED_EDGE('',*,*,#10284,.F.);
#14530=ORIENTED_EDGE('',*,*,#10285,.F.);
#14531=ORIENTED_EDGE('',*,*,#10286,.F.);
#14532=ORIENTED_EDGE('',*,*,#10287,.F.);
#14533=ORIENTED_EDGE('',*,*,#10288,.F.);
#14534=ORIENTED_EDGE('',*,*,#10289,.F.);
#14535=ORIENTED_EDGE('',*,*,#10290,.T.);
#14536=ORIENTED_EDGE('',*,*,#10291,.T.);
#14537=ORIENTED_EDGE('',*,*,#10292,.T.);
#14538=ORIENTED_EDGE('',*,*,#10293,.T.);
#14539=ORIENTED_EDGE('',*,*,#10294,.F.);
#14540=ORIENTED_EDGE('',*,*,#10295,.F.);
#14541=ORIENTED_EDGE('',*,*,#10296,.F.);
#14542=ORIENTED_EDGE('',*,*,#10297,.F.);
#14543=ORIENTED_EDGE('',*,*,#10298,.F.);
#14544=ORIENTED_EDGE('',*,*,#10299,.T.);
#14545=ORIENTED_EDGE('',*,*,#10300,.T.);
#14546=ORIENTED_EDGE('',*,*,#10301,.T.);
#14547=ORIENTED_EDGE('',*,*,#10302,.T.);
#14548=ORIENTED_EDGE('',*,*,#10303,.F.);
#14549=ORIENTED_EDGE('',*,*,#10304,.F.);
#14550=ORIENTED_EDGE('',*,*,#10305,.F.);
#14551=ORIENTED_EDGE('',*,*,#10306,.F.);
#14552=ORIENTED_EDGE('',*,*,#10307,.F.);
#14553=ORIENTED_EDGE('',*,*,#10308,.T.);
#14554=ORIENTED_EDGE('',*,*,#10309,.T.);
#14555=ORIENTED_EDGE('',*,*,#10310,.T.);
#14556=ORIENTED_EDGE('',*,*,#10311,.T.);
#14557=ORIENTED_EDGE('',*,*,#10312,.F.);
#14558=ORIENTED_EDGE('',*,*,#10313,.F.);
#14559=ORIENTED_EDGE('',*,*,#10314,.F.);
#14560=ORIENTED_EDGE('',*,*,#10315,.F.);
#14561=ORIENTED_EDGE('',*,*,#10316,.F.);
#14562=ORIENTED_EDGE('',*,*,#10317,.T.);
#14563=ORIENTED_EDGE('',*,*,#10318,.T.);
#14564=ORIENTED_EDGE('',*,*,#10319,.T.);
#14565=ORIENTED_EDGE('',*,*,#10320,.T.);
#14566=ORIENTED_EDGE('',*,*,#10321,.F.);
#14567=ORIENTED_EDGE('',*,*,#10322,.F.);
#14568=ORIENTED_EDGE('',*,*,#10323,.F.);
#14569=ORIENTED_EDGE('',*,*,#10324,.F.);
#14570=ORIENTED_EDGE('',*,*,#10325,.F.);
#14571=ORIENTED_EDGE('',*,*,#10326,.T.);
#14572=ORIENTED_EDGE('',*,*,#10327,.T.);
#14573=ORIENTED_EDGE('',*,*,#10328,.T.);
#14574=ORIENTED_EDGE('',*,*,#10329,.T.);
#14575=ORIENTED_EDGE('',*,*,#10330,.F.);
#14576=ORIENTED_EDGE('',*,*,#10331,.F.);
#14577=ORIENTED_EDGE('',*,*,#10332,.F.);
#14578=ORIENTED_EDGE('',*,*,#10333,.F.);
#14579=ORIENTED_EDGE('',*,*,#10334,.F.);
#14580=ORIENTED_EDGE('',*,*,#10335,.T.);
#14581=ORIENTED_EDGE('',*,*,#10336,.T.);
#14582=ORIENTED_EDGE('',*,*,#10337,.T.);
#14583=ORIENTED_EDGE('',*,*,#10338,.T.);
#14584=ORIENTED_EDGE('',*,*,#10339,.T.);
#14585=ORIENTED_EDGE('',*,*,#9620,.T.);
#14586=ORIENTED_EDGE('',*,*,#10340,.T.);
#14587=ORIENTED_EDGE('',*,*,#9646,.T.);
#14588=ORIENTED_EDGE('',*,*,#10284,.T.);
#14589=ORIENTED_EDGE('',*,*,#10279,.T.);
#14590=ORIENTED_EDGE('',*,*,#10276,.T.);
#14591=ORIENTED_EDGE('',*,*,#10341,.F.);
#14592=ORIENTED_EDGE('',*,*,#10342,.T.);
#14593=ORIENTED_EDGE('',*,*,#9734,.T.);
#14594=ORIENTED_EDGE('',*,*,#10343,.T.);
#14595=ORIENTED_EDGE('',*,*,#9760,.T.);
#14596=ORIENTED_EDGE('',*,*,#10344,.T.);
#14597=ORIENTED_EDGE('',*,*,#9791,.T.);
#14598=ORIENTED_EDGE('',*,*,#10345,.T.);
#14599=ORIENTED_EDGE('',*,*,#9817,.T.);
#14600=ORIENTED_EDGE('',*,*,#10346,.T.);
#14601=ORIENTED_EDGE('',*,*,#9848,.T.);
#14602=ORIENTED_EDGE('',*,*,#10347,.T.);
#14603=ORIENTED_EDGE('',*,*,#9874,.T.);
#14604=ORIENTED_EDGE('',*,*,#10348,.T.);
#14605=ORIENTED_EDGE('',*,*,#9905,.T.);
#14606=ORIENTED_EDGE('',*,*,#10349,.T.);
#14607=ORIENTED_EDGE('',*,*,#9931,.T.);
#14608=ORIENTED_EDGE('',*,*,#10350,.T.);
#14609=ORIENTED_EDGE('',*,*,#9962,.T.);
#14610=ORIENTED_EDGE('',*,*,#10351,.T.);
#14611=ORIENTED_EDGE('',*,*,#9988,.T.);
#14612=ORIENTED_EDGE('',*,*,#10220,.F.);
#14613=ORIENTED_EDGE('',*,*,#10352,.T.);
#14614=ORIENTED_EDGE('',*,*,#10251,.T.);
#14615=ORIENTED_EDGE('',*,*,#10353,.T.);
#14616=ORIENTED_EDGE('',*,*,#10225,.F.);
#14617=ORIENTED_EDGE('',*,*,#10271,.T.);
#14618=ORIENTED_EDGE('',*,*,#10354,.T.);
#14619=ORIENTED_EDGE('',*,*,#10268,.F.);
#14620=ORIENTED_EDGE('',*,*,#10355,.F.);
#14621=ORIENTED_EDGE('',*,*,#10353,.F.);
#14622=ORIENTED_EDGE('',*,*,#10250,.F.);
#14623=ORIENTED_EDGE('',*,*,#10254,.F.);
#14624=ORIENTED_EDGE('',*,*,#10257,.F.);
#14625=ORIENTED_EDGE('',*,*,#10260,.F.);
#14626=ORIENTED_EDGE('',*,*,#10263,.F.);
#14627=ORIENTED_EDGE('',*,*,#10266,.F.);
#14628=ORIENTED_EDGE('',*,*,#10269,.F.);
#14629=ORIENTED_EDGE('',*,*,#10354,.F.);
#14630=ORIENTED_EDGE('',*,*,#10274,.F.);
#14631=ORIENTED_EDGE('',*,*,#10356,.F.);
#14632=ORIENTED_EDGE('',*,*,#10246,.F.);
#14633=ORIENTED_EDGE('',*,*,#10357,.F.);
#14634=ORIENTED_EDGE('',*,*,#10244,.F.);
#14635=ORIENTED_EDGE('',*,*,#10241,.F.);
#14636=ORIENTED_EDGE('',*,*,#10238,.F.);
#14637=ORIENTED_EDGE('',*,*,#10235,.F.);
#14638=ORIENTED_EDGE('',*,*,#10232,.F.);
#14639=ORIENTED_EDGE('',*,*,#10229,.F.);
#14640=ORIENTED_EDGE('',*,*,#10226,.F.);
#14641=ORIENTED_EDGE('',*,*,#10352,.F.);
#14642=ORIENTED_EDGE('',*,*,#10219,.F.);
#14643=ORIENTED_EDGE('',*,*,#10228,.F.);
#14644=ORIENTED_EDGE('',*,*,#10231,.F.);
#14645=ORIENTED_EDGE('',*,*,#10234,.F.);
#14646=ORIENTED_EDGE('',*,*,#10237,.F.);
#14647=ORIENTED_EDGE('',*,*,#10240,.F.);
#14648=ORIENTED_EDGE('',*,*,#10243,.F.);
#14649=ORIENTED_EDGE('',*,*,#10358,.F.);
#14650=ORIENTED_EDGE('',*,*,#10248,.F.);
#14651=ORIENTED_EDGE('',*,*,#10359,.F.);
#14652=ORIENTED_EDGE('',*,*,#10272,.T.);
#14653=ORIENTED_EDGE('',*,*,#10355,.T.);
#14654=ORIENTED_EDGE('',*,*,#10270,.T.);
#14655=ORIENTED_EDGE('',*,*,#10267,.T.);
#14656=ORIENTED_EDGE('',*,*,#10264,.T.);
#14657=ORIENTED_EDGE('',*,*,#10261,.T.);
#14658=ORIENTED_EDGE('',*,*,#10258,.T.);
#14659=ORIENTED_EDGE('',*,*,#10255,.T.);
#14660=ORIENTED_EDGE('',*,*,#10252,.T.);
#14661=ORIENTED_EDGE('',*,*,#10245,.T.);
#14662=ORIENTED_EDGE('',*,*,#10358,.T.);
#14663=ORIENTED_EDGE('',*,*,#10242,.F.);
#14664=ORIENTED_EDGE('',*,*,#10357,.T.);
#14665=ORIENTED_EDGE('',*,*,#10163,.F.);
#14666=ORIENTED_EDGE('',*,*,#10360,.T.);
#14667=ORIENTED_EDGE('',*,*,#10194,.T.);
#14668=ORIENTED_EDGE('',*,*,#10361,.T.);
#14669=ORIENTED_EDGE('',*,*,#10168,.F.);
#14670=ORIENTED_EDGE('',*,*,#10214,.T.);
#14671=ORIENTED_EDGE('',*,*,#10362,.T.);
#14672=ORIENTED_EDGE('',*,*,#10211,.F.);
#14673=ORIENTED_EDGE('',*,*,#10363,.F.);
#14674=ORIENTED_EDGE('',*,*,#10361,.F.);
#14675=ORIENTED_EDGE('',*,*,#10193,.F.);
#14676=ORIENTED_EDGE('',*,*,#10197,.F.);
#14677=ORIENTED_EDGE('',*,*,#10200,.F.);
#14678=ORIENTED_EDGE('',*,*,#10203,.F.);
#14679=ORIENTED_EDGE('',*,*,#10206,.F.);
#14680=ORIENTED_EDGE('',*,*,#10209,.F.);
#14681=ORIENTED_EDGE('',*,*,#10212,.F.);
#14682=ORIENTED_EDGE('',*,*,#10362,.F.);
#14683=ORIENTED_EDGE('',*,*,#10217,.F.);
#14684=ORIENTED_EDGE('',*,*,#10364,.F.);
#14685=ORIENTED_EDGE('',*,*,#10189,.F.);
#14686=ORIENTED_EDGE('',*,*,#10365,.F.);
#14687=ORIENTED_EDGE('',*,*,#10187,.F.);
#14688=ORIENTED_EDGE('',*,*,#10184,.F.);
#14689=ORIENTED_EDGE('',*,*,#10181,.F.);
#14690=ORIENTED_EDGE('',*,*,#10178,.F.);
#14691=ORIENTED_EDGE('',*,*,#10175,.F.);
#14692=ORIENTED_EDGE('',*,*,#10172,.F.);
#14693=ORIENTED_EDGE('',*,*,#10169,.F.);
#14694=ORIENTED_EDGE('',*,*,#10360,.F.);
#14695=ORIENTED_EDGE('',*,*,#10162,.F.);
#14696=ORIENTED_EDGE('',*,*,#10171,.F.);
#14697=ORIENTED_EDGE('',*,*,#10174,.F.);
#14698=ORIENTED_EDGE('',*,*,#10177,.F.);
#14699=ORIENTED_EDGE('',*,*,#10180,.F.);
#14700=ORIENTED_EDGE('',*,*,#10183,.F.);
#14701=ORIENTED_EDGE('',*,*,#10186,.F.);
#14702=ORIENTED_EDGE('',*,*,#10366,.F.);
#14703=ORIENTED_EDGE('',*,*,#10191,.F.);
#14704=ORIENTED_EDGE('',*,*,#10367,.F.);
#14705=ORIENTED_EDGE('',*,*,#10215,.T.);
#14706=ORIENTED_EDGE('',*,*,#10363,.T.);
#14707=ORIENTED_EDGE('',*,*,#10213,.T.);
#14708=ORIENTED_EDGE('',*,*,#10210,.T.);
#14709=ORIENTED_EDGE('',*,*,#10207,.T.);
#14710=ORIENTED_EDGE('',*,*,#10204,.T.);
#14711=ORIENTED_EDGE('',*,*,#10201,.T.);
#14712=ORIENTED_EDGE('',*,*,#10198,.T.);
#14713=ORIENTED_EDGE('',*,*,#10195,.T.);
#14714=ORIENTED_EDGE('',*,*,#10188,.T.);
#14715=ORIENTED_EDGE('',*,*,#10366,.T.);
#14716=ORIENTED_EDGE('',*,*,#10185,.F.);
#14717=ORIENTED_EDGE('',*,*,#10365,.T.);
#14718=ORIENTED_EDGE('',*,*,#10106,.F.);
#14719=ORIENTED_EDGE('',*,*,#10368,.T.);
#14720=ORIENTED_EDGE('',*,*,#10137,.T.);
#14721=ORIENTED_EDGE('',*,*,#10369,.T.);
#14722=ORIENTED_EDGE('',*,*,#10111,.F.);
#14723=ORIENTED_EDGE('',*,*,#10157,.T.);
#14724=ORIENTED_EDGE('',*,*,#10370,.T.);
#14725=ORIENTED_EDGE('',*,*,#10154,.F.);
#14726=ORIENTED_EDGE('',*,*,#10371,.F.);
#14727=ORIENTED_EDGE('',*,*,#10369,.F.);
#14728=ORIENTED_EDGE('',*,*,#10136,.F.);
#14729=ORIENTED_EDGE('',*,*,#10140,.F.);
#14730=ORIENTED_EDGE('',*,*,#10143,.F.);
#14731=ORIENTED_EDGE('',*,*,#10146,.F.);
#14732=ORIENTED_EDGE('',*,*,#10149,.F.);
#14733=ORIENTED_EDGE('',*,*,#10152,.F.);
#14734=ORIENTED_EDGE('',*,*,#10155,.F.);
#14735=ORIENTED_EDGE('',*,*,#10370,.F.);
#14736=ORIENTED_EDGE('',*,*,#10160,.F.);
#14737=ORIENTED_EDGE('',*,*,#10372,.F.);
#14738=ORIENTED_EDGE('',*,*,#10132,.F.);
#14739=ORIENTED_EDGE('',*,*,#10373,.F.);
#14740=ORIENTED_EDGE('',*,*,#10130,.F.);
#14741=ORIENTED_EDGE('',*,*,#10127,.F.);
#14742=ORIENTED_EDGE('',*,*,#10124,.F.);
#14743=ORIENTED_EDGE('',*,*,#10121,.F.);
#14744=ORIENTED_EDGE('',*,*,#10118,.F.);
#14745=ORIENTED_EDGE('',*,*,#10115,.F.);
#14746=ORIENTED_EDGE('',*,*,#10112,.F.);
#14747=ORIENTED_EDGE('',*,*,#10368,.F.);
#14748=ORIENTED_EDGE('',*,*,#10105,.F.);
#14749=ORIENTED_EDGE('',*,*,#10114,.F.);
#14750=ORIENTED_EDGE('',*,*,#10117,.F.);
#14751=ORIENTED_EDGE('',*,*,#10120,.F.);
#14752=ORIENTED_EDGE('',*,*,#10123,.F.);
#14753=ORIENTED_EDGE('',*,*,#10126,.F.);
#14754=ORIENTED_EDGE('',*,*,#10129,.F.);
#14755=ORIENTED_EDGE('',*,*,#10374,.F.);
#14756=ORIENTED_EDGE('',*,*,#10134,.F.);
#14757=ORIENTED_EDGE('',*,*,#10375,.F.);
#14758=ORIENTED_EDGE('',*,*,#10158,.T.);
#14759=ORIENTED_EDGE('',*,*,#10371,.T.);
#14760=ORIENTED_EDGE('',*,*,#10156,.T.);
#14761=ORIENTED_EDGE('',*,*,#10153,.T.);
#14762=ORIENTED_EDGE('',*,*,#10150,.T.);
#14763=ORIENTED_EDGE('',*,*,#10147,.T.);
#14764=ORIENTED_EDGE('',*,*,#10144,.T.);
#14765=ORIENTED_EDGE('',*,*,#10141,.T.);
#14766=ORIENTED_EDGE('',*,*,#10138,.T.);
#14767=ORIENTED_EDGE('',*,*,#10131,.T.);
#14768=ORIENTED_EDGE('',*,*,#10374,.T.);
#14769=ORIENTED_EDGE('',*,*,#10128,.F.);
#14770=ORIENTED_EDGE('',*,*,#10373,.T.);
#14771=ORIENTED_EDGE('',*,*,#10049,.F.);
#14772=ORIENTED_EDGE('',*,*,#10376,.T.);
#14773=ORIENTED_EDGE('',*,*,#10080,.T.);
#14774=ORIENTED_EDGE('',*,*,#10377,.T.);
#14775=ORIENTED_EDGE('',*,*,#10054,.F.);
#14776=ORIENTED_EDGE('',*,*,#10100,.T.);
#14777=ORIENTED_EDGE('',*,*,#10378,.T.);
#14778=ORIENTED_EDGE('',*,*,#10097,.F.);
#14779=ORIENTED_EDGE('',*,*,#10379,.F.);
#14780=ORIENTED_EDGE('',*,*,#10377,.F.);
#14781=ORIENTED_EDGE('',*,*,#10079,.F.);
#14782=ORIENTED_EDGE('',*,*,#10083,.F.);
#14783=ORIENTED_EDGE('',*,*,#10086,.F.);
#14784=ORIENTED_EDGE('',*,*,#10089,.F.);
#14785=ORIENTED_EDGE('',*,*,#10092,.F.);
#14786=ORIENTED_EDGE('',*,*,#10095,.F.);
#14787=ORIENTED_EDGE('',*,*,#10098,.F.);
#14788=ORIENTED_EDGE('',*,*,#10378,.F.);
#14789=ORIENTED_EDGE('',*,*,#10103,.F.);
#14790=ORIENTED_EDGE('',*,*,#10380,.F.);
#14791=ORIENTED_EDGE('',*,*,#10075,.F.);
#14792=ORIENTED_EDGE('',*,*,#10381,.F.);
#14793=ORIENTED_EDGE('',*,*,#10073,.F.);
#14794=ORIENTED_EDGE('',*,*,#10070,.F.);
#14795=ORIENTED_EDGE('',*,*,#10067,.F.);
#14796=ORIENTED_EDGE('',*,*,#10064,.F.);
#14797=ORIENTED_EDGE('',*,*,#10061,.F.);
#14798=ORIENTED_EDGE('',*,*,#10058,.F.);
#14799=ORIENTED_EDGE('',*,*,#10055,.F.);
#14800=ORIENTED_EDGE('',*,*,#10376,.F.);
#14801=ORIENTED_EDGE('',*,*,#10048,.F.);
#14802=ORIENTED_EDGE('',*,*,#10057,.F.);
#14803=ORIENTED_EDGE('',*,*,#10060,.F.);
#14804=ORIENTED_EDGE('',*,*,#10063,.F.);
#14805=ORIENTED_EDGE('',*,*,#10066,.F.);
#14806=ORIENTED_EDGE('',*,*,#10069,.F.);
#14807=ORIENTED_EDGE('',*,*,#10072,.F.);
#14808=ORIENTED_EDGE('',*,*,#10382,.F.);
#14809=ORIENTED_EDGE('',*,*,#10077,.F.);
#14810=ORIENTED_EDGE('',*,*,#10383,.F.);
#14811=ORIENTED_EDGE('',*,*,#10101,.T.);
#14812=ORIENTED_EDGE('',*,*,#10379,.T.);
#14813=ORIENTED_EDGE('',*,*,#10099,.T.);
#14814=ORIENTED_EDGE('',*,*,#10096,.T.);
#14815=ORIENTED_EDGE('',*,*,#10093,.T.);
#14816=ORIENTED_EDGE('',*,*,#10090,.T.);
#14817=ORIENTED_EDGE('',*,*,#10087,.T.);
#14818=ORIENTED_EDGE('',*,*,#10084,.T.);
#14819=ORIENTED_EDGE('',*,*,#10081,.T.);
#14820=ORIENTED_EDGE('',*,*,#10074,.T.);
#14821=ORIENTED_EDGE('',*,*,#10382,.T.);
#14822=ORIENTED_EDGE('',*,*,#10071,.F.);
#14823=ORIENTED_EDGE('',*,*,#10381,.T.);
#14824=ORIENTED_EDGE('',*,*,#9992,.F.);
#14825=ORIENTED_EDGE('',*,*,#10384,.T.);
#14826=ORIENTED_EDGE('',*,*,#10023,.T.);
#14827=ORIENTED_EDGE('',*,*,#10385,.T.);
#14828=ORIENTED_EDGE('',*,*,#9997,.F.);
#14829=ORIENTED_EDGE('',*,*,#10043,.T.);
#14830=ORIENTED_EDGE('',*,*,#10386,.T.);
#14831=ORIENTED_EDGE('',*,*,#10040,.F.);
#14832=ORIENTED_EDGE('',*,*,#10387,.F.);
#14833=ORIENTED_EDGE('',*,*,#10385,.F.);
#14834=ORIENTED_EDGE('',*,*,#10022,.F.);
#14835=ORIENTED_EDGE('',*,*,#10026,.F.);
#14836=ORIENTED_EDGE('',*,*,#10029,.F.);
#14837=ORIENTED_EDGE('',*,*,#10032,.F.);
#14838=ORIENTED_EDGE('',*,*,#10035,.F.);
#14839=ORIENTED_EDGE('',*,*,#10038,.F.);
#14840=ORIENTED_EDGE('',*,*,#10041,.F.);
#14841=ORIENTED_EDGE('',*,*,#10386,.F.);
#14842=ORIENTED_EDGE('',*,*,#10046,.F.);
#14843=ORIENTED_EDGE('',*,*,#10388,.F.);
#14844=ORIENTED_EDGE('',*,*,#10018,.F.);
#14845=ORIENTED_EDGE('',*,*,#10389,.F.);
#14846=ORIENTED_EDGE('',*,*,#10016,.F.);
#14847=ORIENTED_EDGE('',*,*,#10013,.F.);
#14848=ORIENTED_EDGE('',*,*,#10010,.F.);
#14849=ORIENTED_EDGE('',*,*,#10007,.F.);
#14850=ORIENTED_EDGE('',*,*,#10004,.F.);
#14851=ORIENTED_EDGE('',*,*,#10001,.F.);
#14852=ORIENTED_EDGE('',*,*,#9998,.F.);
#14853=ORIENTED_EDGE('',*,*,#10384,.F.);
#14854=ORIENTED_EDGE('',*,*,#9991,.F.);
#14855=ORIENTED_EDGE('',*,*,#10000,.F.);
#14856=ORIENTED_EDGE('',*,*,#10003,.F.);
#14857=ORIENTED_EDGE('',*,*,#10006,.F.);
#14858=ORIENTED_EDGE('',*,*,#10009,.F.);
#14859=ORIENTED_EDGE('',*,*,#10012,.F.);
#14860=ORIENTED_EDGE('',*,*,#10015,.F.);
#14861=ORIENTED_EDGE('',*,*,#10390,.F.);
#14862=ORIENTED_EDGE('',*,*,#10020,.F.);
#14863=ORIENTED_EDGE('',*,*,#10391,.F.);
#14864=ORIENTED_EDGE('',*,*,#10044,.T.);
#14865=ORIENTED_EDGE('',*,*,#10387,.T.);
#14866=ORIENTED_EDGE('',*,*,#10042,.T.);
#14867=ORIENTED_EDGE('',*,*,#10039,.T.);
#14868=ORIENTED_EDGE('',*,*,#10036,.T.);
#14869=ORIENTED_EDGE('',*,*,#10033,.T.);
#14870=ORIENTED_EDGE('',*,*,#10030,.T.);
#14871=ORIENTED_EDGE('',*,*,#10027,.T.);
#14872=ORIENTED_EDGE('',*,*,#10024,.T.);
#14873=ORIENTED_EDGE('',*,*,#10017,.T.);
#14874=ORIENTED_EDGE('',*,*,#10390,.T.);
#14875=ORIENTED_EDGE('',*,*,#10014,.F.);
#14876=ORIENTED_EDGE('',*,*,#10389,.T.);
#14877=ORIENTED_EDGE('',*,*,#10392,.T.);
#14878=ORIENTED_EDGE('',*,*,#10222,.F.);
#14879=ORIENTED_EDGE('',*,*,#10224,.F.);
#14880=ORIENTED_EDGE('',*,*,#10393,.F.);
#14881=ORIENTED_EDGE('',*,*,#10223,.F.);
#14882=ORIENTED_EDGE('',*,*,#10394,.T.);
#14883=ORIENTED_EDGE('',*,*,#10165,.F.);
#14884=ORIENTED_EDGE('',*,*,#10167,.F.);
#14885=ORIENTED_EDGE('',*,*,#10395,.F.);
#14886=ORIENTED_EDGE('',*,*,#10166,.F.);
#14887=ORIENTED_EDGE('',*,*,#10396,.T.);
#14888=ORIENTED_EDGE('',*,*,#10108,.F.);
#14889=ORIENTED_EDGE('',*,*,#10110,.F.);
#14890=ORIENTED_EDGE('',*,*,#10397,.F.);
#14891=ORIENTED_EDGE('',*,*,#10109,.F.);
#14892=ORIENTED_EDGE('',*,*,#10398,.T.);
#14893=ORIENTED_EDGE('',*,*,#10051,.F.);
#14894=ORIENTED_EDGE('',*,*,#10053,.F.);
#14895=ORIENTED_EDGE('',*,*,#10399,.F.);
#14896=ORIENTED_EDGE('',*,*,#10052,.F.);
#14897=ORIENTED_EDGE('',*,*,#10400,.T.);
#14898=ORIENTED_EDGE('',*,*,#9994,.F.);
#14899=ORIENTED_EDGE('',*,*,#9996,.F.);
#14900=ORIENTED_EDGE('',*,*,#10401,.F.);
#14901=ORIENTED_EDGE('',*,*,#9995,.F.);
#14902=ORIENTED_EDGE('',*,*,#9935,.F.);
#14903=ORIENTED_EDGE('',*,*,#10402,.T.);
#14904=ORIENTED_EDGE('',*,*,#9966,.T.);
#14905=ORIENTED_EDGE('',*,*,#10403,.T.);
#14906=ORIENTED_EDGE('',*,*,#9940,.F.);
#14907=ORIENTED_EDGE('',*,*,#9986,.T.);
#14908=ORIENTED_EDGE('',*,*,#10404,.T.);
#14909=ORIENTED_EDGE('',*,*,#9983,.F.);
#14910=ORIENTED_EDGE('',*,*,#10405,.F.);
#14911=ORIENTED_EDGE('',*,*,#10403,.F.);
#14912=ORIENTED_EDGE('',*,*,#9965,.F.);
#14913=ORIENTED_EDGE('',*,*,#9969,.F.);
#14914=ORIENTED_EDGE('',*,*,#9972,.F.);
#14915=ORIENTED_EDGE('',*,*,#9975,.F.);
#14916=ORIENTED_EDGE('',*,*,#9978,.F.);
#14917=ORIENTED_EDGE('',*,*,#9981,.F.);
#14918=ORIENTED_EDGE('',*,*,#9984,.F.);
#14919=ORIENTED_EDGE('',*,*,#10404,.F.);
#14920=ORIENTED_EDGE('',*,*,#9989,.F.);
#14921=ORIENTED_EDGE('',*,*,#10351,.F.);
#14922=ORIENTED_EDGE('',*,*,#9961,.F.);
#14923=ORIENTED_EDGE('',*,*,#10406,.F.);
#14924=ORIENTED_EDGE('',*,*,#9959,.F.);
#14925=ORIENTED_EDGE('',*,*,#9956,.F.);
#14926=ORIENTED_EDGE('',*,*,#9953,.F.);
#14927=ORIENTED_EDGE('',*,*,#9950,.F.);
#14928=ORIENTED_EDGE('',*,*,#9947,.F.);
#14929=ORIENTED_EDGE('',*,*,#9944,.F.);
#14930=ORIENTED_EDGE('',*,*,#9941,.F.);
#14931=ORIENTED_EDGE('',*,*,#10402,.F.);
#14932=ORIENTED_EDGE('',*,*,#9934,.F.);
#14933=ORIENTED_EDGE('',*,*,#9943,.F.);
#14934=ORIENTED_EDGE('',*,*,#9946,.F.);
#14935=ORIENTED_EDGE('',*,*,#9949,.F.);
#14936=ORIENTED_EDGE('',*,*,#9952,.F.);
#14937=ORIENTED_EDGE('',*,*,#9955,.F.);
#14938=ORIENTED_EDGE('',*,*,#9958,.F.);
#14939=ORIENTED_EDGE('',*,*,#10407,.F.);
#14940=ORIENTED_EDGE('',*,*,#9963,.F.);
#14941=ORIENTED_EDGE('',*,*,#10350,.F.);
#14942=ORIENTED_EDGE('',*,*,#9987,.T.);
#14943=ORIENTED_EDGE('',*,*,#10405,.T.);
#14944=ORIENTED_EDGE('',*,*,#9985,.T.);
#14945=ORIENTED_EDGE('',*,*,#9982,.T.);
#14946=ORIENTED_EDGE('',*,*,#9979,.T.);
#14947=ORIENTED_EDGE('',*,*,#9976,.T.);
#14948=ORIENTED_EDGE('',*,*,#9973,.T.);
#14949=ORIENTED_EDGE('',*,*,#9970,.T.);
#14950=ORIENTED_EDGE('',*,*,#9967,.T.);
#14951=ORIENTED_EDGE('',*,*,#9960,.T.);
#14952=ORIENTED_EDGE('',*,*,#10407,.T.);
#14953=ORIENTED_EDGE('',*,*,#9957,.F.);
#14954=ORIENTED_EDGE('',*,*,#10406,.T.);
#14955=ORIENTED_EDGE('',*,*,#9878,.F.);
#14956=ORIENTED_EDGE('',*,*,#10408,.T.);
#14957=ORIENTED_EDGE('',*,*,#9909,.T.);
#14958=ORIENTED_EDGE('',*,*,#10409,.T.);
#14959=ORIENTED_EDGE('',*,*,#9883,.F.);
#14960=ORIENTED_EDGE('',*,*,#9929,.T.);
#14961=ORIENTED_EDGE('',*,*,#10410,.T.);
#14962=ORIENTED_EDGE('',*,*,#9926,.F.);
#14963=ORIENTED_EDGE('',*,*,#10411,.F.);
#14964=ORIENTED_EDGE('',*,*,#10409,.F.);
#14965=ORIENTED_EDGE('',*,*,#9908,.F.);
#14966=ORIENTED_EDGE('',*,*,#9912,.F.);
#14967=ORIENTED_EDGE('',*,*,#9915,.F.);
#14968=ORIENTED_EDGE('',*,*,#9918,.F.);
#14969=ORIENTED_EDGE('',*,*,#9921,.F.);
#14970=ORIENTED_EDGE('',*,*,#9924,.F.);
#14971=ORIENTED_EDGE('',*,*,#9927,.F.);
#14972=ORIENTED_EDGE('',*,*,#10410,.F.);
#14973=ORIENTED_EDGE('',*,*,#9932,.F.);
#14974=ORIENTED_EDGE('',*,*,#10349,.F.);
#14975=ORIENTED_EDGE('',*,*,#9904,.F.);
#14976=ORIENTED_EDGE('',*,*,#10412,.F.);
#14977=ORIENTED_EDGE('',*,*,#9902,.F.);
#14978=ORIENTED_EDGE('',*,*,#9899,.F.);
#14979=ORIENTED_EDGE('',*,*,#9896,.F.);
#14980=ORIENTED_EDGE('',*,*,#9893,.F.);
#14981=ORIENTED_EDGE('',*,*,#9890,.F.);
#14982=ORIENTED_EDGE('',*,*,#9887,.F.);
#14983=ORIENTED_EDGE('',*,*,#9884,.F.);
#14984=ORIENTED_EDGE('',*,*,#10408,.F.);
#14985=ORIENTED_EDGE('',*,*,#9877,.F.);
#14986=ORIENTED_EDGE('',*,*,#9886,.F.);
#14987=ORIENTED_EDGE('',*,*,#9889,.F.);
#14988=ORIENTED_EDGE('',*,*,#9892,.F.);
#14989=ORIENTED_EDGE('',*,*,#9895,.F.);
#14990=ORIENTED_EDGE('',*,*,#9898,.F.);
#14991=ORIENTED_EDGE('',*,*,#9901,.F.);
#14992=ORIENTED_EDGE('',*,*,#10413,.F.);
#14993=ORIENTED_EDGE('',*,*,#9906,.F.);
#14994=ORIENTED_EDGE('',*,*,#10348,.F.);
#14995=ORIENTED_EDGE('',*,*,#9930,.T.);
#14996=ORIENTED_EDGE('',*,*,#10411,.T.);
#14997=ORIENTED_EDGE('',*,*,#9928,.T.);
#14998=ORIENTED_EDGE('',*,*,#9925,.T.);
#14999=ORIENTED_EDGE('',*,*,#9922,.T.);
#15000=ORIENTED_EDGE('',*,*,#9919,.T.);
#15001=ORIENTED_EDGE('',*,*,#9916,.T.);
#15002=ORIENTED_EDGE('',*,*,#9913,.T.);
#15003=ORIENTED_EDGE('',*,*,#9910,.T.);
#15004=ORIENTED_EDGE('',*,*,#9903,.T.);
#15005=ORIENTED_EDGE('',*,*,#10413,.T.);
#15006=ORIENTED_EDGE('',*,*,#9900,.F.);
#15007=ORIENTED_EDGE('',*,*,#10412,.T.);
#15008=ORIENTED_EDGE('',*,*,#9821,.F.);
#15009=ORIENTED_EDGE('',*,*,#10414,.T.);
#15010=ORIENTED_EDGE('',*,*,#9852,.T.);
#15011=ORIENTED_EDGE('',*,*,#10415,.T.);
#15012=ORIENTED_EDGE('',*,*,#9826,.F.);
#15013=ORIENTED_EDGE('',*,*,#9872,.T.);
#15014=ORIENTED_EDGE('',*,*,#10416,.T.);
#15015=ORIENTED_EDGE('',*,*,#9869,.F.);
#15016=ORIENTED_EDGE('',*,*,#10417,.F.);
#15017=ORIENTED_EDGE('',*,*,#10415,.F.);
#15018=ORIENTED_EDGE('',*,*,#9851,.F.);
#15019=ORIENTED_EDGE('',*,*,#9855,.F.);
#15020=ORIENTED_EDGE('',*,*,#9858,.F.);
#15021=ORIENTED_EDGE('',*,*,#9861,.F.);
#15022=ORIENTED_EDGE('',*,*,#9864,.F.);
#15023=ORIENTED_EDGE('',*,*,#9867,.F.);
#15024=ORIENTED_EDGE('',*,*,#9870,.F.);
#15025=ORIENTED_EDGE('',*,*,#10416,.F.);
#15026=ORIENTED_EDGE('',*,*,#9875,.F.);
#15027=ORIENTED_EDGE('',*,*,#10347,.F.);
#15028=ORIENTED_EDGE('',*,*,#9847,.F.);
#15029=ORIENTED_EDGE('',*,*,#10418,.F.);
#15030=ORIENTED_EDGE('',*,*,#9845,.F.);
#15031=ORIENTED_EDGE('',*,*,#9842,.F.);
#15032=ORIENTED_EDGE('',*,*,#9839,.F.);
#15033=ORIENTED_EDGE('',*,*,#9836,.F.);
#15034=ORIENTED_EDGE('',*,*,#9833,.F.);
#15035=ORIENTED_EDGE('',*,*,#9830,.F.);
#15036=ORIENTED_EDGE('',*,*,#9827,.F.);
#15037=ORIENTED_EDGE('',*,*,#10414,.F.);
#15038=ORIENTED_EDGE('',*,*,#9820,.F.);
#15039=ORIENTED_EDGE('',*,*,#9829,.F.);
#15040=ORIENTED_EDGE('',*,*,#9832,.F.);
#15041=ORIENTED_EDGE('',*,*,#9835,.F.);
#15042=ORIENTED_EDGE('',*,*,#9838,.F.);
#15043=ORIENTED_EDGE('',*,*,#9841,.F.);
#15044=ORIENTED_EDGE('',*,*,#9844,.F.);
#15045=ORIENTED_EDGE('',*,*,#10419,.F.);
#15046=ORIENTED_EDGE('',*,*,#9849,.F.);
#15047=ORIENTED_EDGE('',*,*,#10346,.F.);
#15048=ORIENTED_EDGE('',*,*,#9873,.T.);
#15049=ORIENTED_EDGE('',*,*,#10417,.T.);
#15050=ORIENTED_EDGE('',*,*,#9871,.T.);
#15051=ORIENTED_EDGE('',*,*,#9868,.T.);
#15052=ORIENTED_EDGE('',*,*,#9865,.T.);
#15053=ORIENTED_EDGE('',*,*,#9862,.T.);
#15054=ORIENTED_EDGE('',*,*,#9859,.T.);
#15055=ORIENTED_EDGE('',*,*,#9856,.T.);
#15056=ORIENTED_EDGE('',*,*,#9853,.T.);
#15057=ORIENTED_EDGE('',*,*,#9846,.T.);
#15058=ORIENTED_EDGE('',*,*,#10419,.T.);
#15059=ORIENTED_EDGE('',*,*,#9843,.F.);
#15060=ORIENTED_EDGE('',*,*,#10418,.T.);
#15061=ORIENTED_EDGE('',*,*,#9764,.F.);
#15062=ORIENTED_EDGE('',*,*,#10420,.T.);
#15063=ORIENTED_EDGE('',*,*,#9795,.T.);
#15064=ORIENTED_EDGE('',*,*,#10421,.T.);
#15065=ORIENTED_EDGE('',*,*,#9769,.F.);
#15066=ORIENTED_EDGE('',*,*,#9815,.T.);
#15067=ORIENTED_EDGE('',*,*,#10422,.T.);
#15068=ORIENTED_EDGE('',*,*,#9812,.F.);
#15069=ORIENTED_EDGE('',*,*,#10423,.F.);
#15070=ORIENTED_EDGE('',*,*,#10421,.F.);
#15071=ORIENTED_EDGE('',*,*,#9794,.F.);
#15072=ORIENTED_EDGE('',*,*,#9798,.F.);
#15073=ORIENTED_EDGE('',*,*,#9801,.F.);
#15074=ORIENTED_EDGE('',*,*,#9804,.F.);
#15075=ORIENTED_EDGE('',*,*,#9807,.F.);
#15076=ORIENTED_EDGE('',*,*,#9810,.F.);
#15077=ORIENTED_EDGE('',*,*,#9813,.F.);
#15078=ORIENTED_EDGE('',*,*,#10422,.F.);
#15079=ORIENTED_EDGE('',*,*,#9818,.F.);
#15080=ORIENTED_EDGE('',*,*,#10345,.F.);
#15081=ORIENTED_EDGE('',*,*,#9790,.F.);
#15082=ORIENTED_EDGE('',*,*,#10424,.F.);
#15083=ORIENTED_EDGE('',*,*,#9788,.F.);
#15084=ORIENTED_EDGE('',*,*,#9785,.F.);
#15085=ORIENTED_EDGE('',*,*,#9782,.F.);
#15086=ORIENTED_EDGE('',*,*,#9779,.F.);
#15087=ORIENTED_EDGE('',*,*,#9776,.F.);
#15088=ORIENTED_EDGE('',*,*,#9773,.F.);
#15089=ORIENTED_EDGE('',*,*,#9770,.F.);
#15090=ORIENTED_EDGE('',*,*,#10420,.F.);
#15091=ORIENTED_EDGE('',*,*,#9763,.F.);
#15092=ORIENTED_EDGE('',*,*,#9772,.F.);
#15093=ORIENTED_EDGE('',*,*,#9775,.F.);
#15094=ORIENTED_EDGE('',*,*,#9778,.F.);
#15095=ORIENTED_EDGE('',*,*,#9781,.F.);
#15096=ORIENTED_EDGE('',*,*,#9784,.F.);
#15097=ORIENTED_EDGE('',*,*,#9787,.F.);
#15098=ORIENTED_EDGE('',*,*,#10425,.F.);
#15099=ORIENTED_EDGE('',*,*,#9792,.F.);
#15100=ORIENTED_EDGE('',*,*,#10344,.F.);
#15101=ORIENTED_EDGE('',*,*,#9816,.T.);
#15102=ORIENTED_EDGE('',*,*,#10423,.T.);
#15103=ORIENTED_EDGE('',*,*,#9814,.T.);
#15104=ORIENTED_EDGE('',*,*,#9811,.T.);
#15105=ORIENTED_EDGE('',*,*,#9808,.T.);
#15106=ORIENTED_EDGE('',*,*,#9805,.T.);
#15107=ORIENTED_EDGE('',*,*,#9802,.T.);
#15108=ORIENTED_EDGE('',*,*,#9799,.T.);
#15109=ORIENTED_EDGE('',*,*,#9796,.T.);
#15110=ORIENTED_EDGE('',*,*,#9789,.T.);
#15111=ORIENTED_EDGE('',*,*,#10425,.T.);
#15112=ORIENTED_EDGE('',*,*,#9786,.F.);
#15113=ORIENTED_EDGE('',*,*,#10424,.T.);
#15114=ORIENTED_EDGE('',*,*,#9707,.F.);
#15115=ORIENTED_EDGE('',*,*,#10426,.T.);
#15116=ORIENTED_EDGE('',*,*,#9738,.T.);
#15117=ORIENTED_EDGE('',*,*,#10427,.T.);
#15118=ORIENTED_EDGE('',*,*,#9712,.F.);
#15119=ORIENTED_EDGE('',*,*,#9758,.T.);
#15120=ORIENTED_EDGE('',*,*,#10428,.T.);
#15121=ORIENTED_EDGE('',*,*,#9755,.F.);
#15122=ORIENTED_EDGE('',*,*,#10429,.F.);
#15123=ORIENTED_EDGE('',*,*,#10427,.F.);
#15124=ORIENTED_EDGE('',*,*,#9737,.F.);
#15125=ORIENTED_EDGE('',*,*,#9741,.F.);
#15126=ORIENTED_EDGE('',*,*,#9744,.F.);
#15127=ORIENTED_EDGE('',*,*,#9747,.F.);
#15128=ORIENTED_EDGE('',*,*,#9750,.F.);
#15129=ORIENTED_EDGE('',*,*,#9753,.F.);
#15130=ORIENTED_EDGE('',*,*,#9756,.F.);
#15131=ORIENTED_EDGE('',*,*,#10428,.F.);
#15132=ORIENTED_EDGE('',*,*,#9761,.F.);
#15133=ORIENTED_EDGE('',*,*,#10343,.F.);
#15134=ORIENTED_EDGE('',*,*,#9733,.F.);
#15135=ORIENTED_EDGE('',*,*,#10430,.F.);
#15136=ORIENTED_EDGE('',*,*,#9731,.F.);
#15137=ORIENTED_EDGE('',*,*,#9728,.F.);
#15138=ORIENTED_EDGE('',*,*,#9725,.F.);
#15139=ORIENTED_EDGE('',*,*,#9722,.F.);
#15140=ORIENTED_EDGE('',*,*,#9719,.F.);
#15141=ORIENTED_EDGE('',*,*,#9716,.F.);
#15142=ORIENTED_EDGE('',*,*,#9713,.F.);
#15143=ORIENTED_EDGE('',*,*,#10426,.F.);
#15144=ORIENTED_EDGE('',*,*,#9706,.F.);
#15145=ORIENTED_EDGE('',*,*,#9715,.F.);
#15146=ORIENTED_EDGE('',*,*,#9718,.F.);
#15147=ORIENTED_EDGE('',*,*,#9721,.F.);
#15148=ORIENTED_EDGE('',*,*,#9724,.F.);
#15149=ORIENTED_EDGE('',*,*,#9727,.F.);
#15150=ORIENTED_EDGE('',*,*,#9730,.F.);
#15151=ORIENTED_EDGE('',*,*,#10431,.F.);
#15152=ORIENTED_EDGE('',*,*,#9735,.F.);
#15153=ORIENTED_EDGE('',*,*,#10342,.F.);
#15154=ORIENTED_EDGE('',*,*,#9759,.T.);
#15155=ORIENTED_EDGE('',*,*,#10429,.T.);
#15156=ORIENTED_EDGE('',*,*,#9757,.T.);
#15157=ORIENTED_EDGE('',*,*,#9754,.T.);
#15158=ORIENTED_EDGE('',*,*,#9751,.T.);
#15159=ORIENTED_EDGE('',*,*,#9748,.T.);
#15160=ORIENTED_EDGE('',*,*,#9745,.T.);
#15161=ORIENTED_EDGE('',*,*,#9742,.T.);
#15162=ORIENTED_EDGE('',*,*,#9739,.T.);
#15163=ORIENTED_EDGE('',*,*,#9732,.T.);
#15164=ORIENTED_EDGE('',*,*,#10431,.T.);
#15165=ORIENTED_EDGE('',*,*,#9729,.F.);
#15166=ORIENTED_EDGE('',*,*,#10430,.T.);
#15167=ORIENTED_EDGE('',*,*,#10432,.T.);
#15168=ORIENTED_EDGE('',*,*,#9937,.F.);
#15169=ORIENTED_EDGE('',*,*,#9939,.F.);
#15170=ORIENTED_EDGE('',*,*,#10433,.F.);
#15171=ORIENTED_EDGE('',*,*,#9938,.F.);
#15172=ORIENTED_EDGE('',*,*,#10434,.T.);
#15173=ORIENTED_EDGE('',*,*,#9880,.F.);
#15174=ORIENTED_EDGE('',*,*,#9882,.F.);
#15175=ORIENTED_EDGE('',*,*,#10435,.F.);
#15176=ORIENTED_EDGE('',*,*,#9881,.F.);
#15177=ORIENTED_EDGE('',*,*,#10436,.T.);
#15178=ORIENTED_EDGE('',*,*,#9823,.F.);
#15179=ORIENTED_EDGE('',*,*,#9825,.F.);
#15180=ORIENTED_EDGE('',*,*,#10437,.F.);
#15181=ORIENTED_EDGE('',*,*,#9824,.F.);
#15182=ORIENTED_EDGE('',*,*,#10438,.T.);
#15183=ORIENTED_EDGE('',*,*,#9766,.F.);
#15184=ORIENTED_EDGE('',*,*,#9768,.F.);
#15185=ORIENTED_EDGE('',*,*,#10439,.F.);
#15186=ORIENTED_EDGE('',*,*,#9767,.F.);
#15187=ORIENTED_EDGE('',*,*,#10440,.T.);
#15188=ORIENTED_EDGE('',*,*,#9709,.F.);
#15189=ORIENTED_EDGE('',*,*,#9711,.F.);
#15190=ORIENTED_EDGE('',*,*,#10441,.F.);
#15191=ORIENTED_EDGE('',*,*,#9710,.F.);
#15192=ORIENTED_EDGE('',*,*,#9650,.F.);
#15193=ORIENTED_EDGE('',*,*,#10442,.T.);
#15194=ORIENTED_EDGE('',*,*,#9681,.T.);
#15195=ORIENTED_EDGE('',*,*,#10443,.T.);
#15196=ORIENTED_EDGE('',*,*,#9655,.F.);
#15197=ORIENTED_EDGE('',*,*,#9701,.T.);
#15198=ORIENTED_EDGE('',*,*,#10444,.T.);
#15199=ORIENTED_EDGE('',*,*,#9698,.F.);
#15200=ORIENTED_EDGE('',*,*,#10445,.F.);
#15201=ORIENTED_EDGE('',*,*,#10443,.F.);
#15202=ORIENTED_EDGE('',*,*,#9680,.F.);
#15203=ORIENTED_EDGE('',*,*,#9684,.F.);
#15204=ORIENTED_EDGE('',*,*,#9687,.F.);
#15205=ORIENTED_EDGE('',*,*,#9690,.F.);
#15206=ORIENTED_EDGE('',*,*,#9693,.F.);
#15207=ORIENTED_EDGE('',*,*,#9696,.F.);
#15208=ORIENTED_EDGE('',*,*,#9699,.F.);
#15209=ORIENTED_EDGE('',*,*,#10444,.F.);
#15210=ORIENTED_EDGE('',*,*,#9704,.F.);
#15211=ORIENTED_EDGE('',*,*,#10446,.F.);
#15212=ORIENTED_EDGE('',*,*,#9676,.F.);
#15213=ORIENTED_EDGE('',*,*,#10447,.F.);
#15214=ORIENTED_EDGE('',*,*,#9674,.F.);
#15215=ORIENTED_EDGE('',*,*,#9671,.F.);
#15216=ORIENTED_EDGE('',*,*,#9668,.F.);
#15217=ORIENTED_EDGE('',*,*,#9665,.F.);
#15218=ORIENTED_EDGE('',*,*,#9662,.F.);
#15219=ORIENTED_EDGE('',*,*,#9659,.F.);
#15220=ORIENTED_EDGE('',*,*,#9656,.F.);
#15221=ORIENTED_EDGE('',*,*,#10442,.F.);
#15222=ORIENTED_EDGE('',*,*,#9649,.F.);
#15223=ORIENTED_EDGE('',*,*,#9658,.F.);
#15224=ORIENTED_EDGE('',*,*,#9661,.F.);
#15225=ORIENTED_EDGE('',*,*,#9664,.F.);
#15226=ORIENTED_EDGE('',*,*,#9667,.F.);
#15227=ORIENTED_EDGE('',*,*,#9670,.F.);
#15228=ORIENTED_EDGE('',*,*,#9673,.F.);
#15229=ORIENTED_EDGE('',*,*,#10448,.F.);
#15230=ORIENTED_EDGE('',*,*,#9678,.F.);
#15231=ORIENTED_EDGE('',*,*,#10449,.F.);
#15232=ORIENTED_EDGE('',*,*,#9702,.T.);
#15233=ORIENTED_EDGE('',*,*,#10445,.T.);
#15234=ORIENTED_EDGE('',*,*,#9700,.T.);
#15235=ORIENTED_EDGE('',*,*,#9697,.T.);
#15236=ORIENTED_EDGE('',*,*,#9694,.T.);
#15237=ORIENTED_EDGE('',*,*,#9691,.T.);
#15238=ORIENTED_EDGE('',*,*,#9688,.T.);
#15239=ORIENTED_EDGE('',*,*,#9685,.T.);
#15240=ORIENTED_EDGE('',*,*,#9682,.T.);
#15241=ORIENTED_EDGE('',*,*,#9675,.T.);
#15242=ORIENTED_EDGE('',*,*,#10448,.T.);
#15243=ORIENTED_EDGE('',*,*,#9672,.F.);
#15244=ORIENTED_EDGE('',*,*,#10447,.T.);
#15245=ORIENTED_EDGE('',*,*,#10450,.T.);
#15246=ORIENTED_EDGE('',*,*,#9652,.F.);
#15247=ORIENTED_EDGE('',*,*,#9654,.F.);
#15248=ORIENTED_EDGE('',*,*,#10451,.F.);
#15249=ORIENTED_EDGE('',*,*,#9653,.F.);
#15250=ORIENTED_EDGE('',*,*,#9593,.F.);
#15251=ORIENTED_EDGE('',*,*,#10452,.T.);
#15252=ORIENTED_EDGE('',*,*,#9624,.T.);
#15253=ORIENTED_EDGE('',*,*,#10453,.T.);
#15254=ORIENTED_EDGE('',*,*,#9598,.F.);
#15255=ORIENTED_EDGE('',*,*,#9644,.T.);
#15256=ORIENTED_EDGE('',*,*,#10454,.T.);
#15257=ORIENTED_EDGE('',*,*,#9641,.F.);
#15258=ORIENTED_EDGE('',*,*,#10455,.F.);
#15259=ORIENTED_EDGE('',*,*,#10453,.F.);
#15260=ORIENTED_EDGE('',*,*,#9623,.F.);
#15261=ORIENTED_EDGE('',*,*,#9627,.F.);
#15262=ORIENTED_EDGE('',*,*,#9630,.F.);
#15263=ORIENTED_EDGE('',*,*,#9633,.F.);
#15264=ORIENTED_EDGE('',*,*,#9636,.F.);
#15265=ORIENTED_EDGE('',*,*,#9639,.F.);
#15266=ORIENTED_EDGE('',*,*,#9642,.F.);
#15267=ORIENTED_EDGE('',*,*,#10454,.F.);
#15268=ORIENTED_EDGE('',*,*,#9647,.F.);
#15269=ORIENTED_EDGE('',*,*,#10340,.F.);
#15270=ORIENTED_EDGE('',*,*,#9619,.F.);
#15271=ORIENTED_EDGE('',*,*,#10456,.F.);
#15272=ORIENTED_EDGE('',*,*,#9617,.F.);
#15273=ORIENTED_EDGE('',*,*,#9614,.F.);
#15274=ORIENTED_EDGE('',*,*,#9611,.F.);
#15275=ORIENTED_EDGE('',*,*,#9608,.F.);
#15276=ORIENTED_EDGE('',*,*,#9605,.F.);
#15277=ORIENTED_EDGE('',*,*,#9602,.F.);
#15278=ORIENTED_EDGE('',*,*,#9599,.F.);
#15279=ORIENTED_EDGE('',*,*,#10452,.F.);
#15280=ORIENTED_EDGE('',*,*,#9592,.F.);
#15281=ORIENTED_EDGE('',*,*,#9601,.F.);
#15282=ORIENTED_EDGE('',*,*,#9604,.F.);
#15283=ORIENTED_EDGE('',*,*,#9607,.F.);
#15284=ORIENTED_EDGE('',*,*,#9610,.F.);
#15285=ORIENTED_EDGE('',*,*,#9613,.F.);
#15286=ORIENTED_EDGE('',*,*,#9616,.F.);
#15287=ORIENTED_EDGE('',*,*,#10457,.F.);
#15288=ORIENTED_EDGE('',*,*,#9621,.F.);
#15289=ORIENTED_EDGE('',*,*,#10339,.F.);
#15290=ORIENTED_EDGE('',*,*,#9645,.T.);
#15291=ORIENTED_EDGE('',*,*,#10455,.T.);
#15292=ORIENTED_EDGE('',*,*,#9643,.T.);
#15293=ORIENTED_EDGE('',*,*,#9640,.T.);
#15294=ORIENTED_EDGE('',*,*,#9637,.T.);
#15295=ORIENTED_EDGE('',*,*,#9634,.T.);
#15296=ORIENTED_EDGE('',*,*,#9631,.T.);
#15297=ORIENTED_EDGE('',*,*,#9628,.T.);
#15298=ORIENTED_EDGE('',*,*,#9625,.T.);
#15299=ORIENTED_EDGE('',*,*,#9618,.T.);
#15300=ORIENTED_EDGE('',*,*,#10457,.T.);
#15301=ORIENTED_EDGE('',*,*,#9615,.F.);
#15302=ORIENTED_EDGE('',*,*,#10456,.T.);
#15303=ORIENTED_EDGE('',*,*,#10458,.T.);
#15304=ORIENTED_EDGE('',*,*,#9595,.F.);
#15305=ORIENTED_EDGE('',*,*,#9597,.F.);
#15306=ORIENTED_EDGE('',*,*,#10459,.F.);
#15307=ORIENTED_EDGE('',*,*,#9596,.F.);
#15308=ORIENTED_EDGE('',*,*,#10460,.F.);
#15309=ORIENTED_EDGE('',*,*,#10461,.T.);
#15310=ORIENTED_EDGE('',*,*,#10462,.F.);
#15311=ORIENTED_EDGE('',*,*,#10461,.F.);
#15312=ORIENTED_EDGE('',*,*,#10463,.F.);
#15313=ORIENTED_EDGE('',*,*,#10464,.T.);
#15314=ORIENTED_EDGE('',*,*,#10392,.F.);
#15315=ORIENTED_EDGE('',*,*,#10465,.T.);
#15316=ORIENTED_EDGE('',*,*,#10466,.T.);
#15317=ORIENTED_EDGE('',*,*,#10465,.F.);
#15318=ORIENTED_EDGE('',*,*,#10393,.T.);
#15319=ORIENTED_EDGE('',*,*,#10464,.F.);
#15320=ORIENTED_EDGE('',*,*,#10433,.T.);
#15321=ORIENTED_EDGE('',*,*,#10432,.F.);
#15322=ORIENTED_EDGE('',*,*,#10466,.F.);
#15323=ORIENTED_EDGE('',*,*,#10460,.T.);
#15324=ORIENTED_EDGE('',*,*,#10467,.F.);
#15325=ORIENTED_EDGE('',*,*,#10468,.T.);
#15326=ORIENTED_EDGE('',*,*,#10469,.F.);
#15327=ORIENTED_EDGE('',*,*,#10468,.F.);
#15328=ORIENTED_EDGE('',*,*,#10470,.F.);
#15329=ORIENTED_EDGE('',*,*,#10471,.T.);
#15330=ORIENTED_EDGE('',*,*,#10394,.F.);
#15331=ORIENTED_EDGE('',*,*,#10472,.T.);
#15332=ORIENTED_EDGE('',*,*,#10473,.T.);
#15333=ORIENTED_EDGE('',*,*,#10472,.F.);
#15334=ORIENTED_EDGE('',*,*,#10395,.T.);
#15335=ORIENTED_EDGE('',*,*,#10471,.F.);
#15336=ORIENTED_EDGE('',*,*,#10435,.T.);
#15337=ORIENTED_EDGE('',*,*,#10434,.F.);
#15338=ORIENTED_EDGE('',*,*,#10473,.F.);
#15339=ORIENTED_EDGE('',*,*,#10467,.T.);
#15340=ORIENTED_EDGE('',*,*,#10474,.F.);
#15341=ORIENTED_EDGE('',*,*,#10475,.T.);
#15342=ORIENTED_EDGE('',*,*,#10476,.F.);
#15343=ORIENTED_EDGE('',*,*,#10475,.F.);
#15344=ORIENTED_EDGE('',*,*,#10477,.F.);
#15345=ORIENTED_EDGE('',*,*,#10478,.T.);
#15346=ORIENTED_EDGE('',*,*,#10396,.F.);
#15347=ORIENTED_EDGE('',*,*,#10479,.T.);
#15348=ORIENTED_EDGE('',*,*,#10480,.T.);
#15349=ORIENTED_EDGE('',*,*,#10479,.F.);
#15350=ORIENTED_EDGE('',*,*,#10397,.T.);
#15351=ORIENTED_EDGE('',*,*,#10478,.F.);
#15352=ORIENTED_EDGE('',*,*,#10437,.T.);
#15353=ORIENTED_EDGE('',*,*,#10436,.F.);
#15354=ORIENTED_EDGE('',*,*,#10480,.F.);
#15355=ORIENTED_EDGE('',*,*,#10474,.T.);
#15356=ORIENTED_EDGE('',*,*,#10481,.F.);
#15357=ORIENTED_EDGE('',*,*,#10482,.T.);
#15358=ORIENTED_EDGE('',*,*,#10483,.F.);
#15359=ORIENTED_EDGE('',*,*,#10482,.F.);
#15360=ORIENTED_EDGE('',*,*,#10484,.F.);
#15361=ORIENTED_EDGE('',*,*,#10485,.T.);
#15362=ORIENTED_EDGE('',*,*,#10398,.F.);
#15363=ORIENTED_EDGE('',*,*,#10486,.T.);
#15364=ORIENTED_EDGE('',*,*,#10487,.T.);
#15365=ORIENTED_EDGE('',*,*,#10486,.F.);
#15366=ORIENTED_EDGE('',*,*,#10399,.T.);
#15367=ORIENTED_EDGE('',*,*,#10485,.F.);
#15368=ORIENTED_EDGE('',*,*,#10439,.T.);
#15369=ORIENTED_EDGE('',*,*,#10438,.F.);
#15370=ORIENTED_EDGE('',*,*,#10487,.F.);
#15371=ORIENTED_EDGE('',*,*,#10481,.T.);
#15372=ORIENTED_EDGE('',*,*,#10488,.F.);
#15373=ORIENTED_EDGE('',*,*,#10489,.T.);
#15374=ORIENTED_EDGE('',*,*,#10490,.F.);
#15375=ORIENTED_EDGE('',*,*,#10489,.F.);
#15376=ORIENTED_EDGE('',*,*,#10491,.F.);
#15377=ORIENTED_EDGE('',*,*,#10492,.T.);
#15378=ORIENTED_EDGE('',*,*,#10400,.F.);
#15379=ORIENTED_EDGE('',*,*,#10493,.T.);
#15380=ORIENTED_EDGE('',*,*,#10494,.T.);
#15381=ORIENTED_EDGE('',*,*,#10493,.F.);
#15382=ORIENTED_EDGE('',*,*,#10401,.T.);
#15383=ORIENTED_EDGE('',*,*,#10492,.F.);
#15384=ORIENTED_EDGE('',*,*,#10441,.T.);
#15385=ORIENTED_EDGE('',*,*,#10440,.F.);
#15386=ORIENTED_EDGE('',*,*,#10494,.F.);
#15387=ORIENTED_EDGE('',*,*,#10488,.T.);
#15388=ORIENTED_EDGE('',*,*,#10495,.F.);
#15389=ORIENTED_EDGE('',*,*,#10496,.T.);
#15390=ORIENTED_EDGE('',*,*,#10497,.F.);
#15391=ORIENTED_EDGE('',*,*,#10496,.F.);
#15392=ORIENTED_EDGE('',*,*,#10498,.F.);
#15393=ORIENTED_EDGE('',*,*,#10499,.T.);
#15394=ORIENTED_EDGE('',*,*,#10450,.F.);
#15395=ORIENTED_EDGE('',*,*,#10500,.T.);
#15396=ORIENTED_EDGE('',*,*,#10501,.T.);
#15397=ORIENTED_EDGE('',*,*,#10500,.F.);
#15398=ORIENTED_EDGE('',*,*,#10451,.T.);
#15399=ORIENTED_EDGE('',*,*,#10499,.F.);
#15400=ORIENTED_EDGE('',*,*,#10459,.T.);
#15401=ORIENTED_EDGE('',*,*,#10458,.F.);
#15402=ORIENTED_EDGE('',*,*,#10501,.F.);
#15403=ORIENTED_EDGE('',*,*,#10495,.T.);
#15404=ORIENTED_EDGE('',*,*,#10502,.F.);
#15405=ORIENTED_EDGE('',*,*,#10503,.T.);
#15406=ORIENTED_EDGE('',*,*,#10504,.T.);
#15407=ORIENTED_EDGE('',*,*,#10335,.F.);
#15408=ORIENTED_EDGE('',*,*,#10505,.F.);
#15409=ORIENTED_EDGE('',*,*,#10338,.F.);
#15410=ORIENTED_EDGE('',*,*,#10506,.F.);
#15411=ORIENTED_EDGE('',*,*,#10507,.T.);
#15412=ORIENTED_EDGE('',*,*,#10463,.T.);
#15413=ORIENTED_EDGE('',*,*,#10508,.T.);
#15414=ORIENTED_EDGE('',*,*,#10506,.T.);
#15415=ORIENTED_EDGE('',*,*,#10337,.F.);
#15416=ORIENTED_EDGE('',*,*,#10509,.F.);
#15417=ORIENTED_EDGE('',*,*,#10510,.T.);
#15418=ORIENTED_EDGE('',*,*,#10509,.T.);
#15419=ORIENTED_EDGE('',*,*,#10336,.F.);
#15420=ORIENTED_EDGE('',*,*,#10504,.F.);
#15421=ORIENTED_EDGE('',*,*,#10462,.T.);
#15422=ORIENTED_EDGE('',*,*,#10511,.F.);
#15423=ORIENTED_EDGE('',*,*,#10329,.F.);
#15424=ORIENTED_EDGE('',*,*,#10512,.F.);
#15425=ORIENTED_EDGE('',*,*,#10513,.T.);
#15426=ORIENTED_EDGE('',*,*,#10470,.T.);
#15427=ORIENTED_EDGE('',*,*,#10514,.T.);
#15428=ORIENTED_EDGE('',*,*,#10512,.T.);
#15429=ORIENTED_EDGE('',*,*,#10328,.F.);
#15430=ORIENTED_EDGE('',*,*,#10515,.F.);
#15431=ORIENTED_EDGE('',*,*,#10516,.T.);
#15432=ORIENTED_EDGE('',*,*,#10515,.T.);
#15433=ORIENTED_EDGE('',*,*,#10327,.F.);
#15434=ORIENTED_EDGE('',*,*,#10517,.F.);
#15435=ORIENTED_EDGE('',*,*,#10469,.T.);
#15436=ORIENTED_EDGE('',*,*,#10518,.F.);
#15437=ORIENTED_EDGE('',*,*,#10519,.T.);
#15438=ORIENTED_EDGE('',*,*,#10517,.T.);
#15439=ORIENTED_EDGE('',*,*,#10326,.F.);
#15440=ORIENTED_EDGE('',*,*,#10520,.F.);
#15441=ORIENTED_EDGE('',*,*,#10320,.F.);
#15442=ORIENTED_EDGE('',*,*,#10521,.F.);
#15443=ORIENTED_EDGE('',*,*,#10522,.T.);
#15444=ORIENTED_EDGE('',*,*,#10477,.T.);
#15445=ORIENTED_EDGE('',*,*,#10523,.T.);
#15446=ORIENTED_EDGE('',*,*,#10521,.T.);
#15447=ORIENTED_EDGE('',*,*,#10319,.F.);
#15448=ORIENTED_EDGE('',*,*,#10524,.F.);
#15449=ORIENTED_EDGE('',*,*,#10525,.T.);
#15450=ORIENTED_EDGE('',*,*,#10524,.T.);
#15451=ORIENTED_EDGE('',*,*,#10318,.F.);
#15452=ORIENTED_EDGE('',*,*,#10526,.F.);
#15453=ORIENTED_EDGE('',*,*,#10476,.T.);
#15454=ORIENTED_EDGE('',*,*,#10527,.F.);
#15455=ORIENTED_EDGE('',*,*,#10528,.T.);
#15456=ORIENTED_EDGE('',*,*,#10526,.T.);
#15457=ORIENTED_EDGE('',*,*,#10317,.F.);
#15458=ORIENTED_EDGE('',*,*,#10529,.F.);
#15459=ORIENTED_EDGE('',*,*,#10311,.F.);
#15460=ORIENTED_EDGE('',*,*,#10530,.F.);
#15461=ORIENTED_EDGE('',*,*,#10531,.T.);
#15462=ORIENTED_EDGE('',*,*,#10484,.T.);
#15463=ORIENTED_EDGE('',*,*,#10532,.T.);
#15464=ORIENTED_EDGE('',*,*,#10530,.T.);
#15465=ORIENTED_EDGE('',*,*,#10310,.F.);
#15466=ORIENTED_EDGE('',*,*,#10533,.F.);
#15467=ORIENTED_EDGE('',*,*,#10534,.T.);
#15468=ORIENTED_EDGE('',*,*,#10533,.T.);
#15469=ORIENTED_EDGE('',*,*,#10309,.F.);
#15470=ORIENTED_EDGE('',*,*,#10535,.F.);
#15471=ORIENTED_EDGE('',*,*,#10483,.T.);
#15472=ORIENTED_EDGE('',*,*,#10536,.F.);
#15473=ORIENTED_EDGE('',*,*,#10537,.T.);
#15474=ORIENTED_EDGE('',*,*,#10535,.T.);
#15475=ORIENTED_EDGE('',*,*,#10308,.F.);
#15476=ORIENTED_EDGE('',*,*,#10538,.F.);
#15477=ORIENTED_EDGE('',*,*,#10539,.T.);
#15478=ORIENTED_EDGE('',*,*,#10540,.T.);
#15479=ORIENTED_EDGE('',*,*,#10299,.F.);
#15480=ORIENTED_EDGE('',*,*,#10541,.F.);
#15481=ORIENTED_EDGE('',*,*,#10302,.F.);
#15482=ORIENTED_EDGE('',*,*,#10542,.F.);
#15483=ORIENTED_EDGE('',*,*,#10543,.T.);
#15484=ORIENTED_EDGE('',*,*,#10491,.T.);
#15485=ORIENTED_EDGE('',*,*,#10544,.T.);
#15486=ORIENTED_EDGE('',*,*,#10542,.T.);
#15487=ORIENTED_EDGE('',*,*,#10301,.F.);
#15488=ORIENTED_EDGE('',*,*,#10545,.F.);
#15489=ORIENTED_EDGE('',*,*,#10546,.T.);
#15490=ORIENTED_EDGE('',*,*,#10545,.T.);
#15491=ORIENTED_EDGE('',*,*,#10300,.F.);
#15492=ORIENTED_EDGE('',*,*,#10540,.F.);
#15493=ORIENTED_EDGE('',*,*,#10490,.T.);
#15494=ORIENTED_EDGE('',*,*,#10505,.T.);
#15495=ORIENTED_EDGE('',*,*,#10547,.T.);
#15496=ORIENTED_EDGE('',*,*,#10548,.F.);
#15497=ORIENTED_EDGE('',*,*,#10285,.T.);
#15498=ORIENTED_EDGE('',*,*,#10511,.T.);
#15499=ORIENTED_EDGE('',*,*,#10549,.T.);
#15500=ORIENTED_EDGE('',*,*,#10550,.F.);
#15501=ORIENTED_EDGE('',*,*,#10330,.T.);
#15502=ORIENTED_EDGE('',*,*,#10518,.T.);
#15503=ORIENTED_EDGE('',*,*,#10325,.T.);
#15504=ORIENTED_EDGE('',*,*,#10551,.F.);
#15505=ORIENTED_EDGE('',*,*,#10552,.T.);
#15506=ORIENTED_EDGE('',*,*,#10520,.T.);
#15507=ORIENTED_EDGE('',*,*,#10553,.T.);
#15508=ORIENTED_EDGE('',*,*,#10554,.F.);
#15509=ORIENTED_EDGE('',*,*,#10321,.T.);
#15510=ORIENTED_EDGE('',*,*,#10527,.T.);
#15511=ORIENTED_EDGE('',*,*,#10316,.T.);
#15512=ORIENTED_EDGE('',*,*,#10555,.F.);
#15513=ORIENTED_EDGE('',*,*,#10556,.T.);
#15514=ORIENTED_EDGE('',*,*,#10529,.T.);
#15515=ORIENTED_EDGE('',*,*,#10557,.T.);
#15516=ORIENTED_EDGE('',*,*,#10558,.F.);
#15517=ORIENTED_EDGE('',*,*,#10312,.T.);
#15518=ORIENTED_EDGE('',*,*,#10536,.T.);
#15519=ORIENTED_EDGE('',*,*,#10307,.T.);
#15520=ORIENTED_EDGE('',*,*,#10559,.F.);
#15521=ORIENTED_EDGE('',*,*,#10560,.T.);
#15522=ORIENTED_EDGE('',*,*,#10541,.T.);
#15523=ORIENTED_EDGE('',*,*,#10561,.T.);
#15524=ORIENTED_EDGE('',*,*,#10562,.F.);
#15525=ORIENTED_EDGE('',*,*,#10303,.T.);
#15526=ORIENTED_EDGE('',*,*,#10563,.F.);
#15527=ORIENTED_EDGE('',*,*,#10564,.T.);
#15528=ORIENTED_EDGE('',*,*,#10565,.T.);
#15529=ORIENTED_EDGE('',*,*,#10290,.F.);
#15530=ORIENTED_EDGE('',*,*,#10566,.F.);
#15531=ORIENTED_EDGE('',*,*,#10293,.F.);
#15532=ORIENTED_EDGE('',*,*,#10567,.F.);
#15533=ORIENTED_EDGE('',*,*,#10568,.T.);
#15534=ORIENTED_EDGE('',*,*,#10498,.T.);
#15535=ORIENTED_EDGE('',*,*,#10569,.T.);
#15536=ORIENTED_EDGE('',*,*,#10567,.T.);
#15537=ORIENTED_EDGE('',*,*,#10292,.F.);
#15538=ORIENTED_EDGE('',*,*,#10570,.F.);
#15539=ORIENTED_EDGE('',*,*,#10571,.T.);
#15540=ORIENTED_EDGE('',*,*,#10570,.T.);
#15541=ORIENTED_EDGE('',*,*,#10291,.F.);
#15542=ORIENTED_EDGE('',*,*,#10565,.F.);
#15543=ORIENTED_EDGE('',*,*,#10497,.T.);
#15544=ORIENTED_EDGE('',*,*,#10566,.T.);
#15545=ORIENTED_EDGE('',*,*,#10572,.T.);
#15546=ORIENTED_EDGE('',*,*,#10573,.F.);
#15547=ORIENTED_EDGE('',*,*,#10294,.T.);
#15548=ORIENTED_EDGE('',*,*,#10324,.T.);
#15549=ORIENTED_EDGE('',*,*,#10574,.F.);
#15550=ORIENTED_EDGE('',*,*,#10575,.T.);
#15551=ORIENTED_EDGE('',*,*,#10551,.T.);
#15552=ORIENTED_EDGE('',*,*,#10323,.T.);
#15553=ORIENTED_EDGE('',*,*,#10576,.T.);
#15554=ORIENTED_EDGE('',*,*,#10577,.T.);
#15555=ORIENTED_EDGE('',*,*,#10574,.T.);
#15556=ORIENTED_EDGE('',*,*,#10322,.T.);
#15557=ORIENTED_EDGE('',*,*,#10554,.T.);
#15558=ORIENTED_EDGE('',*,*,#10578,.T.);
#15559=ORIENTED_EDGE('',*,*,#10576,.F.);
#15560=ORIENTED_EDGE('',*,*,#10315,.T.);
#15561=ORIENTED_EDGE('',*,*,#10579,.F.);
#15562=ORIENTED_EDGE('',*,*,#10580,.T.);
#15563=ORIENTED_EDGE('',*,*,#10555,.T.);
#15564=ORIENTED_EDGE('',*,*,#10314,.T.);
#15565=ORIENTED_EDGE('',*,*,#10581,.T.);
#15566=ORIENTED_EDGE('',*,*,#10582,.T.);
#15567=ORIENTED_EDGE('',*,*,#10579,.T.);
#15568=ORIENTED_EDGE('',*,*,#10313,.T.);
#15569=ORIENTED_EDGE('',*,*,#10558,.T.);
#15570=ORIENTED_EDGE('',*,*,#10583,.T.);
#15571=ORIENTED_EDGE('',*,*,#10581,.F.);
#15572=ORIENTED_EDGE('',*,*,#10306,.T.);
#15573=ORIENTED_EDGE('',*,*,#10584,.F.);
#15574=ORIENTED_EDGE('',*,*,#10585,.T.);
#15575=ORIENTED_EDGE('',*,*,#10559,.T.);
#15576=ORIENTED_EDGE('',*,*,#10305,.T.);
#15577=ORIENTED_EDGE('',*,*,#10586,.T.);
#15578=ORIENTED_EDGE('',*,*,#10587,.T.);
#15579=ORIENTED_EDGE('',*,*,#10584,.T.);
#15580=ORIENTED_EDGE('',*,*,#10304,.T.);
#15581=ORIENTED_EDGE('',*,*,#10562,.T.);
#15582=ORIENTED_EDGE('',*,*,#10588,.T.);
#15583=ORIENTED_EDGE('',*,*,#10586,.F.);
#15584=ORIENTED_EDGE('',*,*,#10589,.F.);
#15585=ORIENTED_EDGE('',*,*,#10590,.F.);
#15586=ORIENTED_EDGE('',*,*,#10591,.F.);
#15587=ORIENTED_EDGE('',*,*,#10592,.F.);
#15588=ORIENTED_EDGE('',*,*,#10549,.F.);
#15589=ORIENTED_EDGE('',*,*,#10513,.F.);
#15590=ORIENTED_EDGE('',*,*,#10514,.F.);
#15591=ORIENTED_EDGE('',*,*,#10516,.F.);
#15592=ORIENTED_EDGE('',*,*,#10519,.F.);
#15593=ORIENTED_EDGE('',*,*,#10552,.F.);
#15594=ORIENTED_EDGE('',*,*,#10575,.F.);
#15595=ORIENTED_EDGE('',*,*,#10577,.F.);
#15596=ORIENTED_EDGE('',*,*,#10578,.F.);
#15597=ORIENTED_EDGE('',*,*,#10553,.F.);
#15598=ORIENTED_EDGE('',*,*,#10522,.F.);
#15599=ORIENTED_EDGE('',*,*,#10523,.F.);
#15600=ORIENTED_EDGE('',*,*,#10525,.F.);
#15601=ORIENTED_EDGE('',*,*,#10528,.F.);
#15602=ORIENTED_EDGE('',*,*,#10556,.F.);
#15603=ORIENTED_EDGE('',*,*,#10580,.F.);
#15604=ORIENTED_EDGE('',*,*,#10582,.F.);
#15605=ORIENTED_EDGE('',*,*,#10583,.F.);
#15606=ORIENTED_EDGE('',*,*,#10557,.F.);
#15607=ORIENTED_EDGE('',*,*,#10531,.F.);
#15608=ORIENTED_EDGE('',*,*,#10532,.F.);
#15609=ORIENTED_EDGE('',*,*,#10534,.F.);
#15610=ORIENTED_EDGE('',*,*,#10537,.F.);
#15611=ORIENTED_EDGE('',*,*,#10560,.F.);
#15612=ORIENTED_EDGE('',*,*,#10585,.F.);
#15613=ORIENTED_EDGE('',*,*,#10587,.F.);
#15614=ORIENTED_EDGE('',*,*,#10588,.F.);
#15615=ORIENTED_EDGE('',*,*,#10561,.F.);
#15616=ORIENTED_EDGE('',*,*,#10543,.F.);
#15617=ORIENTED_EDGE('',*,*,#10544,.F.);
#15618=ORIENTED_EDGE('',*,*,#10546,.F.);
#15619=ORIENTED_EDGE('',*,*,#10539,.F.);
#15620=ORIENTED_EDGE('',*,*,#10593,.F.);
#15621=ORIENTED_EDGE('',*,*,#10594,.F.);
#15622=ORIENTED_EDGE('',*,*,#10595,.F.);
#15623=ORIENTED_EDGE('',*,*,#10596,.F.);
#15624=ORIENTED_EDGE('',*,*,#10572,.F.);
#15625=ORIENTED_EDGE('',*,*,#10568,.F.);
#15626=ORIENTED_EDGE('',*,*,#10569,.F.);
#15627=ORIENTED_EDGE('',*,*,#10571,.F.);
#15628=ORIENTED_EDGE('',*,*,#10564,.F.);
#15629=ORIENTED_EDGE('',*,*,#10597,.F.);
#15630=ORIENTED_EDGE('',*,*,#10598,.F.);
#15631=ORIENTED_EDGE('',*,*,#10599,.F.);
#15632=ORIENTED_EDGE('',*,*,#10600,.F.);
#15633=ORIENTED_EDGE('',*,*,#10547,.F.);
#15634=ORIENTED_EDGE('',*,*,#10507,.F.);
#15635=ORIENTED_EDGE('',*,*,#10508,.F.);
#15636=ORIENTED_EDGE('',*,*,#10510,.F.);
#15637=ORIENTED_EDGE('',*,*,#10503,.F.);
#15638=ORIENTED_EDGE('',*,*,#10283,.T.);
#15639=ORIENTED_EDGE('',*,*,#10601,.F.);
#15640=ORIENTED_EDGE('',*,*,#10278,.T.);
#15641=ORIENTED_EDGE('',*,*,#10281,.T.);
#15642=ORIENTED_EDGE('',*,*,#10359,.T.);
#15643=ORIENTED_EDGE('',*,*,#10247,.T.);
#15644=ORIENTED_EDGE('',*,*,#10356,.T.);
#15645=ORIENTED_EDGE('',*,*,#10273,.T.);
#15646=ORIENTED_EDGE('',*,*,#10367,.T.);
#15647=ORIENTED_EDGE('',*,*,#10190,.T.);
#15648=ORIENTED_EDGE('',*,*,#10364,.T.);
#15649=ORIENTED_EDGE('',*,*,#10216,.T.);
#15650=ORIENTED_EDGE('',*,*,#10375,.T.);
#15651=ORIENTED_EDGE('',*,*,#10133,.T.);
#15652=ORIENTED_EDGE('',*,*,#10372,.T.);
#15653=ORIENTED_EDGE('',*,*,#10159,.T.);
#15654=ORIENTED_EDGE('',*,*,#10383,.T.);
#15655=ORIENTED_EDGE('',*,*,#10076,.T.);
#15656=ORIENTED_EDGE('',*,*,#10380,.T.);
#15657=ORIENTED_EDGE('',*,*,#10102,.T.);
#15658=ORIENTED_EDGE('',*,*,#10391,.T.);
#15659=ORIENTED_EDGE('',*,*,#10019,.T.);
#15660=ORIENTED_EDGE('',*,*,#10388,.T.);
#15661=ORIENTED_EDGE('',*,*,#10045,.T.);
#15662=ORIENTED_EDGE('',*,*,#10449,.T.);
#15663=ORIENTED_EDGE('',*,*,#9677,.T.);
#15664=ORIENTED_EDGE('',*,*,#10446,.T.);
#15665=ORIENTED_EDGE('',*,*,#9703,.T.);
#15666=ORIENTED_EDGE('',*,*,#10331,.T.);
#15667=ORIENTED_EDGE('',*,*,#10550,.T.);
#15668=ORIENTED_EDGE('',*,*,#10592,.T.);
#15669=ORIENTED_EDGE('',*,*,#10602,.F.);
#15670=ORIENTED_EDGE('',*,*,#10332,.T.);
#15671=ORIENTED_EDGE('',*,*,#10602,.T.);
#15672=ORIENTED_EDGE('',*,*,#10591,.T.);
#15673=ORIENTED_EDGE('',*,*,#10603,.T.);
#15674=ORIENTED_EDGE('',*,*,#10333,.T.);
#15675=ORIENTED_EDGE('',*,*,#10603,.F.);
#15676=ORIENTED_EDGE('',*,*,#10590,.T.);
#15677=ORIENTED_EDGE('',*,*,#10604,.T.);
#15678=ORIENTED_EDGE('',*,*,#10502,.T.);
#15679=ORIENTED_EDGE('',*,*,#10334,.T.);
#15680=ORIENTED_EDGE('',*,*,#10604,.F.);
#15681=ORIENTED_EDGE('',*,*,#10589,.T.);
#15682=ORIENTED_EDGE('',*,*,#10286,.T.);
#15683=ORIENTED_EDGE('',*,*,#10548,.T.);
#15684=ORIENTED_EDGE('',*,*,#10600,.T.);
#15685=ORIENTED_EDGE('',*,*,#10605,.F.);
#15686=ORIENTED_EDGE('',*,*,#10287,.T.);
#15687=ORIENTED_EDGE('',*,*,#10605,.T.);
#15688=ORIENTED_EDGE('',*,*,#10599,.T.);
#15689=ORIENTED_EDGE('',*,*,#10606,.T.);
#15690=ORIENTED_EDGE('',*,*,#10288,.T.);
#15691=ORIENTED_EDGE('',*,*,#10606,.F.);
#15692=ORIENTED_EDGE('',*,*,#10598,.T.);
#15693=ORIENTED_EDGE('',*,*,#10607,.T.);
#15694=ORIENTED_EDGE('',*,*,#10563,.T.);
#15695=ORIENTED_EDGE('',*,*,#10289,.T.);
#15696=ORIENTED_EDGE('',*,*,#10607,.F.);
#15697=ORIENTED_EDGE('',*,*,#10597,.T.);
#15698=ORIENTED_EDGE('',*,*,#10295,.T.);
#15699=ORIENTED_EDGE('',*,*,#10573,.T.);
#15700=ORIENTED_EDGE('',*,*,#10596,.T.);
#15701=ORIENTED_EDGE('',*,*,#10608,.F.);
#15702=ORIENTED_EDGE('',*,*,#10538,.T.);
#15703=ORIENTED_EDGE('',*,*,#10298,.T.);
#15704=ORIENTED_EDGE('',*,*,#10609,.F.);
#15705=ORIENTED_EDGE('',*,*,#10593,.T.);
#15706=ORIENTED_EDGE('',*,*,#10296,.T.);
#15707=ORIENTED_EDGE('',*,*,#10608,.T.);
#15708=ORIENTED_EDGE('',*,*,#10595,.T.);
#15709=ORIENTED_EDGE('',*,*,#10610,.T.);
#15710=ORIENTED_EDGE('',*,*,#10297,.T.);
#15711=ORIENTED_EDGE('',*,*,#10610,.F.);
#15712=ORIENTED_EDGE('',*,*,#10594,.T.);
#15713=ORIENTED_EDGE('',*,*,#10609,.T.);
#15714=ORIENTED_EDGE('',*,*,#10282,.T.);
#15715=ORIENTED_EDGE('',*,*,#10341,.T.);
#15716=ORIENTED_EDGE('',*,*,#10275,.T.);
#15717=ORIENTED_EDGE('',*,*,#10601,.T.);
#16930=CYLINDRICAL_SURFACE('',#18966,1.2645);
#16931=CYLINDRICAL_SURFACE('',#18972,1.2645);
#16932=CYLINDRICAL_SURFACE('',#18973,1.2645);
#16933=CYLINDRICAL_SURFACE('',#18974,1.2645);
#16934=CYLINDRICAL_SURFACE('',#18975,1.2645);
#16935=CYLINDRICAL_SURFACE('',#18976,1.2645);
#16936=CYLINDRICAL_SURFACE('',#18977,1.2645);
#16937=CYLINDRICAL_SURFACE('',#18978,1.2645);
#16938=CYLINDRICAL_SURFACE('',#18980,1.543);
#16939=CYLINDRICAL_SURFACE('',#18982,1.543);
#16940=CYLINDRICAL_SURFACE('',#18983,1.543);
#16941=CYLINDRICAL_SURFACE('',#18984,1.543);
#16942=CYLINDRICAL_SURFACE('',#18985,1.543);
#16943=CYLINDRICAL_SURFACE('',#18986,1.543);
#16944=CYLINDRICAL_SURFACE('',#18987,1.543);
#16945=CYLINDRICAL_SURFACE('',#18988,1.543);
#16946=CYLINDRICAL_SURFACE('',#18990,1.2645);
#16947=CYLINDRICAL_SURFACE('',#18996,1.2645);
#16948=CYLINDRICAL_SURFACE('',#18997,1.2645);
#16949=CYLINDRICAL_SURFACE('',#18998,1.2645);
#16950=CYLINDRICAL_SURFACE('',#18999,1.2645);
#16951=CYLINDRICAL_SURFACE('',#19000,1.2645);
#16952=CYLINDRICAL_SURFACE('',#19001,1.2645);
#16953=CYLINDRICAL_SURFACE('',#19002,1.2645);
#16954=CYLINDRICAL_SURFACE('',#19004,1.54299999999999);
#16955=CYLINDRICAL_SURFACE('',#19006,1.54299999999999);
#16956=CYLINDRICAL_SURFACE('',#19007,1.54299999999999);
#16957=CYLINDRICAL_SURFACE('',#19008,1.54299999999999);
#16958=CYLINDRICAL_SURFACE('',#19009,1.54299999999999);
#16959=CYLINDRICAL_SURFACE('',#19010,1.54299999999999);
#16960=CYLINDRICAL_SURFACE('',#19011,1.54299999999999);
#16961=CYLINDRICAL_SURFACE('',#19012,1.54299999999999);
#16962=CYLINDRICAL_SURFACE('',#19014,1.2645);
#16963=CYLINDRICAL_SURFACE('',#19020,1.2645);
#16964=CYLINDRICAL_SURFACE('',#19021,1.2645);
#16965=CYLINDRICAL_SURFACE('',#19022,1.2645);
#16966=CYLINDRICAL_SURFACE('',#19023,1.2645);
#16967=CYLINDRICAL_SURFACE('',#19024,1.2645);
#16968=CYLINDRICAL_SURFACE('',#19025,1.2645);
#16969=CYLINDRICAL_SURFACE('',#19026,1.2645);
#16970=CYLINDRICAL_SURFACE('',#19028,1.543);
#16971=CYLINDRICAL_SURFACE('',#19030,1.543);
#16972=CYLINDRICAL_SURFACE('',#19031,1.543);
#16973=CYLINDRICAL_SURFACE('',#19032,1.543);
#16974=CYLINDRICAL_SURFACE('',#19033,1.543);
#16975=CYLINDRICAL_SURFACE('',#19034,1.543);
#16976=CYLINDRICAL_SURFACE('',#19035,1.543);
#16977=CYLINDRICAL_SURFACE('',#19036,1.543);
#16978=CYLINDRICAL_SURFACE('',#19038,1.2645);
#16979=CYLINDRICAL_SURFACE('',#19044,1.2645);
#16980=CYLINDRICAL_SURFACE('',#19045,1.2645);
#16981=CYLINDRICAL_SURFACE('',#19046,1.2645);
#16982=CYLINDRICAL_SURFACE('',#19047,1.2645);
#16983=CYLINDRICAL_SURFACE('',#19048,1.2645);
#16984=CYLINDRICAL_SURFACE('',#19049,1.2645);
#16985=CYLINDRICAL_SURFACE('',#19050,1.2645);
#16986=CYLINDRICAL_SURFACE('',#19052,1.543);
#16987=CYLINDRICAL_SURFACE('',#19054,1.543);
#16988=CYLINDRICAL_SURFACE('',#19055,1.543);
#16989=CYLINDRICAL_SURFACE('',#19056,1.543);
#16990=CYLINDRICAL_SURFACE('',#19057,1.543);
#16991=CYLINDRICAL_SURFACE('',#19058,1.543);
#16992=CYLINDRICAL_SURFACE('',#19059,1.543);
#16993=CYLINDRICAL_SURFACE('',#19060,1.543);
#16994=CYLINDRICAL_SURFACE('',#19062,1.2645);
#16995=CYLINDRICAL_SURFACE('',#19068,1.2645);
#16996=CYLINDRICAL_SURFACE('',#19069,1.2645);
#16997=CYLINDRICAL_SURFACE('',#19070,1.2645);
#16998=CYLINDRICAL_SURFACE('',#19071,1.2645);
#16999=CYLINDRICAL_SURFACE('',#19072,1.2645);
#17000=CYLINDRICAL_SURFACE('',#19073,1.2645);
#17001=CYLINDRICAL_SURFACE('',#19074,1.2645);
#17002=CYLINDRICAL_SURFACE('',#19076,1.54300000000001);
#17003=CYLINDRICAL_SURFACE('',#19078,1.54300000000001);
#17004=CYLINDRICAL_SURFACE('',#19079,1.54300000000001);
#17005=CYLINDRICAL_SURFACE('',#19080,1.54300000000001);
#17006=CYLINDRICAL_SURFACE('',#19081,1.54300000000001);
#17007=CYLINDRICAL_SURFACE('',#19082,1.54300000000001);
#17008=CYLINDRICAL_SURFACE('',#19083,1.54300000000001);
#17009=CYLINDRICAL_SURFACE('',#19084,1.54300000000001);
#17010=CYLINDRICAL_SURFACE('',#19086,1.2645);
#17011=CYLINDRICAL_SURFACE('',#19092,1.2645);
#17012=CYLINDRICAL_SURFACE('',#19093,1.2645);
#17013=CYLINDRICAL_SURFACE('',#19094,1.2645);
#17014=CYLINDRICAL_SURFACE('',#19095,1.2645);
#17015=CYLINDRICAL_SURFACE('',#19096,1.2645);
#17016=CYLINDRICAL_SURFACE('',#19097,1.2645);
#17017=CYLINDRICAL_SURFACE('',#19098,1.2645);
#17018=CYLINDRICAL_SURFACE('',#19100,1.54300000000001);
#17019=CYLINDRICAL_SURFACE('',#19102,1.54300000000001);
#17020=CYLINDRICAL_SURFACE('',#19103,1.54300000000001);
#17021=CYLINDRICAL_SURFACE('',#19104,1.54300000000001);
#17022=CYLINDRICAL_SURFACE('',#19105,1.54300000000001);
#17023=CYLINDRICAL_SURFACE('',#19106,1.54300000000001);
#17024=CYLINDRICAL_SURFACE('',#19107,1.54300000000001);
#17025=CYLINDRICAL_SURFACE('',#19108,1.54300000000001);
#17026=CYLINDRICAL_SURFACE('',#19110,1.2645);
#17027=CYLINDRICAL_SURFACE('',#19116,1.2645);
#17028=CYLINDRICAL_SURFACE('',#19117,1.2645);
#17029=CYLINDRICAL_SURFACE('',#19118,1.2645);
#17030=CYLINDRICAL_SURFACE('',#19119,1.2645);
#17031=CYLINDRICAL_SURFACE('',#19120,1.2645);
#17032=CYLINDRICAL_SURFACE('',#19121,1.2645);
#17033=CYLINDRICAL_SURFACE('',#19122,1.2645);
#17034=CYLINDRICAL_SURFACE('',#19124,1.543);
#17035=CYLINDRICAL_SURFACE('',#19126,1.543);
#17036=CYLINDRICAL_SURFACE('',#19127,1.543);
#17037=CYLINDRICAL_SURFACE('',#19128,1.543);
#17038=CYLINDRICAL_SURFACE('',#19129,1.543);
#17039=CYLINDRICAL_SURFACE('',#19130,1.543);
#17040=CYLINDRICAL_SURFACE('',#19131,1.543);
#17041=CYLINDRICAL_SURFACE('',#19132,1.543);
#17042=CYLINDRICAL_SURFACE('',#19134,1.2645);
#17043=CYLINDRICAL_SURFACE('',#19140,1.2645);
#17044=CYLINDRICAL_SURFACE('',#19141,1.2645);
#17045=CYLINDRICAL_SURFACE('',#19142,1.2645);
#17046=CYLINDRICAL_SURFACE('',#19143,1.2645);
#17047=CYLINDRICAL_SURFACE('',#19144,1.2645);
#17048=CYLINDRICAL_SURFACE('',#19145,1.2645);
#17049=CYLINDRICAL_SURFACE('',#19146,1.2645);
#17050=CYLINDRICAL_SURFACE('',#19148,1.54300000000001);
#17051=CYLINDRICAL_SURFACE('',#19150,1.54300000000001);
#17052=CYLINDRICAL_SURFACE('',#19151,1.54300000000001);
#17053=CYLINDRICAL_SURFACE('',#19152,1.54300000000001);
#17054=CYLINDRICAL_SURFACE('',#19153,1.54300000000001);
#17055=CYLINDRICAL_SURFACE('',#19154,1.54300000000001);
#17056=CYLINDRICAL_SURFACE('',#19155,1.54300000000001);
#17057=CYLINDRICAL_SURFACE('',#19156,1.54300000000001);
#17058=CYLINDRICAL_SURFACE('',#19158,1.2645);
#17059=CYLINDRICAL_SURFACE('',#19164,1.2645);
#17060=CYLINDRICAL_SURFACE('',#19165,1.2645);
#17061=CYLINDRICAL_SURFACE('',#19166,1.2645);
#17062=CYLINDRICAL_SURFACE('',#19167,1.2645);
#17063=CYLINDRICAL_SURFACE('',#19168,1.2645);
#17064=CYLINDRICAL_SURFACE('',#19169,1.2645);
#17065=CYLINDRICAL_SURFACE('',#19170,1.2645);
#17066=CYLINDRICAL_SURFACE('',#19172,1.54300000000001);
#17067=CYLINDRICAL_SURFACE('',#19174,1.54300000000001);
#17068=CYLINDRICAL_SURFACE('',#19175,1.54300000000001);
#17069=CYLINDRICAL_SURFACE('',#19176,1.54300000000001);
#17070=CYLINDRICAL_SURFACE('',#19177,1.54300000000001);
#17071=CYLINDRICAL_SURFACE('',#19178,1.54300000000001);
#17072=CYLINDRICAL_SURFACE('',#19179,1.54300000000001);
#17073=CYLINDRICAL_SURFACE('',#19180,1.54300000000001);
#17074=CYLINDRICAL_SURFACE('',#19182,1.2645);
#17075=CYLINDRICAL_SURFACE('',#19188,1.2645);
#17076=CYLINDRICAL_SURFACE('',#19189,1.2645);
#17077=CYLINDRICAL_SURFACE('',#19190,1.2645);
#17078=CYLINDRICAL_SURFACE('',#19191,1.2645);
#17079=CYLINDRICAL_SURFACE('',#19192,1.2645);
#17080=CYLINDRICAL_SURFACE('',#19193,1.2645);
#17081=CYLINDRICAL_SURFACE('',#19194,1.2645);
#17082=CYLINDRICAL_SURFACE('',#19196,1.543);
#17083=CYLINDRICAL_SURFACE('',#19198,1.543);
#17084=CYLINDRICAL_SURFACE('',#19199,1.543);
#17085=CYLINDRICAL_SURFACE('',#19200,1.543);
#17086=CYLINDRICAL_SURFACE('',#19201,1.543);
#17087=CYLINDRICAL_SURFACE('',#19202,1.543);
#17088=CYLINDRICAL_SURFACE('',#19203,1.543);
#17089=CYLINDRICAL_SURFACE('',#19204,1.543);
#17090=CYLINDRICAL_SURFACE('',#19206,1.2645);
#17091=CYLINDRICAL_SURFACE('',#19212,1.2645);
#17092=CYLINDRICAL_SURFACE('',#19213,1.2645);
#17093=CYLINDRICAL_SURFACE('',#19214,1.2645);
#17094=CYLINDRICAL_SURFACE('',#19215,1.2645);
#17095=CYLINDRICAL_SURFACE('',#19216,1.2645);
#17096=CYLINDRICAL_SURFACE('',#19217,1.2645);
#17097=CYLINDRICAL_SURFACE('',#19218,1.2645);
#17098=CYLINDRICAL_SURFACE('',#19220,1.54299999999999);
#17099=CYLINDRICAL_SURFACE('',#19222,1.54299999999999);
#17100=CYLINDRICAL_SURFACE('',#19223,1.54299999999999);
#17101=CYLINDRICAL_SURFACE('',#19224,1.54299999999999);
#17102=CYLINDRICAL_SURFACE('',#19225,1.54299999999999);
#17103=CYLINDRICAL_SURFACE('',#19226,1.54299999999999);
#17104=CYLINDRICAL_SURFACE('',#19227,1.54299999999999);
#17105=CYLINDRICAL_SURFACE('',#19228,1.54299999999999);
#17106=CYLINDRICAL_SURFACE('',#19230,1.2645);
#17107=CYLINDRICAL_SURFACE('',#19236,1.2645);
#17108=CYLINDRICAL_SURFACE('',#19237,1.2645);
#17109=CYLINDRICAL_SURFACE('',#19238,1.2645);
#17110=CYLINDRICAL_SURFACE('',#19239,1.2645);
#17111=CYLINDRICAL_SURFACE('',#19240,1.2645);
#17112=CYLINDRICAL_SURFACE('',#19241,1.2645);
#17113=CYLINDRICAL_SURFACE('',#19242,1.2645);
#17114=CYLINDRICAL_SURFACE('',#19244,1.543);
#17115=CYLINDRICAL_SURFACE('',#19246,1.543);
#17116=CYLINDRICAL_SURFACE('',#19247,1.543);
#17117=CYLINDRICAL_SURFACE('',#19248,1.543);
#17118=CYLINDRICAL_SURFACE('',#19249,1.543);
#17119=CYLINDRICAL_SURFACE('',#19250,1.543);
#17120=CYLINDRICAL_SURFACE('',#19251,1.543);
#17121=CYLINDRICAL_SURFACE('',#19252,1.543);
#17122=CYLINDRICAL_SURFACE('',#19272,1.543);
#17123=CYLINDRICAL_SURFACE('',#19273,1.2645);
#17124=CYLINDRICAL_SURFACE('',#19275,1.54299999999999);
#17125=CYLINDRICAL_SURFACE('',#19276,1.2645);
#17126=CYLINDRICAL_SURFACE('',#19278,1.543);
#17127=CYLINDRICAL_SURFACE('',#19279,1.2645);
#17128=CYLINDRICAL_SURFACE('',#19281,1.54300000000001);
#17129=CYLINDRICAL_SURFACE('',#19282,1.2645);
#17130=CYLINDRICAL_SURFACE('',#19284,1.54300000000001);
#17131=CYLINDRICAL_SURFACE('',#19285,1.2645);
#17132=CYLINDRICAL_SURFACE('',#19297,1.543);
#17133=CYLINDRICAL_SURFACE('',#19298,1.2645);
#17134=CYLINDRICAL_SURFACE('',#19300,1.54300000000001);
#17135=CYLINDRICAL_SURFACE('',#19301,1.2645);
#17136=CYLINDRICAL_SURFACE('',#19303,1.54300000000001);
#17137=CYLINDRICAL_SURFACE('',#19304,1.2645);
#17138=CYLINDRICAL_SURFACE('',#19306,1.543);
#17139=CYLINDRICAL_SURFACE('',#19307,1.2645);
#17140=CYLINDRICAL_SURFACE('',#19309,1.543);
#17141=CYLINDRICAL_SURFACE('',#19310,1.2645);
#17142=CYLINDRICAL_SURFACE('',#19322,1.54299999999999);
#17143=CYLINDRICAL_SURFACE('',#19323,1.2645);
#17144=CYLINDRICAL_SURFACE('',#19327,1.543);
#17145=CYLINDRICAL_SURFACE('',#19328,1.2645);
#17146=CYLINDRICAL_SURFACE('',#19331,1.5);
#17147=CYLINDRICAL_SURFACE('',#19334,3.);
#17148=CYLINDRICAL_SURFACE('',#19338,1.5);
#17149=CYLINDRICAL_SURFACE('',#19341,3.);
#17150=CYLINDRICAL_SURFACE('',#19345,1.5);
#17151=CYLINDRICAL_SURFACE('',#19348,3.);
#17152=CYLINDRICAL_SURFACE('',#19352,1.5);
#17153=CYLINDRICAL_SURFACE('',#19355,3.);
#17154=CYLINDRICAL_SURFACE('',#19359,1.5);
#17155=CYLINDRICAL_SURFACE('',#19362,3.);
#17156=CYLINDRICAL_SURFACE('',#19366,1.5);
#17157=CYLINDRICAL_SURFACE('',#19369,3.);
#17158=CYLINDRICAL_SURFACE('',#19397,45.9999999999998);
#17159=CYLINDRICAL_SURFACE('',#19399,1.);
#17160=CYLINDRICAL_SURFACE('',#19402,45.9999999999998);
#17161=CYLINDRICAL_SURFACE('',#19404,1.);
#17162=CYLINDRICAL_SURFACE('',#19407,45.9999999999998);
#17163=CYLINDRICAL_SURFACE('',#19409,1.);
#17164=CYLINDRICAL_SURFACE('',#19421,1.);
#17165=CYLINDRICAL_SURFACE('',#19422,45.9999999999998);
#17166=CYLINDRICAL_SURFACE('',#19424,1.);
#17167=CYLINDRICAL_SURFACE('',#19425,45.9999999999998);
#17168=CYLINDRICAL_SURFACE('',#19427,1.);
#17169=CYLINDRICAL_SURFACE('',#19428,45.9999999999998);
#17170=CYLINDRICAL_SURFACE('',#19429,10.);
#17733=ADVANCED_FACE('',(#1135),#16930,.F.);
#17734=ADVANCED_FACE('',(#1136),#16931,.F.);
#17735=ADVANCED_FACE('',(#1137),#16932,.F.);
#17736=ADVANCED_FACE('',(#1138),#16933,.F.);
#17737=ADVANCED_FACE('',(#1139),#16934,.F.);
#17738=ADVANCED_FACE('',(#1140),#16935,.F.);
#17739=ADVANCED_FACE('',(#1141),#16936,.F.);
#17740=ADVANCED_FACE('',(#1142),#16937,.F.);
#17741=ADVANCED_FACE('',(#1143),#16938,.F.);
#17742=ADVANCED_FACE('',(#1144),#16939,.F.);
#17743=ADVANCED_FACE('',(#1145),#16940,.F.);
#17744=ADVANCED_FACE('',(#1146),#16941,.F.);
#17745=ADVANCED_FACE('',(#1147),#16942,.F.);
#17746=ADVANCED_FACE('',(#1148),#16943,.F.);
#17747=ADVANCED_FACE('',(#1149),#16944,.F.);
#17748=ADVANCED_FACE('',(#1150),#16945,.F.);
#17749=ADVANCED_FACE('',(#1151),#16946,.F.);
#17750=ADVANCED_FACE('',(#1152),#16947,.F.);
#17751=ADVANCED_FACE('',(#1153),#16948,.F.);
#17752=ADVANCED_FACE('',(#1154),#16949,.F.);
#17753=ADVANCED_FACE('',(#1155),#16950,.F.);
#17754=ADVANCED_FACE('',(#1156),#16951,.F.);
#17755=ADVANCED_FACE('',(#1157),#16952,.F.);
#17756=ADVANCED_FACE('',(#1158),#16953,.F.);
#17757=ADVANCED_FACE('',(#1159),#16954,.F.);
#17758=ADVANCED_FACE('',(#1160),#16955,.F.);
#17759=ADVANCED_FACE('',(#1161),#16956,.F.);
#17760=ADVANCED_FACE('',(#1162),#16957,.F.);
#17761=ADVANCED_FACE('',(#1163),#16958,.F.);
#17762=ADVANCED_FACE('',(#1164),#16959,.F.);
#17763=ADVANCED_FACE('',(#1165),#16960,.F.);
#17764=ADVANCED_FACE('',(#1166),#16961,.F.);
#17765=ADVANCED_FACE('',(#1167),#16962,.F.);
#17766=ADVANCED_FACE('',(#1168),#16963,.F.);
#17767=ADVANCED_FACE('',(#1169),#16964,.F.);
#17768=ADVANCED_FACE('',(#1170),#16965,.F.);
#17769=ADVANCED_FACE('',(#1171),#16966,.F.);
#17770=ADVANCED_FACE('',(#1172),#16967,.F.);
#17771=ADVANCED_FACE('',(#1173),#16968,.F.);
#17772=ADVANCED_FACE('',(#1174),#16969,.F.);
#17773=ADVANCED_FACE('',(#1175),#16970,.F.);
#17774=ADVANCED_FACE('',(#1176),#16971,.F.);
#17775=ADVANCED_FACE('',(#1177),#16972,.F.);
#17776=ADVANCED_FACE('',(#1178),#16973,.F.);
#17777=ADVANCED_FACE('',(#1179),#16974,.F.);
#17778=ADVANCED_FACE('',(#1180),#16975,.F.);
#17779=ADVANCED_FACE('',(#1181),#16976,.F.);
#17780=ADVANCED_FACE('',(#1182),#16977,.F.);
#17781=ADVANCED_FACE('',(#1183),#16978,.F.);
#17782=ADVANCED_FACE('',(#1184),#16979,.F.);
#17783=ADVANCED_FACE('',(#1185),#16980,.F.);
#17784=ADVANCED_FACE('',(#1186),#16981,.F.);
#17785=ADVANCED_FACE('',(#1187),#16982,.F.);
#17786=ADVANCED_FACE('',(#1188),#16983,.F.);
#17787=ADVANCED_FACE('',(#1189),#16984,.F.);
#17788=ADVANCED_FACE('',(#1190),#16985,.F.);
#17789=ADVANCED_FACE('',(#1191),#16986,.F.);
#17790=ADVANCED_FACE('',(#1192),#16987,.F.);
#17791=ADVANCED_FACE('',(#1193),#16988,.F.);
#17792=ADVANCED_FACE('',(#1194),#16989,.F.);
#17793=ADVANCED_FACE('',(#1195),#16990,.F.);
#17794=ADVANCED_FACE('',(#1196),#16991,.F.);
#17795=ADVANCED_FACE('',(#1197),#16992,.F.);
#17796=ADVANCED_FACE('',(#1198),#16993,.F.);
#17797=ADVANCED_FACE('',(#1199),#16994,.F.);
#17798=ADVANCED_FACE('',(#1200),#16995,.F.);
#17799=ADVANCED_FACE('',(#1201),#16996,.F.);
#17800=ADVANCED_FACE('',(#1202),#16997,.F.);
#17801=ADVANCED_FACE('',(#1203),#16998,.F.);
#17802=ADVANCED_FACE('',(#1204),#16999,.F.);
#17803=ADVANCED_FACE('',(#1205),#17000,.F.);
#17804=ADVANCED_FACE('',(#1206),#17001,.F.);
#17805=ADVANCED_FACE('',(#1207),#17002,.F.);
#17806=ADVANCED_FACE('',(#1208),#17003,.F.);
#17807=ADVANCED_FACE('',(#1209),#17004,.F.);
#17808=ADVANCED_FACE('',(#1210),#17005,.F.);
#17809=ADVANCED_FACE('',(#1211),#17006,.F.);
#17810=ADVANCED_FACE('',(#1212),#17007,.F.);
#17811=ADVANCED_FACE('',(#1213),#17008,.F.);
#17812=ADVANCED_FACE('',(#1214),#17009,.F.);
#17813=ADVANCED_FACE('',(#1215),#17010,.F.);
#17814=ADVANCED_FACE('',(#1216),#17011,.F.);
#17815=ADVANCED_FACE('',(#1217),#17012,.F.);
#17816=ADVANCED_FACE('',(#1218),#17013,.F.);
#17817=ADVANCED_FACE('',(#1219),#17014,.F.);
#17818=ADVANCED_FACE('',(#1220),#17015,.F.);
#17819=ADVANCED_FACE('',(#1221),#17016,.F.);
#17820=ADVANCED_FACE('',(#1222),#17017,.F.);
#17821=ADVANCED_FACE('',(#1223),#17018,.F.);
#17822=ADVANCED_FACE('',(#1224),#17019,.F.);
#17823=ADVANCED_FACE('',(#1225),#17020,.F.);
#17824=ADVANCED_FACE('',(#1226),#17021,.F.);
#17825=ADVANCED_FACE('',(#1227),#17022,.F.);
#17826=ADVANCED_FACE('',(#1228),#17023,.F.);
#17827=ADVANCED_FACE('',(#1229),#17024,.F.);
#17828=ADVANCED_FACE('',(#1230),#17025,.F.);
#17829=ADVANCED_FACE('',(#1231),#17026,.F.);
#17830=ADVANCED_FACE('',(#1232),#17027,.F.);
#17831=ADVANCED_FACE('',(#1233),#17028,.F.);
#17832=ADVANCED_FACE('',(#1234),#17029,.F.);
#17833=ADVANCED_FACE('',(#1235),#17030,.F.);
#17834=ADVANCED_FACE('',(#1236),#17031,.F.);
#17835=ADVANCED_FACE('',(#1237),#17032,.F.);
#17836=ADVANCED_FACE('',(#1238),#17033,.F.);
#17837=ADVANCED_FACE('',(#1239),#17034,.F.);
#17838=ADVANCED_FACE('',(#1240),#17035,.F.);
#17839=ADVANCED_FACE('',(#1241),#17036,.F.);
#17840=ADVANCED_FACE('',(#1242),#17037,.F.);
#17841=ADVANCED_FACE('',(#1243),#17038,.F.);
#17842=ADVANCED_FACE('',(#1244),#17039,.F.);
#17843=ADVANCED_FACE('',(#1245),#17040,.F.);
#17844=ADVANCED_FACE('',(#1246),#17041,.F.);
#17845=ADVANCED_FACE('',(#1247),#17042,.F.);
#17846=ADVANCED_FACE('',(#1248),#17043,.F.);
#17847=ADVANCED_FACE('',(#1249),#17044,.F.);
#17848=ADVANCED_FACE('',(#1250),#17045,.F.);
#17849=ADVANCED_FACE('',(#1251),#17046,.F.);
#17850=ADVANCED_FACE('',(#1252),#17047,.F.);
#17851=ADVANCED_FACE('',(#1253),#17048,.F.);
#17852=ADVANCED_FACE('',(#1254),#17049,.F.);
#17853=ADVANCED_FACE('',(#1255),#17050,.F.);
#17854=ADVANCED_FACE('',(#1256),#17051,.F.);
#17855=ADVANCED_FACE('',(#1257),#17052,.F.);
#17856=ADVANCED_FACE('',(#1258),#17053,.F.);
#17857=ADVANCED_FACE('',(#1259),#17054,.F.);
#17858=ADVANCED_FACE('',(#1260),#17055,.F.);
#17859=ADVANCED_FACE('',(#1261),#17056,.F.);
#17860=ADVANCED_FACE('',(#1262),#17057,.F.);
#17861=ADVANCED_FACE('',(#1263),#17058,.F.);
#17862=ADVANCED_FACE('',(#1264),#17059,.F.);
#17863=ADVANCED_FACE('',(#1265),#17060,.F.);
#17864=ADVANCED_FACE('',(#1266),#17061,.F.);
#17865=ADVANCED_FACE('',(#1267),#17062,.F.);
#17866=ADVANCED_FACE('',(#1268),#17063,.F.);
#17867=ADVANCED_FACE('',(#1269),#17064,.F.);
#17868=ADVANCED_FACE('',(#1270),#17065,.F.);
#17869=ADVANCED_FACE('',(#1271),#17066,.F.);
#17870=ADVANCED_FACE('',(#1272),#17067,.F.);
#17871=ADVANCED_FACE('',(#1273),#17068,.F.);
#17872=ADVANCED_FACE('',(#1274),#17069,.F.);
#17873=ADVANCED_FACE('',(#1275),#17070,.F.);
#17874=ADVANCED_FACE('',(#1276),#17071,.F.);
#17875=ADVANCED_FACE('',(#1277),#17072,.F.);
#17876=ADVANCED_FACE('',(#1278),#17073,.F.);
#17877=ADVANCED_FACE('',(#1279),#17074,.F.);
#17878=ADVANCED_FACE('',(#1280),#17075,.F.);
#17879=ADVANCED_FACE('',(#1281),#17076,.F.);
#17880=ADVANCED_FACE('',(#1282),#17077,.F.);
#17881=ADVANCED_FACE('',(#1283),#17078,.F.);
#17882=ADVANCED_FACE('',(#1284),#17079,.F.);
#17883=ADVANCED_FACE('',(#1285),#17080,.F.);
#17884=ADVANCED_FACE('',(#1286),#17081,.F.);
#17885=ADVANCED_FACE('',(#1287),#17082,.F.);
#17886=ADVANCED_FACE('',(#1288),#17083,.F.);
#17887=ADVANCED_FACE('',(#1289),#17084,.F.);
#17888=ADVANCED_FACE('',(#1290),#17085,.F.);
#17889=ADVANCED_FACE('',(#1291),#17086,.F.);
#17890=ADVANCED_FACE('',(#1292),#17087,.F.);
#17891=ADVANCED_FACE('',(#1293),#17088,.F.);
#17892=ADVANCED_FACE('',(#1294),#17089,.F.);
#17893=ADVANCED_FACE('',(#1295),#17090,.F.);
#17894=ADVANCED_FACE('',(#1296),#17091,.F.);
#17895=ADVANCED_FACE('',(#1297),#17092,.F.);
#17896=ADVANCED_FACE('',(#1298),#17093,.F.);
#17897=ADVANCED_FACE('',(#1299),#17094,.F.);
#17898=ADVANCED_FACE('',(#1300),#17095,.F.);
#17899=ADVANCED_FACE('',(#1301),#17096,.F.);
#17900=ADVANCED_FACE('',(#1302),#17097,.F.);
#17901=ADVANCED_FACE('',(#1303),#17098,.F.);
#17902=ADVANCED_FACE('',(#1304),#17099,.F.);
#17903=ADVANCED_FACE('',(#1305),#17100,.F.);
#17904=ADVANCED_FACE('',(#1306),#17101,.F.);
#17905=ADVANCED_FACE('',(#1307),#17102,.F.);
#17906=ADVANCED_FACE('',(#1308),#17103,.F.);
#17907=ADVANCED_FACE('',(#1309),#17104,.F.);
#17908=ADVANCED_FACE('',(#1310),#17105,.F.);
#17909=ADVANCED_FACE('',(#1311),#17106,.F.);
#17910=ADVANCED_FACE('',(#1312),#17107,.F.);
#17911=ADVANCED_FACE('',(#1313),#17108,.F.);
#17912=ADVANCED_FACE('',(#1314),#17109,.F.);
#17913=ADVANCED_FACE('',(#1315),#17110,.F.);
#17914=ADVANCED_FACE('',(#1316),#17111,.F.);
#17915=ADVANCED_FACE('',(#1317),#17112,.F.);
#17916=ADVANCED_FACE('',(#1318),#17113,.F.);
#17917=ADVANCED_FACE('',(#1319),#17114,.F.);
#17918=ADVANCED_FACE('',(#1320),#17115,.F.);
#17919=ADVANCED_FACE('',(#1321),#17116,.F.);
#17920=ADVANCED_FACE('',(#1322),#17117,.F.);
#17921=ADVANCED_FACE('',(#1323),#17118,.F.);
#17922=ADVANCED_FACE('',(#1324),#17119,.F.);
#17923=ADVANCED_FACE('',(#1325),#17120,.F.);
#17924=ADVANCED_FACE('',(#1326),#17121,.F.);
#17925=ADVANCED_FACE('',(#1327),#470,.F.);
#17926=ADVANCED_FACE('',(#1328),#471,.F.);
#17927=ADVANCED_FACE('',(#1329),#472,.F.);
#17928=ADVANCED_FACE('',(#1330,#350,#351,#352,#353,#354,#355,#356),#473,
 .F.);
#17929=ADVANCED_FACE('',(#1331),#474,.F.);
#17930=ADVANCED_FACE('',(#1332),#17122,.F.);
#17931=ADVANCED_FACE('',(#1333),#646,.F.);
#17932=ADVANCED_FACE('',(#1334),#647,.F.);
#17933=ADVANCED_FACE('',(#1335),#17123,.F.);
#17934=ADVANCED_FACE('',(#1336),#475,.F.);
#17935=ADVANCED_FACE('',(#1337),#17124,.F.);
#17936=ADVANCED_FACE('',(#1338),#648,.F.);
#17937=ADVANCED_FACE('',(#1339),#649,.F.);
#17938=ADVANCED_FACE('',(#1340),#17125,.F.);
#17939=ADVANCED_FACE('',(#1341),#476,.F.);
#17940=ADVANCED_FACE('',(#1342),#17126,.F.);
#17941=ADVANCED_FACE('',(#1343),#650,.F.);
#17942=ADVANCED_FACE('',(#1344),#651,.F.);
#17943=ADVANCED_FACE('',(#1345),#17127,.F.);
#17944=ADVANCED_FACE('',(#1346),#477,.F.);
#17945=ADVANCED_FACE('',(#1347),#17128,.F.);
#17946=ADVANCED_FACE('',(#1348),#652,.F.);
#17947=ADVANCED_FACE('',(#1349),#653,.F.);
#17948=ADVANCED_FACE('',(#1350),#17129,.F.);
#17949=ADVANCED_FACE('',(#1351),#478,.F.);
#17950=ADVANCED_FACE('',(#1352),#17130,.F.);
#17951=ADVANCED_FACE('',(#1353),#654,.F.);
#17952=ADVANCED_FACE('',(#1354),#655,.F.);
#17953=ADVANCED_FACE('',(#1355),#17131,.F.);
#17954=ADVANCED_FACE('',(#1356),#479,.F.);
#17955=ADVANCED_FACE('',(#1357),#480,.F.);
#17956=ADVANCED_FACE('',(#1358),#481,.F.);
#17957=ADVANCED_FACE('',(#1359),#482,.F.);
#17958=ADVANCED_FACE('',(#1360),#483,.F.);
#17959=ADVANCED_FACE('',(#1361),#484,.F.);
#17960=ADVANCED_FACE('',(#1362),#485,.F.);
#17961=ADVANCED_FACE('',(#1363),#486,.F.);
#17962=ADVANCED_FACE('',(#1364),#487,.F.);
#17963=ADVANCED_FACE('',(#1365),#488,.F.);
#17964=ADVANCED_FACE('',(#1366),#489,.T.);
#17965=ADVANCED_FACE('',(#1367),#17132,.F.);
#17966=ADVANCED_FACE('',(#1368),#656,.F.);
#17967=ADVANCED_FACE('',(#1369),#657,.F.);
#17968=ADVANCED_FACE('',(#1370),#17133,.F.);
#17969=ADVANCED_FACE('',(#1371),#490,.T.);
#17970=ADVANCED_FACE('',(#1372),#17134,.F.);
#17971=ADVANCED_FACE('',(#1373),#658,.F.);
#17972=ADVANCED_FACE('',(#1374),#659,.F.);
#17973=ADVANCED_FACE('',(#1375),#17135,.F.);
#17974=ADVANCED_FACE('',(#1376),#491,.T.);
#17975=ADVANCED_FACE('',(#1377),#17136,.F.);
#17976=ADVANCED_FACE('',(#1378),#660,.F.);
#17977=ADVANCED_FACE('',(#1379),#661,.F.);
#17978=ADVANCED_FACE('',(#1380),#17137,.F.);
#17979=ADVANCED_FACE('',(#1381),#492,.T.);
#17980=ADVANCED_FACE('',(#1382),#17138,.F.);
#17981=ADVANCED_FACE('',(#1383),#662,.F.);
#17982=ADVANCED_FACE('',(#1384),#663,.F.);
#17983=ADVANCED_FACE('',(#1385),#17139,.F.);
#17984=ADVANCED_FACE('',(#1386),#493,.T.);
#17985=ADVANCED_FACE('',(#1387),#17140,.F.);
#17986=ADVANCED_FACE('',(#1388),#664,.F.);
#17987=ADVANCED_FACE('',(#1389),#665,.F.);
#17988=ADVANCED_FACE('',(#1390),#17141,.F.);
#17989=ADVANCED_FACE('',(#1391),#494,.F.);
#17990=ADVANCED_FACE('',(#1392),#495,.F.);
#17991=ADVANCED_FACE('',(#1393),#496,.F.);
#17992=ADVANCED_FACE('',(#1394),#497,.F.);
#17993=ADVANCED_FACE('',(#1395),#498,.F.);
#17994=ADVANCED_FACE('',(#1396),#499,.F.);
#17995=ADVANCED_FACE('',(#1397),#500,.F.);
#17996=ADVANCED_FACE('',(#1398),#501,.F.);
#17997=ADVANCED_FACE('',(#1399),#502,.F.);
#17998=ADVANCED_FACE('',(#1400),#503,.F.);
#17999=ADVANCED_FACE('',(#1401),#504,.F.);
#18000=ADVANCED_FACE('',(#1402),#17142,.F.);
#18001=ADVANCED_FACE('',(#1403),#666,.F.);
#18002=ADVANCED_FACE('',(#1404),#667,.F.);
#18003=ADVANCED_FACE('',(#1405),#17143,.F.);
#18004=ADVANCED_FACE('',(#1406),#505,.F.);
#18005=ADVANCED_FACE('',(#1407),#506,.F.);
#18006=ADVANCED_FACE('',(#1408),#507,.T.);
#18007=ADVANCED_FACE('',(#1409),#17144,.F.);
#18008=ADVANCED_FACE('',(#1410),#668,.F.);
#18009=ADVANCED_FACE('',(#1411),#669,.F.);
#18010=ADVANCED_FACE('',(#1412),#17145,.F.);
#18011=ADVANCED_FACE('',(#1413),#508,.F.);
#18012=ADVANCED_FACE('',(#1414),#509,.F.);
#18013=ADVANCED_FACE('',(#1415),#17146,.F.);
#18014=ADVANCED_FACE('',(#1416,#357),#17147,.F.);
#18015=ADVANCED_FACE('',(#1417,#358),#510,.F.);
#18016=ADVANCED_FACE('',(#1418),#17148,.F.);
#18017=ADVANCED_FACE('',(#1419,#359),#17149,.F.);
#18018=ADVANCED_FACE('',(#1420,#360),#511,.F.);
#18019=ADVANCED_FACE('',(#1421),#17150,.F.);
#18020=ADVANCED_FACE('',(#1422,#361),#17151,.F.);
#18021=ADVANCED_FACE('',(#1423,#362),#512,.F.);
#18022=ADVANCED_FACE('',(#1424),#17152,.F.);
#18023=ADVANCED_FACE('',(#1425,#363),#17153,.F.);
#18024=ADVANCED_FACE('',(#1426,#364),#513,.F.);
#18025=ADVANCED_FACE('',(#1427),#17154,.F.);
#18026=ADVANCED_FACE('',(#1428,#365),#17155,.F.);
#18027=ADVANCED_FACE('',(#1429,#366),#514,.F.);
#18028=ADVANCED_FACE('',(#1430),#17156,.F.);
#18029=ADVANCED_FACE('',(#1431,#367),#17157,.F.);
#18030=ADVANCED_FACE('',(#1432,#368),#515,.F.);
#18031=ADVANCED_FACE('',(#1433),#516,.T.);
#18032=ADVANCED_FACE('',(#1434,#369),#517,.T.);
#18033=ADVANCED_FACE('',(#1435),#518,.T.);
#18034=ADVANCED_FACE('',(#1436,#370),#519,.T.);
#18035=ADVANCED_FACE('',(#1437,#371),#520,.T.);
#18036=ADVANCED_FACE('',(#1438),#521,.T.);
#18037=ADVANCED_FACE('',(#1439,#372),#522,.T.);
#18038=ADVANCED_FACE('',(#1440),#523,.T.);
#18039=ADVANCED_FACE('',(#1441,#373),#524,.T.);
#18040=ADVANCED_FACE('',(#1442),#525,.T.);
#18041=ADVANCED_FACE('',(#1443,#374),#526,.T.);
#18042=ADVANCED_FACE('',(#1444),#527,.T.);
#18043=ADVANCED_FACE('',(#1445,#375),#528,.T.);
#18044=ADVANCED_FACE('',(#1446),#529,.T.);
#18045=ADVANCED_FACE('',(#1447,#376),#530,.T.);
#18046=ADVANCED_FACE('',(#1448),#531,.T.);
#18047=ADVANCED_FACE('',(#1449),#532,.T.);
#18048=ADVANCED_FACE('',(#1450,#377),#533,.T.);
#18049=ADVANCED_FACE('',(#1451),#534,.T.);
#18050=ADVANCED_FACE('',(#1452,#378),#535,.T.);
#18051=ADVANCED_FACE('',(#1453),#256,.F.);
#18052=ADVANCED_FACE('',(#1454),#257,.F.);
#18053=ADVANCED_FACE('',(#1455),#258,.F.);
#18054=ADVANCED_FACE('',(#1456),#259,.F.);
#18055=ADVANCED_FACE('',(#1457),#260,.F.);
#18056=ADVANCED_FACE('',(#1458),#261,.F.);
#18057=ADVANCED_FACE('',(#1459),#262,.F.);
#18058=ADVANCED_FACE('',(#1460),#263,.F.);
#18059=ADVANCED_FACE('',(#1461),#536,.T.);
#18060=ADVANCED_FACE('',(#1462,#379),#537,.T.);
#18061=ADVANCED_FACE('',(#1463),#538,.T.);
#18062=ADVANCED_FACE('',(#1464,#380),#539,.T.);
#18063=ADVANCED_FACE('',(#1465),#264,.F.);
#18064=ADVANCED_FACE('',(#1466),#17158,.T.);
#18065=ADVANCED_FACE('',(#1467),#17159,.F.);
#18066=ADVANCED_FACE('',(#1468),#540,.F.);
#18067=ADVANCED_FACE('',(#1469),#17160,.T.);
#18068=ADVANCED_FACE('',(#1470),#17161,.F.);
#18069=ADVANCED_FACE('',(#1471),#541,.F.);
#18070=ADVANCED_FACE('',(#1472),#17162,.T.);
#18071=ADVANCED_FACE('',(#1473),#17163,.F.);
#18072=ADVANCED_FACE('',(#1474),#542,.F.);
#18073=ADVANCED_FACE('',(#1475,#381,#382,#383,#384,#385,#386,#387),#543,
 .F.);
#18074=ADVANCED_FACE('',(#1476),#544,.F.);
#18075=ADVANCED_FACE('',(#1477),#17164,.F.);
#18076=ADVANCED_FACE('',(#1478),#17165,.T.);
#18077=ADVANCED_FACE('',(#1479),#265,.F.);
#18078=ADVANCED_FACE('',(#1480),#545,.F.);
#18079=ADVANCED_FACE('',(#1481),#17166,.F.);
#18080=ADVANCED_FACE('',(#1482),#17167,.T.);
#18081=ADVANCED_FACE('',(#1483),#266,.F.);
#18082=ADVANCED_FACE('',(#1484),#546,.F.);
#18083=ADVANCED_FACE('',(#1485),#267,.F.);
#18084=ADVANCED_FACE('',(#1486),#17168,.F.);
#18085=ADVANCED_FACE('',(#1487),#17169,.T.);
#18086=ADVANCED_FACE('',(#1488),#17170,.F.);
#18271=CLOSED_SHELL('',(#17733,#17734,#17735,#17736,#17737,#17738,#17739,
#17740,#17741,#17742,#17743,#17744,#17745,#17746,#17747,#17748,#17749,#17750,
#17751,#17752,#17753,#17754,#17755,#17756,#17757,#17758,#17759,#17760,#17761,
#17762,#17763,#17764,#17765,#17766,#17767,#17768,#17769,#17770,#17771,#17772,
#17773,#17774,#17775,#17776,#17777,#17778,#17779,#17780,#17781,#17782,#17783,
#17784,#17785,#17786,#17787,#17788,#17789,#17790,#17791,#17792,#17793,#17794,
#17795,#17796,#17797,#17798,#17799,#17800,#17801,#17802,#17803,#17804,#17805,
#17806,#17807,#17808,#17809,#17810,#17811,#17812,#17813,#17814,#17815,#17816,
#17817,#17818,#17819,#17820,#17821,#17822,#17823,#17824,#17825,#17826,#17827,
#17828,#17829,#17830,#17831,#17832,#17833,#17834,#17835,#17836,#17837,#17838,
#17839,#17840,#17841,#17842,#17843,#17844,#17845,#17846,#17847,#17848,#17849,
#17850,#17851,#17852,#17853,#17854,#17855,#17856,#17857,#17858,#17859,#17860,
#17861,#17862,#17863,#17864,#17865,#17866,#17867,#17868,#17869,#17870,#17871,
#17872,#17873,#17874,#17875,#17876,#17877,#17878,#17879,#17880,#17881,#17882,
#17883,#17884,#17885,#17886,#17887,#17888,#17889,#17890,#17891,#17892,#17893,
#17894,#17895,#17896,#17897,#17898,#17899,#17900,#17901,#17902,#17903,#17904,
#17905,#17906,#17907,#17908,#17909,#17910,#17911,#17912,#17913,#17914,#17915,
#17916,#17917,#17918,#17919,#17920,#17921,#17922,#17923,#17924,#17925,#17926,
#17927,#17928,#17929,#17930,#17931,#17932,#17933,#17934,#17935,#17936,#17937,
#17938,#17939,#17940,#17941,#17942,#17943,#17944,#17945,#17946,#17947,#17948,
#17949,#17950,#17951,#17952,#17953,#17954,#17955,#17956,#17957,#17958,#17959,
#17960,#17961,#17962,#17963,#17964,#17965,#17966,#17967,#17968,#17969,#17970,
#17971,#17972,#17973,#17974,#17975,#17976,#17977,#17978,#17979,#17980,#17981,
#17982,#17983,#17984,#17985,#17986,#17987,#17988,#17989,#17990,#17991,#17992,
#17993,#17994,#17995,#17996,#17997,#17998,#17999,#18000,#18001,#18002,#18003,
#18004,#18005,#18006,#18007,#18008,#18009,#18010,#18011,#18012,#18013,#18014,
#18015,#18016,#18017,#18018,#18019,#18020,#18021,#18022,#18023,#18024,#18025,
#18026,#18027,#18028,#18029,#18030,#18031,#18032,#18033,#18034,#18035,#18036,
#18037,#18038,#18039,#18040,#18041,#18042,#18043,#18044,#18045,#18046,#18047,
#18048,#18049,#18050,#18051,#18052,#18053,#18054,#18055,#18056,#18057,#18058,
#18059,#18060,#18061,#18062,#18063,#18064,#18065,#18066,#18067,#18068,#18069,
#18070,#18071,#18072,#18073,#18074,#18075,#18076,#18077,#18078,#18079,#18080,
#18081,#18082,#18083,#18084,#18085,#18086));
#18965=AXIS2_PLACEMENT_3D('',#52671,#21181,#21182);
#18966=AXIS2_PLACEMENT_3D('',#52672,#21183,#21184);
#18967=AXIS2_PLACEMENT_3D('',#52682,#21186,#21187);
#18968=AXIS2_PLACEMENT_3D('',#52686,#21189,#21190);
#18969=AXIS2_PLACEMENT_3D('',#52688,#21191,#21192);
#18970=AXIS2_PLACEMENT_3D('',#52689,#21193,#21194);
#18971=AXIS2_PLACEMENT_3D('',#52691,#21195,#21196);
#18972=AXIS2_PLACEMENT_3D('',#52702,#21197,#21198);
#18973=AXIS2_PLACEMENT_3D('',#52753,#21200,#21201);
#18974=AXIS2_PLACEMENT_3D('',#52804,#21203,#21204);
#18975=AXIS2_PLACEMENT_3D('',#52852,#21206,#21207);
#18976=AXIS2_PLACEMENT_3D('',#52903,#21209,#21210);
#18977=AXIS2_PLACEMENT_3D('',#52954,#21212,#21213);
#18978=AXIS2_PLACEMENT_3D('',#53002,#21215,#21216);
#18979=AXIS2_PLACEMENT_3D('',#53021,#21218,#21219);
#18980=AXIS2_PLACEMENT_3D('',#53041,#21220,#21221);
#18981=AXIS2_PLACEMENT_3D('',#53055,#21223,#21224);
#18982=AXIS2_PLACEMENT_3D('',#53065,#21225,#21226);
#18983=AXIS2_PLACEMENT_3D('',#53089,#21228,#21229);
#18984=AXIS2_PLACEMENT_3D('',#53114,#21231,#21232);
#18985=AXIS2_PLACEMENT_3D('',#53139,#21234,#21235);
#18986=AXIS2_PLACEMENT_3D('',#53163,#21237,#21238);
#18987=AXIS2_PLACEMENT_3D('',#53188,#21240,#21241);
#18988=AXIS2_PLACEMENT_3D('',#53213,#21243,#21244);
#18989=AXIS2_PLACEMENT_3D('',#53224,#21246,#21247);
#18990=AXIS2_PLACEMENT_3D('',#53230,#21248,#21249);
#18991=AXIS2_PLACEMENT_3D('',#53240,#21251,#21252);
#18992=AXIS2_PLACEMENT_3D('',#53244,#21254,#21255);
#18993=AXIS2_PLACEMENT_3D('',#53246,#21256,#21257);
#18994=AXIS2_PLACEMENT_3D('',#53247,#21258,#21259);
#18995=AXIS2_PLACEMENT_3D('',#53249,#21260,#21261);
#18996=AXIS2_PLACEMENT_3D('',#53260,#21262,#21263);
#18997=AXIS2_PLACEMENT_3D('',#53311,#21265,#21266);
#18998=AXIS2_PLACEMENT_3D('',#53362,#21268,#21269);
#18999=AXIS2_PLACEMENT_3D('',#53410,#21271,#21272);
#19000=AXIS2_PLACEMENT_3D('',#53461,#21274,#21275);
#19001=AXIS2_PLACEMENT_3D('',#53512,#21277,#21278);
#19002=AXIS2_PLACEMENT_3D('',#53560,#21280,#21281);
#19003=AXIS2_PLACEMENT_3D('',#53579,#21283,#21284);
#19004=AXIS2_PLACEMENT_3D('',#53599,#21285,#21286);
#19005=AXIS2_PLACEMENT_3D('',#53613,#21288,#21289);
#19006=AXIS2_PLACEMENT_3D('',#53623,#21290,#21291);
#19007=AXIS2_PLACEMENT_3D('',#53647,#21293,#21294);
#19008=AXIS2_PLACEMENT_3D('',#53672,#21296,#21297);
#19009=AXIS2_PLACEMENT_3D('',#53697,#21299,#21300);
#19010=AXIS2_PLACEMENT_3D('',#53721,#21302,#21303);
#19011=AXIS2_PLACEMENT_3D('',#53746,#21305,#21306);
#19012=AXIS2_PLACEMENT_3D('',#53771,#21308,#21309);
#19013=AXIS2_PLACEMENT_3D('',#53782,#21311,#21312);
#19014=AXIS2_PLACEMENT_3D('',#53788,#21313,#21314);
#19015=AXIS2_PLACEMENT_3D('',#53798,#21316,#21317);
#19016=AXIS2_PLACEMENT_3D('',#53802,#21319,#21320);
#19017=AXIS2_PLACEMENT_3D('',#53804,#21321,#21322);
#19018=AXIS2_PLACEMENT_3D('',#53805,#21323,#21324);
#19019=AXIS2_PLACEMENT_3D('',#53807,#21325,#21326);
#19020=AXIS2_PLACEMENT_3D('',#53818,#21327,#21328);
#19021=AXIS2_PLACEMENT_3D('',#53869,#21330,#21331);
#19022=AXIS2_PLACEMENT_3D('',#53920,#21333,#21334);
#19023=AXIS2_PLACEMENT_3D('',#53968,#21336,#21337);
#19024=AXIS2_PLACEMENT_3D('',#54019,#21339,#21340);
#19025=AXIS2_PLACEMENT_3D('',#54070,#21342,#21343);
#19026=AXIS2_PLACEMENT_3D('',#54118,#21345,#21346);
#19027=AXIS2_PLACEMENT_3D('',#54137,#21348,#21349);
#19028=AXIS2_PLACEMENT_3D('',#54157,#21350,#21351);
#19029=AXIS2_PLACEMENT_3D('',#54171,#21353,#21354);
#19030=AXIS2_PLACEMENT_3D('',#54181,#21355,#21356);
#19031=AXIS2_PLACEMENT_3D('',#54205,#21358,#21359);
#19032=AXIS2_PLACEMENT_3D('',#54230,#21361,#21362);
#19033=AXIS2_PLACEMENT_3D('',#54255,#21364,#21365);
#19034=AXIS2_PLACEMENT_3D('',#54279,#21367,#21368);
#19035=AXIS2_PLACEMENT_3D('',#54304,#21370,#21371);
#19036=AXIS2_PLACEMENT_3D('',#54329,#21373,#21374);
#19037=AXIS2_PLACEMENT_3D('',#54340,#21376,#21377);
#19038=AXIS2_PLACEMENT_3D('',#54346,#21378,#21379);
#19039=AXIS2_PLACEMENT_3D('',#54356,#21381,#21382);
#19040=AXIS2_PLACEMENT_3D('',#54360,#21384,#21385);
#19041=AXIS2_PLACEMENT_3D('',#54362,#21386,#21387);
#19042=AXIS2_PLACEMENT_3D('',#54363,#21388,#21389);
#19043=AXIS2_PLACEMENT_3D('',#54365,#21390,#21391);
#19044=AXIS2_PLACEMENT_3D('',#54376,#21392,#21393);
#19045=AXIS2_PLACEMENT_3D('',#54427,#21395,#21396);
#19046=AXIS2_PLACEMENT_3D('',#54478,#21398,#21399);
#19047=AXIS2_PLACEMENT_3D('',#54526,#21401,#21402);
#19048=AXIS2_PLACEMENT_3D('',#54577,#21404,#21405);
#19049=AXIS2_PLACEMENT_3D('',#54628,#21407,#21408);
#19050=AXIS2_PLACEMENT_3D('',#54676,#21410,#21411);
#19051=AXIS2_PLACEMENT_3D('',#54695,#21413,#21414);
#19052=AXIS2_PLACEMENT_3D('',#54715,#21415,#21416);
#19053=AXIS2_PLACEMENT_3D('',#54729,#21418,#21419);
#19054=AXIS2_PLACEMENT_3D('',#54739,#21420,#21421);
#19055=AXIS2_PLACEMENT_3D('',#54763,#21423,#21424);
#19056=AXIS2_PLACEMENT_3D('',#54788,#21426,#21427);
#19057=AXIS2_PLACEMENT_3D('',#54813,#21429,#21430);
#19058=AXIS2_PLACEMENT_3D('',#54837,#21432,#21433);
#19059=AXIS2_PLACEMENT_3D('',#54862,#21435,#21436);
#19060=AXIS2_PLACEMENT_3D('',#54887,#21438,#21439);
#19061=AXIS2_PLACEMENT_3D('',#54898,#21441,#21442);
#19062=AXIS2_PLACEMENT_3D('',#54904,#21443,#21444);
#19063=AXIS2_PLACEMENT_3D('',#54914,#21446,#21447);
#19064=AXIS2_PLACEMENT_3D('',#54918,#21449,#21450);
#19065=AXIS2_PLACEMENT_3D('',#54920,#21451,#21452);
#19066=AXIS2_PLACEMENT_3D('',#54921,#21453,#21454);
#19067=AXIS2_PLACEMENT_3D('',#54923,#21455,#21456);
#19068=AXIS2_PLACEMENT_3D('',#54934,#21457,#21458);
#19069=AXIS2_PLACEMENT_3D('',#54985,#21460,#21461);
#19070=AXIS2_PLACEMENT_3D('',#55036,#21463,#21464);
#19071=AXIS2_PLACEMENT_3D('',#55084,#21466,#21467);
#19072=AXIS2_PLACEMENT_3D('',#55135,#21469,#21470);
#19073=AXIS2_PLACEMENT_3D('',#55186,#21472,#21473);
#19074=AXIS2_PLACEMENT_3D('',#55234,#21475,#21476);
#19075=AXIS2_PLACEMENT_3D('',#55253,#21478,#21479);
#19076=AXIS2_PLACEMENT_3D('',#55273,#21480,#21481);
#19077=AXIS2_PLACEMENT_3D('',#55287,#21483,#21484);
#19078=AXIS2_PLACEMENT_3D('',#55297,#21485,#21486);
#19079=AXIS2_PLACEMENT_3D('',#55321,#21488,#21489);
#19080=AXIS2_PLACEMENT_3D('',#55346,#21491,#21492);
#19081=AXIS2_PLACEMENT_3D('',#55371,#21494,#21495);
#19082=AXIS2_PLACEMENT_3D('',#55395,#21497,#21498);
#19083=AXIS2_PLACEMENT_3D('',#55420,#21500,#21501);
#19084=AXIS2_PLACEMENT_3D('',#55445,#21503,#21504);
#19085=AXIS2_PLACEMENT_3D('',#55456,#21506,#21507);
#19086=AXIS2_PLACEMENT_3D('',#55462,#21508,#21509);
#19087=AXIS2_PLACEMENT_3D('',#55472,#21511,#21512);
#19088=AXIS2_PLACEMENT_3D('',#55476,#21514,#21515);
#19089=AXIS2_PLACEMENT_3D('',#55478,#21516,#21517);
#19090=AXIS2_PLACEMENT_3D('',#55479,#21518,#21519);
#19091=AXIS2_PLACEMENT_3D('',#55481,#21520,#21521);
#19092=AXIS2_PLACEMENT_3D('',#55492,#21522,#21523);
#19093=AXIS2_PLACEMENT_3D('',#55543,#21525,#21526);
#19094=AXIS2_PLACEMENT_3D('',#55594,#21528,#21529);
#19095=AXIS2_PLACEMENT_3D('',#55642,#21531,#21532);
#19096=AXIS2_PLACEMENT_3D('',#55693,#21534,#21535);
#19097=AXIS2_PLACEMENT_3D('',#55744,#21537,#21538);
#19098=AXIS2_PLACEMENT_3D('',#55792,#21540,#21541);
#19099=AXIS2_PLACEMENT_3D('',#55811,#21543,#21544);
#19100=AXIS2_PLACEMENT_3D('',#55831,#21545,#21546);
#19101=AXIS2_PLACEMENT_3D('',#55845,#21548,#21549);
#19102=AXIS2_PLACEMENT_3D('',#55855,#21550,#21551);
#19103=AXIS2_PLACEMENT_3D('',#55879,#21553,#21554);
#19104=AXIS2_PLACEMENT_3D('',#55904,#21556,#21557);
#19105=AXIS2_PLACEMENT_3D('',#55929,#21559,#21560);
#19106=AXIS2_PLACEMENT_3D('',#55953,#21562,#21563);
#19107=AXIS2_PLACEMENT_3D('',#55978,#21565,#21566);
#19108=AXIS2_PLACEMENT_3D('',#56003,#21568,#21569);
#19109=AXIS2_PLACEMENT_3D('',#56014,#21571,#21572);
#19110=AXIS2_PLACEMENT_3D('',#56020,#21573,#21574);
#19111=AXIS2_PLACEMENT_3D('',#56030,#21576,#21577);
#19112=AXIS2_PLACEMENT_3D('',#56034,#21579,#21580);
#19113=AXIS2_PLACEMENT_3D('',#56036,#21581,#21582);
#19114=AXIS2_PLACEMENT_3D('',#56037,#21583,#21584);
#19115=AXIS2_PLACEMENT_3D('',#56039,#21585,#21586);
#19116=AXIS2_PLACEMENT_3D('',#56050,#21587,#21588);
#19117=AXIS2_PLACEMENT_3D('',#56101,#21590,#21591);
#19118=AXIS2_PLACEMENT_3D('',#56152,#21593,#21594);
#19119=AXIS2_PLACEMENT_3D('',#56200,#21596,#21597);
#19120=AXIS2_PLACEMENT_3D('',#56251,#21599,#21600);
#19121=AXIS2_PLACEMENT_3D('',#56302,#21602,#21603);
#19122=AXIS2_PLACEMENT_3D('',#56350,#21605,#21606);
#19123=AXIS2_PLACEMENT_3D('',#56369,#21608,#21609);
#19124=AXIS2_PLACEMENT_3D('',#56389,#21610,#21611);
#19125=AXIS2_PLACEMENT_3D('',#56403,#21613,#21614);
#19126=AXIS2_PLACEMENT_3D('',#56413,#21615,#21616);
#19127=AXIS2_PLACEMENT_3D('',#56437,#21618,#21619);
#19128=AXIS2_PLACEMENT_3D('',#56462,#21621,#21622);
#19129=AXIS2_PLACEMENT_3D('',#56487,#21624,#21625);
#19130=AXIS2_PLACEMENT_3D('',#56511,#21627,#21628);
#19131=AXIS2_PLACEMENT_3D('',#56536,#21630,#21631);
#19132=AXIS2_PLACEMENT_3D('',#56561,#21633,#21634);
#19133=AXIS2_PLACEMENT_3D('',#56572,#21636,#21637);
#19134=AXIS2_PLACEMENT_3D('',#56578,#21638,#21639);
#19135=AXIS2_PLACEMENT_3D('',#56588,#21641,#21642);
#19136=AXIS2_PLACEMENT_3D('',#56592,#21644,#21645);
#19137=AXIS2_PLACEMENT_3D('',#56594,#21646,#21647);
#19138=AXIS2_PLACEMENT_3D('',#56595,#21648,#21649);
#19139=AXIS2_PLACEMENT_3D('',#56597,#21650,#21651);
#19140=AXIS2_PLACEMENT_3D('',#56608,#21652,#21653);
#19141=AXIS2_PLACEMENT_3D('',#56659,#21655,#21656);
#19142=AXIS2_PLACEMENT_3D('',#56710,#21658,#21659);
#19143=AXIS2_PLACEMENT_3D('',#56758,#21661,#21662);
#19144=AXIS2_PLACEMENT_3D('',#56809,#21664,#21665);
#19145=AXIS2_PLACEMENT_3D('',#56860,#21667,#21668);
#19146=AXIS2_PLACEMENT_3D('',#56908,#21670,#21671);
#19147=AXIS2_PLACEMENT_3D('',#56927,#21673,#21674);
#19148=AXIS2_PLACEMENT_3D('',#56947,#21675,#21676);
#19149=AXIS2_PLACEMENT_3D('',#56961,#21678,#21679);
#19150=AXIS2_PLACEMENT_3D('',#56971,#21680,#21681);
#19151=AXIS2_PLACEMENT_3D('',#56995,#21683,#21684);
#19152=AXIS2_PLACEMENT_3D('',#57020,#21686,#21687);
#19153=AXIS2_PLACEMENT_3D('',#57045,#21689,#21690);
#19154=AXIS2_PLACEMENT_3D('',#57069,#21692,#21693);
#19155=AXIS2_PLACEMENT_3D('',#57094,#21695,#21696);
#19156=AXIS2_PLACEMENT_3D('',#57119,#21698,#21699);
#19157=AXIS2_PLACEMENT_3D('',#57130,#21701,#21702);
#19158=AXIS2_PLACEMENT_3D('',#57136,#21703,#21704);
#19159=AXIS2_PLACEMENT_3D('',#57146,#21706,#21707);
#19160=AXIS2_PLACEMENT_3D('',#57150,#21709,#21710);
#19161=AXIS2_PLACEMENT_3D('',#57152,#21711,#21712);
#19162=AXIS2_PLACEMENT_3D('',#57153,#21713,#21714);
#19163=AXIS2_PLACEMENT_3D('',#57155,#21715,#21716);
#19164=AXIS2_PLACEMENT_3D('',#57166,#21717,#21718);
#19165=AXIS2_PLACEMENT_3D('',#57217,#21720,#21721);
#19166=AXIS2_PLACEMENT_3D('',#57268,#21723,#21724);
#19167=AXIS2_PLACEMENT_3D('',#57316,#21726,#21727);
#19168=AXIS2_PLACEMENT_3D('',#57367,#21729,#21730);
#19169=AXIS2_PLACEMENT_3D('',#57418,#21732,#21733);
#19170=AXIS2_PLACEMENT_3D('',#57466,#21735,#21736);
#19171=AXIS2_PLACEMENT_3D('',#57485,#21738,#21739);
#19172=AXIS2_PLACEMENT_3D('',#57505,#21740,#21741);
#19173=AXIS2_PLACEMENT_3D('',#57519,#21743,#21744);
#19174=AXIS2_PLACEMENT_3D('',#57529,#21745,#21746);
#19175=AXIS2_PLACEMENT_3D('',#57553,#21748,#21749);
#19176=AXIS2_PLACEMENT_3D('',#57578,#21751,#21752);
#19177=AXIS2_PLACEMENT_3D('',#57603,#21754,#21755);
#19178=AXIS2_PLACEMENT_3D('',#57627,#21757,#21758);
#19179=AXIS2_PLACEMENT_3D('',#57652,#21760,#21761);
#19180=AXIS2_PLACEMENT_3D('',#57677,#21763,#21764);
#19181=AXIS2_PLACEMENT_3D('',#57688,#21766,#21767);
#19182=AXIS2_PLACEMENT_3D('',#57694,#21768,#21769);
#19183=AXIS2_PLACEMENT_3D('',#57704,#21771,#21772);
#19184=AXIS2_PLACEMENT_3D('',#57708,#21774,#21775);
#19185=AXIS2_PLACEMENT_3D('',#57710,#21776,#21777);
#19186=AXIS2_PLACEMENT_3D('',#57711,#21778,#21779);
#19187=AXIS2_PLACEMENT_3D('',#57713,#21780,#21781);
#19188=AXIS2_PLACEMENT_3D('',#57724,#21782,#21783);
#19189=AXIS2_PLACEMENT_3D('',#57775,#21785,#21786);
#19190=AXIS2_PLACEMENT_3D('',#57826,#21788,#21789);
#19191=AXIS2_PLACEMENT_3D('',#57874,#21791,#21792);
#19192=AXIS2_PLACEMENT_3D('',#57925,#21794,#21795);
#19193=AXIS2_PLACEMENT_3D('',#57976,#21797,#21798);
#19194=AXIS2_PLACEMENT_3D('',#58024,#21800,#21801);
#19195=AXIS2_PLACEMENT_3D('',#58043,#21803,#21804);
#19196=AXIS2_PLACEMENT_3D('',#58063,#21805,#21806);
#19197=AXIS2_PLACEMENT_3D('',#58077,#21808,#21809);
#19198=AXIS2_PLACEMENT_3D('',#58087,#21810,#21811);
#19199=AXIS2_PLACEMENT_3D('',#58111,#21813,#21814);
#19200=AXIS2_PLACEMENT_3D('',#58136,#21816,#21817);
#19201=AXIS2_PLACEMENT_3D('',#58161,#21819,#21820);
#19202=AXIS2_PLACEMENT_3D('',#58185,#21822,#21823);
#19203=AXIS2_PLACEMENT_3D('',#58210,#21825,#21826);
#19204=AXIS2_PLACEMENT_3D('',#58235,#21828,#21829);
#19205=AXIS2_PLACEMENT_3D('',#58246,#21831,#21832);
#19206=AXIS2_PLACEMENT_3D('',#58252,#21833,#21834);
#19207=AXIS2_PLACEMENT_3D('',#58262,#21836,#21837);
#19208=AXIS2_PLACEMENT_3D('',#58266,#21839,#21840);
#19209=AXIS2_PLACEMENT_3D('',#58268,#21841,#21842);
#19210=AXIS2_PLACEMENT_3D('',#58269,#21843,#21844);
#19211=AXIS2_PLACEMENT_3D('',#58271,#21845,#21846);
#19212=AXIS2_PLACEMENT_3D('',#58282,#21847,#21848);
#19213=AXIS2_PLACEMENT_3D('',#58333,#21850,#21851);
#19214=AXIS2_PLACEMENT_3D('',#58384,#21853,#21854);
#19215=AXIS2_PLACEMENT_3D('',#58432,#21856,#21857);
#19216=AXIS2_PLACEMENT_3D('',#58483,#21859,#21860);
#19217=AXIS2_PLACEMENT_3D('',#58534,#21862,#21863);
#19218=AXIS2_PLACEMENT_3D('',#58582,#21865,#21866);
#19219=AXIS2_PLACEMENT_3D('',#58601,#21868,#21869);
#19220=AXIS2_PLACEMENT_3D('',#58621,#21870,#21871);
#19221=AXIS2_PLACEMENT_3D('',#58635,#21873,#21874);
#19222=AXIS2_PLACEMENT_3D('',#58645,#21875,#21876);
#19223=AXIS2_PLACEMENT_3D('',#58669,#21878,#21879);
#19224=AXIS2_PLACEMENT_3D('',#58694,#21881,#21882);
#19225=AXIS2_PLACEMENT_3D('',#58719,#21884,#21885);
#19226=AXIS2_PLACEMENT_3D('',#58743,#21887,#21888);
#19227=AXIS2_PLACEMENT_3D('',#58768,#21890,#21891);
#19228=AXIS2_PLACEMENT_3D('',#58793,#21893,#21894);
#19229=AXIS2_PLACEMENT_3D('',#58804,#21896,#21897);
#19230=AXIS2_PLACEMENT_3D('',#58810,#21898,#21899);
#19231=AXIS2_PLACEMENT_3D('',#58820,#21901,#21902);
#19232=AXIS2_PLACEMENT_3D('',#58824,#21904,#21905);
#19233=AXIS2_PLACEMENT_3D('',#58826,#21906,#21907);
#19234=AXIS2_PLACEMENT_3D('',#58827,#21908,#21909);
#19235=AXIS2_PLACEMENT_3D('',#58829,#21910,#21911);
#19236=AXIS2_PLACEMENT_3D('',#58840,#21912,#21913);
#19237=AXIS2_PLACEMENT_3D('',#58891,#21915,#21916);
#19238=AXIS2_PLACEMENT_3D('',#58942,#21918,#21919);
#19239=AXIS2_PLACEMENT_3D('',#58990,#21921,#21922);
#19240=AXIS2_PLACEMENT_3D('',#59041,#21924,#21925);
#19241=AXIS2_PLACEMENT_3D('',#59092,#21927,#21928);
#19242=AXIS2_PLACEMENT_3D('',#59140,#21930,#21931);
#19243=AXIS2_PLACEMENT_3D('',#59159,#21933,#21934);
#19244=AXIS2_PLACEMENT_3D('',#59179,#21935,#21936);
#19245=AXIS2_PLACEMENT_3D('',#59193,#21938,#21939);
#19246=AXIS2_PLACEMENT_3D('',#59203,#21940,#21941);
#19247=AXIS2_PLACEMENT_3D('',#59227,#21943,#21944);
#19248=AXIS2_PLACEMENT_3D('',#59252,#21946,#21947);
#19249=AXIS2_PLACEMENT_3D('',#59277,#21949,#21950);
#19250=AXIS2_PLACEMENT_3D('',#59301,#21952,#21953);
#19251=AXIS2_PLACEMENT_3D('',#59326,#21955,#21956);
#19252=AXIS2_PLACEMENT_3D('',#59351,#21958,#21959);
#19253=AXIS2_PLACEMENT_3D('',#59362,#21961,#21962);
#19254=AXIS2_PLACEMENT_3D('',#59368,#21963,#21964);
#19255=AXIS2_PLACEMENT_3D('',#59377,#21969,#21970);
#19256=AXIS2_PLACEMENT_3D('',#59383,#21974,#21975);
#19257=AXIS2_PLACEMENT_3D('',#59389,#21979,#21980);
#19258=AXIS2_PLACEMENT_3D('',#59423,#21982,#21983);
#19259=AXIS2_PLACEMENT_3D('',#59425,#21984,#21985);
#19260=AXIS2_PLACEMENT_3D('',#59471,#21991,#21992);
#19261=AXIS2_PLACEMENT_3D('',#59473,#21993,#21994);
#19262=AXIS2_PLACEMENT_3D('',#59519,#22000,#22001);
#19263=AXIS2_PLACEMENT_3D('',#59521,#22002,#22003);
#19264=AXIS2_PLACEMENT_3D('',#59545,#22009,#22010);
#19265=AXIS2_PLACEMENT_3D('',#59547,#22011,#22012);
#19266=AXIS2_PLACEMENT_3D('',#59593,#22018,#22019);
#19267=AXIS2_PLACEMENT_3D('',#59595,#22020,#22021);
#19268=AXIS2_PLACEMENT_3D('',#59641,#22027,#22028);
#19269=AXIS2_PLACEMENT_3D('',#59643,#22029,#22030);
#19270=AXIS2_PLACEMENT_3D('',#59817,#22035,#22036);
#19271=AXIS2_PLACEMENT_3D('',#60623,#22037,#22038);
#19272=AXIS2_PLACEMENT_3D('',#60782,#22039,#22040);
#19273=AXIS2_PLACEMENT_3D('',#61463,#22041,#22042);
#19274=AXIS2_PLACEMENT_3D('',#61464,#22043,#22044);
#19275=AXIS2_PLACEMENT_3D('',#61623,#22045,#22046);
#19276=AXIS2_PLACEMENT_3D('',#62304,#22047,#22048);
#19277=AXIS2_PLACEMENT_3D('',#62305,#22049,#22050);
#19278=AXIS2_PLACEMENT_3D('',#62464,#22051,#22052);
#19279=AXIS2_PLACEMENT_3D('',#63145,#22053,#22054);
#19280=AXIS2_PLACEMENT_3D('',#63146,#22055,#22056);
#19281=AXIS2_PLACEMENT_3D('',#63305,#22057,#22058);
#19282=AXIS2_PLACEMENT_3D('',#63986,#22059,#22060);
#19283=AXIS2_PLACEMENT_3D('',#63987,#22061,#22062);
#19284=AXIS2_PLACEMENT_3D('',#64146,#22063,#22064);
#19285=AXIS2_PLACEMENT_3D('',#64827,#22065,#22066);
#19286=AXIS2_PLACEMENT_3D('',#64828,#22067,#22068);
#19287=AXIS2_PLACEMENT_3D('',#64830,#22070,#22071);
#19288=AXIS2_PLACEMENT_3D('',#64832,#22073,#22074);
#19289=AXIS2_PLACEMENT_3D('',#64834,#22076,#22077);
#19290=AXIS2_PLACEMENT_3D('',#64836,#22079,#22080);
#19291=AXIS2_PLACEMENT_3D('',#64838,#22082,#22083);
#19292=AXIS2_PLACEMENT_3D('',#64840,#22085,#22086);
#19293=AXIS2_PLACEMENT_3D('',#64842,#22088,#22089);
#19294=AXIS2_PLACEMENT_3D('',#64844,#22091,#22092);
#19295=AXIS2_PLACEMENT_3D('',#64846,#22094,#22095);
#19296=AXIS2_PLACEMENT_3D('',#64848,#22097,#22098);
#19297=AXIS2_PLACEMENT_3D('',#65007,#22099,#22100);
#19298=AXIS2_PLACEMENT_3D('',#65527,#22101,#22102);
#19299=AXIS2_PLACEMENT_3D('',#65528,#22103,#22104);
#19300=AXIS2_PLACEMENT_3D('',#65687,#22105,#22106);
#19301=AXIS2_PLACEMENT_3D('',#66207,#22107,#22108);
#19302=AXIS2_PLACEMENT_3D('',#66208,#22109,#22110);
#19303=AXIS2_PLACEMENT_3D('',#66367,#22111,#22112);
#19304=AXIS2_PLACEMENT_3D('',#66887,#22113,#22114);
#19305=AXIS2_PLACEMENT_3D('',#66888,#22115,#22116);
#19306=AXIS2_PLACEMENT_3D('',#67047,#22117,#22118);
#19307=AXIS2_PLACEMENT_3D('',#67567,#22119,#22120);
#19308=AXIS2_PLACEMENT_3D('',#67568,#22121,#22122);
#19309=AXIS2_PLACEMENT_3D('',#67727,#22123,#22124);
#19310=AXIS2_PLACEMENT_3D('',#68247,#22125,#22126);
#19311=AXIS2_PLACEMENT_3D('',#68248,#22127,#22128);
#19312=AXIS2_PLACEMENT_3D('',#68250,#22130,#22131);
#19313=AXIS2_PLACEMENT_3D('',#68252,#22133,#22134);
#19314=AXIS2_PLACEMENT_3D('',#68254,#22136,#22137);
#19315=AXIS2_PLACEMENT_3D('',#68256,#22139,#22140);
#19316=AXIS2_PLACEMENT_3D('',#68258,#22142,#22143);
#19317=AXIS2_PLACEMENT_3D('',#68260,#22145,#22146);
#19318=AXIS2_PLACEMENT_3D('',#68262,#22148,#22149);
#19319=AXIS2_PLACEMENT_3D('',#68264,#22151,#22152);
#19320=AXIS2_PLACEMENT_3D('',#68266,#22154,#22155);
#19321=AXIS2_PLACEMENT_3D('',#68268,#22157,#22158);
#19322=AXIS2_PLACEMENT_3D('',#68427,#22159,#22160);
#19323=AXIS2_PLACEMENT_3D('',#69108,#22161,#22162);
#19324=AXIS2_PLACEMENT_3D('',#69109,#22163,#22164);
#19325=AXIS2_PLACEMENT_3D('',#69111,#22166,#22167);
#19326=AXIS2_PLACEMENT_3D('',#69113,#22169,#22170);
#19327=AXIS2_PLACEMENT_3D('',#69272,#22171,#22172);
#19328=AXIS2_PLACEMENT_3D('',#69792,#22173,#22174);
#19329=AXIS2_PLACEMENT_3D('',#69793,#22175,#22176);
#19330=AXIS2_PLACEMENT_3D('',#69795,#22178,#22179);
#19331=AXIS2_PLACEMENT_3D('',#69797,#22181,#22182);
#19332=AXIS2_PLACEMENT_3D('',#69799,#22183,#22184);
#19333=AXIS2_PLACEMENT_3D('',#69802,#22186,#22187);
#19334=AXIS2_PLACEMENT_3D('',#69803,#22188,#22189);
#19335=AXIS2_PLACEMENT_3D('',#69805,#22190,#22191);
#19336=AXIS2_PLACEMENT_3D('',#69809,#22194,#22195);
#19337=AXIS2_PLACEMENT_3D('',#69810,#22196,#22197);
#19338=AXIS2_PLACEMENT_3D('',#69811,#22198,#22199);
#19339=AXIS2_PLACEMENT_3D('',#69813,#22200,#22201);
#19340=AXIS2_PLACEMENT_3D('',#69816,#22203,#22204);
#19341=AXIS2_PLACEMENT_3D('',#69817,#22205,#22206);
#19342=AXIS2_PLACEMENT_3D('',#69819,#22207,#22208);
#19343=AXIS2_PLACEMENT_3D('',#69823,#22211,#22212);
#19344=AXIS2_PLACEMENT_3D('',#69824,#22213,#22214);
#19345=AXIS2_PLACEMENT_3D('',#69825,#22215,#22216);
#19346=AXIS2_PLACEMENT_3D('',#69827,#22217,#22218);
#19347=AXIS2_PLACEMENT_3D('',#69830,#22220,#22221);
#19348=AXIS2_PLACEMENT_3D('',#69831,#22222,#22223);
#19349=AXIS2_PLACEMENT_3D('',#69833,#22224,#22225);
#19350=AXIS2_PLACEMENT_3D('',#69837,#22228,#22229);
#19351=AXIS2_PLACEMENT_3D('',#69838,#22230,#22231);
#19352=AXIS2_PLACEMENT_3D('',#69839,#22232,#22233);
#19353=AXIS2_PLACEMENT_3D('',#69841,#22234,#22235);
#19354=AXIS2_PLACEMENT_3D('',#69844,#22237,#22238);
#19355=AXIS2_PLACEMENT_3D('',#69845,#22239,#22240);
#19356=AXIS2_PLACEMENT_3D('',#69847,#22241,#22242);
#19357=AXIS2_PLACEMENT_3D('',#69851,#22245,#22246);
#19358=AXIS2_PLACEMENT_3D('',#69852,#22247,#22248);
#19359=AXIS2_PLACEMENT_3D('',#69853,#22249,#22250);
#19360=AXIS2_PLACEMENT_3D('',#69855,#22251,#22252);
#19361=AXIS2_PLACEMENT_3D('',#69858,#22254,#22255);
#19362=AXIS2_PLACEMENT_3D('',#69859,#22256,#22257);
#19363=AXIS2_PLACEMENT_3D('',#69861,#22258,#22259);
#19364=AXIS2_PLACEMENT_3D('',#69865,#22262,#22263);
#19365=AXIS2_PLACEMENT_3D('',#69866,#22264,#22265);
#19366=AXIS2_PLACEMENT_3D('',#69867,#22266,#22267);
#19367=AXIS2_PLACEMENT_3D('',#69869,#22268,#22269);
#19368=AXIS2_PLACEMENT_3D('',#69872,#22271,#22272);
#19369=AXIS2_PLACEMENT_3D('',#69873,#22273,#22274);
#19370=AXIS2_PLACEMENT_3D('',#69875,#22275,#22276);
#19371=AXIS2_PLACEMENT_3D('',#69879,#22279,#22280);
#19372=AXIS2_PLACEMENT_3D('',#69880,#22281,#22282);
#19373=AXIS2_PLACEMENT_3D('',#69881,#22283,#22284);
#19374=AXIS2_PLACEMENT_3D('',#69892,#22287,#22288);
#19375=AXIS2_PLACEMENT_3D('',#69903,#22291,#22292);
#19376=AXIS2_PLACEMENT_3D('',#69907,#22295,#22296);
#19377=AXIS2_PLACEMENT_3D('',#69909,#22298,#22299);
#19378=AXIS2_PLACEMENT_3D('',#69920,#22302,#22303);
#19379=AXIS2_PLACEMENT_3D('',#69924,#22306,#22307);
#19380=AXIS2_PLACEMENT_3D('',#69928,#22310,#22311);
#19381=AXIS2_PLACEMENT_3D('',#69937,#22313,#22314);
#19382=AXIS2_PLACEMENT_3D('',#69948,#22317,#22318);
#19383=AXIS2_PLACEMENT_3D('',#69952,#22321,#22322);
#19384=AXIS2_PLACEMENT_3D('',#69956,#22325,#22326);
#19385=AXIS2_PLACEMENT_3D('',#69965,#22328,#22329);
#19386=AXIS2_PLACEMENT_3D('',#69976,#22332,#22333);
#19387=AXIS2_PLACEMENT_3D('',#69980,#22336,#22337);
#19388=AXIS2_PLACEMENT_3D('',#69984,#22340,#22341);
#19389=AXIS2_PLACEMENT_3D('',#69993,#22343,#22344);
#19390=AXIS2_PLACEMENT_3D('',#70004,#22347,#22348);
#19391=AXIS2_PLACEMENT_3D('',#70015,#22351,#22352);
#19392=AXIS2_PLACEMENT_3D('',#70019,#22355,#22356);
#19393=AXIS2_PLACEMENT_3D('',#86269,#22366,#22367);
#19394=AXIS2_PLACEMENT_3D('',#86280,#22370,#22371);
#19395=AXIS2_PLACEMENT_3D('',#86291,#22374,#22375);
#19396=AXIS2_PLACEMENT_3D('',#86295,#22378,#22379);
#19397=AXIS2_PLACEMENT_3D('',#88337,#22382,#22383);
#19398=AXIS2_PLACEMENT_3D('',#88340,#22385,#22386);
#19399=AXIS2_PLACEMENT_3D('',#88341,#22387,#22388);
#19400=AXIS2_PLACEMENT_3D('',#88344,#22390,#22391);
#19401=AXIS2_PLACEMENT_3D('',#88345,#22392,#22393);
#19402=AXIS2_PLACEMENT_3D('',#88347,#22395,#22396);
#19403=AXIS2_PLACEMENT_3D('',#88350,#22398,#22399);
#19404=AXIS2_PLACEMENT_3D('',#88351,#22400,#22401);
#19405=AXIS2_PLACEMENT_3D('',#88354,#22403,#22404);
#19406=AXIS2_PLACEMENT_3D('',#88355,#22405,#22406);
#19407=AXIS2_PLACEMENT_3D('',#88357,#22408,#22409);
#19408=AXIS2_PLACEMENT_3D('',#88360,#22411,#22412);
#19409=AXIS2_PLACEMENT_3D('',#88361,#22413,#22414);
#19410=AXIS2_PLACEMENT_3D('',#88364,#22416,#22417);
#19411=AXIS2_PLACEMENT_3D('',#88365,#22418,#22419);
#19412=AXIS2_PLACEMENT_3D('',#88367,#22421,#22422);
#19413=AXIS2_PLACEMENT_3D('',#88374,#22423,#22424);
#19414=AXIS2_PLACEMENT_3D('',#88376,#22425,#22426);
#19415=AXIS2_PLACEMENT_3D('',#88384,#22428,#22429);
#19416=AXIS2_PLACEMENT_3D('',#88386,#22430,#22431);
#19417=AXIS2_PLACEMENT_3D('',#88394,#22433,#22434);
#19418=AXIS2_PLACEMENT_3D('',#88396,#22435,#22436);
#19419=AXIS2_PLACEMENT_3D('',#88398,#22438,#22439);
#19420=AXIS2_PLACEMENT_3D('',#88399,#22440,#22441);
#19421=AXIS2_PLACEMENT_3D('',#88401,#22443,#22444);
#19422=AXIS2_PLACEMENT_3D('',#88403,#22446,#22447);
#19423=AXIS2_PLACEMENT_3D('',#90415,#22449,#22450);
#19424=AXIS2_PLACEMENT_3D('',#90417,#22452,#22453);
#19425=AXIS2_PLACEMENT_3D('',#90419,#22455,#22456);
#19426=AXIS2_PLACEMENT_3D('',#92431,#22458,#22459);
#19427=AXIS2_PLACEMENT_3D('',#94444,#22462,#22463);
#19428=AXIS2_PLACEMENT_3D('',#94446,#22465,#22466);
#19429=AXIS2_PLACEMENT_3D('',#94447,#22467,#22468);
#21181=DIRECTION('axis',(0.,0.,1.));
#21182=DIRECTION('refdir',(1.,0.,0.));
#21183=DIRECTION('center_axis',(0.,0.,-1.));
#21184=DIRECTION('ref_axis',(1.,0.,0.));
#21185=DIRECTION('',(0.,0.,-1.));
#21186=DIRECTION('center_axis',(0.,0.,1.));
#21187=DIRECTION('ref_axis',(1.,0.,0.));
#21188=DIRECTION('',(0.,0.,-1.));
#21189=DIRECTION('center_axis',(0.,0.,1.));
#21190=DIRECTION('ref_axis',(1.,0.,0.));
#21191=DIRECTION('center_axis',(0.,0.,1.));
#21192=DIRECTION('ref_axis',(1.,0.,0.));
#21193=DIRECTION('center_axis',(0.,0.,1.));
#21194=DIRECTION('ref_axis',(1.,0.,0.));
#21195=DIRECTION('center_axis',(0.,0.,1.));
#21196=DIRECTION('ref_axis',(1.,0.,0.));
#21197=DIRECTION('center_axis',(0.,0.,-1.));
#21198=DIRECTION('ref_axis',(1.,0.,0.));
#21199=DIRECTION('',(0.,0.,-1.));
#21200=DIRECTION('center_axis',(0.,0.,-1.));
#21201=DIRECTION('ref_axis',(1.,0.,0.));
#21202=DIRECTION('',(0.,0.,-1.));
#21203=DIRECTION('center_axis',(0.,0.,-1.));
#21204=DIRECTION('ref_axis',(1.,0.,0.));
#21205=DIRECTION('',(0.,0.,-1.));
#21206=DIRECTION('center_axis',(0.,0.,-1.));
#21207=DIRECTION('ref_axis',(1.,0.,0.));
#21208=DIRECTION('',(0.,0.,-1.));
#21209=DIRECTION('center_axis',(0.,0.,-1.));
#21210=DIRECTION('ref_axis',(1.,0.,0.));
#21211=DIRECTION('',(0.,0.,-1.));
#21212=DIRECTION('center_axis',(0.,0.,-1.));
#21213=DIRECTION('ref_axis',(1.,0.,0.));
#21214=DIRECTION('',(0.,0.,-1.));
#21215=DIRECTION('center_axis',(0.,0.,-1.));
#21216=DIRECTION('ref_axis',(0.937375356024964,-0.348320889291861,0.));
#21217=DIRECTION('',(0.,0.,-1.));
#21218=DIRECTION('center_axis',(0.,0.,1.));
#21219=DIRECTION('ref_axis',(1.,0.,0.));
#21220=DIRECTION('center_axis',(0.,0.,-1.));
#21221=DIRECTION('ref_axis',(0.793245518852996,0.608901918883199,0.));
#21222=DIRECTION('',(1.22464679914735E-16,-4.24456931042874E-30,-1.));
#21223=DIRECTION('center_axis',(0.,0.,1.));
#21224=DIRECTION('ref_axis',(1.,-3.45370740000048E-14,0.));
#21225=DIRECTION('center_axis',(0.,0.,-1.));
#21226=DIRECTION('ref_axis',(1.,-3.45370740000048E-14,0.));
#21227=DIRECTION('',(1.22464679914735E-16,-4.24456931042874E-30,-1.));
#21228=DIRECTION('center_axis',(0.,0.,-1.));
#21229=DIRECTION('ref_axis',(1.,-3.45370740000048E-14,0.));
#21230=DIRECTION('',(1.22464679914735E-16,-4.24456931042874E-30,-1.));
#21231=DIRECTION('center_axis',(0.,0.,-1.));
#21232=DIRECTION('ref_axis',(1.,-3.45370740000048E-14,0.));
#21233=DIRECTION('',(1.22464679914735E-16,-4.24456931042874E-30,-1.));
#21234=DIRECTION('center_axis',(0.,0.,-1.));
#21235=DIRECTION('ref_axis',(1.,-3.45370740000048E-14,0.));
#21236=DIRECTION('',(1.22464679914735E-16,-4.24456931042874E-30,-1.));
#21237=DIRECTION('center_axis',(0.,0.,-1.));
#21238=DIRECTION('ref_axis',(1.,-3.45370740000048E-14,0.));
#21239=DIRECTION('',(1.22464679914735E-16,-4.24456931042874E-30,-1.));
#21240=DIRECTION('center_axis',(0.,0.,-1.));
#21241=DIRECTION('ref_axis',(1.,-3.45370740000048E-14,0.));
#21242=DIRECTION('',(1.22464679914735E-16,-4.24456931042874E-30,-1.));
#21243=DIRECTION('center_axis',(0.,0.,-1.));
#21244=DIRECTION('ref_axis',(-0.609079509840797,-0.793109166944939,0.));
#21245=DIRECTION('',(1.22464679914735E-16,-4.24456931042874E-30,-1.));
#21246=DIRECTION('center_axis',(0.,0.,-1.));
#21247=DIRECTION('ref_axis',(1.,-3.45370740000048E-14,0.));
#21248=DIRECTION('center_axis',(0.,0.,1.));
#21249=DIRECTION('ref_axis',(-1.,0.,0.));
#21250=DIRECTION('',(0.,0.,1.));
#21251=DIRECTION('center_axis',(0.,0.,-1.));
#21252=DIRECTION('ref_axis',(-1.,0.,0.));
#21253=DIRECTION('',(0.,0.,1.));
#21254=DIRECTION('center_axis',(0.,0.,-1.));
#21255=DIRECTION('ref_axis',(-1.,0.,0.));
#21256=DIRECTION('center_axis',(0.,0.,-1.));
#21257=DIRECTION('ref_axis',(-1.,0.,0.));
#21258=DIRECTION('center_axis',(0.,0.,-1.));
#21259=DIRECTION('ref_axis',(-1.,0.,0.));
#21260=DIRECTION('center_axis',(0.,0.,-1.));
#21261=DIRECTION('ref_axis',(-1.,0.,0.));
#21262=DIRECTION('center_axis',(0.,0.,1.));
#21263=DIRECTION('ref_axis',(-1.,0.,0.));
#21264=DIRECTION('',(0.,0.,1.));
#21265=DIRECTION('center_axis',(0.,0.,1.));
#21266=DIRECTION('ref_axis',(-1.,0.,0.));
#21267=DIRECTION('',(0.,0.,1.));
#21268=DIRECTION('center_axis',(0.,0.,1.));
#21269=DIRECTION('ref_axis',(-1.,0.,0.));
#21270=DIRECTION('',(0.,0.,1.));
#21271=DIRECTION('center_axis',(0.,0.,1.));
#21272=DIRECTION('ref_axis',(-1.,0.,0.));
#21273=DIRECTION('',(0.,0.,1.));
#21274=DIRECTION('center_axis',(0.,0.,1.));
#21275=DIRECTION('ref_axis',(-1.,0.,0.));
#21276=DIRECTION('',(0.,0.,1.));
#21277=DIRECTION('center_axis',(0.,0.,1.));
#21278=DIRECTION('ref_axis',(-1.,0.,0.));
#21279=DIRECTION('',(0.,0.,1.));
#21280=DIRECTION('center_axis',(0.,0.,1.));
#21281=DIRECTION('ref_axis',(-0.937374823573184,-0.348322322183265,0.));
#21282=DIRECTION('',(0.,0.,1.));
#21283=DIRECTION('center_axis',(0.,0.,-1.));
#21284=DIRECTION('ref_axis',(-1.,0.,0.));
#21285=DIRECTION('center_axis',(0.,0.,1.));
#21286=DIRECTION('ref_axis',(-0.793244897475727,0.608902728380094,0.));
#21287=DIRECTION('',(-1.22464679914735E-16,-2.12978345412769E-30,1.));
#21288=DIRECTION('center_axis',(0.,0.,-1.));
#21289=DIRECTION('ref_axis',(-1.,-1.72685370000025E-14,0.));
#21290=DIRECTION('center_axis',(0.,0.,1.));
#21291=DIRECTION('ref_axis',(-1.,-1.72685370000025E-14,0.));
#21292=DIRECTION('',(-1.22464679914735E-16,-2.12978345412769E-30,1.));
#21293=DIRECTION('center_axis',(0.,0.,1.));
#21294=DIRECTION('ref_axis',(-1.,-1.72685370000025E-14,0.));
#21295=DIRECTION('',(-1.22464679914735E-16,-2.12978345412769E-30,1.));
#21296=DIRECTION('center_axis',(0.,0.,1.));
#21297=DIRECTION('ref_axis',(-1.,-1.72685370000025E-14,0.));
#21298=DIRECTION('',(-1.22464679914735E-16,-2.12978345412769E-30,1.));
#21299=DIRECTION('center_axis',(0.,0.,1.));
#21300=DIRECTION('ref_axis',(-1.,-1.72685370000025E-14,0.));
#21301=DIRECTION('',(-1.22464679914735E-16,-2.12978345412769E-30,1.));
#21302=DIRECTION('center_axis',(0.,0.,1.));
#21303=DIRECTION('ref_axis',(-1.,-1.72685370000025E-14,0.));
#21304=DIRECTION('',(-1.22464679914735E-16,-2.12978345412769E-30,1.));
#21305=DIRECTION('center_axis',(0.,0.,1.));
#21306=DIRECTION('ref_axis',(-1.,-1.72685370000025E-14,0.));
#21307=DIRECTION('',(-1.22464679914735E-16,-2.12978345412769E-30,1.));
#21308=DIRECTION('center_axis',(0.,0.,1.));
#21309=DIRECTION('ref_axis',(0.609080360598175,-0.793108513592937,0.));
#21310=DIRECTION('',(-1.22464679914735E-16,-2.12978345412769E-30,1.));
#21311=DIRECTION('center_axis',(0.,0.,1.));
#21312=DIRECTION('ref_axis',(-1.,-1.72685370000025E-14,0.));
#21313=DIRECTION('center_axis',(0.,0.,-1.));
#21314=DIRECTION('ref_axis',(0.5,0.866025403784439,0.));
#21315=DIRECTION('',(0.,0.,-1.));
#21316=DIRECTION('center_axis',(0.,0.,1.));
#21317=DIRECTION('ref_axis',(0.5,0.866025403784439,0.));
#21318=DIRECTION('',(0.,0.,-1.));
#21319=DIRECTION('center_axis',(0.,0.,1.));
#21320=DIRECTION('ref_axis',(0.5,0.866025403784439,0.));
#21321=DIRECTION('center_axis',(0.,0.,1.));
#21322=DIRECTION('ref_axis',(0.5,0.866025403784439,0.));
#21323=DIRECTION('center_axis',(0.,0.,1.));
#21324=DIRECTION('ref_axis',(0.5,0.866025403784439,0.));
#21325=DIRECTION('center_axis',(0.,0.,1.));
#21326=DIRECTION('ref_axis',(0.5,0.866025403784439,0.));
#21327=DIRECTION('center_axis',(0.,0.,-1.));
#21328=DIRECTION('ref_axis',(0.5,0.866025403784439,0.));
#21329=DIRECTION('',(0.,0.,-1.));
#21330=DIRECTION('center_axis',(0.,0.,-1.));
#21331=DIRECTION('ref_axis',(0.5,0.866025403784439,0.));
#21332=DIRECTION('',(0.,0.,-1.));
#21333=DIRECTION('center_axis',(0.,0.,-1.));
#21334=DIRECTION('ref_axis',(0.5,0.866025403784439,0.));
#21335=DIRECTION('',(0.,0.,-1.));
#21336=DIRECTION('center_axis',(0.,0.,-1.));
#21337=DIRECTION('ref_axis',(0.5,0.866025403784439,0.));
#21338=DIRECTION('',(0.,0.,-1.));
#21339=DIRECTION('center_axis',(0.,0.,-1.));
#21340=DIRECTION('ref_axis',(0.5,0.866025403784439,0.));
#21341=DIRECTION('',(0.,0.,-1.));
#21342=DIRECTION('center_axis',(0.,0.,-1.));
#21343=DIRECTION('ref_axis',(0.5,0.866025403784439,0.));
#21344=DIRECTION('',(0.,0.,-1.));
#21345=DIRECTION('center_axis',(0.,0.,-1.));
#21346=DIRECTION('ref_axis',(0.77034243979566,0.637630398781041,0.));
#21347=DIRECTION('',(0.,0.,-1.));
#21348=DIRECTION('center_axis',(0.,0.,1.));
#21349=DIRECTION('ref_axis',(0.5,0.866025403784439,0.));
#21350=DIRECTION('center_axis',(0.,0.,-1.));
#21351=DIRECTION('ref_axis',(-0.130701796389753,0.991421726824912,0.));
#21352=DIRECTION('',(6.12323399573733E-17,1.06057523872487E-16,-1.));
#21353=DIRECTION('center_axis',(0.,0.,1.));
#21354=DIRECTION('ref_axis',(0.500000000000046,0.866025403784412,0.));
#21355=DIRECTION('center_axis',(0.,0.,-1.));
#21356=DIRECTION('ref_axis',(0.500000000000046,0.866025403784412,0.));
#21357=DIRECTION('',(6.12323399573733E-17,1.06057523872487E-16,-1.));
#21358=DIRECTION('center_axis',(0.,0.,-1.));
#21359=DIRECTION('ref_axis',(0.500000000000046,0.866025403784412,0.));
#21360=DIRECTION('',(6.12323399573733E-17,1.06057523872487E-16,-1.));
#21361=DIRECTION('center_axis',(0.,0.,-1.));
#21362=DIRECTION('ref_axis',(0.500000000000046,0.866025403784412,0.));
#21363=DIRECTION('',(6.12323399573733E-17,1.06057523872487E-16,-1.));
#21364=DIRECTION('center_axis',(0.,0.,-1.));
#21365=DIRECTION('ref_axis',(0.500000000000046,0.866025403784412,0.));
#21366=DIRECTION('',(6.12323399573733E-17,1.06057523872487E-16,-1.));
#21367=DIRECTION('center_axis',(0.,0.,-1.));
#21368=DIRECTION('ref_axis',(0.500000000000046,0.866025403784412,0.));
#21369=DIRECTION('',(6.12323399573733E-17,1.06057523872487E-16,-1.));
#21370=DIRECTION('center_axis',(0.,0.,-1.));
#21371=DIRECTION('ref_axis',(0.500000000000046,0.866025403784412,0.));
#21372=DIRECTION('',(6.12323399573733E-17,1.06057523872487E-16,-1.));
#21373=DIRECTION('center_axis',(0.,0.,-1.));
#21374=DIRECTION('ref_axis',(0.382312913538214,-0.924032919403807,0.));
#21375=DIRECTION('',(6.12323399573733E-17,1.06057523872487E-16,-1.));
#21376=DIRECTION('center_axis',(0.,0.,-1.));
#21377=DIRECTION('ref_axis',(0.500000000000046,0.866025403784412,0.));
#21378=DIRECTION('center_axis',(0.,0.,-1.));
#21379=DIRECTION('ref_axis',(-0.5,0.866025403784439,0.));
#21380=DIRECTION('',(0.,0.,-1.));
#21381=DIRECTION('center_axis',(0.,0.,1.));
#21382=DIRECTION('ref_axis',(-0.5,0.866025403784439,0.));
#21383=DIRECTION('',(0.,0.,-1.));
#21384=DIRECTION('center_axis',(0.,0.,1.));
#21385=DIRECTION('ref_axis',(-0.5,0.866025403784439,0.));
#21386=DIRECTION('center_axis',(0.,0.,1.));
#21387=DIRECTION('ref_axis',(-0.5,0.866025403784439,0.));
#21388=DIRECTION('center_axis',(0.,0.,1.));
#21389=DIRECTION('ref_axis',(-0.5,0.866025403784439,0.));
#21390=DIRECTION('center_axis',(0.,0.,1.));
#21391=DIRECTION('ref_axis',(-0.5,0.866025403784439,0.));
#21392=DIRECTION('center_axis',(0.,0.,-1.));
#21393=DIRECTION('ref_axis',(-0.5,0.866025403784439,0.));
#21394=DIRECTION('',(0.,0.,-1.));
#21395=DIRECTION('center_axis',(0.,0.,-1.));
#21396=DIRECTION('ref_axis',(-0.5,0.866025403784439,0.));
#21397=DIRECTION('',(0.,0.,-1.));
#21398=DIRECTION('center_axis',(0.,0.,-1.));
#21399=DIRECTION('ref_axis',(-0.5,0.866025403784439,0.));
#21400=DIRECTION('',(0.,0.,-1.));
#21401=DIRECTION('center_axis',(0.,0.,-1.));
#21402=DIRECTION('ref_axis',(-0.5,0.866025403784439,0.));
#21403=DIRECTION('',(0.,0.,-1.));
#21404=DIRECTION('center_axis',(0.,0.,-1.));
#21405=DIRECTION('ref_axis',(-0.5,0.866025403784439,0.));
#21406=DIRECTION('',(0.,0.,-1.));
#21407=DIRECTION('center_axis',(0.,0.,-1.));
#21408=DIRECTION('ref_axis',(-0.5,0.866025403784439,0.));
#21409=DIRECTION('',(0.,0.,-1.));
#21410=DIRECTION('center_axis',(0.,0.,-1.));
#21411=DIRECTION('ref_axis',(-0.167034001011808,0.985951135962623,0.));
#21412=DIRECTION('',(0.,0.,-1.));
#21413=DIRECTION('center_axis',(0.,0.,1.));
#21414=DIRECTION('ref_axis',(-0.5,0.866025403784439,0.));
#21415=DIRECTION('center_axis',(0.,0.,-1.));
#21416=DIRECTION('ref_axis',(-0.923947020235643,0.382520461933313,0.));
#21417=DIRECTION('',(-6.12323399573632E-17,1.06057523872493E-16,-1.));
#21418=DIRECTION('center_axis',(0.,0.,1.));
#21419=DIRECTION('ref_axis',(-0.499999999999964,0.86602540378446,0.));
#21420=DIRECTION('center_axis',(0.,0.,-1.));
#21421=DIRECTION('ref_axis',(-0.499999999999964,0.86602540378446,0.));
#21422=DIRECTION('',(-6.12323399573632E-17,1.06057523872493E-16,-1.));
#21423=DIRECTION('center_axis',(0.,0.,-1.));
#21424=DIRECTION('ref_axis',(-0.499999999999964,0.86602540378446,0.));
#21425=DIRECTION('',(-6.12323399573632E-17,1.06057523872493E-16,-1.));
#21426=DIRECTION('center_axis',(0.,0.,-1.));
#21427=DIRECTION('ref_axis',(-0.499999999999964,0.86602540378446,0.));
#21428=DIRECTION('',(-6.12323399573632E-17,1.06057523872493E-16,-1.));
#21429=DIRECTION('center_axis',(0.,0.,-1.));
#21430=DIRECTION('ref_axis',(-0.499999999999964,0.86602540378446,0.));
#21431=DIRECTION('',(-6.12323399573632E-17,1.06057523872493E-16,-1.));
#21432=DIRECTION('center_axis',(0.,0.,-1.));
#21433=DIRECTION('ref_axis',(-0.499999999999964,0.86602540378446,0.));
#21434=DIRECTION('',(-6.12323399573632E-17,1.06057523872493E-16,-1.));
#21435=DIRECTION('center_axis',(0.,0.,-1.));
#21436=DIRECTION('ref_axis',(-0.499999999999964,0.86602540378446,0.));
#21437=DIRECTION('',(-6.12323399573632E-17,1.06057523872493E-16,-1.));
#21438=DIRECTION('center_axis',(0.,0.,-1.));
#21439=DIRECTION('ref_axis',(0.991392525759238,-0.130923106702819,0.));
#21440=DIRECTION('',(-6.12323399573632E-17,1.06057523872493E-16,-1.));
#21441=DIRECTION('center_axis',(0.,0.,-1.));
#21442=DIRECTION('ref_axis',(-0.499999999999964,0.86602540378446,0.));
#21443=DIRECTION('center_axis',(0.,0.,-1.));
#21444=DIRECTION('ref_axis',(-1.,9.25185853854297E-17,0.));
#21445=DIRECTION('',(0.,0.,-1.));
#21446=DIRECTION('center_axis',(0.,0.,1.));
#21447=DIRECTION('ref_axis',(-1.,9.25185853854297E-17,0.));
#21448=DIRECTION('',(0.,0.,-1.));
#21449=DIRECTION('center_axis',(0.,0.,1.));
#21450=DIRECTION('ref_axis',(-1.,9.25185853854297E-17,0.));
#21451=DIRECTION('center_axis',(0.,0.,1.));
#21452=DIRECTION('ref_axis',(-1.,9.25185853854297E-17,0.));
#21453=DIRECTION('center_axis',(0.,0.,1.));
#21454=DIRECTION('ref_axis',(-1.,9.25185853854297E-17,0.));
#21455=DIRECTION('center_axis',(0.,0.,1.));
#21456=DIRECTION('ref_axis',(-1.,9.25185853854297E-17,0.));
#21457=DIRECTION('center_axis',(0.,0.,-1.));
#21458=DIRECTION('ref_axis',(-1.,9.25185853854297E-17,0.));
#21459=DIRECTION('',(0.,0.,-1.));
#21460=DIRECTION('center_axis',(0.,0.,-1.));
#21461=DIRECTION('ref_axis',(-1.,9.25185853854297E-17,0.));
#21462=DIRECTION('',(0.,0.,-1.));
#21463=DIRECTION('center_axis',(0.,0.,-1.));
#21464=DIRECTION('ref_axis',(-1.,9.25185853854297E-17,0.));
#21465=DIRECTION('',(0.,0.,-1.));
#21466=DIRECTION('center_axis',(0.,0.,-1.));
#21467=DIRECTION('ref_axis',(-1.,9.25185853854297E-17,0.));
#21468=DIRECTION('',(0.,0.,-1.));
#21469=DIRECTION('center_axis',(0.,0.,-1.));
#21470=DIRECTION('ref_axis',(-1.,9.25185853854297E-17,0.));
#21471=DIRECTION('',(0.,0.,-1.));
#21472=DIRECTION('center_axis',(0.,0.,-1.));
#21473=DIRECTION('ref_axis',(-1.,9.25185853854297E-17,0.));
#21474=DIRECTION('',(0.,0.,-1.));
#21475=DIRECTION('center_axis',(0.,0.,-1.));
#21476=DIRECTION('ref_axis',(-0.937375356024962,0.348320889291865,0.));
#21477=DIRECTION('',(0.,0.,-1.));
#21478=DIRECTION('center_axis',(0.,0.,1.));
#21479=DIRECTION('ref_axis',(-1.,9.25185853854297E-17,0.));
#21480=DIRECTION('center_axis',(0.,0.,-1.));
#21481=DIRECTION('ref_axis',(-0.793245518852988,-0.608901918883209,0.));
#21482=DIRECTION('',(-1.22464679914735E-16,2.65847991820293E-30,-1.));
#21483=DIRECTION('center_axis',(0.,0.,1.));
#21484=DIRECTION('ref_axis',(-1.,2.15856712500029E-14,0.));
#21485=DIRECTION('center_axis',(0.,0.,-1.));
#21486=DIRECTION('ref_axis',(-1.,2.15856712500029E-14,0.));
#21487=DIRECTION('',(-1.22464679914735E-16,2.65847991820293E-30,-1.));
#21488=DIRECTION('center_axis',(0.,0.,-1.));
#21489=DIRECTION('ref_axis',(-1.,2.15856712500029E-14,0.));
#21490=DIRECTION('',(-1.22464679914735E-16,2.65847991820293E-30,-1.));
#21491=DIRECTION('center_axis',(0.,0.,-1.));
#21492=DIRECTION('ref_axis',(-1.,2.15856712500029E-14,0.));
#21493=DIRECTION('',(-1.22464679914735E-16,2.65847991820293E-30,-1.));
#21494=DIRECTION('center_axis',(0.,0.,-1.));
#21495=DIRECTION('ref_axis',(-1.,2.15856712500029E-14,0.));
#21496=DIRECTION('',(-1.22464679914735E-16,2.65847991820293E-30,-1.));
#21497=DIRECTION('center_axis',(0.,0.,-1.));
#21498=DIRECTION('ref_axis',(-1.,2.15856712500029E-14,0.));
#21499=DIRECTION('',(-1.22464679914735E-16,2.65847991820293E-30,-1.));
#21500=DIRECTION('center_axis',(0.,0.,-1.));
#21501=DIRECTION('ref_axis',(-1.,2.15856712500029E-14,0.));
#21502=DIRECTION('',(-1.22464679914735E-16,2.65847991820293E-30,-1.));
#21503=DIRECTION('center_axis',(0.,0.,-1.));
#21504=DIRECTION('ref_axis',(0.609079509840783,0.793109166944949,0.));
#21505=DIRECTION('',(-1.22464679914735E-16,2.65847991820293E-30,-1.));
#21506=DIRECTION('center_axis',(0.,0.,-1.));
#21507=DIRECTION('ref_axis',(-1.,2.15856712500029E-14,0.));
#21508=DIRECTION('center_axis',(0.,0.,-1.));
#21509=DIRECTION('ref_axis',(-0.5,-0.866025403784438,0.));
#21510=DIRECTION('',(0.,0.,-1.));
#21511=DIRECTION('center_axis',(0.,0.,1.));
#21512=DIRECTION('ref_axis',(-0.5,-0.866025403784438,0.));
#21513=DIRECTION('',(0.,0.,-1.));
#21514=DIRECTION('center_axis',(0.,0.,1.));
#21515=DIRECTION('ref_axis',(-0.5,-0.866025403784438,0.));
#21516=DIRECTION('center_axis',(0.,0.,1.));
#21517=DIRECTION('ref_axis',(-0.5,-0.866025403784438,0.));
#21518=DIRECTION('center_axis',(0.,0.,1.));
#21519=DIRECTION('ref_axis',(-0.5,-0.866025403784438,0.));
#21520=DIRECTION('center_axis',(0.,0.,1.));
#21521=DIRECTION('ref_axis',(-0.5,-0.866025403784438,0.));
#21522=DIRECTION('center_axis',(0.,0.,-1.));
#21523=DIRECTION('ref_axis',(-0.5,-0.866025403784438,0.));
#21524=DIRECTION('',(0.,0.,-1.));
#21525=DIRECTION('center_axis',(0.,0.,-1.));
#21526=DIRECTION('ref_axis',(-0.5,-0.866025403784438,0.));
#21527=DIRECTION('',(0.,0.,-1.));
#21528=DIRECTION('center_axis',(0.,0.,-1.));
#21529=DIRECTION('ref_axis',(-0.5,-0.866025403784438,0.));
#21530=DIRECTION('',(0.,0.,-1.));
#21531=DIRECTION('center_axis',(0.,0.,-1.));
#21532=DIRECTION('ref_axis',(-0.5,-0.866025403784438,0.));
#21533=DIRECTION('',(0.,0.,-1.));
#21534=DIRECTION('center_axis',(0.,0.,-1.));
#21535=DIRECTION('ref_axis',(-0.5,-0.866025403784438,0.));
#21536=DIRECTION('',(0.,0.,-1.));
#21537=DIRECTION('center_axis',(0.,0.,-1.));
#21538=DIRECTION('ref_axis',(-0.5,-0.866025403784438,0.));
#21539=DIRECTION('',(0.,0.,-1.));
#21540=DIRECTION('center_axis',(0.,0.,-1.));
#21541=DIRECTION('ref_axis',(-0.770342439795701,-0.637630398780992,0.));
#21542=DIRECTION('',(0.,0.,-1.));
#21543=DIRECTION('center_axis',(0.,0.,1.));
#21544=DIRECTION('ref_axis',(-0.5,-0.866025403784438,0.));
#21545=DIRECTION('center_axis',(0.,0.,-1.));
#21546=DIRECTION('ref_axis',(0.130701796389773,-0.99142172682491,0.));
#21547=DIRECTION('',(-6.12323399573712E-17,-1.06057523872489E-16,-1.));
#21548=DIRECTION('center_axis',(0.,0.,1.));
#21549=DIRECTION('ref_axis',(-0.500000000000029,-0.866025403784422,0.));
#21550=DIRECTION('center_axis',(0.,0.,-1.));
#21551=DIRECTION('ref_axis',(-0.500000000000029,-0.866025403784422,0.));
#21552=DIRECTION('',(-6.12323399573712E-17,-1.06057523872489E-16,-1.));
#21553=DIRECTION('center_axis',(0.,0.,-1.));
#21554=DIRECTION('ref_axis',(-0.500000000000029,-0.866025403784422,0.));
#21555=DIRECTION('',(-6.12323399573712E-17,-1.06057523872489E-16,-1.));
#21556=DIRECTION('center_axis',(0.,0.,-1.));
#21557=DIRECTION('ref_axis',(-0.500000000000029,-0.866025403784422,0.));
#21558=DIRECTION('',(-6.12323399573712E-17,-1.06057523872489E-16,-1.));
#21559=DIRECTION('center_axis',(0.,0.,-1.));
#21560=DIRECTION('ref_axis',(-0.500000000000029,-0.866025403784422,0.));
#21561=DIRECTION('',(-6.12323399573712E-17,-1.06057523872489E-16,-1.));
#21562=DIRECTION('center_axis',(0.,0.,-1.));
#21563=DIRECTION('ref_axis',(-0.500000000000029,-0.866025403784422,0.));
#21564=DIRECTION('',(-6.12323399573712E-17,-1.06057523872489E-16,-1.));
#21565=DIRECTION('center_axis',(0.,0.,-1.));
#21566=DIRECTION('ref_axis',(-0.500000000000029,-0.866025403784422,0.));
#21567=DIRECTION('',(-6.12323399573712E-17,-1.06057523872489E-16,-1.));
#21568=DIRECTION('center_axis',(0.,0.,-1.));
#21569=DIRECTION('ref_axis',(-0.382312913538216,0.924032919403806,0.));
#21570=DIRECTION('',(-6.12323399573712E-17,-1.06057523872489E-16,-1.));
#21571=DIRECTION('center_axis',(0.,0.,-1.));
#21572=DIRECTION('ref_axis',(-0.500000000000029,-0.866025403784422,0.));
#21573=DIRECTION('center_axis',(0.,0.,-1.));
#21574=DIRECTION('ref_axis',(0.499999999999999,-0.866025403784439,0.));
#21575=DIRECTION('',(0.,0.,-1.));
#21576=DIRECTION('center_axis',(0.,0.,1.));
#21577=DIRECTION('ref_axis',(0.499999999999999,-0.866025403784439,0.));
#21578=DIRECTION('',(0.,0.,-1.));
#21579=DIRECTION('center_axis',(0.,0.,1.));
#21580=DIRECTION('ref_axis',(0.499999999999999,-0.866025403784439,0.));
#21581=DIRECTION('center_axis',(0.,0.,1.));
#21582=DIRECTION('ref_axis',(0.499999999999999,-0.866025403784439,0.));
#21583=DIRECTION('center_axis',(0.,0.,1.));
#21584=DIRECTION('ref_axis',(0.499999999999999,-0.866025403784439,0.));
#21585=DIRECTION('center_axis',(0.,0.,1.));
#21586=DIRECTION('ref_axis',(0.499999999999999,-0.866025403784439,0.));
#21587=DIRECTION('center_axis',(0.,0.,-1.));
#21588=DIRECTION('ref_axis',(0.499999999999999,-0.866025403784439,0.));
#21589=DIRECTION('',(0.,0.,-1.));
#21590=DIRECTION('center_axis',(0.,0.,-1.));
#21591=DIRECTION('ref_axis',(0.499999999999999,-0.866025403784439,0.));
#21592=DIRECTION('',(0.,0.,-1.));
#21593=DIRECTION('center_axis',(0.,0.,-1.));
#21594=DIRECTION('ref_axis',(0.499999999999999,-0.866025403784439,0.));
#21595=DIRECTION('',(0.,0.,-1.));
#21596=DIRECTION('center_axis',(0.,0.,-1.));
#21597=DIRECTION('ref_axis',(0.499999999999999,-0.866025403784439,0.));
#21598=DIRECTION('',(0.,0.,-1.));
#21599=DIRECTION('center_axis',(0.,0.,-1.));
#21600=DIRECTION('ref_axis',(0.499999999999999,-0.866025403784439,0.));
#21601=DIRECTION('',(0.,0.,-1.));
#21602=DIRECTION('center_axis',(0.,0.,-1.));
#21603=DIRECTION('ref_axis',(0.499999999999999,-0.866025403784439,0.));
#21604=DIRECTION('',(0.,0.,-1.));
#21605=DIRECTION('center_axis',(0.,0.,-1.));
#21606=DIRECTION('ref_axis',(0.167034001011813,-0.985951135962623,0.));
#21607=DIRECTION('',(0.,0.,-1.));
#21608=DIRECTION('center_axis',(0.,0.,1.));
#21609=DIRECTION('ref_axis',(0.499999999999999,-0.866025403784439,0.));
#21610=DIRECTION('center_axis',(0.,0.,-1.));
#21611=DIRECTION('ref_axis',(0.923947020235649,-0.382520461933299,0.));
#21612=DIRECTION('',(6.12323399573637E-17,-1.06057523872493E-16,-1.));
#21613=DIRECTION('center_axis',(0.,0.,1.));
#21614=DIRECTION('ref_axis',(0.499999999999968,-0.866025403784457,0.));
#21615=DIRECTION('center_axis',(0.,0.,-1.));
#21616=DIRECTION('ref_axis',(0.499999999999968,-0.866025403784457,0.));
#21617=DIRECTION('',(6.12323399573637E-17,-1.06057523872493E-16,-1.));
#21618=DIRECTION('center_axis',(0.,0.,-1.));
#21619=DIRECTION('ref_axis',(0.499999999999968,-0.866025403784457,0.));
#21620=DIRECTION('',(6.12323399573637E-17,-1.06057523872493E-16,-1.));
#21621=DIRECTION('center_axis',(0.,0.,-1.));
#21622=DIRECTION('ref_axis',(0.499999999999968,-0.866025403784457,0.));
#21623=DIRECTION('',(6.12323399573637E-17,-1.06057523872493E-16,-1.));
#21624=DIRECTION('center_axis',(0.,0.,-1.));
#21625=DIRECTION('ref_axis',(0.499999999999968,-0.866025403784457,0.));
#21626=DIRECTION('',(6.12323399573637E-17,-1.06057523872493E-16,-1.));
#21627=DIRECTION('center_axis',(0.,0.,-1.));
#21628=DIRECTION('ref_axis',(0.499999999999968,-0.866025403784457,0.));
#21629=DIRECTION('',(6.12323399573637E-17,-1.06057523872493E-16,-1.));
#21630=DIRECTION('center_axis',(0.,0.,-1.));
#21631=DIRECTION('ref_axis',(0.499999999999968,-0.866025403784457,0.));
#21632=DIRECTION('',(6.12323399573637E-17,-1.06057523872493E-16,-1.));
#21633=DIRECTION('center_axis',(0.,0.,-1.));
#21634=DIRECTION('ref_axis',(-0.99139252575924,0.130923106702811,0.));
#21635=DIRECTION('',(6.12323399573637E-17,-1.06057523872493E-16,-1.));
#21636=DIRECTION('center_axis',(0.,0.,-1.));
#21637=DIRECTION('ref_axis',(0.499999999999968,-0.866025403784457,0.));
#21638=DIRECTION('center_axis',(0.,0.,1.));
#21639=DIRECTION('ref_axis',(-0.5,-0.866025403784439,0.));
#21640=DIRECTION('',(0.,0.,1.));
#21641=DIRECTION('center_axis',(0.,0.,-1.));
#21642=DIRECTION('ref_axis',(-0.5,-0.866025403784439,0.));
#21643=DIRECTION('',(0.,0.,1.));
#21644=DIRECTION('center_axis',(0.,0.,-1.));
#21645=DIRECTION('ref_axis',(-0.5,-0.866025403784439,0.));
#21646=DIRECTION('center_axis',(0.,0.,-1.));
#21647=DIRECTION('ref_axis',(-0.5,-0.866025403784439,0.));
#21648=DIRECTION('center_axis',(0.,0.,-1.));
#21649=DIRECTION('ref_axis',(-0.5,-0.866025403784439,0.));
#21650=DIRECTION('center_axis',(0.,0.,-1.));
#21651=DIRECTION('ref_axis',(-0.5,-0.866025403784439,0.));
#21652=DIRECTION('center_axis',(0.,0.,1.));
#21653=DIRECTION('ref_axis',(-0.5,-0.866025403784439,0.));
#21654=DIRECTION('',(0.,0.,1.));
#21655=DIRECTION('center_axis',(0.,0.,1.));
#21656=DIRECTION('ref_axis',(-0.5,-0.866025403784439,0.));
#21657=DIRECTION('',(0.,0.,1.));
#21658=DIRECTION('center_axis',(0.,0.,1.));
#21659=DIRECTION('ref_axis',(-0.5,-0.866025403784439,0.));
#21660=DIRECTION('',(0.,0.,1.));
#21661=DIRECTION('center_axis',(0.,0.,1.));
#21662=DIRECTION('ref_axis',(-0.5,-0.866025403784439,0.));
#21663=DIRECTION('',(0.,0.,1.));
#21664=DIRECTION('center_axis',(0.,0.,1.));
#21665=DIRECTION('ref_axis',(-0.5,-0.866025403784439,0.));
#21666=DIRECTION('',(0.,0.,1.));
#21667=DIRECTION('center_axis',(0.,0.,1.));
#21668=DIRECTION('ref_axis',(-0.5,-0.866025403784439,0.));
#21669=DIRECTION('',(0.,0.,1.));
#21670=DIRECTION('center_axis',(0.,0.,1.));
#21671=DIRECTION('ref_axis',(-0.167031392512161,-0.985951577875632,0.));
#21672=DIRECTION('',(0.,0.,1.));
#21673=DIRECTION('center_axis',(0.,0.,-1.));
#21674=DIRECTION('ref_axis',(-0.5,-0.866025403784439,0.));
#21675=DIRECTION('center_axis',(0.,0.,1.));
#21676=DIRECTION('ref_axis',(-0.923947690185482,-0.382518843720034,0.));
#21677=DIRECTION('',(-6.12323399573653E-17,-1.06057523872492E-16,1.));
#21678=DIRECTION('center_axis',(0.,0.,-1.));
#21679=DIRECTION('ref_axis',(-0.499999999999981,-0.86602540378445,0.));
#21680=DIRECTION('center_axis',(0.,0.,1.));
#21681=DIRECTION('ref_axis',(-0.499999999999981,-0.86602540378445,0.));
#21682=DIRECTION('',(-6.12323399573653E-17,-1.06057523872492E-16,1.));
#21683=DIRECTION('center_axis',(0.,0.,1.));
#21684=DIRECTION('ref_axis',(-0.499999999999981,-0.86602540378445,0.));
#21685=DIRECTION('',(-6.12323399573653E-17,-1.06057523872492E-16,1.));
#21686=DIRECTION('center_axis',(0.,0.,1.));
#21687=DIRECTION('ref_axis',(-0.499999999999981,-0.86602540378445,0.));
#21688=DIRECTION('',(-6.12323399573653E-17,-1.06057523872492E-16,1.));
#21689=DIRECTION('center_axis',(0.,0.,1.));
#21690=DIRECTION('ref_axis',(-0.499999999999981,-0.86602540378445,0.));
#21691=DIRECTION('',(-6.12323399573653E-17,-1.06057523872492E-16,1.));
#21692=DIRECTION('center_axis',(0.,0.,1.));
#21693=DIRECTION('ref_axis',(-0.499999999999981,-0.86602540378445,0.));
#21694=DIRECTION('',(-6.12323399573653E-17,-1.06057523872492E-16,1.));
#21695=DIRECTION('center_axis',(0.,0.,1.));
#21696=DIRECTION('ref_axis',(-0.499999999999981,-0.86602540378445,0.));
#21697=DIRECTION('',(-6.12323399573653E-17,-1.06057523872492E-16,1.));
#21698=DIRECTION('center_axis',(0.,0.,1.));
#21699=DIRECTION('ref_axis',(0.99139229699987,0.130924838931818,0.));
#21700=DIRECTION('',(-6.12323399573653E-17,-1.06057523872492E-16,1.));
#21701=DIRECTION('center_axis',(0.,0.,1.));
#21702=DIRECTION('ref_axis',(-0.499999999999981,-0.86602540378445,0.));
#21703=DIRECTION('center_axis',(0.,0.,1.));
#21704=DIRECTION('ref_axis',(0.5,-0.866025403784439,0.));
#21705=DIRECTION('',(0.,0.,1.));
#21706=DIRECTION('center_axis',(0.,0.,-1.));
#21707=DIRECTION('ref_axis',(0.5,-0.866025403784439,0.));
#21708=DIRECTION('',(0.,0.,1.));
#21709=DIRECTION('center_axis',(0.,0.,-1.));
#21710=DIRECTION('ref_axis',(0.5,-0.866025403784439,0.));
#21711=DIRECTION('center_axis',(0.,0.,-1.));
#21712=DIRECTION('ref_axis',(0.5,-0.866025403784439,0.));
#21713=DIRECTION('center_axis',(0.,0.,-1.));
#21714=DIRECTION('ref_axis',(0.5,-0.866025403784439,0.));
#21715=DIRECTION('center_axis',(0.,0.,-1.));
#21716=DIRECTION('ref_axis',(0.5,-0.866025403784439,0.));
#21717=DIRECTION('center_axis',(0.,0.,1.));
#21718=DIRECTION('ref_axis',(0.5,-0.866025403784439,0.));
#21719=DIRECTION('',(0.,0.,1.));
#21720=DIRECTION('center_axis',(0.,0.,1.));
#21721=DIRECTION('ref_axis',(0.5,-0.866025403784439,0.));
#21722=DIRECTION('',(0.,0.,1.));
#21723=DIRECTION('center_axis',(0.,0.,1.));
#21724=DIRECTION('ref_axis',(0.5,-0.866025403784439,0.));
#21725=DIRECTION('',(0.,0.,1.));
#21726=DIRECTION('center_axis',(0.,0.,1.));
#21727=DIRECTION('ref_axis',(0.5,-0.866025403784439,0.));
#21728=DIRECTION('',(0.,0.,1.));
#21729=DIRECTION('center_axis',(0.,0.,1.));
#21730=DIRECTION('ref_axis',(0.5,-0.866025403784439,0.));
#21731=DIRECTION('',(0.,0.,1.));
#21732=DIRECTION('center_axis',(0.,0.,1.));
#21733=DIRECTION('ref_axis',(0.5,-0.866025403784439,0.));
#21734=DIRECTION('',(0.,0.,1.));
#21735=DIRECTION('center_axis',(0.,0.,1.));
#21736=DIRECTION('ref_axis',(0.770342508707589,-0.637630315526244,0.));
#21737=DIRECTION('',(0.,0.,1.));
#21738=DIRECTION('center_axis',(0.,0.,-1.));
#21739=DIRECTION('ref_axis',(0.5,-0.866025403784439,0.));
#21740=DIRECTION('center_axis',(0.,0.,1.));
#21741=DIRECTION('ref_axis',(-0.130701828608467,-0.991421722577432,0.));
#21742=DIRECTION('',(6.12323399573711E-17,-1.06057523872489E-16,1.));
#21743=DIRECTION('center_axis',(0.,0.,-1.));
#21744=DIRECTION('ref_axis',(0.500000000000028,-0.866025403784423,0.));
#21745=DIRECTION('center_axis',(0.,0.,1.));
#21746=DIRECTION('ref_axis',(0.500000000000028,-0.866025403784422,0.));
#21747=DIRECTION('',(6.12323399573711E-17,-1.06057523872489E-16,1.));
#21748=DIRECTION('center_axis',(0.,0.,1.));
#21749=DIRECTION('ref_axis',(0.500000000000028,-0.866025403784422,0.));
#21750=DIRECTION('',(6.12323399573711E-17,-1.06057523872489E-16,1.));
#21751=DIRECTION('center_axis',(0.,0.,1.));
#21752=DIRECTION('ref_axis',(0.500000000000028,-0.866025403784422,0.));
#21753=DIRECTION('',(6.12323399573711E-17,-1.06057523872489E-16,1.));
#21754=DIRECTION('center_axis',(0.,0.,1.));
#21755=DIRECTION('ref_axis',(0.500000000000028,-0.866025403784422,0.));
#21756=DIRECTION('',(6.12323399573711E-17,-1.06057523872489E-16,1.));
#21757=DIRECTION('center_axis',(0.,0.,1.));
#21758=DIRECTION('ref_axis',(0.500000000000028,-0.866025403784422,0.));
#21759=DIRECTION('',(6.12323399573711E-17,-1.06057523872489E-16,1.));
#21760=DIRECTION('center_axis',(0.,0.,1.));
#21761=DIRECTION('ref_axis',(0.500000000000028,-0.866025403784422,0.));
#21762=DIRECTION('',(6.12323399573711E-17,-1.06057523872489E-16,1.));
#21763=DIRECTION('center_axis',(0.,0.,1.));
#21764=DIRECTION('ref_axis',(0.382312780236439,0.924032974556582,0.));
#21765=DIRECTION('',(6.12323399573711E-17,-1.06057523872489E-16,1.));
#21766=DIRECTION('center_axis',(0.,0.,1.));
#21767=DIRECTION('ref_axis',(0.500000000000028,-0.866025403784422,0.));
#21768=DIRECTION('center_axis',(0.,0.,1.));
#21769=DIRECTION('ref_axis',(1.,-9.25185853854297E-17,0.));
#21770=DIRECTION('',(0.,0.,1.));
#21771=DIRECTION('center_axis',(0.,0.,-1.));
#21772=DIRECTION('ref_axis',(1.,-9.25185853854297E-17,0.));
#21773=DIRECTION('',(0.,0.,1.));
#21774=DIRECTION('center_axis',(0.,0.,-1.));
#21775=DIRECTION('ref_axis',(1.,-9.25185853854297E-17,0.));
#21776=DIRECTION('center_axis',(0.,0.,-1.));
#21777=DIRECTION('ref_axis',(1.,-9.25185853854297E-17,0.));
#21778=DIRECTION('center_axis',(0.,0.,-1.));
#21779=DIRECTION('ref_axis',(1.,-9.25185853854297E-17,0.));
#21780=DIRECTION('center_axis',(0.,0.,-1.));
#21781=DIRECTION('ref_axis',(1.,-9.25185853854297E-17,0.));
#21782=DIRECTION('center_axis',(0.,0.,1.));
#21783=DIRECTION('ref_axis',(1.,-9.25185853854297E-17,0.));
#21784=DIRECTION('',(0.,0.,1.));
#21785=DIRECTION('center_axis',(0.,0.,1.));
#21786=DIRECTION('ref_axis',(1.,-9.25185853854297E-17,0.));
#21787=DIRECTION('',(0.,0.,1.));
#21788=DIRECTION('center_axis',(0.,0.,1.));
#21789=DIRECTION('ref_axis',(1.,-9.25185853854297E-17,0.));
#21790=DIRECTION('',(0.,0.,1.));
#21791=DIRECTION('center_axis',(0.,0.,1.));
#21792=DIRECTION('ref_axis',(1.,-9.25185853854297E-17,0.));
#21793=DIRECTION('',(0.,0.,1.));
#21794=DIRECTION('center_axis',(0.,0.,1.));
#21795=DIRECTION('ref_axis',(1.,-9.25185853854297E-17,0.));
#21796=DIRECTION('',(0.,0.,1.));
#21797=DIRECTION('center_axis',(0.,0.,1.));
#21798=DIRECTION('ref_axis',(1.,-9.25185853854297E-17,0.));
#21799=DIRECTION('',(0.,0.,1.));
#21800=DIRECTION('center_axis',(0.,0.,1.));
#21801=DIRECTION('ref_axis',(0.937374823573167,0.34832232218331,0.));
#21802=DIRECTION('',(0.,0.,1.));
#21803=DIRECTION('center_axis',(0.,0.,-1.));
#21804=DIRECTION('ref_axis',(1.,-9.25185853854297E-17,0.));
#21805=DIRECTION('center_axis',(0.,0.,1.));
#21806=DIRECTION('ref_axis',(0.793244897475736,-0.608902728380083,0.));
#21807=DIRECTION('',(1.22464679914735E-16,3.89210500104523E-30,1.));
#21808=DIRECTION('center_axis',(0.,0.,-1.));
#21809=DIRECTION('ref_axis',(1.,3.16589845000044E-14,0.));
#21810=DIRECTION('center_axis',(0.,0.,1.));
#21811=DIRECTION('ref_axis',(1.,3.16589845000044E-14,0.));
#21812=DIRECTION('',(1.22464679914735E-16,3.89210500104523E-30,1.));
#21813=DIRECTION('center_axis',(0.,0.,1.));
#21814=DIRECTION('ref_axis',(1.,3.16589845000044E-14,0.));
#21815=DIRECTION('',(1.22464679914735E-16,3.89210500104523E-30,1.));
#21816=DIRECTION('center_axis',(0.,0.,1.));
#21817=DIRECTION('ref_axis',(1.,3.16589845000044E-14,0.));
#21818=DIRECTION('',(1.22464679914735E-16,3.89210500104523E-30,1.));
#21819=DIRECTION('center_axis',(0.,0.,1.));
#21820=DIRECTION('ref_axis',(1.,3.16589845000044E-14,0.));
#21821=DIRECTION('',(1.22464679914735E-16,3.89210500104523E-30,1.));
#21822=DIRECTION('center_axis',(0.,0.,1.));
#21823=DIRECTION('ref_axis',(1.,3.16589845000044E-14,0.));
#21824=DIRECTION('',(1.22464679914735E-16,3.89210500104523E-30,1.));
#21825=DIRECTION('center_axis',(0.,0.,1.));
#21826=DIRECTION('ref_axis',(1.,3.16589845000044E-14,0.));
#21827=DIRECTION('',(1.22464679914735E-16,3.89210500104523E-30,1.));
#21828=DIRECTION('center_axis',(0.,0.,1.));
#21829=DIRECTION('ref_axis',(-0.609080360598175,0.793108513592936,0.));
#21830=DIRECTION('',(1.22464679914735E-16,3.89210500104523E-30,1.));
#21831=DIRECTION('center_axis',(0.,0.,1.));
#21832=DIRECTION('ref_axis',(1.,3.16589845000044E-14,0.));
#21833=DIRECTION('center_axis',(0.,0.,1.));
#21834=DIRECTION('ref_axis',(0.5,0.866025403784438,0.));
#21835=DIRECTION('',(0.,0.,1.));
#21836=DIRECTION('center_axis',(0.,0.,-1.));
#21837=DIRECTION('ref_axis',(0.5,0.866025403784438,0.));
#21838=DIRECTION('',(0.,0.,1.));
#21839=DIRECTION('center_axis',(0.,0.,-1.));
#21840=DIRECTION('ref_axis',(0.5,0.866025403784438,0.));
#21841=DIRECTION('center_axis',(0.,0.,-1.));
#21842=DIRECTION('ref_axis',(0.5,0.866025403784438,0.));
#21843=DIRECTION('center_axis',(0.,0.,-1.));
#21844=DIRECTION('ref_axis',(0.5,0.866025403784438,0.));
#21845=DIRECTION('center_axis',(0.,0.,-1.));
#21846=DIRECTION('ref_axis',(0.5,0.866025403784438,0.));
#21847=DIRECTION('center_axis',(0.,0.,1.));
#21848=DIRECTION('ref_axis',(0.5,0.866025403784438,0.));
#21849=DIRECTION('',(0.,0.,1.));
#21850=DIRECTION('center_axis',(0.,0.,1.));
#21851=DIRECTION('ref_axis',(0.5,0.866025403784438,0.));
#21852=DIRECTION('',(0.,0.,1.));
#21853=DIRECTION('center_axis',(0.,0.,1.));
#21854=DIRECTION('ref_axis',(0.5,0.866025403784438,0.));
#21855=DIRECTION('',(0.,0.,1.));
#21856=DIRECTION('center_axis',(0.,0.,1.));
#21857=DIRECTION('ref_axis',(0.5,0.866025403784438,0.));
#21858=DIRECTION('',(0.,0.,1.));
#21859=DIRECTION('center_axis',(0.,0.,1.));
#21860=DIRECTION('ref_axis',(0.5,0.866025403784438,0.));
#21861=DIRECTION('',(0.,0.,1.));
#21862=DIRECTION('center_axis',(0.,0.,1.));
#21863=DIRECTION('ref_axis',(0.5,0.866025403784438,0.));
#21864=DIRECTION('',(0.,0.,1.));
#21865=DIRECTION('center_axis',(0.,0.,1.));
#21866=DIRECTION('ref_axis',(0.167031392512228,0.98595157787562,0.));
#21867=DIRECTION('',(0.,0.,1.));
#21868=DIRECTION('center_axis',(0.,0.,-1.));
#21869=DIRECTION('ref_axis',(0.5,0.866025403784438,0.));
#21870=DIRECTION('center_axis',(0.,0.,1.));
#21871=DIRECTION('ref_axis',(0.923947690185483,0.382518843720034,0.));
#21872=DIRECTION('',(6.12323399573657E-17,1.06057523872492E-16,1.));
#21873=DIRECTION('center_axis',(0.,0.,-1.));
#21874=DIRECTION('ref_axis',(0.499999999999984,0.866025403784448,0.));
#21875=DIRECTION('center_axis',(0.,0.,1.));
#21876=DIRECTION('ref_axis',(0.499999999999984,0.866025403784448,0.));
#21877=DIRECTION('',(6.12323399573657E-17,1.06057523872492E-16,1.));
#21878=DIRECTION('center_axis',(0.,0.,1.));
#21879=DIRECTION('ref_axis',(0.499999999999984,0.866025403784448,0.));
#21880=DIRECTION('',(6.12323399573657E-17,1.06057523872492E-16,1.));
#21881=DIRECTION('center_axis',(0.,0.,1.));
#21882=DIRECTION('ref_axis',(0.499999999999984,0.866025403784448,0.));
#21883=DIRECTION('',(6.12323399573657E-17,1.06057523872492E-16,1.));
#21884=DIRECTION('center_axis',(0.,0.,1.));
#21885=DIRECTION('ref_axis',(0.499999999999984,0.866025403784448,0.));
#21886=DIRECTION('',(6.12323399573657E-17,1.06057523872492E-16,1.));
#21887=DIRECTION('center_axis',(0.,0.,1.));
#21888=DIRECTION('ref_axis',(0.499999999999984,0.866025403784448,0.));
#21889=DIRECTION('',(6.12323399573657E-17,1.06057523872492E-16,1.));
#21890=DIRECTION('center_axis',(0.,0.,1.));
#21891=DIRECTION('ref_axis',(0.499999999999984,0.866025403784448,0.));
#21892=DIRECTION('',(6.12323399573657E-17,1.06057523872492E-16,1.));
#21893=DIRECTION('center_axis',(0.,0.,1.));
#21894=DIRECTION('ref_axis',(-0.991392296999871,-0.130924838931808,0.));
#21895=DIRECTION('',(6.12323399573657E-17,1.06057523872492E-16,1.));
#21896=DIRECTION('center_axis',(0.,0.,1.));
#21897=DIRECTION('ref_axis',(0.499999999999984,0.866025403784448,0.));
#21898=DIRECTION('center_axis',(0.,0.,1.));
#21899=DIRECTION('ref_axis',(-0.499999999999999,0.866025403784439,0.));
#21900=DIRECTION('',(0.,0.,1.));
#21901=DIRECTION('center_axis',(0.,0.,-1.));
#21902=DIRECTION('ref_axis',(-0.499999999999999,0.866025403784439,0.));
#21903=DIRECTION('',(0.,0.,1.));
#21904=DIRECTION('center_axis',(0.,0.,-1.));
#21905=DIRECTION('ref_axis',(-0.499999999999999,0.866025403784439,0.));
#21906=DIRECTION('center_axis',(0.,0.,-1.));
#21907=DIRECTION('ref_axis',(-0.499999999999999,0.866025403784439,0.));
#21908=DIRECTION('center_axis',(0.,0.,-1.));
#21909=DIRECTION('ref_axis',(-0.499999999999999,0.866025403784439,0.));
#21910=DIRECTION('center_axis',(0.,0.,-1.));
#21911=DIRECTION('ref_axis',(-0.499999999999999,0.866025403784439,0.));
#21912=DIRECTION('center_axis',(0.,0.,1.));
#21913=DIRECTION('ref_axis',(-0.499999999999999,0.866025403784439,0.));
#21914=DIRECTION('',(0.,0.,1.));
#21915=DIRECTION('center_axis',(0.,0.,1.));
#21916=DIRECTION('ref_axis',(-0.499999999999999,0.866025403784439,0.));
#21917=DIRECTION('',(0.,0.,1.));
#21918=DIRECTION('center_axis',(0.,0.,1.));
#21919=DIRECTION('ref_axis',(-0.499999999999999,0.866025403784439,0.));
#21920=DIRECTION('',(0.,0.,1.));
#21921=DIRECTION('center_axis',(0.,0.,1.));
#21922=DIRECTION('ref_axis',(-0.499999999999999,0.866025403784439,0.));
#21923=DIRECTION('',(0.,0.,1.));
#21924=DIRECTION('center_axis',(0.,0.,1.));
#21925=DIRECTION('ref_axis',(-0.499999999999999,0.866025403784439,0.));
#21926=DIRECTION('',(0.,0.,1.));
#21927=DIRECTION('center_axis',(0.,0.,1.));
#21928=DIRECTION('ref_axis',(-0.499999999999999,0.866025403784439,0.));
#21929=DIRECTION('',(0.,0.,1.));
#21930=DIRECTION('center_axis',(0.,0.,1.));
#21931=DIRECTION('ref_axis',(-0.770342508707554,0.637630315526286,0.));
#21932=DIRECTION('',(0.,0.,1.));
#21933=DIRECTION('center_axis',(0.,0.,-1.));
#21934=DIRECTION('ref_axis',(-0.499999999999999,0.866025403784439,0.));
#21935=DIRECTION('center_axis',(0.,0.,1.));
#21936=DIRECTION('ref_axis',(0.130701828608463,0.991421722577433,0.));
#21937=DIRECTION('',(-6.12323399573709E-17,1.06057523872489E-16,1.));
#21938=DIRECTION('center_axis',(0.,0.,-1.));
#21939=DIRECTION('ref_axis',(-0.500000000000026,0.866025403784424,0.));
#21940=DIRECTION('center_axis',(0.,0.,1.));
#21941=DIRECTION('ref_axis',(-0.500000000000026,0.866025403784424,0.));
#21942=DIRECTION('',(-6.12323399573709E-17,1.06057523872489E-16,1.));
#21943=DIRECTION('center_axis',(0.,0.,1.));
#21944=DIRECTION('ref_axis',(-0.500000000000026,0.866025403784424,0.));
#21945=DIRECTION('',(-6.12323399573709E-17,1.06057523872489E-16,1.));
#21946=DIRECTION('center_axis',(0.,0.,1.));
#21947=DIRECTION('ref_axis',(-0.500000000000026,0.866025403784424,0.));
#21948=DIRECTION('',(-6.12323399573709E-17,1.06057523872489E-16,1.));
#21949=DIRECTION('center_axis',(0.,0.,1.));
#21950=DIRECTION('ref_axis',(-0.500000000000026,0.866025403784424,0.));
#21951=DIRECTION('',(-6.12323399573709E-17,1.06057523872489E-16,1.));
#21952=DIRECTION('center_axis',(0.,0.,1.));
#21953=DIRECTION('ref_axis',(-0.500000000000026,0.866025403784424,0.));
#21954=DIRECTION('',(-6.12323399573709E-17,1.06057523872489E-16,1.));
#21955=DIRECTION('center_axis',(0.,0.,1.));
#21956=DIRECTION('ref_axis',(-0.500000000000026,0.866025403784424,0.));
#21957=DIRECTION('',(-6.12323399573709E-17,1.06057523872489E-16,1.));
#21958=DIRECTION('center_axis',(0.,0.,1.));
#21959=DIRECTION('ref_axis',(-0.382312780236439,-0.924032974556582,0.));
#21960=DIRECTION('',(-6.12323399573709E-17,1.06057523872489E-16,1.));
#21961=DIRECTION('center_axis',(0.,0.,1.));
#21962=DIRECTION('ref_axis',(-0.500000000000026,0.866025403784424,0.));
#21963=DIRECTION('center_axis',(0.,-1.,0.));
#21964=DIRECTION('ref_axis',(-1.,0.,0.));
#21965=DIRECTION('',(0.,0.,-1.));
#21966=DIRECTION('',(-1.,0.,0.));
#21967=DIRECTION('',(0.,0.,-1.));
#21968=DIRECTION('',(1.,0.,0.));
#21969=DIRECTION('center_axis',(1.,0.,0.));
#21970=DIRECTION('ref_axis',(0.,-1.,0.));
#21971=DIRECTION('',(0.,-1.,0.));
#21972=DIRECTION('',(0.,0.,-1.));
#21973=DIRECTION('',(0.,1.,0.));
#21974=DIRECTION('center_axis',(0.,1.,0.));
#21975=DIRECTION('ref_axis',(1.,0.,0.));
#21976=DIRECTION('',(0.,0.,1.));
#21977=DIRECTION('',(-1.,0.,0.));
#21978=DIRECTION('',(1.,0.,0.));
#21979=DIRECTION('center_axis',(0.,0.,-1.));
#21980=DIRECTION('ref_axis',(-1.,0.,0.));
#21981=DIRECTION('',(0.939692620785908,-0.342020143325669,0.));
#21982=DIRECTION('center_axis',(0.,0.,1.));
#21983=DIRECTION('ref_axis',(-0.901760301405889,-0.43223646168314,0.));
#21984=DIRECTION('center_axis',(0.,0.,-1.));
#21985=DIRECTION('ref_axis',(0.939692620785908,-0.34202014332567,0.));
#21986=DIRECTION('',(0.4486637512204,-0.893700642464152,0.));
#21987=DIRECTION('',(0.893700642464153,0.4486637512204,0.));
#21988=DIRECTION('',(-0.4486637512204,0.893700642464153,0.));
#21989=DIRECTION('',(-0.893700642464153,-0.4486637512204,0.));
#21990=DIRECTION('',(0.766044443118978,0.64278760968654,0.));
#21991=DIRECTION('center_axis',(0.,0.,1.));
#21992=DIRECTION('ref_axis',(-0.0765523944434513,-0.997065559983382,0.));
#21993=DIRECTION('center_axis',(0.,0.,-1.));
#21994=DIRECTION('ref_axis',(0.766044443118978,0.642787609686539,0.));
#21995=DIRECTION('',(0.99829933536263,-0.058296114917988,0.));
#21996=DIRECTION('',(0.0582961149179888,0.99829933536263,0.));
#21997=DIRECTION('',(-0.99829933536263,0.0582961149179891,0.));
#21998=DIRECTION('',(-0.0582961149179891,-0.99829933536263,0.));
#21999=DIRECTION('',(-0.173648177666931,0.984807753012208,0.));
#22000=DIRECTION('center_axis',(0.,0.,1.));
#22001=DIRECTION('ref_axis',(0.825207906962445,-0.564829098300239,0.));
#22002=DIRECTION('center_axis',(0.,0.,-1.));
#22003=DIRECTION('ref_axis',(-0.173648177666929,0.984807753012208,0.));
#22004=DIRECTION('',(0.54963558414223,0.835404527546164,0.));
#22005=DIRECTION('',(-0.835404527546164,0.54963558414223,0.));
#22006=DIRECTION('',(-0.54963558414223,-0.835404527546164,0.));
#22007=DIRECTION('',(0.835404527546164,-0.54963558414223,0.));
#22008=DIRECTION('',(-0.939692620785909,0.342020143325668,0.));
#22009=DIRECTION('center_axis',(0.,0.,1.));
#22010=DIRECTION('ref_axis',(0.901760301405891,0.432236461683135,0.));
#22011=DIRECTION('center_axis',(0.,0.,-1.));
#22012=DIRECTION('ref_axis',(-0.939692620785908,0.342020143325669,0.));
#22013=DIRECTION('',(-0.4486637512204,0.893700642464152,0.));
#22014=DIRECTION('',(-0.893700642464153,-0.4486637512204,0.));
#22015=DIRECTION('',(0.448663751220399,-0.893700642464153,0.));
#22016=DIRECTION('',(0.893700642464153,0.448663751220399,0.));
#22017=DIRECTION('',(-0.766044443118978,-0.64278760968654,0.));
#22018=DIRECTION('center_axis',(0.,0.,1.));
#22019=DIRECTION('ref_axis',(0.0765523944434456,0.997065559983382,0.));
#22020=DIRECTION('center_axis',(0.,0.,-1.));
#22021=DIRECTION('ref_axis',(-0.766044443118979,-0.642787609686539,0.));
#22022=DIRECTION('',(-0.99829933536263,0.0582961149179884,0.));
#22023=DIRECTION('',(-0.0582961149179891,-0.99829933536263,0.));
#22024=DIRECTION('',(0.99829933536263,-0.0582961149179895,0.));
#22025=DIRECTION('',(0.0582961149179895,0.99829933536263,0.));
#22026=DIRECTION('',(0.173648177666931,-0.984807753012208,0.));
#22027=DIRECTION('center_axis',(0.,0.,1.));
#22028=DIRECTION('ref_axis',(-0.82520790696244,0.564829098300246,0.));
#22029=DIRECTION('center_axis',(0.,0.,-1.));
#22030=DIRECTION('ref_axis',(0.173648177666929,-0.984807753012208,0.));
#22031=DIRECTION('',(-0.54963558414223,-0.835404527546164,0.));
#22032=DIRECTION('',(0.835404527546163,-0.549635584142231,0.));
#22033=DIRECTION('',(0.549635584142231,0.835404527546163,0.));
#22034=DIRECTION('',(-0.835404527546163,0.549635584142231,0.));
#22035=DIRECTION('center_axis',(0.,0.,1.));
#22036=DIRECTION('ref_axis',(1.,0.,0.));
#22037=DIRECTION('center_axis',(0.,0.,1.));
#22038=DIRECTION('ref_axis',(1.,0.,0.));
#22039=DIRECTION('center_axis',(0.,0.,1.));
#22040=DIRECTION('ref_axis',(-0.500000000000026,0.866025403784424,0.));
#22041=DIRECTION('center_axis',(0.,0.,1.));
#22042=DIRECTION('ref_axis',(-0.499999999999999,0.866025403784439,0.));
#22043=DIRECTION('center_axis',(0.,0.,1.));
#22044=DIRECTION('ref_axis',(1.,0.,0.));
#22045=DIRECTION('center_axis',(0.,0.,1.));
#22046=DIRECTION('ref_axis',(0.499999999999984,0.866025403784448,0.));
#22047=DIRECTION('center_axis',(0.,0.,1.));
#22048=DIRECTION('ref_axis',(0.5,0.866025403784438,0.));
#22049=DIRECTION('center_axis',(0.,0.,1.));
#22050=DIRECTION('ref_axis',(1.,0.,0.));
#22051=DIRECTION('center_axis',(0.,0.,1.));
#22052=DIRECTION('ref_axis',(1.,3.16589845000044E-14,0.));
#22053=DIRECTION('center_axis',(0.,0.,1.));
#22054=DIRECTION('ref_axis',(1.,-9.25185853854297E-17,0.));
#22055=DIRECTION('center_axis',(0.,0.,1.));
#22056=DIRECTION('ref_axis',(1.,0.,0.));
#22057=DIRECTION('center_axis',(0.,0.,1.));
#22058=DIRECTION('ref_axis',(0.500000000000028,-0.866025403784422,0.));
#22059=DIRECTION('center_axis',(0.,0.,1.));
#22060=DIRECTION('ref_axis',(0.5,-0.866025403784439,0.));
#22061=DIRECTION('center_axis',(0.,0.,1.));
#22062=DIRECTION('ref_axis',(1.,0.,0.));
#22063=DIRECTION('center_axis',(0.,0.,1.));
#22064=DIRECTION('ref_axis',(-0.499999999999981,-0.86602540378445,0.));
#22065=DIRECTION('center_axis',(0.,0.,1.));
#22066=DIRECTION('ref_axis',(-0.5,-0.866025403784439,0.));
#22067=DIRECTION('center_axis',(0.,0.,1.));
#22068=DIRECTION('ref_axis',(-0.499999999999999,0.866025403784439,0.));
#22069=DIRECTION('',(0.54963558414223,0.835404527546164,0.));
#22070=DIRECTION('center_axis',(0.,0.,1.));
#22071=DIRECTION('ref_axis',(-0.499999999999999,0.866025403784439,0.));
#22072=DIRECTION('',(0.54963558414223,0.835404527546164,0.));
#22073=DIRECTION('center_axis',(0.,0.,1.));
#22074=DIRECTION('ref_axis',(0.5,0.866025403784438,0.));
#22075=DIRECTION('',(0.99829933536263,-0.0582961149179893,-3.10967490252419E-18));
#22076=DIRECTION('center_axis',(0.,0.,1.));
#22077=DIRECTION('ref_axis',(0.5,0.866025403784438,0.));
#22078=DIRECTION('',(0.99829933536263,-0.0582961149179893,-3.10967490252419E-18));
#22079=DIRECTION('center_axis',(0.,0.,1.));
#22080=DIRECTION('ref_axis',(1.,-1.66533453693773E-16,0.));
#22081=DIRECTION('',(0.4486637512204,-0.893700642464152,2.01331172658311E-19));
#22082=DIRECTION('center_axis',(0.,0.,1.));
#22083=DIRECTION('ref_axis',(1.,-1.66533453693773E-16,0.));
#22084=DIRECTION('',(0.4486637512204,-0.893700642464152,2.01331172658311E-19));
#22085=DIRECTION('center_axis',(0.,0.,1.));
#22086=DIRECTION('ref_axis',(0.5,-0.866025403784439,0.));
#22087=DIRECTION('',(-0.54963558414223,-0.835404527546164,-1.46475409989076E-17));
#22088=DIRECTION('center_axis',(0.,0.,1.));
#22089=DIRECTION('ref_axis',(0.5,-0.866025403784439,0.));
#22090=DIRECTION('',(-0.54963558414223,-0.835404527546164,-1.46475409989076E-17));
#22091=DIRECTION('center_axis',(0.,0.,1.));
#22092=DIRECTION('ref_axis',(-0.5,-0.866025403784439,0.));
#22093=DIRECTION('',(-0.99829933536263,0.0582961149179884,-2.12383052760723E-18));
#22094=DIRECTION('center_axis',(0.,0.,1.));
#22095=DIRECTION('ref_axis',(-0.5,-0.866025403784439,0.));
#22096=DIRECTION('',(-0.99829933536263,0.0582961149179884,-2.12383052760723E-18));
#22097=DIRECTION('center_axis',(0.,0.,1.));
#22098=DIRECTION('ref_axis',(1.,0.,0.));
#22099=DIRECTION('center_axis',(0.,0.,-1.));
#22100=DIRECTION('ref_axis',(0.499999999999968,-0.866025403784457,0.));
#22101=DIRECTION('center_axis',(0.,0.,-1.));
#22102=DIRECTION('ref_axis',(0.499999999999999,-0.866025403784439,0.));
#22103=DIRECTION('center_axis',(0.,0.,1.));
#22104=DIRECTION('ref_axis',(1.,0.,0.));
#22105=DIRECTION('center_axis',(0.,0.,-1.));
#22106=DIRECTION('ref_axis',(-0.500000000000029,-0.866025403784422,0.));
#22107=DIRECTION('center_axis',(0.,0.,-1.));
#22108=DIRECTION('ref_axis',(-0.5,-0.866025403784438,0.));
#22109=DIRECTION('center_axis',(0.,0.,1.));
#22110=DIRECTION('ref_axis',(1.,0.,0.));
#22111=DIRECTION('center_axis',(0.,0.,-1.));
#22112=DIRECTION('ref_axis',(-1.,2.15856712500029E-14,0.));
#22113=DIRECTION('center_axis',(0.,0.,-1.));
#22114=DIRECTION('ref_axis',(-1.,9.25185853854297E-17,0.));
#22115=DIRECTION('center_axis',(0.,0.,1.));
#22116=DIRECTION('ref_axis',(1.,0.,0.));
#22117=DIRECTION('center_axis',(0.,0.,-1.));
#22118=DIRECTION('ref_axis',(-0.499999999999964,0.86602540378446,0.));
#22119=DIRECTION('center_axis',(0.,0.,-1.));
#22120=DIRECTION('ref_axis',(-0.5,0.866025403784439,0.));
#22121=DIRECTION('center_axis',(0.,0.,1.));
#22122=DIRECTION('ref_axis',(1.,0.,0.));
#22123=DIRECTION('center_axis',(0.,0.,-1.));
#22124=DIRECTION('ref_axis',(0.500000000000046,0.866025403784412,0.));
#22125=DIRECTION('center_axis',(0.,0.,-1.));
#22126=DIRECTION('ref_axis',(0.5,0.866025403784439,0.));
#22127=DIRECTION('center_axis',(0.,0.,-1.));
#22128=DIRECTION('ref_axis',(0.499999999999999,-0.866025403784439,0.));
#22129=DIRECTION('',(0.54963558414223,0.835404527546164,0.));
#22130=DIRECTION('center_axis',(0.,0.,-1.));
#22131=DIRECTION('ref_axis',(0.499999999999999,-0.866025403784439,0.));
#22132=DIRECTION('',(0.54963558414223,0.835404527546164,0.));
#22133=DIRECTION('center_axis',(0.,0.,-1.));
#22134=DIRECTION('ref_axis',(-0.5,-0.866025403784438,0.));
#22135=DIRECTION('',(0.99829933536263,-0.0582961149179893,-3.10967490252419E-18));
#22136=DIRECTION('center_axis',(0.,0.,-1.));
#22137=DIRECTION('ref_axis',(-0.5,-0.866025403784438,0.));
#22138=DIRECTION('',(0.99829933536263,-0.0582961149179893,-3.10967490252419E-18));
#22139=DIRECTION('center_axis',(0.,0.,-1.));
#22140=DIRECTION('ref_axis',(-1.,1.66533453693773E-16,0.));
#22141=DIRECTION('',(0.4486637512204,-0.893700642464152,2.01331172658311E-19));
#22142=DIRECTION('center_axis',(0.,0.,-1.));
#22143=DIRECTION('ref_axis',(-1.,1.66533453693773E-16,0.));
#22144=DIRECTION('',(0.4486637512204,-0.893700642464152,2.01331172658311E-19));
#22145=DIRECTION('center_axis',(0.,0.,-1.));
#22146=DIRECTION('ref_axis',(-0.5,0.866025403784439,0.));
#22147=DIRECTION('',(-0.54963558414223,-0.835404527546164,-1.46475409989076E-17));
#22148=DIRECTION('center_axis',(0.,0.,-1.));
#22149=DIRECTION('ref_axis',(-0.5,0.866025403784439,0.));
#22150=DIRECTION('',(-0.54963558414223,-0.835404527546164,-1.46475409989076E-17));
#22151=DIRECTION('center_axis',(0.,0.,-1.));
#22152=DIRECTION('ref_axis',(0.5,0.866025403784439,0.));
#22153=DIRECTION('',(-0.99829933536263,0.0582961149179884,-2.12383052760723E-18));
#22154=DIRECTION('center_axis',(0.,0.,-1.));
#22155=DIRECTION('ref_axis',(0.5,0.866025403784439,0.));
#22156=DIRECTION('',(-0.99829933536263,0.0582961149179884,-2.12383052760723E-18));
#22157=DIRECTION('center_axis',(0.,0.,1.));
#22158=DIRECTION('ref_axis',(1.,0.,0.));
#22159=DIRECTION('center_axis',(0.,0.,1.));
#22160=DIRECTION('ref_axis',(-1.,-1.72685370000025E-14,0.));
#22161=DIRECTION('center_axis',(0.,0.,1.));
#22162=DIRECTION('ref_axis',(-1.,0.,0.));
#22163=DIRECTION('center_axis',(0.,0.,1.));
#22164=DIRECTION('ref_axis',(-1.,0.,0.));
#22165=DIRECTION('',(-0.4486637512204,0.893700642464152,2.01331172658311E-19));
#22166=DIRECTION('center_axis',(0.,0.,1.));
#22167=DIRECTION('ref_axis',(-1.,0.,0.));
#22168=DIRECTION('',(-0.4486637512204,0.893700642464152,2.01331172658311E-19));
#22169=DIRECTION('center_axis',(0.,0.,1.));
#22170=DIRECTION('ref_axis',(1.,0.,0.));
#22171=DIRECTION('center_axis',(0.,0.,-1.));
#22172=DIRECTION('ref_axis',(1.,-3.45370740000048E-14,0.));
#22173=DIRECTION('center_axis',(0.,0.,-1.));
#22174=DIRECTION('ref_axis',(1.,0.,0.));
#22175=DIRECTION('center_axis',(0.,0.,-1.));
#22176=DIRECTION('ref_axis',(1.,0.,0.));
#22177=DIRECTION('',(-0.4486637512204,0.893700642464152,2.01331172658311E-19));
#22178=DIRECTION('center_axis',(0.,0.,-1.));
#22179=DIRECTION('ref_axis',(1.,0.,0.));
#22180=DIRECTION('',(-0.4486637512204,0.893700642464152,2.01331172658311E-19));
#22181=DIRECTION('center_axis',(-0.54963558414223,-0.835404527546164,0.));
#22182=DIRECTION('ref_axis',(0.,0.,1.));
#22183=DIRECTION('center_axis',(-0.54963558414223,-0.835404527546164,0.));
#22184=DIRECTION('ref_axis',(0.,0.,1.));
#22185=DIRECTION('',(-0.54963558414223,-0.835404527546164,0.));
#22186=DIRECTION('center_axis',(0.549635584142231,0.835404527546164,0.));
#22187=DIRECTION('ref_axis',(0.,0.,1.));
#22188=DIRECTION('center_axis',(-0.54963558414223,-0.835404527546164,0.));
#22189=DIRECTION('ref_axis',(0.,0.,1.));
#22190=DIRECTION('center_axis',(-0.549635584142231,-0.835404527546163,0.));
#22191=DIRECTION('ref_axis',(0.,0.,1.));
#22192=DIRECTION('',(-0.54963558414223,-0.835404527546164,0.));
#22193=DIRECTION('',(-0.54963558414223,-0.835404527546164,0.));
#22194=DIRECTION('center_axis',(-0.54963558414223,-0.835404527546164,0.));
#22195=DIRECTION('ref_axis',(0.,0.,1.));
#22196=DIRECTION('center_axis',(-0.54963558414223,-0.835404527546164,0.));
#22197=DIRECTION('ref_axis',(0.,0.,1.));
#22198=DIRECTION('center_axis',(-0.99829933536263,0.0582961149179893,3.10967490252419E-18));
#22199=DIRECTION('ref_axis',(0.0582961149179893,0.99829933536263,0.));
#22200=DIRECTION('center_axis',(-0.99829933536263,0.0582961149179893,3.10967490252419E-18));
#22201=DIRECTION('ref_axis',(0.0582961149179893,0.99829933536263,0.));
#22202=DIRECTION('',(-0.99829933536263,0.0582961149179893,3.10967490252419E-18));
#22203=DIRECTION('center_axis',(0.99829933536263,-0.0582961149179891,0.));
#22204=DIRECTION('ref_axis',(0.0582961149179893,0.99829933536263,0.));
#22205=DIRECTION('center_axis',(-0.99829933536263,0.0582961149179893,3.10967490252419E-18));
#22206=DIRECTION('ref_axis',(-2.31296463463574E-17,-1.84314369322536E-16,
1.));
#22207=DIRECTION('center_axis',(-0.99829933536263,0.0582961149179895,0.));
#22208=DIRECTION('ref_axis',(0.0582961149179893,0.99829933536263,0.));
#22209=DIRECTION('',(-0.99829933536263,0.0582961149179893,3.10967490252419E-18));
#22210=DIRECTION('',(-0.99829933536263,0.0582961149179893,3.10967490252419E-18));
#22211=DIRECTION('center_axis',(-0.99829933536263,0.0582961149179893,3.10967490252419E-18));
#22212=DIRECTION('ref_axis',(0.0582961149179893,0.99829933536263,0.));
#22213=DIRECTION('center_axis',(-0.99829933536263,0.0582961149179893,3.10967490252419E-18));
#22214=DIRECTION('ref_axis',(0.0582961149179893,0.99829933536263,0.));
#22215=DIRECTION('center_axis',(-0.4486637512204,0.893700642464152,-2.01331172658311E-19));
#22216=DIRECTION('ref_axis',(0.,-2.2527808876045E-19,-1.));
#22217=DIRECTION('center_axis',(-0.4486637512204,0.893700642464152,-2.01331172658311E-19));
#22218=DIRECTION('ref_axis',(0.,-2.2527808876045E-19,-1.));
#22219=DIRECTION('',(-0.4486637512204,0.893700642464152,-2.01331172658311E-19));
#22220=DIRECTION('center_axis',(0.4486637512204,-0.893700642464153,0.));
#22221=DIRECTION('ref_axis',(0.,-2.2527808876045E-19,-1.));
#22222=DIRECTION('center_axis',(-0.4486637512204,0.893700642464152,-2.01331172658311E-19));
#22223=DIRECTION('ref_axis',(-1.09446763118966E-16,-5.47201845937903E-17,
1.));
#22224=DIRECTION('center_axis',(-0.448663751220399,0.893700642464153,0.));
#22225=DIRECTION('ref_axis',(0.,-2.2527808876045E-19,-1.));
#22226=DIRECTION('',(-0.4486637512204,0.893700642464152,-2.01331172658311E-19));
#22227=DIRECTION('',(-0.4486637512204,0.893700642464152,-2.01331172658311E-19));
#22228=DIRECTION('center_axis',(-0.4486637512204,0.893700642464152,-2.01331172658311E-19));
#22229=DIRECTION('ref_axis',(0.,-2.2527808876045E-19,-1.));
#22230=DIRECTION('center_axis',(-0.4486637512204,0.893700642464152,-2.01331172658311E-19));
#22231=DIRECTION('ref_axis',(0.,-2.2527808876045E-19,-1.));
#22232=DIRECTION('center_axis',(0.54963558414223,0.835404527546164,1.46475409989076E-17));
#22233=DIRECTION('ref_axis',(0.,1.75334709304627E-17,-1.));
#22234=DIRECTION('center_axis',(0.54963558414223,0.835404527546164,1.46475409989076E-17));
#22235=DIRECTION('ref_axis',(0.,1.75334709304627E-17,-1.));
#22236=DIRECTION('',(0.54963558414223,0.835404527546164,1.46475409989076E-17));
#22237=DIRECTION('center_axis',(-0.54963558414223,-0.835404527546164,0.));
#22238=DIRECTION('ref_axis',(0.,1.75334709304627E-17,-1.));
#22239=DIRECTION('center_axis',(0.54963558414223,0.835404527546164,1.46475409989076E-17));
#22240=DIRECTION('ref_axis',(2.12365727119358E-15,-1.41474591865194E-15,
1.));
#22241=DIRECTION('center_axis',(0.549635584142231,0.835404527546164,0.));
#22242=DIRECTION('ref_axis',(0.,1.75334709304627E-17,-1.));
#22243=DIRECTION('',(0.54963558414223,0.835404527546164,1.46475409989076E-17));
#22244=DIRECTION('',(0.54963558414223,0.835404527546164,1.46475409989076E-17));
#22245=DIRECTION('center_axis',(0.54963558414223,0.835404527546164,1.46475409989076E-17));
#22246=DIRECTION('ref_axis',(0.,1.75334709304627E-17,-1.));
#22247=DIRECTION('center_axis',(0.54963558414223,0.835404527546164,1.46475409989076E-17));
#22248=DIRECTION('ref_axis',(0.,1.75334709304627E-17,-1.));
#22249=DIRECTION('center_axis',(0.99829933536263,-0.0582961149179884,2.12383052760723E-18));
#22250=DIRECTION('ref_axis',(-0.0582961149179884,-0.99829933536263,0.));
#22251=DIRECTION('center_axis',(0.99829933536263,-0.0582961149179884,2.12383052760723E-18));
#22252=DIRECTION('ref_axis',(-0.0582961149179884,-0.99829933536263,0.));
#22253=DIRECTION('',(0.99829933536263,-0.0582961149179884,2.12383052760723E-18));
#22254=DIRECTION('center_axis',(-0.99829933536263,0.0582961149179888,0.));
#22255=DIRECTION('ref_axis',(-0.0582961149179884,-0.99829933536263,0.));
#22256=DIRECTION('center_axis',(0.99829933536263,-0.0582961149179884,2.12383052760723E-18));
#22257=DIRECTION('ref_axis',(6.93889390390723E-17,1.07046894496735E-15,
1.));
#22258=DIRECTION('center_axis',(0.99829933536263,-0.0582961149179891,0.));
#22259=DIRECTION('ref_axis',(-0.0582961149179884,-0.99829933536263,0.));
#22260=DIRECTION('',(0.99829933536263,-0.0582961149179884,2.12383052760723E-18));
#22261=DIRECTION('',(0.99829933536263,-0.0582961149179884,2.12383052760723E-18));
#22262=DIRECTION('center_axis',(0.99829933536263,-0.0582961149179884,2.12383052760723E-18));
#22263=DIRECTION('ref_axis',(-0.0582961149179884,-0.99829933536263,0.));
#22264=DIRECTION('center_axis',(0.99829933536263,-0.0582961149179884,2.12383052760723E-18));
#22265=DIRECTION('ref_axis',(-0.0582961149179884,-0.99829933536263,0.));
#22266=DIRECTION('center_axis',(0.4486637512204,-0.893700642464152,-2.01331172658311E-19));
#22267=DIRECTION('ref_axis',(0.,-2.2527808876045E-19,1.));
#22268=DIRECTION('center_axis',(0.4486637512204,-0.893700642464152,-2.01331172658311E-19));
#22269=DIRECTION('ref_axis',(0.,-2.2527808876045E-19,1.));
#22270=DIRECTION('',(0.4486637512204,-0.893700642464152,-2.01331172658311E-19));
#22271=DIRECTION('center_axis',(-0.4486637512204,0.893700642464153,0.));
#22272=DIRECTION('ref_axis',(0.,-2.2527808876045E-19,1.));
#22273=DIRECTION('center_axis',(0.4486637512204,-0.893700642464152,-2.01331172658311E-19));
#22274=DIRECTION('ref_axis',(0.,-2.2527808876045E-19,1.));
#22275=DIRECTION('center_axis',(0.4486637512204,-0.893700642464153,0.));
#22276=DIRECTION('ref_axis',(0.,-2.2527808876045E-19,1.));
#22277=DIRECTION('',(0.4486637512204,-0.893700642464152,-2.01331172658311E-19));
#22278=DIRECTION('',(0.4486637512204,-0.893700642464152,-2.01331172658311E-19));
#22279=DIRECTION('center_axis',(0.4486637512204,-0.893700642464152,-2.01331172658311E-19));
#22280=DIRECTION('ref_axis',(0.,-2.2527808876045E-19,1.));
#22281=DIRECTION('center_axis',(0.4486637512204,-0.893700642464152,-2.01331172658311E-19));
#22282=DIRECTION('ref_axis',(0.,-2.2527808876045E-19,1.));
#22283=DIRECTION('center_axis',(-0.835404527546164,0.54963558414223,0.));
#22284=DIRECTION('ref_axis',(-0.54963558414223,-0.835404527546164,0.));
#22285=DIRECTION('',(-0.54963558414223,-0.835404527546164,0.));
#22286=DIRECTION('',(0.,0.,1.));
#22287=DIRECTION('center_axis',(0.549635584142231,0.835404527546163,0.));
#22288=DIRECTION('ref_axis',(-0.835404527546163,0.549635584142231,0.));
#22289=DIRECTION('',(0.,0.,1.));
#22290=DIRECTION('',(-0.835404527546163,0.549635584142231,0.));
#22291=DIRECTION('center_axis',(0.835404527546163,-0.549635584142231,0.));
#22292=DIRECTION('ref_axis',(0.549635584142231,0.835404527546163,0.));
#22293=DIRECTION('',(0.549635584142231,0.835404527546163,0.));
#22294=DIRECTION('',(0.,0.,1.));
#22295=DIRECTION('center_axis',(-0.549635584142231,-0.835404527546164,0.));
#22296=DIRECTION('ref_axis',(0.835404527546163,-0.549635584142231,0.));
#22297=DIRECTION('',(0.835404527546163,-0.549635584142231,0.));
#22298=DIRECTION('center_axis',(0.99829933536263,-0.0582961149179895,0.));
#22299=DIRECTION('ref_axis',(0.0582961149179895,0.99829933536263,0.));
#22300=DIRECTION('',(0.,0.,1.));
#22301=DIRECTION('',(0.0582961149179895,0.99829933536263,0.));
#22302=DIRECTION('center_axis',(-0.0582961149179895,-0.99829933536263,0.));
#22303=DIRECTION('ref_axis',(0.99829933536263,-0.0582961149179895,0.));
#22304=DIRECTION('',(0.99829933536263,-0.0582961149179895,0.));
#22305=DIRECTION('',(0.,0.,1.));
#22306=DIRECTION('center_axis',(-0.99829933536263,0.0582961149179891,0.));
#22307=DIRECTION('ref_axis',(-0.0582961149179891,-0.99829933536263,0.));
#22308=DIRECTION('',(-0.0582961149179891,-0.99829933536263,0.));
#22309=DIRECTION('',(0.,0.,1.));
#22310=DIRECTION('center_axis',(0.0582961149179884,0.99829933536263,0.));
#22311=DIRECTION('ref_axis',(-0.99829933536263,0.0582961149179884,0.));
#22312=DIRECTION('',(-0.99829933536263,0.0582961149179884,0.));
#22313=DIRECTION('center_axis',(0.448663751220399,-0.893700642464153,0.));
#22314=DIRECTION('ref_axis',(0.893700642464153,0.448663751220399,0.));
#22315=DIRECTION('',(0.,0.,1.));
#22316=DIRECTION('',(0.893700642464153,0.448663751220399,0.));
#22317=DIRECTION('center_axis',(-0.893700642464153,-0.448663751220399,0.));
#22318=DIRECTION('ref_axis',(0.448663751220399,-0.893700642464153,0.));
#22319=DIRECTION('',(0.448663751220399,-0.893700642464153,0.));
#22320=DIRECTION('',(0.,0.,1.));
#22321=DIRECTION('center_axis',(-0.4486637512204,0.893700642464153,0.));
#22322=DIRECTION('ref_axis',(-0.893700642464153,-0.4486637512204,0.));
#22323=DIRECTION('',(-0.893700642464153,-0.4486637512204,0.));
#22324=DIRECTION('',(0.,0.,1.));
#22325=DIRECTION('center_axis',(0.893700642464152,0.4486637512204,0.));
#22326=DIRECTION('ref_axis',(-0.448663751220401,0.893700642464152,0.));
#22327=DIRECTION('',(-0.4486637512204,0.893700642464152,0.));
#22328=DIRECTION('center_axis',(-0.549635584142231,-0.835404527546164,0.));
#22329=DIRECTION('ref_axis',(0.835404527546164,-0.54963558414223,0.));
#22330=DIRECTION('',(0.,0.,1.));
#22331=DIRECTION('',(0.835404527546164,-0.54963558414223,0.));
#22332=DIRECTION('center_axis',(-0.835404527546164,0.549635584142231,0.));
#22333=DIRECTION('ref_axis',(-0.54963558414223,-0.835404527546164,0.));
#22334=DIRECTION('',(-0.54963558414223,-0.835404527546164,0.));
#22335=DIRECTION('',(0.,0.,1.));
#22336=DIRECTION('center_axis',(0.54963558414223,0.835404527546164,0.));
#22337=DIRECTION('ref_axis',(-0.835404527546164,0.54963558414223,0.));
#22338=DIRECTION('',(-0.835404527546164,0.54963558414223,0.));
#22339=DIRECTION('',(0.,0.,1.));
#22340=DIRECTION('center_axis',(0.835404527546164,-0.54963558414223,0.));
#22341=DIRECTION('ref_axis',(0.54963558414223,0.835404527546164,0.));
#22342=DIRECTION('',(0.54963558414223,0.835404527546164,0.));
#22343=DIRECTION('center_axis',(-0.058296114917988,-0.99829933536263,0.));
#22344=DIRECTION('ref_axis',(0.99829933536263,-0.058296114917988,0.));
#22345=DIRECTION('',(0.99829933536263,-0.058296114917988,0.));
#22346=DIRECTION('',(0.,0.,1.));
#22347=DIRECTION('center_axis',(-0.99829933536263,0.0582961149179891,0.));
#22348=DIRECTION('ref_axis',(-0.0582961149179891,-0.99829933536263,0.));
#22349=DIRECTION('',(0.,0.,1.));
#22350=DIRECTION('',(-0.0582961149179891,-0.99829933536263,0.));
#22351=DIRECTION('center_axis',(0.0582961149179891,0.99829933536263,0.));
#22352=DIRECTION('ref_axis',(-0.99829933536263,0.0582961149179891,0.));
#22353=DIRECTION('',(-0.99829933536263,0.0582961149179891,0.));
#22354=DIRECTION('',(0.,0.,1.));
#22355=DIRECTION('center_axis',(0.99829933536263,-0.0582961149179888,0.));
#22356=DIRECTION('ref_axis',(0.0582961149179888,0.99829933536263,0.));
#22357=DIRECTION('',(0.0582961149179888,0.99829933536263,0.));
#22358=DIRECTION('',(0.,0.,-1.));
#22359=DIRECTION('',(0.,0.,-1.));
#22360=DIRECTION('',(0.,0.,1.));
#22361=DIRECTION('',(0.,0.,-1.));
#22362=DIRECTION('',(0.,0.,1.));
#22363=DIRECTION('',(0.,0.,-1.));
#22364=DIRECTION('',(0.,0.,1.));
#22365=DIRECTION('',(0.,0.,-1.));
#22366=DIRECTION('center_axis',(-0.893700642464152,-0.448663751220401,0.));
#22367=DIRECTION('ref_axis',(0.448663751220401,-0.893700642464152,0.));
#22368=DIRECTION('',(0.4486637512204,-0.893700642464152,0.));
#22369=DIRECTION('',(0.,0.,1.));
#22370=DIRECTION('center_axis',(-0.4486637512204,0.893700642464153,0.));
#22371=DIRECTION('ref_axis',(-0.893700642464153,-0.4486637512204,0.));
#22372=DIRECTION('',(0.,0.,1.));
#22373=DIRECTION('',(-0.893700642464153,-0.4486637512204,0.));
#22374=DIRECTION('center_axis',(0.893700642464153,0.4486637512204,0.));
#22375=DIRECTION('ref_axis',(-0.4486637512204,0.893700642464153,0.));
#22376=DIRECTION('',(-0.4486637512204,0.893700642464153,0.));
#22377=DIRECTION('',(0.,0.,1.));
#22378=DIRECTION('center_axis',(0.4486637512204,-0.893700642464153,0.));
#22379=DIRECTION('ref_axis',(0.893700642464153,0.4486637512204,0.));
#22380=DIRECTION('',(0.893700642464153,0.4486637512204,0.));
#22381=DIRECTION('',(0.,0.,-1.));
#22382=DIRECTION('center_axis',(0.,0.,1.));
#22383=DIRECTION('ref_axis',(-0.766044443118979,-0.642787609686539,0.));
#22384=DIRECTION('',(0.,0.,1.));
#22385=DIRECTION('center_axis',(0.,0.,1.));
#22386=DIRECTION('ref_axis',(-0.766044443118979,-0.642787609686539,0.));
#22387=DIRECTION('center_axis',(0.,0.,1.));
#22388=DIRECTION('ref_axis',(0.0765523944434456,0.997065559983382,0.));
#22389=DIRECTION('',(0.,0.,-1.));
#22390=DIRECTION('center_axis',(0.,0.,-1.));
#22391=DIRECTION('ref_axis',(0.0765523944434456,0.997065559983382,0.));
#22392=DIRECTION('center_axis',(-0.64278760968654,0.766044443118978,0.));
#22393=DIRECTION('ref_axis',(-0.766044443118978,-0.64278760968654,0.));
#22394=DIRECTION('',(0.766044443118978,0.64278760968654,0.));
#22395=DIRECTION('center_axis',(0.,0.,1.));
#22396=DIRECTION('ref_axis',(-0.939692620785908,0.342020143325669,0.));
#22397=DIRECTION('',(0.,0.,1.));
#22398=DIRECTION('center_axis',(0.,0.,1.));
#22399=DIRECTION('ref_axis',(-0.939692620785908,0.342020143325669,0.));
#22400=DIRECTION('center_axis',(0.,0.,1.));
#22401=DIRECTION('ref_axis',(0.901760301405891,0.432236461683135,0.));
#22402=DIRECTION('',(0.,0.,-1.));
#22403=DIRECTION('center_axis',(0.,0.,-1.));
#22404=DIRECTION('ref_axis',(0.901760301405891,0.432236461683135,0.));
#22405=DIRECTION('center_axis',(0.342020143325668,0.939692620785909,0.));
#22406=DIRECTION('ref_axis',(-0.939692620785909,0.342020143325668,0.));
#22407=DIRECTION('',(0.939692620785909,-0.342020143325668,0.));
#22408=DIRECTION('center_axis',(0.,0.,1.));
#22409=DIRECTION('ref_axis',(-0.173648177666929,0.984807753012208,0.));
#22410=DIRECTION('',(0.,0.,1.));
#22411=DIRECTION('center_axis',(0.,0.,1.));
#22412=DIRECTION('ref_axis',(-0.173648177666929,0.984807753012208,0.));
#22413=DIRECTION('center_axis',(0.,0.,1.));
#22414=DIRECTION('ref_axis',(0.825207906962445,-0.564829098300239,0.));
#22415=DIRECTION('',(0.,0.,-1.));
#22416=DIRECTION('center_axis',(0.,0.,-1.));
#22417=DIRECTION('ref_axis',(0.825207906962445,-0.564829098300239,0.));
#22418=DIRECTION('center_axis',(0.984807753012208,0.173648177666931,0.));
#22419=DIRECTION('ref_axis',(-0.173648177666931,0.984807753012208,0.));
#22420=DIRECTION('',(0.173648177666931,-0.984807753012208,0.));
#22421=DIRECTION('center_axis',(0.,0.,1.));
#22422=DIRECTION('ref_axis',(1.,0.,0.));
#22423=DIRECTION('center_axis',(0.,0.,1.));
#22424=DIRECTION('ref_axis',(0.173648177666929,-0.984807753012208,0.));
#22425=DIRECTION('center_axis',(0.,0.,-1.));
#22426=DIRECTION('ref_axis',(-0.82520790696244,0.564829098300246,0.));
#22427=DIRECTION('',(-0.173648177666931,0.984807753012208,0.));
#22428=DIRECTION('center_axis',(0.,0.,1.));
#22429=DIRECTION('ref_axis',(0.766044443118978,0.642787609686539,0.));
#22430=DIRECTION('center_axis',(0.,0.,-1.));
#22431=DIRECTION('ref_axis',(-0.0765523944434513,-0.997065559983382,0.));
#22432=DIRECTION('',(-0.766044443118978,-0.64278760968654,0.));
#22433=DIRECTION('center_axis',(0.,0.,1.));
#22434=DIRECTION('ref_axis',(0.939692620785908,-0.34202014332567,0.));
#22435=DIRECTION('center_axis',(0.,0.,-1.));
#22436=DIRECTION('ref_axis',(-0.901760301405889,-0.43223646168314,0.));
#22437=DIRECTION('',(-0.939692620785908,0.342020143325669,0.));
#22438=DIRECTION('center_axis',(0.,0.,-1.));
#22439=DIRECTION('ref_axis',(1.,0.,0.));
#22440=DIRECTION('center_axis',(-0.984807753012208,-0.173648177666931,0.));
#22441=DIRECTION('ref_axis',(0.173648177666931,-0.984807753012208,0.));
#22442=DIRECTION('',(0.,0.,-1.));
#22443=DIRECTION('center_axis',(0.,0.,1.));
#22444=DIRECTION('ref_axis',(-0.82520790696244,0.564829098300246,0.));
#22445=DIRECTION('',(0.,0.,1.));
#22446=DIRECTION('center_axis',(0.,0.,1.));
#22447=DIRECTION('ref_axis',(0.173648177666929,-0.984807753012208,0.));
#22448=DIRECTION('',(0.,0.,1.));
#22449=DIRECTION('center_axis',(-0.342020143325669,-0.939692620785908,0.));
#22450=DIRECTION('ref_axis',(0.939692620785908,-0.342020143325669,0.));
#22451=DIRECTION('',(0.,0.,-1.));
#22452=DIRECTION('center_axis',(0.,0.,1.));
#22453=DIRECTION('ref_axis',(-0.901760301405889,-0.43223646168314,0.));
#22454=DIRECTION('',(0.,0.,1.));
#22455=DIRECTION('center_axis',(0.,0.,1.));
#22456=DIRECTION('ref_axis',(0.939692620785908,-0.34202014332567,0.));
#22457=DIRECTION('',(0.,0.,1.));
#22458=DIRECTION('center_axis',(0.64278760968654,-0.766044443118978,0.));
#22459=DIRECTION('ref_axis',(0.766044443118978,0.64278760968654,0.));
#22460=DIRECTION('',(0.,0.,-1.));
#22461=DIRECTION('',(0.,0.,1.));
#22462=DIRECTION('center_axis',(0.,0.,1.));
#22463=DIRECTION('ref_axis',(-0.0765523944434513,-0.997065559983382,0.));
#22464=DIRECTION('',(0.,0.,1.));
#22465=DIRECTION('center_axis',(0.,0.,1.));
#22466=DIRECTION('ref_axis',(0.766044443118978,0.642787609686539,0.));
#22467=DIRECTION('center_axis',(0.,0.,1.));
#22468=DIRECTION('ref_axis',(-1.,1.22464679914735E-16,0.));
#52671=CARTESIAN_POINT('',(0.,0.,0.));
#52672=CARTESIAN_POINT('Origin',(53.1951359564886,14.3971354987959,15.5));
#52673=CARTESIAN_POINT('',(51.9326028526449,14.3970877066932,14.1934196736194));
#52674=CARTESIAN_POINT('',(51.9314232360955,14.3954626592386,14.0565803263806));
#52675=CARTESIAN_POINT('',(51.9306359564886,14.3971354987959,15.5));
#52676=CARTESIAN_POINT('',(52.2370198037663,15.2223467977324,14.));
#52677=CARTESIAN_POINT('Ctrl Pts',(51.9314232360955,14.3954626592386,14.0565803263806));
#52678=CARTESIAN_POINT('Ctrl Pts',(51.9340308380707,14.6945947257524,14.0377202175871));
#52679=CARTESIAN_POINT('Ctrl Pts',(52.0414421537953,14.9952702831595,14.0188601087935));
#52680=CARTESIAN_POINT('Ctrl Pts',(52.2370198037663,15.2223467977324,14.));
#52681=CARTESIAN_POINT('',(51.9306359564886,14.3971354987959,14.));
#52682=CARTESIAN_POINT('Origin',(53.1951359564886,14.3971354987959,14.));
#52683=CARTESIAN_POINT('',(51.9306359564886,14.3971354987959,13.));
#52684=CARTESIAN_POINT('',(51.9306359564886,14.3971354987959,15.5));
#52685=CARTESIAN_POINT('',(52.6278006430704,15.5272199611918,13.));
#52686=CARTESIAN_POINT('Origin',(53.1951359564886,14.3971354987959,13.));
#52687=CARTESIAN_POINT('',(53.7624712699068,13.2670510364,13.));
#52688=CARTESIAN_POINT('Origin',(53.1951359564886,14.3971354987959,13.));
#52689=CARTESIAN_POINT('Origin',(53.1951359564886,14.3971354987959,13.));
#52690=CARTESIAN_POINT('',(54.1550391816747,15.2234704396199,14.));
#52691=CARTESIAN_POINT('Origin',(53.1951359564886,14.3971354987959,14.));
#52692=CARTESIAN_POINT('Ctrl Pts',(54.1550492157916,15.2234767486837,14.));
#52693=CARTESIAN_POINT('Ctrl Pts',(53.8967914626893,15.5213134049997,14.024908160387));
#52694=CARTESIAN_POINT('Ctrl Pts',(53.487740680999,15.6908539055355,14.049816320774));
#52695=CARTESIAN_POINT('Ctrl Pts',(53.0948318338552,15.6595885868543,14.074724481161));
#52696=CARTESIAN_POINT('Ctrl Pts',(52.6820419543228,15.626741255404,14.1008929846199));
#52697=CARTESIAN_POINT('Ctrl Pts',(52.2870688888724,15.3722525873919,14.1270614880789));
#52698=CARTESIAN_POINT('Ctrl Pts',(52.0867822938008,15.0099588798403,14.1532299915378));
#52699=CARTESIAN_POINT('Ctrl Pts',(51.9842486685495,14.8244882185226,14.1666265522317));
#52700=CARTESIAN_POINT('Ctrl Pts',(51.9327378835252,14.6107643391081,14.1800231129255));
#52701=CARTESIAN_POINT('Ctrl Pts',(51.9326028526449,14.3970877066932,14.1934196736194));
#52702=CARTESIAN_POINT('Origin',(53.1951359564886,14.3971354987959,15.5));
#52703=CARTESIAN_POINT('',(51.9293004715569,14.396357843321,14.6934196736194));
#52704=CARTESIAN_POINT('',(51.9290361749446,14.3977594574901,14.5565803263806));
#52705=CARTESIAN_POINT('',(51.9306359564886,14.3971354987959,15.5));
#52706=CARTESIAN_POINT('Ctrl Pts',(51.9290361749446,14.3977594574901,14.5565803263806));
#52707=CARTESIAN_POINT('Ctrl Pts',(51.9288104788003,14.4349272053691,14.5542330751329));
#52708=CARTESIAN_POINT('Ctrl Pts',(51.9303086019301,14.4720763914416,14.5518858238852));
#52709=CARTESIAN_POINT('Ctrl Pts',(51.9335904462524,14.5090671744586,14.5495385726375));
#52710=CARTESIAN_POINT('Ctrl Pts',(51.9701783294547,14.9214616440634,14.5233700691785));
#52711=CARTESIAN_POINT('Ctrl Pts',(52.228466159159,15.3141680878373,14.4972015657196));
#52712=CARTESIAN_POINT('Ctrl Pts',(52.5926396873008,15.5111367764164,14.4710330622607));
#52713=CARTESIAN_POINT('Ctrl Pts',(52.9568132154426,15.7081054649956,14.4448645588018));
#52714=CARTESIAN_POINT('Ctrl Pts',(53.4268724420219,15.7093363983799,14.4186960553428));
#52715=CARTESIAN_POINT('Ctrl Pts',(53.7920269612472,15.514187779113,14.3925275518839));
#52716=CARTESIAN_POINT('Ctrl Pts',(54.1571814804725,15.3190391598462,14.366359048425));
#52717=CARTESIAN_POINT('Ctrl Pts',(54.417431292344,14.9275109879282,14.340190544966));
#52718=CARTESIAN_POINT('Ctrl Pts',(54.4560979757245,14.5153505128056,14.3140220415071));
#52719=CARTESIAN_POINT('Ctrl Pts',(54.4947646591051,14.103190037683,14.2878535380482));
#52720=CARTESIAN_POINT('Ctrl Pts',(54.3118482139948,13.6703972593558,14.2616850345893));
#52721=CARTESIAN_POINT('Ctrl Pts',(53.9893291901183,13.4106746119161,14.2355165311303));
#52722=CARTESIAN_POINT('Ctrl Pts',(53.6668101662417,13.1509519644765,14.2093480276714));
#52723=CARTESIAN_POINT('Ctrl Pts',(53.2046885635989,13.0642994479243,14.1831795242125));
#52724=CARTESIAN_POINT('Ctrl Pts',(52.8102658096442,13.1903246291658,14.1570110207536));
#52725=CARTESIAN_POINT('Ctrl Pts',(52.4158430556895,13.3163498104073,14.1308425172946));
#52726=CARTESIAN_POINT('Ctrl Pts',(52.089119150423,13.6550526894425,14.1046740138357));
#52727=CARTESIAN_POINT('Ctrl Pts',(51.976572074359,14.0527844617314,14.0785055103768));
#52728=CARTESIAN_POINT('Ctrl Pts',(51.9451396903252,14.163863827329,14.0711971157114));
#52729=CARTESIAN_POINT('Ctrl Pts',(51.9304127761573,14.2795473576308,14.063888721046));
#52730=CARTESIAN_POINT('Ctrl Pts',(51.9314232360955,14.3954626592386,14.0565803263806));
#52731=CARTESIAN_POINT('Ctrl Pts',(51.9326028526449,14.3970877066932,14.1934196736194));
#52732=CARTESIAN_POINT('Ctrl Pts',(51.9324741176125,14.1933737996841,14.2061916163845));
#52733=CARTESIAN_POINT('Ctrl Pts',(51.9790420088886,13.9897028365794,14.2189635591495));
#52734=CARTESIAN_POINT('Ctrl Pts',(52.0726123421383,13.8105984338676,14.2317355019146));
#52735=CARTESIAN_POINT('Ctrl Pts',(52.2643291102402,13.4436304425376,14.2579040053735));
#52736=CARTESIAN_POINT('Ctrl Pts',(52.6533627711367,13.1797932069689,14.2840725088324));
#52737=CARTESIAN_POINT('Ctrl Pts',(53.0652069371965,13.1373261840987,14.3102410122914));
#52738=CARTESIAN_POINT('Ctrl Pts',(53.4770511032563,13.0948591612284,14.3364095157503));
#52739=CARTESIAN_POINT('Ctrl Pts',(53.9117057744794,13.2737623510566,14.3625780192092));
#52740=CARTESIAN_POINT('Ctrl Pts',(54.174295890408,13.5938472660216,14.3887465226681));
#52741=CARTESIAN_POINT('Ctrl Pts',(54.4368860063367,13.9139321809865,14.4149150261271));
#52742=CARTESIAN_POINT('Ctrl Pts',(54.5274115669709,14.3751988210882,14.441083529586));
#52743=CARTESIAN_POINT('Ctrl Pts',(54.4052653400132,14.7707929840486,14.4672520330449));
#52744=CARTESIAN_POINT('Ctrl Pts',(54.2831191130554,15.1663871470091,14.4934205365038));
#52745=CARTESIAN_POINT('Ctrl Pts',(53.9483010985055,15.4963088328283,14.5195890399628));
#52746=CARTESIAN_POINT('Ctrl Pts',(53.550954854306,15.6126255371819,14.5457575434217));
#52747=CARTESIAN_POINT('Ctrl Pts',(53.1536086101064,15.7289422415355,14.5719260468806));
#52748=CARTESIAN_POINT('Ctrl Pts',(52.6937341362572,15.6316539644235,14.5980945503396));
#52749=CARTESIAN_POINT('Ctrl Pts',(52.3775410563803,15.3643818135364,14.6242630537985));
#52750=CARTESIAN_POINT('Ctrl Pts',(52.0990020785416,15.1289379773151,14.6473152604055));
#52751=CARTESIAN_POINT('Ctrl Pts',(51.9319612775611,14.7615849808525,14.6703674670124));
#52752=CARTESIAN_POINT('Ctrl Pts',(51.9293004715569,14.396357843321,14.6934196736194));
#52753=CARTESIAN_POINT('Origin',(53.1951359564886,14.3971354987959,15.5));
#52754=CARTESIAN_POINT('',(51.9308136275137,14.3982246453427,15.1934196736194));
#52755=CARTESIAN_POINT('',(51.932525975067,14.3974029423036,15.0565803263806));
#52756=CARTESIAN_POINT('',(51.9306359564886,14.3971354987959,15.5));
#52757=CARTESIAN_POINT('Ctrl Pts',(51.932525975067,14.3974029423036,15.0565803263806));
#52758=CARTESIAN_POINT('Ctrl Pts',(51.9321561072822,14.5888155966727,15.0445774292198));
#52759=CARTESIAN_POINT('Ctrl Pts',(51.9730705675611,14.7800782049927,15.0325745320589));
#52760=CARTESIAN_POINT('Ctrl Pts',(52.0560982976485,14.9508677919232,15.0205716348981));
#52761=CARTESIAN_POINT('Ctrl Pts',(52.2371138818755,15.323220219546,14.9944031314392));
#52762=CARTESIAN_POINT('Ctrl Pts',(52.6183020364058,15.5982603906742,14.9682346279803));
#52763=CARTESIAN_POINT('Ctrl Pts',(53.028733536876,15.6526576817852,14.9420661245214));
#52764=CARTESIAN_POINT('Ctrl Pts',(53.4391650373463,15.7070549728961,14.9158976210624));
#52765=CARTESIAN_POINT('Ctrl Pts',(53.8788398837565,15.5408093839899,14.8897291176035));
#52766=CARTESIAN_POINT('Ctrl Pts',(54.1506024967829,15.2284660841227,14.8635606141446));
#52767=CARTESIAN_POINT('Ctrl Pts',(54.4223651098093,14.9161227842554,14.8373921106856));
#52768=CARTESIAN_POINT('Ctrl Pts',(54.5262154894519,14.4576817734273,14.8112236072267));
#52769=CARTESIAN_POINT('Ctrl Pts',(54.4155861975138,14.0587161328242,14.7850551037678));
#52770=CARTESIAN_POINT('Ctrl Pts',(54.3049569055756,13.6597504922211,14.7588866003089));
#52771=CARTESIAN_POINT('Ctrl Pts',(53.9798479420568,13.320260221843,14.7327180968499));
#52772=CARTESIAN_POINT('Ctrl Pts',(53.5860414121493,13.1924713804069,14.706549593391));
#52773=CARTESIAN_POINT('Ctrl Pts',(53.1922348822418,13.0646825389707,14.6803810899321));
#52774=CARTESIAN_POINT('Ctrl Pts',(52.7297307859455,13.1485951264765,14.6542125864732));
#52775=CARTESIAN_POINT('Ctrl Pts',(52.4059227061476,13.4065926679472,14.6280440830142));
#52776=CARTESIAN_POINT('Ctrl Pts',(52.1111594252056,13.6414484561238,14.604222830803));
#52777=CARTESIAN_POINT('Ctrl Pts',(51.9313266688913,14.0205598299628,14.5804015785918));
#52778=CARTESIAN_POINT('Ctrl Pts',(51.9290361749446,14.3977594574901,14.5565803263806));
#52779=CARTESIAN_POINT('Ctrl Pts',(51.9293004715569,14.396357843321,14.6934196736194));
#52780=CARTESIAN_POINT('Ctrl Pts',(51.9289407723092,14.3469848614482,14.6965359704714));
#52781=CARTESIAN_POINT('Ctrl Pts',(51.9315850846113,14.2976507292224,14.6996522673233));
#52782=CARTESIAN_POINT('Ctrl Pts',(51.9373640512186,14.2486865756559,14.7027685641753));
#52783=CARTESIAN_POINT('Ctrl Pts',(51.985891811838,13.8375195133245,14.7289370676342));
#52784=CARTESIAN_POINT('Ctrl Pts',(52.2554590189813,13.452441413324,14.7551055710931));
#52785=CARTESIAN_POINT('Ctrl Pts',(52.6251876598399,13.2661248639499,14.781274074552));
#52786=CARTESIAN_POINT('Ctrl Pts',(52.9949163006986,13.0798083145759,14.807442578011));
#52787=CARTESIAN_POINT('Ctrl Pts',(53.4648063752726,13.0922533158284,14.8336110814699));
#52788=CARTESIAN_POINT('Ctrl Pts',(53.8241540209967,13.2978798810904,14.8597795849288));
#52789=CARTESIAN_POINT('Ctrl Pts',(54.1835016667209,13.5035064463524,14.8859480883877));
#52790=CARTESIAN_POINT('Ctrl Pts',(54.4323068835952,13.902314575624,14.9121165918467));
#52791=CARTESIAN_POINT('Ctrl Pts',(54.4590022406867,14.3154737155563,14.9382850953056));
#52792=CARTESIAN_POINT('Ctrl Pts',(54.4856975977781,14.7286328554886,14.9644535987645));
#52793=CARTESIAN_POINT('Ctrl Pts',(54.2902830950867,15.1561430060816,14.9906221022235));
#52794=CARTESIAN_POINT('Ctrl Pts',(53.9603850245763,15.4063036567383,15.0167906056824));
#52795=CARTESIAN_POINT('Ctrl Pts',(53.6304869540658,15.656464307395,15.0429591091413));
#52796=CARTESIAN_POINT('Ctrl Pts',(53.1661053157362,15.7292754581154,15.0691276126002));
#52797=CARTESIAN_POINT('Ctrl Pts',(52.7754743036767,15.592087662659,15.0952961160592));
#52798=CARTESIAN_POINT('Ctrl Pts',(52.3848432916172,15.4548998672026,15.1214646195181));
#52799=CARTESIAN_POINT('Ctrl Pts',(52.0679629058276,15.1077131255694,15.147633122977));
#52800=CARTESIAN_POINT('Ctrl Pts',(51.966926104032,14.7062101297548,15.1738016264359));
#52801=CARTESIAN_POINT('Ctrl Pts',(51.9416776248439,14.6058769852609,15.1803409754971));
#52802=CARTESIAN_POINT('Ctrl Pts',(51.9299079202419,14.502151956084,15.1868803245583));
#52803=CARTESIAN_POINT('Ctrl Pts',(51.9308136275137,14.3982246453427,15.1934196736194));
#52804=CARTESIAN_POINT('Origin',(53.1951359564886,14.3971354987959,15.5));
#52805=CARTESIAN_POINT('',(51.9321336144334,14.3964211293814,15.6934196736194));
#52806=CARTESIAN_POINT('',(51.9298800777713,14.396145855272,15.5565803263806));
#52807=CARTESIAN_POINT('',(51.9306359564886,14.3971354987959,15.5));
#52808=CARTESIAN_POINT('Ctrl Pts',(51.9298800777713,14.396145855272,15.5565803263806));
#52809=CARTESIAN_POINT('Ctrl Pts',(51.9328341793634,14.7397024926117,15.5349217833067));
#52810=CARTESIAN_POINT('Ctrl Pts',(52.0781516403077,15.0854616424501,15.5132632402327));
#52811=CARTESIAN_POINT('Ctrl Pts',(52.3278732854,15.32010983553,15.4916046971588));
#52812=CARTESIAN_POINT('Ctrl Pts',(52.6295944912569,15.6036188430973,15.4654361936999));
#52813=CARTESIAN_POINT('Ctrl Pts',(53.0837270081696,15.7249258591405,15.439267690241));
#52814=CARTESIAN_POINT('Ctrl Pts',(53.4866324184766,15.629635385456,15.413099186782));
#52815=CARTESIAN_POINT('Ctrl Pts',(53.8895378287836,15.5343449117715,15.3869306833231));
#52816=CARTESIAN_POINT('Ctrl Pts',(54.2412161324849,15.2224569483592,15.3607621798642));
#52817=CARTESIAN_POINT('Ctrl Pts',(54.3839705956172,14.8338257457023,15.3345936764052));
#52818=CARTESIAN_POINT('Ctrl Pts',(54.5267250587495,14.4451945430454,15.3084251729463));
#52819=CARTESIAN_POINT('Ctrl Pts',(54.460555681313,13.9798201011439,15.2822566694874));
#52820=CARTESIAN_POINT('Ctrl Pts',(54.2151336032284,13.6463818912608,15.2560881660285));
#52821=CARTESIAN_POINT('Ctrl Pts',(53.9697115251439,13.3129436813777,15.2299196625695));
#52822=CARTESIAN_POINT('Ctrl Pts',(53.5450367464114,13.111441703513,15.2037511591106));
#52823=CARTESIAN_POINT('Ctrl Pts',(53.1315384766945,13.1322317596502,15.1775826556517));
#52824=CARTESIAN_POINT('Ctrl Pts',(52.7180402069775,13.1530218157874,15.1514141521928));
#52825=CARTESIAN_POINT('Ctrl Pts',(52.3157184462761,13.3961039059265,15.1252456487338));
#52826=CARTESIAN_POINT('Ctrl Pts',(52.1049790728871,13.7524772930548,15.0990771452749));
#52827=CARTESIAN_POINT('Ctrl Pts',(51.99090105541,13.9453903155784,15.0849115389768));
#52828=CARTESIAN_POINT('Ctrl Pts',(51.9329624864653,14.1715011232728,15.0707459326787));
#52829=CARTESIAN_POINT('Ctrl Pts',(51.932525975067,14.3974029423036,15.0565803263806));
#52830=CARTESIAN_POINT('Ctrl Pts',(51.9308136275137,14.3982246453427,15.1934196736194));
#52831=CARTESIAN_POINT('Ctrl Pts',(51.9335322876909,14.0862661905168,15.2130488280172));
#52832=CARTESIAN_POINT('Ctrl Pts',(52.0504588679335,13.7724851395516,15.232677982415));
#52833=CARTESIAN_POINT('Ctrl Pts',(52.2598657119041,13.5431471347949,15.2523071368127));
#52834=CARTESIAN_POINT('Ctrl Pts',(52.5390353393737,13.2374063856457,15.2784756402716));
#52835=CARTESIAN_POINT('Ctrl Pts',(52.9825678121147,13.0817441373434,15.3046441437306));
#52836=CARTESIAN_POINT('Ctrl Pts',(53.3915779035484,13.1459611997424,15.3308126471895));
#52837=CARTESIAN_POINT('Ctrl Pts',(53.8005879949821,13.2101782621413,15.3569811506484));
#52838=CARTESIAN_POINT('Ctrl Pts',(54.1750757051085,13.4942746352416,15.3831496541074));
#52839=CARTESIAN_POINT('Ctrl Pts',(54.3471162900744,13.8708581246834,15.4093181575663));
#52840=CARTESIAN_POINT('Ctrl Pts',(54.5191568750402,14.2474416141252,15.4354866610252));
#52841=CARTESIAN_POINT('Ctrl Pts',(54.4887503348454,14.7165122199085,15.4616551644841));
#52842=CARTESIAN_POINT('Ctrl Pts',(54.2695313251181,15.0677331084555,15.4878236679431));
#52843=CARTESIAN_POINT('Ctrl Pts',(54.0503123153908,15.4189539970025,15.513992171402));
#52844=CARTESIAN_POINT('Ctrl Pts',(53.642280836131,15.6523251683133,15.5401606748609));
#52845=CARTESIAN_POINT('Ctrl Pts',(53.2284030520588,15.6632002142321,15.5663291783198));
#52846=CARTESIAN_POINT('Ctrl Pts',(52.8145252679866,15.6740752601509,15.5924976817788));
#52847=CARTESIAN_POINT('Ctrl Pts',(52.3948011791021,15.4624541806777,15.6186661852377));
#52848=CARTESIAN_POINT('Ctrl Pts',(52.1574400564301,15.1232303837968,15.6448346886966));
#52849=CARTESIAN_POINT('Ctrl Pts',(52.010543532722,14.9132937439633,15.6610296836709));
#52850=CARTESIAN_POINT('Ctrl Pts',(51.9334928433345,14.6544846908102,15.6772246786452));
#52851=CARTESIAN_POINT('Ctrl Pts',(51.9321336144334,14.3964211293814,15.6934196736194));
#52852=CARTESIAN_POINT('Origin',(53.1951359564886,14.3971354987959,15.5));
#52853=CARTESIAN_POINT('',(51.9286427349006,14.3970459914357,16.1934196736194));
#52854=CARTESIAN_POINT('',(51.9301690580704,14.3981838623804,16.0565803263806));
#52855=CARTESIAN_POINT('',(51.9306359564886,14.3971354987959,15.5));
#52856=CARTESIAN_POINT('Ctrl Pts',(51.9301690580704,14.3981838623804,16.0565803263806));
#52857=CARTESIAN_POINT('Ctrl Pts',(51.9294463895002,14.4798551199685,16.0514346408525));
#52858=CARTESIAN_POINT('Ctrl Pts',(51.9366958070815,14.5613987134005,16.0462889553244));
#52859=CARTESIAN_POINT('Ctrl Pts',(51.9523897974866,14.6412833003865,16.0411432697963));
#52860=CARTESIAN_POINT('Ctrl Pts',(52.0322019507863,15.0475382258844,16.0149747663373));
#52861=CARTESIAN_POINT('Ctrl Pts',(52.3304122644718,15.4108870194284,15.9888062628784));
#52862=CARTESIAN_POINT('Ctrl Pts',(52.7132996891177,15.5683997628469,15.9626377594195));
#52863=CARTESIAN_POINT('Ctrl Pts',(53.0961871137635,15.7259125062655,15.9364692559606));
#52864=CARTESIAN_POINT('Ctrl Pts',(53.5637516493698,15.6775891995586,15.9103007525016));
#52865=CARTESIAN_POINT('Ctrl Pts',(53.9063318003261,15.4450985880149,15.8841322490427));
#52866=CARTESIAN_POINT('Ctrl Pts',(54.2489119512824,15.2126079764712,15.8579637455838));
#52867=CARTESIAN_POINT('Ctrl Pts',(54.4665077175887,14.7959500600907,15.8317952421249));
#52868=CARTESIAN_POINT('Ctrl Pts',(54.4615465710813,14.3819592010216,15.8056267386659));
#52869=CARTESIAN_POINT('Ctrl Pts',(54.4565854245739,13.9679683419524,15.779458235207));
#52870=CARTESIAN_POINT('Ctrl Pts',(54.2290673652527,13.5566445401947,15.7532897317481));
#52871=CARTESIAN_POINT('Ctrl Pts',(53.8810141954492,13.3324302783772,15.7271212282891));
#52872=CARTESIAN_POINT('Ctrl Pts',(53.5329610256457,13.1082160165598,15.7009527248302));
#52873=CARTESIAN_POINT('Ctrl Pts',(53.0643727453599,13.0711112946827,15.6747842213713));
#52874=CARTESIAN_POINT('Ctrl Pts',(52.6853699093616,13.2377543099066,15.6486157179124));
#52875=CARTESIAN_POINT('Ctrl Pts',(52.3063670733632,13.4043973251305,15.6224472144534));
#52876=CARTESIAN_POINT('Ctrl Pts',(52.0169496816522,13.7747880774553,15.5962787109945));
#52877=CARTESIAN_POINT('Ctrl Pts',(51.9468959331972,14.1828389531634,15.5701102075356));
#52878=CARTESIAN_POINT('Ctrl Pts',(51.9348226546909,14.2531636963187,15.5656002471506));
#52879=CARTESIAN_POINT('Ctrl Pts',(51.9292649449293,14.324607025577,15.5610902867656));
#52880=CARTESIAN_POINT('Ctrl Pts',(51.9298800777713,14.396145855272,15.5565803263806));
#52881=CARTESIAN_POINT('Ctrl Pts',(51.9321336144334,14.3964211293814,15.6934196736194));
#52882=CARTESIAN_POINT('Ctrl Pts',(51.9312965483521,14.2374955401126,15.7033931821041));
#52883=CARTESIAN_POINT('Ctrl Pts',(51.9591660436084,14.0788526842429,15.7133666905887));
#52884=CARTESIAN_POINT('Ctrl Pts',(52.0171074139709,13.932081398796,15.7233401990734));
#52885=CARTESIAN_POINT('Ctrl Pts',(52.1691340506433,13.5469827249647,15.7495087025323));
#52886=CARTESIAN_POINT('Ctrl Pts',(52.5281854804477,13.2436118915905,15.7756772059913));
#52887=CARTESIAN_POINT('Ctrl Pts',(52.9332587743737,13.1580039865908,15.8018457094502));
#52888=CARTESIAN_POINT('Ctrl Pts',(53.3383320682997,13.072396081591,15.8280142129091));
#52889=CARTESIAN_POINT('Ctrl Pts',(53.7894272263473,13.2045511049655,15.854182716368));
#52890=CARTESIAN_POINT('Ctrl Pts',(54.0842678175164,13.4952091732588,15.880351219827));
#52891=CARTESIAN_POINT('Ctrl Pts',(54.3791084086854,13.7858672415521,15.9065197232859));
#52892=CARTESIAN_POINT('Ctrl Pts',(54.517694432976,14.2350283547642,15.9326882267448));
#52893=CARTESIAN_POINT('Ctrl Pts',(54.4378822697682,14.6412833306956,15.9588567302037));
#52894=CARTESIAN_POINT('Ctrl Pts',(54.3580701065605,15.047538306627,15.9850252336627));
#52895=CARTESIAN_POINT('Ctrl Pts',(54.0598597558545,15.4108871452777,16.0111937371216));
#52896=CARTESIAN_POINT('Ctrl Pts',(53.676972283676,15.5683999082504,16.0373622405805));
#52897=CARTESIAN_POINT('Ctrl Pts',(53.2940848114976,15.7259126712231,16.0635307440394));
#52898=CARTESIAN_POINT('Ctrl Pts',(52.8265202178467,15.6775893585178,16.0896992474984));
#52899=CARTESIAN_POINT('Ctrl Pts',(52.4839400243616,15.4450987181119,16.1158677509573));
#52900=CARTESIAN_POINT('Ctrl Pts',(52.1455210707975,15.2154320860769,16.1417183918447));
#52901=CARTESIAN_POINT('Ctrl Pts',(51.9290686466627,14.8060450268197,16.167569032732));
#52902=CARTESIAN_POINT('Ctrl Pts',(51.9286427349006,14.3970459914357,16.1934196736194));
#52903=CARTESIAN_POINT('Origin',(53.1951359564886,14.3971354987959,15.5));
#52904=CARTESIAN_POINT('',(51.9319412138059,14.397962888141,16.6934196736194));
#52905=CARTESIAN_POINT('',(51.9324421154971,14.3967173588992,16.5565803263806));
#52906=CARTESIAN_POINT('',(51.9306359564886,14.3971354987959,15.5));
#52907=CARTESIAN_POINT('Ctrl Pts',(51.9324421154971,14.3967173588992,16.5565803263806));
#52908=CARTESIAN_POINT('Ctrl Pts',(51.9331582847598,14.6327178878915,16.5417789949394));
#52909=CARTESIAN_POINT('Ctrl Pts',(51.9967468970028,14.8690767992861,16.5269776634981));
#52910=CARTESIAN_POINT('Ctrl Pts',(52.1207407212383,15.0677330252045,16.5121763320569));
#52911=CARTESIAN_POINT('Ctrl Pts',(52.339959703752,15.4189538701487,16.486007828598));
#52912=CARTESIAN_POINT('Ctrl Pts',(52.747991132356,15.652325012491,16.4598393251391));
#52913=CARTESIAN_POINT('Ctrl Pts',(53.1618688650479,15.6632000570604,16.4336708216802));
#52914=CARTESIAN_POINT('Ctrl Pts',(53.5757465977399,15.6740751016298,16.4075023182212));
#52915=CARTESIAN_POINT('Ctrl Pts',(53.9954706345197,15.4624540484263,16.3813338147623));
#52916=CARTESIAN_POINT('Ctrl Pts',(54.2328317277253,15.1232302936571,16.3551653113034));
#52917=CARTESIAN_POINT('Ctrl Pts',(54.470192820931,14.784006538888,16.3289968078444));
#52918=CARTESIAN_POINT('Ctrl Pts',(54.5251909705625,14.3171800825532,16.3028283043855));
#52919=CARTESIAN_POINT('Ctrl Pts',(54.3731643527629,13.9320814565291,16.2766598009266));
#52920=CARTESIAN_POINT('Ctrl Pts',(54.2211377349633,13.546982830505,16.2504912974677));
#52921=CARTESIAN_POINT('Ctrl Pts',(53.8620863497326,13.2436120347917,16.2243227940088));
#52922=CARTESIAN_POINT('Ctrl Pts',(53.4570131060934,13.1580041404195,16.1981542905498));
#52923=CARTESIAN_POINT('Ctrl Pts',(53.0519398624543,13.0723962460472,16.1719857870909));
#52924=CARTESIAN_POINT('Ctrl Pts',(52.6008447604067,13.204551253016,16.145817283632));
#52925=CARTESIAN_POINT('Ctrl Pts',(52.3060042058399,13.4952092852263,16.119648780173));
#52926=CARTESIAN_POINT('Ctrl Pts',(52.0691400952495,13.7287133104327,16.0986259622422));
#52927=CARTESIAN_POINT('Ctrl Pts',(51.9331215373257,14.0645140395593,16.0776031443114));
#52928=CARTESIAN_POINT('Ctrl Pts',(51.9301690580704,14.3981838623804,16.0565803263806));
#52929=CARTESIAN_POINT('Ctrl Pts',(51.9286427349006,14.3970459914357,16.1934196736194));
#52930=CARTESIAN_POINT('Ctrl Pts',(51.9286374978387,14.3920168903888,16.193737536191));
#52931=CARTESIAN_POINT('Ctrl Pts',(51.9286649228095,14.386987848009,16.1940553987625));
#52932=CARTESIAN_POINT('Ctrl Pts',(51.9287251846806,14.3819591991371,16.1943732613341));
#52933=CARTESIAN_POINT('Ctrl Pts',(51.9336863318039,13.9679682886746,16.220541764793));
#52934=CARTESIAN_POINT('Ctrl Pts',(52.1612044193698,13.5566444358558,16.2467102682519));
#52935=CARTESIAN_POINT('Ctrl Pts',(52.5092576323814,13.332430146203,16.2728787717108));
#52936=CARTESIAN_POINT('Ctrl Pts',(52.857310845393,13.1082158565502,16.2990472751698));
#52937=CARTESIAN_POINT('Ctrl Pts',(53.3258991838504,13.0711111300635,16.3252157786287));
#52938=CARTESIAN_POINT('Ctrl Pts',(53.7049020668992,13.2377541659764,16.3513842820876));
#52939=CARTESIAN_POINT('Ctrl Pts',(54.083904949948,13.4043972018893,16.3775527855466));
#52940=CARTESIAN_POINT('Ctrl Pts',(54.3733223775883,13.7747880002018,16.4037212890055));
#52941=CARTESIAN_POINT('Ctrl Pts',(54.4433761347398,14.1828389265634,16.4298897924644));
#52942=CARTESIAN_POINT('Ctrl Pts',(54.5134298918913,14.5908898529249,16.4560582959233));
#52943=CARTESIAN_POINT('Ctrl Pts',(54.3641199785539,15.0366009073353,16.4822267993823));
#52944=CARTESIAN_POINT('Ctrl Pts',(54.0623987352411,15.3201099501039,16.5083953028412));
#52945=CARTESIAN_POINT('Ctrl Pts',(53.7606774919283,15.6036189928724,16.5345638063001));
#52946=CARTESIAN_POINT('Ctrl Pts',(53.30654491864,15.724926023999,16.560732309759));
#52947=CARTESIAN_POINT('Ctrl Pts',(52.9036394583144,15.6296355384739,16.586900813218));
#52948=CARTESIAN_POINT('Ctrl Pts',(52.5007339979887,15.5343450529489,16.6130693166769));
#52949=CARTESIAN_POINT('Ctrl Pts',(52.1490556506257,15.2224570507722,16.6392378201358));
#52950=CARTESIAN_POINT('Ctrl Pts',(52.0063011697735,14.8338257998906,16.6654063235947));
#52951=CARTESIAN_POINT('Ctrl Pts',(51.9553616723993,14.6951493782073,16.6747441069363));
#52952=CARTESIAN_POINT('Ctrl Pts',(51.9310243942125,14.5467012595068,16.6840818902779));
#52953=CARTESIAN_POINT('Ctrl Pts',(51.9319412138059,14.397962888141,16.6934196736194));
#52954=CARTESIAN_POINT('Origin',(53.1951359564886,14.3971354987959,15.5));
#52955=CARTESIAN_POINT('',(51.9310991161132,14.3960665614756,17.1934196736194));
#52956=CARTESIAN_POINT('',(51.9288577112775,14.3966710926088,17.0565803263806));
#52957=CARTESIAN_POINT('',(51.9306359564886,14.3971354987959,15.5));
#52958=CARTESIAN_POINT('Ctrl Pts',(51.9288577112775,14.3966710926088,17.0565803263806));
#52959=CARTESIAN_POINT('Ctrl Pts',(51.9307115507732,14.783795951987,17.0321233490263));
#52960=CARTESIAN_POINT('Ctrl Pts',(52.121565621024,15.1725044294775,17.0076663716719));
#52961=CARTESIAN_POINT('Ctrl Pts',(52.4298869834431,15.406303531382,16.9832093943176));
#52962=CARTESIAN_POINT('Ctrl Pts',(52.7597850130333,15.6564641509158,16.9570408908587));
#52963=CARTESIAN_POINT('Ctrl Pts',(53.2241665936333,15.7292752927444,16.9308723873998));
#52964=CARTESIAN_POINT('Ctrl Pts',(53.6147975571804,15.5920875143541,16.9047038839408));
#52965=CARTESIAN_POINT('Ctrl Pts',(54.0054285207274,15.4548997359638,16.8785353804819));
#52966=CARTESIAN_POINT('Ctrl Pts',(54.3223088672216,15.1077130373545,16.852366877023));
#52967=CARTESIAN_POINT('Ctrl Pts',(54.4233456564843,14.706210091365,16.8261983735641));
#52968=CARTESIAN_POINT('Ctrl Pts',(54.524382445747,14.3047071453755,16.8000298701051));
#52969=CARTESIAN_POINT('Ctrl Pts',(54.4095756777782,13.8488879520058,16.7738613666462));
#52970=CARTESIAN_POINT('Ctrl Pts',(54.13040608496,13.5431472408216,16.7476928631873));
#52971=CARTESIAN_POINT('Ctrl Pts',(53.8512364921418,13.2374065296375,16.7215243597283));
#52972=CARTESIAN_POINT('Ctrl Pts',(53.4077040744743,13.0817443006388,16.6953558562694));
#52973=CARTESIAN_POINT('Ctrl Pts',(52.998694033819,13.1459613550608,16.6691873528105));
#52974=CARTESIAN_POINT('Ctrl Pts',(52.5896839931637,13.2101784094827,16.6430188493516));
#52975=CARTESIAN_POINT('Ctrl Pts',(52.2151963295206,13.4942747473253,16.6168503458927));
#52976=CARTESIAN_POINT('Ctrl Pts',(52.0431557659108,13.8708581900196,16.5906818424337));
#52977=CARTESIAN_POINT('Ctrl Pts',(51.9684241449892,14.0344399087392,16.579314670416));
#52978=CARTESIAN_POINT('Ctrl Pts',(51.9318921096253,14.2154729472068,16.5679474983983));
#52979=CARTESIAN_POINT('Ctrl Pts',(51.9324421154971,14.3967173588992,16.5565803263806));
#52980=CARTESIAN_POINT('Ctrl Pts',(51.9319412138059,14.397962888141,16.6934196736194));
#52981=CARTESIAN_POINT('Ctrl Pts',(51.9335937188396,14.1298720781913,16.7102503937368));
#52982=CARTESIAN_POINT('Ctrl Pts',(52.0172907607076,13.8608383066004,16.7270811138542));
#52983=CARTESIAN_POINT('Ctrl Pts',(52.1751381831274,13.6463817981057,16.7439118339715));
#52984=CARTESIAN_POINT('Ctrl Pts',(52.4205602916747,13.3129435467891,16.7700803374305));
#52985=CARTESIAN_POINT('Ctrl Pts',(52.8452351231106,13.1114415437426,16.7962488408894));
#52986=CARTESIAN_POINT('Ctrl Pts',(53.25873344417,13.1322316025356,16.8224173443483));
#52987=CARTESIAN_POINT('Ctrl Pts',(53.6722317652293,13.1530216613285,16.8485858478072));
#52988=CARTESIAN_POINT('Ctrl Pts',(54.0745535759121,13.3961037819609,16.8747543512662));
#52989=CARTESIAN_POINT('Ctrl Pts',(54.285292975442,13.7524772131894,16.9009228547251));
#52990=CARTESIAN_POINT('Ctrl Pts',(54.496032374972,14.108850644418,16.927091358184));
#52991=CARTESIAN_POINT('Ctrl Pts',(54.515189363349,14.5785153862427,16.9532598616429));
#52992=CARTESIAN_POINT('Ctrl Pts',(54.3341737566947,14.9508678603537,16.9794283651019));
#52993=CARTESIAN_POINT('Ctrl Pts',(54.1531581500404,15.3232203344646,17.0055968685608));
#52994=CARTESIAN_POINT('Ctrl Pts',(53.7719699483548,15.5982605408617,17.0317653720197));
#52995=CARTESIAN_POINT('Ctrl Pts',(53.3615383968383,15.652657838236,17.0579338754786));
#52996=CARTESIAN_POINT('Ctrl Pts',(52.9511068453218,15.7070551356103,17.0841023789376));
#52997=CARTESIAN_POINT('Ctrl Pts',(52.5114319439746,15.5408095239618,17.1102708823965));
#52998=CARTESIAN_POINT('Ctrl Pts',(52.2396692974107,15.2284661862235,17.1364393858554));
#52999=CARTESIAN_POINT('Ctrl Pts',(52.0424205472225,15.0017634594966,17.1554328151101));
#53000=CARTESIAN_POINT('Ctrl Pts',(51.9336286302043,14.6980958787159,17.1744262443648));
#53001=CARTESIAN_POINT('Ctrl Pts',(51.9310991161132,14.3960665614756,17.1934196736194));
#53002=CARTESIAN_POINT('Origin',(53.1951359564886,14.3971354987959,15.5));
#53003=CARTESIAN_POINT('',(51.929081218047,14.3977505022101,17.6934196736194));
#53004=CARTESIAN_POINT('',(51.9314271328212,14.3981451355535,17.5565803263806));
#53005=CARTESIAN_POINT('',(51.9306359564886,14.3971354987959,15.5));
#53006=CARTESIAN_POINT('',(54.1532521092111,15.2223467977324,18.));
#53007=CARTESIAN_POINT('Ctrl Pts',(51.929081218047,14.3977505022101,17.6934196736194));
#53008=CARTESIAN_POINT('Ctrl Pts',(51.9314396049108,14.022694300038,17.7171076053695));
#53009=CARTESIAN_POINT('Ctrl Pts',(52.1089957350005,13.6457772873263,17.7407955371196));
#53010=CARTESIAN_POINT('Ctrl Pts',(52.4009425562916,13.4106743694811,17.7644834688697));
#53011=CARTESIAN_POINT('Ctrl Pts',(52.7234616974046,13.1509517569817,17.7906519723286));
#53012=CARTESIAN_POINT('Ctrl Pts',(53.1855836521257,13.0642995791891,17.8168204757875));
#53013=CARTESIAN_POINT('Ctrl Pts',(53.5800062339574,13.190324595469,17.8429889792464));
#53014=CARTESIAN_POINT('Ctrl Pts',(53.974428815789,13.3163496117488,17.8691574827054));
#53015=CARTESIAN_POINT('Ctrl Pts',(54.3011520247311,13.6550518221011,17.8953259861643));
#53016=CARTESIAN_POINT('Ctrl Pts',(54.4136991111698,14.0527836440546,17.9214944896232));
#53017=CARTESIAN_POINT('Ctrl Pts',(54.5262461976084,14.4505154660081,17.9476629930821));
#53018=CARTESIAN_POINT('Ctrl Pts',(54.4246171615437,14.9072768995628,17.9738314965411));
#53019=CARTESIAN_POINT('Ctrl Pts',(54.1532521092111,15.2223467977324,18.));
#53020=CARTESIAN_POINT('',(52.2352328551172,15.2234705191483,18.));
#53021=CARTESIAN_POINT('Origin',(53.1951359564886,14.3971354987959,18.));
#53022=CARTESIAN_POINT('Ctrl Pts',(52.2352228301846,15.2234768233202,18.));
#53023=CARTESIAN_POINT('Ctrl Pts',(52.4934806168631,15.521313638849,17.975091839613));
#53024=CARTESIAN_POINT('Ctrl Pts',(52.9025313044196,15.6908537017463,17.950183679226));
#53025=CARTESIAN_POINT('Ctrl Pts',(53.295440078112,15.6595882927142,17.925275518839));
#53026=CARTESIAN_POINT('Ctrl Pts',(53.7082298804764,15.6267408663411,17.8991070153801));
#53027=CARTESIAN_POINT('Ctrl Pts',(54.1032028915872,15.3722524867281,17.8729385119211));
#53028=CARTESIAN_POINT('Ctrl Pts',(54.3034894678616,15.0099588806278,17.8467700084622));
#53029=CARTESIAN_POINT('Ctrl Pts',(54.5037760441361,14.6476652745274,17.8206015050033));
#53030=CARTESIAN_POINT('Ctrl Pts',(54.5093761855741,14.1775664419396,17.7944330015443));
#53031=CARTESIAN_POINT('Ctrl Pts',(54.3176594419829,13.8105984641279,17.7682644980854));
#53032=CARTESIAN_POINT('Ctrl Pts',(54.1259426983917,13.4436304863162,17.7420959946265));
#53033=CARTESIAN_POINT('Ctrl Pts',(53.7369090697714,13.1797933632805,17.7159274911676));
#53034=CARTESIAN_POINT('Ctrl Pts',(53.3250649526276,13.1373263636934,17.6897589877086));
#53035=CARTESIAN_POINT('Ctrl Pts',(52.9132208354839,13.0948593641063,17.6635904842497));
#53036=CARTESIAN_POINT('Ctrl Pts',(52.4785662298169,13.2737624879677,17.6374219807908));
#53037=CARTESIAN_POINT('Ctrl Pts',(52.2159761485057,13.5938473532064,17.6112534773319));
#53038=CARTESIAN_POINT('Ctrl Pts',(52.0331020154043,13.8167622552358,17.5930290936814));
#53039=CARTESIAN_POINT('Ctrl Pts',(51.9336803654542,14.1081512772947,17.574804710031));
#53040=CARTESIAN_POINT('Ctrl Pts',(51.9314271328212,14.3981451355535,17.5565803263806));
#53041=CARTESIAN_POINT('Origin',(53.1951359564886,14.3971354987959,19.1042117235887));
#53042=CARTESIAN_POINT('',(51.6501838308085,14.3978968813702,14.3957882764113));
#53043=CARTESIAN_POINT('',(51.654536051996,14.3970771807141,14.3542117235887));
#53044=CARTESIAN_POINT('',(51.6521359564886,14.397135498796,19.1042117235887));
#53045=CARTESIAN_POINT('',(53.5936497983458,12.9064860705774,14.));
#53046=CARTESIAN_POINT('Ctrl Pts',(51.654536051996,14.3970771807141,14.3542117235887));
#53047=CARTESIAN_POINT('Ctrl Pts',(51.6547008227736,14.6578150564091,14.3408151628949));
#53048=CARTESIAN_POINT('Ctrl Pts',(51.8403375140876,15.4280419867602,14.3012500987421));
#53049=CARTESIAN_POINT('Ctrl Pts',(53.0509994556171,16.2080945317645,14.2355165311303));
#53050=CARTESIAN_POINT('Ctrl Pts',(54.6273366519326,15.5169696210012,14.1570110207535));
#53051=CARTESIAN_POINT('Ctrl Pts',(54.9168336227569,13.8187144824051,14.0785055103768));
#53052=CARTESIAN_POINT('Ctrl Pts',(54.0838395965459,13.0375346028627,14.0261685034589));
#53053=CARTESIAN_POINT('Ctrl Pts',(53.5936497983458,12.9064860705774,14.));
#53054=CARTESIAN_POINT('',(52.7955932879501,12.9041246312965,14.));
#53055=CARTESIAN_POINT('Origin',(53.1951359564886,14.3971354987959,14.));
#53056=CARTESIAN_POINT('Ctrl Pts',(51.6501838308085,14.3978968813702,14.3957882764113));
#53057=CARTESIAN_POINT('Ctrl Pts',(51.6499084261818,14.443250645686,14.3934410251636));
#53058=CARTESIAN_POINT('Ctrl Pts',(51.6721169602754,14.9939590280816,14.3649252704569));
#53059=CARTESIAN_POINT('Ctrl Pts',(52.3307362917628,15.9953382094595,14.3102410122914));
#53060=CARTESIAN_POINT('Ctrl Pts',(54.0514987748276,15.9998443309588,14.2317355019146));
#53061=CARTESIAN_POINT('Ctrl Pts',(55.0042044918326,14.5665632650764,14.1532299915378));
#53062=CARTESIAN_POINT('Ctrl Pts',(54.3453458049291,13.0076586982508,14.0759848242329));
#53063=CARTESIAN_POINT('Ctrl Pts',(53.2607152655111,12.7814238100544,14.024908160387));
#53064=CARTESIAN_POINT('Ctrl Pts',(52.7955875161457,12.9041113834231,14.));
#53065=CARTESIAN_POINT('Origin',(53.1951359564886,14.3971354987959,19.1042117235887));
#53066=CARTESIAN_POINT('',(51.654442242504,14.3974618454408,14.8957882764113));
#53067=CARTESIAN_POINT('',(51.6505063374695,14.3961865684695,14.8542117235887));
#53068=CARTESIAN_POINT('',(51.6521359564886,14.397135498796,19.1042117235887));
#53069=CARTESIAN_POINT('Ctrl Pts',(51.6505063374695,14.3961865684695,14.8542117235887));
#53070=CARTESIAN_POINT('Ctrl Pts',(51.6537531731077,14.8418532139508,14.8311595169817));
#53071=CARTESIAN_POINT('Ctrl Pts',(52.0889693478695,15.798972462477,14.7819388069158));
#53072=CARTESIAN_POINT('Ctrl Pts',(53.7056220123855,16.1409817745025,14.706549593391));
#53073=CARTESIAN_POINT('Ctrl Pts',(54.9313021937626,14.9332257573755,14.6280440830142));
#53074=CARTESIAN_POINT('Ctrl Pts',(54.5999120631369,13.2446506074896,14.5495385726375));
#53075=CARTESIAN_POINT('Ctrl Pts',(53.0087562916135,12.5897333550461,14.4710330622607));
#53076=CARTESIAN_POINT('Ctrl Pts',(51.8276307116252,13.3907563492144,14.4059241125778));
#53077=CARTESIAN_POINT('Ctrl Pts',(51.6543789636963,14.148496272438,14.3669836663538));
#53078=CARTESIAN_POINT('Ctrl Pts',(51.654536051996,14.3970771807141,14.3542117235887));
#53079=CARTESIAN_POINT('Ctrl Pts',(51.654442242504,14.3974618454408,14.8957882764113));
#53080=CARTESIAN_POINT('Ctrl Pts',(51.6539909131311,14.6310322097678,14.8837853792505));
#53081=CARTESIAN_POINT('Ctrl Pts',(51.8127636494607,15.3732462698704,14.8456139786307));
#53082=CARTESIAN_POINT('Ctrl Pts',(52.9564001587445,16.1984187666638,14.781274074552));
#53083=CARTESIAN_POINT('Ctrl Pts',(54.5659334636339,15.5898376428623,14.7027685641752));
#53084=CARTESIAN_POINT('Ctrl Pts',(54.9461022318155,13.911606374279,14.6242630537985));
#53085=CARTESIAN_POINT('Ctrl Pts',(53.7559643179138,12.6688223002735,14.5457575434217));
#53086=CARTESIAN_POINT('Ctrl Pts',(52.1134816424644,12.9668195987494,14.4695992842926));
#53087=CARTESIAN_POINT('Ctrl Pts',(51.6529787949523,13.9376208629641,14.4196095286225));
#53088=CARTESIAN_POINT('Ctrl Pts',(51.6501838308085,14.3978968813702,14.3957882764113));
#53089=CARTESIAN_POINT('Origin',(53.1951359564886,14.3971354987959,19.1042117235887));
#53090=CARTESIAN_POINT('',(51.6512135991451,14.3959278910795,15.3957882764113));
#53091=CARTESIAN_POINT('',(51.6523527586964,14.3984645245941,15.3542117235887));
#53092=CARTESIAN_POINT('',(51.6521359564886,14.397135498796,19.1042117235887));
#53093=CARTESIAN_POINT('Ctrl Pts',(51.6523527586964,14.3984645245941,15.3542117235887));
#53094=CARTESIAN_POINT('Ctrl Pts',(51.651247573785,14.5252813221218,15.3476723745276));
#53095=CARTESIAN_POINT('Ctrl Pts',(51.7230815929517,15.1583461258636,15.3149645220075));
#53096=CARTESIAN_POINT('Ctrl Pts',(52.5930520129352,16.1115202855033,15.2560881660285));
#53097=CARTESIAN_POINT('Ctrl Pts',(54.2930303473182,15.8449779235543,15.1775826556517));
#53098=CARTESIAN_POINT('Ctrl Pts',(55.0083911483926,14.2799763521069,15.0990771452749));
#53099=CARTESIAN_POINT('Ctrl Pts',(54.0975810662168,12.8200452881305,15.0205716348981));
#53100=CARTESIAN_POINT('Ctrl Pts',(52.3774378038973,12.7744874306393,14.9420661245214));
#53101=CARTESIAN_POINT('Ctrl Pts',(51.6803897960552,13.7702239867045,14.8866128207515));
#53102=CARTESIAN_POINT('Ctrl Pts',(51.6500674162048,14.3359394264926,14.8573280204407));
#53103=CARTESIAN_POINT('Ctrl Pts',(51.6505063374695,14.3961865684695,14.8542117235887));
#53104=CARTESIAN_POINT('Ctrl Pts',(51.6512135991451,14.3959278910795,15.3957882764113));
#53105=CARTESIAN_POINT('Ctrl Pts',(51.6548183273038,14.8151512136696,15.3741297333373));
#53106=CARTESIAN_POINT('Ctrl Pts',(52.0463881522717,15.7468276199562,15.3263026868045));
#53107=CARTESIAN_POINT('Ctrl Pts',(53.6133427309768,16.1653895531783,15.2523071368127));
#53108=CARTESIAN_POINT('Ctrl Pts',(54.9007439708605,15.0236502232965,15.1738016264359));
#53109=CARTESIAN_POINT('Ctrl Pts',(54.6585153839456,13.3200374976642,15.0952961160592));
#53110=CARTESIAN_POINT('Ctrl Pts',(53.1038933588347,12.5823920603089,15.0167906056824));
#53111=CARTESIAN_POINT('Ctrl Pts',(51.8562787823209,13.3361985618968,14.9502879924664));
#53112=CARTESIAN_POINT('Ctrl Pts',(51.6549748934233,14.1218062449943,14.9099538827094));
#53113=CARTESIAN_POINT('Ctrl Pts',(51.654442242504,14.3974618454408,14.8957882764113));
#53114=CARTESIAN_POINT('Origin',(53.1951359564886,14.3971354987959,19.1042117235887));
#53115=CARTESIAN_POINT('',(51.6515662259554,14.3984147593818,15.8957882764113));
#53116=CARTESIAN_POINT('',(51.6539634663413,14.3962637929782,15.8542117235887));
#53117=CARTESIAN_POINT('',(51.6521359564886,14.397135498796,19.1042117235887));
#53118=CARTESIAN_POINT('Ctrl Pts',(51.6539634663413,14.3962637929782,15.8542117235887));
#53119=CARTESIAN_POINT('Ctrl Pts',(51.6556220588242,14.7111646038003,15.8380167286145));
#53120=CARTESIAN_POINT('Ctrl Pts',(51.9015651465378,15.5372739892809,15.7956532301813));
#53121=CARTESIAN_POINT('Ctrl Pts',(53.2428638938474,16.2135446545079,15.7271212282891));
#53122=CARTESIAN_POINT('Ctrl Pts',(54.7365592022647,15.3592345303502,15.6486157179124));
#53123=CARTESIAN_POINT('Ctrl Pts',(54.8478695024322,13.6420911264981,15.5701102075356));
#53124=CARTESIAN_POINT('Ctrl Pts',(53.4769690594307,12.6020894569994,15.4916046971588));
#53125=CARTESIAN_POINT('Ctrl Pts',(51.9885611628802,13.1244613999964,15.4196385358432));
#53126=CARTESIAN_POINT('Ctrl Pts',(51.6556701906089,14.0177987311608,15.3738408779865));
#53127=CARTESIAN_POINT('Ctrl Pts',(51.6523527586964,14.3984645245941,15.3542117235887));
#53128=CARTESIAN_POINT('Ctrl Pts',(51.6515662259554,14.3984147593818,15.8957882764113));
#53129=CARTESIAN_POINT('Ctrl Pts',(51.6506843931331,14.4980737158535,15.8906425908832));
#53130=CARTESIAN_POINT('Ctrl Pts',(51.7045173377561,15.1036026015034,15.8593284018961));
#53131=CARTESIAN_POINT('Ctrl Pts',(52.503850750664,16.077535486755,15.8018457094502));
#53132=CARTESIAN_POINT('Ctrl Pts',(54.2154808300007,15.9006366439348,15.7233401990734));
#53133=CARTESIAN_POINT('Ctrl Pts',(55.0120413695279,14.3753622311824,15.6448346886966));
#53134=CARTESIAN_POINT('Ctrl Pts',(54.1791579400318,12.8696146010229,15.5663291783198));
#53135=CARTESIAN_POINT('Ctrl Pts',(52.4637802022359,12.7337840295962,15.4878236679431));
#53136=CARTESIAN_POINT('Ctrl Pts',(51.6965951513912,13.7156125454117,15.4309767006402));
#53137=CARTESIAN_POINT('Ctrl Pts',(51.6504629862743,14.3086329806648,15.4002982367963));
#53138=CARTESIAN_POINT('Ctrl Pts',(51.6512135991451,14.3959278910795,15.3957882764113));
#53139=CARTESIAN_POINT('Origin',(53.1951359564886,14.3971354987959,19.1042117235887));
#53140=CARTESIAN_POINT('',(51.65433991327,14.3966252656123,16.3957882764113));
#53141=CARTESIAN_POINT('',(51.6497037375007,14.3970262778732,16.3542117235887));
#53142=CARTESIAN_POINT('',(51.6521359564886,14.397135498796,19.1042117235887));
#53143=CARTESIAN_POINT('Ctrl Pts',(51.6497037375007,14.3970262778732,16.3542117235887));
#53144=CARTESIAN_POINT('Ctrl Pts',(51.6502234542653,14.8961053696862,16.3283610827013));
#53145=CARTESIAN_POINT('Ctrl Pts',(52.1817212113122,15.9013530800272,16.2763419383551));
#53146=CARTESIAN_POINT('Ctrl Pts',(53.8864212481313,16.0775356953633,16.1981542905498));
#53147=CARTESIAN_POINT('Ctrl Pts',(54.9780904560539,14.7474117142528,16.119648780173));
#53148=CARTESIAN_POINT('Ctrl Pts',(54.4707636814861,13.1031516960174,16.0411432697963));
#53149=CARTESIAN_POINT('Ctrl Pts',(52.8194236367236,12.6193671146013,15.9626377594195));
#53150=CARTESIAN_POINT('Ctrl Pts',(51.7761788820818,13.5008286667841,15.900327244017));
#53151=CARTESIAN_POINT('Ctrl Pts',(51.6529420405103,14.2023356124785,15.8641852320734));
#53152=CARTESIAN_POINT('Ctrl Pts',(51.6539634663413,14.3962637929782,15.8542117235887));
#53153=CARTESIAN_POINT('Ctrl Pts',(51.65433991327,14.3966252656123,16.3957882764113));
#53154=CARTESIAN_POINT('Ctrl Pts',(51.6552138153438,14.684603767973,16.38098694497));
#53155=CARTESIAN_POINT('Ctrl Pts',(51.869991852728,15.4829338669789,16.3400171100699));
#53156=CARTESIAN_POINT('Ctrl Pts',(53.1474080250528,16.2135444290179,16.2728787717109));
#53157=CARTESIAN_POINT('Ctrl Pts',(54.6839066935017,15.4388557336608,16.1943732613341));
#53158=CARTESIAN_POINT('Ctrl Pts',(54.8852403705633,13.7299275672916,16.1158677509573));
#53159=CARTESIAN_POINT('Ctrl Pts',(53.5708482296119,12.6193673352972,16.0373622405805));
#53160=CARTESIAN_POINT('Ctrl Pts',(52.0277463399597,13.0714419423033,15.9640024157318));
#53161=CARTESIAN_POINT('Ctrl Pts',(51.6551689744653,13.9912557743182,15.9168110943421));
#53162=CARTESIAN_POINT('Ctrl Pts',(51.6515662259554,14.3984147593818,15.8957882764113));
#53163=CARTESIAN_POINT('Origin',(53.1951359564886,14.3971354987959,19.1042117235887));
#53164=CARTESIAN_POINT('',(51.6499660613832,14.3965688093956,16.8957882764113));
#53165=CARTESIAN_POINT('',(51.6537286904076,14.3981451166365,16.8542117235887));
#53166=CARTESIAN_POINT('',(51.6521359564886,14.397135498796,19.1042117235887));
#53167=CARTESIAN_POINT('Ctrl Pts',(51.6537286904076,14.3981451166365,16.8542117235887));
#53168=CARTESIAN_POINT('Ctrl Pts',(51.6526099457397,14.579642393835,16.8448739402472));
#53169=CARTESIAN_POINT('Ctrl Pts',(51.7655324660037,15.2684267173499,16.8093676534467));
#53170=CARTESIAN_POINT('Ctrl Pts',(52.7769291300874,16.1653897727513,16.7476928631873));
#53171=CARTESIAN_POINT('Ctrl Pts',(54.4393883485545,15.72131682132,16.6691873528105));
#53172=CARTESIAN_POINT('Ctrl Pts',(54.9859724441168,14.0896865557083,16.5906818424337));
#53173=CARTESIAN_POINT('Ctrl Pts',(53.9264918015332,12.7337838230954,16.5121763320569));
#53174=CARTESIAN_POINT('Ctrl Pts',(52.2111138507866,12.869614411397,16.4336708216802));
#53175=CARTESIAN_POINT('Ctrl Pts',(51.6524858829683,13.8795429426784,16.3810159521908));
#53176=CARTESIAN_POINT('Ctrl Pts',(51.6496973470012,14.3908895416808,16.3545295861603));
#53177=CARTESIAN_POINT('Ctrl Pts',(51.6497037375007,14.3970262778732,16.3542117235887));
#53178=CARTESIAN_POINT('Ctrl Pts',(51.6499660613832,14.3965688093956,16.8957882764113));
#53179=CARTESIAN_POINT('Ctrl Pts',(51.6522282000482,14.8689560438919,16.8713312990569));
#53180=CARTESIAN_POINT('Ctrl Pts',(52.1343035201105,15.8507887260607,16.8207058182437));
#53181=CARTESIAN_POINT('Ctrl Pts',(53.7972198251956,16.11152007286,16.7439118339715));
#53182=CARTESIAN_POINT('Ctrl Pts',(54.9572349488979,14.8405614110472,16.6654063235948));
#53183=CARTESIAN_POINT('Ctrl Pts',(54.5369577413632,13.1719279226262,16.586900813218));
#53184=CARTESIAN_POINT('Ctrl Pts',(52.9133028885494,12.602089679815,16.5083953028412));
#53185=CARTESIAN_POINT('Ctrl Pts',(51.8008704508192,13.4460106212472,16.4446911239056));
#53186=CARTESIAN_POINT('Ctrl Pts',(51.6536687712691,14.1754626501585,16.407155448429));
#53187=CARTESIAN_POINT('Ctrl Pts',(51.65433991327,14.3966252656123,16.3957882764113));
#53188=CARTESIAN_POINT('Origin',(53.1951359564886,14.3971354987959,19.1042117235887));
#53189=CARTESIAN_POINT('',(51.6531013855762,14.3983675031589,17.3957882764113));
#53190=CARTESIAN_POINT('',(51.6527011247771,14.3958311332086,17.3542117235887));
#53191=CARTESIAN_POINT('',(51.6521359564886,14.397135498796,19.1042117235887));
#53192=CARTESIAN_POINT('Ctrl Pts',(51.6527011247771,14.3958311332086,17.3542117235887));
#53193=CARTESIAN_POINT('Ctrl Pts',(51.6557877520943,14.7643809445978,17.3352182943341));
#53194=CARTESIAN_POINT('Ctrl Pts',(51.9714428864125,15.6454595543576,17.2900563616205));
#53195=CARTESIAN_POINT('Ctrl Pts',(53.4338717842849,16.1984189929661,17.2187259254479));
#53196=CARTESIAN_POINT('Ctrl Pts',(54.8293009543941,15.1915695541269,17.1402204150712));
#53197=CARTESIAN_POINT('Ctrl Pts',(54.7591722875712,13.4722511753948,17.0617149046944));
#53198=CARTESIAN_POINT('Ctrl Pts',(53.2863785654276,12.582391834622,16.9832093943176));
#53199=CARTESIAN_POINT('Ctrl Pts',(51.9166698060744,13.232298629585,16.9140416672824));
#53200=CARTESIAN_POINT('Ctrl Pts',(51.6557451516705,14.0710086043769,16.8710424437061));
#53201=CARTESIAN_POINT('Ctrl Pts',(51.6537286904076,14.3981451166365,16.8542117235887));
#53202=CARTESIAN_POINT('Ctrl Pts',(51.6531013855762,14.3983675031589,17.3957882764113));
#53203=CARTESIAN_POINT('Ctrl Pts',(51.6519028634372,14.5526188015874,17.3878441566028));
#53204=CARTESIAN_POINT('Ctrl Pts',(51.7435010772427,15.2135959185484,17.3537315333353));
#53205=CARTESIAN_POINT('Ctrl Pts',(52.6846499703254,16.1409815416267,17.293450406609));
#53206=CARTESIAN_POINT('Ctrl Pts',(54.36812854879,15.7848349642755,17.2149448962322));
#53207=CARTESIAN_POINT('Ctrl Pts',(54.9996481235109,14.1841565112764,17.1364393858554));
#53208=CARTESIAN_POINT('Ctrl Pts',(54.0128340063977,12.7744876345319,17.0579338754786));
#53209=CARTESIAN_POINT('Ctrl Pts',(52.292690959438,12.8200454826231,16.9794283651019));
#53210=CARTESIAN_POINT('Ctrl Pts',(51.6656274258073,13.8251612032116,16.9253798320794));
#53211=CARTESIAN_POINT('Ctrl Pts',(51.6498077544378,14.3635106325159,16.8974998025159));
#53212=CARTESIAN_POINT('Ctrl Pts',(51.6499660613832,14.3965688093956,16.8957882764113));
#53213=CARTESIAN_POINT('Origin',(53.1951359564886,14.3971354987959,19.1042117235887));
#53214=CARTESIAN_POINT('',(51.6537934596096,14.3955992295121,17.8957882764113));
#53215=CARTESIAN_POINT('',(51.650238794436,14.3978859537331,17.8542117235887));
#53216=CARTESIAN_POINT('',(51.6521359564886,14.397135498796,19.1042117235887));
#53217=CARTESIAN_POINT('',(52.7966221146313,12.9064860705774,18.));
#53218=CARTESIAN_POINT('Ctrl Pts',(52.7966221146313,12.9064860705774,18.));
#53219=CARTESIAN_POINT('Ctrl Pts',(52.3064323164312,13.0375346028627,17.9738314965411));
#53220=CARTESIAN_POINT('Ctrl Pts',(51.7535553056072,13.5560194656624,17.9390942553448));
#53221=CARTESIAN_POINT('Ctrl Pts',(51.6526562271057,14.2291272515896,17.9043570141486));
#53222=CARTESIAN_POINT('Ctrl Pts',(51.6537934596096,14.3955992295121,17.8957882764113));
#53223=CARTESIAN_POINT('',(53.5946788045247,12.9041246263415,18.));
#53224=CARTESIAN_POINT('Origin',(53.1951359564886,14.3971354987959,18.));
#53225=CARTESIAN_POINT('Ctrl Pts',(53.5946845822246,12.9041113672218,18.));
#53226=CARTESIAN_POINT('Ctrl Pts',(53.1295569761736,12.7814239312717,17.975091839613));
#53227=CARTESIAN_POINT('Ctrl Pts',(52.0976014587089,12.9966708391238,17.9264957474759));
#53228=CARTESIAN_POINT('Ctrl Pts',(51.6531166045831,13.9402254397343,17.8778996553388));
#53229=CARTESIAN_POINT('Ctrl Pts',(51.650238794436,14.3978859537331,17.8542117235887));
#53230=CARTESIAN_POINT('Origin',(53.1951359564886,14.3971354987959,4.5));
#53231=CARTESIAN_POINT('',(54.457664959728,14.3970890371748,5.80658032638058));
#53232=CARTESIAN_POINT('',(54.4588632108481,14.3954785432618,5.94341967361942));
#53233=CARTESIAN_POINT('',(54.4596359564886,14.3971354987959,4.5));
#53234=CARTESIAN_POINT('',(54.153252109211,15.2223467977324,6.));
#53235=CARTESIAN_POINT('Ctrl Pts',(54.4588632108481,14.3954785432618,5.94341967361942));
#53236=CARTESIAN_POINT('Ctrl Pts',(54.4562503558692,14.6946046444959,5.96227978241295));
#53237=CARTESIAN_POINT('Ctrl Pts',(54.348829759182,14.9952702831595,5.98113989120648));
#53238=CARTESIAN_POINT('Ctrl Pts',(54.153252109211,15.2223467977324,6.00000000000001));
#53239=CARTESIAN_POINT('',(54.4596359564886,14.3971354987959,6.));
#53240=CARTESIAN_POINT('Origin',(53.1951359564886,14.3971354987959,6.));
#53241=CARTESIAN_POINT('',(54.4596359564886,14.3971354987959,7.));
#53242=CARTESIAN_POINT('',(54.4596359564886,14.3971354987959,4.5));
#53243=CARTESIAN_POINT('',(52.6278006430704,15.5272199611918,7.));
#53244=CARTESIAN_POINT('Origin',(53.1951359564886,14.3971354987959,7.));
#53245=CARTESIAN_POINT('',(53.7624712699068,13.2670510364,7.));
#53246=CARTESIAN_POINT('Origin',(53.1951359564886,14.3971354987959,7.));
#53247=CARTESIAN_POINT('Origin',(53.1951359564886,14.3971354987959,7.));
#53248=CARTESIAN_POINT('',(52.2352360662266,15.2234730828751,6.));
#53249=CARTESIAN_POINT('Origin',(53.1951359564886,14.3971354987959,6.));
#53250=CARTESIAN_POINT('Ctrl Pts',(52.2352263046383,15.223479246524,6.));
#53251=CARTESIAN_POINT('Ctrl Pts',(52.4934849626836,15.5213201221341,5.97509183961299));
#53252=CARTESIAN_POINT('Ctrl Pts',(52.9025331767737,15.6908484929834,5.95018367922598));
#53253=CARTESIAN_POINT('Ctrl Pts',(53.2954400519545,15.6595806594193,5.92527551883897));
#53254=CARTESIAN_POINT('Ctrl Pts',(53.7082278597432,15.6267306858339,5.89910701538004));
#53255=CARTESIAN_POINT('Ctrl Pts',(54.1031995108901,15.3722499881178,5.87293851192112));
#53256=CARTESIAN_POINT('Ctrl Pts',(54.3034856243485,15.009959026203,5.84677000846219));
#53257=CARTESIAN_POINT('Ctrl Pts',(54.4060190030454,14.8244897704715,5.83337344776832));
#53258=CARTESIAN_POINT('Ctrl Pts',(54.457529785952,14.6107659273806,5.81997688707445));
#53259=CARTESIAN_POINT('Ctrl Pts',(54.457664959728,14.3970890371748,5.80658032638058));
#53260=CARTESIAN_POINT('Origin',(53.1951359564886,14.3971354987959,4.5));
#53261=CARTESIAN_POINT('',(54.4609673117159,14.396357828719,5.30658032638058));
#53262=CARTESIAN_POINT('',(54.4612320294125,14.3977598345137,5.44341967361942));
#53263=CARTESIAN_POINT('',(54.4596359564886,14.3971354987959,4.5));
#53264=CARTESIAN_POINT('Ctrl Pts',(54.4612320294125,14.3977598345137,5.44341967361942));
#53265=CARTESIAN_POINT('Ctrl Pts',(54.4614577199909,14.4349274614079,5.44576692486713));
#53266=CARTESIAN_POINT('Ctrl Pts',(54.4599595944507,14.4720765205797,5.44811417611484));
#53267=CARTESIAN_POINT('Ctrl Pts',(54.4566777507412,14.5090671702315,5.45046142736255));
#53268=CARTESIAN_POINT('Ctrl Pts',(54.4200898743707,14.9214601530044,5.47662993082147));
#53269=CARTESIAN_POINT('Ctrl Pts',(54.1618024272562,15.3141643064504,5.5027984342804));
#53270=CARTESIAN_POINT('Ctrl Pts',(53.7976302145161,15.5111328144605,5.52896693773933));
#53271=CARTESIAN_POINT('Ctrl Pts',(53.4334580017759,15.7081013224707,5.55513544119826));
#53272=CARTESIAN_POINT('Ctrl Pts',(52.9634010234101,15.709334185045,5.58130394465719));
#53273=CARTESIAN_POINT('Ctrl Pts',(52.598247155701,15.5141854678806,5.60747244811611));
#53274=CARTESIAN_POINT('Ctrl Pts',(52.2330932879918,15.3190367507161,5.63364095157504));
#53275=CARTESIAN_POINT('Ctrl Pts',(51.9728425309394,14.9275064538129,5.65980945503396));
#53276=CARTESIAN_POINT('Ctrl Pts',(51.9341769083662,14.5153483233265,5.68597795849289));
#53277=CARTESIAN_POINT('Ctrl Pts',(51.8955112857929,14.1031901928401,5.71214646195181));
#53278=CARTESIAN_POINT('Ctrl Pts',(52.0784307976988,13.6704042287705,5.73831496541074));
#53279=CARTESIAN_POINT('Ctrl Pts',(52.4009468670997,13.4106806439539,5.76448346886967));
#53280=CARTESIAN_POINT('Ctrl Pts',(52.7234629365007,13.1509570591374,5.7906519723286));
#53281=CARTESIAN_POINT('Ctrl Pts',(53.1855755633968,13.0642958535739,5.81682047578752));
#53282=CARTESIAN_POINT('Ctrl Pts',(53.5800025789138,13.1903251026303,5.84298897924645));
#53283=CARTESIAN_POINT('Ctrl Pts',(53.9744295944309,13.3163543516866,5.86915748270537));
#53284=CARTESIAN_POINT('Ctrl Pts',(54.3011709985689,13.6550740553627,5.8953259861643));
#53285=CARTESIAN_POINT('Ctrl Pts',(54.4137178903471,14.0528046923318,5.92149448962323));
#53286=CARTESIAN_POINT('Ctrl Pts',(54.4451502229132,14.1638837408548,5.92880288428863));
#53287=CARTESIAN_POINT('Ctrl Pts',(54.4598757063537,14.2795655532322,5.93611127895402));
#53288=CARTESIAN_POINT('Ctrl Pts',(54.4588632108481,14.3954785432618,5.94341967361942));
#53289=CARTESIAN_POINT('Ctrl Pts',(54.457664959728,14.3970890371748,5.80658032638058));
#53290=CARTESIAN_POINT('Ctrl Pts',(54.4577938309935,14.1933748843944,5.79380838361552));
#53291=CARTESIAN_POINT('Ctrl Pts',(54.4112262077565,13.9897034081911,5.78103644085047));
#53292=CARTESIAN_POINT('Ctrl Pts',(54.3176561881973,13.8105991567174,5.76826449808541));
#53293=CARTESIAN_POINT('Ctrl Pts',(54.1259400628177,13.4436314752601,5.74209599462648));
#53294=CARTESIAN_POINT('Ctrl Pts',(53.7369072362884,13.1797973384592,5.71592749116756));
#53295=CARTESIAN_POINT('Ctrl Pts',(53.3250643574771,13.1373309568652,5.68975898770863));
#53296=CARTESIAN_POINT('Ctrl Pts',(52.9132214786658,13.0948645752712,5.6635904842497));
#53297=CARTESIAN_POINT('Ctrl Pts',(52.4785685475723,13.2737659488842,5.63742198079078));
#53298=CARTESIAN_POINT('Ctrl Pts',(52.2159793451474,13.5938495375153,5.61125347733185));
#53299=CARTESIAN_POINT('Ctrl Pts',(51.9533901427224,13.9139331261464,5.58508497387292));
#53300=CARTESIAN_POINT('Ctrl Pts',(51.8628646689658,14.3751989297955,5.558916470414));
#53301=CARTESIAN_POINT('Ctrl Pts',(51.9850104565428,14.7707919534968,5.53274796695507));
#53302=CARTESIAN_POINT('Ctrl Pts',(52.1071562441199,15.1663849771981,5.50657946349614));
#53303=CARTESIAN_POINT('Ctrl Pts',(52.4419732930305,15.4963052209516,5.48041096003722));
#53304=CARTESIAN_POINT('Ctrl Pts',(52.8393182643656,15.6126214609836,5.45424245657829));
#53305=CARTESIAN_POINT('Ctrl Pts',(53.2366632357006,15.7289377010156,5.42807395311936));
#53306=CARTESIAN_POINT('Ctrl Pts',(53.69653612946,15.6316499373263,5.40190544966044));
#53307=CARTESIAN_POINT('Ctrl Pts',(54.0127281594174,15.3643787057253,5.37573694620151));
#53308=CARTESIAN_POINT('Ctrl Pts',(54.2912662123671,15.1289356793162,5.35268473959453));
#53309=CARTESIAN_POINT('Ctrl Pts',(54.4583064998761,14.7615838076199,5.32963253298755));
#53310=CARTESIAN_POINT('Ctrl Pts',(54.4609673117159,14.396357828719,5.30658032638058));
#53311=CARTESIAN_POINT('Origin',(53.1951359564886,14.3971354987959,4.5));
#53312=CARTESIAN_POINT('',(54.4594541523146,14.3982246410602,4.80658032638058));
#53313=CARTESIAN_POINT('',(54.4577421278041,14.3974029482829,4.94341967361942));
#53314=CARTESIAN_POINT('',(54.4596359564886,14.3971354987959,4.5));
#53315=CARTESIAN_POINT('Ctrl Pts',(54.4577421278041,14.3974029482829,4.94341967361942));
#53316=CARTESIAN_POINT('Ctrl Pts',(54.4581119948619,14.5888150279108,4.95542257078024));
#53317=CARTESIAN_POINT('Ctrl Pts',(54.4171976582396,14.7800770605195,4.96742546794106));
#53318=CARTESIAN_POINT('Ctrl Pts',(54.3341701782111,14.9508661287462,4.97942836510187));
#53319=CARTESIAN_POINT('Ctrl Pts',(54.1531551391583,15.3232174255002,5.0055968685608));
#53320=CARTESIAN_POINT('Ctrl Pts',(53.7719681306168,15.5982567367276,5.03176537201973));
#53321=CARTESIAN_POINT('Ctrl Pts',(53.3615378715941,15.6526538764831,5.05793387547865));
#53322=CARTESIAN_POINT('Ctrl Pts',(52.9511076125715,15.7070510162386,5.08410237893758));
#53323=CARTESIAN_POINT('Ctrl Pts',(52.5114341030678,15.5408059845222,5.11027088239651));
#53324=CARTESIAN_POINT('Ctrl Pts',(52.2396723049569,15.2284636038326,5.13643938585543));
#53325=CARTESIAN_POINT('Ctrl Pts',(51.9679105068461,14.9161212231431,5.16260788931436));
#53326=CARTESIAN_POINT('Ctrl Pts',(51.8640604201282,14.4576814934805,5.18877639277329));
#53327=CARTESIAN_POINT('Ctrl Pts',(51.974689389455,14.0587171002307,5.21494489623222));
#53328=CARTESIAN_POINT('Ctrl Pts',(52.0853183587818,13.659752706981,5.24111339969114));
#53329=CARTESIAN_POINT('Ctrl Pts',(52.4104263841535,13.3202636501442,5.26728190315006));
#53330=CARTESIAN_POINT('Ctrl Pts',(52.804231701646,13.1924751167177,5.29345040660899));
#53331=CARTESIAN_POINT('Ctrl Pts',(53.1980370191385,13.0646865832913,5.31961891006791));
#53332=CARTESIAN_POINT('Ctrl Pts',(53.6605396287519,13.1485985732751,5.34578741352685));
#53333=CARTESIAN_POINT('Ctrl Pts',(53.9843467807452,13.406595474317,5.37195591698577));
#53334=CARTESIAN_POINT('Ctrl Pts',(54.2791092171044,13.6414506795096,5.39577716919699));
#53335=CARTESIAN_POINT('Ctrl Pts',(54.4589415919506,14.0205614348097,5.4195984214082));
#53336=CARTESIAN_POINT('Ctrl Pts',(54.4612320294125,14.3977598345137,5.44341967361942));
#53337=CARTESIAN_POINT('Ctrl Pts',(54.4609673117159,14.396357828719,5.30658032638058));
#53338=CARTESIAN_POINT('Ctrl Pts',(54.4613270117525,14.3469850034748,5.30346402952863));
#53339=CARTESIAN_POINT('Ctrl Pts',(54.4586827097295,14.2976510284966,5.30034773267668));
#53340=CARTESIAN_POINT('Ctrl Pts',(54.4529037631581,14.2486870321021,5.29723143582473));
#53341=CARTESIAN_POINT('Ctrl Pts',(54.4043761707862,13.8375212895923,5.27106293236581));
#53342=CARTESIAN_POINT('Ctrl Pts',(54.134809819887,13.4524445040854,5.24489442890688));
#53343=CARTESIAN_POINT('Ctrl Pts',(53.7650823822708,13.2661285769126,5.21872592544795));
#53344=CARTESIAN_POINT('Ctrl Pts',(53.3953549446545,13.0798126497399,5.19255742198903));
#53345=CARTESIAN_POINT('Ctrl Pts',(52.9254664203212,13.0922575809014,5.1663889185301));
#53346=CARTESIAN_POINT('Ctrl Pts',(52.5661199525803,13.2978834669457,5.14022041507117));
#53347=CARTESIAN_POINT('Ctrl Pts',(52.2067734848394,13.5035093529901,5.11405191161225));
#53348=CARTESIAN_POINT('Ctrl Pts',(51.9579690736908,13.9023161939173,5.08788340815332));
#53349=CARTESIAN_POINT('Ctrl Pts',(51.9312738021255,14.315473986753,5.06171490469439));
#53350=CARTESIAN_POINT('Ctrl Pts',(51.9045785305602,14.7286317795887,5.03554640123547));
#53351=CARTESIAN_POINT('Ctrl Pts',(52.0999923985782,15.1561405243328,5.00937789777654));
#53352=CARTESIAN_POINT('Ctrl Pts',(52.4298893914915,15.4063003551787,4.98320939431761));
#53353=CARTESIAN_POINT('Ctrl Pts',(52.7597863844047,15.6564601860247,4.95704089085869));
#53354=CARTESIAN_POINT('Ctrl Pts',(53.2241665022132,15.7292711029725,4.93087238739976));
#53355=CARTESIAN_POINT('Ctrl Pts',(53.6147962366242,15.5920837570554,4.90470388394083));
#53356=CARTESIAN_POINT('Ctrl Pts',(54.0054259710351,15.4548964111382,4.87853538048191));
#53357=CARTESIAN_POINT('Ctrl Pts',(54.3223053220485,15.107710802356,4.85236687702298));
#53358=CARTESIAN_POINT('Ctrl Pts',(54.4233417938017,14.706209118673,4.82619837356406));
#53359=CARTESIAN_POINT('Ctrl Pts',(54.4485901905141,14.6058763020728,4.8196590245029));
#53360=CARTESIAN_POINT('Ctrl Pts',(54.460359856649,14.5021516119852,4.81311967544174));
#53361=CARTESIAN_POINT('Ctrl Pts',(54.4594541523146,14.3982246410602,4.80658032638058));
#53362=CARTESIAN_POINT('Origin',(53.1951359564886,14.3971354987959,4.5));
#53363=CARTESIAN_POINT('',(54.4581341693109,14.3964211317122,4.30658032638058));
#53364=CARTESIAN_POINT('',(54.4603880160508,14.3961458582298,4.44341967361942));
#53365=CARTESIAN_POINT('',(54.4596359564886,14.3971354987959,4.5));
#53366=CARTESIAN_POINT('Ctrl Pts',(54.4603880160508,14.3961458582298,4.44341967361942));
#53367=CARTESIAN_POINT('Ctrl Pts',(54.4574339233842,14.7397014586706,4.46507821669335));
#53368=CARTESIAN_POINT('Ctrl Pts',(54.312116901092,15.0854595650489,4.48673675976727));
#53369=CARTESIAN_POINT('Ctrl Pts',(54.0623960097695,15.3201070497197,4.50839530284119));
#53370=CARTESIAN_POINT('Ctrl Pts',(53.7606757146401,15.6036152013657,4.53456380630012));
#53371=CARTESIAN_POINT('Ctrl Pts',(53.3065445684699,15.7249218506019,4.56073230975905));
#53372=CARTESIAN_POINT('Ctrl Pts',(52.9036403743547,15.6296316648431,4.58690081321798));
#53373=CARTESIAN_POINT('Ctrl Pts',(52.5007361802396,15.5343414790843,4.6130693166769));
#53374=CARTESIAN_POINT('Ctrl Pts',(52.1490589381795,15.2224544583304,4.63923782013583));
#53375=CARTESIAN_POINT('Ctrl Pts',(52.0063049058888,14.8338244281946,4.66540632359475));
#53376=CARTESIAN_POINT('Ctrl Pts',(51.863550873598,14.4451943980587,4.69157482705368));
#53377=CARTESIAN_POINT('Ctrl Pts',(51.9297200510767,13.9798213585408,4.71774333051261));
#53378=CARTESIAN_POINT('Ctrl Pts',(52.1751413884872,13.6463841561873,4.74391183397154));
#53379=CARTESIAN_POINT('Ctrl Pts',(52.4205627258978,13.3129469538339,4.77008033743046));
#53380=CARTESIAN_POINT('Ctrl Pts',(52.8452362232402,13.111445588645,4.79624884088939));
#53381=CARTESIAN_POINT('Ctrl Pts',(53.2587332445463,13.1322355800464,4.82241734434831));
#53382=CARTESIAN_POINT('Ctrl Pts',(53.6722302658525,13.1530255714477,4.84858584780724));
#53383=CARTESIAN_POINT('Ctrl Pts',(54.0745508111225,13.3961069194393,4.87475435126617));
#53384=CARTESIAN_POINT('Ctrl Pts',(54.2852895489753,13.7524792345754,4.90092285472509));
#53385=CARTESIAN_POINT('Ctrl Pts',(54.3993672224223,13.9453916768054,4.9150884610232));
#53386=CARTESIAN_POINT('Ctrl Pts',(54.4573056172638,14.1715018075515,4.92925406732131));
#53387=CARTESIAN_POINT('Ctrl Pts',(54.4577421278041,14.3974029482829,4.94341967361942));
#53388=CARTESIAN_POINT('Ctrl Pts',(54.4594541523146,14.3982246410602,4.80658032638058));
#53389=CARTESIAN_POINT('Ctrl Pts',(54.4567355009545,14.0862672062605,4.78695117198281));
#53390=CARTESIAN_POINT('Ctrl Pts',(54.3398093025916,13.7724871818732,4.76732201758504));
#53391=CARTESIAN_POINT('Ctrl Pts',(54.1304031431366,13.5431499271195,4.74769286318727));
#53392=CARTESIAN_POINT('Ctrl Pts',(53.8512344282254,13.2374101778329,4.72152435972835));
#53393=CARTESIAN_POINT('Ctrl Pts',(53.4077034059102,13.0817484378434,4.69535585626942));
#53394=CARTESIAN_POINT('Ctrl Pts',(52.9986946517684,13.1459652901465,4.66918735281049));
#53395=CARTESIAN_POINT('Ctrl Pts',(52.5896858976267,13.2101821424497,4.64301884935157));
#53396=CARTESIAN_POINT('Ctrl Pts',(52.2151994116584,13.4942775870456,4.61685034589264));
#53397=CARTESIAN_POINT('Ctrl Pts',(52.0431593891151,13.8708598453683,4.59068184243372));
#53398=CARTESIAN_POINT('Ctrl Pts',(51.8711193665719,14.247442103691,4.56451333897479));
#53399=CARTESIAN_POINT('Ctrl Pts',(51.9015258074537,14.7165111757404,4.53834483551586));
#53400=CARTESIAN_POINT('Ctrl Pts',(52.1207441004937,15.0677309159732,4.51217633205694));
#53401=CARTESIAN_POINT('Ctrl Pts',(52.3399623935336,15.4189506562059,4.48600782859801));
#53402=CARTESIAN_POINT('Ctrl Pts',(52.7479925387317,15.6523210646219,4.45983932513909));
#53403=CARTESIAN_POINT('Ctrl Pts',(53.1618689696675,15.6631960750064,4.43367082168016));
#53404=CARTESIAN_POINT('Ctrl Pts',(53.5757454006032,15.6740710853908,4.40750231822123));
#53405=CARTESIAN_POINT('Ctrl Pts',(53.9954681172766,15.4624506977437,4.38133381476231));
#53406=CARTESIAN_POINT('Ctrl Pts',(54.2328284639311,15.1232280099042,4.35516531130338));
#53407=CARTESIAN_POINT('Ctrl Pts',(54.3797245073824,14.9132920564272,4.33897031632911));
#53408=CARTESIAN_POINT('Ctrl Pts',(54.4567749448579,14.6544838494259,4.32277532135484));
#53409=CARTESIAN_POINT('Ctrl Pts',(54.4581341693109,14.3964211317122,4.30658032638058));
#53410=CARTESIAN_POINT('Origin',(53.1951359564886,14.3971354987959,4.5));
#53411=CARTESIAN_POINT('',(54.461625037427,14.3970459917425,3.80658032638058));
#53412=CARTESIAN_POINT('',(54.4600990366243,14.3981838592136,3.94341967361942));
#53413=CARTESIAN_POINT('',(54.4596359564886,14.3971354987959,4.5));
#53414=CARTESIAN_POINT('Ctrl Pts',(54.4600990366243,14.3981838592136,3.94341967361942));
#53415=CARTESIAN_POINT('Ctrl Pts',(54.460821703013,14.4798548702781,3.94856535914753));
#53416=CARTESIAN_POINT('Ctrl Pts',(54.4535723073139,14.5613982175719,3.95371104467563));
#53417=CARTESIAN_POINT('Ctrl Pts',(54.4378783642807,14.6412825634277,3.95885673020374));
#53418=CARTESIAN_POINT('Ctrl Pts',(54.3580664518924,15.0475362626526,3.98502523366266));
#53419=CARTESIAN_POINT('Ctrl Pts',(54.0598570383511,15.410883959442,4.0111937371216));
#53420=CARTESIAN_POINT('Ctrl Pts',(53.6769707694449,15.5683962274082,4.03736224058052));
#53421=CARTESIAN_POINT('Ctrl Pts',(53.2940845005387,15.7259084953743,4.06353074403945));
#53422=CARTESIAN_POINT('Ctrl Pts',(52.8265213762676,15.6775853345172,4.08969924749837));
#53423=CARTESIAN_POINT('Ctrl Pts',(52.4839422593842,15.4450954247484,4.1158677509573));
#53424=CARTESIAN_POINT('Ctrl Pts',(52.1413631425007,15.2126055149797,4.14203625441622));
#53425=CARTESIAN_POINT('Ctrl Pts',(51.9237680330049,14.7959488562993,4.16820475787515));
#53426=CARTESIAN_POINT('Ctrl Pts',(51.9287291645367,14.3819592468436,4.19437326133408));
#53427=CARTESIAN_POINT('Ctrl Pts',(51.9336902960684,13.967969637388,4.22054176479301));
#53428=CARTESIAN_POINT('Ctrl Pts',(52.1612076686277,13.5566470771571,4.24671026825193));
#53429=CARTESIAN_POINT('Ctrl Pts',(52.5092597878395,13.3324334921487,4.27287877171086));
#53430=CARTESIAN_POINT('Ctrl Pts',(52.8573119070513,13.1082199071402,4.29904727516979));
#53431=CARTESIAN_POINT('Ctrl Pts',(53.3258987729157,13.0711152973543,4.32521577862871));
#53432=CARTESIAN_POINT('Ctrl Pts',(53.7049004648973,13.2377578095269,4.35138428208764));
#53433=CARTESIAN_POINT('Ctrl Pts',(54.0839021568789,13.4044003216995,4.37755278554656));
#53434=CARTESIAN_POINT('Ctrl Pts',(54.3733186749776,13.7747899558306,4.40372128900549));
#53435=CARTESIAN_POINT('Ctrl Pts',(54.4433722119826,14.1828395999241,4.42988979246442));
#53436=CARTESIAN_POINT('Ctrl Pts',(54.4554454540469,14.2531641308192,4.43439975284942));
#53437=CARTESIAN_POINT('Ctrl Pts',(54.4610031470343,14.3246072444484,4.43890971323442));
#53438=CARTESIAN_POINT('Ctrl Pts',(54.4603880160508,14.3961458582298,4.44341967361942));
#53439=CARTESIAN_POINT('Ctrl Pts',(54.4581341693109,14.3964211317122,4.30658032638058));
#53440=CARTESIAN_POINT('Ctrl Pts',(54.4589712326528,14.237496062036,4.29660681789592));
#53441=CARTESIAN_POINT('Ctrl Pts',(54.4311018285097,14.0788537248349,4.28663330941126));
#53442=CARTESIAN_POINT('Ctrl Pts',(54.3731606475783,13.9320829192412,4.2766598009266));
#53443=CARTESIAN_POINT('Ctrl Pts',(54.2211345079355,13.5469855044494,4.25049129746767));
#53444=CARTESIAN_POINT('Ctrl Pts',(53.8620842520145,13.2436156628976,4.22432279400875));
#53445=CARTESIAN_POINT('Ctrl Pts',(53.4570122824292,13.1580080377804,4.19815429054982));
#53446=CARTESIAN_POINT('Ctrl Pts',(53.0519403128439,13.0724004126631,4.17198578709089));
#53447=CARTESIAN_POINT('Ctrl Pts',(52.6008466295945,13.2045550039804,4.14581728363197));
#53448=CARTESIAN_POINT('Ctrl Pts',(52.3060070023708,13.4952121220022,4.11964878017304));
#53449=CARTESIAN_POINT('Ctrl Pts',(52.0111673751471,13.7858692400241,4.09348027671411));
#53450=CARTESIAN_POINT('Ctrl Pts',(51.8725818039492,14.2350288847506,4.06731177325519));
#53451=CARTESIAN_POINT('Ctrl Pts',(51.9523937062209,14.6412825324807,4.04114326979626));
#53452=CARTESIAN_POINT('Ctrl Pts',(52.0322056084927,15.0475361802107,4.01497476633734));
#53453=CARTESIAN_POINT('Ctrl Pts',(52.3304149842342,15.4108838309442,3.98880626287841));
#53454=CARTESIAN_POINT('Ctrl Pts',(52.7133012046075,15.5683960789447,3.96263775941948));
#53455=CARTESIAN_POINT('Ctrl Pts',(53.0961874249807,15.7259083269452,3.93646925596055));
#53456=CARTESIAN_POINT('Ctrl Pts',(53.5637504899858,15.6775851722127,3.91030075250163));
#53457=CARTESIAN_POINT('Ctrl Pts',(53.9063295634455,15.4450952919135,3.8841322490427));
#53458=CARTESIAN_POINT('Ctrl Pts',(54.2447474105889,15.2154294107524,3.85828160815533));
#53459=CARTESIAN_POINT('Ctrl Pts',(54.4611991270569,14.8060436899639,3.83243096726795));
#53460=CARTESIAN_POINT('Ctrl Pts',(54.461625037427,14.3970459917425,3.80658032638058));
#53461=CARTESIAN_POINT('Origin',(53.1951359564886,14.3971354987959,4.5));
#53462=CARTESIAN_POINT('',(54.458326569365,14.3979628849946,3.30658032638058));
#53463=CARTESIAN_POINT('',(54.4578259861007,14.3967173602322,3.44341967361942));
#53464=CARTESIAN_POINT('',(54.4596359564886,14.3971354987959,4.5));
#53465=CARTESIAN_POINT('Ctrl Pts',(54.4578259861007,14.3967173602322,3.44341967361942));
#53466=CARTESIAN_POINT('Ctrl Pts',(54.4571098189798,14.6327171768276,3.45822100506063));
#53467=CARTESIAN_POINT('Ctrl Pts',(54.3935213986439,14.8690753747194,3.47302233650185));
#53468=CARTESIAN_POINT('Ctrl Pts',(54.2695279486697,15.0677310009766,3.48782366794306));
#53469=CARTESIAN_POINT('Ctrl Pts',(54.0503096278436,15.4189507857301,3.51399217140199));
#53470=CARTESIAN_POINT('Ctrl Pts',(53.6422794309233,15.6523212237234,3.54016067486092));
#53471=CARTESIAN_POINT('Ctrl Pts',(53.228402947526,15.6631962354854,3.56632917831984));
#53472=CARTESIAN_POINT('Ctrl Pts',(52.8145264641287,15.6740712472475,3.59249768177877));
#53473=CARTESIAN_POINT('Ctrl Pts',(52.3948036942543,15.4624508327782,3.61866618523769));
#53474=CARTESIAN_POINT('Ctrl Pts',(52.1574433175134,15.1232281019409,3.64483468869662));
#53475=CARTESIAN_POINT('Ctrl Pts',(51.9200829407725,14.7840053711036,3.67100319215555));
#53476=CARTESIAN_POINT('Ctrl Pts',(51.865084957165,14.3171803238982,3.69717169561448));
#53477=CARTESIAN_POINT('Ctrl Pts',(52.0171111160778,13.932082860293,3.7233401990734));
#53478=CARTESIAN_POINT('Ctrl Pts',(52.1691372749905,13.5469853966878,3.74950870253233));
#53479=CARTESIAN_POINT('Ctrl Pts',(52.5281875764236,13.2436155166828,3.77567720599125));
#53480=CARTESIAN_POINT('Ctrl Pts',(52.933259597354,13.1580078807144,3.80184570945018));
#53481=CARTESIAN_POINT('Ctrl Pts',(53.3383316182844,13.072400244746,3.82801421290911));
#53482=CARTESIAN_POINT('Ctrl Pts',(53.7894253587122,13.2045548528142,3.85418271636804));
#53483=CARTESIAN_POINT('Ctrl Pts',(54.0842650233083,13.4952120076785,3.88035121982696));
#53484=CARTESIAN_POINT('Ctrl Pts',(54.3211284189289,13.7287153280572,3.90137403775778));
#53485=CARTESIAN_POINT('Ctrl Pts',(54.4571465662818,14.0645150435707,3.9223968556886));
#53486=CARTESIAN_POINT('Ctrl Pts',(54.4600990366243,14.3981838592136,3.94341967361942));
#53487=CARTESIAN_POINT('Ctrl Pts',(54.461625037427,14.3970459917425,3.80658032638058));
#53488=CARTESIAN_POINT('Ctrl Pts',(54.4616302744719,14.3920169071375,3.80626246380903));
#53489=CARTESIAN_POINT('Ctrl Pts',(54.4616028495907,14.3869878811994,3.80594460123748));
#53490=CARTESIAN_POINT('Ctrl Pts',(54.4615425879167,14.3819592487679,3.80562673866592));
#53491=CARTESIAN_POINT('Ctrl Pts',(54.4565814570138,13.9679696917871,3.779458235207));
#53492=CARTESIAN_POINT('Ctrl Pts',(54.2290641132938,13.5566471836914,3.75328973174807));
#53493=CARTESIAN_POINT('Ctrl Pts',(53.8810120381993,13.3324336271042,3.72712122828914));
#53494=CARTESIAN_POINT('Ctrl Pts',(53.5329599631049,13.1082200705171,3.70095272483021));
#53495=CARTESIAN_POINT('Ctrl Pts',(53.0643731566361,13.0711154654387,3.67478422137129));
#53496=CARTESIAN_POINT('Ctrl Pts',(52.6853715126953,13.2377579564865,3.64861571791236));
#53497=CARTESIAN_POINT('Ctrl Pts',(52.3063698687544,13.4044004475342,3.62244721445344));
#53498=CARTESIAN_POINT('Ctrl Pts',(52.0169533873414,13.7747900347083,3.59627871099451));
#53499=CARTESIAN_POINT('Ctrl Pts',(51.9468998592157,14.182839627083,3.57011020753558));
#53500=CARTESIAN_POINT('Ctrl Pts',(51.8768463310901,14.5908892194578,3.54394170407666));
#53501=CARTESIAN_POINT('Ctrl Pts',(52.0261557562516,15.0365988170334,3.51777320061773));
#53502=CARTESIAN_POINT('Ctrl Pts',(52.327876013137,15.3201069327361,3.4916046971588));
#53503=CARTESIAN_POINT('Ctrl Pts',(52.6295962700224,15.6036150484389,3.46543619369988));
#53504=CARTESIAN_POINT('Ctrl Pts',(53.0837273586317,15.7249216822689,3.43926769024095));
#53505=CARTESIAN_POINT('Ctrl Pts',(53.4866315016751,15.6296315086021,3.41309918678203));
#53506=CARTESIAN_POINT('Ctrl Pts',(53.8895356447186,15.5343413349353,3.3869306833231));
#53507=CARTESIAN_POINT('Ctrl Pts',(54.2412128421963,15.2224543537718,3.36076217986417));
#53508=CARTESIAN_POINT('Ctrl Pts',(54.3839668563951,14.8338243728713,3.33459367640525));
#53509=CARTESIAN_POINT('Ctrl Pts',(54.4349061872521,14.6951484043591,3.32525589306369));
#53510=CARTESIAN_POINT('Ctrl Pts',(54.4592433859174,14.5467007705307,3.31591810972213));
#53511=CARTESIAN_POINT('Ctrl Pts',(54.458326569365,14.3979628849946,3.30658032638058));
#53512=CARTESIAN_POINT('Origin',(53.1951359564886,14.3971354987959,4.5));
#53513=CARTESIAN_POINT('',(54.4591686783466,14.3960664985434,2.80658032638058));
#53514=CARTESIAN_POINT('',(54.4614103817624,14.3966710984295,2.94341967361942));
#53515=CARTESIAN_POINT('',(54.4596359564886,14.3971354987959,4.5));
#53516=CARTESIAN_POINT('Ctrl Pts',(54.4614103817624,14.3966710984295,2.94341967361942));
#53517=CARTESIAN_POINT('Ctrl Pts',(54.4595565487343,14.7837947911815,2.96787665097374));
#53518=CARTESIAN_POINT('Ctrl Pts',(54.2687030511239,15.172502088678,2.99233362832806));
#53519=CARTESIAN_POINT('Ctrl Pts',(53.9603826185353,15.4063004831901,3.01679060568238));
#53520=CARTESIAN_POINT('Ctrl Pts',(53.6304855838459,15.6564603458274,3.04295910914131));
#53521=CARTESIAN_POINT('Ctrl Pts',(53.1661054070793,15.729271271822,3.06912761260024));
#53522=CARTESIAN_POINT('Ctrl Pts',(52.7754756231319,15.5920839084722,3.09529611605917));
#53523=CARTESIAN_POINT('Ctrl Pts',(52.3848458391846,15.4548965451224,3.12146461951809));
#53524=CARTESIAN_POINT('Ctrl Pts',(52.0679664480565,15.1077108924282,3.14763312297702));
#53525=CARTESIAN_POINT('Ctrl Pts',(51.9669299635083,14.7062091578755,3.17380162643594));
#53526=CARTESIAN_POINT('Ctrl Pts',(51.8658934789601,14.3047074233228,3.19997012989487));
#53527=CARTESIAN_POINT('Ctrl Pts',(51.980699900992,13.8488896069116,3.2261386333538));
#53528=CARTESIAN_POINT('Ctrl Pts',(52.2598686512828,13.5431498188588,3.25230713681273));
#53529=CARTESIAN_POINT('Ctrl Pts',(52.5390374015737,13.237410030806,3.27847564027165));
#53530=CARTESIAN_POINT('Ctrl Pts',(52.9825684801236,13.0817482711116,3.30464414373058));
#53531=CARTESIAN_POINT('Ctrl Pts',(53.3915772861129,13.1459651315609,3.3308126471895));
#53532=CARTESIAN_POINT('Ctrl Pts',(53.8005860921022,13.2101819920102,3.35698115064843));
#53533=CARTESIAN_POINT('Ctrl Pts',(54.1750726255309,13.4942774726031,3.38314965410736));
#53534=CARTESIAN_POINT('Ctrl Pts',(54.3471126698793,13.8708597786564,3.40931815756629));
#53535=CARTESIAN_POINT('Ctrl Pts',(54.4218440652422,14.0344410036375,3.420685329584));
#53536=CARTESIAN_POINT('Ctrl Pts',(54.4583759903277,14.2154734956486,3.43205250160171));
#53537=CARTESIAN_POINT('Ctrl Pts',(54.4578259861007,14.3967173602322,3.44341967361942));
#53538=CARTESIAN_POINT('Ctrl Pts',(54.458326569365,14.3979628849946,3.30658032638058));
#53539=CARTESIAN_POINT('Ctrl Pts',(54.4566740698126,14.1298729507199,3.28974960626321));
#53540=CARTESIAN_POINT('Ctrl Pts',(54.3729773016518,13.8608400579149,3.27291888614584));
#53541=CARTESIAN_POINT('Ctrl Pts',(54.2151303952057,13.6463842512931,3.25608816602847));
#53542=CARTESIAN_POINT('Ctrl Pts',(53.9697090888974,13.3129470912529,3.22991966256954));
#53543=CARTESIAN_POINT('Ctrl Pts',(53.5450356453608,13.11144575181,3.20375115911061));
#53544=CARTESIAN_POINT('Ctrl Pts',(53.1315386764807,13.1322357404855,3.17758265565169));
#53545=CARTESIAN_POINT('Ctrl Pts',(52.7180417076007,13.153025729161,3.15141415219276));
#53546=CARTESIAN_POINT('Ctrl Pts',(52.3157212133773,13.396107045955,3.12524564873383));
#53547=CARTESIAN_POINT('Ctrl Pts',(52.1049825022091,13.7524793160883,3.09907714527491));
#53548=CARTESIAN_POINT('Ctrl Pts',(51.8942437910409,14.1088515862216,3.07290864181598));
#53549=CARTESIAN_POINT('Ctrl Pts',(51.8750868629279,14.5785148096942,3.04674013835705));
#53550=CARTESIAN_POINT('Ctrl Pts',(52.0561018790939,14.9508660589359,3.02057163489813));
#53551=CARTESIAN_POINT('Ctrl Pts',(52.2371168952598,15.3232173081776,2.9944031314392));
#53552=CARTESIAN_POINT('Ctrl Pts',(52.6183038557047,15.5982565831885,2.96823462798028));
#53553=CARTESIAN_POINT('Ctrl Pts',(53.0287340625826,15.6526537166303,2.94206612452135));
#53554=CARTESIAN_POINT('Ctrl Pts',(53.4391642694604,15.7070508500722,2.91589762106242));
#53555=CARTESIAN_POINT('Ctrl Pts',(53.8788377227713,15.5408058419451,2.88972911760349));
#53556=CARTESIAN_POINT('Ctrl Pts',(54.150599486686,15.2284634997803,2.86356061414457));
#53557=CARTESIAN_POINT('Ctrl Pts',(54.3478475962364,15.0017614956533,2.8445671848899));
#53558=CARTESIAN_POINT('Ctrl Pts',(54.4566391704649,14.6980948440071,2.82557375563524));
#53559=CARTESIAN_POINT('Ctrl Pts',(54.4591686783466,14.3960664985434,2.80658032638058));
#53560=CARTESIAN_POINT('Origin',(53.1951359564886,14.3971354987959,4.5));
#53561=CARTESIAN_POINT('',(54.4611870990995,14.3977489718831,2.30658032638058));
#53562=CARTESIAN_POINT('',(54.4588409672492,14.3981450852038,2.44341967361942));
#53563=CARTESIAN_POINT('',(54.4596359564886,14.3971354987959,4.5));
#53564=CARTESIAN_POINT('',(52.2370198037663,15.2223467977324,2.));
#53565=CARTESIAN_POINT('Ctrl Pts',(54.4611870990995,14.3977489718831,2.30658032638058));
#53566=CARTESIAN_POINT('Ctrl Pts',(54.4588273697934,14.0226957918939,2.2828923946305));
#53567=CARTESIAN_POINT('Ctrl Pts',(54.2812687919142,13.6457847405029,2.25920446288042));
#53568=CARTESIAN_POINT('Ctrl Pts',(53.9893248675414,13.4106809034345,2.23551653113033));
#53569=CARTESIAN_POINT('Ctrl Pts',(53.6668089267086,13.1509572754522,2.20934802767141));
#53570=CARTESIAN_POINT('Ctrl Pts',(53.2046966949687,13.064295685136,2.18317952421248));
#53571=CARTESIAN_POINT('Ctrl Pts',(52.8102694972366,13.190325107422,2.15701102075355));
#53572=CARTESIAN_POINT('Ctrl Pts',(52.4158422995045,13.316354529708,2.13084251729463));
#53573=CARTESIAN_POINT('Ctrl Pts',(52.0891001357801,13.6550749645963,2.1046740138357));
#53574=CARTESIAN_POINT('Ctrl Pts',(51.9765532487624,14.05280555706,2.07850551037678));
#53575=CARTESIAN_POINT('Ctrl Pts',(51.8640063617447,14.4505361495237,2.05233700691785));
#53576=CARTESIAN_POINT('Ctrl Pts',(51.9656547514336,14.9072768995629,2.02616850345892));
#53577=CARTESIAN_POINT('Ctrl Pts',(52.2370198037663,15.2223467977324,2.));
#53578=CARTESIAN_POINT('',(54.1550359790163,15.2234729584199,2.));
#53579=CARTESIAN_POINT('Origin',(53.1951359564886,14.3971354987959,2.));
#53580=CARTESIAN_POINT('Ctrl Pts',(54.1550457523823,15.2234791283661,2.));
#53581=CARTESIAN_POINT('Ctrl Pts',(53.8967871302309,15.5213198394325,2.02490816038701));
#53582=CARTESIAN_POINT('Ctrl Pts',(53.4877388130256,15.6908487049404,2.04981632077402));
#53583=CARTESIAN_POINT('Ctrl Pts',(53.0948318598941,15.6595809742728,2.07472448116103));
#53584=CARTESIAN_POINT('Ctrl Pts',(52.6820439702103,15.6267311087904,2.10089298461996));
#53585=CARTESIAN_POINT('Ctrl Pts',(52.2870722649439,15.3722500867662,2.12706148807889));
#53586=CARTESIAN_POINT('Ctrl Pts',(52.0867861333633,15.0099590154002,2.15322999153781));
#53587=CARTESIAN_POINT('Ctrl Pts',(51.8865000017826,14.6476679440343,2.17939849499674));
#53588=CARTESIAN_POINT('Ctrl Pts',(51.8808994438879,14.1775668233265,2.20556699845567));
#53589=CARTESIAN_POINT('Ctrl Pts',(52.0726155940678,13.8105991317322,2.23173550191459));
#53590=CARTESIAN_POINT('Ctrl Pts',(52.2643317442477,13.4436314401379,2.25790400537352));
#53591=CARTESIAN_POINT('Ctrl Pts',(52.6533646025024,13.1797971776571,2.28407250883245));
#53592=CARTESIAN_POINT('Ctrl Pts',(53.065207531184,13.1373307700534,2.31024101229137));
#53593=CARTESIAN_POINT('Ctrl Pts',(53.4770504598656,13.0948643624498,2.3364095157503));
#53594=CARTESIAN_POINT('Ctrl Pts',(53.9117034589741,13.2737658097233,2.36257801920922));
#53595=CARTESIAN_POINT('Ctrl Pts',(54.1742926968884,13.5938494504631,2.38874652266815));
#53596=CARTESIAN_POINT('Ctrl Pts',(54.3571662426276,13.8167634997217,2.40697090631857));
#53597=CARTESIAN_POINT('Ctrl Pts',(54.456587675354,14.1081518882761,2.425195289969));
#53598=CARTESIAN_POINT('Ctrl Pts',(54.4588409672492,14.3981450852038,2.44341967361942));
#53599=CARTESIAN_POINT('Origin',(53.1951359564886,14.3971354987959,0.895788276411274));
#53600=CARTESIAN_POINT('',(54.7400835567429,14.3978973414314,5.60421172358873));
#53601=CARTESIAN_POINT('',(54.7357308572386,14.3970788042278,5.64578827641127));
#53602=CARTESIAN_POINT('',(54.7381359564886,14.3971354987959,0.895788276411274));
#53603=CARTESIAN_POINT('',(52.7966221146314,12.9064860705774,6.));
#53604=CARTESIAN_POINT('Ctrl Pts',(54.7357308572386,14.3970788042278,5.64578827641127));
#53605=CARTESIAN_POINT('Ctrl Pts',(54.7355659120932,14.6578169944908,5.65918483710514));
#53606=CARTESIAN_POINT('Ctrl Pts',(54.5499292284113,15.4280437939379,5.69874990125794));
#53607=CARTESIAN_POINT('Ctrl Pts',(53.3392716219708,16.2080719085829,5.76448346886966));
#53608=CARTESIAN_POINT('Ctrl Pts',(51.7629444164752,15.5169955192796,5.84298897924645));
#53609=CARTESIAN_POINT('Ctrl Pts',(51.4734277108623,13.8186461670281,5.92149448962322));
#53610=CARTESIAN_POINT('Ctrl Pts',(52.3064323164313,13.0375346028627,5.97383149654107));
#53611=CARTESIAN_POINT('Ctrl Pts',(52.7966221146314,12.9064860705774,6.));
#53612=CARTESIAN_POINT('',(53.5946738441132,12.904124289093,6.));
#53613=CARTESIAN_POINT('Origin',(53.1951359564886,14.3971354987959,6.));
#53614=CARTESIAN_POINT('Ctrl Pts',(54.7400835567429,14.3978973414314,5.60421172358873));
#53615=CARTESIAN_POINT('Ctrl Pts',(54.740358954578,14.443250958116,5.60655897483644));
#53616=CARTESIAN_POINT('Ctrl Pts',(54.7181503847516,14.9939574593074,5.63507472954307));
#53617=CARTESIAN_POINT('Ctrl Pts',(54.0595320288467,15.9953308004787,5.68975898770864));
#53618=CARTESIAN_POINT('Ctrl Pts',(52.3387777758966,15.9998439842325,5.76826449808541));
#53619=CARTESIAN_POINT('Ctrl Pts',(51.386068598834,14.5665551393412,5.8467700084622));
#53620=CARTESIAN_POINT('Ctrl Pts',(52.0449383322286,13.007675117235,5.92401517576705));
#53621=CARTESIAN_POINT('Ctrl Pts',(53.1295481846289,12.781420423434,5.97509183961299));
#53622=CARTESIAN_POINT('Ctrl Pts',(53.5946794545978,12.9041113494969,6.));
#53623=CARTESIAN_POINT('Origin',(53.1951359564886,14.3971354987959,0.895788276411274));
#53624=CARTESIAN_POINT('',(54.7358250212096,14.397461852737,5.10421172358873));
#53625=CARTESIAN_POINT('',(54.7397605362559,14.3961865506515,5.14578827641127));
#53626=CARTESIAN_POINT('',(54.7381359564886,14.3971354987959,0.895788276411274));
#53627=CARTESIAN_POINT('Ctrl Pts',(54.7397605362559,14.3961865506515,5.14578827641127));
#53628=CARTESIAN_POINT('Ctrl Pts',(54.7365136934968,14.8418517823193,5.16884048301825));
#53629=CARTESIAN_POINT('Ctrl Pts',(54.3012988565586,15.7989681003252,5.21806119308416));
#53630=CARTESIAN_POINT('Ctrl Pts',(52.6846517467245,16.1409756074537,5.29345040660899));
#53631=CARTESIAN_POINT('Ctrl Pts',(51.4589751002972,14.933224869348,5.37195591698576));
#53632=CARTESIAN_POINT('Ctrl Pts',(51.7903649128864,13.2446527814935,5.45046142736255));
#53633=CARTESIAN_POINT('Ctrl Pts',(53.3815143142557,12.5897421777335,5.52896693773932));
#53634=CARTESIAN_POINT('Ctrl Pts',(54.5626373610633,13.3907557638884,5.59407588742224));
#53635=CARTESIAN_POINT('Ctrl Pts',(54.7358881117761,14.1484975960505,5.63301633364622));
#53636=CARTESIAN_POINT('Ctrl Pts',(54.7357308572386,14.3970788042278,5.64578827641127));
#53637=CARTESIAN_POINT('Ctrl Pts',(54.7358250212096,14.397461852737,5.10421172358873));
#53638=CARTESIAN_POINT('Ctrl Pts',(54.7362763496954,14.6310315157388,5.11621462074954));
#53639=CARTESIAN_POINT('Ctrl Pts',(54.5775040932279,15.3732433417349,5.15438602136928));
#53640=CARTESIAN_POINT('Ctrl Pts',(53.4338710221273,16.1984132586634,5.21872592544796));
#53641=CARTESIAN_POINT('Ctrl Pts',(51.8243426112988,15.5898341745865,5.29723143582474));
#53642=CARTESIAN_POINT('Ctrl Pts',(51.4441749154368,13.9116075960113,5.37573694620152));
#53643=CARTESIAN_POINT('Ctrl Pts',(52.6343093950298,12.6688279644592,5.45424245657829));
#53644=CARTESIAN_POINT('Ctrl Pts',(54.2767867908486,12.9668231409662,5.53040071570737));
#53645=CARTESIAN_POINT('Ctrl Pts',(54.7372886615245,13.9376228212707,5.58039047137751));
#53646=CARTESIAN_POINT('Ctrl Pts',(54.7400835567429,14.3978973414314,5.60421172358873));
#53647=CARTESIAN_POINT('Origin',(53.1951359564886,14.3971354987959,0.895788276411274));
#53648=CARTESIAN_POINT('',(54.7390536535266,14.3959278946887,4.60421172358873));
#53649=CARTESIAN_POINT('',(54.7379141108259,14.3984645193683,4.64578827641127));
#53650=CARTESIAN_POINT('',(54.7381359564886,14.3971354987959,0.895788276411274));
#53651=CARTESIAN_POINT('Ctrl Pts',(54.7379141108259,14.3984645193683,4.64578827641127));
#53652=CARTESIAN_POINT('Ctrl Pts',(54.7390192921529,14.5252809022368,4.65232762547243));
#53653=CARTESIAN_POINT('Ctrl Pts',(54.6671855077626,15.158343636416,4.68503547799252));
#53654=CARTESIAN_POINT('Ctrl Pts',(53.7972179286764,16.1115146859015,4.74391183397153));
#53655=CARTESIAN_POINT('Ctrl Pts',(52.0972451605188,15.8449731797319,4.82241734434831));
#53656=CARTESIAN_POINT('Ctrl Pts',(51.3818866828157,14.2799767547255,4.90092285472509));
#53657=CARTESIAN_POINT('Ctrl Pts',(52.2926938154427,12.820050407037,4.97942836510186));
#53658=CARTESIAN_POINT('Ctrl Pts',(54.0128314027411,12.7744928061304,5.05793387547865));
#53659=CARTESIAN_POINT('Ctrl Pts',(54.7098771965036,13.7702259631725,5.11338717924845));
#53660=CARTESIAN_POINT('Ctrl Pts',(54.7401994584832,14.3359395997999,5.14267197955932));
#53661=CARTESIAN_POINT('Ctrl Pts',(54.7397605362559,14.3961865506515,5.14578827641127));
#53662=CARTESIAN_POINT('Ctrl Pts',(54.7390536535266,14.3959278946887,4.60421172358873));
#53663=CARTESIAN_POINT('Ctrl Pts',(54.7354489362591,14.815149952008,4.62587026666265));
#53664=CARTESIAN_POINT('Ctrl Pts',(54.3438802932754,15.7468235466057,4.6736973131955));
#53665=CARTESIAN_POINT('Ctrl Pts',(52.7769304442279,16.1653842141838,4.74769286318728));
#53666=CARTESIAN_POINT('Ctrl Pts',(51.4895330907317,15.0236483351255,4.82619837356406));
#53667=CARTESIAN_POINT('Ctrl Pts',(51.7317609456535,13.3200407432483,4.90470388394085));
#53668=CARTESIAN_POINT('Ctrl Pts',(53.2863782799342,12.5823975487372,4.98320939431761));
#53669=CARTESIAN_POINT('Ctrl Pts',(54.5339890873504,13.3362017488983,5.04971200753359));
#53670=CARTESIAN_POINT('Ctrl Pts',(54.7352923713373,14.1218070799821,5.09004611729062));
#53671=CARTESIAN_POINT('Ctrl Pts',(54.7358250212096,14.397461852737,5.10421172358873));
#53672=CARTESIAN_POINT('Origin',(53.1951359564886,14.3971354987959,0.895788276411274));
#53673=CARTESIAN_POINT('',(54.7387010277811,14.3984147555176,4.10421172358872));
#53674=CARTESIAN_POINT('',(54.7363034079594,14.3962637958223,4.14578827641127));
#53675=CARTESIAN_POINT('',(54.7381359564886,14.3971354987959,0.895788276411274));
#53676=CARTESIAN_POINT('Ctrl Pts',(54.7363034079594,14.3962637958223,4.14578827641127));
#53677=CARTESIAN_POINT('Ctrl Pts',(54.7346448209044,14.7111635771051,4.16198327138554));
#53678=CARTESIAN_POINT('Ctrl Pts',(54.4887025372849,15.537270261699,4.20434676981873));
#53679=CARTESIAN_POINT('Ctrl Pts',(53.147408175106,16.2135387160798,4.27287877171085));
#53680=CARTESIAN_POINT('Ctrl Pts',(51.6537177503359,15.3592313846778,4.35138428208763));
#53681=CARTESIAN_POINT('Ctrl Pts',(51.5424078137269,13.6420935954197,4.42988979246441));
#53682=CARTESIAN_POINT('Ctrl Pts',(52.9133037754092,12.6020953249299,4.50839530284119));
#53683=CARTESIAN_POINT('Ctrl Pts',(54.4017068046157,13.124465562129,4.58036146415681));
#53684=CARTESIAN_POINT('Ctrl Pts',(54.7345966896724,14.0177999706171,4.62615912201351));
#53685=CARTESIAN_POINT('Ctrl Pts',(54.7379141108259,14.3984645193683,4.64578827641127));
#53686=CARTESIAN_POINT('Ctrl Pts',(54.7387010277811,14.3984147555176,4.10421172358872));
#53687=CARTESIAN_POINT('Ctrl Pts',(54.7395828579414,14.49807341117,4.10935740911683));
#53688=CARTESIAN_POINT('Ctrl Pts',(54.6857500758113,15.1036004690399,4.14067159810387));
#53689=CARTESIAN_POINT('Ctrl Pts',(53.8864190756817,16.077530414512,4.19815429054983));
#53690=CARTESIAN_POINT('Ctrl Pts',(52.1747941628695,15.9006321056092,4.2766598009266));
#53691=CARTESIAN_POINT('Ctrl Pts',(51.3782360277522,14.3753622969642,4.35516531130339));
#53692=CARTESIAN_POINT('Ctrl Pts',(52.2111169431944,12.8696192117062,4.43367082168016));
#53693=CARTESIAN_POINT('Ctrl Pts',(53.9264895031678,12.7337890506155,4.51217633205695));
#53694=CARTESIAN_POINT('Ctrl Pts',(54.6936722382488,13.7156146023329,4.5690232993598));
#53695=CARTESIAN_POINT('Ctrl Pts',(54.7398042641295,14.3086332477416,4.59970176320372));
#53696=CARTESIAN_POINT('Ctrl Pts',(54.7390536535266,14.3959278946887,4.60421172358873));
#53697=CARTESIAN_POINT('Origin',(53.1951359564886,14.3971354987959,0.895788276411274));
#53698=CARTESIAN_POINT('',(54.7359273488899,14.3966252672389,3.60421172358873));
#53699=CARTESIAN_POINT('',(54.740563122869,14.3970262782475,3.64578827641127));
#53700=CARTESIAN_POINT('',(54.7381359564886,14.3971354987959,0.895788276411274));
#53701=CARTESIAN_POINT('Ctrl Pts',(54.740563122869,14.3970262782475,3.64578827641127));
#53702=CARTESIAN_POINT('Ctrl Pts',(54.7400434078029,14.8961037383943,3.67163891729865));
#53703=CARTESIAN_POINT('Ctrl Pts',(54.208547388428,15.9013481621327,3.72365806164495));
#53704=CARTESIAN_POINT('Ctrl Pts',(52.5038529249194,16.0775302015138,3.80184570945018));
#53705=CARTESIAN_POINT('Ctrl Pts',(51.4121872860838,14.7474105690538,3.88035121982695));
#53706=CARTESIAN_POINT('Ctrl Pts',(51.9195124019995,13.1031559265556,3.95885673020373));
#53707=CARTESIAN_POINT('Ctrl Pts',(53.5708470479161,12.6193729267869,4.03736224058052));
#53708=CARTESIAN_POINT('Ctrl Pts',(54.6140883917719,13.5008315971724,4.09967275598302));
#53709=CARTESIAN_POINT('Ctrl Pts',(54.7373248304478,14.202336249353,4.13581476792661));
#53710=CARTESIAN_POINT('Ctrl Pts',(54.7363034079594,14.3962637958223,4.14578827641127));
#53711=CARTESIAN_POINT('Ctrl Pts',(54.7359273488899,14.3966252672389,3.60421172358873));
#53712=CARTESIAN_POINT('Ctrl Pts',(54.7350534494295,14.6846029003007,3.61901305502994));
#53713=CARTESIAN_POINT('Ctrl Pts',(54.5202760602344,15.482930589367,3.65998288993008));
#53714=CARTESIAN_POINT('Ctrl Pts',(53.2428637439183,16.2135389463141,3.72712122828915));
#53715=CARTESIAN_POINT('Ctrl Pts',(51.7063697132749,15.4388525891942,3.80562673866593));
#53716=CARTESIAN_POINT('Ctrl Pts',(51.5050366439836,13.7299295812751,3.88413224904271));
#53717=CARTESIAN_POINT('Ctrl Pts',(52.8194248174382,12.6193727014466,3.96263775941949));
#53718=CARTESIAN_POINT('Ctrl Pts',(54.3625220492744,13.0714459438974,4.03599758426816));
#53719=CARTESIAN_POINT('Ctrl Pts',(54.7350982901468,13.9912569994582,4.0831889056579));
#53720=CARTESIAN_POINT('Ctrl Pts',(54.7387010277811,14.3984147555176,4.10421172358872));
#53721=CARTESIAN_POINT('Origin',(53.1951359564886,14.3971354987959,0.895788276411274));
#53722=CARTESIAN_POINT('',(54.740301190334,14.3965688164982,3.10421172358873));
#53723=CARTESIAN_POINT('',(54.7365381831935,14.3981451127971,3.14578827641127));
#53724=CARTESIAN_POINT('',(54.7381359564886,14.3971354987959,0.895788276411274));
#53725=CARTESIAN_POINT('Ctrl Pts',(54.7365381831935,14.3981451127971,3.14578827641127));
#53726=CARTESIAN_POINT('Ctrl Pts',(54.7376569241507,14.5796417971643,3.15512605975283));
#53727=CARTESIAN_POINT('Ctrl Pts',(54.6247347728585,15.2684238709215,3.19063234655331));
#53728=CARTESIAN_POINT('Ctrl Pts',(53.6133414157458,16.1653839899769,3.25230713681272));
#53729=CARTESIAN_POINT('Ctrl Pts',(51.9508876322963,15.7213124929433,3.3308126471895));
#53730=CARTESIAN_POINT('Ctrl Pts',(51.4043053238161,14.0896875604189,3.40931815756628));
#53731=CARTESIAN_POINT('Ctrl Pts',(52.4637825025118,12.7337892614639,3.48782366794306));
#53732=CARTESIAN_POINT('Ctrl Pts',(54.1791548450535,12.8696194053218,3.56632917831983));
#53733=CARTESIAN_POINT('Ctrl Pts',(54.737780986498,13.8795446348882,3.61898404780924));
#53734=CARTESIAN_POINT('Ctrl Pts',(54.7405695133476,14.3908895621182,3.64547041383972));
#53735=CARTESIAN_POINT('Ctrl Pts',(54.740563122869,14.3970262782475,3.64578827641127));
#53736=CARTESIAN_POINT('Ctrl Pts',(54.740301190334,14.3965688164982,3.10421172358873));
#53737=CARTESIAN_POINT('Ctrl Pts',(54.7380390595611,14.8689546274245,3.12866870094305));
#53738=CARTESIAN_POINT('Ctrl Pts',(54.2559651859222,15.850784329065,3.17929418175629));
#53739=CARTESIAN_POINT('Ctrl Pts',(52.5930539078611,16.1115149029784,3.25608816602847));
#53740=CARTESIAN_POINT('Ctrl Pts',(51.4330422815012,14.8405600699842,3.33459367640525));
#53741=CARTESIAN_POINT('Ctrl Pts',(51.8533182226522,13.1719316222439,3.41309918678203));
#53742=CARTESIAN_POINT('Ctrl Pts',(53.4769681733105,12.6020950974316,3.49160469715881));
#53743=CARTESIAN_POINT('Ctrl Pts',(54.5893972536881,13.4460134923652,3.55530887609438));
#53744=CARTESIAN_POINT('Ctrl Pts',(54.7365984888838,14.175463319392,3.59284455157101));
#53745=CARTESIAN_POINT('Ctrl Pts',(54.7359273488899,14.3966252672389,3.60421172358873));
#53746=CARTESIAN_POINT('Origin',(53.1951359564886,14.3971354987959,0.895788276411274));
#53747=CARTESIAN_POINT('',(54.73716587472,14.3983674417199,2.60421172358873));
#53748=CARTESIAN_POINT('',(54.7375657625992,14.3958310564158,2.64578827641127));
#53749=CARTESIAN_POINT('',(54.7381359564886,14.3971354987959,0.895788276411274));
#53750=CARTESIAN_POINT('Ctrl Pts',(54.7375657625992,14.3958310564158,2.64578827641127));
#53751=CARTESIAN_POINT('Ctrl Pts',(54.734479142859,14.7643796819994,2.66478170566593));
#53752=CARTESIAN_POINT('Ctrl Pts',(54.4188250031304,15.6454555959149,2.70994363837952));
#53753=CARTESIAN_POINT('Ctrl Pts',(52.9564009216582,16.198413027115,2.78127407455204));
#53754=CARTESIAN_POINT('Ctrl Pts',(51.5609762954032,15.1915669978344,2.85977958492882));
#53755=CARTESIAN_POINT('Ctrl Pts',(51.6311047416152,13.472254177388,2.9382850953056));
#53756=CARTESIAN_POINT('Ctrl Pts',(53.1038936445493,12.5823977792548,3.01679060568238));
#53757=CARTESIAN_POINT('Ctrl Pts',(54.4735979274945,13.2323024338895,3.0859583327176));
#53758=CARTESIAN_POINT('Ctrl Pts',(54.7345217286191,14.0710096690757,3.1289575562939));
#53759=CARTESIAN_POINT('Ctrl Pts',(54.7365381831935,14.3981451127971,3.14578827641127));
#53760=CARTESIAN_POINT('Ctrl Pts',(54.73716587472,14.3983674417199,2.60421172358873));
#53761=CARTESIAN_POINT('Ctrl Pts',(54.7383644283813,14.5526183883782,2.61215584339723));
#53762=CARTESIAN_POINT('Ctrl Pts',(54.6467666252149,15.2135939671077,2.64626846666466));
#53763=CARTESIAN_POINT('Ctrl Pts',(53.7056202382209,16.1409758479641,2.70654959339102));
#53764=CARTESIAN_POINT('Ctrl Pts',(52.0221470001078,15.7848310056966,2.78505510376779));
#53765=CARTESIAN_POINT('Ctrl Pts',(51.3906291820654,14.1841570315506,2.86356061414457));
#53766=CARTESIAN_POINT('Ctrl Pts',(52.3774404052229,12.7744925974775,2.94206612452135));
#53767=CARTESIAN_POINT('Ctrl Pts',(54.0975782126823,12.8200502087089,3.02057163489813));
#53768=CARTESIAN_POINT('Ctrl Pts',(54.7246398714755,13.8251629314517,3.07462016792059));
#53769=CARTESIAN_POINT('Ctrl Pts',(54.7404594967271,14.3635107392415,3.10250019748412));
#53770=CARTESIAN_POINT('Ctrl Pts',(54.740301190334,14.3965688164982,3.10421172358873));
#53771=CARTESIAN_POINT('Origin',(53.1951359564886,14.3971354987959,0.895788276411274));
#53772=CARTESIAN_POINT('',(54.7364807484814,14.3955730757723,2.10421172358873));
#53773=CARTESIAN_POINT('',(54.7400287307462,14.397884086359,2.14578827641127));
#53774=CARTESIAN_POINT('',(54.7381359564886,14.3971354987959,0.895788276411274));
#53775=CARTESIAN_POINT('',(53.5936497983459,12.9064860705774,2.));
#53776=CARTESIAN_POINT('Ctrl Pts',(53.5936497983459,12.9064860705774,2.));
#53777=CARTESIAN_POINT('Ctrl Pts',(54.083839596546,13.0375346028627,2.02616850345893));
#53778=CARTESIAN_POINT('Ctrl Pts',(54.6367230898564,13.5559776050111,2.06090574465517));
#53779=CARTESIAN_POINT('Ctrl Pts',(54.737618997593,14.2290968579424,2.09564298585141));
#53780=CARTESIAN_POINT('Ctrl Pts',(54.7364807484814,14.3955730757723,2.10421172358873));
#53781=CARTESIAN_POINT('',(52.7955982877704,12.9041242545674,2.));
#53782=CARTESIAN_POINT('Origin',(53.1951359564886,14.3971354987959,2.));
#53783=CARTESIAN_POINT('Ctrl Pts',(52.7955926848293,12.9041113294173,2.));
#53784=CARTESIAN_POINT('Ctrl Pts',(53.2607241041145,12.7814202621555,2.02490816038701));
#53785=CARTESIAN_POINT('Ctrl Pts',(54.2926583006945,12.9966875828164,2.0735042525241));
#53786=CARTESIAN_POINT('Ctrl Pts',(54.7371492824905,13.9402272601641,2.12210034466119));
#53787=CARTESIAN_POINT('Ctrl Pts',(54.7400287307462,14.397884086359,2.14578827641127));
#53788=CARTESIAN_POINT('Origin',(14.1292828945603,53.2669068454841,15.5));
#53789=CARTESIAN_POINT('',(13.4980577522811,52.1734972976428,14.1934196736194));
#53790=CARTESIAN_POINT('',(13.4988747128346,52.1716629874611,14.0565803263806));
#53791=CARTESIAN_POINT('',(13.4970328945603,52.1718177223987,15.5));
#53792=CARTESIAN_POINT('',(12.9355708698302,52.8497595669186,14.));
#53793=CARTESIAN_POINT('Ctrl Pts',(13.4988747128346,52.1716629874611,14.0565803263806));
#53794=CARTESIAN_POINT('Ctrl Pts',(13.2411227471438,52.3234873105789,14.0377202175871));
#53795=CARTESIAN_POINT('Ctrl Pts',(13.0344360750677,52.5668460963447,14.0188601087935));
#53796=CARTESIAN_POINT('Ctrl Pts',(12.9355708698302,52.8497595669186,14.));
#53797=CARTESIAN_POINT('',(13.4970328945603,52.1718177223987,14.));
#53798=CARTESIAN_POINT('Origin',(14.1292828945603,53.2669068454841,14.));
#53799=CARTESIAN_POINT('',(13.4970328945603,52.1718177223987,13.));
#53800=CARTESIAN_POINT('',(13.4970328945603,52.1718177223987,15.5));
#53801=CARTESIAN_POINT('',(12.8669333849943,53.3406222827979,13.));
#53802=CARTESIAN_POINT('Origin',(14.1292828945603,53.2669068454841,13.));
#53803=CARTESIAN_POINT('',(15.3916324041264,53.1931914081703,13.));
#53804=CARTESIAN_POINT('Origin',(14.1292828945603,53.2669068454841,13.));
#53805=CARTESIAN_POINT('Origin',(14.1292828945603,53.2669068454841,13.));
#53806=CARTESIAN_POINT('',(13.8936073831512,54.5113748561459,14.));
#53807=CARTESIAN_POINT('Origin',(14.1292828945603,53.2669068454841,14.));
#53808=CARTESIAN_POINT('Ctrl Pts',(13.893606936201,54.511386694654,14.));
#53809=CARTESIAN_POINT('Ctrl Pts',(13.5065438623108,54.43664727626,14.024908160387));
#53810=CARTESIAN_POINT('Ctrl Pts',(13.1551923299505,54.1671690811723,14.049816320774));
#53811=CARTESIAN_POINT('Ctrl Pts',(12.9858145310893,53.8112673891924,14.074724481161));
#53812=CARTESIAN_POINT('Ctrl Pts',(12.8078662825437,53.43735721225,14.10089298462));
#53813=CARTESIAN_POINT('Ctrl Pts',(12.8307732764863,52.9680562770306,14.1270614880789));
#53814=CARTESIAN_POINT('Ctrl Pts',(13.0443854893126,52.6134561814805,14.1532299915378));
#53815=CARTESIAN_POINT('Ctrl Pts',(13.1537409585151,52.4319241458582,14.1666265522317));
#53816=CARTESIAN_POINT('Ctrl Pts',(13.3130758736166,52.2804525587352,14.1800231129255));
#53817=CARTESIAN_POINT('Ctrl Pts',(13.4980577522811,52.1734972976428,14.1934196736194));
#53818=CARTESIAN_POINT('Origin',(14.1292828945603,53.2669068454841,15.5));
#53819=CARTESIAN_POINT('',(13.4970386657413,52.17027240687,14.6934196736194));
#53820=CARTESIAN_POINT('',(13.4956926805926,52.1707443397673,14.5565803263806));
#53821=CARTESIAN_POINT('',(13.4970328945603,52.1718177223987,15.5));
#53822=CARTESIAN_POINT('Ctrl Pts',(13.4956926805926,52.1707443397673,14.5565803263806));
#53823=CARTESIAN_POINT('Ctrl Pts',(13.4633916214762,52.1891327536446,14.5542330751329));
#53824=CARTESIAN_POINT('Ctrl Pts',(13.4319685470764,52.2090047577526,14.5518858238852));
#53825=CARTESIAN_POINT('Ctrl Pts',(13.4015745144389,52.230342308046,14.5495385726374));
#53826=CARTESIAN_POINT('Ctrl Pts',(13.0627244024285,52.4682255594459,14.5233700691785));
#53827=CARTESIAN_POINT('Ctrl Pts',(12.8517746061391,52.8882625646258,14.4972015657196));
#53828=CARTESIAN_POINT('Ctrl Pts',(12.8632814695834,53.3021304033103,14.4710330622607));
#53829=CARTESIAN_POINT('Ctrl Pts',(12.8747883330277,53.7159982419948,14.4448645588017));
#53830=CARTESIAN_POINT('Ctrl Pts',(13.1087518562058,54.1236969141838,14.4186960553428));
#53831=CARTESIAN_POINT('Ctrl Pts',(13.460332770227,54.3423556782116,14.3925275518839));
#53832=CARTESIAN_POINT('Ctrl Pts',(13.8119136842482,54.5610144422395,14.366359048425));
#53833=CARTESIAN_POINT('Ctrl Pts',(14.2811119891126,54.5906332981061,14.340190544966));
#53834=CARTESIAN_POINT('Ctrl Pts',(14.6573867068861,54.4180393977443,14.3140220415071));
#53835=CARTESIAN_POINT('Ctrl Pts',(15.0336614246596,54.2454454973824,14.2878535380482));
#53836=CARTESIAN_POINT('Ctrl Pts',(15.3170125553422,53.8706388407919,14.2616850345893));
#53837=CARTESIAN_POINT('Ctrl Pts',(15.3806795111647,53.461467903109,14.2355165311303));
#53838=CARTESIAN_POINT('Ctrl Pts',(15.4443464669872,53.052296965426,14.2093480276714));
#53839=CARTESIAN_POINT('Ctrl Pts',(15.2883292479495,52.6087617466505,14.1831795242125));
#53840=CARTESIAN_POINT('Ctrl Pts',(14.981976715725,52.3301941698058,14.1570110207536));
#53841=CARTESIAN_POINT('Ctrl Pts',(14.6756241835006,52.0516265929611,14.1308425172946));
#53842=CARTESIAN_POINT('Ctrl Pts',(14.2189363380893,51.938026658047,14.1046740138357));
#53843=CARTESIAN_POINT('Ctrl Pts',(13.8182170120758,52.0394239070104,14.0785055103768));
#53844=CARTESIAN_POINT('Ctrl Pts',(13.7063032761926,52.067742343889,14.0711971157114));
#53845=CARTESIAN_POINT('Ctrl Pts',(13.5987550004656,52.1128302370619,14.063888721046));
#53846=CARTESIAN_POINT('Ctrl Pts',(13.4988747128346,52.1716629874611,14.0565803263806));
#53847=CARTESIAN_POINT('Ctrl Pts',(13.4980577522811,52.1734972976428,14.1934196736194));
#53848=CARTESIAN_POINT('Ctrl Pts',(13.6744148054729,52.0715288518372,14.2061916163845));
#53849=CARTESIAN_POINT('Ctrl Pts',(13.8740829845723,52.0100223374604,14.2189635591495));
#53850=CARTESIAN_POINT('Ctrl Pts',(14.0759771073047,52.00150441778,14.2317355019146));
#53851=CARTESIAN_POINT('Ctrl Pts',(14.4896390807605,51.9840520055104,14.2579040053735));
#53852=CARTESIAN_POINT('Ctrl Pts',(14.9126455959621,52.1890464368519,14.2840725088324));
#53853=CARTESIAN_POINT('Ctrl Pts',(15.1553451745864,52.5244804183786,14.3102410122914));
#53854=CARTESIAN_POINT('Ctrl Pts',(15.3980447532108,52.8599143999052,14.3364095157503));
#53855=CARTESIAN_POINT('Ctrl Pts',(15.460437395258,53.325787931617,14.3625780192092));
#53856=CARTESIAN_POINT('Ctrl Pts',(15.3145307999442,53.7132400695012,14.3887465226681));
#53857=CARTESIAN_POINT('Ctrl Pts',(15.1686242046305,54.1006922073853,14.4149150261271));
#53858=CARTESIAN_POINT('Ctrl Pts',(14.8144183719558,54.409722951442,14.441083529586));
#53859=CARTESIAN_POINT('Ctrl Pts',(14.4107506896371,54.5017382932332,14.4672520330449));
#53860=CARTESIAN_POINT('Ctrl Pts',(14.0070830073184,54.5937536350245,14.4934205365039));
#53861=CARTESIAN_POINT('Ctrl Pts',(13.5539534753558,54.4687535745504,14.5195890399628));
#53862=CARTESIAN_POINT('Ctrl Pts',(13.2545471544402,54.1828000037796,14.5457575434217));
#53863=CARTESIAN_POINT('Ctrl Pts',(12.9551408335246,53.8968464330087,14.5719260468806));
#53864=CARTESIAN_POINT('Ctrl Pts',(12.8094577236562,53.4499393519412,14.5980945503396));
#53865=CARTESIAN_POINT('Ctrl Pts',(12.8828256503828,53.0424720659447,14.6242630537985));
#53866=CARTESIAN_POINT('Ctrl Pts',(12.9474564997503,52.6835283427349,14.6473152604055));
#53867=CARTESIAN_POINT('Ctrl Pts',(13.1820731109759,52.3551902889475,14.6703674670124));
#53868=CARTESIAN_POINT('Ctrl Pts',(13.4970386657413,52.17027240687,14.6934196736194));
#53869=CARTESIAN_POINT('Origin',(14.1292828945603,53.2669068454841,15.5));
#53870=CARTESIAN_POINT('',(13.4961785456119,52.1725162395268,15.1934196736194));
#53871=CARTESIAN_POINT('',(13.4977463410385,52.1735883352515,15.0565803263806));
#53872=CARTESIAN_POINT('',(13.4970328945603,52.1718177223987,15.5));
#53873=CARTESIAN_POINT('Ctrl Pts',(13.4977463410385,52.1735883352515,15.0565803263806));
#53874=CARTESIAN_POINT('Ctrl Pts',(13.3317931989842,52.2689743399829,15.0445774292198));
#53875=CARTESIAN_POINT('Ctrl Pts',(13.186612163033,52.4000385957214,15.0325745320589));
#53876=CARTESIAN_POINT('Ctrl Pts',(13.0802179156269,52.5573375001258,15.0205716348981));
#53877=CARTESIAN_POINT('Ctrl Pts',(12.8482590648635,52.9002777810297,14.9944031314392));
#53878=CARTESIAN_POINT('Ctrl Pts',(12.800661371336,53.3679164545856,14.9682346279803));
#53879=CARTESIAN_POINT('Ctrl Pts',(12.9587676726968,53.7505591757409,14.9420661245213));
#53880=CARTESIAN_POINT('Ctrl Pts',(13.1168739740577,54.1332018968962,14.9158976210624));
#53881=CARTESIAN_POINT('Ctrl Pts',(13.4806842703069,54.4308486656509,14.8897291176035));
#53882=CARTESIAN_POINT('Ctrl Pts',(13.887062777462,54.5100303359217,14.8635606141446));
#53883=CARTESIAN_POINT('Ctrl Pts',(14.2934412846171,54.5892120061924,14.8373921106856));
#53884=CARTESIAN_POINT('Ctrl Pts',(14.7423880026779,54.4499285779793,14.8112236072267));
#53885=CARTESIAN_POINT('Ctrl Pts',(15.0325877125755,54.1546380042325,14.7850551037678));
#53886=CARTESIAN_POINT('Ctrl Pts',(15.322787422473,53.8593474304858,14.7588866003089));
#53887=CARTESIAN_POINT('Ctrl Pts',(15.4542401242071,53.4080497112055,14.7327180968499));
#53888=CARTESIAN_POINT('Ctrl Pts',(15.3680052510694,53.0031088631455,14.706549593391));
#53889=CARTESIAN_POINT('Ctrl Pts',(15.2817703779317,52.5981680150856,14.6803810899321));
#53890=CARTESIAN_POINT('Ctrl Pts',(14.9778479299221,52.239584038246,14.6542125864732));
#53891=CARTESIAN_POINT('Ctrl Pts',(14.5925114920515,52.0881567986362,14.6280440830142));
#53892=CARTESIAN_POINT('Ctrl Pts',(14.2417387974228,51.9503122148961,14.604222830803));
#53893=CARTESIAN_POINT('Ctrl Pts',(13.8235023586795,51.9841281668449,14.5804015785918));
#53894=CARTESIAN_POINT('Ctrl Pts',(13.4956926805926,52.1707443397673,14.5565803263806));
#53895=CARTESIAN_POINT('Ctrl Pts',(13.4970386657413,52.17027240687,14.6934196736194));
#53896=CARTESIAN_POINT('Ctrl Pts',(13.5396170697753,52.1452744089077,14.6965359704714));
#53897=CARTESIAN_POINT('Ctrl Pts',(13.5836638346913,52.1228973859148,14.6996522673233));
#53898=CARTESIAN_POINT('Ctrl Pts',(13.6289575157408,52.1034200423295,14.7027685641753));
#53899=CARTESIAN_POINT('Ctrl Pts',(14.0093024910506,51.9398627956362,14.7289370676342));
#53900=CARTESIAN_POINT('Ctrl Pts',(14.4775734783483,51.9807757931753,14.7551055710931));
#53901=CARTESIAN_POINT('Ctrl Pts',(14.823792639393,52.2078118983851,14.781274074552));
#53902=CARTESIAN_POINT('Ctrl Pts',(15.1700118004377,52.434848003595,14.807442578011));
#53903=CARTESIAN_POINT('Ctrl Pts',(15.3941791352292,52.8480072164757,14.8336110814699));
#53904=CARTESIAN_POINT('Ctrl Pts',(15.3957751288567,53.2620246601267,14.8597795849288));
#53905=CARTESIAN_POINT('Ctrl Pts',(15.3973711224841,53.6760421037777,14.8859480883878));
#53906=CARTESIAN_POINT('Ctrl Pts',(15.1763957749473,54.0909177781991,14.9121165918467));
#53907=CARTESIAN_POINT('Ctrl Pts',(14.83193716646,54.3206161896323,14.9382850953056));
#53908=CARTESIAN_POINT('Ctrl Pts',(14.4874785579727,54.5503146010655,14.9644535987645));
#53909=CARTESIAN_POINT('Ctrl Pts',(14.0195366885348,54.5948357495104,14.9906221022235));
#53910=CARTESIAN_POINT('Ctrl Pts',(13.6379422013928,54.4342159762724,15.0167906056824));
#53911=CARTESIAN_POINT('Ctrl Pts',(13.2563477142507,54.2735962030343,15.0429591091413));
#53912=CARTESIAN_POINT('Ctrl Pts',(12.9611006094046,53.9078355081131,15.0691276126002));
#53913=CARTESIAN_POINT('Ctrl Pts',(12.8845932246477,53.5009452588027,15.0952961160592));
#53914=CARTESIAN_POINT('Ctrl Pts',(12.8080858398908,53.0940550094922,15.1214646195181));
#53915=CARTESIAN_POINT('Ctrl Pts',(12.9503181752231,52.6460352057925,15.147633122977));
#53916=CARTESIAN_POINT('Ctrl Pts',(13.2475115476967,52.3577832908858,15.1738016264359));
#53917=CARTESIAN_POINT('Ctrl Pts',(13.3217783549033,52.2857508992711,15.1803409754971));
#53918=CARTESIAN_POINT('Ctrl Pts',(13.4057220070296,52.2236955258253,15.1868803245583));
#53919=CARTESIAN_POINT('Ctrl Pts',(13.4961785456119,52.1725162395268,15.1934196736194));
#53920=CARTESIAN_POINT('Origin',(14.1292828945603,53.2669068454841,15.5));
#53921=CARTESIAN_POINT('',(13.4984004295476,52.1727576237481,15.6934196736194));
#53922=CARTESIAN_POINT('',(13.4975120618698,52.1706683776322,15.5565803263806));
#53923=CARTESIAN_POINT('',(13.4970328945603,52.1718177223987,15.5));
#53924=CARTESIAN_POINT('Ctrl Pts',(13.4975120618698,52.1706683776322,15.5565803263806));
#53925=CARTESIAN_POINT('Ctrl Pts',(13.2014603606288,52.3450050094651,15.5349217833067));
#53926=CARTESIAN_POINT('Ctrl Pts',(12.9746829017777,52.6437331734245,15.5132632402327));
#53927=CARTESIAN_POINT('Ctrl Pts',(12.8963324343973,52.9773225319626,15.4916046971588));
#53928=CARTESIAN_POINT('Ctrl Pts',(12.8016670421014,53.3803752328285,15.4654361936999));
#53929=CARTESIAN_POINT('Ctrl Pts',(12.9236783333193,53.8343190010791,15.439267690241));
#53930=CARTESIAN_POINT('Ctrl Pts',(13.2076549868354,54.1356000609316,15.413099186782));
#53931=CARTESIAN_POINT('Ctrl Pts',(13.4916316403516,54.4368811207841,15.3869306833231));
#53932=CARTESIAN_POINT('Ctrl Pts',(13.9375736561661,54.5854994722384,15.3607621798642));
#53933=CARTESIAN_POINT('Ctrl Pts',(14.3455153495113,54.5148128681013,15.3345936764052));
#53934=CARTESIAN_POINT('Ctrl Pts',(14.7534570428566,54.4441262639641,15.3084251729463));
#53935=CARTESIAN_POINT('Ctrl Pts',(15.1233984137326,54.1541347042354,15.2822566694874));
#53936=CARTESIAN_POINT('Ctrl Pts',(15.2894533218141,53.7748738751902,15.2560881660285));
#53937=CARTESIAN_POINT('Ctrl Pts',(15.4555082298957,53.3956130461449,15.2299196625695));
#53938=CARTESIAN_POINT('Ctrl Pts',(15.4176766751828,52.9270829477831,15.2037511591106));
#53939=CARTESIAN_POINT('Ctrl Pts',(15.1929228414795,52.579377997485,15.1775826556517));
#53940=CARTESIAN_POINT('Ctrl Pts',(14.9681690077762,52.2316730471868,15.1514141521927));
#53941=CARTESIAN_POINT('Ctrl Pts',(14.5564928950826,52.0047932449523,15.1252456487338));
#53942=CARTESIAN_POINT('Ctrl Pts',(14.1424948347361,52.0004742879611,15.0990771452749));
#53943=CARTESIAN_POINT('Ctrl Pts',(13.9183882655449,51.9981363382785,15.0849115389768));
#53944=CARTESIAN_POINT('Ctrl Pts',(13.6936012952866,52.0610154646128,15.0707459326787));
#53945=CARTESIAN_POINT('Ctrl Pts',(13.4977463410385,52.1735883352515,15.0565803263806));
#53946=CARTESIAN_POINT('Ctrl Pts',(13.4961785456119,52.1725162395268,15.1934196736194));
#53947=CARTESIAN_POINT('Ctrl Pts',(13.7677018035866,52.018891451597,15.2130488280172));
#53948=CARTESIAN_POINT('Ctrl Pts',(14.0979074320564,51.9632623188715,15.2326779824149));
#53949=CARTESIAN_POINT('Ctrl Pts',(14.4012233710795,52.0299449584561,15.2523071368127));
#53950=CARTESIAN_POINT('Ctrl Pts',(14.8055874123741,52.1188425670469,15.2784756402716));
#53951=CARTESIAN_POINT('Ctrl Pts',(15.1621610853483,52.4251218103423,15.3046441437306));
#53952=CARTESIAN_POINT('Ctrl Pts',(15.3110525132995,52.8114434442094,15.3308126471895));
#53953=CARTESIAN_POINT('Ctrl Pts',(15.4599439412506,53.1977650780765,15.3569811506484));
#53954=CARTESIAN_POINT('Ctrl Pts',(15.4011531241786,53.6641291025153,15.3831496541074));
#53955=CARTESIAN_POINT('Ctrl Pts',(15.161042564887,54.0014123408011,15.4093181575663));
#53956=CARTESIAN_POINT('Ctrl Pts',(14.9209320055955,54.338695579087,15.4354866610252));
#53957=CARTESIAN_POINT('Ctrl Pts',(14.4995017040844,54.5468980312199,15.4616551644841));
#53958=CARTESIAN_POINT('Ctrl Pts',(14.0857260162278,54.5326592450683,15.4878236679431));
#53959=CARTESIAN_POINT('Ctrl Pts',(13.6719503283713,54.5184204589168,15.513992171402));
#53960=CARTESIAN_POINT('Ctrl Pts',(13.2658292541693,54.2817404344808,15.5401606748609));
#53961=CARTESIAN_POINT('Ctrl Pts',(13.0494723111738,53.9287493069653,15.5663291783198));
#53962=CARTESIAN_POINT('Ctrl Pts',(12.8331153681783,53.5757581794499,15.5924976817788));
#53963=CARTESIAN_POINT('Ctrl Pts',(12.8065225563893,53.1064559488549,15.6186661852377));
#53964=CARTESIAN_POINT('Ctrl Pts',(12.9816184085214,52.7312833144481,15.6448346886966));
#53965=CARTESIAN_POINT('Ctrl Pts',(13.0899806023986,52.4990988894489,15.6610296836709));
#53966=CARTESIAN_POINT('Ctrl Pts',(13.2755904595332,52.3029665221486,15.6772246786452));
#53967=CARTESIAN_POINT('Ctrl Pts',(13.4984004295476,52.1727576237481,15.6934196736194));
#53968=CARTESIAN_POINT('Origin',(14.1292828945603,53.2669068454841,15.5));
#53969=CARTESIAN_POINT('',(13.4961138435273,52.1700468646075,16.1934196736194));
#53970=CARTESIAN_POINT('',(13.4958915862187,52.1719376453661,16.0565803263806));
#53971=CARTESIAN_POINT('',(13.4970328945603,52.1718177223987,15.5));
#53972=CARTESIAN_POINT('Ctrl Pts',(13.4958915862187,52.1719376453661,16.0565803263806));
#53973=CARTESIAN_POINT('Ctrl Pts',(13.424800873756,52.2121474216226,16.0514346408525));
#53974=CARTESIAN_POINT('Ctrl Pts',(13.3578067644457,52.2591973943854,16.0462889553244));
#53975=CARTESIAN_POINT('Ctrl Pts',(13.2964716828247,52.3127310779992,16.0411432697963));
#53976=CARTESIAN_POINT('Ctrl Pts',(12.9845506983831,52.5849778713888,16.0149747663373));
#53977=CARTESIAN_POINT('Ctrl Pts',(12.8189865827469,53.0249099405019,15.9888062628784));
#53978=CARTESIAN_POINT('Ctrl Pts',(12.8740202534737,53.4352565161154,15.9626377594195));
#53979=CARTESIAN_POINT('Ctrl Pts',(12.9290539242004,53.8456030917289,15.9364692559605));
#53980=CARTESIAN_POINT('Ctrl Pts',(13.20468538129,54.2263641738429,15.9103007525016));
#53981=CARTESIAN_POINT('Ctrl Pts',(13.5773182028765,54.4068019672842,15.8841322490427));
#53982=CARTESIAN_POINT('Ctrl Pts',(13.9499510244629,54.5872397607254,15.8579637455838));
#53983=CARTESIAN_POINT('Ctrl Pts',(14.4195852105461,54.5673542654938,15.8317952421248));
#53984=CARTESIAN_POINT('Ctrl Pts',(14.7756312098701,54.3560623738526,15.8056267386659));
#53985=CARTESIAN_POINT('Ctrl Pts',(15.1316772091941,54.1447704822114,15.779458235207));
#53986=CARTESIAN_POINT('Ctrl Pts',(15.3741350217589,53.7420721941606,15.7532897317481));
#53987=CARTESIAN_POINT('Ctrl Pts',(15.3942836818793,53.3285422092164,15.7271212282891));
#53988=CARTESIAN_POINT('Ctrl Pts',(15.4144323419997,52.9150122242722,15.7009527248302));
#53989=CARTESIAN_POINT('Ctrl Pts',(15.2122718496755,52.4906505424345,15.6747842213713));
#53990=CARTESIAN_POINT('Ctrl Pts',(14.8784533736736,52.2457459854386,15.6486157179124));
#53991=CARTESIAN_POINT('Ctrl Pts',(14.5446348976717,52.0008414284427,15.6224472144534));
#53992=CARTESIAN_POINT('Ctrl Pts',(14.0791584379921,51.9353939962885,15.5962787109945));
#53993=CARTESIAN_POINT('Ctrl Pts',(13.6907491702475,52.078751096952,15.5701102075356));
#53994=CARTESIAN_POINT('Ctrl Pts',(13.6238095222296,52.1034577006719,15.5656002471506));
#53995=CARTESIAN_POINT('Ctrl Pts',(13.5591589344204,52.1343662450031,15.5610902867656));
#53996=CARTESIAN_POINT('Ctrl Pts',(13.4975120618698,52.1706683776322,15.5565803263806));
#53997=CARTESIAN_POINT('Ctrl Pts',(13.4984004295476,52.1727576237481,15.6934196736194));
#53998=CARTESIAN_POINT('Ctrl Pts',(13.6356154845652,52.0925699142095,15.7033931821041));
#53999=CARTESIAN_POINT('Ctrl Pts',(13.7869389649625,52.0373841810022,15.7133666905887));
#54000=CARTESIAN_POINT('Ctrl Pts',(13.9430173010127,52.0141772385597,15.7233401990734));
#54001=CARTESIAN_POINT('Ctrl Pts',(14.352535825319,51.9532868352966,15.7495087025323));
#54002=CARTESIAN_POINT('Ctrl Pts',(14.7947883578784,52.1125490669891,15.7756772059912));
#54003=CARTESIAN_POINT('Ctrl Pts',(15.0714636060597,52.4205488559651,15.8018457094502));
#54004=CARTESIAN_POINT('Ctrl Pts',(15.3481388542411,52.728548644941,15.8280142129091));
#54005=CARTESIAN_POINT('Ctrl Pts',(15.4592368180444,53.1852859912004,15.854182716368));
#54006=CARTESIAN_POINT('Ctrl Pts',(15.3549398499385,53.5859544394514,15.880351219827));
#54007=CARTESIAN_POINT('Ctrl Pts',(15.2506428818326,53.9866228877023,15.9065197232859));
#54008=CARTESIAN_POINT('Ctrl Pts',(14.9309509818175,54.3312224379448,15.9326882267448));
#54009=CARTESIAN_POINT('Ctrl Pts',(14.5392177979356,54.4652305557052,15.9588567302037));
#54010=CARTESIAN_POINT('Ctrl Pts',(14.1474846140537,54.5992386734655,15.9850252336627));
#54011=CARTESIAN_POINT('Ctrl Pts',(13.6837101463051,54.5226553587437,16.0111937371216));
#54012=CARTESIAN_POINT('Ctrl Pts',(13.3558563789031,54.2698214801479,16.0373622405805));
#54013=CARTESIAN_POINT('Ctrl Pts',(13.0280026115012,54.016987601552,16.0635307440394));
#54014=CARTESIAN_POINT('Ctrl Pts',(12.836069544446,53.5879031590821,16.0896992474984));
#54015=CARTESIAN_POINT('Ctrl Pts',(12.8661222463432,53.174974717257,16.1158677509573));
#54016=CARTESIAN_POINT('Ctrl Pts',(12.8958099052365,52.7670620187505,16.1417183918447));
#54017=CARTESIAN_POINT('Ctrl Pts',(13.1421232693052,52.3749152184319,16.167569032732));
#54018=CARTESIAN_POINT('Ctrl Pts',(13.4961138435273,52.1700468646075,16.1934196736194));
#54019=CARTESIAN_POINT('Origin',(14.1292828945603,53.2669068454841,15.5));
#54020=CARTESIAN_POINT('',(13.4969690270882,52.1733618792496,16.6934196736194));
#54021=CARTESIAN_POINT('',(13.4982981440081,52.173172919003,16.5565803263806));
#54022=CARTESIAN_POINT('',(13.4970328945603,52.1718177223987,15.5));
#54023=CARTESIAN_POINT('Ctrl Pts',(13.4982981440081,52.173172919003,16.5565803263806));
#54024=CARTESIAN_POINT('Ctrl Pts',(13.2942737914494,52.291793394842,16.5417789949394));
#54025=CARTESIAN_POINT('Ctrl Pts',(13.121375289642,52.4650421903572,16.5269776634981));
#54026=CARTESIAN_POINT('Ctrl Pts',(13.0113308722452,52.6717520885803,16.5121763320569));
#54027=CARTESIAN_POINT('Ctrl Pts',(12.8167742049128,53.0372116898416,16.486007828598));
#54028=CARTESIAN_POINT('Ctrl Pts',(12.8186845812821,53.5072628063503,16.4598393251391));
#54029=CARTESIAN_POINT('Ctrl Pts',(13.0162053670574,53.8711289302741,16.4336708216802));
#54030=CARTESIAN_POINT('Ctrl Pts',(13.2137261528326,54.234995054198,16.4075023182212));
#54031=CARTESIAN_POINT('Ctrl Pts',(13.6068573480137,54.492676185537,16.3813338147623));
#54032=CARTESIAN_POINT('Ctrl Pts',(14.0193142510176,54.5286250418801,16.3551653113034));
#54033=CARTESIAN_POINT('Ctrl Pts',(14.4317711540215,54.5645738982232,16.3289968078444));
#54034=CARTESIAN_POINT('Ctrl Pts',(14.8635537648482,54.3787904795703,16.3028283043855));
#54035=CARTESIAN_POINT('Ctrl Pts',(15.1210456285731,54.0545822792718,16.2766598009266));
#54036=CARTESIAN_POINT('Ctrl Pts',(15.3785374922981,53.7303740789732,16.2504912974677));
#54037=CARTESIAN_POINT('Ctrl Pts',(15.4617386089214,53.267741097029,16.2243227940087));
#54038=CARTESIAN_POINT('Ctrl Pts',(15.3333406086023,52.8741334617557,16.1981542905498));
#54039=CARTESIAN_POINT('Ctrl Pts',(15.2049426082832,52.4805258264823,16.1719857870909));
#54040=CARTESIAN_POINT('Ctrl Pts',(14.8649454910218,52.1559435378799,16.145817283632));
#54041=CARTESIAN_POINT('Ctrl Pts',(14.4658080057675,52.0459331524117,16.119648780173));
#54042=CARTESIAN_POINT('Ctrl Pts',(14.1451555582542,51.9575548350262,16.0986259622422));
#54043=CARTESIAN_POINT('Ctrl Pts',(13.7863343457911,52.0076596690573,16.0776031443114));
#54044=CARTESIAN_POINT('Ctrl Pts',(13.4958915862187,52.1719376453661,16.0565803263806));
#54045=CARTESIAN_POINT('Ctrl Pts',(13.4961138435273,52.1700468646075,16.1934196736194));
#54046=CARTESIAN_POINT('Ctrl Pts',(13.5004665539579,52.1675277788309,16.193737536191));
#54047=CARTESIAN_POINT('Ctrl Pts',(13.5048355445965,52.1650370085359,16.1940553987625));
#54048=CARTESIAN_POINT('Ctrl Pts',(13.5092206128964,52.1625748725828,16.1943732613341));
#54049=CARTESIAN_POINT('Ctrl Pts',(13.8702278067029,51.9598759109143,16.220541764793));
#54050=CARTESIAN_POINT('Ctrl Pts',(14.3402037234666,51.9512504287578,16.2467102682519));
#54051=CARTESIAN_POINT('Ctrl Pts',(14.7084055750498,52.1405661950787,16.2728787717108));
#54052=CARTESIAN_POINT('Ctrl Pts',(15.076607426633,52.3298819613996,16.2990472751698));
#54053=CARTESIAN_POINT('Ctrl Pts',(15.3430352130359,52.7171389761979,16.3252157786287));
#54054=CARTESIAN_POINT('Ctrl Pts',(15.3882195489486,53.1286865903088,16.3513842820876));
#54055=CARTESIAN_POINT('Ctrl Pts',(15.4334038848614,53.5402342044196,16.3775527855466));
#54056=CARTESIAN_POINT('Ctrl Pts',(15.2573447702841,53.976072417843,16.4037212890055));
#54057=CARTESIAN_POINT('Ctrl Pts',(14.9389892027717,54.240766195907,16.4298897924644));
#54058=CARTESIAN_POINT('Ctrl Pts',(14.6206336352594,54.505459973971,16.4560582959233));
#54059=CARTESIAN_POINT('Ctrl Pts',(14.1599816148119,54.5990093166755,16.4822267993823));
#54060=CARTESIAN_POINT('Ctrl Pts',(13.7635949875347,54.4794655848163,16.5083953028412));
#54061=CARTESIAN_POINT('Ctrl Pts',(13.3672083602574,54.3599218529572,16.5345638063001));
#54062=CARTESIAN_POINT('Ctrl Pts',(13.0350871261504,54.0272850465344,16.560732309759));
#54063=CARTESIAN_POINT('Ctrl Pts',(12.916158385472,53.6307134674394,16.586900813218));
#54064=CARTESIAN_POINT('Ctrl Pts',(12.7972296447936,53.2341418883445,16.6130693166769));
#54065=CARTESIAN_POINT('Ctrl Pts',(12.891493397544,52.7736355365774,16.6392378201358));
#54066=CARTESIAN_POINT('Ctrl Pts',(13.1566806746197,52.4556909263592,16.6654063235948));
#54067=CARTESIAN_POINT('Ctrl Pts',(13.2513082234268,52.3422378246374,16.6747441069363));
#54068=CARTESIAN_POINT('Ctrl Pts',(13.3676994181703,52.2469370707529,16.6840818902779));
#54069=CARTESIAN_POINT('Ctrl Pts',(13.4969690270882,52.1733618792496,16.6934196736194));
#54070=CARTESIAN_POINT('Origin',(14.1292828945603,53.2669068454841,15.5));
#54071=CARTESIAN_POINT('',(13.498190246218,52.1716844371558,17.1934196736194));
#54072=CARTESIAN_POINT('',(13.4965460097018,52.1700456009992,17.0565803263806));
#54073=CARTESIAN_POINT('',(13.4970328945603,52.1718177223987,15.5));
#54074=CARTESIAN_POINT('Ctrl Pts',(13.4965460097018,52.1700456009992,17.0565803263806));
#54075=CARTESIAN_POINT('Ctrl Pts',(13.1622129933252,52.3652134872718,17.0321233490263));
#54076=CARTESIAN_POINT('Ctrl Pts',(12.9210086316388,52.724852170666,17.0076663716719));
#54077=CARTESIAN_POINT('Ctrl Pts',(12.8726933551042,53.1087658234733,16.9832093943176));
#54078=CARTESIAN_POINT('Ctrl Pts',(12.8209969225157,53.5195461748581,16.9570408908587));
#54079=CARTESIAN_POINT('Ctrl Pts',(12.9901314007569,53.9581179567514,16.9308723873998));
#54080=CARTESIAN_POINT('Ctrl Pts',(13.3042549587021,54.2278203840484,16.9047038839408));
#54081=CARTESIAN_POINT('Ctrl Pts',(13.6183785166473,54.4975228113455,16.8785353804819));
#54082=CARTESIAN_POINT('Ctrl Pts',(14.0774911542964,54.5983558840463,16.852366877023));
#54083=CARTESIAN_POINT('Ctrl Pts',(14.4757212681973,54.4851048462746,16.8261983735641));
#54084=CARTESIAN_POINT('Ctrl Pts',(14.8739513820981,54.371853808503,16.8000298701051));
#54085=CARTESIAN_POINT('Ctrl Pts',(15.2112989722506,54.0445186602589,16.7738613666462));
#54086=CARTESIAN_POINT('Ctrl Pts',(15.3364933887363,53.6498803767018,16.7476928631873));
#54087=CARTESIAN_POINT('Ctrl Pts',(15.4616878052219,53.2552420931447,16.7215243597283));
#54088=CARTESIAN_POINT('Ctrl Pts',(15.3747290480406,52.7933006742746,16.6953558562694));
#54089=CARTESIAN_POINT('Ctrl Pts',(15.1146104479144,52.4711961414872,16.6691873528105));
#54090=CARTESIAN_POINT('Ctrl Pts',(14.8544918477881,52.1490916086999,16.6430188493516));
#54091=CARTESIAN_POINT('Ctrl Pts',(14.4212134047168,51.9668239619953,16.6168503458926));
#54092=CARTESIAN_POINT('Ctrl Pts',(14.0090623276641,52.00612418165,16.5906818424337));
#54093=CARTESIAN_POINT('Ctrl Pts',(13.8300306074324,52.0231955574683,16.579314670416));
#54094=CARTESIAN_POINT('Ctrl Pts',(13.6549853934321,52.0820744013433,16.5679474983983));
#54095=CARTESIAN_POINT('Ctrl Pts',(13.4982981440081,52.173172919003,16.5565803263806));
#54096=CARTESIAN_POINT('Ctrl Pts',(13.4969690270882,52.1733618792496,16.6934196736194));
#54097=CARTESIAN_POINT('Ctrl Pts',(13.7299687153222,52.0407475948441,16.7102503937368));
#54098=CARTESIAN_POINT('Ctrl Pts',(14.0048072977942,51.9787144778412,16.7270811138542));
#54099=CARTESIAN_POINT('Ctrl Pts',(14.2694557749176,52.0081860992865,16.7439118339715));
#54100=CARTESIAN_POINT('Ctrl Pts',(14.6809327967389,52.0540087511013,16.7700803374305));
#54101=CARTESIAN_POINT('Ctrl Pts',(15.0677760389805,52.3210369234002,16.7962488408894));
#54102=CARTESIAN_POINT('Ctrl Pts',(15.2565204673329,52.6895319775572,16.8224173443483));
#54103=CARTESIAN_POINT('Ctrl Pts',(15.4452648956853,53.0580270317142,16.8485858478072));
#54104=CARTESIAN_POINT('Ctrl Pts',(15.4359105101485,53.5279889677293,16.8747543512661));
#54105=CARTESIAN_POINT('Ctrl Pts',(15.2326517793344,53.8886813318345,16.9009228547251));
#54106=CARTESIAN_POINT('Ctrl Pts',(15.0293930485204,54.2493736959397,16.927091358184));
#54107=CARTESIAN_POINT('Ctrl Pts',(14.6322299724291,54.500796488135,16.9532598616429));
#54108=CARTESIAN_POINT('Ctrl Pts',(14.2192554962477,54.5302086092019,16.9794283651019));
#54109=CARTESIAN_POINT('Ctrl Pts',(13.8062810200662,54.5596207302688,17.0055968685608));
#54110=CARTESIAN_POINT('Ctrl Pts',(13.3774951437946,54.3670221802074,17.0317653720197));
#54111=CARTESIAN_POINT('Ctrl Pts',(13.1251699439815,54.0387767018187,17.0579338754786));
#54112=CARTESIAN_POINT('Ctrl Pts',(12.8728447441683,53.7105312234301,17.0841023789376));
#54113=CARTESIAN_POINT('Ctrl Pts',(12.7969802208135,53.2466388167143,17.1102708823965));
#54114=CARTESIAN_POINT('Ctrl Pts',(12.9315961537198,52.8551138190488,17.1364393858554));
#54115=CARTESIAN_POINT('Ctrl Pts',(13.0293020925489,52.570940046702,17.1554328151101));
#54116=CARTESIAN_POINT('Ctrl Pts',(13.2378899597344,52.32488970875,17.1744262443648));
#54117=CARTESIAN_POINT('Ctrl Pts',(13.498190246218,52.1716844371558,17.1934196736194));
#54118=CARTESIAN_POINT('Origin',(14.1292828945603,53.2669068454841,15.5));
#54119=CARTESIAN_POINT('',(13.4957229821349,52.1707788329429,17.6934196736194));
#54120=CARTESIAN_POINT('',(13.4965541629804,52.1730078059394,17.5565803263806));
#54121=CARTESIAN_POINT('',(13.4970328945603,52.1718177223987,15.5));
#54122=CARTESIAN_POINT('',(13.8936870225526,54.5092654229862,18.));
#54123=CARTESIAN_POINT('Ctrl Pts',(13.4957229821349,52.1707788329429,17.6934196736194));
#54124=CARTESIAN_POINT('Ctrl Pts',(13.8217103338362,51.9852932094709,17.7171076053695));
#54125=CARTESIAN_POINT('Ctrl Pts',(14.2369080256434,51.9506029252058,17.7407955371196));
#54126=CARTESIAN_POINT('Ctrl Pts',(14.5864865212314,52.0858847696684,17.7644834688697));
#54127=CARTESIAN_POINT('Ctrl Pts',(14.9726724562246,52.2353331660965,17.7906519723286));
#54128=CARTESIAN_POINT('Ctrl Pts',(15.2787764866269,52.5922161636807,17.8168204757875));
#54129=CARTESIAN_POINT('Ctrl Pts',(15.3668468800596,52.9968087774221,17.8429889792464));
#54130=CARTESIAN_POINT('Ctrl Pts',(15.4549172734922,53.4014013911635,17.8691574827054));
#54131=CARTESIAN_POINT('Ctrl Pts',(15.3249540299554,53.8537036210623,17.8953259861643));
#54132=CARTESIAN_POINT('Ctrl Pts',(15.0367817327077,54.1500381490016,17.9214944896232));
#54133=CARTESIAN_POINT('Ctrl Pts',(14.74860943546,54.4463726769409,17.9476629930821));
#54134=CARTESIAN_POINT('Ctrl Pts',(14.3022280845015,54.5867395029208,17.9738314965411));
#54135=CARTESIAN_POINT('Ctrl Pts',(13.8936870225526,54.5092654229862,18.));
#54136=CARTESIAN_POINT('',(12.9337042190835,52.8487739793662,18.));
#54137=CARTESIAN_POINT('Origin',(14.1292828945603,53.2669068454841,18.));
#54138=CARTESIAN_POINT('Ctrl Pts',(12.9336937527447,52.848768453162,18.));
#54139=CARTESIAN_POINT('Ctrl Pts',(12.8048883200695,53.2213447345786,17.975091839613));
#54140=CARTESIAN_POINT('Ctrl Pts',(12.8625878757539,53.660362859942,17.950183679226));
#54141=CARTESIAN_POINT('Ctrl Pts',(13.0861189278269,53.984999064981,17.925275518839));
#54142=CARTESIAN_POINT('Ctrl Pts',(13.3209605627957,54.3260617336993,17.89910701538));
#54143=CARTESIAN_POINT('Ctrl Pts',(13.7388402922128,54.5408742678445,17.8729385119211));
#54144=CARTESIAN_POINT('Ctrl Pts',(14.1527389844808,54.5331807500212,17.8467700084622));
#54145=CARTESIAN_POINT('Ctrl Pts',(14.5666376767488,54.5254872321979,17.8206015050033));
#54146=CARTESIAN_POINT('Ctrl Pts',(14.9765553318677,54.2952876624062,17.7944330015443));
#54147=CARTESIAN_POINT('Ctrl Pts',(15.1985005516415,53.9457721211068,17.7682644980854));
#54148=CARTESIAN_POINT('Ctrl Pts',(15.4204457714153,53.5962565798076,17.7420959946265));
#54149=CARTESIAN_POINT('Ctrl Pts',(15.4544185558441,53.1274250670007,17.7159274911675));
#54150=CARTESIAN_POINT('Ctrl Pts',(15.2852740004506,52.7495241339714,17.6897589877086));
#54151=CARTESIAN_POINT('Ctrl Pts',(15.1161294450571,52.3716232009421,17.6635904842497));
#54152=CARTESIAN_POINT('Ctrl Pts',(14.7438675498413,52.0846528476904,17.6374219807908));
#54153=CARTESIAN_POINT('Ctrl Pts',(14.3353709232147,52.0172856023794,17.6112534773319));
#54154=CARTESIAN_POINT('Ctrl Pts',(14.0508839155709,51.9703694107086,17.5930290936814));
#54155=CARTESIAN_POINT('Ctrl Pts',(13.7488228128377,52.0299622436843,17.574804710031));
#54156=CARTESIAN_POINT('Ctrl Pts',(13.4965541629804,52.1730078059394,17.5565803263806));
#54157=CARTESIAN_POINT('Origin',(14.1292828945603,53.2669068454841,19.1042117235887));
#54158=CARTESIAN_POINT('',(13.3561475049578,51.9293198574881,14.3957882764113));
#54159=CARTESIAN_POINT('',(13.3590334722299,51.9326791410008,14.3542117235887));
#54160=CARTESIAN_POINT('',(13.3577828945603,51.9306296474448,19.1042117235887));
#54161=CARTESIAN_POINT('',(15.6194800884629,52.8667052421829,14.));
#54162=CARTESIAN_POINT('Ctrl Pts',(13.3590334722299,51.9326791410008,14.3542117235887));
#54163=CARTESIAN_POINT('Ctrl Pts',(13.1333102308069,52.0631907802776,14.3408151628948));
#54164=CARTESIAN_POINT('Ctrl Pts',(12.5590924929827,52.6090703324587,14.301250098742));
#54165=CARTESIAN_POINT('Ctrl Pts',(12.4888785260391,54.0475602728967,14.2355165311303));
#54166=CARTESIAN_POINT('Ctrl Pts',(13.875577901283,55.0671461874891,14.1570110207536));
#54167=CARTESIAN_POINT('Ctrl Pts',(15.4910603626305,54.4687297322861,14.0785055103768));
#54168=CARTESIAN_POINT('Ctrl Pts',(15.7510836294753,53.3567463262428,14.0261685034589));
#54169=CARTESIAN_POINT('Ctrl Pts',(15.6194800884629,52.8667052421829,14.));
#54170=CARTESIAN_POINT('',(15.2224969554152,52.1743874122524,14.));
#54171=CARTESIAN_POINT('Origin',(14.1292828945603,53.2669068454841,14.));
#54172=CARTESIAN_POINT('Ctrl Pts',(13.3561475049578,51.9293198574881,14.3957882764113));
#54173=CARTESIAN_POINT('Ctrl Pts',(13.3167322940313,51.9517582304519,14.3934410251636));
#54174=CARTESIAN_POINT('Ctrl Pts',(12.8509091548948,52.2463455523906,14.3649252704569));
#54175=CARTESIAN_POINT('Ctrl Pts',(12.312999126503,53.317416116839,14.3102410122914));
#54176=CARTESIAN_POINT('Ctrl Pts',(13.1694776941512,54.809893106608,14.2317355019146));
#54177=CARTESIAN_POINT('Ctrl Pts',(14.8870885705587,54.9183199028175,14.1532299915378));
#54178=CARTESIAN_POINT('Ctrl Pts',(15.9077095091603,53.5682793339942,14.0759848242329));
#54179=CARTESIAN_POINT('Ctrl Pts',(15.5613200902447,52.5158444925152,14.024908160387));
#54180=CARTESIAN_POINT('Ctrl Pts',(15.2225055381224,52.1743757967134,14.));
#54181=CARTESIAN_POINT('Origin',(14.1292828945603,53.2669068454841,19.1042117235887));
#54182=CARTESIAN_POINT('',(13.3586534741695,51.9327902292019,14.8957882764113));
#54183=CARTESIAN_POINT('',(13.3577899368159,51.928743983656,14.8542117235887));
#54184=CARTESIAN_POINT('',(13.3577828945603,51.9306296474448,19.1042117235887));
#54185=CARTESIAN_POINT('Ctrl Pts',(13.3577899368159,51.928743983656,14.8542117235887));
#54186=CARTESIAN_POINT('Ctrl Pts',(12.9734547442474,52.1543891335537,14.8311595169817));
#54187=CARTESIAN_POINT('Ctrl Pts',(12.3621732880177,53.0098569651208,14.7819388069158));
#54188=CARTESIAN_POINT('Ctrl Pts',(12.8743108410601,54.5809237767911,14.706549593391));
#54189=CARTESIAN_POINT('Ctrl Pts',(14.53309819057,55.0385159317414,14.6280440830142));
#54190=CARTESIAN_POINT('Ctrl Pts',(15.8297520454146,53.9072361260964,14.5495385726375));
#54191=CARTESIAN_POINT('Ctrl Pts',(15.6013490876951,52.2017963646938,14.4710330622607));
#54192=CARTESIAN_POINT('Ctrl Pts',(14.3170802291729,51.5794230562898,14.4059241125778));
#54193=CARTESIAN_POINT('Ctrl Pts',(13.5742323121468,51.8082526389225,14.3669836663538));
#54194=CARTESIAN_POINT('Ctrl Pts',(13.3590334722299,51.9326791410008,14.3542117235887));
#54195=CARTESIAN_POINT('Ctrl Pts',(13.3586534741695,51.9327902292019,14.8957882764113));
#54196=CARTESIAN_POINT('Ctrl Pts',(13.1561499564235,52.0491845394435,14.8837853792505));
#54197=CARTESIAN_POINT('Ctrl Pts',(12.5927601381537,52.5577927522065,14.8456139786307));
#54198=CARTESIAN_POINT('Ctrl Pts',(12.4499580614657,53.9607971579715,14.781274074552));
#54199=CARTESIAN_POINT('Ctrl Pts',(13.7817713167743,55.0504032414556,14.7027685641753));
#54200=CARTESIAN_POINT('Ctrl Pts',(15.4252464910755,54.5405234556122,14.6242630537985));
#54201=CARTESIAN_POINT('Ctrl Pts',(15.9064600587523,52.8884418877606,14.5457575434217));
#54202=CARTESIAN_POINT('Ctrl Pts',(14.8271456061161,51.6150089076652,14.4695992842926));
#54203=CARTESIAN_POINT('Ctrl Pts',(13.7561556767951,51.7016023764131,14.4196095286225));
#54204=CARTESIAN_POINT('Ctrl Pts',(13.3561475049578,51.9293198574881,14.3957882764113));
#54205=CARTESIAN_POINT('Origin',(14.1292828945603,53.2669068454841,19.1042117235887));
#54206=CARTESIAN_POINT('',(13.3583675961487,51.9292271650606,15.3957882764113));
#54207=CARTESIAN_POINT('',(13.3567403793943,51.9314820095869,15.3542117235887));
#54208=CARTESIAN_POINT('',(13.3577828945603,51.9306296474448,19.1042117235887));
#54209=CARTESIAN_POINT('Ctrl Pts',(13.3567403793943,51.9314820095869,15.3542117235887));
#54210=CARTESIAN_POINT('Ctrl Pts',(13.2463612263437,51.9939332857897,15.3476723745276));
#54211=CARTESIAN_POINT('Ctrl Pts',(12.7340280693376,52.3726757467305,15.3149645220075));
#54212=CARTESIAN_POINT('Ctrl Pts',(12.343540269987,53.6026792252177,15.2560881660285));
#54213=CARTESIAN_POINT('Ctrl Pts',(13.4243618186884,54.9416323741225,15.1775826556517));
#54214=CARTESIAN_POINT('Ctrl Pts',(15.1373732173661,54.7786522269087,15.0990771452749));
#54215=CARTESIAN_POINT('Ctrl Pts',(15.9463055097723,53.2599021305098,15.0205716348981));
#54216=CARTESIAN_POINT('Ctrl Pts',(15.1256881964072,51.7474355457531,14.9420661245214));
#54217=CARTESIAN_POINT('Ctrl Pts',(13.9148311256039,51.641642546183,14.8866128207515));
#54218=CARTESIAN_POINT('Ctrl Pts',(13.4097460280966,51.8982402977282,14.8573280204407));
#54219=CARTESIAN_POINT('Ctrl Pts',(13.3577899368159,51.928743983656,14.8542117235887));
#54220=CARTESIAN_POINT('Ctrl Pts',(13.3583675961486,51.9292271650606,15.3957882764113));
#54221=CARTESIAN_POINT('Ctrl Pts',(12.997111941728,52.141960595601,15.3741297333373));
#54222=CARTESIAN_POINT('Ctrl Pts',(12.3860414668385,52.9469081505226,15.3263026868045));
#54223=CARTESIAN_POINT('Ctrl Pts',(12.8070334555363,54.5132114643008,15.2523071368127));
#54224=CARTESIAN_POINT('Ctrl Pts',(14.4395092097517,55.0572639347494,15.1738016264359));
#54225=CARTESIAN_POINT('Ctrl Pts',(15.7937667074068,53.9956815464663,15.0952961160592));
#54226=CARTESIAN_POINT('Ctrl Pts',(15.6552753932384,52.2805167973031,15.0167906056824));
#54227=CARTESIAN_POINT('Ctrl Pts',(14.3786526271626,51.5769541863948,14.9502879924664));
#54228=CARTESIAN_POINT('Ctrl Pts',(13.5976445334062,51.7954237290868,14.9099538827094));
#54229=CARTESIAN_POINT('Ctrl Pts',(13.3586534741695,51.9327902292019,14.8957882764113));
#54230=CARTESIAN_POINT('Origin',(14.1292828945603,53.2669068454841,19.1042117235887));
#54231=CARTESIAN_POINT('',(13.3563902185847,51.9307759828649,15.8957882764113));
#54232=CARTESIAN_POINT('',(13.3594516225044,51.9317765575137,15.8542117235887));
#54233=CARTESIAN_POINT('',(13.3577828945603,51.9306296474448,19.1042117235887));
#54234=CARTESIAN_POINT('Ctrl Pts',(13.3594516225044,51.9317765575137,15.8542117235887));
#54235=CARTESIAN_POINT('Ctrl Pts',(13.0875688358439,52.0906633350794,15.8380167286145));
#54236=CARTESIAN_POINT('Ctrl Pts',(12.4951087068473,52.7167109460471,15.7956532301813));
#54237=CARTESIAN_POINT('Ctrl Pts',(12.5800904986591,54.2164449634099,15.7271212282891));
#54238=CARTESIAN_POINT('Ctrl Pts',(14.0667923195219,55.0828679235634,15.6486157179124));
#54239=CARTESIAN_POINT('Ctrl Pts',(15.6095371717915,54.3206938223985,15.5701102075356));
#54240=CARTESIAN_POINT('Ctrl Pts',(15.8247548010729,52.6134584968728,15.4916046971588));
#54241=CARTESIAN_POINT('Ctrl Pts',(14.6281635632835,51.5856454904132,15.4196385358432));
#54242=CARTESIAN_POINT('Ctrl Pts',(13.6880653197304,51.7440221062451,15.3738408779865));
#54243=CARTESIAN_POINT('Ctrl Pts',(13.3567403793943,51.9314820095869,15.3542117235887));
#54244=CARTESIAN_POINT('Ctrl Pts',(13.3563902185847,51.9307759828649,15.8957882764113));
#54245=CARTESIAN_POINT('Ctrl Pts',(13.2696421210522,51.9798417675732,15.8906425908832));
#54246=CARTESIAN_POINT('Ctrl Pts',(12.7721552352232,52.3292268802209,15.8593284018961));
#54247=CARTESIAN_POINT('Ctrl Pts',(12.3283713567551,53.5084362707541,15.8018457094502));
#54248=CARTESIAN_POINT('Ctrl Pts',(13.3373852079753,54.9023018690978,15.7233401990734));
#54249=CARTESIAN_POINT('Ctrl Pts',(15.0565917302206,54.8295063313936,15.6448346886966));
#54250=CARTESIAN_POINT('Ctrl Pts',(15.9441656443073,53.3553344251959,15.5663291783198));
#54251=CARTESIAN_POINT('Ctrl Pts',(15.2041095597138,51.8018585649929,15.4878236679431));
#54252=CARTESIAN_POINT('Ctrl Pts',(13.9702286955569,51.6283710932553,15.4309767006402));
#54253=CARTESIAN_POINT('Ctrl Pts',(13.4335918937727,51.8849296635608,15.4002982367963));
#54254=CARTESIAN_POINT('Ctrl Pts',(13.3583675961486,51.9292271650606,15.3957882764113));
#54255=CARTESIAN_POINT('Origin',(14.1292828945603,53.2669068454841,19.1042117235887));
#54256=CARTESIAN_POINT('',(13.3593268090703,51.9322833195368,16.3957882764113));
#54257=CARTESIAN_POINT('',(13.356661426989,51.9284687668027,16.3542117235887));
#54258=CARTESIAN_POINT('',(13.3577828945603,51.9306296474448,19.1042117235887));
#54259=CARTESIAN_POINT('Ctrl Pts',(13.356661426989,51.9284687668027,16.3542117235887));
#54260=CARTESIAN_POINT('Ctrl Pts',(12.9247061434582,52.1784583832132,16.3283610827014));
#54261=CARTESIAN_POINT('Ctrl Pts',(12.3198850098697,53.141372730953,16.2763419383551));
#54262=CARTESIAN_POINT('Ctrl Pts',(13.0196563589383,54.7057774673455,16.1981542905498));
#54263=CARTESIAN_POINT('Ctrl Pts',(14.7174120024405,54.9861287238479,16.1196487801731));
#54264=CARTESIAN_POINT('Ctrl Pts',(15.8877194798386,53.7246409278238,16.0411432697963));
#54265=CARTESIAN_POINT('Ctrl Pts',(15.4810192232586,52.0526463245539,15.9626377594195));
#54266=CARTESIAN_POINT('Ctrl Pts',(14.1960288388142,51.5899006730013,15.900327244017));
#54267=CARTESIAN_POINT('Ctrl Pts',(13.5268876287458,51.8339278933634,15.8641852320734));
#54268=CARTESIAN_POINT('Ctrl Pts',(13.3594516225044,51.9317765575137,15.8542117235887));
#54269=CARTESIAN_POINT('Ctrl Pts',(13.3593268090703,51.9322833195368,16.3957882764113));
#54270=CARTESIAN_POINT('Ctrl Pts',(13.1103670811162,52.0770293806041,16.3809869449701));
#54271=CARTESIAN_POINT('Ctrl Pts',(12.5263819999043,52.6621976201272,16.3400171100699));
#54272=CARTESIAN_POINT('Ctrl Pts',(12.5323627785853,54.1337776405724,16.2728787717109));
#54273=CARTESIAN_POINT('Ctrl Pts',(13.9715120885841,55.0770800976453,16.1943732613341));
#54274=CARTESIAN_POINT('Ctrl Pts',(15.5521540067467,54.3969761475115,16.1158677509573));
#54275=CARTESIAN_POINT('Ctrl Pts',(15.8567312853937,52.7033991815805,16.0373622405805));
#54276=CARTESIAN_POINT('Ctrl Pts',(14.6936723389742,51.5930711363043,15.9640024157319));
#54277=CARTESIAN_POINT('Ctrl Pts',(13.7108015891028,51.7303165780056,15.9168110943421));
#54278=CARTESIAN_POINT('Ctrl Pts',(13.3563902185847,51.9307759828649,15.8957882764113));
#54279=CARTESIAN_POINT('Origin',(14.1292828945603,53.2669068454841,19.1042117235887));
#54280=CARTESIAN_POINT('',(13.3571887756701,51.9284672248908,16.8957882764113));
#54281=CARTESIAN_POINT('',(13.3577049605868,51.9325138973624,16.8542117235887));
#54282=CARTESIAN_POINT('',(13.3577828945603,51.9306296474448,19.1042117235887));
#54283=CARTESIAN_POINT('Ctrl Pts',(13.3577049605868,51.9325138973624,16.8542117235887));
#54284=CARTESIAN_POINT('Ctrl Pts',(13.1999643464624,52.02229366841,16.8448739402472));
#54285=CARTESIAN_POINT('Ctrl Pts',(12.6599209222933,52.4644795705919,16.8093676534467));
#54286=CARTESIAN_POINT('Ctrl Pts',(12.38882648105,53.7888562103795,16.7476928631873));
#54287=CARTESIAN_POINT('Ctrl Pts',(13.6046344626092,55.0065515658014,16.6691873528105));
#54288=CARTESIAN_POINT('Ctrl Pts',(15.2909596525271,54.6640921689023,16.5906818424337));
#54289=CARTESIAN_POINT('Ctrl Pts',(15.9354654978243,53.0686037624672,16.512176332057));
#54290=CARTESIAN_POINT('Ctrl Pts',(14.9601438503283,51.6509582729447,16.4336708216802));
#54291=CARTESIAN_POINT('Ctrl Pts',(13.8062061827166,51.672136525716,16.3810159521908));
#54292=CARTESIAN_POINT('Ctrl Pts',(13.3619728008082,51.9253948645857,16.3545295861603));
#54293=CARTESIAN_POINT('Ctrl Pts',(13.356661426989,51.9284687668027,16.3542117235887));
#54294=CARTESIAN_POINT('Ctrl Pts',(13.3571887756701,51.9284672248908,16.8957882764113));
#54295=CARTESIAN_POINT('Ctrl Pts',(12.9492205318827,52.1666198927584,16.871331299057));
#54296=CARTESIAN_POINT('Ctrl Pts',(12.3399661957944,53.0750256353043,16.8207058182437));
#54297=CARTESIAN_POINT('Ctrl Pts',(12.9456243299004,54.6455189484075,16.7439118339715));
#54298=CARTESIAN_POINT('Ctrl Pts',(14.6263142466089,55.0146421540478,16.6654063235947));
#54299=CARTESIAN_POINT('Ctrl Pts',(15.8612545351151,53.8163547667627,16.586900813218));
#54300=CARTESIAN_POINT('Ctrl Pts',(15.5429215283993,52.1253094303059,16.5083953028412));
#54301=CARTESIAN_POINT('Ctrl Pts',(14.2558484377857,51.5838751930056,16.4446911239056));
#54302=CARTESIAN_POINT('Ctrl Pts',(13.5505236662164,51.8211207946266,16.407155448429));
#54303=CARTESIAN_POINT('Ctrl Pts',(13.3593268090703,51.9322833195368,16.3957882764113));
#54304=CARTESIAN_POINT('Origin',(14.1292828945603,53.2669068454841,19.1042117235887));
#54305=CARTESIAN_POINT('',(13.3571987246687,51.9320818411207,17.3957882764113));
#54306=CARTESIAN_POINT('',(13.3591951473145,51.9304670067728,17.3542117235887));
#54307=CARTESIAN_POINT('',(13.3577828945603,51.9306296474448,19.1042117235887));
#54308=CARTESIAN_POINT('Ctrl Pts',(13.3591951473145,51.9304670067728,17.3542117235887));
#54309=CARTESIAN_POINT('Ctrl Pts',(13.0415649835786,52.117414997338,17.3352182943341));
#54310=CARTESIAN_POINT('Ctrl Pts',(12.4363561313197,52.8313196200715,17.2900563616205));
#54311=CARTESIAN_POINT('Ctrl Pts',(12.6886936446445,54.3742998061272,17.2187259254479));
#54312=CARTESIAN_POINT('Ctrl Pts',(14.2583653103316,55.0793521495312,17.1402204150712));
#54313=CARTESIAN_POINT('Ctrl Pts',(15.7122742697831,54.1589598165365,17.0617149046944));
#54314=CARTESIAN_POINT('Ctrl Pts',(15.7465182007044,52.4385534884905,16.9832093943176));
#54315=CARTESIAN_POINT('Ctrl Pts',(14.4988281136715,51.5773043644133,16.9140416672824));
#54316=CARTESIAN_POINT('Ctrl Pts',(13.6420217015477,51.7706919591752,16.8710424437061));
#54317=CARTESIAN_POINT('Ctrl Pts',(13.3577049605868,51.9325138973624,16.8542117235887));
#54318=CARTESIAN_POINT('Ctrl Pts',(13.3571987246687,51.9320818411208,17.3957882764113));
#54319=CARTESIAN_POINT('Ctrl Pts',(13.2230139283874,52.0081695343042,17.3878441566028));
#54320=CARTESIAN_POINT('Ctrl Pts',(12.6963900910873,52.417984443011,17.3537315333353));
#54321=CARTESIAN_POINT('Ctrl Pts',(12.3638250796578,53.6967359986949,17.293450406609));
#54322=CARTESIAN_POINT('Ctrl Pts',(13.5139962436502,54.9765978264215,17.2149448962322));
#54323=CARTESIAN_POINT('Ctrl Pts',(15.2159841085891,54.7231706136823,17.1364393858554));
#54324=CARTESIAN_POINT('Ctrl Pts',(15.9433860453712,53.1637302055401,17.0579338754786));
#54325=CARTESIAN_POINT('Ctrl Pts',(15.043860342301,51.6968216692226,16.9794283651019));
#54326=CARTESIAN_POINT('Ctrl Pts',(13.8598729208803,51.6563265828795,16.9253798320794));
#54327=CARTESIAN_POINT('Ctrl Pts',(13.3857388409122,51.9118010399395,16.8974998025159));
#54328=CARTESIAN_POINT('Ctrl Pts',(13.3571887756701,51.9284672248908,16.8957882764113));
#54329=CARTESIAN_POINT('Origin',(14.1292828945603,53.2669068454841,19.1042117235887));
#54330=CARTESIAN_POINT('',(13.3599426557471,51.9312965605688,17.8957882764113));
#54331=CARTESIAN_POINT('',(13.3561844802682,51.9293619476186,17.8542117235887));
#54332=CARTESIAN_POINT('',(13.3577828945603,51.9306296474448,19.1042117235887));
#54333=CARTESIAN_POINT('',(15.2209662466057,52.1764590205668,18.));
#54334=CARTESIAN_POINT('Ctrl Pts',(15.2209662466057,52.1764590205668,18.));
#54335=CARTESIAN_POINT('Ctrl Pts',(14.8623799894179,51.8174664687922,17.9738314965411));
#54336=CARTESIAN_POINT('Ctrl Pts',(14.136921272848,51.597902680369,17.9390942553448));
#54337=CARTESIAN_POINT('Ctrl Pts',(13.5035430816838,51.8470756229631,17.9043570141486));
#54338=CARTESIAN_POINT('Ctrl Pts',(13.3599426557471,51.9312965605688,17.8957882764113));
#54339=CARTESIAN_POINT('',(15.6220396093989,52.866415579935,18.));
#54340=CARTESIAN_POINT('Origin',(14.1292828945603,53.2669068454841,18.));
#54341=CARTESIAN_POINT('Ctrl Pts',(15.6220539738783,52.8664139542998,18.));
#54342=CARTESIAN_POINT('Ctrl Pts',(15.4957406336878,52.4022578052826,17.975091839613));
#54343=CARTESIAN_POINT('Ctrl Pts',(14.7933534445257,51.6161821464323,17.9264957474759));
#54344=CARTESIAN_POINT('Ctrl Pts',(13.7539689671603,51.7030240140342,17.8778996553388));
#54345=CARTESIAN_POINT('Ctrl Pts',(13.3561844802682,51.9293619476186,17.8542117235887));
#54346=CARTESIAN_POINT('Origin',(-39.0658530619283,38.8697713466882,15.5));
#54347=CARTESIAN_POINT('',(-38.4345426068235,37.7764071067805,14.1934196736194));
#54348=CARTESIAN_POINT('',(-38.4325424620228,37.7762177647969,14.0565803263806));
#54349=CARTESIAN_POINT('',(-38.4336030619283,37.7746822236028,15.5));
#54350=CARTESIAN_POINT('',(-39.3014489339362,37.6274127691862,14.));
#54351=CARTESIAN_POINT('Ctrl Pts',(-38.4325424620228,37.7762177647969,14.0565803263806));
#54352=CARTESIAN_POINT('Ctrl Pts',(-38.6929044073908,37.6289035868348,14.0377202175871));
#54353=CARTESIAN_POINT('Ctrl Pts',(-39.0070060787276,37.5715758131853,14.0188601087935));
#54354=CARTESIAN_POINT('Ctrl Pts',(-39.3014489339362,37.6274127691862,14.));
#54355=CARTESIAN_POINT('',(-38.4336030619283,37.7746822236028,14.));
#54356=CARTESIAN_POINT('Origin',(-39.0658530619283,38.8697713466882,14.));
#54357=CARTESIAN_POINT('',(-38.4336030619283,37.7746822236028,13.));
#54358=CARTESIAN_POINT('',(-38.4336030619283,37.7746822236028,15.5));
#54359=CARTESIAN_POINT('',(-39.7608672580762,37.8134023216061,13.));
#54360=CARTESIAN_POINT('Origin',(-39.0658530619283,38.8697713466882,13.));
#54361=CARTESIAN_POINT('',(-38.3708388657805,39.9261403717704,13.));
#54362=CARTESIAN_POINT('Origin',(-39.0658530619283,38.8697713466882,13.));
#54363=CARTESIAN_POINT('Origin',(-39.0658530619283,38.8697713466882,13.));
#54364=CARTESIAN_POINT('',(-40.2614318702746,39.2879073628688,14.));
#54365=CARTESIAN_POINT('Origin',(-39.0658530619283,38.8697713466882,14.));
#54366=CARTESIAN_POINT('Ctrl Pts',(-40.261442519219,39.2879130030575,14.));
#54367=CARTESIAN_POINT('Ctrl Pts',(-40.3902451808538,38.9153391953948,14.024908160387));
#54368=CARTESIAN_POINT('Ctrl Pts',(-40.3325529350425,38.4763144202223,14.049816320774));
#54369=CARTESIAN_POINT('Ctrl Pts',(-40.109022770241,38.1516757839093,14.074724481161));
#54370=CARTESIAN_POINT('Ctrl Pts',(-39.8741820674394,37.8106105608956,14.10089298462));
#54371=CARTESIAN_POINT('Ctrl Pts',(-39.4562961811819,37.5958001287034,14.1270614880789));
#54372=CARTESIAN_POINT('Ctrl Pts',(-39.0423952919771,37.6034944064735,14.1532299915378));
#54373=CARTESIAN_POINT('Ctrl Pts',(-38.8305051320303,37.6074333729988,14.1666265522317));
#54374=CARTESIAN_POINT('Ctrl Pts',(-38.619659348036,37.6696856996876,14.1800231129255));
#54375=CARTESIAN_POINT('Ctrl Pts',(-38.4345426068235,37.7764071067805,14.1934196736194));
#54376=CARTESIAN_POINT('Origin',(-39.0658530619283,38.8697713466882,15.5));
#54377=CARTESIAN_POINT('',(-38.4322601856233,37.7739115851766,14.6934196736194));
#54378=CARTESIAN_POINT('',(-38.4333416483911,37.7729821125454,14.5565803263806));
#54379=CARTESIAN_POINT('',(-38.4336030619283,37.7746822236028,15.5));
#54380=CARTESIAN_POINT('Ctrl Pts',(-38.4333416483911,37.7729821125454,14.5565803263806));
#54381=CARTESIAN_POINT('Ctrl Pts',(-38.4654171032337,37.7542027235003,14.5542330751329));
#54382=CARTESIAN_POINT('Ctrl Pts',(-38.4983383982293,37.7369254869309,14.5518858238852));
#54383=CARTESIAN_POINT('Ctrl Pts',(-38.5320143785611,37.721272199783,14.5495385726375));
#54384=CARTESIAN_POINT('Ctrl Pts',(-38.9074535262253,37.5467603748252,14.5233700691785));
#54385=CARTESIAN_POINT('Ctrl Pts',(-39.3766930387427,37.5740903519378,14.4972015657196));
#54386=CARTESIAN_POINT('Ctrl Pts',(-39.7293604226538,37.7909904189904,14.4710330622607));
#54387=CARTESIAN_POINT('Ctrl Pts',(-40.0820278065649,38.007890486043,14.4448645588018));
#54388=CARTESIAN_POINT('Ctrl Pts',(-40.3181230618696,38.4143606430356,14.4186960553428));
#54389=CARTESIAN_POINT('Ctrl Pts',(-40.3316969948736,38.8281685539702,14.3925275518839));
#54390=CARTESIAN_POINT('Ctrl Pts',(-40.3452709278776,39.2419764649047,14.366359048425));
#54391=CARTESIAN_POINT('Ctrl Pts',(-40.1363235385809,39.6631221297811,14.340190544966));
#54392=CARTESIAN_POINT('Ctrl Pts',(-39.7987141516887,39.9026904288663,14.3140220415071));
#54393=CARTESIAN_POINT('Ctrl Pts',(-39.4611047647966,40.1422587279515,14.2878535380482));
#54394=CARTESIAN_POINT('Ctrl Pts',(-38.9948333803092,40.2002496612456,14.2616850345893));
#54395=CARTESIAN_POINT('Ctrl Pts',(-38.6086468373336,40.0507988707032,14.2355165311303));
#54396=CARTESIAN_POINT('Ctrl Pts',(-38.222460294358,39.9013480801608,14.2093480276714));
#54397=CARTESIAN_POINT('Ctrl Pts',(-37.9163585928944,39.5444555657821,14.1831795242125));
#54398=CARTESIAN_POINT('Ctrl Pts',(-37.8282870218578,39.139867719385,14.1570110207536));
#54399=CARTESIAN_POINT('Ctrl Pts',(-37.7402154508212,38.7352798729879,14.1308425172946));
#54400=CARTESIAN_POINT('Ctrl Pts',(-37.8701740102116,38.2829966945726,14.1046740138357));
#54401=CARTESIAN_POINT('Ctrl Pts',(-38.1583471155032,37.9866613986385,14.0785055103768));
#54402=CARTESIAN_POINT('Ctrl Pts',(-38.2388287062341,37.9039002541438,14.0711971157114));
#54403=CARTESIAN_POINT('Ctrl Pts',(-38.3316507930811,37.8333028094348,14.063888721046));
#54404=CARTESIAN_POINT('Ctrl Pts',(-38.4325424620228,37.7762177647969,14.0565803263806));
#54405=CARTESIAN_POINT('Ctrl Pts',(-38.4345426068235,37.7764071067805,14.1934196736194));
#54406=CARTESIAN_POINT('Ctrl Pts',(-38.2580569790832,37.8781526020867,14.2061916163845));
#54407=CARTESIAN_POINT('Ctrl Pts',(-38.1049570809751,38.0203170861652,14.2189635591495));
#54408=CARTESIAN_POINT('Ctrl Pts',(-37.9966332783609,38.1909038725226,14.2317355019146));
#54409=CARTESIAN_POINT('Ctrl Pts',(-37.7746880461016,38.5404200730694,14.2579040053735));
#54410=CARTESIAN_POINT('Ctrl Pts',(-37.7407134737351,39.0092534864306,14.2840725088324));
#54411=CARTESIAN_POINT('Ctrl Pts',(-37.909858143811,39.3871556515896,14.3102410122914));
#54412=CARTESIAN_POINT('Ctrl Pts',(-38.0790028138868,39.7650578167486,14.3364095157503));
#54413=CARTESIAN_POINT('Ctrl Pts',(-38.451266726405,40.0520287337055,14.3625780192092));
#54414=CARTESIAN_POINT('Ctrl Pts',(-38.8597647299447,40.1193961008256,14.3887465226681));
#54415=CARTESIAN_POINT('Ctrl Pts',(-39.2682627334845,40.1867634679457,14.4149150261271));
#54416=CARTESIAN_POINT('Ctrl Pts',(-39.7129948280458,40.034527285229,14.441083529586));
#54417=CARTESIAN_POINT('Ctrl Pts',(-39.9945169439557,39.7309476936789,14.4672520330449));
#54418=CARTESIAN_POINT('Ctrl Pts',(-40.2760390598657,39.4273681021289,14.4934205365039));
#54419=CARTESIAN_POINT('Ctrl Pts',(-40.3943511971242,38.9724451017455,14.5195890399628));
#54420=CARTESIAN_POINT('Ctrl Pts',(-40.2964110981384,38.570173729657,14.5457575434217));
#54421=CARTESIAN_POINT('Ctrl Pts',(-40.1984709991526,38.1679023575684,14.5719260468806));
#54422=CARTESIAN_POINT('Ctrl Pts',(-39.8842786639225,37.8182826137747,14.5980945503396));
#54423=CARTESIAN_POINT('Ctrl Pts',(-39.4947165862022,37.6780870841148,14.6242630537985));
#54424=CARTESIAN_POINT('Ctrl Pts',(-39.1515458154338,37.5545868495612,14.6473152604055));
#54425=CARTESIAN_POINT('Ctrl Pts',(-38.7498873821672,37.59360186782,14.6703674670124));
#54426=CARTESIAN_POINT('Ctrl Pts',(-38.4322601856233,37.7739115851766,14.6934196736194));
#54427=CARTESIAN_POINT('Origin',(-39.0658530619283,38.8697713466882,15.5));
#54428=CARTESIAN_POINT('',(-38.4346334551116,37.7742886171168,15.1934196736194));
#54429=CARTESIAN_POINT('',(-38.4347780105727,37.7761824162226,15.0565803263806));
#54430=CARTESIAN_POINT('',(-38.4336030619283,37.7746822236028,15.5));
#54431=CARTESIAN_POINT('Ctrl Pts',(-38.4347780105727,37.7761824162226,15.0565803263806));
#54432=CARTESIAN_POINT('Ctrl Pts',(-38.6003617341532,37.6801555214811,15.0445774292198));
#54433=CARTESIAN_POINT('Ctrl Pts',(-38.7864577331936,37.6199570207433,15.0325745320589));
#54434=CARTESIAN_POINT('Ctrl Pts',(-38.9758802222155,37.6064663135108,15.0205716348981));
#54435=CARTESIAN_POINT('Ctrl Pts',(-39.388855772431,37.5770541129273,14.9944031314392));
#54436=CARTESIAN_POINT('Ctrl Pts',(-39.8176427771529,37.7696531482711,14.9682346279803));
#54437=CARTESIAN_POINT('Ctrl Pts',(-40.0699686232679,38.097899483489,14.9420661245214));
#54438=CARTESIAN_POINT('Ctrl Pts',(-40.3222944693828,38.4261458187069,14.9158976210624));
#54439=CARTESIAN_POINT('Ctrl Pts',(-40.3981591568908,38.8900394537988,14.8897291176035));
#54440=CARTESIAN_POINT('Ctrl Pts',(-40.2635428887314,39.2815654536187,14.8635606141446));
#54441=CARTESIAN_POINT('Ctrl Pts',(-40.1289266205721,39.6730914534386,14.8373921106856));
#54442=CARTESIAN_POINT('Ctrl Pts',(-39.7838293967455,39.9922498179864,14.8112236072267));
#54443=CARTESIAN_POINT('Ctrl Pts',(-39.3829992856625,40.0959251593025,14.7850551037678));
#54444=CARTESIAN_POINT('Ctrl Pts',(-38.9821691745794,40.1996005006187,14.7588866003089));
#54445=CARTESIAN_POINT('Ctrl Pts',(-38.52560617624,40.0877928187031,14.7327180968499));
#54446=CARTESIAN_POINT('Ctrl Pts',(-38.2180337582993,39.8106400014137,14.706549593391));
#54447=CARTESIAN_POINT('Ctrl Pts',(-37.9104613403587,39.5334871841242,14.6803810899321));
#54448=CARTESIAN_POINT('Ctrl Pts',(-37.7518795028169,39.0909892314608,14.6542125864732));
#54449=CARTESIAN_POINT('Ctrl Pts',(-37.8134079754514,38.681563441615,14.6280440830142));
#54450=CARTESIAN_POINT('Ctrl Pts',(-37.869417493424,38.308862151417,14.604222830803));
#54451=CARTESIAN_POINT('Ctrl Pts',(-38.1078215318973,37.9635661257619,14.5804015785918));
#54452=CARTESIAN_POINT('Ctrl Pts',(-38.4333416483911,37.7729821125454,14.5565803263806));
#54453=CARTESIAN_POINT('Ctrl Pts',(-38.4322601856233,37.7739115851766,14.6934196736194));
#54454=CARTESIAN_POINT('Ctrl Pts',(-38.389321969358,37.7982866315292,14.6965359704714));
#54455=CARTESIAN_POINT('Ctrl Pts',(-38.3479194071466,37.825243810264,14.6996522673233));
#54456=CARTESIAN_POINT('Ctrl Pts',(-38.3084045871421,37.8547306967159,14.7027685641753));
#54457=CARTESIAN_POINT('Ctrl Pts',(-37.976586486013,38.1023411545029,14.7289370676342));
#54458=CARTESIAN_POINT('Ctrl Pts',(-37.7778821039656,38.528333385603,14.7551055710931));
#54459=CARTESIAN_POINT('Ctrl Pts',(-37.8013916118278,38.941687151427,14.781274074552));
#54460=CARTESIAN_POINT('Ctrl Pts',(-37.82490111969,39.355040917251,14.807442578011));
#54461=CARTESIAN_POINT('Ctrl Pts',(-38.0706245174618,39.755756217799,14.8336110814699));
#54462=CARTESIAN_POINT('Ctrl Pts',(-38.428377122171,39.9641476765194,14.8597795849288));
#54463=CARTESIAN_POINT('Ctrl Pts',(-38.7861297268802,40.1725391352398,14.8859480883877));
#54464=CARTESIAN_POINT('Ctrl Pts',(-39.2559115385268,40.1886067521326,14.9121165918467));
#54465=CARTESIAN_POINT('Ctrl Pts',(-39.6270665080505,40.005145553951,14.9382850953056));
#54466=CARTESIAN_POINT('Ctrl Pts',(-39.9982214775741,39.8216843557693,14.9644535987645));
#54467=CARTESIAN_POINT('Ctrl Pts',(-40.2707496049748,39.4386943425132,14.9906221022234));
#54468=CARTESIAN_POINT('Ctrl Pts',(-40.3224461866044,39.0279128196441,15.0167906056824));
#54469=CARTESIAN_POINT('Ctrl Pts',(-40.3741427682341,38.6171312967749,15.0429591091413));
#54470=CARTESIAN_POINT('Ctrl Pts',(-40.2050078040927,38.1785582642928,15.0691276126002));
#54471=CARTESIAN_POINT('Ctrl Pts',(-39.8908833495191,37.9088550679237,15.0952961160592));
#54472=CARTESIAN_POINT('Ctrl Pts',(-39.5767588949456,37.6391518715546,15.1214646195181));
#54473=CARTESIAN_POINT('Ctrl Pts',(-39.1176449499399,37.5383185112986,15.147633122977));
#54474=CARTESIAN_POINT('Ctrl Pts',(-38.7194137008706,37.6515698720153,15.1738016264359));
#54475=CARTESIAN_POINT('Ctrl Pts',(-38.61989814589,37.679870694817,15.1803409754971));
#54476=CARTESIAN_POINT('Ctrl Pts',(-38.5241845298854,37.7215404565648,15.1868803245583));
#54477=CARTESIAN_POINT('Ctrl Pts',(-38.4346334551116,37.7742886171168,15.1934196736194));
#54478=CARTESIAN_POINT('Origin',(-39.0658530619283,38.8697713466882,15.5));
#54479=CARTESIAN_POINT('',(-38.4337315549884,37.7763335227174,15.6934196736194));
#54480=CARTESIAN_POINT('',(-38.4323663903519,37.7745195378425,15.5565803263806));
#54481=CARTESIAN_POINT('',(-38.4336030619283,37.7746822236028,15.5));
#54482=CARTESIAN_POINT('Ctrl Pts',(-38.4323663903519,37.7745195378425,15.5565803263806));
#54483=CARTESIAN_POINT('Ctrl Pts',(-38.7313730076302,37.6052990985956,15.5349217833067));
#54484=CARTESIAN_POINT('Ctrl Pts',(-39.1034689296549,37.5582680121359,15.5132632402327));
#54485=CARTESIAN_POINT('Ctrl Pts',(-39.4315419163111,37.6572094658042,15.4916046971588));
#54486=CARTESIAN_POINT('Ctrl Pts',(-39.8279295706787,37.7767535073269,15.4654361936999));
#54487=CARTESIAN_POINT('Ctrl Pts',(-40.1600516656647,38.1093911753228,15.439267690241));
#54488=CARTESIAN_POINT('Ctrl Pts',(-40.2789807143,38.5059637820164,15.413099186782));
#54489=CARTESIAN_POINT('Ctrl Pts',(-40.3979097629354,38.9025363887101,15.3869306833231));
#54490=CARTESIAN_POINT('Ctrl Pts',(-40.3036457652202,39.3630439341015,15.3607621798642));
#54491=CARTESIAN_POINT('Ctrl Pts',(-40.0384578014032,39.6809893678464,15.3345936764052));
#54492=CARTESIAN_POINT('Ctrl Pts',(-39.7732698375861,39.9989348015912,15.3084251729463));
#54493=CARTESIAN_POINT('Ctrl Pts',(-39.3371579076672,40.1743181236895,15.2822566694874));
#54494=CARTESIAN_POINT('Ctrl Pts',(-38.9256798191233,40.1284953536109,15.2560881660285));
#54495=CARTESIAN_POINT('Ctrl Pts',(-38.5142017305794,40.0826725835323,15.2299196625695));
#54496=CARTESIAN_POINT('Ctrl Pts',(-38.1273574834104,39.8156437212769,15.2037511591106));
#54497=CARTESIAN_POINT('Ctrl Pts',(-37.938612567216,39.4471477114983,15.1775826556517));
#54498=CARTESIAN_POINT('Ctrl Pts',(-37.7498676510216,39.0786517017197,15.1514141521928));
#54499=CARTESIAN_POINT('Ctrl Pts',(-37.7592220658018,38.608688544418,15.1252456487338));
#54500=CARTESIAN_POINT('Ctrl Pts',(-37.9624813210464,38.2479952475117,15.0990771452749));
#54501=CARTESIAN_POINT('Ctrl Pts',(-38.0725101803872,38.0527437595402,15.0849115389768));
#54502=CARTESIAN_POINT('Ctrl Pts',(-38.239359037454,37.8895116538818,15.0707459326787));
#54503=CARTESIAN_POINT('Ctrl Pts',(-38.4347780105727,37.7761824162226,15.0565803263806));
#54504=CARTESIAN_POINT('Ctrl Pts',(-38.4346334551116,37.7742886171168,15.1934196736194));
#54505=CARTESIAN_POINT('Ctrl Pts',(-38.1658281265106,37.9326226925712,15.2130488280172));
#54506=CARTESIAN_POINT('Ctrl Pts',(-37.952548489957,38.1907752905067,15.232677982415));
#54507=CARTESIAN_POINT('Ctrl Pts',(-37.8586391249355,38.4867967233546,15.2523071368127));
#54508=CARTESIAN_POINT('Ctrl Pts',(-37.7334443512028,38.8814361322879,15.2784756402716));
#54509=CARTESIAN_POINT('Ctrl Pts',(-37.8204033568707,39.3433788684653,15.3046441437306));
#54510=CARTESIAN_POINT('Ctrl Pts',(-38.0805226988896,39.6654843197861,15.3308126471895));
#54511=CARTESIAN_POINT('Ctrl Pts',(-38.3406420409086,39.987589771107,15.3569811506484));
#54512=CARTESIAN_POINT('Ctrl Pts',(-38.7739217192785,40.1698579375712,15.3831496541074));
#54513=CARTESIAN_POINT('Ctrl Pts',(-39.1860739715826,40.1305576058447,15.4093181575663));
#54514=CARTESIAN_POINT('Ctrl Pts',(-39.5982262238866,40.0912572741182,15.4354866610252));
#54515=CARTESIAN_POINT('Ctrl Pts',(-39.9892510501248,39.8303884442009,15.4616551644841));
#54516=CARTESIAN_POINT('Ctrl Pts',(-40.1838082722999,39.4649278007734,15.4878236679431));
#54517=CARTESIAN_POINT('Ctrl Pts',(-40.378365494475,39.0994671573459,15.513992171402));
#54518=CARTESIAN_POINT('Ctrl Pts',(-40.3764551125872,38.6294147004082,15.5401606748609));
#54519=CARTESIAN_POINT('Ctrl Pts',(-40.1789337635325,38.2655475388609,15.5663291783198));
#54520=CARTESIAN_POINT('Ctrl Pts',(-39.9814124144779,37.9016803773136,15.5924976817788));
#54521=CARTESIAN_POINT('Ctrl Pts',(-39.5882800982565,37.6439985111567,15.6186661852377));
#54522=CARTESIAN_POINT('Ctrl Pts',(-39.1758220190741,37.6080495523,15.6448346886966));
#54523=CARTESIAN_POINT('Ctrl Pts',(-38.9205626180182,37.5858016920459,15.6610296836709));
#54524=CARTESIAN_POINT('Ctrl Pts',(-38.6579013630336,37.6484785302017,15.6772246786452));
#54525=CARTESIAN_POINT('Ctrl Pts',(-38.4337315549884,37.7763335227174,15.6934196736194));
#54526=CARTESIAN_POINT('Origin',(-39.0658530619283,38.8697713466882,15.5));
#54527=CARTESIAN_POINT('',(-38.4325272584341,37.7729978925048,16.1934196736194));
#54528=CARTESIAN_POINT('',(-38.4342758514651,37.7737507965446,16.0565803263806));
#54529=CARTESIAN_POINT('',(-38.4336030619283,37.7746822236028,15.5));
#54530=CARTESIAN_POINT('Ctrl Pts',(-38.4342758514651,37.7737507965446,16.0565803263806));
#54531=CARTESIAN_POINT('Ctrl Pts',(-38.5046440871601,37.732289208729,16.0514346408525));
#54532=CARTESIAN_POINT('Ctrl Pts',(-38.5788878157804,37.6977955005524,16.0462889553244));
#54533=CARTESIAN_POINT('Ctrl Pts',(-38.6559170964541,37.6714445317291,16.0411432697963));
#54534=CARTESIAN_POINT('Ctrl Pts',(-39.0476512952768,37.5374360667672,16.0149747663373));
#54535=CARTESIAN_POINT('Ctrl Pts',(-39.5114269646143,37.6140195799122,15.9888062628784));
#54536=CARTESIAN_POINT('Ctrl Pts',(-39.8392815814542,37.8668541135745,15.9626377594195));
#54537=CARTESIAN_POINT('Ctrl Pts',(-40.1671361982942,38.1196886472368,15.9364692559606));
#54538=CARTESIAN_POINT('Ctrl Pts',(-40.3590697626365,38.5487742014165,15.9103007525016));
#54539=CARTESIAN_POINT('Ctrl Pts',(-40.3290169828723,38.9617037131001,15.8841322490427));
#54540=CARTESIAN_POINT('Ctrl Pts',(-40.2989642031082,39.3746332247836,15.8579637455838));
#54541=CARTESIAN_POINT('Ctrl Pts',(-40.0469250792374,39.771406693971,15.8317952421249));
#54542=CARTESIAN_POINT('Ctrl Pts',(-39.6859169501041,39.974106180808,15.8056267386659));
#54543=CARTESIAN_POINT('Ctrl Pts',(-39.3249088209707,40.176805667645,15.779458235207));
#54544=CARTESIAN_POINT('Ctrl Pts',(-38.8549316865748,40.1854311721316,15.7532897317481));
#54545=CARTESIAN_POINT('Ctrl Pts',(-38.4867288810043,39.9961149153207,15.7271212282891));
#54546=CARTESIAN_POINT('Ctrl Pts',(-38.1185260754338,39.8067986585099,15.7009527248302));
#54547=CARTESIAN_POINT('Ctrl Pts',(-37.8520975986887,39.4195406404017,15.6747842213713));
#54548=CARTESIAN_POINT('Ctrl Pts',(-37.806913145733,39.0079919599958,15.6486157179124));
#54549=CARTESIAN_POINT('Ctrl Pts',(-37.7617286927774,38.5964432795898,15.6224472144534));
#54550=CARTESIAN_POINT('Ctrl Pts',(-37.9377882636113,38.1606039368861,15.5962787109945));
#54551=CARTESIAN_POINT('Ctrl Pts',(-38.2561446559028,37.8959094730591,15.5701102075356));
#54552=CARTESIAN_POINT('Ctrl Pts',(-38.3110111758702,37.8502912149167,15.5656002471506));
#54553=CARTESIAN_POINT('Ctrl Pts',(-38.3701042153675,37.8097563252262,15.5610902867656));
#54554=CARTESIAN_POINT('Ctrl Pts',(-38.4323663903519,37.7745195378425,15.5565803263806));
#54555=CARTESIAN_POINT('Ctrl Pts',(-38.4337315549884,37.7763335227174,15.6934196736194));
#54556=CARTESIAN_POINT('Ctrl Pts',(-38.2956790587637,37.8550716053588,15.7033931821041));
#54557=CARTESIAN_POINT('Ctrl Pts',(-38.1722247361697,37.9585289981308,15.7133666905887));
#54558=CARTESIAN_POINT('Ctrl Pts',(-38.0740874997393,38.0820936667169,15.7233401990734));
#54559=CARTESIAN_POINT('Ctrl Pts',(-37.8165949017303,38.4063027915471,15.7495087025323));
#54560=CARTESIAN_POINT('Ctrl Pts',(-37.7333935478559,38.868937092764,15.7756772059912));
#54561=CARTESIAN_POINT('Ctrl Pts',(-37.8617919143246,39.2625458504732,15.8018457094502));
#54562=CARTESIAN_POINT('Ctrl Pts',(-37.9901902807933,39.6561546081824,15.8280142129091));
#54563=CARTESIAN_POINT('Ctrl Pts',(-38.3301883676052,39.9807378223839,15.854182716368));
#54564=CARTESIAN_POINT('Ctrl Pts',(-38.7293269910635,40.0907485215641,15.880351219827));
#54565=CARTESIAN_POINT('Ctrl Pts',(-39.128465614522,40.2007592207442,15.9065197232859));
#54566=CARTESIAN_POINT('Ctrl Pts',(-39.5867447746269,40.0961974049031,15.9326882267448));
#54567=CARTESIAN_POINT('Ctrl Pts',(-39.898666648561,39.8239498351585,15.9588567302037));
#54568=CARTESIAN_POINT('Ctrl Pts',(-40.2105885224951,39.551702265414,15.9850252336627));
#54569=CARTESIAN_POINT('Ctrl Pts',(-40.3761531102584,39.1117689417661,16.0111937371216));
#54570=CARTESIAN_POINT('Ctrl Pts',(-40.3211192825961,38.701421195982,16.0373622405805));
#54571=CARTESIAN_POINT('Ctrl Pts',(-40.2660854549337,38.291073450198,16.0635307440394));
#54572=CARTESIAN_POINT('Ctrl Pts',(-39.9904532118458,37.9103112822778,16.0896992474984));
#54573=CARTESIAN_POINT('Ctrl Pts',(-39.617819327633,37.7298729742913,16.1158677509573));
#54574=CARTESIAN_POINT('Ctrl Pts',(-39.249711738356,37.5516264074058,16.1417183918447));
#54575=CARTESIAN_POINT('Ctrl Pts',(-38.7869447075706,37.5688666846833,16.167569032732));
#54576=CARTESIAN_POINT('Ctrl Pts',(-38.4325272584341,37.7729978925048,16.1934196736194));
#54577=CARTESIAN_POINT('Origin',(-39.0658530619283,38.8697713466882,15.5));
#54578=CARTESIAN_POINT('',(-38.4349705604869,37.7753960169021,16.6934196736194));
#54579=CARTESIAN_POINT('',(-38.4341423505256,37.7764525809616,16.5565803263806));
#54580=CARTESIAN_POINT('',(-38.4336030619283,37.7746822236028,15.5));
#54581=CARTESIAN_POINT('Ctrl Pts',(-38.4341423505256,37.7764525809616,16.5565803263806));
#54582=CARTESIAN_POINT('Ctrl Pts',(-38.6388834301988,37.6590722267018,16.5417789949394));
#54583=CARTESIAN_POINT('Ctrl Pts',(-38.8753711836181,37.5959619576061,16.5269776634982));
#54584=CARTESIAN_POINT('Ctrl Pts',(-39.1094100531277,37.604015667637,16.5121763320569));
#54585=CARTESIAN_POINT('Ctrl Pts',(-39.5231868130501,37.6182544906534,16.486007828598));
#54586=CARTESIAN_POINT('Ctrl Pts',(-39.929308939441,37.8549351283607,16.4598393251391));
#54587=CARTESIAN_POINT('Ctrl Pts',(-40.1456664429884,38.2079271704546,16.4336708216802));
#54588=CARTESIAN_POINT('Ctrl Pts',(-40.3620239465357,38.5609192125485,16.4075023182212));
#54589=CARTESIAN_POINT('Ctrl Pts',(-40.3886168272394,39.0302226590291,16.3813338147623));
#54590=CARTESIAN_POINT('Ctrl Pts',(-40.2135205214552,39.4053962654636,16.3551653113034));
#54591=CARTESIAN_POINT('Ctrl Pts',(-40.0384242156709,39.780569871898,16.3289968078445));
#54592=CARTESIAN_POINT('Ctrl Pts',(-39.6616387233988,40.0616136382864,16.3028283043855));
#54593=CARTESIAN_POINT('Ctrl Pts',(-39.2521191380692,40.122504199314,16.2766598009266));
#54594=CARTESIAN_POINT('Ctrl Pts',(-38.8425995527396,40.1833947603415,16.2504912974677));
#54595=CARTESIAN_POINT('Ctrl Pts',(-38.4003458743526,40.0241321160083,16.2243227940087));
#54596=CARTESIAN_POINT('Ctrl Pts',(-38.1236699093341,39.7161315290339,16.1981542905498));
#54597=CARTESIAN_POINT('Ctrl Pts',(-37.8469939443156,39.4081309420595,16.1719857870909));
#54598=CARTESIAN_POINT('Ctrl Pts',(-37.7358956926656,38.951392412444,16.145817283632));
#54599=CARTESIAN_POINT('Ctrl Pts',(-37.8401929309945,38.5507229261018,16.119648780173));
#54600=CARTESIAN_POINT('Ctrl Pts',(-37.9239815150654,38.2288397249847,16.0986259622422));
#54601=CARTESIAN_POINT('Ctrl Pts',(-38.1467847875343,37.9431430780994,16.0776031443114));
#54602=CARTESIAN_POINT('Ctrl Pts',(-38.4342758514651,37.7737507965446,16.0565803263806));
#54603=CARTESIAN_POINT('Ctrl Pts',(-38.4325272584341,37.7729978925048,16.1934196736194));
#54604=CARTESIAN_POINT('Ctrl Pts',(-38.4281692990986,37.775507914246,16.193737536191));
#54605=CARTESIAN_POINT('Ctrl Pts',(-38.42382772163,37.7780461928786,16.1940553987625));
#54606=CARTESIAN_POINT('Ctrl Pts',(-38.4195029034438,37.7806127124219,16.1943732613341));
#54607=CARTESIAN_POINT('Ctrl Pts',(-38.063455888805,37.9919052065918,16.220541764793));
#54608=CARTESIAN_POINT('Ctrl Pts',(-37.820997384865,38.3946046429843,16.2467102682519));
#54609=CARTESIAN_POINT('Ctrl Pts',(-37.8008486672723,38.8081358071838,16.2728787717109));
#54610=CARTESIAN_POINT('Ctrl Pts',(-37.7806999496796,39.2216669713833,16.2990472751698));
#54611=CARTESIAN_POINT('Ctrl Pts',(-37.9828610184341,39.6460298633898,16.3252157786287));
#54612=CARTESIAN_POINT('Ctrl Pts',(-38.3166804464026,39.8909351187555,16.3513842820876));
#54613=CARTESIAN_POINT('Ctrl Pts',(-38.6504998743712,40.1358403741212,16.3775527855465));
#54614=CARTESIAN_POINT('Ctrl Pts',(-39.1159776615536,40.2012879928461,16.4037212890055));
#54615=CARTESIAN_POINT('Ctrl Pts',(-39.5043880368528,40.0579304834052,16.4298897924644));
#54616=CARTESIAN_POINT('Ctrl Pts',(-39.8927984121519,39.9145729739643,16.4560582959233));
#54617=CARTESIAN_POINT('Ctrl Pts',(-40.2041413755678,39.5624103363577,16.4822267993823));
#54618=CARTESIAN_POINT('Ctrl Pts',(-40.2988070379275,39.1593564860685,16.5083953028412));
#54619=CARTESIAN_POINT('Ctrl Pts',(-40.3934727002873,38.7563026357793,16.5345638063001));
#54620=CARTESIAN_POINT('Ctrl Pts',(-40.271461061591,38.3023575728075,16.560732309759));
#54621=CARTESIAN_POINT('Ctrl Pts',(-39.9874835980573,38.001075653904,16.586900813218));
#54622=CARTESIAN_POINT('Ctrl Pts',(-39.7035061345237,37.6997937350004,16.6130693166769));
#54623=CARTESIAN_POINT('Ctrl Pts',(-39.2575628461526,37.5511749601651,16.6392378201358));
#54624=CARTESIAN_POINT('Ctrl Pts',(-38.849619989904,37.6218617656895,16.6654063235947));
#54625=CARTESIAN_POINT('Ctrl Pts',(-38.7040525518056,37.6470851444788,16.6747441069363));
#54626=CARTESIAN_POINT('Ctrl Pts',(-38.5633236984099,37.7002326432607,16.6840818902779));
#54627=CARTESIAN_POINT('Ctrl Pts',(-38.4349705604869,37.7753960169021,16.6934196736194));
#54628=CARTESIAN_POINT('Origin',(-39.0658530619283,38.8697713466882,15.5));
#54629=CARTESIAN_POINT('',(-38.4329072841441,37.7756148875603,17.1934196736194));
#54630=CARTESIAN_POINT('',(-38.4323100738575,37.7733715239653,17.0565803263806));
#54631=CARTESIAN_POINT('',(-38.4336030619283,37.7746822236028,15.5));
#54632=CARTESIAN_POINT('Ctrl Pts',(-38.4323100738575,37.7733715239653,17.0565803263806));
#54633=CARTESIAN_POINT('Ctrl Pts',(-38.7684978446967,37.5814140598882,17.0321233490263));
#54634=CARTESIAN_POINT('Ctrl Pts',(-39.2005574419278,37.5523442127138,17.0076663716719));
#54635=CARTESIAN_POINT('Ctrl Pts',(-39.5571950289671,37.7024591900708,16.9832093943176));
#54636=CARTESIAN_POINT('Ctrl Pts',(-39.9387905055794,37.8630793782195,16.9570408908587));
#54637=CARTESIAN_POINT('Ctrl Pts',(-40.2340383736987,38.2288410235792,16.9308723873998));
#54638=CARTESIAN_POINT('Ctrl Pts',(-40.3105459562687,38.6357323277609,16.9047038839408));
#54639=CARTESIAN_POINT('Ctrl Pts',(-40.3870535388386,39.0426236319427,16.8785353804819));
#54640=CARTESIAN_POINT('Ctrl Pts',(-40.2448208358592,39.4906445949467,16.852366877023));
#54641=CARTESIAN_POINT('Ctrl Pts',(-39.9476266935978,39.7788972563362,16.8261983735641));
#54642=CARTESIAN_POINT('Ctrl Pts',(-39.6504325513363,40.0671499177256,16.8000298701051));
#54643=CARTESIAN_POINT('Ctrl Pts',(-39.1982769697929,40.1956342775006,16.7738613666462));
#54644=CARTESIAN_POINT('Ctrl Pts',(-38.7939118807236,40.106736438769,16.7476928631873));
#54645=CARTESIAN_POINT('Ctrl Pts',(-38.3895467916544,40.0178386000373,16.7215243597283));
#54646=CARTESIAN_POINT('Ctrl Pts',(-38.0329721950595,39.711558562799,16.6953558562694));
#54647=CARTESIAN_POINT('Ctrl Pts',(-37.8840803814008,39.3252359279146,16.6691873528105));
#54648=CARTESIAN_POINT('Ctrl Pts',(-37.7351885677422,38.9389132930302,16.6430188493516));
#54649=CARTESIAN_POINT('Ctrl Pts',(-37.7939795370199,38.4725480604996,16.6168503458926));
#54650=CARTESIAN_POINT('Ctrl Pts',(-38.0340907183856,38.1352639483972,16.5906818424337));
#54651=CARTESIAN_POINT('Ctrl Pts',(-38.1383911078307,37.9887532193016,16.579314670416));
#54652=CARTESIAN_POINT('Ctrl Pts',(-38.2769046668091,37.8665987062389,16.5679474983983));
#54653=CARTESIAN_POINT('Ctrl Pts',(-38.4341423505256,37.7764525809616,16.5565803263806));
#54654=CARTESIAN_POINT('Ctrl Pts',(-38.4349705604869,37.7753960169021,16.6934196736194));
#54655=CARTESIAN_POINT('Ctrl Pts',(-38.2036227489616,37.9108728917195,16.7102503937368));
#54656=CARTESIAN_POINT('Ctrl Pts',(-38.0124806835606,38.1178740898994,16.7270811138542));
#54657=CARTESIAN_POINT('Ctrl Pts',(-37.9056793271332,38.3618028680121,16.7439118339715));
#54658=CARTESIAN_POINT('Ctrl Pts',(-37.7396239447374,38.7410647789261,16.7700803374305));
#54659=CARTESIAN_POINT('Ctrl Pts',(-37.7774556040718,39.2095962148701,16.7962488408894));
#54660=CARTESIAN_POINT('Ctrl Pts',(-38.0022100801908,39.5573021560724,16.8224173443483));
#54661=CARTESIAN_POINT('Ctrl Pts',(-38.2269645563097,39.9050080972747,16.8485858478072));
#54662=CARTESIAN_POINT('Ctrl Pts',(-38.6386418492131,40.1318885437353,16.8747543512662));
#54663=CARTESIAN_POINT('Ctrl Pts',(-39.0526410872976,40.1362075141882,16.9009228547251));
#54664=CARTESIAN_POINT('Ctrl Pts',(-39.4666403253822,40.1405264846412,16.927091358184));
#54665=CARTESIAN_POINT('Ctrl Pts',(-39.8829615086478,39.9222839790863,16.9532598616429));
#54666=CARTESIAN_POINT('Ctrl Pts',(-40.1149210262726,39.5793427181871,16.9794283651019));
#54667=CARTESIAN_POINT('Ctrl Pts',(-40.3468805438973,39.2364014572879,17.0055968685608));
#54668=CARTESIAN_POINT('Ctrl Pts',(-40.3944783958811,38.7687614410443,17.0317653720197));
#54669=CARTESIAN_POINT('Ctrl Pts',(-40.236371633473,38.3861176323113,17.0579338754786));
#54670=CARTESIAN_POINT('Ctrl Pts',(-40.0782648710649,38.0034738235784,17.0841023789376));
#54671=CARTESIAN_POINT('Ctrl Pts',(-39.714453494265,37.7058262223561,17.1102708823965));
#54672=CARTESIAN_POINT('Ctrl Pts',(-39.3080738473792,37.6266443201347,17.1364393858554));
#54673=CARTESIAN_POINT('Ctrl Pts',(-39.0131183836182,37.5691730986546,17.1554328151101));
#54674=CARTESIAN_POINT('Ctrl Pts',(-38.6957377885278,37.6267904626672,17.1744262443648));
#54675=CARTESIAN_POINT('Ctrl Pts',(-38.4329072841441,37.7756148875603,17.1934196736194));
#54676=CARTESIAN_POINT('Origin',(-39.0658530619283,38.8697713466882,15.5));
#54677=CARTESIAN_POINT('',(-38.4333577759012,37.7730251466967,17.6934196736194));
#54678=CARTESIAN_POINT('',(-38.4348713855213,37.7748596688486,17.5565803263806));
#54679=CARTESIAN_POINT('',(-38.4336030619283,37.7746822236028,15.5));
#54680=CARTESIAN_POINT('',(-40.2595650866584,39.2869186252538,18.));
#54681=CARTESIAN_POINT('Ctrl Pts',(-38.4333577759012,37.7730251466967,17.6934196736194));
#54682=CARTESIAN_POINT('Ctrl Pts',(-38.1097262681979,37.9625959827323,17.7171076053695));
#54683=CARTESIAN_POINT('Ctrl Pts',(-37.8720798795257,38.3048233518517,17.7407955371196));
#54684=CARTESIAN_POINT('Ctrl Pts',(-37.814449821825,38.6752097670202,17.7644834688697));
#54685=CARTESIAN_POINT('Ctrl Pts',(-37.7507848138289,39.0843826018939,17.7906519723286));
#54686=CARTESIAN_POINT('Ctrl Pts',(-37.9068123877648,39.5279208384947,17.8168204757875));
#54687=CARTESIAN_POINT('Ctrl Pts',(-38.2131597275407,39.8064869141386,17.8429889792464));
#54688=CARTESIAN_POINT('Ctrl Pts',(-38.5195070673165,40.0850529897826,17.8691574827054));
#54689=CARTESIAN_POINT('Ctrl Pts',(-38.9761741729324,40.1986469044696,17.8953259861643));
#54690=CARTESIAN_POINT('Ctrl Pts',(-39.3768946753638,40.0972493078634,17.9214944896232));
#54691=CARTESIAN_POINT('Ctrl Pts',(-39.7776151777952,39.9958517112573,17.9476629930821));
#54692=CARTESIAN_POINT('Ctrl Pts',(-40.1223890770422,39.6794626033579,17.9738314965411));
#54693=CARTESIAN_POINT('Ctrl Pts',(-40.2595650866584,39.2869186252538,18.));
#54694=CARTESIAN_POINT('',(-39.301526156426,37.6253017999342,18.));
#54695=CARTESIAN_POINT('Origin',(-39.0658530619283,38.8697713466882,18.));
#54696=CARTESIAN_POINT('Ctrl Pts',(-39.301526596644,37.6252897660473,18.));
#54697=CARTESIAN_POINT('Ctrl Pts',(-39.6885864653113,37.7000302410441,17.975091839613));
#54698=CARTESIAN_POINT('Ctrl Pts',(-40.03994654915,37.9695057059561,17.950183679226));
#54699=CARTESIAN_POINT('Ctrl Pts',(-40.2093266637559,38.3254078043634,17.925275518839));
#54700=CARTESIAN_POINT('Ctrl Pts',(-40.3872773452222,38.6993184082981,17.89910701538));
#54701=CARTESIAN_POINT('Ctrl Pts',(-40.3643659014498,39.1686232325653,17.8729385119211));
#54702=CARTESIAN_POINT('Ctrl Pts',(-40.1507520928544,39.5232247114421,17.8467700084622));
#54703=CARTESIAN_POINT('Ctrl Pts',(-39.9371382842589,39.8778261903188,17.8206015050033));
#54704=CARTESIAN_POINT('Ctrl Pts',(-39.5328221108402,40.1177243238052,17.7944330015443));
#54705=CARTESIAN_POINT('Ctrl Pts',(-39.1191596128741,40.1351764464735,17.7682644980854));
#54706=CARTESIAN_POINT('Ctrl Pts',(-38.705497114908,40.1526285691419,17.7420959946265));
#54707=CARTESIAN_POINT('Ctrl Pts',(-38.2824882923945,39.9476346809922,17.7159274911676));
#54708=CARTESIAN_POINT('Ctrl Pts',(-38.0397877964566,39.6122000494563,17.6897589877086));
#54709=CARTESIAN_POINT('Ctrl Pts',(-37.7970873005187,39.2767654179205,17.6635904842497));
#54710=CARTESIAN_POINT('Ctrl Pts',(-37.7346951311565,38.8108900429983,17.6374219807908));
#54711=CARTESIAN_POINT('Ctrl Pts',(-37.8806022560883,38.4234367664048,17.6112534773319));
#54712=CARTESIAN_POINT('Ctrl Pts',(-37.9822155342897,38.1536048606431,17.5930290936814));
#54713=CARTESIAN_POINT('Ctrl Pts',(-38.184855409418,37.9218082144096,17.574804710031));
#54714=CARTESIAN_POINT('Ctrl Pts',(-38.4348713855213,37.7748596688486,17.5565803263806));
#54715=CARTESIAN_POINT('Origin',(-39.0658530619283,38.8697713466882,19.1042117235887));
#54716=CARTESIAN_POINT('',(-38.2940340733258,37.531419596366,14.3957882764113));
#54717=CARTESIAN_POINT('',(-38.2954995370357,37.5355989289914,14.3542117235887));
#54718=CARTESIAN_POINT('',(-38.2943530619284,37.5334941486488,19.1042117235887));
#54719=CARTESIAN_POINT('',(-37.9741697098829,39.9602191716055,14.));
#54720=CARTESIAN_POINT('Ctrl Pts',(-38.2954995370357,37.5355989289914,14.3542117235887));
#54721=CARTESIAN_POINT('Ctrl Pts',(-38.5213873438296,37.4053726489247,14.3408151628949));
#54722=CARTESIAN_POINT('Ctrl Pts',(-39.2812420752165,37.1810251467921,14.301250098742));
#54723=CARTESIAN_POINT('Ctrl Pts',(-40.5621358440549,37.8394569175814,14.2355165311304));
#54724=CARTESIAN_POINT('Ctrl Pts',(-40.7517455388365,39.5501918673983,14.1570110207535));
#54725=CARTESIAN_POINT('Ctrl Pts',(-39.4258164610498,40.6499822516744,14.0785055103768));
#54726=CARTESIAN_POINT('Ctrl Pts',(-38.3327559670706,40.3192117233802,14.0261685034589));
#54727=CARTESIAN_POINT('Ctrl Pts',(-37.9741697098829,39.9602191716055,14.));
#54728=CARTESIAN_POINT('',(-37.5730942570913,39.2702598116582,14.));
#54729=CARTESIAN_POINT('Origin',(-39.0658530619283,38.8697713466882,14.));
#54730=CARTESIAN_POINT('Ctrl Pts',(-38.2940340733258,37.531419596366,14.3957882764113));
#54731=CARTESIAN_POINT('Ctrl Pts',(-38.33317399173,37.5085041378475,14.3934410251636));
#54732=CARTESIAN_POINT('Ctrl Pts',(-38.8212071098194,37.2523822679137,14.3649252704569));
#54733=CARTESIAN_POINT('Ctrl Pts',(-40.0177412802272,37.3220721610693,14.3102410122914));
#54734=CARTESIAN_POINT('Ctrl Pts',(-40.8820235552812,38.8100518816852,14.2317355019146));
#54735=CARTESIAN_POINT('Ctrl Pts',(-40.1171224362185,40.3517547545305,14.1532299915378));
#54736=CARTESIAN_POINT('Ctrl Pts',(-38.4376290919279,40.5606360835951,14.0759848242329));
#54737=CARTESIAN_POINT('Ctrl Pts',(-37.6993939872544,39.7344135992461,14.024908160387));
#54738=CARTESIAN_POINT('Ctrl Pts',(-37.573079654256,39.2702614469549,14.));
#54739=CARTESIAN_POINT('Origin',(-39.0658530619283,38.8697713466882,19.1042117235887));
#54740=CARTESIAN_POINT('',(-38.2957867873204,37.5353247514265,14.8957882764113));
#54741=CARTESIAN_POINT('',(-38.2927144236218,37.5325537808421,14.8542117235887));
#54742=CARTESIAN_POINT('',(-38.2943530619284,37.5334941486488,19.1042117235887));
#54743=CARTESIAN_POINT('Ctrl Pts',(-38.2927144236218,37.5325537808421,14.8542117235887));
#54744=CARTESIAN_POINT('Ctrl Pts',(-38.6802974716782,37.3125317216241,14.8311595169817));
#54745=CARTESIAN_POINT('Ctrl Pts',(-39.7267977629897,37.2108801077358,14.7819388069158));
#54746=CARTESIAN_POINT('Ctrl Pts',(-40.8313162888141,38.4399409113082,14.706549593391));
#54747=CARTESIAN_POINT('Ctrl Pts',(-40.3982068515902,40.1052936742774,14.6280440830142));
#54748=CARTESIAN_POINT('Ctrl Pts',(-38.7701602990205,40.6625900679474,14.5495385726375));
#54749=CARTESIAN_POINT('Ctrl Pts',(-37.4074005907986,39.6120654537968,14.4710330622607));
#54750=CARTESIAN_POINT('Ctrl Pts',(-37.5105490854526,38.1886638489126,14.4059241125778));
#54751=CARTESIAN_POINT('Ctrl Pts',(-38.0801438046488,37.6597533768028,14.3669836663538));
#54752=CARTESIAN_POINT('Ctrl Pts',(-38.2954995370357,37.5355989289914,14.3542117235887));
#54753=CARTESIAN_POINT('Ctrl Pts',(-38.2957867873204,37.5353247514265,14.8957882764113));
#54754=CARTESIAN_POINT('Ctrl Pts',(-38.4978395239631,37.4181483982544,14.8837853792505));
#54755=CARTESIAN_POINT('Ctrl Pts',(-39.2200040297691,37.1845419759791,14.8456139786307));
#54756=CARTESIAN_POINT('Ctrl Pts',(-40.5064460859517,37.7623754838001,14.781274074552));
#54757=CARTESIAN_POINT('Ctrl Pts',(-40.7841666383236,39.4605673674226,14.7027685641753));
#54758=CARTESIAN_POINT('Ctrl Pts',(-39.5208569909583,40.6289217126118,14.6242630537985));
#54759=CARTESIAN_POINT('Ctrl Pts',(-37.8495006293028,40.2196233657655,14.5457575434217));
#54760=CARTESIAN_POINT('Ctrl Pts',(-37.2863317343909,38.6481881568849,14.4695992842926));
#54761=CARTESIAN_POINT('Ctrl Pts',(-37.8968197279324,37.7639788153404,14.4196095286225));
#54762=CARTESIAN_POINT('Ctrl Pts',(-38.2940340733258,37.531419596366,14.3957882764113));
#54763=CARTESIAN_POINT('Origin',(-39.0658530619283,38.8697713466882,19.1042117235887));
#54764=CARTESIAN_POINT('',(-38.2928440194275,37.5332956321379,15.3957882764113));
#54765=CARTESIAN_POINT('',(-38.2956103942192,37.5330138522408,15.3542117235887));
#54766=CARTESIAN_POINT('',(-38.2943530619284,37.5334941486488,19.1042117235887));
#54767=CARTESIAN_POINT('Ctrl Pts',(-38.2956103942192,37.5330138522408,15.3542117235887));
#54768=CARTESIAN_POINT('Ctrl Pts',(-38.4048846594434,37.4686481648294,15.3476723745276));
#54769=CARTESIAN_POINT('Ctrl Pts',(-38.9890534180561,37.2143251749767,15.3149645220075));
#54770=CARTESIAN_POINT('Ctrl Pts',(-40.2495149974676,37.4911553124801,15.2560881660285));
#54771=CARTESIAN_POINT('Ctrl Pts',(-40.8686733596744,39.0966551680435,15.1775826556517));
#54772=CARTESIAN_POINT('Ctrl Pts',(-39.8710199775172,40.4986802936762,15.0990771452749));
#54773=CARTESIAN_POINT('Ctrl Pts',(-38.151273037136,40.4398609986214,15.0205716348981));
#54774=CARTESIAN_POINT('Ctrl Pts',(-37.2517446794564,38.9729482851087,14.9420661245214));
#54775=CARTESIAN_POINT('Ctrl Pts',(-37.765555298795,37.8714157983081,14.8866128207515));
#54776=CARTESIAN_POINT('Ctrl Pts',(-38.2403192732087,37.5622973130857,14.8573280204407));
#54777=CARTESIAN_POINT('Ctrl Pts',(-38.2927144236218,37.5325537808421,14.8542117235887));
#54778=CARTESIAN_POINT('Ctrl Pts',(-38.2928440194275,37.5332956321379,15.3957882764113));
#54779=CARTESIAN_POINT('Ctrl Pts',(-38.6577053958295,37.3268052108187,15.3741297333373));
#54780=CARTESIAN_POINT('Ctrl Pts',(-39.6603483962762,37.2000760884311,15.3263026868045));
#54781=CARTESIAN_POINT('Ctrl Pts',(-40.8063139857151,38.3478206288557,15.2523071368127));
#54782=CARTESIAN_POINT('Ctrl Pts',(-40.4612384258706,40.0336169338117,15.1738016264359));
#54783=CARTESIAN_POINT('Ctrl Pts',(-38.8647480157521,40.6756488816116,15.0952961160592));
#54784=CARTESIAN_POINT('Ctrl Pts',(-37.4486135593306,39.6981268544225,15.0167906056824));
#54785=CARTESIAN_POINT('Ctrl Pts',(-37.4776219436003,38.2407538193379,14.9502879924664));
#54786=CARTESIAN_POINT('Ctrl Pts',(-38.0573277319451,37.6736142047346,14.9099538827094));
#54787=CARTESIAN_POINT('Ctrl Pts',(-38.2957867873204,37.5353247514265,14.8957882764113));
#54788=CARTESIAN_POINT('Origin',(-39.0658530619283,38.8697713466882,19.1042117235887));
#54789=CARTESIAN_POINT('',(-38.2951740301017,37.5323575792927,15.8957882764113));
#54790=CARTESIAN_POINT('',(-38.2945098549625,37.5355091383948,15.8542117235887));
#54791=CARTESIAN_POINT('',(-38.2943530619284,37.5334941486488,19.1042117235887));
#54792=CARTESIAN_POINT('Ctrl Pts',(-38.2945098549625,37.5355091383948,15.8542117235887));
#54793=CARTESIAN_POINT('Ctrl Pts',(-38.5680519773933,37.379494703083,15.8380167286145));
#54794=CARTESIAN_POINT('Ctrl Pts',(-39.406457455491,37.1794324424244,15.7956532301813));
#54795=CARTESIAN_POINT('Ctrl Pts',(-40.6627777316899,38.0028980795747,15.7271212282892));
#54796=CARTESIAN_POINT('Ctrl Pts',(-40.6697711344255,39.7236357807725,15.6486157179124));
#54797=CARTESIAN_POINT('Ctrl Pts',(-39.2383326839261,40.6786075590939,15.5701102075356));
#54798=CARTESIAN_POINT('Ctrl Pts',(-37.6522103975089,40.0113720173278,15.4916046971588));
#54799=CARTESIAN_POINT('Ctrl Pts',(-37.3603930477839,38.4611828913061,15.4196385358432));
#54800=CARTESIAN_POINT('Ctrl Pts',(-37.9676019940363,37.7262202408736,15.3738408779865));
#54801=CARTESIAN_POINT('Ctrl Pts',(-38.2956103942192,37.5330138522408,15.3542117235887));
#54802=CARTESIAN_POINT('Ctrl Pts',(-38.2951740301017,37.5323575792927,15.8957882764113));
#54803=CARTESIAN_POINT('Ctrl Pts',(-38.3810405288581,37.4817642775928,15.8906425908832));
#54804=CARTESIAN_POINT('Ctrl Pts',(-38.9323618573136,37.2256198547756,15.8593284018961));
#54805=CARTESIAN_POINT('Ctrl Pts',(-40.1754824724718,37.4308969968639,15.8018457094502));
#54806=CARTESIAN_POINT('Ctrl Pts',(-40.8781004790679,39.0016657040982,15.7233401990734));
#54807=CARTESIAN_POINT('Ctrl Pts',(-39.9554519188483,40.454148415738,15.6448346886966));
#54808=CARTESIAN_POINT('Ctrl Pts',(-38.2349899535507,40.4857241059463,15.5663291783198));
#54809=CARTESIAN_POINT('Ctrl Pts',(-37.2596657788943,39.0680749435715,15.4878236679431));
#54810=CARTESIAN_POINT('Ctrl Pts',(-37.726362925197,37.9127558858067,15.4309767006402));
#54811=CARTESIAN_POINT('Ctrl Pts',(-38.2168689019889,37.5762931512624,15.4002982367963));
#54812=CARTESIAN_POINT('Ctrl Pts',(-38.2928440194275,37.5332956321379,15.3957882764113));
#54813=CARTESIAN_POINT('Origin',(-39.0658530619283,38.8697713466882,19.1042117235887));
#54814=CARTESIAN_POINT('',(-38.295011126227,37.5356544186406,16.3957882764113));
#54815=CARTESIAN_POINT('',(-38.2930403179255,37.531438851785,16.3542117235887));
#54816=CARTESIAN_POINT('',(-38.2943530619284,37.5334941486488,19.1042117235887));
#54817=CARTESIAN_POINT('Ctrl Pts',(-38.2930403179255,37.531438851785,16.3542117235887));
#54818=CARTESIAN_POINT('Ctrl Pts',(-38.7255164935029,37.2823487342141,16.3283610827013));
#54819=CARTESIAN_POINT('Ctrl Pts',(-39.8618384352914,37.240015326582,16.276341938355));
#54820=CARTESIAN_POINT('Ctrl Pts',(-40.8667697353107,38.628241232664,16.1981542905498));
#54821=CARTESIAN_POINT('Ctrl Pts',(-40.2606815765474,40.2387207543455,16.119648780173));
#54822=CARTESIAN_POINT('Ctrl Pts',(-38.5830428006473,40.6214939022527,16.0411432697963));
#54823=CARTESIAN_POINT('Ctrl Pts',(-37.3383997450109,39.4332806175246,15.9626377594195));
#54824=CARTESIAN_POINT('Ctrl Pts',(-37.5801461044556,38.0890698220828,15.900327244017));
#54825=CARTESIAN_POINT('Ctrl Pts',(-38.1260519651447,37.6315889023455,15.8641852320734));
#54826=CARTESIAN_POINT('Ctrl Pts',(-38.2945098549625,37.5355091383948,15.8542117235887));
#54827=CARTESIAN_POINT('Ctrl Pts',(-38.295011126227,37.5356544186406,16.3957882764113));
#54828=CARTESIAN_POINT('Ctrl Pts',(-38.544845436971,37.3924216099234,16.3809869449701));
#54829=CARTESIAN_POINT('Ctrl Pts',(-39.3436107151108,37.1792592329343,16.3400171100699));
#54830=CARTESIAN_POINT('Ctrl Pts',(-40.6150494715949,37.9202307686755,16.2728787717109));
#54831=CARTESIAN_POINT('Ctrl Pts',(-40.7123989731982,39.6382265407265,16.1943732613341));
#54832=CARTESIAN_POINT('Ctrl Pts',(-39.333086957597,40.6670534245635,16.1158677509573));
#54833=CARTESIAN_POINT('Ctrl Pts',(-37.7141132310224,40.0840350136354,16.0373622405805));
#54834=CARTESIAN_POINT('Ctrl Pts',(-37.3340693749042,38.521628139946,15.9640024157318));
#54835=CARTESIAN_POINT('Ctrl Pts',(-37.9443644518928,37.7390576903556,15.9168110943421));
#54836=CARTESIAN_POINT('Ctrl Pts',(-38.2951740301017,37.5323575792927,15.8957882764113));
#54837=CARTESIAN_POINT('Origin',(-39.0658530619283,38.8697713466882,19.1042117235887));
#54838=CARTESIAN_POINT('',(-38.2927752994979,37.5318947737649,16.8957882764113));
#54839=CARTESIAN_POINT('',(-38.2960217454206,37.5343651514648,16.8542117235887));
#54840=CARTESIAN_POINT('',(-38.2943530619284,37.5334941486488,19.1042117235887));
#54841=CARTESIAN_POINT('Ctrl Pts',(-38.2960217454206,37.5343651514648,16.8542117235887));
#54842=CARTESIAN_POINT('Ctrl Pts',(-38.4526440402526,37.4426474088561,16.8448739402472));
#54843=CARTESIAN_POINT('Ctrl Pts',(-39.1056117500068,37.1960483659351,16.8093676534467));
#54844=CARTESIAN_POINT('Ctrl Pts',(-40.3881062726607,37.6234631732891,16.7476928631873));
#54845=CARTESIAN_POINT('Ctrl Pts',(-40.834758606014,39.2852359660895,16.6691873528105));
#54846=CARTESIAN_POINT('Ctrl Pts',(-39.6950143769496,40.5744102242793,16.5906818424337));
#54847=CARTESIAN_POINT('Ctrl Pts',(-37.9910233315818,40.3348238050802,16.5121763320569));
#54848=CARTESIAN_POINT('Ctrl Pts',(-37.250965136829,38.7813435147693,16.4336708216802));
#54849=CARTESIAN_POINT('Ctrl Pts',(-37.8462764933252,37.7925906195586,16.3810159521908));
#54850=CARTESIAN_POINT('Ctrl Pts',(-38.2877225391555,37.5345016936567,16.3545295861603));
#54851=CARTESIAN_POINT('Ctrl Pts',(-38.2930403179255,37.531438851785,16.3542117235887));
#54852=CARTESIAN_POINT('Ctrl Pts',(-38.2927752994979,37.5318947737649,16.8957882764113));
#54853=CARTESIAN_POINT('Ctrl Pts',(-38.7030067984342,37.2976596080307,16.871331299057));
#54854=CARTESIAN_POINT('Ctrl Pts',(-39.7943393979825,37.2242325343385,16.8207058182437));
#54855=CARTESIAN_POINT('Ctrl Pts',(-40.8516003110939,38.5339981005298,16.7439118339715));
#54856=CARTESIAN_POINT('Ctrl Pts',(-40.3309240105073,40.1740843304588,16.6654063235948));
#54857=CARTESIAN_POINT('Ctrl Pts',(-38.6757020358417,40.644431583443,16.586900813218));
#54858=CARTESIAN_POINT('Ctrl Pts',(-37.3703767628973,39.5232213878114,16.5083953028412));
#54859=CARTESIAN_POINT('Ctrl Pts',(-37.5450179797371,38.1378625018882,16.4446911239056));
#54860=CARTESIAN_POINT('Ctrl Pts',(-38.1031426043017,37.6456547913594,16.407155448429));
#54861=CARTESIAN_POINT('Ctrl Pts',(-38.295011126227,37.5356544186406,16.3957882764113));
#54862=CARTESIAN_POINT('Origin',(-39.0658530619283,38.8697713466882,19.1042117235887));
#54863=CARTESIAN_POINT('',(-38.2959007276492,37.5337106753505,17.3957882764113));
#54864=CARTESIAN_POINT('',(-38.2935040424574,37.5346322273253,17.3542117235887));
#54865=CARTESIAN_POINT('',(-38.2943530619284,37.5334941486488,19.1042117235887));
#54866=CARTESIAN_POINT('Ctrl Pts',(-38.2935040424574,37.5346322273253,17.3542117235887));
#54867=CARTESIAN_POINT('Ctrl Pts',(-38.6142216923301,37.353029943727,17.3352182943341));
#54868=CARTESIAN_POINT('Ctrl Pts',(-39.5350880316607,37.1858556050909,17.2900563616205));
#54869=CARTESIAN_POINT('Ctrl Pts',(-40.7451827384013,38.1758790339381,17.218725925448));
#54870=CARTESIAN_POINT('Ctrl Pts',(-40.5709395934168,39.8877854279213,17.1402204150712));
#54871=CARTESIAN_POINT('Ctrl Pts',(-39.0468978715213,40.6867135087542,17.0617149046944));
#54872=CARTESIAN_POINT('Ctrl Pts',(-37.5398562037872,39.8561642112719,16.9832093943176));
#54873=CARTESIAN_POINT('Ctrl Pts',(-37.4178373052429,38.3450042264081,16.9140416672824));
#54874=CARTESIAN_POINT('Ctrl Pts',(-38.013720699012,37.6996801517363,16.8710424437061));
#54875=CARTESIAN_POINT('Ctrl Pts',(-38.2960217454206,37.5343651514648,16.8542117235887));
#54876=CARTESIAN_POINT('Ctrl Pts',(-38.2959007276492,37.5337106753505,17.3957882764113));
#54877=CARTESIAN_POINT('Ctrl Pts',(-38.4288872990661,37.4555469373629,17.3878441566028));
#54878=CARTESIAN_POINT('Ctrl Pts',(-39.0471107626292,37.2043843657908,17.3537315333353));
#54879=CARTESIAN_POINT('Ctrl Pts',(-40.3208285827552,37.5557507395872,17.293450406609));
#54880=CARTESIAN_POINT('Ctrl Pts',(-40.8541369642561,39.1917640019411,17.2149448962322));
#54881=CARTESIAN_POINT('Ctrl Pts',(-39.7836658898432,40.5390185509755,17.1364393858554));
#54882=CARTESIAN_POINT('Ctrl Pts',(-38.0694451486085,40.389246627264,17.0579338754786));
#54883=CARTESIAN_POINT('Ctrl Pts',(-37.248825754395,38.87677605618,16.9794283651019));
#54884=CARTESIAN_POINT('Ctrl Pts',(-37.8057511921981,37.8311625054488,16.9253798320794));
#54885=CARTESIAN_POINT('Ctrl Pts',(-38.2640668491777,37.5482868076194,16.8974998025159));
#54886=CARTESIAN_POINT('Ctrl Pts',(-38.2927752994979,37.5318947737649,16.8957882764113));
#54887=CARTESIAN_POINT('Origin',(-39.0658530619283,38.8697713466882,19.1042117235887));
#54888=CARTESIAN_POINT('',(-38.2938718037177,37.5356881270255,17.8957882764113));
#54889=CARTESIAN_POINT('',(-38.2940537528419,37.5314721085808,17.8542117235887));
#54890=CARTESIAN_POINT('',(-38.2943530619284,37.5334941486488,19.1042117235887));
#54891=CARTESIAN_POINT('',(-37.5756558680257,39.2699729499893,18.));
#54892=CARTESIAN_POINT('Ctrl Pts',(-37.5756558680257,39.2699729499893,18.));
#54893=CARTESIAN_POINT('Ctrl Pts',(-37.4440523270134,38.7799318659294,17.9738314965411));
#54894=CARTESIAN_POINT('Ctrl Pts',(-37.6166680705089,38.0418709533316,17.9390942553448));
#54895=CARTESIAN_POINT('Ctrl Pts',(-38.1491376523637,37.6179382396386,17.9043570141486));
#54896=CARTESIAN_POINT('Ctrl Pts',(-38.2938718037177,37.5356881270255,17.8957882764113));
#54897=CARTESIAN_POINT('',(-37.9726405222314,39.962294313691,18.));
#54898=CARTESIAN_POINT('Origin',(-39.0658530619283,38.8697713466882,18.));
#54899=CARTESIAN_POINT('Ctrl Pts',(-37.972631799081,39.9623061512025,18.));
#54900=CARTESIAN_POINT('Ctrl Pts',(-37.6338216029696,39.6208387086168,17.975091839613));
#54901=CARTESIAN_POINT('Ctrl Pts',(-37.3042322663879,38.6195093398435,17.9264957474759));
#54902=CARTESIAN_POINT('Ctrl Pts',(-37.899143973177,37.7627950030077,17.8778996553388));
#54903=CARTESIAN_POINT('Ctrl Pts',(-38.2940537528419,37.5314721085808,17.8542117235887));
#54904=CARTESIAN_POINT('Origin',(-53.1951359564886,-14.3971354987959,15.5));
#54905=CARTESIAN_POINT('',(-51.9326028526449,-14.3970877066932,14.1934196736194));
#54906=CARTESIAN_POINT('',(-51.9314232360955,-14.3954626592386,14.0565803263806));
#54907=CARTESIAN_POINT('',(-51.9306359564886,-14.3971354987959,15.5));
#54908=CARTESIAN_POINT('',(-52.2370198037663,-15.2223467977324,14.));
#54909=CARTESIAN_POINT('Ctrl Pts',(-51.9314232360955,-14.3954626592386,
14.0565803263806));
#54910=CARTESIAN_POINT('Ctrl Pts',(-51.9340308380707,-14.6945947257524,
14.0377202175871));
#54911=CARTESIAN_POINT('Ctrl Pts',(-52.0414421537953,-14.9952702831595,
14.0188601087935));
#54912=CARTESIAN_POINT('Ctrl Pts',(-52.2370198037663,-15.2223467977324,
14.));
#54913=CARTESIAN_POINT('',(-51.9306359564886,-14.3971354987959,14.));
#54914=CARTESIAN_POINT('Origin',(-53.1951359564886,-14.3971354987959,14.));
#54915=CARTESIAN_POINT('',(-51.9306359564886,-14.3971354987959,13.));
#54916=CARTESIAN_POINT('',(-51.9306359564886,-14.3971354987959,15.5));
#54917=CARTESIAN_POINT('',(-52.6278006430704,-15.5272199611918,13.));
#54918=CARTESIAN_POINT('Origin',(-53.1951359564886,-14.3971354987959,13.));
#54919=CARTESIAN_POINT('',(-53.7624712699068,-13.2670510364,13.));
#54920=CARTESIAN_POINT('Origin',(-53.1951359564886,-14.3971354987959,13.));
#54921=CARTESIAN_POINT('Origin',(-53.1951359564886,-14.3971354987959,13.));
#54922=CARTESIAN_POINT('',(-54.1550391816747,-15.22347043962,14.));
#54923=CARTESIAN_POINT('Origin',(-53.1951359564886,-14.3971354987959,14.));
#54924=CARTESIAN_POINT('Ctrl Pts',(-54.1550492157916,-15.2234767486838,
14.));
#54925=CARTESIAN_POINT('Ctrl Pts',(-53.8967914626892,-15.5213134049997,
14.024908160387));
#54926=CARTESIAN_POINT('Ctrl Pts',(-53.4877406809989,-15.6908539055355,
14.049816320774));
#54927=CARTESIAN_POINT('Ctrl Pts',(-53.0948318338551,-15.6595885868543,
14.074724481161));
#54928=CARTESIAN_POINT('Ctrl Pts',(-52.6820419543228,-15.626741255404,14.1008929846199));
#54929=CARTESIAN_POINT('Ctrl Pts',(-52.2870688888724,-15.3722525873919,
14.1270614880789));
#54930=CARTESIAN_POINT('Ctrl Pts',(-52.0867822938008,-15.0099588798403,
14.1532299915378));
#54931=CARTESIAN_POINT('Ctrl Pts',(-51.9842486685495,-14.8244882185226,
14.1666265522317));
#54932=CARTESIAN_POINT('Ctrl Pts',(-51.9327378835252,-14.6107643391081,
14.1800231129255));
#54933=CARTESIAN_POINT('Ctrl Pts',(-51.9326028526449,-14.3970877066932,
14.1934196736194));
#54934=CARTESIAN_POINT('Origin',(-53.1951359564886,-14.3971354987959,15.5));
#54935=CARTESIAN_POINT('',(-51.9293004715569,-14.396357843321,14.6934196736194));
#54936=CARTESIAN_POINT('',(-51.9290361749446,-14.3977594574901,14.5565803263806));
#54937=CARTESIAN_POINT('',(-51.9306359564886,-14.3971354987959,15.5));
#54938=CARTESIAN_POINT('Ctrl Pts',(-51.9290361749446,-14.3977594574901,
14.5565803263806));
#54939=CARTESIAN_POINT('Ctrl Pts',(-51.9288104788004,-14.4349272053691,
14.5542330751329));
#54940=CARTESIAN_POINT('Ctrl Pts',(-51.9303086019301,-14.4720763914416,
14.5518858238852));
#54941=CARTESIAN_POINT('Ctrl Pts',(-51.9335904462524,-14.5090671744586,
14.5495385726375));
#54942=CARTESIAN_POINT('Ctrl Pts',(-51.9701783294547,-14.9214616440634,
14.5233700691785));
#54943=CARTESIAN_POINT('Ctrl Pts',(-52.228466159159,-15.3141680878373,14.4972015657196));
#54944=CARTESIAN_POINT('Ctrl Pts',(-52.5926396873008,-15.5111367764164,
14.4710330622607));
#54945=CARTESIAN_POINT('Ctrl Pts',(-52.9568132154426,-15.7081054649955,
14.4448645588018));
#54946=CARTESIAN_POINT('Ctrl Pts',(-53.4268724420219,-15.7093363983798,
14.4186960553428));
#54947=CARTESIAN_POINT('Ctrl Pts',(-53.7920269612472,-15.514187779113,14.3925275518839));
#54948=CARTESIAN_POINT('Ctrl Pts',(-54.1571814804725,-15.3190391598462,
14.366359048425));
#54949=CARTESIAN_POINT('Ctrl Pts',(-54.4174312923439,-14.9275109879282,
14.340190544966));
#54950=CARTESIAN_POINT('Ctrl Pts',(-54.4560979757245,-14.5153505128056,
14.3140220415071));
#54951=CARTESIAN_POINT('Ctrl Pts',(-54.4947646591051,-14.103190037683,14.2878535380482));
#54952=CARTESIAN_POINT('Ctrl Pts',(-54.3118482139948,-13.6703972593558,
14.2616850345893));
#54953=CARTESIAN_POINT('Ctrl Pts',(-53.9893291901183,-13.4106746119161,
14.2355165311303));
#54954=CARTESIAN_POINT('Ctrl Pts',(-53.6668101662417,-13.1509519644764,
14.2093480276714));
#54955=CARTESIAN_POINT('Ctrl Pts',(-53.2046885635989,-13.0642994479243,
14.1831795242125));
#54956=CARTESIAN_POINT('Ctrl Pts',(-52.8102658096442,-13.1903246291658,
14.1570110207536));
#54957=CARTESIAN_POINT('Ctrl Pts',(-52.4158430556895,-13.3163498104073,
14.1308425172946));
#54958=CARTESIAN_POINT('Ctrl Pts',(-52.089119150423,-13.6550526894425,14.1046740138357));
#54959=CARTESIAN_POINT('Ctrl Pts',(-51.976572074359,-14.0527844617314,14.0785055103768));
#54960=CARTESIAN_POINT('Ctrl Pts',(-51.9451396903252,-14.163863827329,14.0711971157114));
#54961=CARTESIAN_POINT('Ctrl Pts',(-51.9304127761573,-14.2795473576308,
14.063888721046));
#54962=CARTESIAN_POINT('Ctrl Pts',(-51.9314232360955,-14.3954626592386,
14.0565803263806));
#54963=CARTESIAN_POINT('Ctrl Pts',(-51.9326028526449,-14.3970877066932,
14.1934196736194));
#54964=CARTESIAN_POINT('Ctrl Pts',(-51.9324741176124,-14.1933737996841,
14.2061916163845));
#54965=CARTESIAN_POINT('Ctrl Pts',(-51.9790420088886,-13.9897028365794,
14.2189635591495));
#54966=CARTESIAN_POINT('Ctrl Pts',(-52.0726123421383,-13.8105984338676,
14.2317355019146));
#54967=CARTESIAN_POINT('Ctrl Pts',(-52.2643291102402,-13.4436304425376,
14.2579040053735));
#54968=CARTESIAN_POINT('Ctrl Pts',(-52.6533627711367,-13.1797932069689,
14.2840725088324));
#54969=CARTESIAN_POINT('Ctrl Pts',(-53.0652069371965,-13.1373261840987,
14.3102410122914));
#54970=CARTESIAN_POINT('Ctrl Pts',(-53.4770511032563,-13.0948591612284,
14.3364095157503));
#54971=CARTESIAN_POINT('Ctrl Pts',(-53.9117057744794,-13.2737623510566,
14.3625780192092));
#54972=CARTESIAN_POINT('Ctrl Pts',(-54.174295890408,-13.5938472660216,14.3887465226681));
#54973=CARTESIAN_POINT('Ctrl Pts',(-54.4368860063367,-13.9139321809865,
14.4149150261271));
#54974=CARTESIAN_POINT('Ctrl Pts',(-54.5274115669709,-14.3751988210882,
14.441083529586));
#54975=CARTESIAN_POINT('Ctrl Pts',(-54.4052653400131,-14.7707929840487,
14.4672520330449));
#54976=CARTESIAN_POINT('Ctrl Pts',(-54.2831191130553,-15.1663871470091,
14.4934205365038));
#54977=CARTESIAN_POINT('Ctrl Pts',(-53.9483010985055,-15.4963088328283,
14.5195890399628));
#54978=CARTESIAN_POINT('Ctrl Pts',(-53.5509548543059,-15.6126255371819,
14.5457575434217));
#54979=CARTESIAN_POINT('Ctrl Pts',(-53.1536086101064,-15.7289422415355,
14.5719260468806));
#54980=CARTESIAN_POINT('Ctrl Pts',(-52.6937341362571,-15.6316539644235,
14.5980945503395));
#54981=CARTESIAN_POINT('Ctrl Pts',(-52.3775410563803,-15.3643818135364,
14.6242630537985));
#54982=CARTESIAN_POINT('Ctrl Pts',(-52.0990020785416,-15.1289379773151,
14.6473152604054));
#54983=CARTESIAN_POINT('Ctrl Pts',(-51.9319612775611,-14.7615849808525,
14.6703674670124));
#54984=CARTESIAN_POINT('Ctrl Pts',(-51.9293004715569,-14.396357843321,14.6934196736194));
#54985=CARTESIAN_POINT('Origin',(-53.1951359564886,-14.3971354987959,15.5));
#54986=CARTESIAN_POINT('',(-51.9308136275137,-14.3982246453427,15.1934196736194));
#54987=CARTESIAN_POINT('',(-51.932525975067,-14.3974029423036,15.0565803263806));
#54988=CARTESIAN_POINT('',(-51.9306359564886,-14.3971354987959,15.5));
#54989=CARTESIAN_POINT('Ctrl Pts',(-51.932525975067,-14.3974029423036,15.0565803263806));
#54990=CARTESIAN_POINT('Ctrl Pts',(-51.9321561072822,-14.5888155966727,
15.0445774292198));
#54991=CARTESIAN_POINT('Ctrl Pts',(-51.9730705675611,-14.7800782049927,
15.0325745320589));
#54992=CARTESIAN_POINT('Ctrl Pts',(-52.0560982976485,-14.9508677919232,
15.0205716348981));
#54993=CARTESIAN_POINT('Ctrl Pts',(-52.2371138818754,-15.3232202195459,
14.9944031314392));
#54994=CARTESIAN_POINT('Ctrl Pts',(-52.6183020364058,-15.5982603906742,
14.9682346279803));
#54995=CARTESIAN_POINT('Ctrl Pts',(-53.0287335368761,-15.6526576817852,
14.9420661245214));
#54996=CARTESIAN_POINT('Ctrl Pts',(-53.4391650373463,-15.7070549728962,
14.9158976210624));
#54997=CARTESIAN_POINT('Ctrl Pts',(-53.8788398837565,-15.5408093839899,
14.8897291176035));
#54998=CARTESIAN_POINT('Ctrl Pts',(-54.1506024967829,-15.2284660841227,
14.8635606141446));
#54999=CARTESIAN_POINT('Ctrl Pts',(-54.4223651098093,-14.9161227842554,
14.8373921106857));
#55000=CARTESIAN_POINT('Ctrl Pts',(-54.5262154894519,-14.4576817734273,
14.8112236072267));
#55001=CARTESIAN_POINT('Ctrl Pts',(-54.4155861975138,-14.0587161328242,
14.7850551037678));
#55002=CARTESIAN_POINT('Ctrl Pts',(-54.3049569055756,-13.6597504922211,
14.7588866003089));
#55003=CARTESIAN_POINT('Ctrl Pts',(-53.9798479420568,-13.320260221843,14.7327180968499));
#55004=CARTESIAN_POINT('Ctrl Pts',(-53.5860414121493,-13.1924713804069,
14.706549593391));
#55005=CARTESIAN_POINT('Ctrl Pts',(-53.1922348822418,-13.0646825389707,
14.6803810899321));
#55006=CARTESIAN_POINT('Ctrl Pts',(-52.7297307859455,-13.1485951264764,
14.6542125864732));
#55007=CARTESIAN_POINT('Ctrl Pts',(-52.4059227061476,-13.4065926679472,
14.6280440830142));
#55008=CARTESIAN_POINT('Ctrl Pts',(-52.1111594252055,-13.6414484561238,
14.604222830803));
#55009=CARTESIAN_POINT('Ctrl Pts',(-51.9313266688913,-14.0205598299628,
14.5804015785918));
#55010=CARTESIAN_POINT('Ctrl Pts',(-51.9290361749446,-14.3977594574901,
14.5565803263806));
#55011=CARTESIAN_POINT('Ctrl Pts',(-51.9293004715569,-14.396357843321,14.6934196736194));
#55012=CARTESIAN_POINT('Ctrl Pts',(-51.9289407723091,-14.3469848614482,
14.6965359704714));
#55013=CARTESIAN_POINT('Ctrl Pts',(-51.9315850846113,-14.2976507292223,
14.6996522673233));
#55014=CARTESIAN_POINT('Ctrl Pts',(-51.9373640512185,-14.2486865756559,
14.7027685641753));
#55015=CARTESIAN_POINT('Ctrl Pts',(-51.985891811838,-13.8375195133245,14.7289370676342));
#55016=CARTESIAN_POINT('Ctrl Pts',(-52.2554590189813,-13.452441413324,14.7551055710931));
#55017=CARTESIAN_POINT('Ctrl Pts',(-52.62518765984,-13.2661248639499,14.781274074552));
#55018=CARTESIAN_POINT('Ctrl Pts',(-52.9949163006986,-13.0798083145759,
14.807442578011));
#55019=CARTESIAN_POINT('Ctrl Pts',(-53.4648063752726,-13.0922533158284,
14.8336110814699));
#55020=CARTESIAN_POINT('Ctrl Pts',(-53.8241540209967,-13.2978798810904,
14.8597795849288));
#55021=CARTESIAN_POINT('Ctrl Pts',(-54.1835016667209,-13.5035064463524,
14.8859480883877));
#55022=CARTESIAN_POINT('Ctrl Pts',(-54.4323068835952,-13.902314575624,14.9121165918467));
#55023=CARTESIAN_POINT('Ctrl Pts',(-54.4590022406867,-14.3154737155563,
14.9382850953056));
#55024=CARTESIAN_POINT('Ctrl Pts',(-54.4856975977781,-14.7286328554886,
14.9644535987645));
#55025=CARTESIAN_POINT('Ctrl Pts',(-54.2902830950867,-15.1561430060817,
14.9906221022234));
#55026=CARTESIAN_POINT('Ctrl Pts',(-53.9603850245762,-15.4063036567383,
15.0167906056824));
#55027=CARTESIAN_POINT('Ctrl Pts',(-53.6304869540657,-15.656464307395,15.0429591091413));
#55028=CARTESIAN_POINT('Ctrl Pts',(-53.1661053157362,-15.7292754581154,
15.0691276126002));
#55029=CARTESIAN_POINT('Ctrl Pts',(-52.7754743036767,-15.592087662659,15.0952961160592));
#55030=CARTESIAN_POINT('Ctrl Pts',(-52.3848432916172,-15.4548998672026,
15.1214646195181));
#55031=CARTESIAN_POINT('Ctrl Pts',(-52.0679629058276,-15.1077131255694,
15.147633122977));
#55032=CARTESIAN_POINT('Ctrl Pts',(-51.9669261040319,-14.7062101297548,
15.1738016264359));
#55033=CARTESIAN_POINT('Ctrl Pts',(-51.9416776248439,-14.6058769852609,
15.1803409754971));
#55034=CARTESIAN_POINT('Ctrl Pts',(-51.9299079202419,-14.502151956084,15.1868803245583));
#55035=CARTESIAN_POINT('Ctrl Pts',(-51.9308136275137,-14.3982246453427,
15.1934196736194));
#55036=CARTESIAN_POINT('Origin',(-53.1951359564886,-14.3971354987959,15.5));
#55037=CARTESIAN_POINT('',(-51.9321336144333,-14.3964211293814,15.6934196736194));
#55038=CARTESIAN_POINT('',(-51.9298800777713,-14.396145855272,15.5565803263806));
#55039=CARTESIAN_POINT('',(-51.9306359564886,-14.3971354987959,15.5));
#55040=CARTESIAN_POINT('Ctrl Pts',(-51.9298800777713,-14.396145855272,15.5565803263806));
#55041=CARTESIAN_POINT('Ctrl Pts',(-51.9328341793634,-14.7397024926117,
15.5349217833067));
#55042=CARTESIAN_POINT('Ctrl Pts',(-52.0781516403077,-15.0854616424501,
15.5132632402327));
#55043=CARTESIAN_POINT('Ctrl Pts',(-52.3278732854,-15.32010983553,15.4916046971588));
#55044=CARTESIAN_POINT('Ctrl Pts',(-52.6295944912569,-15.6036188430972,
15.4654361936999));
#55045=CARTESIAN_POINT('Ctrl Pts',(-53.0837270081697,-15.7249258591405,
15.439267690241));
#55046=CARTESIAN_POINT('Ctrl Pts',(-53.4866324184767,-15.629635385456,15.413099186782));
#55047=CARTESIAN_POINT('Ctrl Pts',(-53.8895378287837,-15.5343449117715,
15.3869306833231));
#55048=CARTESIAN_POINT('Ctrl Pts',(-54.2412161324849,-15.2224569483592,
15.3607621798642));
#55049=CARTESIAN_POINT('Ctrl Pts',(-54.3839705956172,-14.8338257457023,
15.3345936764052));
#55050=CARTESIAN_POINT('Ctrl Pts',(-54.5267250587495,-14.4451945430454,
15.3084251729463));
#55051=CARTESIAN_POINT('Ctrl Pts',(-54.4605556813129,-13.9798201011439,
15.2822566694874));
#55052=CARTESIAN_POINT('Ctrl Pts',(-54.2151336032284,-13.6463818912608,
15.2560881660285));
#55053=CARTESIAN_POINT('Ctrl Pts',(-53.9697115251439,-13.3129436813777,
15.2299196625696));
#55054=CARTESIAN_POINT('Ctrl Pts',(-53.5450367464114,-13.111441703513,15.2037511591106));
#55055=CARTESIAN_POINT('Ctrl Pts',(-53.1315384766945,-13.1322317596502,
15.1775826556517));
#55056=CARTESIAN_POINT('Ctrl Pts',(-52.7180402069775,-13.1530218157874,
15.1514141521928));
#55057=CARTESIAN_POINT('Ctrl Pts',(-52.3157184462761,-13.3961039059265,
15.1252456487338));
#55058=CARTESIAN_POINT('Ctrl Pts',(-52.1049790728871,-13.7524772930548,
15.0990771452749));
#55059=CARTESIAN_POINT('Ctrl Pts',(-51.99090105541,-13.9453903155784,15.0849115389768));
#55060=CARTESIAN_POINT('Ctrl Pts',(-51.9329624864653,-14.1715011232728,
15.0707459326787));
#55061=CARTESIAN_POINT('Ctrl Pts',(-51.932525975067,-14.3974029423036,15.0565803263806));
#55062=CARTESIAN_POINT('Ctrl Pts',(-51.9308136275137,-14.3982246453427,
15.1934196736194));
#55063=CARTESIAN_POINT('Ctrl Pts',(-51.9335322876909,-14.0862661905168,
15.2130488280172));
#55064=CARTESIAN_POINT('Ctrl Pts',(-52.0504588679336,-13.7724851395516,
15.2326779824149));
#55065=CARTESIAN_POINT('Ctrl Pts',(-52.2598657119042,-13.5431471347949,
15.2523071368127));
#55066=CARTESIAN_POINT('Ctrl Pts',(-52.5390353393738,-13.2374063856457,
15.2784756402716));
#55067=CARTESIAN_POINT('Ctrl Pts',(-52.9825678121147,-13.0817441373434,
15.3046441437306));
#55068=CARTESIAN_POINT('Ctrl Pts',(-53.3915779035484,-13.1459611997424,
15.3308126471895));
#55069=CARTESIAN_POINT('Ctrl Pts',(-53.8005879949821,-13.2101782621413,
15.3569811506484));
#55070=CARTESIAN_POINT('Ctrl Pts',(-54.1750757051085,-13.4942746352416,
15.3831496541073));
#55071=CARTESIAN_POINT('Ctrl Pts',(-54.3471162900744,-13.8708581246834,
15.4093181575663));
#55072=CARTESIAN_POINT('Ctrl Pts',(-54.5191568750402,-14.2474416141252,
15.4354866610252));
#55073=CARTESIAN_POINT('Ctrl Pts',(-54.4887503348454,-14.7165122199085,
15.4616551644841));
#55074=CARTESIAN_POINT('Ctrl Pts',(-54.2695313251181,-15.0677331084555,
15.4878236679431));
#55075=CARTESIAN_POINT('Ctrl Pts',(-54.0503123153908,-15.4189539970025,
15.513992171402));
#55076=CARTESIAN_POINT('Ctrl Pts',(-53.642280836131,-15.6523251683133,15.5401606748609));
#55077=CARTESIAN_POINT('Ctrl Pts',(-53.2284030520588,-15.6632002142321,
15.5663291783198));
#55078=CARTESIAN_POINT('Ctrl Pts',(-52.8145252679866,-15.6740752601508,
15.5924976817788));
#55079=CARTESIAN_POINT('Ctrl Pts',(-52.3948011791021,-15.4624541806777,
15.6186661852377));
#55080=CARTESIAN_POINT('Ctrl Pts',(-52.1574400564301,-15.1232303837968,
15.6448346886966));
#55081=CARTESIAN_POINT('Ctrl Pts',(-52.010543532722,-14.9132937439633,15.6610296836709));
#55082=CARTESIAN_POINT('Ctrl Pts',(-51.9334928433345,-14.6544846908102,
15.6772246786452));
#55083=CARTESIAN_POINT('Ctrl Pts',(-51.9321336144333,-14.3964211293814,
15.6934196736194));
#55084=CARTESIAN_POINT('Origin',(-53.1951359564886,-14.3971354987959,15.5));
#55085=CARTESIAN_POINT('',(-51.9286427349007,-14.3970459914357,16.1934196736194));
#55086=CARTESIAN_POINT('',(-51.9301690580705,-14.3981838623804,16.0565803263806));
#55087=CARTESIAN_POINT('',(-51.9306359564886,-14.3971354987959,15.5));
#55088=CARTESIAN_POINT('Ctrl Pts',(-51.9301690580705,-14.3981838623804,
16.0565803263806));
#55089=CARTESIAN_POINT('Ctrl Pts',(-51.9294463895002,-14.4798551199685,
16.0514346408525));
#55090=CARTESIAN_POINT('Ctrl Pts',(-51.9366958070815,-14.5613987134005,
16.0462889553244));
#55091=CARTESIAN_POINT('Ctrl Pts',(-51.9523897974866,-14.6412833003864,
16.0411432697963));
#55092=CARTESIAN_POINT('Ctrl Pts',(-52.0322019507863,-15.0475382258844,
16.0149747663373));
#55093=CARTESIAN_POINT('Ctrl Pts',(-52.3304122644718,-15.4108870194283,
15.9888062628784));
#55094=CARTESIAN_POINT('Ctrl Pts',(-52.7132996891177,-15.5683997628469,
15.9626377594195));
#55095=CARTESIAN_POINT('Ctrl Pts',(-53.0961871137635,-15.7259125062655,
15.9364692559606));
#55096=CARTESIAN_POINT('Ctrl Pts',(-53.5637516493698,-15.6775891995586,
15.9103007525016));
#55097=CARTESIAN_POINT('Ctrl Pts',(-53.9063318003261,-15.4450985880149,
15.8841322490427));
#55098=CARTESIAN_POINT('Ctrl Pts',(-54.2489119512824,-15.2126079764712,
15.8579637455838));
#55099=CARTESIAN_POINT('Ctrl Pts',(-54.4665077175887,-14.7959500600907,
15.8317952421249));
#55100=CARTESIAN_POINT('Ctrl Pts',(-54.4615465710813,-14.3819592010216,
15.8056267386659));
#55101=CARTESIAN_POINT('Ctrl Pts',(-54.4565854245739,-13.9679683419524,
15.779458235207));
#55102=CARTESIAN_POINT('Ctrl Pts',(-54.2290673652527,-13.5566445401947,
15.7532897317481));
#55103=CARTESIAN_POINT('Ctrl Pts',(-53.8810141954492,-13.3324302783772,
15.7271212282891));
#55104=CARTESIAN_POINT('Ctrl Pts',(-53.5329610256457,-13.1082160165598,
15.7009527248302));
#55105=CARTESIAN_POINT('Ctrl Pts',(-53.0643727453599,-13.0711112946827,
15.6747842213713));
#55106=CARTESIAN_POINT('Ctrl Pts',(-52.6853699093616,-13.2377543099066,
15.6486157179124));
#55107=CARTESIAN_POINT('Ctrl Pts',(-52.3063670733632,-13.4043973251304,
15.6224472144534));
#55108=CARTESIAN_POINT('Ctrl Pts',(-52.0169496816522,-13.7747880774553,
15.5962787109945));
#55109=CARTESIAN_POINT('Ctrl Pts',(-51.9468959331972,-14.1828389531634,
15.5701102075356));
#55110=CARTESIAN_POINT('Ctrl Pts',(-51.9348226546909,-14.2531636963187,
15.5656002471506));
#55111=CARTESIAN_POINT('Ctrl Pts',(-51.9292649449293,-14.324607025577,15.5610902867656));
#55112=CARTESIAN_POINT('Ctrl Pts',(-51.9298800777713,-14.396145855272,15.5565803263806));
#55113=CARTESIAN_POINT('Ctrl Pts',(-51.9321336144333,-14.3964211293814,
15.6934196736194));
#55114=CARTESIAN_POINT('Ctrl Pts',(-51.9312965483521,-14.2374955401126,
15.7033931821041));
#55115=CARTESIAN_POINT('Ctrl Pts',(-51.9591660436084,-14.0788526842429,
15.7133666905887));
#55116=CARTESIAN_POINT('Ctrl Pts',(-52.0171074139709,-13.932081398796,15.7233401990734));
#55117=CARTESIAN_POINT('Ctrl Pts',(-52.1691340506433,-13.5469827249646,
15.7495087025323));
#55118=CARTESIAN_POINT('Ctrl Pts',(-52.5281854804478,-13.2436118915905,
15.7756772059912));
#55119=CARTESIAN_POINT('Ctrl Pts',(-52.9332587743738,-13.1580039865908,
15.8018457094502));
#55120=CARTESIAN_POINT('Ctrl Pts',(-53.3383320682997,-13.072396081591,15.8280142129091));
#55121=CARTESIAN_POINT('Ctrl Pts',(-53.7894272263473,-13.2045511049655,
15.854182716368));
#55122=CARTESIAN_POINT('Ctrl Pts',(-54.0842678175163,-13.4952091732588,
15.880351219827));
#55123=CARTESIAN_POINT('Ctrl Pts',(-54.3791084086854,-13.7858672415521,
15.9065197232859));
#55124=CARTESIAN_POINT('Ctrl Pts',(-54.517694432976,-14.2350283547642,15.9326882267448));
#55125=CARTESIAN_POINT('Ctrl Pts',(-54.4378822697683,-14.6412833306956,
15.9588567302037));
#55126=CARTESIAN_POINT('Ctrl Pts',(-54.3580701065605,-15.047538306627,15.9850252336626));
#55127=CARTESIAN_POINT('Ctrl Pts',(-54.0598597558545,-15.4108871452777,
16.0111937371216));
#55128=CARTESIAN_POINT('Ctrl Pts',(-53.676972283676,-15.5683999082504,16.0373622405805));
#55129=CARTESIAN_POINT('Ctrl Pts',(-53.2940848114975,-15.7259126712231,
16.0635307440394));
#55130=CARTESIAN_POINT('Ctrl Pts',(-52.8265202178467,-15.6775893585178,
16.0896992474984));
#55131=CARTESIAN_POINT('Ctrl Pts',(-52.4839400243616,-15.4450987181119,
16.1158677509573));
#55132=CARTESIAN_POINT('Ctrl Pts',(-52.1455210707975,-15.2154320860769,
16.1417183918447));
#55133=CARTESIAN_POINT('Ctrl Pts',(-51.9290686466627,-14.8060450268197,
16.167569032732));
#55134=CARTESIAN_POINT('Ctrl Pts',(-51.9286427349007,-14.3970459914357,
16.1934196736194));
#55135=CARTESIAN_POINT('Origin',(-53.1951359564886,-14.3971354987959,15.5));
#55136=CARTESIAN_POINT('',(-51.9319412138059,-14.3979628881409,16.6934196736194));
#55137=CARTESIAN_POINT('',(-51.9324421154971,-14.3967173588992,16.5565803263806));
#55138=CARTESIAN_POINT('',(-51.9306359564886,-14.3971354987959,15.5));
#55139=CARTESIAN_POINT('Ctrl Pts',(-51.9324421154971,-14.3967173588992,
16.5565803263806));
#55140=CARTESIAN_POINT('Ctrl Pts',(-51.9331582847598,-14.6327178878915,
16.5417789949394));
#55141=CARTESIAN_POINT('Ctrl Pts',(-51.9967468970028,-14.869076799286,16.5269776634982));
#55142=CARTESIAN_POINT('Ctrl Pts',(-52.1207407212382,-15.0677330252045,
16.5121763320569));
#55143=CARTESIAN_POINT('Ctrl Pts',(-52.339959703752,-15.4189538701487,16.486007828598));
#55144=CARTESIAN_POINT('Ctrl Pts',(-52.747991132356,-15.652325012491,16.4598393251391));
#55145=CARTESIAN_POINT('Ctrl Pts',(-53.1618688650479,-15.6632000570604,
16.4336708216802));
#55146=CARTESIAN_POINT('Ctrl Pts',(-53.5757465977398,-15.6740751016298,
16.4075023182212));
#55147=CARTESIAN_POINT('Ctrl Pts',(-53.9954706345197,-15.4624540484263,
16.3813338147623));
#55148=CARTESIAN_POINT('Ctrl Pts',(-54.2328317277253,-15.1232302936571,
16.3551653113034));
#55149=CARTESIAN_POINT('Ctrl Pts',(-54.470192820931,-14.784006538888,16.3289968078444));
#55150=CARTESIAN_POINT('Ctrl Pts',(-54.5251909705625,-14.3171800825531,
16.3028283043855));
#55151=CARTESIAN_POINT('Ctrl Pts',(-54.3731643527629,-13.9320814565291,
16.2766598009266));
#55152=CARTESIAN_POINT('Ctrl Pts',(-54.2211377349632,-13.546982830505,16.2504912974677));
#55153=CARTESIAN_POINT('Ctrl Pts',(-53.8620863497326,-13.2436120347917,
16.2243227940088));
#55154=CARTESIAN_POINT('Ctrl Pts',(-53.4570131060935,-13.1580041404195,
16.1981542905498));
#55155=CARTESIAN_POINT('Ctrl Pts',(-53.0519398624543,-13.0723962460472,
16.1719857870909));
#55156=CARTESIAN_POINT('Ctrl Pts',(-52.6008447604068,-13.204551253016,16.145817283632));
#55157=CARTESIAN_POINT('Ctrl Pts',(-52.3060042058399,-13.4952092852263,
16.119648780173));
#55158=CARTESIAN_POINT('Ctrl Pts',(-52.0691400952495,-13.7287133104327,
16.0986259622422));
#55159=CARTESIAN_POINT('Ctrl Pts',(-51.9331215373257,-14.0645140395593,
16.0776031443114));
#55160=CARTESIAN_POINT('Ctrl Pts',(-51.9301690580705,-14.3981838623804,
16.0565803263806));
#55161=CARTESIAN_POINT('Ctrl Pts',(-51.9286427349007,-14.3970459914357,
16.1934196736194));
#55162=CARTESIAN_POINT('Ctrl Pts',(-51.9286374978387,-14.3920168903888,
16.193737536191));
#55163=CARTESIAN_POINT('Ctrl Pts',(-51.9286649228095,-14.386987848009,16.1940553987625));
#55164=CARTESIAN_POINT('Ctrl Pts',(-51.9287251846806,-14.3819591991371,
16.1943732613341));
#55165=CARTESIAN_POINT('Ctrl Pts',(-51.9336863318039,-13.9679682886745,
16.220541764793));
#55166=CARTESIAN_POINT('Ctrl Pts',(-52.1612044193698,-13.5566444358558,
16.2467102682519));
#55167=CARTESIAN_POINT('Ctrl Pts',(-52.5092576323814,-13.332430146203,16.2728787717108));
#55168=CARTESIAN_POINT('Ctrl Pts',(-52.857310845393,-13.1082158565502,16.2990472751698));
#55169=CARTESIAN_POINT('Ctrl Pts',(-53.3258991838504,-13.0711111300635,
16.3252157786287));
#55170=CARTESIAN_POINT('Ctrl Pts',(-53.7049020668993,-13.2377541659764,
16.3513842820876));
#55171=CARTESIAN_POINT('Ctrl Pts',(-54.0839049499481,-13.4043972018893,
16.3775527855466));
#55172=CARTESIAN_POINT('Ctrl Pts',(-54.3733223775883,-13.7747880002018,
16.4037212890055));
#55173=CARTESIAN_POINT('Ctrl Pts',(-54.4433761347398,-14.1828389265634,
16.4298897924644));
#55174=CARTESIAN_POINT('Ctrl Pts',(-54.5134298918912,-14.5908898529249,
16.4560582959233));
#55175=CARTESIAN_POINT('Ctrl Pts',(-54.3641199785539,-15.0366009073354,
16.4822267993823));
#55176=CARTESIAN_POINT('Ctrl Pts',(-54.0623987352411,-15.3201099501039,
16.5083953028412));
#55177=CARTESIAN_POINT('Ctrl Pts',(-53.7606774919283,-15.6036189928724,
16.5345638063001));
#55178=CARTESIAN_POINT('Ctrl Pts',(-53.30654491864,-15.724926023999,16.560732309759));
#55179=CARTESIAN_POINT('Ctrl Pts',(-52.9036394583143,-15.6296355384739,
16.586900813218));
#55180=CARTESIAN_POINT('Ctrl Pts',(-52.5007339979887,-15.5343450529489,
16.6130693166769));
#55181=CARTESIAN_POINT('Ctrl Pts',(-52.1490556506257,-15.2224570507722,
16.6392378201358));
#55182=CARTESIAN_POINT('Ctrl Pts',(-52.0063011697735,-14.8338257998905,
16.6654063235947));
#55183=CARTESIAN_POINT('Ctrl Pts',(-51.9553616723993,-14.6951493782072,
16.6747441069363));
#55184=CARTESIAN_POINT('Ctrl Pts',(-51.9310243942125,-14.5467012595068,
16.6840818902779));
#55185=CARTESIAN_POINT('Ctrl Pts',(-51.9319412138059,-14.3979628881409,
16.6934196736194));
#55186=CARTESIAN_POINT('Origin',(-53.1951359564886,-14.3971354987959,15.5));
#55187=CARTESIAN_POINT('',(-51.9310991161132,-14.3960665614756,17.1934196736194));
#55188=CARTESIAN_POINT('',(-51.9288577112775,-14.3966710926088,17.0565803263806));
#55189=CARTESIAN_POINT('',(-51.9306359564886,-14.3971354987959,15.5));
#55190=CARTESIAN_POINT('Ctrl Pts',(-51.9288577112775,-14.3966710926088,
17.0565803263806));
#55191=CARTESIAN_POINT('Ctrl Pts',(-51.9307115507732,-14.7837959519869,
17.0321233490263));
#55192=CARTESIAN_POINT('Ctrl Pts',(-52.121565621024,-15.1725044294775,17.0076663716719));
#55193=CARTESIAN_POINT('Ctrl Pts',(-52.4298869834431,-15.406303531382,16.9832093943176));
#55194=CARTESIAN_POINT('Ctrl Pts',(-52.7597850130333,-15.6564641509158,
16.9570408908587));
#55195=CARTESIAN_POINT('Ctrl Pts',(-53.2241665936332,-15.7292752927444,
16.9308723873998));
#55196=CARTESIAN_POINT('Ctrl Pts',(-53.6147975571803,-15.5920875143541,
16.9047038839408));
#55197=CARTESIAN_POINT('Ctrl Pts',(-54.0054285207274,-15.4548997359637,
16.8785353804819));
#55198=CARTESIAN_POINT('Ctrl Pts',(-54.3223088672216,-15.1077130373545,
16.852366877023));
#55199=CARTESIAN_POINT('Ctrl Pts',(-54.4233456564843,-14.706210091365,16.8261983735641));
#55200=CARTESIAN_POINT('Ctrl Pts',(-54.524382445747,-14.3047071453755,16.8000298701051));
#55201=CARTESIAN_POINT('Ctrl Pts',(-54.4095756777782,-13.8488879520058,
16.7738613666462));
#55202=CARTESIAN_POINT('Ctrl Pts',(-54.13040608496,-13.5431472408217,16.7476928631873));
#55203=CARTESIAN_POINT('Ctrl Pts',(-53.8512364921418,-13.2374065296375,
16.7215243597284));
#55204=CARTESIAN_POINT('Ctrl Pts',(-53.4077040744743,-13.0817443006388,
16.6953558562694));
#55205=CARTESIAN_POINT('Ctrl Pts',(-52.9986940338189,-13.1459613550607,
16.6691873528105));
#55206=CARTESIAN_POINT('Ctrl Pts',(-52.5896839931636,-13.2101784094827,
16.6430188493516));
#55207=CARTESIAN_POINT('Ctrl Pts',(-52.2151963295206,-13.4942747473253,
16.6168503458927));
#55208=CARTESIAN_POINT('Ctrl Pts',(-52.0431557659108,-13.8708581900196,
16.5906818424337));
#55209=CARTESIAN_POINT('Ctrl Pts',(-51.9684241449893,-14.0344399087392,
16.579314670416));
#55210=CARTESIAN_POINT('Ctrl Pts',(-51.9318921096253,-14.2154729472068,
16.5679474983983));
#55211=CARTESIAN_POINT('Ctrl Pts',(-51.9324421154971,-14.3967173588992,
16.5565803263806));
#55212=CARTESIAN_POINT('Ctrl Pts',(-51.9319412138059,-14.3979628881409,
16.6934196736194));
#55213=CARTESIAN_POINT('Ctrl Pts',(-51.9335937188396,-14.1298720781913,
16.7102503937368));
#55214=CARTESIAN_POINT('Ctrl Pts',(-52.0172907607077,-13.8608383066004,
16.7270811138542));
#55215=CARTESIAN_POINT('Ctrl Pts',(-52.1751381831274,-13.6463817981057,
16.7439118339715));
#55216=CARTESIAN_POINT('Ctrl Pts',(-52.4205602916747,-13.3129435467891,
16.7700803374304));
#55217=CARTESIAN_POINT('Ctrl Pts',(-52.8452351231106,-13.1114415437426,
16.7962488408894));
#55218=CARTESIAN_POINT('Ctrl Pts',(-53.25873344417,-13.1322316025356,16.8224173443483));
#55219=CARTESIAN_POINT('Ctrl Pts',(-53.6722317652293,-13.1530216613285,
16.8485858478072));
#55220=CARTESIAN_POINT('Ctrl Pts',(-54.0745535759121,-13.3961037819609,
16.8747543512662));
#55221=CARTESIAN_POINT('Ctrl Pts',(-54.2852929754421,-13.7524772131894,
16.9009228547251));
#55222=CARTESIAN_POINT('Ctrl Pts',(-54.496032374972,-14.108850644418,16.927091358184));
#55223=CARTESIAN_POINT('Ctrl Pts',(-54.5151893633491,-14.5785153862427,
16.9532598616429));
#55224=CARTESIAN_POINT('Ctrl Pts',(-54.3341737566947,-14.9508678603537,
16.9794283651019));
#55225=CARTESIAN_POINT('Ctrl Pts',(-54.1531581500404,-15.3232203344646,
17.0055968685608));
#55226=CARTESIAN_POINT('Ctrl Pts',(-53.7719699483547,-15.5982605408617,
17.0317653720197));
#55227=CARTESIAN_POINT('Ctrl Pts',(-53.3615383968383,-15.652657838236,17.0579338754786));
#55228=CARTESIAN_POINT('Ctrl Pts',(-52.9511068453218,-15.7070551356103,
17.0841023789376));
#55229=CARTESIAN_POINT('Ctrl Pts',(-52.5114319439747,-15.5408095239618,
17.1102708823965));
#55230=CARTESIAN_POINT('Ctrl Pts',(-52.2396692974108,-15.2284661862234,
17.1364393858554));
#55231=CARTESIAN_POINT('Ctrl Pts',(-52.0424205472225,-15.0017634594966,
17.1554328151101));
#55232=CARTESIAN_POINT('Ctrl Pts',(-51.9336286302044,-14.6980958787158,
17.1744262443647));
#55233=CARTESIAN_POINT('Ctrl Pts',(-51.9310991161132,-14.3960665614756,
17.1934196736194));
#55234=CARTESIAN_POINT('Origin',(-53.1951359564886,-14.3971354987959,15.5));
#55235=CARTESIAN_POINT('',(-51.929081218047,-14.3977505022101,17.6934196736194));
#55236=CARTESIAN_POINT('',(-51.9314271328212,-14.3981451355535,17.5565803263806));
#55237=CARTESIAN_POINT('',(-51.9306359564886,-14.3971354987959,15.5));
#55238=CARTESIAN_POINT('',(-54.1532521092111,-15.2223467977324,18.));
#55239=CARTESIAN_POINT('Ctrl Pts',(-51.929081218047,-14.3977505022101,17.6934196736194));
#55240=CARTESIAN_POINT('Ctrl Pts',(-51.9314396049108,-14.022694300038,17.7171076053695));
#55241=CARTESIAN_POINT('Ctrl Pts',(-52.1089957350005,-13.6457772873263,
17.7407955371196));
#55242=CARTESIAN_POINT('Ctrl Pts',(-52.4009425562916,-13.4106743694811,
17.7644834688697));
#55243=CARTESIAN_POINT('Ctrl Pts',(-52.7234616974047,-13.1509517569817,
17.7906519723286));
#55244=CARTESIAN_POINT('Ctrl Pts',(-53.1855836521258,-13.0642995791891,
17.8168204757875));
#55245=CARTESIAN_POINT('Ctrl Pts',(-53.5800062339574,-13.190324595469,17.8429889792464));
#55246=CARTESIAN_POINT('Ctrl Pts',(-53.974428815789,-13.3163496117488,17.8691574827054));
#55247=CARTESIAN_POINT('Ctrl Pts',(-54.3011520247311,-13.6550518221011,
17.8953259861643));
#55248=CARTESIAN_POINT('Ctrl Pts',(-54.4136991111698,-14.0527836440546,
17.9214944896232));
#55249=CARTESIAN_POINT('Ctrl Pts',(-54.5262461976084,-14.4505154660081,
17.9476629930822));
#55250=CARTESIAN_POINT('Ctrl Pts',(-54.4246171615437,-14.9072768995629,
17.9738314965411));
#55251=CARTESIAN_POINT('Ctrl Pts',(-54.153252109211,-15.2223467977324,18.));
#55252=CARTESIAN_POINT('',(-52.2352328551172,-15.2234705191484,18.));
#55253=CARTESIAN_POINT('Origin',(-53.1951359564886,-14.3971354987959,18.));
#55254=CARTESIAN_POINT('Ctrl Pts',(-52.2352228301846,-15.2234768233202,
18.));
#55255=CARTESIAN_POINT('Ctrl Pts',(-52.4934806168631,-15.521313638849,17.975091839613));
#55256=CARTESIAN_POINT('Ctrl Pts',(-52.9025313044196,-15.6908537017463,
17.950183679226));
#55257=CARTESIAN_POINT('Ctrl Pts',(-53.295440078112,-15.6595882927142,17.925275518839));
#55258=CARTESIAN_POINT('Ctrl Pts',(-53.7082298804764,-15.6267408663411,
17.89910701538));
#55259=CARTESIAN_POINT('Ctrl Pts',(-54.1032028915872,-15.3722524867282,
17.8729385119211));
#55260=CARTESIAN_POINT('Ctrl Pts',(-54.3034894678617,-15.0099588806278,
17.8467700084622));
#55261=CARTESIAN_POINT('Ctrl Pts',(-54.5037760441361,-14.6476652745275,
17.8206015050033));
#55262=CARTESIAN_POINT('Ctrl Pts',(-54.5093761855741,-14.1775664419396,
17.7944330015443));
#55263=CARTESIAN_POINT('Ctrl Pts',(-54.3176594419829,-13.8105984641279,
17.7682644980854));
#55264=CARTESIAN_POINT('Ctrl Pts',(-54.1259426983918,-13.4436304863162,
17.7420959946265));
#55265=CARTESIAN_POINT('Ctrl Pts',(-53.7369090697714,-13.1797933632805,
17.7159274911676));
#55266=CARTESIAN_POINT('Ctrl Pts',(-53.3250649526277,-13.1373263636934,
17.6897589877086));
#55267=CARTESIAN_POINT('Ctrl Pts',(-52.9132208354839,-13.0948593641063,
17.6635904842497));
#55268=CARTESIAN_POINT('Ctrl Pts',(-52.4785662298169,-13.2737624879677,
17.6374219807908));
#55269=CARTESIAN_POINT('Ctrl Pts',(-52.2159761485057,-13.5938473532063,
17.6112534773319));
#55270=CARTESIAN_POINT('Ctrl Pts',(-52.0331020154043,-13.8167622552357,
17.5930290936814));
#55271=CARTESIAN_POINT('Ctrl Pts',(-51.9336803654543,-14.1081512772947,
17.574804710031));
#55272=CARTESIAN_POINT('Ctrl Pts',(-51.9314271328212,-14.3981451355535,
17.5565803263806));
#55273=CARTESIAN_POINT('Origin',(-53.1951359564886,-14.3971354987959,19.1042117235887));
#55274=CARTESIAN_POINT('',(-51.6501838308085,-14.3978968813702,14.3957882764113));
#55275=CARTESIAN_POINT('',(-51.654536051996,-14.3970771807141,14.3542117235887));
#55276=CARTESIAN_POINT('',(-51.6521359564886,-14.3971354987959,19.1042117235887));
#55277=CARTESIAN_POINT('',(-53.5936497983459,-12.9064860705774,14.));
#55278=CARTESIAN_POINT('Ctrl Pts',(-51.654536051996,-14.3970771807141,14.3542117235887));
#55279=CARTESIAN_POINT('Ctrl Pts',(-51.6547008227736,-14.657815056409,14.3408151628949));
#55280=CARTESIAN_POINT('Ctrl Pts',(-51.8403375140876,-15.4280419867602,
14.3012500987421));
#55281=CARTESIAN_POINT('Ctrl Pts',(-53.0509994556171,-16.2080945317645,
14.2355165311303));
#55282=CARTESIAN_POINT('Ctrl Pts',(-54.6273366519326,-15.5169696210013,
14.1570110207536));
#55283=CARTESIAN_POINT('Ctrl Pts',(-54.9168336227569,-13.8187144824051,
14.0785055103768));
#55284=CARTESIAN_POINT('Ctrl Pts',(-54.083839596546,-13.0375346028626,14.0261685034589));
#55285=CARTESIAN_POINT('Ctrl Pts',(-53.5936497983459,-12.9064860705774,
14.));
#55286=CARTESIAN_POINT('',(-52.7955932879502,-12.9041246312965,14.));
#55287=CARTESIAN_POINT('Origin',(-53.1951359564886,-14.3971354987959,14.));
#55288=CARTESIAN_POINT('Ctrl Pts',(-51.6501838308085,-14.3978968813702,
14.3957882764113));
#55289=CARTESIAN_POINT('Ctrl Pts',(-51.6499084261818,-14.443250645686,14.3934410251636));
#55290=CARTESIAN_POINT('Ctrl Pts',(-51.6721169602754,-14.9939590280816,
14.3649252704569));
#55291=CARTESIAN_POINT('Ctrl Pts',(-52.3307362917628,-15.9953382094595,
14.3102410122914));
#55292=CARTESIAN_POINT('Ctrl Pts',(-54.0514987748276,-15.9998443309588,
14.2317355019146));
#55293=CARTESIAN_POINT('Ctrl Pts',(-55.0042044918326,-14.5665632650764,
14.1532299915378));
#55294=CARTESIAN_POINT('Ctrl Pts',(-54.3453458049292,-13.0076586982508,
14.0759848242329));
#55295=CARTESIAN_POINT('Ctrl Pts',(-53.2607152655111,-12.7814238100544,
14.024908160387));
#55296=CARTESIAN_POINT('Ctrl Pts',(-52.7955875161457,-12.9041113834231,
14.));
#55297=CARTESIAN_POINT('Origin',(-53.1951359564886,-14.3971354987959,19.1042117235887));
#55298=CARTESIAN_POINT('',(-51.654442242504,-14.3974618454408,14.8957882764113));
#55299=CARTESIAN_POINT('',(-51.6505063374695,-14.3961865684695,14.8542117235887));
#55300=CARTESIAN_POINT('',(-51.6521359564886,-14.3971354987959,19.1042117235887));
#55301=CARTESIAN_POINT('Ctrl Pts',(-51.6505063374695,-14.3961865684695,
14.8542117235887));
#55302=CARTESIAN_POINT('Ctrl Pts',(-51.6537531731077,-14.8418532139508,
14.8311595169817));
#55303=CARTESIAN_POINT('Ctrl Pts',(-52.0889693478694,-15.7989724624769,
14.7819388069158));
#55304=CARTESIAN_POINT('Ctrl Pts',(-53.7056220123855,-16.1409817745025,
14.706549593391));
#55305=CARTESIAN_POINT('Ctrl Pts',(-54.9313021937626,-14.9332257573755,
14.6280440830142));
#55306=CARTESIAN_POINT('Ctrl Pts',(-54.599912063137,-13.2446506074896,14.5495385726375));
#55307=CARTESIAN_POINT('Ctrl Pts',(-53.0087562916135,-12.5897333550461,
14.4710330622607));
#55308=CARTESIAN_POINT('Ctrl Pts',(-51.8276307116252,-13.3907563492144,
14.4059241125778));
#55309=CARTESIAN_POINT('Ctrl Pts',(-51.6543789636963,-14.148496272438,14.3669836663538));
#55310=CARTESIAN_POINT('Ctrl Pts',(-51.654536051996,-14.3970771807141,14.3542117235887));
#55311=CARTESIAN_POINT('Ctrl Pts',(-51.654442242504,-14.3974618454408,14.8957882764113));
#55312=CARTESIAN_POINT('Ctrl Pts',(-51.6539909131311,-14.6310322097678,
14.8837853792504));
#55313=CARTESIAN_POINT('Ctrl Pts',(-51.8127636494606,-15.3732462698704,
14.8456139786307));
#55314=CARTESIAN_POINT('Ctrl Pts',(-52.9564001587445,-16.1984187666639,
14.7812740745521));
#55315=CARTESIAN_POINT('Ctrl Pts',(-54.5659334636339,-15.5898376428623,
14.7027685641752));
#55316=CARTESIAN_POINT('Ctrl Pts',(-54.9461022318155,-13.911606374279,14.6242630537985));
#55317=CARTESIAN_POINT('Ctrl Pts',(-53.7559643179139,-12.6688223002735,
14.5457575434217));
#55318=CARTESIAN_POINT('Ctrl Pts',(-52.1134816424643,-12.9668195987494,
14.4695992842926));
#55319=CARTESIAN_POINT('Ctrl Pts',(-51.6529787949523,-13.937620862964,14.4196095286225));
#55320=CARTESIAN_POINT('Ctrl Pts',(-51.6501838308085,-14.3978968813702,
14.3957882764113));
#55321=CARTESIAN_POINT('Origin',(-53.1951359564886,-14.3971354987959,19.1042117235887));
#55322=CARTESIAN_POINT('',(-51.6512135991451,-14.3959278910795,15.3957882764113));
#55323=CARTESIAN_POINT('',(-51.6523527586964,-14.398464524594,15.3542117235887));
#55324=CARTESIAN_POINT('',(-51.6521359564886,-14.3971354987959,19.1042117235887));
#55325=CARTESIAN_POINT('Ctrl Pts',(-51.6523527586964,-14.398464524594,15.3542117235887));
#55326=CARTESIAN_POINT('Ctrl Pts',(-51.651247573785,-14.5252813221218,15.3476723745276));
#55327=CARTESIAN_POINT('Ctrl Pts',(-51.7230815929517,-15.1583461258636,
15.3149645220075));
#55328=CARTESIAN_POINT('Ctrl Pts',(-52.5930520129352,-16.1115202855033,
15.2560881660285));
#55329=CARTESIAN_POINT('Ctrl Pts',(-54.2930303473181,-15.8449779235543,
15.1775826556517));
#55330=CARTESIAN_POINT('Ctrl Pts',(-55.0083911483927,-14.2799763521069,
15.0990771452749));
#55331=CARTESIAN_POINT('Ctrl Pts',(-54.0975810662168,-12.8200452881305,
15.0205716348981));
#55332=CARTESIAN_POINT('Ctrl Pts',(-52.3774378038974,-12.7744874306393,
14.9420661245214));
#55333=CARTESIAN_POINT('Ctrl Pts',(-51.6803897960553,-13.7702239867045,
14.8866128207516));
#55334=CARTESIAN_POINT('Ctrl Pts',(-51.6500674162048,-14.3359394264926,
14.8573280204407));
#55335=CARTESIAN_POINT('Ctrl Pts',(-51.6505063374695,-14.3961865684695,
14.8542117235887));
#55336=CARTESIAN_POINT('Ctrl Pts',(-51.6512135991451,-14.3959278910795,
15.3957882764113));
#55337=CARTESIAN_POINT('Ctrl Pts',(-51.6548183273038,-14.8151512136696,
15.3741297333373));
#55338=CARTESIAN_POINT('Ctrl Pts',(-52.0463881522716,-15.7468276199561,
15.3263026868045));
#55339=CARTESIAN_POINT('Ctrl Pts',(-53.6133427309768,-16.1653895531783,
15.2523071368127));
#55340=CARTESIAN_POINT('Ctrl Pts',(-54.9007439708605,-15.0236502232965,
15.1738016264359));
#55341=CARTESIAN_POINT('Ctrl Pts',(-54.6585153839456,-13.3200374976642,
15.0952961160592));
#55342=CARTESIAN_POINT('Ctrl Pts',(-53.1038933588347,-12.5823920603089,
15.0167906056824));
#55343=CARTESIAN_POINT('Ctrl Pts',(-51.856278782321,-13.3361985618968,14.9502879924664));
#55344=CARTESIAN_POINT('Ctrl Pts',(-51.6549748934233,-14.1218062449943,
14.9099538827094));
#55345=CARTESIAN_POINT('Ctrl Pts',(-51.654442242504,-14.3974618454408,14.8957882764113));
#55346=CARTESIAN_POINT('Origin',(-53.1951359564886,-14.3971354987959,19.1042117235887));
#55347=CARTESIAN_POINT('',(-51.6515662259554,-14.3984147593818,15.8957882764113));
#55348=CARTESIAN_POINT('',(-51.6539634663413,-14.3962637929782,15.8542117235887));
#55349=CARTESIAN_POINT('',(-51.6521359564886,-14.3971354987959,19.1042117235887));
#55350=CARTESIAN_POINT('Ctrl Pts',(-51.6539634663413,-14.3962637929782,
15.8542117235887));
#55351=CARTESIAN_POINT('Ctrl Pts',(-51.6556220588241,-14.7111646038003,
15.8380167286145));
#55352=CARTESIAN_POINT('Ctrl Pts',(-51.9015651465377,-15.5372739892809,
15.7956532301813));
#55353=CARTESIAN_POINT('Ctrl Pts',(-53.2428638938474,-16.2135446545079,
15.7271212282891));
#55354=CARTESIAN_POINT('Ctrl Pts',(-54.7365592022647,-15.3592345303502,
15.6486157179124));
#55355=CARTESIAN_POINT('Ctrl Pts',(-54.8478695024322,-13.6420911264981,
15.5701102075356));
#55356=CARTESIAN_POINT('Ctrl Pts',(-53.4769690594307,-12.6020894569994,
15.4916046971588));
#55357=CARTESIAN_POINT('Ctrl Pts',(-51.9885611628803,-13.1244613999964,
15.4196385358432));
#55358=CARTESIAN_POINT('Ctrl Pts',(-51.6556701906089,-14.0177987311608,
15.3738408779865));
#55359=CARTESIAN_POINT('Ctrl Pts',(-51.6523527586964,-14.398464524594,15.3542117235887));
#55360=CARTESIAN_POINT('Ctrl Pts',(-51.6515662259554,-14.3984147593818,
15.8957882764113));
#55361=CARTESIAN_POINT('Ctrl Pts',(-51.6506843931331,-14.4980737158535,
15.8906425908832));
#55362=CARTESIAN_POINT('Ctrl Pts',(-51.7045173377561,-15.1036026015034,
15.8593284018961));
#55363=CARTESIAN_POINT('Ctrl Pts',(-52.503850750664,-16.077535486755,15.8018457094502));
#55364=CARTESIAN_POINT('Ctrl Pts',(-54.2154808300007,-15.9006366439348,
15.7233401990734));
#55365=CARTESIAN_POINT('Ctrl Pts',(-55.0120413695279,-14.3753622311824,
15.6448346886966));
#55366=CARTESIAN_POINT('Ctrl Pts',(-54.1791579400319,-12.8696146010229,
15.5663291783198));
#55367=CARTESIAN_POINT('Ctrl Pts',(-52.4637802022359,-12.7337840295961,
15.4878236679431));
#55368=CARTESIAN_POINT('Ctrl Pts',(-51.6965951513913,-13.7156125454117,
15.4309767006402));
#55369=CARTESIAN_POINT('Ctrl Pts',(-51.6504629862743,-14.3086329806648,
15.4002982367963));
#55370=CARTESIAN_POINT('Ctrl Pts',(-51.6512135991451,-14.3959278910795,
15.3957882764113));
#55371=CARTESIAN_POINT('Origin',(-53.1951359564886,-14.3971354987959,19.1042117235887));
#55372=CARTESIAN_POINT('',(-51.65433991327,-14.3966252656123,16.3957882764113));
#55373=CARTESIAN_POINT('',(-51.6497037375007,-14.3970262778732,16.3542117235887));
#55374=CARTESIAN_POINT('',(-51.6521359564886,-14.3971354987959,19.1042117235887));
#55375=CARTESIAN_POINT('Ctrl Pts',(-51.6497037375007,-14.3970262778732,
16.3542117235887));
#55376=CARTESIAN_POINT('Ctrl Pts',(-51.6502234542653,-14.8961053696861,
16.3283610827014));
#55377=CARTESIAN_POINT('Ctrl Pts',(-52.1817212113122,-15.9013530800272,
16.2763419383551));
#55378=CARTESIAN_POINT('Ctrl Pts',(-53.8864212481312,-16.0775356953633,
16.1981542905498));
#55379=CARTESIAN_POINT('Ctrl Pts',(-54.978090456054,-14.7474117142528,16.119648780173));
#55380=CARTESIAN_POINT('Ctrl Pts',(-54.4707636814861,-13.1031516960174,
16.0411432697963));
#55381=CARTESIAN_POINT('Ctrl Pts',(-52.8194236367236,-12.6193671146013,
15.9626377594195));
#55382=CARTESIAN_POINT('Ctrl Pts',(-51.7761788820818,-13.5008286667841,
15.900327244017));
#55383=CARTESIAN_POINT('Ctrl Pts',(-51.6529420405103,-14.2023356124785,
15.8641852320734));
#55384=CARTESIAN_POINT('Ctrl Pts',(-51.6539634663413,-14.3962637929782,
15.8542117235887));
#55385=CARTESIAN_POINT('Ctrl Pts',(-51.65433991327,-14.3966252656123,16.3957882764113));
#55386=CARTESIAN_POINT('Ctrl Pts',(-51.6552138153438,-14.684603767973,16.3809869449701));
#55387=CARTESIAN_POINT('Ctrl Pts',(-51.869991852728,-15.4829338669789,16.3400171100699));
#55388=CARTESIAN_POINT('Ctrl Pts',(-53.1474080250528,-16.2135444290179,
16.2728787717108));
#55389=CARTESIAN_POINT('Ctrl Pts',(-54.6839066935018,-15.4388557336608,
16.1943732613341));
#55390=CARTESIAN_POINT('Ctrl Pts',(-54.8852403705632,-13.7299275672916,
16.1158677509573));
#55391=CARTESIAN_POINT('Ctrl Pts',(-53.570848229612,-12.6193673352972,16.0373622405805));
#55392=CARTESIAN_POINT('Ctrl Pts',(-52.0277463399596,-13.0714419423033,
15.9640024157318));
#55393=CARTESIAN_POINT('Ctrl Pts',(-51.6551689744654,-13.9912557743182,
15.9168110943421));
#55394=CARTESIAN_POINT('Ctrl Pts',(-51.6515662259554,-14.3984147593818,
15.8957882764113));
#55395=CARTESIAN_POINT('Origin',(-53.1951359564886,-14.3971354987959,19.1042117235887));
#55396=CARTESIAN_POINT('',(-51.6499660613832,-14.3965688093956,16.8957882764113));
#55397=CARTESIAN_POINT('',(-51.6537286904076,-14.3981451166365,16.8542117235887));
#55398=CARTESIAN_POINT('',(-51.6521359564886,-14.3971354987959,19.1042117235887));
#55399=CARTESIAN_POINT('Ctrl Pts',(-51.6537286904076,-14.3981451166365,
16.8542117235887));
#55400=CARTESIAN_POINT('Ctrl Pts',(-51.6526099457396,-14.5796423938349,
16.8448739402472));
#55401=CARTESIAN_POINT('Ctrl Pts',(-51.7655324660036,-15.2684267173499,
16.8093676534467));
#55402=CARTESIAN_POINT('Ctrl Pts',(-52.7769291300874,-16.1653897727513,
16.7476928631873));
#55403=CARTESIAN_POINT('Ctrl Pts',(-54.4393883485545,-15.72131682132,16.6691873528105));
#55404=CARTESIAN_POINT('Ctrl Pts',(-54.9859724441167,-14.0896865557083,
16.5906818424337));
#55405=CARTESIAN_POINT('Ctrl Pts',(-53.9264918015333,-12.7337838230954,
16.5121763320569));
#55406=CARTESIAN_POINT('Ctrl Pts',(-52.2111138507866,-12.8696144113969,
16.4336708216802));
#55407=CARTESIAN_POINT('Ctrl Pts',(-51.6524858829682,-13.8795429426784,
16.3810159521908));
#55408=CARTESIAN_POINT('Ctrl Pts',(-51.6496973470012,-14.3908895416808,
16.3545295861603));
#55409=CARTESIAN_POINT('Ctrl Pts',(-51.6497037375007,-14.3970262778732,
16.3542117235887));
#55410=CARTESIAN_POINT('Ctrl Pts',(-51.6499660613832,-14.3965688093956,
16.8957882764113));
#55411=CARTESIAN_POINT('Ctrl Pts',(-51.6522282000482,-14.8689560438918,
16.8713312990569));
#55412=CARTESIAN_POINT('Ctrl Pts',(-52.1343035201106,-15.8507887260607,
16.8207058182437));
#55413=CARTESIAN_POINT('Ctrl Pts',(-53.7972198251955,-16.11152007286,16.7439118339715));
#55414=CARTESIAN_POINT('Ctrl Pts',(-54.9572349488979,-14.8405614110472,
16.6654063235947));
#55415=CARTESIAN_POINT('Ctrl Pts',(-54.5369577413632,-13.1719279226262,
16.586900813218));
#55416=CARTESIAN_POINT('Ctrl Pts',(-52.9133028885493,-12.602089679815,16.5083953028412));
#55417=CARTESIAN_POINT('Ctrl Pts',(-51.8008704508192,-13.4460106212472,
16.4446911239056));
#55418=CARTESIAN_POINT('Ctrl Pts',(-51.6536687712691,-14.1754626501585,
16.407155448429));
#55419=CARTESIAN_POINT('Ctrl Pts',(-51.65433991327,-14.3966252656123,16.3957882764113));
#55420=CARTESIAN_POINT('Origin',(-53.1951359564886,-14.3971354987959,19.1042117235887));
#55421=CARTESIAN_POINT('',(-51.6531013855762,-14.3983675031589,17.3957882764113));
#55422=CARTESIAN_POINT('',(-51.652701124777,-14.3958311332085,17.3542117235887));
#55423=CARTESIAN_POINT('',(-51.6521359564886,-14.3971354987959,19.1042117235887));
#55424=CARTESIAN_POINT('Ctrl Pts',(-51.652701124777,-14.3958311332085,17.3542117235887));
#55425=CARTESIAN_POINT('Ctrl Pts',(-51.6557877520943,-14.7643809445978,
17.3352182943341));
#55426=CARTESIAN_POINT('Ctrl Pts',(-51.9714428864125,-15.6454595543576,
17.2900563616205));
#55427=CARTESIAN_POINT('Ctrl Pts',(-53.4338717842849,-16.1984189929661,
17.218725925448));
#55428=CARTESIAN_POINT('Ctrl Pts',(-54.829300954394,-15.1915695541269,17.1402204150712));
#55429=CARTESIAN_POINT('Ctrl Pts',(-54.7591722875713,-13.4722511753948,
17.0617149046944));
#55430=CARTESIAN_POINT('Ctrl Pts',(-53.2863785654275,-12.582391834622,16.9832093943176));
#55431=CARTESIAN_POINT('Ctrl Pts',(-51.9166698060745,-13.232298629585,16.9140416672824));
#55432=CARTESIAN_POINT('Ctrl Pts',(-51.6557451516705,-14.0710086043769,
16.8710424437061));
#55433=CARTESIAN_POINT('Ctrl Pts',(-51.6537286904076,-14.3981451166365,
16.8542117235887));
#55434=CARTESIAN_POINT('Ctrl Pts',(-51.6531013855762,-14.3983675031589,
17.3957882764113));
#55435=CARTESIAN_POINT('Ctrl Pts',(-51.6519028634371,-14.5526188015874,
17.3878441566028));
#55436=CARTESIAN_POINT('Ctrl Pts',(-51.7435010772427,-15.2135959185484,
17.3537315333353));
#55437=CARTESIAN_POINT('Ctrl Pts',(-52.6846499703254,-16.1409815416267,
17.293450406609));
#55438=CARTESIAN_POINT('Ctrl Pts',(-54.3681285487899,-15.7848349642756,
17.2149448962322));
#55439=CARTESIAN_POINT('Ctrl Pts',(-54.9996481235109,-14.1841565112764,
17.1364393858554));
#55440=CARTESIAN_POINT('Ctrl Pts',(-54.0128340063977,-12.7744876345319,
17.0579338754786));
#55441=CARTESIAN_POINT('Ctrl Pts',(-52.292690959438,-12.8200454826231,16.9794283651019));
#55442=CARTESIAN_POINT('Ctrl Pts',(-51.6656274258073,-13.8251612032116,
16.9253798320794));
#55443=CARTESIAN_POINT('Ctrl Pts',(-51.6498077544378,-14.3635106325159,
16.8974998025159));
#55444=CARTESIAN_POINT('Ctrl Pts',(-51.6499660613832,-14.3965688093956,
16.8957882764113));
#55445=CARTESIAN_POINT('Origin',(-53.1951359564886,-14.3971354987959,19.1042117235887));
#55446=CARTESIAN_POINT('',(-51.6537934596095,-14.3955992295121,17.8957882764113));
#55447=CARTESIAN_POINT('',(-51.650238794436,-14.3978859537331,17.8542117235887));
#55448=CARTESIAN_POINT('',(-51.6521359564886,-14.3971354987959,19.1042117235887));
#55449=CARTESIAN_POINT('',(-52.7966221146314,-12.9064860705774,18.));
#55450=CARTESIAN_POINT('Ctrl Pts',(-52.7966221146314,-12.9064860705774,
18.));
#55451=CARTESIAN_POINT('Ctrl Pts',(-52.3064323164313,-13.0375346028627,
17.9738314965411));
#55452=CARTESIAN_POINT('Ctrl Pts',(-51.7535553056072,-13.5560194656624,
17.9390942553448));
#55453=CARTESIAN_POINT('Ctrl Pts',(-51.6526562271057,-14.2291272515896,
17.9043570141486));
#55454=CARTESIAN_POINT('Ctrl Pts',(-51.6537934596095,-14.3955992295121,
17.8957882764113));
#55455=CARTESIAN_POINT('',(-53.5946788045247,-12.9041246263415,18.));
#55456=CARTESIAN_POINT('Origin',(-53.1951359564886,-14.3971354987959,18.));
#55457=CARTESIAN_POINT('Ctrl Pts',(-53.5946845822246,-12.9041113672218,
18.));
#55458=CARTESIAN_POINT('Ctrl Pts',(-53.1295569761736,-12.7814239312717,
17.975091839613));
#55459=CARTESIAN_POINT('Ctrl Pts',(-52.0976014587089,-12.9966708391238,
17.9264957474759));
#55460=CARTESIAN_POINT('Ctrl Pts',(-51.6531166045831,-13.9402254397343,
17.8778996553388));
#55461=CARTESIAN_POINT('Ctrl Pts',(-51.650238794436,-14.3978859537331,17.8542117235887));
#55462=CARTESIAN_POINT('Origin',(-14.1292828945604,-53.2669068454841,15.5));
#55463=CARTESIAN_POINT('',(-13.4980577522812,-52.1734972976427,14.1934196736194));
#55464=CARTESIAN_POINT('',(-13.4988747128346,-52.1716629874611,14.0565803263806));
#55465=CARTESIAN_POINT('',(-13.4970328945604,-52.1718177223987,15.5));
#55466=CARTESIAN_POINT('',(-12.9355708698302,-52.8497595669186,14.));
#55467=CARTESIAN_POINT('Ctrl Pts',(-13.4988747128346,-52.1716629874611,
14.0565803263806));
#55468=CARTESIAN_POINT('Ctrl Pts',(-13.2411227471438,-52.3234873105789,
14.0377202175871));
#55469=CARTESIAN_POINT('Ctrl Pts',(-13.0344360750677,-52.5668460963448,
14.0188601087935));
#55470=CARTESIAN_POINT('Ctrl Pts',(-12.9355708698302,-52.8497595669186,
14.));
#55471=CARTESIAN_POINT('',(-13.4970328945604,-52.1718177223987,14.));
#55472=CARTESIAN_POINT('Origin',(-14.1292828945604,-53.2669068454841,14.));
#55473=CARTESIAN_POINT('',(-13.4970328945604,-52.1718177223987,13.));
#55474=CARTESIAN_POINT('',(-13.4970328945604,-52.1718177223987,15.5));
#55475=CARTESIAN_POINT('',(-12.8669333849943,-53.3406222827979,13.));
#55476=CARTESIAN_POINT('Origin',(-14.1292828945604,-53.2669068454841,13.));
#55477=CARTESIAN_POINT('',(-15.3916324041264,-53.1931914081703,13.));
#55478=CARTESIAN_POINT('Origin',(-14.1292828945604,-53.2669068454841,13.));
#55479=CARTESIAN_POINT('Origin',(-14.1292828945604,-53.2669068454841,13.));
#55480=CARTESIAN_POINT('',(-13.8936073831511,-54.5113748561459,14.));
#55481=CARTESIAN_POINT('Origin',(-14.1292828945604,-53.2669068454841,14.));
#55482=CARTESIAN_POINT('Ctrl Pts',(-13.8936069362009,-54.5113866946539,
14.));
#55483=CARTESIAN_POINT('Ctrl Pts',(-13.5065438623107,-54.43664727626,14.024908160387));
#55484=CARTESIAN_POINT('Ctrl Pts',(-13.1551923299505,-54.1671690811723,
14.049816320774));
#55485=CARTESIAN_POINT('Ctrl Pts',(-12.9858145310894,-53.8112673891924,
14.074724481161));
#55486=CARTESIAN_POINT('Ctrl Pts',(-12.8078662825437,-53.43735721225,14.10089298462));
#55487=CARTESIAN_POINT('Ctrl Pts',(-12.8307732764863,-52.9680562770306,
14.1270614880789));
#55488=CARTESIAN_POINT('Ctrl Pts',(-13.0443854893126,-52.6134561814805,
14.1532299915378));
#55489=CARTESIAN_POINT('Ctrl Pts',(-13.1537409585152,-52.4319241458581,
14.1666265522317));
#55490=CARTESIAN_POINT('Ctrl Pts',(-13.3130758736166,-52.2804525587351,
14.1800231129255));
#55491=CARTESIAN_POINT('Ctrl Pts',(-13.4980577522812,-52.1734972976427,
14.1934196736194));
#55492=CARTESIAN_POINT('Origin',(-14.1292828945604,-53.2669068454841,15.5));
#55493=CARTESIAN_POINT('',(-13.4970386657413,-52.17027240687,14.6934196736194));
#55494=CARTESIAN_POINT('',(-13.4956926805926,-52.1707443397673,14.5565803263806));
#55495=CARTESIAN_POINT('',(-13.4970328945604,-52.1718177223987,15.5));
#55496=CARTESIAN_POINT('Ctrl Pts',(-13.4956926805926,-52.1707443397673,
14.5565803263806));
#55497=CARTESIAN_POINT('Ctrl Pts',(-13.4633916214762,-52.1891327536446,
14.5542330751329));
#55498=CARTESIAN_POINT('Ctrl Pts',(-13.4319685470764,-52.2090047577526,
14.5518858238852));
#55499=CARTESIAN_POINT('Ctrl Pts',(-13.4015745144389,-52.230342308046,14.5495385726375));
#55500=CARTESIAN_POINT('Ctrl Pts',(-13.0627244024285,-52.4682255594459,
14.5233700691785));
#55501=CARTESIAN_POINT('Ctrl Pts',(-12.8517746061391,-52.8882625646258,
14.4972015657196));
#55502=CARTESIAN_POINT('Ctrl Pts',(-12.8632814695834,-53.3021304033103,
14.4710330622607));
#55503=CARTESIAN_POINT('Ctrl Pts',(-12.8747883330278,-53.7159982419948,
14.4448645588017));
#55504=CARTESIAN_POINT('Ctrl Pts',(-13.1087518562058,-54.1236969141839,
14.4186960553428));
#55505=CARTESIAN_POINT('Ctrl Pts',(-13.460332770227,-54.3423556782117,14.3925275518839));
#55506=CARTESIAN_POINT('Ctrl Pts',(-13.8119136842483,-54.5610144422395,
14.366359048425));
#55507=CARTESIAN_POINT('Ctrl Pts',(-14.2811119891127,-54.5906332981061,
14.3401905449661));
#55508=CARTESIAN_POINT('Ctrl Pts',(-14.6573867068862,-54.4180393977442,
14.3140220415071));
#55509=CARTESIAN_POINT('Ctrl Pts',(-15.0336614246597,-54.2454454973823,
14.2878535380482));
#55510=CARTESIAN_POINT('Ctrl Pts',(-15.3170125553423,-53.8706388407919,
14.2616850345893));
#55511=CARTESIAN_POINT('Ctrl Pts',(-15.3806795111647,-53.4614679031089,
14.2355165311303));
#55512=CARTESIAN_POINT('Ctrl Pts',(-15.4443464669872,-53.052296965426,14.2093480276714));
#55513=CARTESIAN_POINT('Ctrl Pts',(-15.2883292479495,-52.6087617466505,
14.1831795242125));
#55514=CARTESIAN_POINT('Ctrl Pts',(-14.981976715725,-52.3301941698058,14.1570110207536));
#55515=CARTESIAN_POINT('Ctrl Pts',(-14.6756241835005,-52.0516265929611,
14.1308425172946));
#55516=CARTESIAN_POINT('Ctrl Pts',(-14.2189363380893,-51.938026658047,14.1046740138357));
#55517=CARTESIAN_POINT('Ctrl Pts',(-13.8182170120758,-52.0394239070104,
14.0785055103768));
#55518=CARTESIAN_POINT('Ctrl Pts',(-13.7063032761926,-52.067742343889,14.0711971157114));
#55519=CARTESIAN_POINT('Ctrl Pts',(-13.5987550004656,-52.1128302370619,
14.063888721046));
#55520=CARTESIAN_POINT('Ctrl Pts',(-13.4988747128346,-52.1716629874611,
14.0565803263806));
#55521=CARTESIAN_POINT('Ctrl Pts',(-13.4980577522812,-52.1734972976427,
14.1934196736194));
#55522=CARTESIAN_POINT('Ctrl Pts',(-13.6744148054729,-52.0715288518372,
14.2061916163845));
#55523=CARTESIAN_POINT('Ctrl Pts',(-13.8740829845724,-52.0100223374604,
14.2189635591495));
#55524=CARTESIAN_POINT('Ctrl Pts',(-14.0759771073047,-52.00150441778,14.2317355019146));
#55525=CARTESIAN_POINT('Ctrl Pts',(-14.4896390807605,-51.9840520055104,
14.2579040053735));
#55526=CARTESIAN_POINT('Ctrl Pts',(-14.9126455959621,-52.189046436852,14.2840725088324));
#55527=CARTESIAN_POINT('Ctrl Pts',(-15.1553451745865,-52.5244804183786,
14.3102410122914));
#55528=CARTESIAN_POINT('Ctrl Pts',(-15.3980447532108,-52.8599143999053,
14.3364095157503));
#55529=CARTESIAN_POINT('Ctrl Pts',(-15.460437395258,-53.325787931617,14.3625780192092));
#55530=CARTESIAN_POINT('Ctrl Pts',(-15.3145307999442,-53.7132400695012,
14.3887465226681));
#55531=CARTESIAN_POINT('Ctrl Pts',(-15.1686242046305,-54.1006922073853,
14.4149150261271));
#55532=CARTESIAN_POINT('Ctrl Pts',(-14.8144183719558,-54.4097229514419,
14.441083529586));
#55533=CARTESIAN_POINT('Ctrl Pts',(-14.4107506896372,-54.5017382932332,
14.4672520330449));
#55534=CARTESIAN_POINT('Ctrl Pts',(-14.0070830073185,-54.5937536350245,
14.4934205365038));
#55535=CARTESIAN_POINT('Ctrl Pts',(-13.5539534753558,-54.4687535745504,
14.5195890399628));
#55536=CARTESIAN_POINT('Ctrl Pts',(-13.2545471544402,-54.1828000037796,
14.5457575434217));
#55537=CARTESIAN_POINT('Ctrl Pts',(-12.9551408335246,-53.8968464330088,
14.5719260468806));
#55538=CARTESIAN_POINT('Ctrl Pts',(-12.8094577236562,-53.4499393519412,
14.5980945503396));
#55539=CARTESIAN_POINT('Ctrl Pts',(-12.8828256503828,-53.0424720659447,
14.6242630537985));
#55540=CARTESIAN_POINT('Ctrl Pts',(-12.9474564997503,-52.6835283427349,
14.6473152604055));
#55541=CARTESIAN_POINT('Ctrl Pts',(-13.1820731109759,-52.3551902889475,
14.6703674670124));
#55542=CARTESIAN_POINT('Ctrl Pts',(-13.4970386657413,-52.17027240687,14.6934196736194));
#55543=CARTESIAN_POINT('Origin',(-14.1292828945604,-53.2669068454841,15.5));
#55544=CARTESIAN_POINT('',(-13.496178545612,-52.1725162395268,15.1934196736194));
#55545=CARTESIAN_POINT('',(-13.4977463410386,-52.1735883352515,15.0565803263806));
#55546=CARTESIAN_POINT('',(-13.4970328945604,-52.1718177223987,15.5));
#55547=CARTESIAN_POINT('Ctrl Pts',(-13.4977463410386,-52.1735883352515,
15.0565803263806));
#55548=CARTESIAN_POINT('Ctrl Pts',(-13.3317931989842,-52.2689743399828,
15.0445774292198));
#55549=CARTESIAN_POINT('Ctrl Pts',(-13.186612163033,-52.4000385957214,15.0325745320589));
#55550=CARTESIAN_POINT('Ctrl Pts',(-13.080217915627,-52.5573375001258,15.0205716348981));
#55551=CARTESIAN_POINT('Ctrl Pts',(-12.8482590648636,-52.9002777810298,
14.9944031314392));
#55552=CARTESIAN_POINT('Ctrl Pts',(-12.800661371336,-53.3679164545857,14.9682346279803));
#55553=CARTESIAN_POINT('Ctrl Pts',(-12.9587676726969,-53.7505591757409,
14.9420661245214));
#55554=CARTESIAN_POINT('Ctrl Pts',(-13.1168739740577,-54.1332018968962,
14.9158976210624));
#55555=CARTESIAN_POINT('Ctrl Pts',(-13.480684270307,-54.4308486656509,14.8897291176035));
#55556=CARTESIAN_POINT('Ctrl Pts',(-13.887062777462,-54.5100303359216,14.8635606141446));
#55557=CARTESIAN_POINT('Ctrl Pts',(-14.2934412846171,-54.5892120061924,
14.8373921106856));
#55558=CARTESIAN_POINT('Ctrl Pts',(-14.742388002678,-54.4499285779793,14.8112236072267));
#55559=CARTESIAN_POINT('Ctrl Pts',(-15.0325877125755,-54.1546380042325,
14.7850551037678));
#55560=CARTESIAN_POINT('Ctrl Pts',(-15.322787422473,-53.8593474304858,14.7588866003089));
#55561=CARTESIAN_POINT('Ctrl Pts',(-15.4542401242072,-53.4080497112054,
14.7327180968499));
#55562=CARTESIAN_POINT('Ctrl Pts',(-15.3680052510694,-53.0031088631455,
14.706549593391));
#55563=CARTESIAN_POINT('Ctrl Pts',(-15.2817703779317,-52.5981680150855,
14.6803810899321));
#55564=CARTESIAN_POINT('Ctrl Pts',(-14.9778479299221,-52.239584038246,14.6542125864732));
#55565=CARTESIAN_POINT('Ctrl Pts',(-14.5925114920515,-52.0881567986362,
14.6280440830142));
#55566=CARTESIAN_POINT('Ctrl Pts',(-14.2417387974229,-51.9503122148962,
14.604222830803));
#55567=CARTESIAN_POINT('Ctrl Pts',(-13.8235023586796,-51.9841281668449,
14.5804015785918));
#55568=CARTESIAN_POINT('Ctrl Pts',(-13.4956926805926,-52.1707443397673,
14.5565803263806));
#55569=CARTESIAN_POINT('Ctrl Pts',(-13.4970386657413,-52.17027240687,14.6934196736194));
#55570=CARTESIAN_POINT('Ctrl Pts',(-13.5396170697753,-52.1452744089077,
14.6965359704714));
#55571=CARTESIAN_POINT('Ctrl Pts',(-13.5836638346913,-52.1228973859148,
14.6996522673233));
#55572=CARTESIAN_POINT('Ctrl Pts',(-13.6289575157408,-52.1034200423295,
14.7027685641752));
#55573=CARTESIAN_POINT('Ctrl Pts',(-14.0093024910506,-51.9398627956363,
14.7289370676342));
#55574=CARTESIAN_POINT('Ctrl Pts',(-14.4775734783483,-51.9807757931753,
14.7551055710931));
#55575=CARTESIAN_POINT('Ctrl Pts',(-14.823792639393,-52.2078118983851,14.781274074552));
#55576=CARTESIAN_POINT('Ctrl Pts',(-15.1700118004377,-52.434848003595,14.807442578011));
#55577=CARTESIAN_POINT('Ctrl Pts',(-15.3941791352293,-52.8480072164757,
14.8336110814699));
#55578=CARTESIAN_POINT('Ctrl Pts',(-15.3957751288567,-53.2620246601267,
14.8597795849288));
#55579=CARTESIAN_POINT('Ctrl Pts',(-15.3973711224841,-53.6760421037777,
14.8859480883877));
#55580=CARTESIAN_POINT('Ctrl Pts',(-15.1763957749473,-54.0909177781991,
14.9121165918467));
#55581=CARTESIAN_POINT('Ctrl Pts',(-14.83193716646,-54.3206161896323,14.9382850953056));
#55582=CARTESIAN_POINT('Ctrl Pts',(-14.4874785579727,-54.5503146010655,
14.9644535987645));
#55583=CARTESIAN_POINT('Ctrl Pts',(-14.0195366885349,-54.5948357495104,
14.9906221022235));
#55584=CARTESIAN_POINT('Ctrl Pts',(-13.6379422013928,-54.4342159762724,
15.0167906056824));
#55585=CARTESIAN_POINT('Ctrl Pts',(-13.2563477142508,-54.2735962030343,
15.0429591091413));
#55586=CARTESIAN_POINT('Ctrl Pts',(-12.9611006094046,-53.9078355081131,
15.0691276126002));
#55587=CARTESIAN_POINT('Ctrl Pts',(-12.8845932246477,-53.5009452588027,
15.0952961160591));
#55588=CARTESIAN_POINT('Ctrl Pts',(-12.8080858398908,-53.0940550094922,
15.1214646195181));
#55589=CARTESIAN_POINT('Ctrl Pts',(-12.9503181752232,-52.6460352057925,
15.147633122977));
#55590=CARTESIAN_POINT('Ctrl Pts',(-13.2475115476967,-52.3577832908858,
15.1738016264359));
#55591=CARTESIAN_POINT('Ctrl Pts',(-13.3217783549033,-52.2857508992711,
15.1803409754971));
#55592=CARTESIAN_POINT('Ctrl Pts',(-13.4057220070297,-52.2236955258253,
15.1868803245583));
#55593=CARTESIAN_POINT('Ctrl Pts',(-13.496178545612,-52.1725162395268,15.1934196736194));
#55594=CARTESIAN_POINT('Origin',(-14.1292828945604,-53.2669068454841,15.5));
#55595=CARTESIAN_POINT('',(-13.4984004295476,-52.1727576237481,15.6934196736194));
#55596=CARTESIAN_POINT('',(-13.4975120618698,-52.1706683776322,15.5565803263806));
#55597=CARTESIAN_POINT('',(-13.4970328945604,-52.1718177223987,15.5));
#55598=CARTESIAN_POINT('Ctrl Pts',(-13.4975120618698,-52.1706683776322,
15.5565803263806));
#55599=CARTESIAN_POINT('Ctrl Pts',(-13.2014603606288,-52.3450050094651,
15.5349217833067));
#55600=CARTESIAN_POINT('Ctrl Pts',(-12.9746829017777,-52.6437331734245,
15.5132632402327));
#55601=CARTESIAN_POINT('Ctrl Pts',(-12.8963324343974,-52.9773225319626,
15.4916046971588));
#55602=CARTESIAN_POINT('Ctrl Pts',(-12.8016670421015,-53.3803752328285,
15.4654361936999));
#55603=CARTESIAN_POINT('Ctrl Pts',(-12.9236783333193,-53.8343190010791,
15.439267690241));
#55604=CARTESIAN_POINT('Ctrl Pts',(-13.2076549868355,-54.1356000609316,
15.413099186782));
#55605=CARTESIAN_POINT('Ctrl Pts',(-13.4916316403516,-54.4368811207841,
15.3869306833231));
#55606=CARTESIAN_POINT('Ctrl Pts',(-13.9375736561661,-54.5854994722384,
15.3607621798642));
#55607=CARTESIAN_POINT('Ctrl Pts',(-14.3455153495114,-54.5148128681013,
15.3345936764052));
#55608=CARTESIAN_POINT('Ctrl Pts',(-14.7534570428566,-54.4441262639641,
15.3084251729463));
#55609=CARTESIAN_POINT('Ctrl Pts',(-15.1233984137326,-54.1541347042354,
15.2822566694874));
#55610=CARTESIAN_POINT('Ctrl Pts',(-15.2894533218141,-53.7748738751901,
15.2560881660285));
#55611=CARTESIAN_POINT('Ctrl Pts',(-15.4555082298957,-53.3956130461449,
15.2299196625696));
#55612=CARTESIAN_POINT('Ctrl Pts',(-15.4176766751828,-52.9270829477831,
15.2037511591106));
#55613=CARTESIAN_POINT('Ctrl Pts',(-15.1929228414795,-52.579377997485,15.1775826556517));
#55614=CARTESIAN_POINT('Ctrl Pts',(-14.9681690077762,-52.2316730471868,
15.1514141521928));
#55615=CARTESIAN_POINT('Ctrl Pts',(-14.5564928950826,-52.0047932449524,
15.1252456487338));
#55616=CARTESIAN_POINT('Ctrl Pts',(-14.1424948347361,-52.0004742879611,
15.0990771452749));
#55617=CARTESIAN_POINT('Ctrl Pts',(-13.9183882655449,-51.9981363382785,
15.0849115389768));
#55618=CARTESIAN_POINT('Ctrl Pts',(-13.6936012952867,-52.0610154646128,
15.0707459326787));
#55619=CARTESIAN_POINT('Ctrl Pts',(-13.4977463410386,-52.1735883352515,
15.0565803263806));
#55620=CARTESIAN_POINT('Ctrl Pts',(-13.496178545612,-52.1725162395268,15.1934196736194));
#55621=CARTESIAN_POINT('Ctrl Pts',(-13.7677018035866,-52.018891451597,15.2130488280172));
#55622=CARTESIAN_POINT('Ctrl Pts',(-14.0979074320564,-51.9632623188715,
15.2326779824149));
#55623=CARTESIAN_POINT('Ctrl Pts',(-14.4012233710796,-52.0299449584561,
15.2523071368127));
#55624=CARTESIAN_POINT('Ctrl Pts',(-14.8055874123741,-52.1188425670469,
15.2784756402716));
#55625=CARTESIAN_POINT('Ctrl Pts',(-15.1621610853483,-52.4251218103423,
15.3046441437306));
#55626=CARTESIAN_POINT('Ctrl Pts',(-15.3110525132995,-52.8114434442094,
15.3308126471895));
#55627=CARTESIAN_POINT('Ctrl Pts',(-15.4599439412506,-53.1977650780765,
15.3569811506484));
#55628=CARTESIAN_POINT('Ctrl Pts',(-15.4011531241786,-53.6641291025153,
15.3831496541074));
#55629=CARTESIAN_POINT('Ctrl Pts',(-15.1610425648871,-54.0014123408011,
15.4093181575663));
#55630=CARTESIAN_POINT('Ctrl Pts',(-14.9209320055955,-54.338695579087,15.4354866610252));
#55631=CARTESIAN_POINT('Ctrl Pts',(-14.4995017040844,-54.5468980312198,
15.4616551644841));
#55632=CARTESIAN_POINT('Ctrl Pts',(-14.0857260162278,-54.5326592450683,
15.487823667943));
#55633=CARTESIAN_POINT('Ctrl Pts',(-13.6719503283713,-54.5184204589168,
15.513992171402));
#55634=CARTESIAN_POINT('Ctrl Pts',(-13.2658292541693,-54.2817404344808,
15.5401606748609));
#55635=CARTESIAN_POINT('Ctrl Pts',(-13.0494723111738,-53.9287493069654,
15.5663291783198));
#55636=CARTESIAN_POINT('Ctrl Pts',(-12.8331153681783,-53.5757581794499,
15.5924976817788));
#55637=CARTESIAN_POINT('Ctrl Pts',(-12.8065225563893,-53.1064559488549,
15.6186661852377));
#55638=CARTESIAN_POINT('Ctrl Pts',(-12.9816184085214,-52.7312833144481,
15.6448346886966));
#55639=CARTESIAN_POINT('Ctrl Pts',(-13.0899806023986,-52.4990988894489,
15.6610296836709));
#55640=CARTESIAN_POINT('Ctrl Pts',(-13.2755904595332,-52.3029665221486,
15.6772246786451));
#55641=CARTESIAN_POINT('Ctrl Pts',(-13.4984004295476,-52.1727576237481,
15.6934196736194));
#55642=CARTESIAN_POINT('Origin',(-14.1292828945604,-53.2669068454841,15.5));
#55643=CARTESIAN_POINT('',(-13.4961138435274,-52.1700468646075,16.1934196736194));
#55644=CARTESIAN_POINT('',(-13.4958915862188,-52.1719376453661,16.0565803263806));
#55645=CARTESIAN_POINT('',(-13.4970328945604,-52.1718177223987,15.5));
#55646=CARTESIAN_POINT('Ctrl Pts',(-13.4958915862188,-52.1719376453661,
16.0565803263806));
#55647=CARTESIAN_POINT('Ctrl Pts',(-13.4248008737561,-52.2121474216226,
16.0514346408525));
#55648=CARTESIAN_POINT('Ctrl Pts',(-13.3578067644458,-52.2591973943854,
16.0462889553244));
#55649=CARTESIAN_POINT('Ctrl Pts',(-13.2964716828247,-52.3127310779993,
16.0411432697963));
#55650=CARTESIAN_POINT('Ctrl Pts',(-12.9845506983831,-52.5849778713889,
16.0149747663373));
#55651=CARTESIAN_POINT('Ctrl Pts',(-12.8189865827469,-53.0249099405019,
15.9888062628784));
#55652=CARTESIAN_POINT('Ctrl Pts',(-12.8740202534737,-53.4352565161154,
15.9626377594195));
#55653=CARTESIAN_POINT('Ctrl Pts',(-12.9290539242004,-53.845603091729,15.9364692559605));
#55654=CARTESIAN_POINT('Ctrl Pts',(-13.2046853812901,-54.226364173843,15.9103007525016));
#55655=CARTESIAN_POINT('Ctrl Pts',(-13.5773182028765,-54.4068019672842,
15.8841322490427));
#55656=CARTESIAN_POINT('Ctrl Pts',(-13.9499510244629,-54.5872397607254,
15.8579637455838));
#55657=CARTESIAN_POINT('Ctrl Pts',(-14.4195852105461,-54.5673542654938,
15.8317952421249));
#55658=CARTESIAN_POINT('Ctrl Pts',(-14.7756312098701,-54.3560623738526,
15.8056267386659));
#55659=CARTESIAN_POINT('Ctrl Pts',(-15.1316772091941,-54.1447704822114,
15.779458235207));
#55660=CARTESIAN_POINT('Ctrl Pts',(-15.374135021759,-53.7420721941606,15.7532897317481));
#55661=CARTESIAN_POINT('Ctrl Pts',(-15.3942836818793,-53.3285422092164,
15.7271212282891));
#55662=CARTESIAN_POINT('Ctrl Pts',(-15.4144323419997,-52.9150122242722,
15.7009527248302));
#55663=CARTESIAN_POINT('Ctrl Pts',(-15.2122718496755,-52.4906505424345,
15.6747842213713));
#55664=CARTESIAN_POINT('Ctrl Pts',(-14.8784533736736,-52.2457459854386,
15.6486157179124));
#55665=CARTESIAN_POINT('Ctrl Pts',(-14.5446348976717,-52.0008414284427,
15.6224472144534));
#55666=CARTESIAN_POINT('Ctrl Pts',(-14.0791584379921,-51.9353939962886,
15.5962787109945));
#55667=CARTESIAN_POINT('Ctrl Pts',(-13.6907491702475,-52.0787510969521,
15.5701102075356));
#55668=CARTESIAN_POINT('Ctrl Pts',(-13.6238095222296,-52.1034577006719,
15.5656002471506));
#55669=CARTESIAN_POINT('Ctrl Pts',(-13.5591589344204,-52.1343662450032,
15.5610902867656));
#55670=CARTESIAN_POINT('Ctrl Pts',(-13.4975120618698,-52.1706683776322,
15.5565803263806));
#55671=CARTESIAN_POINT('Ctrl Pts',(-13.4984004295476,-52.1727576237481,
15.6934196736194));
#55672=CARTESIAN_POINT('Ctrl Pts',(-13.6356154845653,-52.0925699142095,
15.7033931821041));
#55673=CARTESIAN_POINT('Ctrl Pts',(-13.7869389649625,-52.0373841810022,
15.7133666905887));
#55674=CARTESIAN_POINT('Ctrl Pts',(-13.9430173010127,-52.0141772385597,
15.7233401990734));
#55675=CARTESIAN_POINT('Ctrl Pts',(-14.352535825319,-51.9532868352966,15.7495087025323));
#55676=CARTESIAN_POINT('Ctrl Pts',(-14.7947883578784,-52.1125490669891,
15.7756772059912));
#55677=CARTESIAN_POINT('Ctrl Pts',(-15.0714636060598,-52.4205488559651,
15.8018457094502));
#55678=CARTESIAN_POINT('Ctrl Pts',(-15.3481388542411,-52.728548644941,15.8280142129091));
#55679=CARTESIAN_POINT('Ctrl Pts',(-15.4592368180444,-53.1852859912004,
15.854182716368));
#55680=CARTESIAN_POINT('Ctrl Pts',(-15.3549398499385,-53.5859544394514,
15.8803512198269));
#55681=CARTESIAN_POINT('Ctrl Pts',(-15.2506428818326,-53.9866228877023,
15.9065197232859));
#55682=CARTESIAN_POINT('Ctrl Pts',(-14.9309509818175,-54.3312224379448,
15.9326882267448));
#55683=CARTESIAN_POINT('Ctrl Pts',(-14.5392177979356,-54.4652305557052,
15.9588567302037));
#55684=CARTESIAN_POINT('Ctrl Pts',(-14.1474846140538,-54.5992386734655,
15.9850252336627));
#55685=CARTESIAN_POINT('Ctrl Pts',(-13.6837101463051,-54.5226553587437,
16.0111937371216));
#55686=CARTESIAN_POINT('Ctrl Pts',(-13.3558563789032,-54.2698214801478,
16.0373622405805));
#55687=CARTESIAN_POINT('Ctrl Pts',(-13.0280026115013,-54.016987601552,16.0635307440394));
#55688=CARTESIAN_POINT('Ctrl Pts',(-12.8360695444461,-53.5879031590822,
16.0896992474984));
#55689=CARTESIAN_POINT('Ctrl Pts',(-12.8661222463432,-53.174974717257,16.1158677509573));
#55690=CARTESIAN_POINT('Ctrl Pts',(-12.8958099052366,-52.7670620187505,
16.1417183918447));
#55691=CARTESIAN_POINT('Ctrl Pts',(-13.1421232693053,-52.3749152184319,
16.167569032732));
#55692=CARTESIAN_POINT('Ctrl Pts',(-13.4961138435274,-52.1700468646075,
16.1934196736194));
#55693=CARTESIAN_POINT('Origin',(-14.1292828945604,-53.2669068454841,15.5));
#55694=CARTESIAN_POINT('',(-13.4969690270882,-52.1733618792496,16.6934196736194));
#55695=CARTESIAN_POINT('',(-13.4982981440081,-52.1731729190029,16.5565803263806));
#55696=CARTESIAN_POINT('',(-13.4970328945604,-52.1718177223987,15.5));
#55697=CARTESIAN_POINT('Ctrl Pts',(-13.4982981440081,-52.1731729190029,
16.5565803263806));
#55698=CARTESIAN_POINT('Ctrl Pts',(-13.2942737914495,-52.2917933948419,
16.5417789949394));
#55699=CARTESIAN_POINT('Ctrl Pts',(-13.121375289642,-52.4650421903572,16.5269776634982));
#55700=CARTESIAN_POINT('Ctrl Pts',(-13.0113308722452,-52.6717520885803,
16.5121763320569));
#55701=CARTESIAN_POINT('Ctrl Pts',(-12.8167742049128,-53.0372116898416,
16.486007828598));
#55702=CARTESIAN_POINT('Ctrl Pts',(-12.8186845812822,-53.5072628063503,
16.4598393251391));
#55703=CARTESIAN_POINT('Ctrl Pts',(-13.0162053670574,-53.8711289302741,
16.4336708216802));
#55704=CARTESIAN_POINT('Ctrl Pts',(-13.2137261528326,-54.234995054198,16.4075023182212));
#55705=CARTESIAN_POINT('Ctrl Pts',(-13.6068573480138,-54.4926761855371,
16.3813338147623));
#55706=CARTESIAN_POINT('Ctrl Pts',(-14.0193142510177,-54.5286250418801,
16.3551653113034));
#55707=CARTESIAN_POINT('Ctrl Pts',(-14.4317711540216,-54.5645738982232,
16.3289968078445));
#55708=CARTESIAN_POINT('Ctrl Pts',(-14.8635537648482,-54.3787904795703,
16.3028283043855));
#55709=CARTESIAN_POINT('Ctrl Pts',(-15.1210456285732,-54.0545822792717,
16.2766598009266));
#55710=CARTESIAN_POINT('Ctrl Pts',(-15.3785374922981,-53.7303740789732,
16.2504912974677));
#55711=CARTESIAN_POINT('Ctrl Pts',(-15.4617386089214,-53.267741097029,16.2243227940088));
#55712=CARTESIAN_POINT('Ctrl Pts',(-15.3333406086023,-52.8741334617557,
16.1981542905498));
#55713=CARTESIAN_POINT('Ctrl Pts',(-15.2049426082832,-52.4805258264823,
16.1719857870909));
#55714=CARTESIAN_POINT('Ctrl Pts',(-14.8649454910218,-52.1559435378799,
16.145817283632));
#55715=CARTESIAN_POINT('Ctrl Pts',(-14.4658080057675,-52.0459331524117,
16.119648780173));
#55716=CARTESIAN_POINT('Ctrl Pts',(-14.1451555582543,-51.9575548350262,
16.0986259622422));
#55717=CARTESIAN_POINT('Ctrl Pts',(-13.7863343457911,-52.0076596690572,
16.0776031443114));
#55718=CARTESIAN_POINT('Ctrl Pts',(-13.4958915862188,-52.1719376453661,
16.0565803263806));
#55719=CARTESIAN_POINT('Ctrl Pts',(-13.4961138435274,-52.1700468646075,
16.1934196736194));
#55720=CARTESIAN_POINT('Ctrl Pts',(-13.5004665539579,-52.1675277788308,
16.193737536191));
#55721=CARTESIAN_POINT('Ctrl Pts',(-13.5048355445966,-52.1650370085359,
16.1940553987625));
#55722=CARTESIAN_POINT('Ctrl Pts',(-13.5092206128964,-52.1625748725828,
16.1943732613341));
#55723=CARTESIAN_POINT('Ctrl Pts',(-13.8702278067029,-51.9598759109143,
16.220541764793));
#55724=CARTESIAN_POINT('Ctrl Pts',(-14.3402037234666,-51.9512504287578,
16.2467102682519));
#55725=CARTESIAN_POINT('Ctrl Pts',(-14.7084055750498,-52.1405661950787,
16.2728787717108));
#55726=CARTESIAN_POINT('Ctrl Pts',(-15.076607426633,-52.3298819613996,16.2990472751698));
#55727=CARTESIAN_POINT('Ctrl Pts',(-15.3430352130359,-52.7171389761979,
16.3252157786287));
#55728=CARTESIAN_POINT('Ctrl Pts',(-15.3882195489487,-53.1286865903088,
16.3513842820876));
#55729=CARTESIAN_POINT('Ctrl Pts',(-15.4334038848614,-53.5402342044196,
16.3775527855465));
#55730=CARTESIAN_POINT('Ctrl Pts',(-15.2573447702841,-53.976072417843,16.4037212890055));
#55731=CARTESIAN_POINT('Ctrl Pts',(-14.9389892027718,-54.240766195907,16.4298897924644));
#55732=CARTESIAN_POINT('Ctrl Pts',(-14.6206336352594,-54.505459973971,16.4560582959233));
#55733=CARTESIAN_POINT('Ctrl Pts',(-14.159981614812,-54.5990093166755,16.4822267993823));
#55734=CARTESIAN_POINT('Ctrl Pts',(-13.7635949875347,-54.4794655848163,
16.5083953028412));
#55735=CARTESIAN_POINT('Ctrl Pts',(-13.3672083602575,-54.3599218529572,
16.5345638063001));
#55736=CARTESIAN_POINT('Ctrl Pts',(-13.0350871261504,-54.0272850465344,
16.560732309759));
#55737=CARTESIAN_POINT('Ctrl Pts',(-12.916158385472,-53.6307134674394,16.586900813218));
#55738=CARTESIAN_POINT('Ctrl Pts',(-12.7972296447937,-53.2341418883445,
16.6130693166769));
#55739=CARTESIAN_POINT('Ctrl Pts',(-12.891493397544,-52.7736355365774,16.6392378201358));
#55740=CARTESIAN_POINT('Ctrl Pts',(-13.1566806746197,-52.4556909263592,
16.6654063235947));
#55741=CARTESIAN_POINT('Ctrl Pts',(-13.2513082234268,-52.3422378246374,
16.6747441069363));
#55742=CARTESIAN_POINT('Ctrl Pts',(-13.3676994181703,-52.2469370707529,
16.6840818902779));
#55743=CARTESIAN_POINT('Ctrl Pts',(-13.4969690270882,-52.1733618792496,
16.6934196736194));
#55744=CARTESIAN_POINT('Origin',(-14.1292828945604,-53.2669068454841,15.5));
#55745=CARTESIAN_POINT('',(-13.498190246218,-52.1716844371558,17.1934196736194));
#55746=CARTESIAN_POINT('',(-13.4965460097018,-52.1700456009991,17.0565803263806));
#55747=CARTESIAN_POINT('',(-13.4970328945604,-52.1718177223987,15.5));
#55748=CARTESIAN_POINT('Ctrl Pts',(-13.4965460097018,-52.1700456009991,
17.0565803263806));
#55749=CARTESIAN_POINT('Ctrl Pts',(-13.1622129933252,-52.3652134872717,
17.0321233490263));
#55750=CARTESIAN_POINT('Ctrl Pts',(-12.9210086316388,-52.724852170666,17.0076663716719));
#55751=CARTESIAN_POINT('Ctrl Pts',(-12.8726933551042,-53.1087658234733,
16.9832093943176));
#55752=CARTESIAN_POINT('Ctrl Pts',(-12.8209969225157,-53.5195461748581,
16.9570408908587));
#55753=CARTESIAN_POINT('Ctrl Pts',(-12.9901314007569,-53.9581179567514,
16.9308723873998));
#55754=CARTESIAN_POINT('Ctrl Pts',(-13.3042549587021,-54.2278203840484,
16.9047038839408));
#55755=CARTESIAN_POINT('Ctrl Pts',(-13.6183785166473,-54.4975228113454,
16.8785353804819));
#55756=CARTESIAN_POINT('Ctrl Pts',(-14.0774911542965,-54.5983558840463,
16.852366877023));
#55757=CARTESIAN_POINT('Ctrl Pts',(-14.4757212681973,-54.4851048462747,
16.8261983735641));
#55758=CARTESIAN_POINT('Ctrl Pts',(-14.8739513820982,-54.371853808503,16.8000298701051));
#55759=CARTESIAN_POINT('Ctrl Pts',(-15.2112989722507,-54.0445186602589,
16.7738613666462));
#55760=CARTESIAN_POINT('Ctrl Pts',(-15.3364933887363,-53.6498803767017,
16.7476928631873));
#55761=CARTESIAN_POINT('Ctrl Pts',(-15.4616878052219,-53.2552420931446,
16.7215243597284));
#55762=CARTESIAN_POINT('Ctrl Pts',(-15.3747290480406,-52.7933006742746,
16.6953558562694));
#55763=CARTESIAN_POINT('Ctrl Pts',(-15.1146104479144,-52.4711961414872,
16.6691873528105));
#55764=CARTESIAN_POINT('Ctrl Pts',(-14.8544918477881,-52.1490916086999,
16.6430188493516));
#55765=CARTESIAN_POINT('Ctrl Pts',(-14.4212134047168,-51.9668239619953,
16.6168503458927));
#55766=CARTESIAN_POINT('Ctrl Pts',(-14.0090623276642,-52.00612418165,16.5906818424337));
#55767=CARTESIAN_POINT('Ctrl Pts',(-13.8300306074324,-52.0231955574683,
16.579314670416));
#55768=CARTESIAN_POINT('Ctrl Pts',(-13.6549853934321,-52.0820744013432,
16.5679474983983));
#55769=CARTESIAN_POINT('Ctrl Pts',(-13.4982981440081,-52.1731729190029,
16.5565803263806));
#55770=CARTESIAN_POINT('Ctrl Pts',(-13.4969690270882,-52.1733618792496,
16.6934196736194));
#55771=CARTESIAN_POINT('Ctrl Pts',(-13.7299687153222,-52.0407475948441,
16.7102503937368));
#55772=CARTESIAN_POINT('Ctrl Pts',(-14.0048072977942,-51.9787144778412,
16.7270811138541));
#55773=CARTESIAN_POINT('Ctrl Pts',(-14.2694557749176,-52.0081860992865,
16.7439118339715));
#55774=CARTESIAN_POINT('Ctrl Pts',(-14.6809327967389,-52.0540087511013,
16.7700803374304));
#55775=CARTESIAN_POINT('Ctrl Pts',(-15.0677760389806,-52.3210369234002,
16.7962488408894));
#55776=CARTESIAN_POINT('Ctrl Pts',(-15.256520467333,-52.6895319775572,16.8224173443483));
#55777=CARTESIAN_POINT('Ctrl Pts',(-15.4452648956854,-53.0580270317142,
16.8485858478072));
#55778=CARTESIAN_POINT('Ctrl Pts',(-15.4359105101485,-53.5279889677293,
16.8747543512661));
#55779=CARTESIAN_POINT('Ctrl Pts',(-15.2326517793345,-53.8886813318345,
16.9009228547251));
#55780=CARTESIAN_POINT('Ctrl Pts',(-15.0293930485204,-54.2493736959397,
16.927091358184));
#55781=CARTESIAN_POINT('Ctrl Pts',(-14.6322299724291,-54.500796488135,16.9532598616429));
#55782=CARTESIAN_POINT('Ctrl Pts',(-14.2192554962477,-54.5302086092019,
16.9794283651019));
#55783=CARTESIAN_POINT('Ctrl Pts',(-13.8062810200663,-54.5596207302688,
17.0055968685608));
#55784=CARTESIAN_POINT('Ctrl Pts',(-13.3774951437947,-54.3670221802074,
17.0317653720197));
#55785=CARTESIAN_POINT('Ctrl Pts',(-13.1251699439815,-54.0387767018188,
17.0579338754786));
#55786=CARTESIAN_POINT('Ctrl Pts',(-12.8728447441683,-53.7105312234301,
17.0841023789376));
#55787=CARTESIAN_POINT('Ctrl Pts',(-12.7969802208136,-53.2466388167143,
17.1102708823965));
#55788=CARTESIAN_POINT('Ctrl Pts',(-12.9315961537199,-52.8551138190488,
17.1364393858554));
#55789=CARTESIAN_POINT('Ctrl Pts',(-13.0293020925489,-52.570940046702,17.1554328151101));
#55790=CARTESIAN_POINT('Ctrl Pts',(-13.2378899597345,-52.32488970875,17.1744262443647));
#55791=CARTESIAN_POINT('Ctrl Pts',(-13.498190246218,-52.1716844371558,17.1934196736194));
#55792=CARTESIAN_POINT('Origin',(-14.1292828945604,-53.2669068454841,15.5));
#55793=CARTESIAN_POINT('',(-13.495722982135,-52.1707788329429,17.6934196736194));
#55794=CARTESIAN_POINT('',(-13.4965541629804,-52.1730078059394,17.5565803263806));
#55795=CARTESIAN_POINT('',(-13.4970328945604,-52.1718177223987,15.5));
#55796=CARTESIAN_POINT('',(-13.8936870225526,-54.5092654229862,18.));
#55797=CARTESIAN_POINT('Ctrl Pts',(-13.495722982135,-52.1707788329429,17.6934196736194));
#55798=CARTESIAN_POINT('Ctrl Pts',(-13.8217103338362,-51.9852932094709,
17.7171076053695));
#55799=CARTESIAN_POINT('Ctrl Pts',(-14.2369080256434,-51.9506029252058,
17.7407955371196));
#55800=CARTESIAN_POINT('Ctrl Pts',(-14.5864865212314,-52.0858847696684,
17.7644834688697));
#55801=CARTESIAN_POINT('Ctrl Pts',(-14.9726724562246,-52.2353331660965,
17.7906519723286));
#55802=CARTESIAN_POINT('Ctrl Pts',(-15.2787764866269,-52.5922161636806,
17.8168204757875));
#55803=CARTESIAN_POINT('Ctrl Pts',(-15.3668468800596,-52.9968087774221,
17.8429889792464));
#55804=CARTESIAN_POINT('Ctrl Pts',(-15.4549172734923,-53.4014013911635,
17.8691574827054));
#55805=CARTESIAN_POINT('Ctrl Pts',(-15.3249540299554,-53.8537036210623,
17.8953259861643));
#55806=CARTESIAN_POINT('Ctrl Pts',(-15.0367817327077,-54.1500381490016,
17.9214944896232));
#55807=CARTESIAN_POINT('Ctrl Pts',(-14.74860943546,-54.4463726769409,17.9476629930821));
#55808=CARTESIAN_POINT('Ctrl Pts',(-14.3022280845015,-54.5867395029208,
17.9738314965411));
#55809=CARTESIAN_POINT('Ctrl Pts',(-13.8936870225526,-54.5092654229862,
18.));
#55810=CARTESIAN_POINT('',(-12.9337042190834,-52.8487739793663,18.));
#55811=CARTESIAN_POINT('Origin',(-14.1292828945604,-53.2669068454841,18.));
#55812=CARTESIAN_POINT('Ctrl Pts',(-12.9336937527446,-52.8487684531621,
18.));
#55813=CARTESIAN_POINT('Ctrl Pts',(-12.8048883200695,-53.2213447345786,
17.975091839613));
#55814=CARTESIAN_POINT('Ctrl Pts',(-12.8625878757539,-53.660362859942,17.950183679226));
#55815=CARTESIAN_POINT('Ctrl Pts',(-13.0861189278269,-53.984999064981,17.925275518839));
#55816=CARTESIAN_POINT('Ctrl Pts',(-13.3209605627957,-54.3260617336993,
17.89910701538));
#55817=CARTESIAN_POINT('Ctrl Pts',(-13.7388402922128,-54.5408742678445,
17.8729385119211));
#55818=CARTESIAN_POINT('Ctrl Pts',(-14.1527389844809,-54.5331807500212,
17.8467700084622));
#55819=CARTESIAN_POINT('Ctrl Pts',(-14.5666376767489,-54.5254872321979,
17.8206015050033));
#55820=CARTESIAN_POINT('Ctrl Pts',(-14.9765553318677,-54.2952876624061,
17.7944330015443));
#55821=CARTESIAN_POINT('Ctrl Pts',(-15.1985005516416,-53.9457721211068,
17.7682644980854));
#55822=CARTESIAN_POINT('Ctrl Pts',(-15.4204457714154,-53.5962565798075,
17.7420959946265));
#55823=CARTESIAN_POINT('Ctrl Pts',(-15.4544185558441,-53.1274250670007,
17.7159274911676));
#55824=CARTESIAN_POINT('Ctrl Pts',(-15.2852740004506,-52.7495241339714,
17.6897589877086));
#55825=CARTESIAN_POINT('Ctrl Pts',(-15.1161294450571,-52.3716232009421,
17.6635904842497));
#55826=CARTESIAN_POINT('Ctrl Pts',(-14.7438675498413,-52.0846528476903,
17.6374219807908));
#55827=CARTESIAN_POINT('Ctrl Pts',(-14.3353709232148,-52.0172856023794,
17.6112534773319));
#55828=CARTESIAN_POINT('Ctrl Pts',(-14.050883915571,-51.9703694107086,17.5930290936814));
#55829=CARTESIAN_POINT('Ctrl Pts',(-13.7488228128377,-52.0299622436843,
17.574804710031));
#55830=CARTESIAN_POINT('Ctrl Pts',(-13.4965541629804,-52.1730078059394,
17.5565803263806));
#55831=CARTESIAN_POINT('Origin',(-14.1292828945604,-53.2669068454841,19.1042117235887));
#55832=CARTESIAN_POINT('',(-13.3561475049579,-51.9293198574881,14.3957882764113));
#55833=CARTESIAN_POINT('',(-13.3590334722299,-51.9326791410007,14.3542117235887));
#55834=CARTESIAN_POINT('',(-13.3577828945603,-51.9306296474448,19.1042117235887));
#55835=CARTESIAN_POINT('',(-15.619480088463,-52.8667052421829,14.));
#55836=CARTESIAN_POINT('Ctrl Pts',(-13.3590334722299,-51.9326791410007,
14.3542117235887));
#55837=CARTESIAN_POINT('Ctrl Pts',(-13.133310230807,-52.0631907802776,14.3408151628949));
#55838=CARTESIAN_POINT('Ctrl Pts',(-12.5590924929827,-52.6090703324587,
14.301250098742));
#55839=CARTESIAN_POINT('Ctrl Pts',(-12.4888785260391,-54.0475602728968,
14.2355165311304));
#55840=CARTESIAN_POINT('Ctrl Pts',(-13.8755779012831,-55.0671461874891,
14.1570110207535));
#55841=CARTESIAN_POINT('Ctrl Pts',(-15.4910603626305,-54.4687297322861,
14.0785055103768));
#55842=CARTESIAN_POINT('Ctrl Pts',(-15.7510836294753,-53.3567463262428,
14.0261685034589));
#55843=CARTESIAN_POINT('Ctrl Pts',(-15.619480088463,-52.8667052421829,14.));
#55844=CARTESIAN_POINT('',(-15.2224969554152,-52.1743874122524,14.));
#55845=CARTESIAN_POINT('Origin',(-14.1292828945604,-53.2669068454841,14.));
#55846=CARTESIAN_POINT('Ctrl Pts',(-13.3561475049579,-51.9293198574881,
14.3957882764113));
#55847=CARTESIAN_POINT('Ctrl Pts',(-13.3167322940314,-51.9517582304518,
14.3934410251636));
#55848=CARTESIAN_POINT('Ctrl Pts',(-12.8509091548949,-52.2463455523905,
14.3649252704569));
#55849=CARTESIAN_POINT('Ctrl Pts',(-12.312999126503,-53.317416116839,14.3102410122914));
#55850=CARTESIAN_POINT('Ctrl Pts',(-13.1694776941513,-54.8098931066082,
14.2317355019146));
#55851=CARTESIAN_POINT('Ctrl Pts',(-14.8870885705588,-54.9183199028175,
14.1532299915378));
#55852=CARTESIAN_POINT('Ctrl Pts',(-15.9077095091603,-53.5682793339942,
14.0759848242329));
#55853=CARTESIAN_POINT('Ctrl Pts',(-15.5613200902447,-52.5158444925152,
14.024908160387));
#55854=CARTESIAN_POINT('Ctrl Pts',(-15.2225055381225,-52.1743757967134,
14.));
#55855=CARTESIAN_POINT('Origin',(-14.1292828945604,-53.2669068454841,19.1042117235887));
#55856=CARTESIAN_POINT('',(-13.3586534741695,-51.9327902292019,14.8957882764113));
#55857=CARTESIAN_POINT('',(-13.3577899368159,-51.928743983656,14.8542117235887));
#55858=CARTESIAN_POINT('',(-13.3577828945603,-51.9306296474448,19.1042117235887));
#55859=CARTESIAN_POINT('Ctrl Pts',(-13.3577899368159,-51.928743983656,14.8542117235887));
#55860=CARTESIAN_POINT('Ctrl Pts',(-12.9734547442474,-52.1543891335537,
14.8311595169817));
#55861=CARTESIAN_POINT('Ctrl Pts',(-12.3621732880177,-53.0098569651208,
14.7819388069158));
#55862=CARTESIAN_POINT('Ctrl Pts',(-12.8743108410601,-54.5809237767912,
14.706549593391));
#55863=CARTESIAN_POINT('Ctrl Pts',(-14.53309819057,-55.0385159317414,14.6280440830142));
#55864=CARTESIAN_POINT('Ctrl Pts',(-15.8297520454146,-53.9072361260964,
14.5495385726375));
#55865=CARTESIAN_POINT('Ctrl Pts',(-15.6013490876951,-52.2017963646938,
14.4710330622607));
#55866=CARTESIAN_POINT('Ctrl Pts',(-14.317080229173,-51.5794230562898,14.4059241125778));
#55867=CARTESIAN_POINT('Ctrl Pts',(-13.5742323121468,-51.8082526389224,
14.3669836663538));
#55868=CARTESIAN_POINT('Ctrl Pts',(-13.3590334722299,-51.9326791410007,
14.3542117235887));
#55869=CARTESIAN_POINT('Ctrl Pts',(-13.3586534741695,-51.9327902292019,
14.8957882764113));
#55870=CARTESIAN_POINT('Ctrl Pts',(-13.1561499564235,-52.0491845394434,
14.8837853792505));
#55871=CARTESIAN_POINT('Ctrl Pts',(-12.5927601381537,-52.5577927522065,
14.8456139786307));
#55872=CARTESIAN_POINT('Ctrl Pts',(-12.4499580614657,-53.9607971579716,
14.781274074552));
#55873=CARTESIAN_POINT('Ctrl Pts',(-13.7817713167744,-55.0504032414555,
14.7027685641753));
#55874=CARTESIAN_POINT('Ctrl Pts',(-15.4252464910755,-54.5405234556122,
14.6242630537985));
#55875=CARTESIAN_POINT('Ctrl Pts',(-15.9064600587524,-52.8884418877605,
14.5457575434217));
#55876=CARTESIAN_POINT('Ctrl Pts',(-14.8271456061161,-51.6150089076653,
14.4695992842926));
#55877=CARTESIAN_POINT('Ctrl Pts',(-13.7561556767952,-51.7016023764131,
14.4196095286225));
#55878=CARTESIAN_POINT('Ctrl Pts',(-13.3561475049579,-51.9293198574881,
14.3957882764113));
#55879=CARTESIAN_POINT('Origin',(-14.1292828945604,-53.2669068454841,19.1042117235887));
#55880=CARTESIAN_POINT('',(-13.3583675961487,-51.9292271650606,15.3957882764113));
#55881=CARTESIAN_POINT('',(-13.3567403793944,-51.9314820095869,15.3542117235887));
#55882=CARTESIAN_POINT('',(-13.3577828945603,-51.9306296474448,19.1042117235887));
#55883=CARTESIAN_POINT('Ctrl Pts',(-13.3567403793944,-51.9314820095869,
15.3542117235887));
#55884=CARTESIAN_POINT('Ctrl Pts',(-13.2463612263438,-51.9939332857897,
15.3476723745276));
#55885=CARTESIAN_POINT('Ctrl Pts',(-12.7340280693376,-52.3726757467305,
15.3149645220075));
#55886=CARTESIAN_POINT('Ctrl Pts',(-12.343540269987,-53.6026792252177,15.2560881660285));
#55887=CARTESIAN_POINT('Ctrl Pts',(-13.4243618186885,-54.9416323741227,
15.1775826556517));
#55888=CARTESIAN_POINT('Ctrl Pts',(-15.1373732173662,-54.7786522269085,
15.0990771452749));
#55889=CARTESIAN_POINT('Ctrl Pts',(-15.9463055097723,-53.2599021305098,
15.0205716348981));
#55890=CARTESIAN_POINT('Ctrl Pts',(-15.1256881964072,-51.7474355457531,
14.9420661245214));
#55891=CARTESIAN_POINT('Ctrl Pts',(-13.9148311256039,-51.641642546183,14.8866128207515));
#55892=CARTESIAN_POINT('Ctrl Pts',(-13.4097460280966,-51.8982402977282,
14.8573280204407));
#55893=CARTESIAN_POINT('Ctrl Pts',(-13.3577899368159,-51.928743983656,14.8542117235887));
#55894=CARTESIAN_POINT('Ctrl Pts',(-13.3583675961487,-51.9292271650606,
15.3957882764113));
#55895=CARTESIAN_POINT('Ctrl Pts',(-12.9971119417281,-52.1419605956009,
15.3741297333373));
#55896=CARTESIAN_POINT('Ctrl Pts',(-12.3860414668385,-52.9469081505226,
15.3263026868045));
#55897=CARTESIAN_POINT('Ctrl Pts',(-12.8070334555363,-54.5132114643009,
15.2523071368127));
#55898=CARTESIAN_POINT('Ctrl Pts',(-14.4395092097517,-55.0572639347494,
15.1738016264359));
#55899=CARTESIAN_POINT('Ctrl Pts',(-15.7937667074069,-53.9956815464662,
15.0952961160592));
#55900=CARTESIAN_POINT('Ctrl Pts',(-15.6552753932384,-52.280516797303,15.0167906056824));
#55901=CARTESIAN_POINT('Ctrl Pts',(-14.3786526271626,-51.5769541863948,
14.9502879924664));
#55902=CARTESIAN_POINT('Ctrl Pts',(-13.5976445334062,-51.7954237290868,
14.9099538827094));
#55903=CARTESIAN_POINT('Ctrl Pts',(-13.3586534741695,-51.9327902292019,
14.8957882764113));
#55904=CARTESIAN_POINT('Origin',(-14.1292828945604,-53.2669068454841,19.1042117235887));
#55905=CARTESIAN_POINT('',(-13.3563902185848,-51.9307759828648,15.8957882764113));
#55906=CARTESIAN_POINT('',(-13.3594516225044,-51.9317765575136,15.8542117235887));
#55907=CARTESIAN_POINT('',(-13.3577828945603,-51.9306296474448,19.1042117235887));
#55908=CARTESIAN_POINT('Ctrl Pts',(-13.3594516225044,-51.9317765575136,
15.8542117235887));
#55909=CARTESIAN_POINT('Ctrl Pts',(-13.087568835844,-52.0906633350794,15.8380167286145));
#55910=CARTESIAN_POINT('Ctrl Pts',(-12.4951087068473,-52.7167109460471,
15.7956532301813));
#55911=CARTESIAN_POINT('Ctrl Pts',(-12.5800904986592,-54.21644496341,15.7271212282892));
#55912=CARTESIAN_POINT('Ctrl Pts',(-14.0667923195219,-55.0828679235634,
15.6486157179124));
#55913=CARTESIAN_POINT('Ctrl Pts',(-15.6095371717916,-54.3206938223985,
15.5701102075356));
#55914=CARTESIAN_POINT('Ctrl Pts',(-15.8247548010729,-52.6134584968727,
15.4916046971588));
#55915=CARTESIAN_POINT('Ctrl Pts',(-14.6281635632835,-51.5856454904132,
15.4196385358432));
#55916=CARTESIAN_POINT('Ctrl Pts',(-13.6880653197304,-51.7440221062451,
15.3738408779865));
#55917=CARTESIAN_POINT('Ctrl Pts',(-13.3567403793944,-51.9314820095869,
15.3542117235887));
#55918=CARTESIAN_POINT('Ctrl Pts',(-13.3563902185848,-51.9307759828648,
15.8957882764113));
#55919=CARTESIAN_POINT('Ctrl Pts',(-13.2696421210522,-51.9798417675732,
15.8906425908832));
#55920=CARTESIAN_POINT('Ctrl Pts',(-12.7721552352232,-52.3292268802208,
15.8593284018961));
#55921=CARTESIAN_POINT('Ctrl Pts',(-12.3283713567552,-53.5084362707541,
15.8018457094502));
#55922=CARTESIAN_POINT('Ctrl Pts',(-13.3373852079754,-54.9023018690979,
15.7233401990734));
#55923=CARTESIAN_POINT('Ctrl Pts',(-15.0565917302206,-54.8295063313936,
15.6448346886966));
#55924=CARTESIAN_POINT('Ctrl Pts',(-15.9441656443073,-53.3553344251958,
15.5663291783198));
#55925=CARTESIAN_POINT('Ctrl Pts',(-15.2041095597138,-51.8018585649929,
15.4878236679431));
#55926=CARTESIAN_POINT('Ctrl Pts',(-13.970228695557,-51.6283710932553,15.4309767006402));
#55927=CARTESIAN_POINT('Ctrl Pts',(-13.4335918937727,-51.8849296635607,
15.4002982367963));
#55928=CARTESIAN_POINT('Ctrl Pts',(-13.3583675961487,-51.9292271650606,
15.3957882764113));
#55929=CARTESIAN_POINT('Origin',(-14.1292828945604,-53.2669068454841,19.1042117235887));
#55930=CARTESIAN_POINT('',(-13.3593268090704,-51.9322833195368,16.3957882764113));
#55931=CARTESIAN_POINT('',(-13.3566614269891,-51.9284687668027,16.3542117235887));
#55932=CARTESIAN_POINT('',(-13.3577828945603,-51.9306296474448,19.1042117235887));
#55933=CARTESIAN_POINT('Ctrl Pts',(-13.3566614269891,-51.9284687668027,
16.3542117235887));
#55934=CARTESIAN_POINT('Ctrl Pts',(-12.9247061434582,-52.1784583832132,
16.3283610827014));
#55935=CARTESIAN_POINT('Ctrl Pts',(-12.3198850098697,-53.141372730953,16.2763419383551));
#55936=CARTESIAN_POINT('Ctrl Pts',(-13.0196563589383,-54.7057774673455,
16.1981542905498));
#55937=CARTESIAN_POINT('Ctrl Pts',(-14.7174120024405,-54.986128723848,16.1196487801731));
#55938=CARTESIAN_POINT('Ctrl Pts',(-15.8877194798387,-53.7246409278238,
16.0411432697963));
#55939=CARTESIAN_POINT('Ctrl Pts',(-15.4810192232586,-52.0526463245539,
15.9626377594195));
#55940=CARTESIAN_POINT('Ctrl Pts',(-14.1960288388143,-51.5899006730013,
15.900327244017));
#55941=CARTESIAN_POINT('Ctrl Pts',(-13.5268876287458,-51.8339278933634,
15.8641852320734));
#55942=CARTESIAN_POINT('Ctrl Pts',(-13.3594516225044,-51.9317765575136,
15.8542117235887));
#55943=CARTESIAN_POINT('Ctrl Pts',(-13.3593268090704,-51.9322833195368,
16.3957882764113));
#55944=CARTESIAN_POINT('Ctrl Pts',(-13.1103670811162,-52.077029380604,16.3809869449701));
#55945=CARTESIAN_POINT('Ctrl Pts',(-12.5263819999043,-52.6621976201272,
16.3400171100699));
#55946=CARTESIAN_POINT('Ctrl Pts',(-12.5323627785853,-54.1337776405725,
16.2728787717109));
#55947=CARTESIAN_POINT('Ctrl Pts',(-13.9715120885842,-55.0770800976454,
16.1943732613341));
#55948=CARTESIAN_POINT('Ctrl Pts',(-15.5521540067467,-54.3969761475115,
16.1158677509573));
#55949=CARTESIAN_POINT('Ctrl Pts',(-15.8567312853938,-52.7033991815804,
16.0373622405805));
#55950=CARTESIAN_POINT('Ctrl Pts',(-14.6936723389742,-51.5930711363043,
15.9640024157318));
#55951=CARTESIAN_POINT('Ctrl Pts',(-13.7108015891029,-51.7303165780055,
15.9168110943421));
#55952=CARTESIAN_POINT('Ctrl Pts',(-13.3563902185848,-51.9307759828648,
15.8957882764113));
#55953=CARTESIAN_POINT('Origin',(-14.1292828945604,-53.2669068454841,19.1042117235887));
#55954=CARTESIAN_POINT('',(-13.3571887756701,-51.9284672248907,16.8957882764113));
#55955=CARTESIAN_POINT('',(-13.3577049605869,-51.9325138973624,16.8542117235887));
#55956=CARTESIAN_POINT('',(-13.3577828945603,-51.9306296474448,19.1042117235887));
#55957=CARTESIAN_POINT('Ctrl Pts',(-13.3577049605869,-51.9325138973624,
16.8542117235887));
#55958=CARTESIAN_POINT('Ctrl Pts',(-13.1999643464624,-52.0222936684099,
16.8448739402472));
#55959=CARTESIAN_POINT('Ctrl Pts',(-12.6599209222933,-52.4644795705918,
16.8093676534467));
#55960=CARTESIAN_POINT('Ctrl Pts',(-12.38882648105,-53.7888562103795,16.7476928631873));
#55961=CARTESIAN_POINT('Ctrl Pts',(-13.6046344626093,-55.0065515658013,
16.6691873528105));
#55962=CARTESIAN_POINT('Ctrl Pts',(-15.2909596525272,-54.6640921689023,
16.5906818424337));
#55963=CARTESIAN_POINT('Ctrl Pts',(-15.9354654978244,-53.0686037624671,
16.5121763320569));
#55964=CARTESIAN_POINT('Ctrl Pts',(-14.9601438503283,-51.6509582729447,
16.4336708216802));
#55965=CARTESIAN_POINT('Ctrl Pts',(-13.8062061827166,-51.672136525716,16.3810159521908));
#55966=CARTESIAN_POINT('Ctrl Pts',(-13.3619728008082,-51.9253948645857,
16.3545295861603));
#55967=CARTESIAN_POINT('Ctrl Pts',(-13.3566614269891,-51.9284687668027,
16.3542117235887));
#55968=CARTESIAN_POINT('Ctrl Pts',(-13.3571887756701,-51.9284672248907,
16.8957882764113));
#55969=CARTESIAN_POINT('Ctrl Pts',(-12.9492205318827,-52.1666198927584,
16.8713312990569));
#55970=CARTESIAN_POINT('Ctrl Pts',(-12.3399661957944,-53.0750256353043,
16.8207058182437));
#55971=CARTESIAN_POINT('Ctrl Pts',(-12.9456243299004,-54.6455189484075,
16.7439118339715));
#55972=CARTESIAN_POINT('Ctrl Pts',(-14.626314246609,-55.0146421540478,16.6654063235948));
#55973=CARTESIAN_POINT('Ctrl Pts',(-15.8612545351151,-53.8163547667627,
16.586900813218));
#55974=CARTESIAN_POINT('Ctrl Pts',(-15.5429215283994,-52.1253094303059,
16.5083953028412));
#55975=CARTESIAN_POINT('Ctrl Pts',(-14.2558484377858,-51.5838751930056,
16.4446911239056));
#55976=CARTESIAN_POINT('Ctrl Pts',(-13.5505236662165,-51.8211207946266,
16.407155448429));
#55977=CARTESIAN_POINT('Ctrl Pts',(-13.3593268090704,-51.9322833195368,
16.3957882764113));
#55978=CARTESIAN_POINT('Origin',(-14.1292828945604,-53.2669068454841,19.1042117235887));
#55979=CARTESIAN_POINT('',(-13.3571987246687,-51.9320818411208,17.3957882764113));
#55980=CARTESIAN_POINT('',(-13.3591951473146,-51.9304670067727,17.3542117235887));
#55981=CARTESIAN_POINT('',(-13.3577828945603,-51.9306296474448,19.1042117235887));
#55982=CARTESIAN_POINT('Ctrl Pts',(-13.3591951473146,-51.9304670067727,
17.3542117235887));
#55983=CARTESIAN_POINT('Ctrl Pts',(-13.0415649835786,-52.117414997338,17.3352182943341));
#55984=CARTESIAN_POINT('Ctrl Pts',(-12.4363561313197,-52.8313196200714,
17.2900563616205));
#55985=CARTESIAN_POINT('Ctrl Pts',(-12.6886936446445,-54.3742998061273,
17.2187259254479));
#55986=CARTESIAN_POINT('Ctrl Pts',(-14.2583653103316,-55.0793521495312,
17.1402204150712));
#55987=CARTESIAN_POINT('Ctrl Pts',(-15.7122742697832,-54.1589598165365,
17.0617149046944));
#55988=CARTESIAN_POINT('Ctrl Pts',(-15.7465182007045,-52.4385534884905,
16.9832093943176));
#55989=CARTESIAN_POINT('Ctrl Pts',(-14.4988281136715,-51.5773043644132,
16.9140416672824));
#55990=CARTESIAN_POINT('Ctrl Pts',(-13.6420217015477,-51.7706919591752,
16.8710424437061));
#55991=CARTESIAN_POINT('Ctrl Pts',(-13.3577049605869,-51.9325138973624,
16.8542117235887));
#55992=CARTESIAN_POINT('Ctrl Pts',(-13.3571987246687,-51.9320818411208,
17.3957882764113));
#55993=CARTESIAN_POINT('Ctrl Pts',(-13.2230139283874,-52.0081695343042,
17.3878441566028));
#55994=CARTESIAN_POINT('Ctrl Pts',(-12.6963900910874,-52.417984443011,17.3537315333353));
#55995=CARTESIAN_POINT('Ctrl Pts',(-12.3638250796578,-53.6967359986948,
17.293450406609));
#55996=CARTESIAN_POINT('Ctrl Pts',(-13.5139962436503,-54.9765978264216,
17.2149448962322));
#55997=CARTESIAN_POINT('Ctrl Pts',(-15.2159841085892,-54.7231706136822,
17.1364393858554));
#55998=CARTESIAN_POINT('Ctrl Pts',(-15.9433860453713,-53.1637302055401,
17.0579338754786));
#55999=CARTESIAN_POINT('Ctrl Pts',(-15.043860342301,-51.6968216692226,16.9794283651019));
#56000=CARTESIAN_POINT('Ctrl Pts',(-13.8598729208803,-51.6563265828795,
16.9253798320794));
#56001=CARTESIAN_POINT('Ctrl Pts',(-13.3857388409123,-51.9118010399394,
16.8974998025159));
#56002=CARTESIAN_POINT('Ctrl Pts',(-13.3571887756701,-51.9284672248907,
16.8957882764113));
#56003=CARTESIAN_POINT('Origin',(-14.1292828945604,-53.2669068454841,19.1042117235887));
#56004=CARTESIAN_POINT('',(-13.3599426557471,-51.9312965605688,17.8957882764113));
#56005=CARTESIAN_POINT('',(-13.3561844802682,-51.9293619476186,17.8542117235887));
#56006=CARTESIAN_POINT('',(-13.3577828945603,-51.9306296474448,19.1042117235887));
#56007=CARTESIAN_POINT('',(-15.2209662466057,-52.1764590205667,18.));
#56008=CARTESIAN_POINT('Ctrl Pts',(-15.2209662466057,-52.1764590205667,
18.));
#56009=CARTESIAN_POINT('Ctrl Pts',(-14.8623799894179,-51.8174664687921,
17.9738314965411));
#56010=CARTESIAN_POINT('Ctrl Pts',(-14.136921272848,-51.597902680369,17.9390942553448));
#56011=CARTESIAN_POINT('Ctrl Pts',(-13.5035430816839,-51.8470756229631,
17.9043570141486));
#56012=CARTESIAN_POINT('Ctrl Pts',(-13.3599426557471,-51.9312965605688,
17.8957882764113));
#56013=CARTESIAN_POINT('',(-15.6220396093989,-52.866415579935,18.));
#56014=CARTESIAN_POINT('Origin',(-14.1292828945604,-53.2669068454841,18.));
#56015=CARTESIAN_POINT('Ctrl Pts',(-15.6220539738783,-52.8664139542998,
18.));
#56016=CARTESIAN_POINT('Ctrl Pts',(-15.4957406336878,-52.4022578052826,
17.975091839613));
#56017=CARTESIAN_POINT('Ctrl Pts',(-14.7933534445258,-51.6161821464322,
17.9264957474759));
#56018=CARTESIAN_POINT('Ctrl Pts',(-13.7539689671603,-51.7030240140342,
17.8778996553388));
#56019=CARTESIAN_POINT('Ctrl Pts',(-13.3561844802682,-51.9293619476186,
17.8542117235887));
#56020=CARTESIAN_POINT('Origin',(39.0658530619283,-38.8697713466883,15.5));
#56021=CARTESIAN_POINT('',(38.4345426068235,-37.7764071067806,14.1934196736194));
#56022=CARTESIAN_POINT('',(38.4325424620227,-37.7762177647969,14.0565803263806));
#56023=CARTESIAN_POINT('',(38.4336030619283,-37.7746822236028,15.5));
#56024=CARTESIAN_POINT('',(39.3014489339361,-37.6274127691862,14.));
#56025=CARTESIAN_POINT('Ctrl Pts',(38.4325424620227,-37.7762177647969,14.0565803263806));
#56026=CARTESIAN_POINT('Ctrl Pts',(38.6929044073907,-37.6289035868348,14.0377202175871));
#56027=CARTESIAN_POINT('Ctrl Pts',(39.0070060787276,-37.5715758131853,14.0188601087935));
#56028=CARTESIAN_POINT('Ctrl Pts',(39.3014489339361,-37.6274127691862,14.));
#56029=CARTESIAN_POINT('',(38.4336030619283,-37.7746822236028,14.));
#56030=CARTESIAN_POINT('Origin',(39.0658530619283,-38.8697713466883,14.));
#56031=CARTESIAN_POINT('',(38.4336030619283,-37.7746822236028,13.));
#56032=CARTESIAN_POINT('',(38.4336030619283,-37.7746822236028,15.5));
#56033=CARTESIAN_POINT('',(39.7608672580761,-37.8134023216062,13.));
#56034=CARTESIAN_POINT('Origin',(39.0658530619283,-38.8697713466883,13.));
#56035=CARTESIAN_POINT('',(38.3708388657804,-39.9261403717704,13.));
#56036=CARTESIAN_POINT('Origin',(39.0658530619283,-38.8697713466883,13.));
#56037=CARTESIAN_POINT('Origin',(39.0658530619283,-38.8697713466883,13.));
#56038=CARTESIAN_POINT('',(40.2614318702746,-39.2879073628688,14.));
#56039=CARTESIAN_POINT('Origin',(39.0658530619283,-38.8697713466883,14.));
#56040=CARTESIAN_POINT('Ctrl Pts',(40.261442519219,-39.2879130030575,14.));
#56041=CARTESIAN_POINT('Ctrl Pts',(40.3902451808538,-38.9153391953948,14.024908160387));
#56042=CARTESIAN_POINT('Ctrl Pts',(40.3325529350425,-38.4763144202222,14.049816320774));
#56043=CARTESIAN_POINT('Ctrl Pts',(40.109022770241,-38.1516757839093,14.074724481161));
#56044=CARTESIAN_POINT('Ctrl Pts',(39.8741820674393,-37.8106105608956,14.10089298462));
#56045=CARTESIAN_POINT('Ctrl Pts',(39.4562961811818,-37.5958001287034,14.1270614880789));
#56046=CARTESIAN_POINT('Ctrl Pts',(39.042395291977,-37.6034944064735,14.1532299915378));
#56047=CARTESIAN_POINT('Ctrl Pts',(38.8305051320303,-37.6074333729988,14.1666265522317));
#56048=CARTESIAN_POINT('Ctrl Pts',(38.619659348036,-37.6696856996876,14.1800231129255));
#56049=CARTESIAN_POINT('Ctrl Pts',(38.4345426068235,-37.7764071067806,14.1934196736194));
#56050=CARTESIAN_POINT('Origin',(39.0658530619283,-38.8697713466883,15.5));
#56051=CARTESIAN_POINT('',(38.4322601856233,-37.7739115851766,14.6934196736194));
#56052=CARTESIAN_POINT('',(38.4333416483911,-37.7729821125454,14.5565803263806));
#56053=CARTESIAN_POINT('',(38.4336030619283,-37.7746822236028,15.5));
#56054=CARTESIAN_POINT('Ctrl Pts',(38.4333416483911,-37.7729821125454,14.5565803263806));
#56055=CARTESIAN_POINT('Ctrl Pts',(38.4654171032337,-37.7542027235003,14.5542330751329));
#56056=CARTESIAN_POINT('Ctrl Pts',(38.4983383982293,-37.7369254869309,14.5518858238852));
#56057=CARTESIAN_POINT('Ctrl Pts',(38.532014378561,-37.721272199783,14.5495385726375));
#56058=CARTESIAN_POINT('Ctrl Pts',(38.9074535262252,-37.5467603748252,14.5233700691785));
#56059=CARTESIAN_POINT('Ctrl Pts',(39.3766930387427,-37.5740903519378,14.4972015657196));
#56060=CARTESIAN_POINT('Ctrl Pts',(39.7293604226538,-37.7909904189904,14.4710330622607));
#56061=CARTESIAN_POINT('Ctrl Pts',(40.0820278065648,-38.007890486043,14.4448645588017));
#56062=CARTESIAN_POINT('Ctrl Pts',(40.3181230618696,-38.4143606430357,14.4186960553428));
#56063=CARTESIAN_POINT('Ctrl Pts',(40.3316969948736,-38.8281685539702,14.3925275518839));
#56064=CARTESIAN_POINT('Ctrl Pts',(40.3452709278776,-39.2419764649047,14.366359048425));
#56065=CARTESIAN_POINT('Ctrl Pts',(40.1363235385808,-39.6631221297811,14.340190544966));
#56066=CARTESIAN_POINT('Ctrl Pts',(39.7987141516887,-39.9026904288663,14.3140220415071));
#56067=CARTESIAN_POINT('Ctrl Pts',(39.4611047647966,-40.1422587279515,14.2878535380482));
#56068=CARTESIAN_POINT('Ctrl Pts',(38.9948333803092,-40.2002496612456,14.2616850345893));
#56069=CARTESIAN_POINT('Ctrl Pts',(38.6086468373336,-40.0507988707032,14.2355165311303));
#56070=CARTESIAN_POINT('Ctrl Pts',(38.222460294358,-39.9013480801609,14.2093480276714));
#56071=CARTESIAN_POINT('Ctrl Pts',(37.9163585928943,-39.5444555657821,14.1831795242125));
#56072=CARTESIAN_POINT('Ctrl Pts',(37.8282870218577,-39.1398677193851,14.1570110207535));
#56073=CARTESIAN_POINT('Ctrl Pts',(37.7402154508211,-38.735279872988,14.1308425172946));
#56074=CARTESIAN_POINT('Ctrl Pts',(37.8701740102116,-38.2829966945726,14.1046740138357));
#56075=CARTESIAN_POINT('Ctrl Pts',(38.1583471155031,-37.9866613986385,14.0785055103768));
#56076=CARTESIAN_POINT('Ctrl Pts',(38.2388287062341,-37.9039002541439,14.0711971157114));
#56077=CARTESIAN_POINT('Ctrl Pts',(38.3316507930811,-37.8333028094348,14.063888721046));
#56078=CARTESIAN_POINT('Ctrl Pts',(38.4325424620227,-37.7762177647969,14.0565803263806));
#56079=CARTESIAN_POINT('Ctrl Pts',(38.4345426068235,-37.7764071067806,14.1934196736194));
#56080=CARTESIAN_POINT('Ctrl Pts',(38.2580569790832,-37.8781526020867,14.2061916163845));
#56081=CARTESIAN_POINT('Ctrl Pts',(38.104957080975,-38.0203170861652,14.2189635591495));
#56082=CARTESIAN_POINT('Ctrl Pts',(37.9966332783609,-38.1909038725227,14.2317355019146));
#56083=CARTESIAN_POINT('Ctrl Pts',(37.7746880461016,-38.5404200730695,14.2579040053735));
#56084=CARTESIAN_POINT('Ctrl Pts',(37.7407134737351,-39.0092534864306,14.2840725088324));
#56085=CARTESIAN_POINT('Ctrl Pts',(37.9098581438109,-39.3871556515897,14.3102410122914));
#56086=CARTESIAN_POINT('Ctrl Pts',(38.0790028138868,-39.7650578167487,14.3364095157503));
#56087=CARTESIAN_POINT('Ctrl Pts',(38.451266726405,-40.0520287337056,14.3625780192092));
#56088=CARTESIAN_POINT('Ctrl Pts',(38.8597647299447,-40.1193961008257,14.3887465226681));
#56089=CARTESIAN_POINT('Ctrl Pts',(39.2682627334845,-40.1867634679457,14.4149150261271));
#56090=CARTESIAN_POINT('Ctrl Pts',(39.7129948280458,-40.034527285229,14.441083529586));
#56091=CARTESIAN_POINT('Ctrl Pts',(39.9945169439557,-39.730947693679,14.4672520330449));
#56092=CARTESIAN_POINT('Ctrl Pts',(40.2760390598657,-39.4273681021289,14.4934205365039));
#56093=CARTESIAN_POINT('Ctrl Pts',(40.3943511971241,-38.9724451017455,14.5195890399628));
#56094=CARTESIAN_POINT('Ctrl Pts',(40.2964110981383,-38.570173729657,14.5457575434217));
#56095=CARTESIAN_POINT('Ctrl Pts',(40.1984709991525,-38.1679023575684,14.5719260468806));
#56096=CARTESIAN_POINT('Ctrl Pts',(39.8842786639224,-37.8182826137747,14.5980945503396));
#56097=CARTESIAN_POINT('Ctrl Pts',(39.4947165862021,-37.6780870841148,14.6242630537985));
#56098=CARTESIAN_POINT('Ctrl Pts',(39.1515458154337,-37.5545868495612,14.6473152604055));
#56099=CARTESIAN_POINT('Ctrl Pts',(38.7498873821672,-37.5936018678201,14.6703674670124));
#56100=CARTESIAN_POINT('Ctrl Pts',(38.4322601856233,-37.7739115851766,14.6934196736194));
#56101=CARTESIAN_POINT('Origin',(39.0658530619283,-38.8697713466883,15.5));
#56102=CARTESIAN_POINT('',(38.4346334551116,-37.7742886171168,15.1934196736194));
#56103=CARTESIAN_POINT('',(38.4347780105726,-37.7761824162226,15.0565803263806));
#56104=CARTESIAN_POINT('',(38.4336030619283,-37.7746822236028,15.5));
#56105=CARTESIAN_POINT('Ctrl Pts',(38.4347780105726,-37.7761824162226,15.0565803263806));
#56106=CARTESIAN_POINT('Ctrl Pts',(38.6003617341531,-37.6801555214811,15.0445774292198));
#56107=CARTESIAN_POINT('Ctrl Pts',(38.7864577331935,-37.6199570207433,15.032574532059));
#56108=CARTESIAN_POINT('Ctrl Pts',(38.9758802222154,-37.6064663135108,15.0205716348981));
#56109=CARTESIAN_POINT('Ctrl Pts',(39.3888557724309,-37.5770541129272,14.9944031314392));
#56110=CARTESIAN_POINT('Ctrl Pts',(39.8176427771529,-37.7696531482711,14.9682346279803));
#56111=CARTESIAN_POINT('Ctrl Pts',(40.0699686232679,-38.097899483489,14.9420661245214));
#56112=CARTESIAN_POINT('Ctrl Pts',(40.3222944693828,-38.4261458187069,14.9158976210624));
#56113=CARTESIAN_POINT('Ctrl Pts',(40.3981591568908,-38.8900394537989,14.8897291176035));
#56114=CARTESIAN_POINT('Ctrl Pts',(40.2635428887314,-39.2815654536187,14.8635606141446));
#56115=CARTESIAN_POINT('Ctrl Pts',(40.1289266205721,-39.6730914534386,14.8373921106856));
#56116=CARTESIAN_POINT('Ctrl Pts',(39.7838293967455,-39.9922498179864,14.8112236072267));
#56117=CARTESIAN_POINT('Ctrl Pts',(39.3829992856624,-40.0959251593026,14.7850551037678));
#56118=CARTESIAN_POINT('Ctrl Pts',(38.9821691745794,-40.1996005006187,14.7588866003089));
#56119=CARTESIAN_POINT('Ctrl Pts',(38.5256061762399,-40.0877928187031,14.7327180968499));
#56120=CARTESIAN_POINT('Ctrl Pts',(38.2180337582993,-39.8106400014137,14.706549593391));
#56121=CARTESIAN_POINT('Ctrl Pts',(37.9104613403587,-39.5334871841242,14.6803810899321));
#56122=CARTESIAN_POINT('Ctrl Pts',(37.7518795028168,-39.0909892314609,14.6542125864732));
#56123=CARTESIAN_POINT('Ctrl Pts',(37.8134079754514,-38.6815634416151,14.6280440830142));
#56124=CARTESIAN_POINT('Ctrl Pts',(37.869417493424,-38.308862151417,14.604222830803));
#56125=CARTESIAN_POINT('Ctrl Pts',(38.1078215318972,-37.963566125762,14.5804015785918));
#56126=CARTESIAN_POINT('Ctrl Pts',(38.4333416483911,-37.7729821125454,14.5565803263806));
#56127=CARTESIAN_POINT('Ctrl Pts',(38.4322601856233,-37.7739115851766,14.6934196736194));
#56128=CARTESIAN_POINT('Ctrl Pts',(38.389321969358,-37.7982866315292,14.6965359704714));
#56129=CARTESIAN_POINT('Ctrl Pts',(38.3479194071466,-37.825243810264,14.6996522673233));
#56130=CARTESIAN_POINT('Ctrl Pts',(38.308404587142,-37.854730696716,14.7027685641753));
#56131=CARTESIAN_POINT('Ctrl Pts',(37.976586486013,-38.102341154503,14.7289370676342));
#56132=CARTESIAN_POINT('Ctrl Pts',(37.7778821039655,-38.528333385603,14.7551055710931));
#56133=CARTESIAN_POINT('Ctrl Pts',(37.8013916118277,-38.941687151427,14.781274074552));
#56134=CARTESIAN_POINT('Ctrl Pts',(37.8249011196899,-39.355040917251,14.807442578011));
#56135=CARTESIAN_POINT('Ctrl Pts',(38.0706245174618,-39.7557562177991,14.8336110814699));
#56136=CARTESIAN_POINT('Ctrl Pts',(38.428377122171,-39.9641476765195,14.8597795849288));
#56137=CARTESIAN_POINT('Ctrl Pts',(38.7861297268802,-40.1725391352399,14.8859480883877));
#56138=CARTESIAN_POINT('Ctrl Pts',(39.2559115385268,-40.1886067521326,14.9121165918467));
#56139=CARTESIAN_POINT('Ctrl Pts',(39.6270665080505,-40.005145553951,14.9382850953056));
#56140=CARTESIAN_POINT('Ctrl Pts',(39.9982214775741,-39.8216843557693,14.9644535987645));
#56141=CARTESIAN_POINT('Ctrl Pts',(40.2707496049748,-39.4386943425132,14.9906221022235));
#56142=CARTESIAN_POINT('Ctrl Pts',(40.3224461866044,-39.0279128196441,15.0167906056824));
#56143=CARTESIAN_POINT('Ctrl Pts',(40.3741427682341,-38.6171312967749,15.0429591091413));
#56144=CARTESIAN_POINT('Ctrl Pts',(40.2050078040926,-38.1785582642928,15.0691276126002));
#56145=CARTESIAN_POINT('Ctrl Pts',(39.8908833495191,-37.9088550679237,15.0952961160591));
#56146=CARTESIAN_POINT('Ctrl Pts',(39.5767588949455,-37.6391518715546,15.1214646195181));
#56147=CARTESIAN_POINT('Ctrl Pts',(39.1176449499399,-37.5383185112986,15.147633122977));
#56148=CARTESIAN_POINT('Ctrl Pts',(38.7194137008705,-37.6515698720153,15.1738016264359));
#56149=CARTESIAN_POINT('Ctrl Pts',(38.6198981458899,-37.679870694817,15.1803409754971));
#56150=CARTESIAN_POINT('Ctrl Pts',(38.5241845298854,-37.7215404565648,15.1868803245583));
#56151=CARTESIAN_POINT('Ctrl Pts',(38.4346334551116,-37.7742886171168,15.1934196736194));
#56152=CARTESIAN_POINT('Origin',(39.0658530619283,-38.8697713466883,15.5));
#56153=CARTESIAN_POINT('',(38.4337315549884,-37.7763335227174,15.6934196736194));
#56154=CARTESIAN_POINT('',(38.4323663903519,-37.7745195378426,15.5565803263806));
#56155=CARTESIAN_POINT('',(38.4336030619283,-37.7746822236028,15.5));
#56156=CARTESIAN_POINT('Ctrl Pts',(38.4323663903519,-37.7745195378426,15.5565803263806));
#56157=CARTESIAN_POINT('Ctrl Pts',(38.7313730076301,-37.6052990985956,15.5349217833067));
#56158=CARTESIAN_POINT('Ctrl Pts',(39.1034689296549,-37.5582680121359,15.5132632402327));
#56159=CARTESIAN_POINT('Ctrl Pts',(39.4315419163111,-37.6572094658042,15.4916046971588));
#56160=CARTESIAN_POINT('Ctrl Pts',(39.8279295706787,-37.7767535073269,15.4654361936999));
#56161=CARTESIAN_POINT('Ctrl Pts',(40.1600516656646,-38.1093911753228,15.439267690241));
#56162=CARTESIAN_POINT('Ctrl Pts',(40.2789807143,-38.5059637820165,15.413099186782));
#56163=CARTESIAN_POINT('Ctrl Pts',(40.3979097629354,-38.9025363887101,15.3869306833231));
#56164=CARTESIAN_POINT('Ctrl Pts',(40.3036457652202,-39.3630439341015,15.3607621798642));
#56165=CARTESIAN_POINT('Ctrl Pts',(40.0384578014032,-39.6809893678464,15.3345936764052));
#56166=CARTESIAN_POINT('Ctrl Pts',(39.7732698375861,-39.9989348015912,15.3084251729463));
#56167=CARTESIAN_POINT('Ctrl Pts',(39.3371579076672,-40.1743181236895,15.2822566694874));
#56168=CARTESIAN_POINT('Ctrl Pts',(38.9256798191233,-40.1284953536109,15.2560881660285));
#56169=CARTESIAN_POINT('Ctrl Pts',(38.5142017305793,-40.0826725835323,15.2299196625696));
#56170=CARTESIAN_POINT('Ctrl Pts',(38.1273574834104,-39.8156437212769,15.2037511591106));
#56171=CARTESIAN_POINT('Ctrl Pts',(37.938612567216,-39.4471477114983,15.1775826556517));
#56172=CARTESIAN_POINT('Ctrl Pts',(37.7498676510216,-39.0786517017197,15.1514141521928));
#56173=CARTESIAN_POINT('Ctrl Pts',(37.7592220658018,-38.6086885444181,15.1252456487338));
#56174=CARTESIAN_POINT('Ctrl Pts',(37.9624813210464,-38.2479952475117,15.0990771452749));
#56175=CARTESIAN_POINT('Ctrl Pts',(38.0725101803872,-38.0527437595403,15.0849115389768));
#56176=CARTESIAN_POINT('Ctrl Pts',(38.239359037454,-37.8895116538819,15.0707459326787));
#56177=CARTESIAN_POINT('Ctrl Pts',(38.4347780105726,-37.7761824162226,15.0565803263806));
#56178=CARTESIAN_POINT('Ctrl Pts',(38.4346334551116,-37.7742886171168,15.1934196736194));
#56179=CARTESIAN_POINT('Ctrl Pts',(38.1658281265106,-37.9326226925712,15.2130488280172));
#56180=CARTESIAN_POINT('Ctrl Pts',(37.9525484899569,-38.1907752905068,15.2326779824149));
#56181=CARTESIAN_POINT('Ctrl Pts',(37.8586391249354,-38.4867967233546,15.2523071368127));
#56182=CARTESIAN_POINT('Ctrl Pts',(37.7334443512028,-38.881436132288,15.2784756402716));
#56183=CARTESIAN_POINT('Ctrl Pts',(37.8204033568707,-39.3433788684654,15.3046441437306));
#56184=CARTESIAN_POINT('Ctrl Pts',(38.0805226988896,-39.6654843197862,15.3308126471895));
#56185=CARTESIAN_POINT('Ctrl Pts',(38.3406420409085,-39.987589771107,15.3569811506484));
#56186=CARTESIAN_POINT('Ctrl Pts',(38.7739217192785,-40.1698579375713,15.3831496541074));
#56187=CARTESIAN_POINT('Ctrl Pts',(39.1860739715826,-40.1305576058448,15.4093181575663));
#56188=CARTESIAN_POINT('Ctrl Pts',(39.5982262238866,-40.0912572741182,15.4354866610252));
#56189=CARTESIAN_POINT('Ctrl Pts',(39.9892510501248,-39.8303884442009,15.4616551644841));
#56190=CARTESIAN_POINT('Ctrl Pts',(40.1838082722999,-39.4649278007734,15.4878236679431));
#56191=CARTESIAN_POINT('Ctrl Pts',(40.378365494475,-39.0994671573459,15.513992171402));
#56192=CARTESIAN_POINT('Ctrl Pts',(40.3764551125871,-38.6294147004082,15.5401606748609));
#56193=CARTESIAN_POINT('Ctrl Pts',(40.1789337635325,-38.2655475388609,15.5663291783198));
#56194=CARTESIAN_POINT('Ctrl Pts',(39.9814124144778,-37.9016803773136,15.5924976817788));
#56195=CARTESIAN_POINT('Ctrl Pts',(39.5882800982564,-37.6439985111568,15.6186661852377));
#56196=CARTESIAN_POINT('Ctrl Pts',(39.175822019074,-37.6080495523001,15.6448346886966));
#56197=CARTESIAN_POINT('Ctrl Pts',(38.9205626180181,-37.5858016920459,15.6610296836709));
#56198=CARTESIAN_POINT('Ctrl Pts',(38.6579013630336,-37.6484785302017,15.6772246786452));
#56199=CARTESIAN_POINT('Ctrl Pts',(38.4337315549884,-37.7763335227174,15.6934196736194));
#56200=CARTESIAN_POINT('Origin',(39.0658530619283,-38.8697713466883,15.5));
#56201=CARTESIAN_POINT('',(38.4325272584341,-37.7729978925048,16.1934196736194));
#56202=CARTESIAN_POINT('',(38.4342758514651,-37.7737507965446,16.0565803263806));
#56203=CARTESIAN_POINT('',(38.4336030619283,-37.7746822236028,15.5));
#56204=CARTESIAN_POINT('Ctrl Pts',(38.4342758514651,-37.7737507965446,16.0565803263806));
#56205=CARTESIAN_POINT('Ctrl Pts',(38.5046440871601,-37.732289208729,16.0514346408525));
#56206=CARTESIAN_POINT('Ctrl Pts',(38.5788878157804,-37.6977955005524,16.0462889553244));
#56207=CARTESIAN_POINT('Ctrl Pts',(38.655917096454,-37.6714445317292,16.0411432697963));
#56208=CARTESIAN_POINT('Ctrl Pts',(39.0476512952768,-37.5374360667673,16.0149747663373));
#56209=CARTESIAN_POINT('Ctrl Pts',(39.5114269646143,-37.6140195799122,15.9888062628784));
#56210=CARTESIAN_POINT('Ctrl Pts',(39.8392815814542,-37.8668541135745,15.9626377594195));
#56211=CARTESIAN_POINT('Ctrl Pts',(40.1671361982941,-38.1196886472368,15.9364692559606));
#56212=CARTESIAN_POINT('Ctrl Pts',(40.3590697626365,-38.5487742014165,15.9103007525016));
#56213=CARTESIAN_POINT('Ctrl Pts',(40.3290169828723,-38.9617037131001,15.8841322490427));
#56214=CARTESIAN_POINT('Ctrl Pts',(40.2989642031081,-39.3746332247836,15.8579637455838));
#56215=CARTESIAN_POINT('Ctrl Pts',(40.0469250792374,-39.771406693971,15.8317952421249));
#56216=CARTESIAN_POINT('Ctrl Pts',(39.685916950104,-39.974106180808,15.8056267386659));
#56217=CARTESIAN_POINT('Ctrl Pts',(39.3249088209707,-40.176805667645,15.779458235207));
#56218=CARTESIAN_POINT('Ctrl Pts',(38.8549316865748,-40.1854311721316,15.7532897317481));
#56219=CARTESIAN_POINT('Ctrl Pts',(38.4867288810042,-39.9961149153208,15.7271212282891));
#56220=CARTESIAN_POINT('Ctrl Pts',(38.1185260754337,-39.80679865851,15.7009527248302));
#56221=CARTESIAN_POINT('Ctrl Pts',(37.8520975986886,-39.4195406404018,15.6747842213713));
#56222=CARTESIAN_POINT('Ctrl Pts',(37.806913145733,-39.0079919599958,15.6486157179124));
#56223=CARTESIAN_POINT('Ctrl Pts',(37.7617286927774,-38.5964432795899,15.6224472144534));
#56224=CARTESIAN_POINT('Ctrl Pts',(37.9377882636112,-38.1606039368862,15.5962787109945));
#56225=CARTESIAN_POINT('Ctrl Pts',(38.2561446559027,-37.8959094730591,15.5701102075356));
#56226=CARTESIAN_POINT('Ctrl Pts',(38.3110111758702,-37.8502912149167,15.5656002471506));
#56227=CARTESIAN_POINT('Ctrl Pts',(38.3701042153674,-37.8097563252262,15.5610902867656));
#56228=CARTESIAN_POINT('Ctrl Pts',(38.4323663903519,-37.7745195378426,15.5565803263806));
#56229=CARTESIAN_POINT('Ctrl Pts',(38.4337315549884,-37.7763335227174,15.6934196736194));
#56230=CARTESIAN_POINT('Ctrl Pts',(38.2956790587637,-37.8550716053588,15.7033931821041));
#56231=CARTESIAN_POINT('Ctrl Pts',(38.1722247361697,-37.9585289981308,15.7133666905887));
#56232=CARTESIAN_POINT('Ctrl Pts',(38.0740874997392,-38.082093666717,15.7233401990734));
#56233=CARTESIAN_POINT('Ctrl Pts',(37.8165949017303,-38.4063027915471,15.7495087025323));
#56234=CARTESIAN_POINT('Ctrl Pts',(37.7333935478558,-38.868937092764,15.7756772059912));
#56235=CARTESIAN_POINT('Ctrl Pts',(37.8617919143246,-39.2625458504732,15.8018457094502));
#56236=CARTESIAN_POINT('Ctrl Pts',(37.9901902807933,-39.6561546081824,15.8280142129091));
#56237=CARTESIAN_POINT('Ctrl Pts',(38.3301883676052,-39.9807378223839,15.854182716368));
#56238=CARTESIAN_POINT('Ctrl Pts',(38.7293269910636,-40.0907485215641,15.8803512198269));
#56239=CARTESIAN_POINT('Ctrl Pts',(39.128465614522,-40.2007592207443,15.9065197232859));
#56240=CARTESIAN_POINT('Ctrl Pts',(39.5867447746269,-40.0961974049031,15.9326882267448));
#56241=CARTESIAN_POINT('Ctrl Pts',(39.898666648561,-39.8239498351585,15.9588567302037));
#56242=CARTESIAN_POINT('Ctrl Pts',(40.2105885224951,-39.551702265414,15.9850252336627));
#56243=CARTESIAN_POINT('Ctrl Pts',(40.3761531102584,-39.1117689417661,16.0111937371216));
#56244=CARTESIAN_POINT('Ctrl Pts',(40.321119282596,-38.701421195982,16.0373622405805));
#56245=CARTESIAN_POINT('Ctrl Pts',(40.2660854549337,-38.291073450198,16.0635307440394));
#56246=CARTESIAN_POINT('Ctrl Pts',(39.9904532118457,-37.9103112822778,16.0896992474984));
#56247=CARTESIAN_POINT('Ctrl Pts',(39.6178193276329,-37.7298729742913,16.1158677509573));
#56248=CARTESIAN_POINT('Ctrl Pts',(39.2497117383559,-37.5516264074059,16.1417183918447));
#56249=CARTESIAN_POINT('Ctrl Pts',(38.7869447075705,-37.5688666846834,16.167569032732));
#56250=CARTESIAN_POINT('Ctrl Pts',(38.4325272584341,-37.7729978925048,16.1934196736194));
#56251=CARTESIAN_POINT('Origin',(39.0658530619283,-38.8697713466883,15.5));
#56252=CARTESIAN_POINT('',(38.4349705604869,-37.7753960169021,16.6934196736194));
#56253=CARTESIAN_POINT('',(38.4341423505256,-37.7764525809616,16.5565803263806));
#56254=CARTESIAN_POINT('',(38.4336030619283,-37.7746822236028,15.5));
#56255=CARTESIAN_POINT('Ctrl Pts',(38.4341423505256,-37.7764525809616,16.5565803263806));
#56256=CARTESIAN_POINT('Ctrl Pts',(38.6388834301988,-37.6590722267018,16.5417789949394));
#56257=CARTESIAN_POINT('Ctrl Pts',(38.8753711836181,-37.5959619576061,16.5269776634982));
#56258=CARTESIAN_POINT('Ctrl Pts',(39.1094100531276,-37.604015667637,16.5121763320569));
#56259=CARTESIAN_POINT('Ctrl Pts',(39.52318681305,-37.6182544906534,16.486007828598));
#56260=CARTESIAN_POINT('Ctrl Pts',(39.929308939441,-37.8549351283607,16.4598393251391));
#56261=CARTESIAN_POINT('Ctrl Pts',(40.1456664429883,-38.2079271704546,16.4336708216802));
#56262=CARTESIAN_POINT('Ctrl Pts',(40.3620239465357,-38.5609192125485,16.4075023182212));
#56263=CARTESIAN_POINT('Ctrl Pts',(40.3886168272394,-39.0302226590291,16.3813338147623));
#56264=CARTESIAN_POINT('Ctrl Pts',(40.2135205214552,-39.4053962654636,16.3551653113034));
#56265=CARTESIAN_POINT('Ctrl Pts',(40.0384242156709,-39.780569871898,16.3289968078445));
#56266=CARTESIAN_POINT('Ctrl Pts',(39.6616387233988,-40.0616136382864,16.3028283043855));
#56267=CARTESIAN_POINT('Ctrl Pts',(39.2521191380692,-40.122504199314,16.2766598009266));
#56268=CARTESIAN_POINT('Ctrl Pts',(38.8425995527396,-40.1833947603416,16.2504912974677));
#56269=CARTESIAN_POINT('Ctrl Pts',(38.4003458743526,-40.0241321160084,16.2243227940088));
#56270=CARTESIAN_POINT('Ctrl Pts',(38.1236699093341,-39.716131529034,16.1981542905498));
#56271=CARTESIAN_POINT('Ctrl Pts',(37.8469939443156,-39.4081309420596,16.1719857870909));
#56272=CARTESIAN_POINT('Ctrl Pts',(37.7358956926655,-38.951392412444,16.145817283632));
#56273=CARTESIAN_POINT('Ctrl Pts',(37.8401929309945,-38.5507229261019,16.119648780173));
#56274=CARTESIAN_POINT('Ctrl Pts',(37.9239815150653,-38.2288397249847,16.0986259622422));
#56275=CARTESIAN_POINT('Ctrl Pts',(38.1467847875343,-37.9431430780994,16.0776031443114));
#56276=CARTESIAN_POINT('Ctrl Pts',(38.4342758514651,-37.7737507965446,16.0565803263806));
#56277=CARTESIAN_POINT('Ctrl Pts',(38.4325272584341,-37.7729978925048,16.1934196736194));
#56278=CARTESIAN_POINT('Ctrl Pts',(38.4281692990986,-37.775507914246,16.193737536191));
#56279=CARTESIAN_POINT('Ctrl Pts',(38.42382772163,-37.7780461928786,16.1940553987625));
#56280=CARTESIAN_POINT('Ctrl Pts',(38.4195029034437,-37.7806127124219,16.1943732613341));
#56281=CARTESIAN_POINT('Ctrl Pts',(38.0634558888049,-37.9919052065918,16.220541764793));
#56282=CARTESIAN_POINT('Ctrl Pts',(37.8209973848649,-38.3946046429843,16.2467102682519));
#56283=CARTESIAN_POINT('Ctrl Pts',(37.8008486672722,-38.8081358071838,16.2728787717108));
#56284=CARTESIAN_POINT('Ctrl Pts',(37.7806999496795,-39.2216669713833,16.2990472751698));
#56285=CARTESIAN_POINT('Ctrl Pts',(37.9828610184341,-39.6460298633899,16.3252157786287));
#56286=CARTESIAN_POINT('Ctrl Pts',(38.3166804464026,-39.8909351187556,16.3513842820876));
#56287=CARTESIAN_POINT('Ctrl Pts',(38.6504998743712,-40.1358403741212,16.3775527855466));
#56288=CARTESIAN_POINT('Ctrl Pts',(39.1159776615536,-40.2012879928461,16.4037212890055));
#56289=CARTESIAN_POINT('Ctrl Pts',(39.5043880368528,-40.0579304834052,16.4298897924644));
#56290=CARTESIAN_POINT('Ctrl Pts',(39.8927984121519,-39.9145729739643,16.4560582959233));
#56291=CARTESIAN_POINT('Ctrl Pts',(40.2041413755678,-39.5624103363577,16.4822267993823));
#56292=CARTESIAN_POINT('Ctrl Pts',(40.2988070379275,-39.1593564860685,16.5083953028412));
#56293=CARTESIAN_POINT('Ctrl Pts',(40.3934727002873,-38.7563026357793,16.5345638063001));
#56294=CARTESIAN_POINT('Ctrl Pts',(40.271461061591,-38.3023575728076,16.560732309759));
#56295=CARTESIAN_POINT('Ctrl Pts',(39.9874835980573,-38.001075653904,16.586900813218));
#56296=CARTESIAN_POINT('Ctrl Pts',(39.7035061345236,-37.6997937350005,16.6130693166769));
#56297=CARTESIAN_POINT('Ctrl Pts',(39.2575628461526,-37.5511749601651,16.6392378201358));
#56298=CARTESIAN_POINT('Ctrl Pts',(38.849619989904,-37.6218617656895,16.6654063235948));
#56299=CARTESIAN_POINT('Ctrl Pts',(38.7040525518055,-37.6470851444788,16.6747441069363));
#56300=CARTESIAN_POINT('Ctrl Pts',(38.5633236984099,-37.7002326432607,16.6840818902779));
#56301=CARTESIAN_POINT('Ctrl Pts',(38.4349705604869,-37.7753960169021,16.6934196736194));
#56302=CARTESIAN_POINT('Origin',(39.0658530619283,-38.8697713466883,15.5));
#56303=CARTESIAN_POINT('',(38.4329072841441,-37.7756148875603,17.1934196736194));
#56304=CARTESIAN_POINT('',(38.4323100738575,-37.7733715239653,17.0565803263806));
#56305=CARTESIAN_POINT('',(38.4336030619283,-37.7746822236028,15.5));
#56306=CARTESIAN_POINT('Ctrl Pts',(38.4323100738575,-37.7733715239653,17.0565803263806));
#56307=CARTESIAN_POINT('Ctrl Pts',(38.7684978446967,-37.5814140598882,17.0321233490263));
#56308=CARTESIAN_POINT('Ctrl Pts',(39.2005574419278,-37.5523442127138,17.0076663716719));
#56309=CARTESIAN_POINT('Ctrl Pts',(39.5571950289671,-37.7024591900708,16.9832093943176));
#56310=CARTESIAN_POINT('Ctrl Pts',(39.9387905055794,-37.8630793782195,16.9570408908587));
#56311=CARTESIAN_POINT('Ctrl Pts',(40.2340383736987,-38.2288410235792,16.9308723873998));
#56312=CARTESIAN_POINT('Ctrl Pts',(40.3105459562687,-38.635732327761,16.9047038839408));
#56313=CARTESIAN_POINT('Ctrl Pts',(40.3870535388386,-39.0426236319427,16.8785353804819));
#56314=CARTESIAN_POINT('Ctrl Pts',(40.2448208358592,-39.4906445949467,16.852366877023));
#56315=CARTESIAN_POINT('Ctrl Pts',(39.9476266935978,-39.7788972563362,16.8261983735641));
#56316=CARTESIAN_POINT('Ctrl Pts',(39.6504325513363,-40.0671499177256,16.8000298701051));
#56317=CARTESIAN_POINT('Ctrl Pts',(39.1982769697929,-40.1956342775007,16.7738613666462));
#56318=CARTESIAN_POINT('Ctrl Pts',(38.7939118807236,-40.1067364387691,16.7476928631873));
#56319=CARTESIAN_POINT('Ctrl Pts',(38.3895467916544,-40.0178386000374,16.7215243597284));
#56320=CARTESIAN_POINT('Ctrl Pts',(38.0329721950594,-39.7115585627991,16.6953558562694));
#56321=CARTESIAN_POINT('Ctrl Pts',(37.8840803814008,-39.3252359279146,16.6691873528105));
#56322=CARTESIAN_POINT('Ctrl Pts',(37.7351885677422,-38.9389132930302,16.6430188493516));
#56323=CARTESIAN_POINT('Ctrl Pts',(37.7939795370199,-38.4725480604997,16.6168503458927));
#56324=CARTESIAN_POINT('Ctrl Pts',(38.0340907183856,-38.1352639483972,16.5906818424337));
#56325=CARTESIAN_POINT('Ctrl Pts',(38.1383911078307,-37.9887532193016,16.579314670416));
#56326=CARTESIAN_POINT('Ctrl Pts',(38.2769046668091,-37.8665987062389,16.5679474983983));
#56327=CARTESIAN_POINT('Ctrl Pts',(38.4341423505256,-37.7764525809616,16.5565803263806));
#56328=CARTESIAN_POINT('Ctrl Pts',(38.4349705604869,-37.7753960169021,16.6934196736194));
#56329=CARTESIAN_POINT('Ctrl Pts',(38.2036227489615,-37.9108728917196,16.7102503937368));
#56330=CARTESIAN_POINT('Ctrl Pts',(38.0124806835606,-38.1178740898995,16.7270811138542));
#56331=CARTESIAN_POINT('Ctrl Pts',(37.9056793271332,-38.3618028680121,16.7439118339715));
#56332=CARTESIAN_POINT('Ctrl Pts',(37.7396239447373,-38.7410647789262,16.7700803374304));
#56333=CARTESIAN_POINT('Ctrl Pts',(37.7774556040718,-39.2095962148701,16.7962488408894));
#56334=CARTESIAN_POINT('Ctrl Pts',(38.0022100801907,-39.5573021560724,16.8224173443483));
#56335=CARTESIAN_POINT('Ctrl Pts',(38.2269645563097,-39.9050080972747,16.8485858478072));
#56336=CARTESIAN_POINT('Ctrl Pts',(38.6386418492131,-40.1318885437354,16.8747543512661));
#56337=CARTESIAN_POINT('Ctrl Pts',(39.0526410872976,-40.1362075141883,16.9009228547251));
#56338=CARTESIAN_POINT('Ctrl Pts',(39.4666403253821,-40.1405264846412,16.927091358184));
#56339=CARTESIAN_POINT('Ctrl Pts',(39.8829615086478,-39.9222839790864,16.9532598616429));
#56340=CARTESIAN_POINT('Ctrl Pts',(40.1149210262726,-39.5793427181871,16.9794283651019));
#56341=CARTESIAN_POINT('Ctrl Pts',(40.3468805438973,-39.2364014572879,17.0055968685608));
#56342=CARTESIAN_POINT('Ctrl Pts',(40.3944783958811,-38.7687614410443,17.0317653720197));
#56343=CARTESIAN_POINT('Ctrl Pts',(40.236371633473,-38.3861176323113,17.0579338754786));
#56344=CARTESIAN_POINT('Ctrl Pts',(40.0782648710649,-38.0034738235784,17.0841023789376));
#56345=CARTESIAN_POINT('Ctrl Pts',(39.7144534942649,-37.7058262223562,17.1102708823965));
#56346=CARTESIAN_POINT('Ctrl Pts',(39.3080738473792,-37.6266443201348,17.1364393858554));
#56347=CARTESIAN_POINT('Ctrl Pts',(39.0131183836182,-37.5691730986546,17.1554328151101));
#56348=CARTESIAN_POINT('Ctrl Pts',(38.6957377885278,-37.6267904626672,17.1744262443648));
#56349=CARTESIAN_POINT('Ctrl Pts',(38.4329072841441,-37.7756148875603,17.1934196736194));
#56350=CARTESIAN_POINT('Origin',(39.0658530619283,-38.8697713466883,15.5));
#56351=CARTESIAN_POINT('',(38.4333577759012,-37.7730251466968,17.6934196736194));
#56352=CARTESIAN_POINT('',(38.4348713855213,-37.7748596688487,17.5565803263806));
#56353=CARTESIAN_POINT('',(38.4336030619283,-37.7746822236028,15.5));
#56354=CARTESIAN_POINT('',(40.2595650866584,-39.2869186252539,18.));
#56355=CARTESIAN_POINT('Ctrl Pts',(38.4333577759012,-37.7730251466968,17.6934196736194));
#56356=CARTESIAN_POINT('Ctrl Pts',(38.1097262681979,-37.9625959827323,17.7171076053695));
#56357=CARTESIAN_POINT('Ctrl Pts',(37.8720798795256,-38.3048233518517,17.7407955371196));
#56358=CARTESIAN_POINT('Ctrl Pts',(37.8144498218249,-38.6752097670202,17.7644834688697));
#56359=CARTESIAN_POINT('Ctrl Pts',(37.7507848138289,-39.084382601894,17.7906519723286));
#56360=CARTESIAN_POINT('Ctrl Pts',(37.9068123877648,-39.5279208384948,17.8168204757875));
#56361=CARTESIAN_POINT('Ctrl Pts',(38.2131597275406,-39.8064869141387,17.8429889792464));
#56362=CARTESIAN_POINT('Ctrl Pts',(38.5195070673165,-40.0850529897826,17.8691574827054));
#56363=CARTESIAN_POINT('Ctrl Pts',(38.9761741729324,-40.1986469044696,17.8953259861643));
#56364=CARTESIAN_POINT('Ctrl Pts',(39.3768946753638,-40.0972493078634,17.9214944896232));
#56365=CARTESIAN_POINT('Ctrl Pts',(39.7776151777952,-39.9958517112573,17.9476629930822));
#56366=CARTESIAN_POINT('Ctrl Pts',(40.1223890770422,-39.679462603358,17.9738314965411));
#56367=CARTESIAN_POINT('Ctrl Pts',(40.2595650866584,-39.2869186252539,18.));
#56368=CARTESIAN_POINT('',(39.301526156426,-37.6253017999342,18.));
#56369=CARTESIAN_POINT('Origin',(39.0658530619283,-38.8697713466883,18.));
#56370=CARTESIAN_POINT('Ctrl Pts',(39.301526596644,-37.6252897660473,18.));
#56371=CARTESIAN_POINT('Ctrl Pts',(39.6885864653113,-37.7000302410441,17.975091839613));
#56372=CARTESIAN_POINT('Ctrl Pts',(40.0399465491499,-37.9695057059562,17.950183679226));
#56373=CARTESIAN_POINT('Ctrl Pts',(40.2093266637559,-38.3254078043634,17.925275518839));
#56374=CARTESIAN_POINT('Ctrl Pts',(40.3872773452222,-38.6993184082982,17.89910701538));
#56375=CARTESIAN_POINT('Ctrl Pts',(40.3643659014498,-39.1686232325653,17.8729385119211));
#56376=CARTESIAN_POINT('Ctrl Pts',(40.1507520928543,-39.5232247114421,17.8467700084622));
#56377=CARTESIAN_POINT('Ctrl Pts',(39.9371382842589,-39.8778261903189,17.8206015050033));
#56378=CARTESIAN_POINT('Ctrl Pts',(39.5328221108402,-40.1177243238052,17.7944330015443));
#56379=CARTESIAN_POINT('Ctrl Pts',(39.1191596128741,-40.1351764464736,17.7682644980854));
#56380=CARTESIAN_POINT('Ctrl Pts',(38.705497114908,-40.1526285691419,17.7420959946265));
#56381=CARTESIAN_POINT('Ctrl Pts',(38.2824882923945,-39.9476346809923,17.7159274911676));
#56382=CARTESIAN_POINT('Ctrl Pts',(38.0397877964566,-39.6122000494564,17.6897589877086));
#56383=CARTESIAN_POINT('Ctrl Pts',(37.7970873005187,-39.2767654179205,17.6635904842497));
#56384=CARTESIAN_POINT('Ctrl Pts',(37.7346951311564,-38.8108900429983,17.6374219807908));
#56385=CARTESIAN_POINT('Ctrl Pts',(37.8806022560882,-38.4234367664048,17.6112534773319));
#56386=CARTESIAN_POINT('Ctrl Pts',(37.9822155342897,-38.1536048606431,17.5930290936814));
#56387=CARTESIAN_POINT('Ctrl Pts',(38.184855409418,-37.9218082144096,17.574804710031));
#56388=CARTESIAN_POINT('Ctrl Pts',(38.4348713855213,-37.7748596688487,17.5565803263806));
#56389=CARTESIAN_POINT('Origin',(39.0658530619283,-38.8697713466883,19.1042117235887));
#56390=CARTESIAN_POINT('',(38.2940340733258,-37.531419596366,14.3957882764113));
#56391=CARTESIAN_POINT('',(38.2954995370357,-37.5355989289915,14.3542117235887));
#56392=CARTESIAN_POINT('',(38.2943530619283,-37.5334941486488,19.1042117235887));
#56393=CARTESIAN_POINT('',(37.9741697098829,-39.9602191716056,14.));
#56394=CARTESIAN_POINT('Ctrl Pts',(38.2954995370357,-37.5355989289915,14.3542117235887));
#56395=CARTESIAN_POINT('Ctrl Pts',(38.5213873438295,-37.4053726489247,14.3408151628949));
#56396=CARTESIAN_POINT('Ctrl Pts',(39.2812420752165,-37.1810251467922,14.3012500987421));
#56397=CARTESIAN_POINT('Ctrl Pts',(40.5621358440548,-37.8394569175814,14.2355165311303));
#56398=CARTESIAN_POINT('Ctrl Pts',(40.7517455388365,-39.5501918673983,14.1570110207536));
#56399=CARTESIAN_POINT('Ctrl Pts',(39.4258164610498,-40.6499822516745,14.0785055103768));
#56400=CARTESIAN_POINT('Ctrl Pts',(38.3327559670706,-40.3192117233802,14.0261685034589));
#56401=CARTESIAN_POINT('Ctrl Pts',(37.9741697098829,-39.9602191716056,14.));
#56402=CARTESIAN_POINT('',(37.5730942570913,-39.2702598116583,14.));
#56403=CARTESIAN_POINT('Origin',(39.0658530619283,-38.8697713466883,14.));
#56404=CARTESIAN_POINT('Ctrl Pts',(38.2940340733258,-37.531419596366,14.3957882764113));
#56405=CARTESIAN_POINT('Ctrl Pts',(38.33317399173,-37.5085041378476,14.3934410251636));
#56406=CARTESIAN_POINT('Ctrl Pts',(38.8212071098193,-37.2523822679137,14.3649252704569));
#56407=CARTESIAN_POINT('Ctrl Pts',(40.0177412802272,-37.3220721610692,14.3102410122913));
#56408=CARTESIAN_POINT('Ctrl Pts',(40.8820235552811,-38.8100518816853,14.2317355019146));
#56409=CARTESIAN_POINT('Ctrl Pts',(40.1171224362185,-40.3517547545304,14.1532299915378));
#56410=CARTESIAN_POINT('Ctrl Pts',(38.4376290919279,-40.5606360835952,14.075984824233));
#56411=CARTESIAN_POINT('Ctrl Pts',(37.6993939872544,-39.7344135992462,14.024908160387));
#56412=CARTESIAN_POINT('Ctrl Pts',(37.5730796542559,-39.270261446955,14.));
#56413=CARTESIAN_POINT('Origin',(39.0658530619283,-38.8697713466883,19.1042117235887));
#56414=CARTESIAN_POINT('',(38.2957867873204,-37.5353247514265,14.8957882764113));
#56415=CARTESIAN_POINT('',(38.2927144236218,-37.5325537808421,14.8542117235887));
#56416=CARTESIAN_POINT('',(38.2943530619283,-37.5334941486488,19.1042117235887));
#56417=CARTESIAN_POINT('Ctrl Pts',(38.2927144236218,-37.5325537808421,14.8542117235887));
#56418=CARTESIAN_POINT('Ctrl Pts',(38.6802974716781,-37.3125317216241,14.8311595169817));
#56419=CARTESIAN_POINT('Ctrl Pts',(39.7267977629897,-37.2108801077358,14.7819388069158));
#56420=CARTESIAN_POINT('Ctrl Pts',(40.831316288814,-38.4399409113081,14.706549593391));
#56421=CARTESIAN_POINT('Ctrl Pts',(40.3982068515902,-40.1052936742774,14.6280440830142));
#56422=CARTESIAN_POINT('Ctrl Pts',(38.7701602990205,-40.6625900679474,14.5495385726375));
#56423=CARTESIAN_POINT('Ctrl Pts',(37.4074005907985,-39.6120654537969,14.4710330622607));
#56424=CARTESIAN_POINT('Ctrl Pts',(37.5105490854526,-38.1886638489127,14.4059241125778));
#56425=CARTESIAN_POINT('Ctrl Pts',(38.0801438046487,-37.6597533768028,14.3669836663538));
#56426=CARTESIAN_POINT('Ctrl Pts',(38.2954995370357,-37.5355989289915,14.3542117235887));
#56427=CARTESIAN_POINT('Ctrl Pts',(38.2957867873204,-37.5353247514265,14.8957882764113));
#56428=CARTESIAN_POINT('Ctrl Pts',(38.4978395239631,-37.4181483982544,14.8837853792504));
#56429=CARTESIAN_POINT('Ctrl Pts',(39.2200040297691,-37.1845419759791,14.8456139786307));
#56430=CARTESIAN_POINT('Ctrl Pts',(40.5064460859517,-37.7623754838001,14.7812740745521));
#56431=CARTESIAN_POINT('Ctrl Pts',(40.7841666383236,-39.4605673674226,14.7027685641753));
#56432=CARTESIAN_POINT('Ctrl Pts',(39.5208569909583,-40.6289217126118,14.6242630537985));
#56433=CARTESIAN_POINT('Ctrl Pts',(37.8495006293029,-40.2196233657656,14.5457575434217));
#56434=CARTESIAN_POINT('Ctrl Pts',(37.2863317343909,-38.6481881568849,14.4695992842926));
#56435=CARTESIAN_POINT('Ctrl Pts',(37.8968197279323,-37.7639788153404,14.4196095286225));
#56436=CARTESIAN_POINT('Ctrl Pts',(38.2940340733258,-37.531419596366,14.3957882764113));
#56437=CARTESIAN_POINT('Origin',(39.0658530619283,-38.8697713466883,19.1042117235887));
#56438=CARTESIAN_POINT('',(38.2928440194274,-37.5332956321379,15.3957882764113));
#56439=CARTESIAN_POINT('',(38.2956103942191,-37.5330138522408,15.3542117235887));
#56440=CARTESIAN_POINT('',(38.2943530619283,-37.5334941486488,19.1042117235887));
#56441=CARTESIAN_POINT('Ctrl Pts',(38.2956103942191,-37.5330138522408,15.3542117235887));
#56442=CARTESIAN_POINT('Ctrl Pts',(38.4048846594434,-37.4686481648294,15.3476723745276));
#56443=CARTESIAN_POINT('Ctrl Pts',(38.9890534180561,-37.2143251749767,15.3149645220075));
#56444=CARTESIAN_POINT('Ctrl Pts',(40.2495149974675,-37.4911553124802,15.2560881660285));
#56445=CARTESIAN_POINT('Ctrl Pts',(40.8686733596745,-39.0966551680434,15.1775826556517));
#56446=CARTESIAN_POINT('Ctrl Pts',(39.8710199775172,-40.4986802936762,15.0990771452749));
#56447=CARTESIAN_POINT('Ctrl Pts',(38.151273037136,-40.4398609986215,15.0205716348981));
#56448=CARTESIAN_POINT('Ctrl Pts',(37.2517446794564,-38.9729482851088,14.9420661245214));
#56449=CARTESIAN_POINT('Ctrl Pts',(37.7655552987949,-37.8714157983081,14.8866128207516));
#56450=CARTESIAN_POINT('Ctrl Pts',(38.2403192732087,-37.5622973130857,14.8573280204407));
#56451=CARTESIAN_POINT('Ctrl Pts',(38.2927144236218,-37.5325537808421,14.8542117235887));
#56452=CARTESIAN_POINT('Ctrl Pts',(38.2928440194274,-37.5332956321379,15.3957882764113));
#56453=CARTESIAN_POINT('Ctrl Pts',(38.6577053958294,-37.3268052108188,15.3741297333373));
#56454=CARTESIAN_POINT('Ctrl Pts',(39.6603483962762,-37.2000760884312,15.3263026868045));
#56455=CARTESIAN_POINT('Ctrl Pts',(40.8063139857151,-38.3478206288557,15.2523071368127));
#56456=CARTESIAN_POINT('Ctrl Pts',(40.4612384258705,-40.0336169338117,15.1738016264359));
#56457=CARTESIAN_POINT('Ctrl Pts',(38.8647480157521,-40.6756488816116,15.0952961160592));
#56458=CARTESIAN_POINT('Ctrl Pts',(37.4486135593306,-39.6981268544226,15.0167906056824));
#56459=CARTESIAN_POINT('Ctrl Pts',(37.4776219436003,-38.2407538193379,14.9502879924664));
#56460=CARTESIAN_POINT('Ctrl Pts',(38.057327731945,-37.6736142047347,14.9099538827094));
#56461=CARTESIAN_POINT('Ctrl Pts',(38.2957867873204,-37.5353247514265,14.8957882764113));
#56462=CARTESIAN_POINT('Origin',(39.0658530619283,-38.8697713466883,19.1042117235887));
#56463=CARTESIAN_POINT('',(38.2951740301017,-37.5323575792927,15.8957882764113));
#56464=CARTESIAN_POINT('',(38.2945098549624,-37.5355091383948,15.8542117235887));
#56465=CARTESIAN_POINT('',(38.2943530619283,-37.5334941486488,19.1042117235887));
#56466=CARTESIAN_POINT('Ctrl Pts',(38.2945098549624,-37.5355091383948,15.8542117235887));
#56467=CARTESIAN_POINT('Ctrl Pts',(38.5680519773933,-37.379494703083,15.8380167286145));
#56468=CARTESIAN_POINT('Ctrl Pts',(39.406457455491,-37.1794324424244,15.7956532301813));
#56469=CARTESIAN_POINT('Ctrl Pts',(40.6627777316899,-38.0028980795747,15.7271212282892));
#56470=CARTESIAN_POINT('Ctrl Pts',(40.6697711344255,-39.7236357807726,15.6486157179124));
#56471=CARTESIAN_POINT('Ctrl Pts',(39.2383326839261,-40.6786075590939,15.5701102075356));
#56472=CARTESIAN_POINT('Ctrl Pts',(37.6522103975089,-40.0113720173278,15.4916046971588));
#56473=CARTESIAN_POINT('Ctrl Pts',(37.3603930477839,-38.4611828913061,15.4196385358432));
#56474=CARTESIAN_POINT('Ctrl Pts',(37.9676019940362,-37.7262202408736,15.3738408779865));
#56475=CARTESIAN_POINT('Ctrl Pts',(38.2956103942191,-37.5330138522408,15.3542117235887));
#56476=CARTESIAN_POINT('Ctrl Pts',(38.2951740301017,-37.5323575792927,15.8957882764113));
#56477=CARTESIAN_POINT('Ctrl Pts',(38.381040528858,-37.4817642775928,15.8906425908832));
#56478=CARTESIAN_POINT('Ctrl Pts',(38.9323618573136,-37.2256198547756,15.8593284018961));
#56479=CARTESIAN_POINT('Ctrl Pts',(40.1754824724718,-37.430896996864,15.8018457094502));
#56480=CARTESIAN_POINT('Ctrl Pts',(40.8781004790678,-39.0016657040982,15.7233401990734));
#56481=CARTESIAN_POINT('Ctrl Pts',(39.9554519188484,-40.454148415738,15.6448346886966));
#56482=CARTESIAN_POINT('Ctrl Pts',(38.2349899535507,-40.4857241059463,15.5663291783198));
#56483=CARTESIAN_POINT('Ctrl Pts',(37.2596657788943,-39.0680749435716,15.4878236679431));
#56484=CARTESIAN_POINT('Ctrl Pts',(37.7263629251969,-37.9127558858068,15.4309767006402));
#56485=CARTESIAN_POINT('Ctrl Pts',(38.2168689019888,-37.5762931512624,15.4002982367963));
#56486=CARTESIAN_POINT('Ctrl Pts',(38.2928440194274,-37.5332956321379,15.3957882764113));
#56487=CARTESIAN_POINT('Origin',(39.0658530619283,-38.8697713466883,19.1042117235887));
#56488=CARTESIAN_POINT('',(38.295011126227,-37.5356544186406,16.3957882764113));
#56489=CARTESIAN_POINT('',(38.2930403179255,-37.5314388517851,16.3542117235887));
#56490=CARTESIAN_POINT('',(38.2943530619283,-37.5334941486488,19.1042117235887));
#56491=CARTESIAN_POINT('Ctrl Pts',(38.2930403179255,-37.5314388517851,16.3542117235887));
#56492=CARTESIAN_POINT('Ctrl Pts',(38.7255164935028,-37.2823487342141,16.3283610827014));
#56493=CARTESIAN_POINT('Ctrl Pts',(39.8618384352913,-37.240015326582,16.276341938355));
#56494=CARTESIAN_POINT('Ctrl Pts',(40.8667697353107,-38.6282412326641,16.1981542905498));
#56495=CARTESIAN_POINT('Ctrl Pts',(40.2606815765474,-40.2387207543454,16.119648780173));
#56496=CARTESIAN_POINT('Ctrl Pts',(38.5830428006472,-40.6214939022528,16.0411432697963));
#56497=CARTESIAN_POINT('Ctrl Pts',(37.3383997450109,-39.4332806175246,15.9626377594195));
#56498=CARTESIAN_POINT('Ctrl Pts',(37.5801461044556,-38.0890698220828,15.900327244017));
#56499=CARTESIAN_POINT('Ctrl Pts',(38.1260519651446,-37.6315889023455,15.8641852320734));
#56500=CARTESIAN_POINT('Ctrl Pts',(38.2945098549624,-37.5355091383948,15.8542117235887));
#56501=CARTESIAN_POINT('Ctrl Pts',(38.295011126227,-37.5356544186406,16.3957882764113));
#56502=CARTESIAN_POINT('Ctrl Pts',(38.5448454369709,-37.3924216099234,16.3809869449701));
#56503=CARTESIAN_POINT('Ctrl Pts',(39.3436107151107,-37.1792592329343,16.3400171100699));
#56504=CARTESIAN_POINT('Ctrl Pts',(40.6150494715948,-37.9202307686755,16.2728787717108));
#56505=CARTESIAN_POINT('Ctrl Pts',(40.7123989731982,-39.6382265407265,16.1943732613341));
#56506=CARTESIAN_POINT('Ctrl Pts',(39.333086957597,-40.6670534245635,16.1158677509573));
#56507=CARTESIAN_POINT('Ctrl Pts',(37.7141132310224,-40.0840350136355,16.0373622405805));
#56508=CARTESIAN_POINT('Ctrl Pts',(37.3340693749042,-38.521628139946,15.9640024157318));
#56509=CARTESIAN_POINT('Ctrl Pts',(37.9443644518927,-37.7390576903556,15.9168110943421));
#56510=CARTESIAN_POINT('Ctrl Pts',(38.2951740301017,-37.5323575792927,15.8957882764113));
#56511=CARTESIAN_POINT('Origin',(39.0658530619283,-38.8697713466883,19.1042117235887));
#56512=CARTESIAN_POINT('',(38.2927752994979,-37.531894773765,16.8957882764113));
#56513=CARTESIAN_POINT('',(38.2960217454205,-37.5343651514648,16.8542117235887));
#56514=CARTESIAN_POINT('',(38.2943530619283,-37.5334941486488,19.1042117235887));
#56515=CARTESIAN_POINT('Ctrl Pts',(38.2960217454205,-37.5343651514648,16.8542117235887));
#56516=CARTESIAN_POINT('Ctrl Pts',(38.4526440402526,-37.4426474088561,16.8448739402472));
#56517=CARTESIAN_POINT('Ctrl Pts',(39.1056117500068,-37.1960483659351,16.8093676534467));
#56518=CARTESIAN_POINT('Ctrl Pts',(40.3881062726606,-37.623463173289,16.7476928631873));
#56519=CARTESIAN_POINT('Ctrl Pts',(40.834758606014,-39.2852359660895,16.6691873528105));
#56520=CARTESIAN_POINT('Ctrl Pts',(39.6950143769496,-40.5744102242793,16.5906818424337));
#56521=CARTESIAN_POINT('Ctrl Pts',(37.9910233315818,-40.3348238050803,16.5121763320569));
#56522=CARTESIAN_POINT('Ctrl Pts',(37.2509651368289,-38.7813435147692,16.4336708216802));
#56523=CARTESIAN_POINT('Ctrl Pts',(37.8462764933252,-37.7925906195587,16.3810159521908));
#56524=CARTESIAN_POINT('Ctrl Pts',(38.2877225391554,-37.5345016936567,16.3545295861603));
#56525=CARTESIAN_POINT('Ctrl Pts',(38.2930403179255,-37.5314388517851,16.3542117235887));
#56526=CARTESIAN_POINT('Ctrl Pts',(38.2927752994979,-37.531894773765,16.8957882764113));
#56527=CARTESIAN_POINT('Ctrl Pts',(38.7030067984342,-37.2976596080307,16.8713312990569));
#56528=CARTESIAN_POINT('Ctrl Pts',(39.7943393979825,-37.2242325343386,16.8207058182437));
#56529=CARTESIAN_POINT('Ctrl Pts',(40.8516003110939,-38.5339981005298,16.7439118339715));
#56530=CARTESIAN_POINT('Ctrl Pts',(40.3309240105073,-40.1740843304588,16.6654063235947));
#56531=CARTESIAN_POINT('Ctrl Pts',(38.6757020358417,-40.644431583443,16.586900813218));
#56532=CARTESIAN_POINT('Ctrl Pts',(37.3703767628973,-39.5232213878114,16.5083953028412));
#56533=CARTESIAN_POINT('Ctrl Pts',(37.5450179797371,-38.1378625018882,16.4446911239056));
#56534=CARTESIAN_POINT('Ctrl Pts',(38.1031426043017,-37.6456547913594,16.407155448429));
#56535=CARTESIAN_POINT('Ctrl Pts',(38.295011126227,-37.5356544186406,16.3957882764113));
#56536=CARTESIAN_POINT('Origin',(39.0658530619283,-38.8697713466883,19.1042117235887));
#56537=CARTESIAN_POINT('',(38.2959007276492,-37.5337106753506,17.3957882764113));
#56538=CARTESIAN_POINT('',(38.2935040424574,-37.5346322273253,17.3542117235887));
#56539=CARTESIAN_POINT('',(38.2943530619283,-37.5334941486488,19.1042117235887));
#56540=CARTESIAN_POINT('Ctrl Pts',(38.2935040424574,-37.5346322273253,17.3542117235887));
#56541=CARTESIAN_POINT('Ctrl Pts',(38.6142216923301,-37.353029943727,17.3352182943341));
#56542=CARTESIAN_POINT('Ctrl Pts',(39.5350880316606,-37.1858556050909,17.2900563616205));
#56543=CARTESIAN_POINT('Ctrl Pts',(40.7451827384013,-38.1758790339381,17.218725925448));
#56544=CARTESIAN_POINT('Ctrl Pts',(40.5709395934168,-39.8877854279213,17.1402204150712));
#56545=CARTESIAN_POINT('Ctrl Pts',(39.0468978715213,-40.6867135087542,17.0617149046944));
#56546=CARTESIAN_POINT('Ctrl Pts',(37.5398562037872,-39.856164211272,16.9832093943176));
#56547=CARTESIAN_POINT('Ctrl Pts',(37.4178373052428,-38.3450042264081,16.9140416672824));
#56548=CARTESIAN_POINT('Ctrl Pts',(38.0137206990119,-37.6996801517363,16.8710424437061));
#56549=CARTESIAN_POINT('Ctrl Pts',(38.2960217454205,-37.5343651514648,16.8542117235887));
#56550=CARTESIAN_POINT('Ctrl Pts',(38.2959007276492,-37.5337106753506,17.3957882764113));
#56551=CARTESIAN_POINT('Ctrl Pts',(38.4288872990661,-37.455546937363,17.3878441566028));
#56552=CARTESIAN_POINT('Ctrl Pts',(39.0471107626292,-37.2043843657909,17.3537315333353));
#56553=CARTESIAN_POINT('Ctrl Pts',(40.3208285827551,-37.5557507395872,17.293450406609));
#56554=CARTESIAN_POINT('Ctrl Pts',(40.8541369642562,-39.1917640019411,17.2149448962322));
#56555=CARTESIAN_POINT('Ctrl Pts',(39.7836658898431,-40.5390185509755,17.1364393858554));
#56556=CARTESIAN_POINT('Ctrl Pts',(38.0694451486085,-40.389246627264,17.0579338754786));
#56557=CARTESIAN_POINT('Ctrl Pts',(37.2488257543949,-38.87677605618,16.9794283651019));
#56558=CARTESIAN_POINT('Ctrl Pts',(37.8057511921981,-37.8311625054488,16.9253798320794));
#56559=CARTESIAN_POINT('Ctrl Pts',(38.2640668491777,-37.5482868076194,16.8974998025159));
#56560=CARTESIAN_POINT('Ctrl Pts',(38.2927752994979,-37.531894773765,16.8957882764113));
#56561=CARTESIAN_POINT('Origin',(39.0658530619283,-38.8697713466883,19.1042117235887));
#56562=CARTESIAN_POINT('',(38.2938718037176,-37.5356881270256,17.8957882764113));
#56563=CARTESIAN_POINT('',(38.2940537528419,-37.5314721085808,17.8542117235887));
#56564=CARTESIAN_POINT('',(38.2943530619283,-37.5334941486488,19.1042117235887));
#56565=CARTESIAN_POINT('',(37.5756558680257,-39.2699729499894,18.));
#56566=CARTESIAN_POINT('Ctrl Pts',(37.5756558680257,-39.2699729499894,18.));
#56567=CARTESIAN_POINT('Ctrl Pts',(37.4440523270134,-38.7799318659295,17.9738314965411));
#56568=CARTESIAN_POINT('Ctrl Pts',(37.6166680705089,-38.0418709533316,17.9390942553448));
#56569=CARTESIAN_POINT('Ctrl Pts',(38.1491376523636,-37.6179382396386,17.9043570141486));
#56570=CARTESIAN_POINT('Ctrl Pts',(38.2938718037176,-37.5356881270256,17.8957882764113));
#56571=CARTESIAN_POINT('',(37.9726405222314,-39.962294313691,18.));
#56572=CARTESIAN_POINT('Origin',(39.0658530619283,-38.8697713466883,18.));
#56573=CARTESIAN_POINT('Ctrl Pts',(37.972631799081,-39.9623061512025,18.));
#56574=CARTESIAN_POINT('Ctrl Pts',(37.6338216029695,-39.6208387086169,17.975091839613));
#56575=CARTESIAN_POINT('Ctrl Pts',(37.3042322663879,-38.6195093398435,17.9264957474759));
#56576=CARTESIAN_POINT('Ctrl Pts',(37.899143973177,-37.7627950030077,17.8778996553388));
#56577=CARTESIAN_POINT('Ctrl Pts',(38.2940537528419,-37.5314721085808,17.8542117235887));
#56578=CARTESIAN_POINT('Origin',(14.1292828945603,53.2669068454841,4.5));
#56579=CARTESIAN_POINT('',(14.7605875520818,54.3602657339262,5.80658032638059));
#56580=CARTESIAN_POINT('',(14.7625813317603,54.3604987677494,5.94341967361941));
#56581=CARTESIAN_POINT('',(14.7615328945603,54.3619959685696,4.5));
#56582=CARTESIAN_POINT('',(13.8936870225526,54.5092654229862,6.));
#56583=CARTESIAN_POINT('Ctrl Pts',(14.7625813317603,54.3604987677494,5.94341967361941));
#56584=CARTESIAN_POINT('Ctrl Pts',(14.5022241622972,54.5077988388625,5.96227978241294));
#56585=CARTESIAN_POINT('Ctrl Pts',(14.1881298777611,54.5651023789871,5.98113989120647));
#56586=CARTESIAN_POINT('Ctrl Pts',(13.8936870225526,54.5092654229862,6.));
#56587=CARTESIAN_POINT('',(14.7615328945603,54.3619959685696,6.));
#56588=CARTESIAN_POINT('Origin',(14.1292828945603,53.2669068454841,6.));
#56589=CARTESIAN_POINT('',(14.7615328945603,54.3619959685696,7.));
#56590=CARTESIAN_POINT('',(14.7615328945603,54.3619959685696,4.5));
#56591=CARTESIAN_POINT('',(12.8669333849943,53.3406222827979,7.));
#56592=CARTESIAN_POINT('Origin',(14.1292828945603,53.2669068454841,7.));
#56593=CARTESIAN_POINT('',(15.3916324041264,53.1931914081703,7.));
#56594=CARTESIAN_POINT('Origin',(14.1292828945603,53.2669068454841,7.));
#56595=CARTESIAN_POINT('Origin',(14.1292828945603,53.2669068454841,7.));
#56596=CARTESIAN_POINT('',(12.9337035820666,52.8487780612894,6.));
#56597=CARTESIAN_POINT('Origin',(14.1292828945603,53.2669068454841,6.));
#56598=CARTESIAN_POINT('Ctrl Pts',(12.9336933707122,52.8487726938778,6.));
#56599=CARTESIAN_POINT('Ctrl Pts',(12.8048848553781,53.2213517629532,5.97509183961299));
#56600=CARTESIAN_POINT('Ctrl Pts',(12.8625933288288,53.6603618768577,5.95018367922598));
#56601=CARTESIAN_POINT('Ctrl Pts',(13.0861255368911,53.9849952189361,5.92527551883898));
#56602=CARTESIAN_POINT('Ctrl Pts',(13.3209683863418,54.3260548798291,5.89910701538005));
#56603=CARTESIAN_POINT('Ctrl Pts',(13.7388407631054,54.540870088853,5.87293851192112));
#56604=CARTESIAN_POINT('Ctrl Pts',(14.1527369297938,54.5331774952646,5.8467700084622));
#56605=CARTESIAN_POINT('Ctrl Pts',(14.3646246721213,54.5292393909301,5.83337344776833));
#56606=CARTESIAN_POINT('Ctrl Pts',(14.5754703413608,54.4669871159197,5.81997688707446));
#56607=CARTESIAN_POINT('Ctrl Pts',(14.7605875520818,54.3602657339262,5.80658032638059));
#56608=CARTESIAN_POINT('Origin',(14.1292828945603,53.2669068454841,4.5));
#56609=CARTESIAN_POINT('',(14.7628720032994,54.3627600319775,5.30658032638059));
#56610=CARTESIAN_POINT('',(14.761790188637,54.3636903053853,5.44341967361941));
#56611=CARTESIAN_POINT('',(14.7615328945603,54.3619959685696,4.5));
#56612=CARTESIAN_POINT('Ctrl Pts',(14.761790188637,54.3636903053853,5.44341967361941));
#56613=CARTESIAN_POINT('Ctrl Pts',(14.7297149272464,54.3824695710557,5.44576692486712));
#56614=CARTESIAN_POINT('Ctrl Pts',(14.6967938380796,54.3997466843015,5.44811417611483));
#56615=CARTESIAN_POINT('Ctrl Pts',(14.6631180766711,54.4153998475156,5.45046142736254));
#56616=CARTESIAN_POINT('Ctrl Pts',(14.2876813696889,54.5899102907896,5.47662993082147));
#56617=CARTESIAN_POINT('Ctrl Pts',(13.8184459253802,54.5625788561695,5.50279843428039));
#56618=CARTESIAN_POINT('Ctrl Pts',(13.4657801062202,54.3456807478706,5.52896693773932));
#56619=CARTESIAN_POINT('Ctrl Pts',(13.1131142870602,54.1287826395717,5.55513544119824));
#56620=CARTESIAN_POINT('Ctrl Pts',(12.8770180930488,53.7223178575942,5.58130394465717));
#56621=CARTESIAN_POINT('Ctrl Pts',(12.8634449158406,53.308510984467,5.6074724481161));
#56622=CARTESIAN_POINT('Ctrl Pts',(12.8498717386324,52.8947041113399,5.63364095157503));
#56623=CARTESIAN_POINT('Ctrl Pts',(13.0588215782272,52.4735551470632,5.65980945503395));
#56624=CARTESIAN_POINT('Ctrl Pts',(13.3964281425195,52.2339907213231,5.68597795849288));
#56625=CARTESIAN_POINT('Ctrl Pts',(13.7340347068117,51.9944262955831,5.7121464619518));
#56626=CARTESIAN_POINT('Ctrl Pts',(14.2002979958013,51.9364464083796,5.73831496541073));
#56627=CARTESIAN_POINT('Ctrl Pts',(14.5864832378068,52.0858916506601,5.76448346886966));
#56628=CARTESIAN_POINT('Ctrl Pts',(14.9726684798122,52.2353368929405,5.79065197232859));
#56629=CARTESIAN_POINT('Ctrl Pts',(15.2787756748334,52.592207264705,5.81682047578751));
#56630=CARTESIAN_POINT('Ctrl Pts',(15.3668446182304,52.9968058417406,5.84298897924644));
#56631=CARTESIAN_POINT('Ctrl Pts',(15.4549135616273,53.4014044187763,5.86915748270536));
#56632=CARTESIAN_POINT('Ctrl Pts',(15.3249442534001,53.8537312010832,5.89532598616429));
#56633=CARTESIAN_POINT('Ctrl Pts',(15.0367728841186,54.1500649721194,5.92149448962322));
#56634=CARTESIAN_POINT('Ctrl Pts',(14.9562917782241,54.2328256907373,5.92880288428862));
#56635=CARTESIAN_POINT('Ctrl Pts',(14.8634711500129,54.3034191895921,5.93611127895402));
#56636=CARTESIAN_POINT('Ctrl Pts',(14.7625813317603,54.3604987677494,5.94341967361941));
#56637=CARTESIAN_POINT('Ctrl Pts',(14.7605875520818,54.3602657339262,5.80658032638059));
#56638=CARTESIAN_POINT('Ctrl Pts',(14.9370736274398,54.2585202625491,5.79380838361553));
#56639=CARTESIAN_POINT('Ctrl Pts',(15.0901745042163,54.1163557782414,5.78103644085048));
#56640=CARTESIAN_POINT('Ctrl Pts',(15.1984983273048,53.9457696468095,5.76826449808542));
#56641=CARTESIAN_POINT('Ctrl Pts',(15.4204436015143,53.5962547881435,5.74209599462649));
#56642=CARTESIAN_POINT('Ctrl Pts',(15.4544141933199,53.1274254670123,5.71592749116756));
#56643=CARTESIAN_POINT('Ctrl Pts',(15.2852697206798,52.7495259168145,5.68975898770864));
#56644=CARTESIAN_POINT('Ctrl Pts',(15.1161252480396,52.3716263666167,5.66359048424971));
#56645=CARTESIAN_POINT('Ctrl Pts',(14.7438657109537,52.0846565873524,5.63742198079079));
#56646=CARTESIAN_POINT('Ctrl Pts',(14.3353706309513,52.0172894645935,5.61125347733186));
#56647=CARTESIAN_POINT('Ctrl Pts',(13.9268755509488,51.9499223418345,5.58508497387293));
#56648=CARTESIAN_POINT('Ctrl Pts',(13.4821449280297,52.1021578755809,5.558916470414));
#56649=CARTESIAN_POINT('Ctrl Pts',(13.2006242325166,52.4057357189425,5.53274796695508));
#56650=CARTESIAN_POINT('Ctrl Pts',(12.9191035370036,52.7093135623041,5.50657946349615));
#56651=CARTESIAN_POINT('Ctrl Pts',(12.8007927688965,53.1642337152808,5.48041096003723));
#56652=CARTESIAN_POINT('Ctrl Pts',(12.8987324301598,53.5665026413488,5.4542424565783));
#56653=CARTESIAN_POINT('Ctrl Pts',(12.9966720914231,53.9687715674169,5.42807395311937));
#56654=CARTESIAN_POINT('Ctrl Pts',(13.3108621820568,54.3183892665762,5.40190544966045));
#56655=CARTESIAN_POINT('Ctrl Pts',(13.7004218404058,54.4585839700534,5.37573694620152));
#56656=CARTESIAN_POINT('Ctrl Pts',(14.0435904799155,54.5820834768109,5.35268473959454));
#56657=CARTESIAN_POINT('Ctrl Pts',(14.4452466462963,54.5430686762864,5.32963253298757));
#56658=CARTESIAN_POINT('Ctrl Pts',(14.7628720032994,54.3627600319775,5.30658032638059));
#56659=CARTESIAN_POINT('Origin',(14.1292828945603,53.2669068454841,4.5));
#56660=CARTESIAN_POINT('',(14.7604987163791,54.3623830037273,4.80658032638059));
#56661=CARTESIAN_POINT('',(14.7603543171395,54.3604895118786,4.94341967361941));
#56662=CARTESIAN_POINT('',(14.7615328945603,54.3619959685696,4.5));
#56663=CARTESIAN_POINT('Ctrl Pts',(14.7603543171395,54.3604895118786,4.94341967361941));
#56664=CARTESIAN_POINT('Ctrl Pts',(14.5947715388364,54.4565158591777,4.95542257078023));
#56665=CARTESIAN_POINT('Ctrl Pts',(14.4086766047111,54.5167140163305,4.96742546794105));
#56666=CARTESIAN_POINT('Ctrl Pts',(14.2192552064615,54.5302046425139,4.97942836510187));
#56667=CARTESIAN_POINT('Ctrl Pts',(13.8062820343284,54.5596166663956,5.00559686856079));
#56668=CARTESIAN_POINT('Ctrl Pts',(13.3774975305931,54.3670187022342,5.03176537201972));
#56669=CARTESIAN_POINT('Ctrl Pts',(13.1251731138615,54.0387742648884,5.05793387547865));
#56670=CARTESIAN_POINT('Ctrl Pts',(12.8728486971299,53.7105298275425,5.08410237893757));
#56671=CARTESIAN_POINT('Ctrl Pts',(12.796984367402,53.2466389170122,5.1102708823965));
#56672=CARTESIAN_POINT('Ctrl Pts',(12.9315998955733,52.8551151331566,5.13643938585542));
#56673=CARTESIAN_POINT('Ctrl Pts',(13.0662154237445,52.4635913493009,5.16260788931435));
#56674=CARTESIAN_POINT('Ctrl Pts',(13.411310809815,52.14443469212,5.18877639277328));
#56675=CARTESIAN_POINT('Ctrl Pts',(13.81213856493,52.0407600014986,5.2149448962322));
#56676=CARTESIAN_POINT('Ctrl Pts',(14.212966320045,51.9370853108772,5.24111339969113));
#56677=CARTESIAN_POINT('Ctrl Pts',(14.6695264442046,52.0488925868152,5.26728190315006));
#56678=CARTESIAN_POINT('Ctrl Pts',(14.9770971987178,52.3260437079763,5.29345040660898));
#56679=CARTESIAN_POINT('Ctrl Pts',(15.284667953231,52.6031948291373,5.31961891006791));
#56680=CARTESIAN_POINT('Ctrl Pts',(15.4432493380979,53.0456897955214,5.34578741352683));
#56681=CARTESIAN_POINT('Ctrl Pts',(15.3817210457035,53.4551134392974,5.37195591698576));
#56682=CARTESIAN_POINT('Ctrl Pts',(15.3257116918039,53.827812775923,5.39577716919698));
#56683=CARTESIAN_POINT('Ctrl Pts',(15.087308341869,54.1731075442457,5.4195984214082));
#56684=CARTESIAN_POINT('Ctrl Pts',(14.761790188637,54.3636903053853,5.44341967361941));
#56685=CARTESIAN_POINT('Ctrl Pts',(14.7628720032994,54.3627600319775,5.30658032638059));
#56686=CARTESIAN_POINT('Ctrl Pts',(14.8058099708876,54.3383851306841,5.30346402952864));
#56687=CARTESIAN_POINT('Ctrl Pts',(14.8472122922316,54.3114281126392,5.30034773267669));
#56688=CARTESIAN_POINT('Ctrl Pts',(14.8867268805692,54.2819414022849,5.29723143582474));
#56689=CARTESIAN_POINT('Ctrl Pts',(15.2185430363193,54.0343324232445,5.27106293236581));
#56690=CARTESIAN_POINT('Ctrl Pts',(15.4172461217553,53.6083427573686,5.24489442890689));
#56691=CARTESIAN_POINT('Ctrl Pts',(15.393736730538,53.1949914739395,5.21872592544796));
#56692=CARTESIAN_POINT('Ctrl Pts',(15.3702273393206,52.7816401905105,5.19255742198903));
#56693=CARTESIAN_POINT('Ctrl Pts',(15.12450547145,52.3809272895283,5.16638891853011));
#56694=CARTESIAN_POINT('Ctrl Pts',(14.7667550258397,52.1725370796236,5.14022041507118));
#56695=CARTESIAN_POINT('Ctrl Pts',(14.4090045802295,51.9641468697189,5.11405191161226));
#56696=CARTESIAN_POINT('Ctrl Pts',(13.9392255568796,51.9480793508917,5.08788340815333));
#56697=CARTESIAN_POINT('Ctrl Pts',(13.5680728067532,52.1315394490878,5.0617149046944));
#56698=CARTESIAN_POINT('Ctrl Pts',(13.1969200566268,52.3149995472839,5.03554640123547));
#56699=CARTESIAN_POINT('Ctrl Pts',(12.9243935797239,52.6979872625031,5.00937789777655));
#56700=CARTESIAN_POINT('Ctrl Pts',(12.8726973119175,53.1087663210662,4.98320939431762));
#56701=CARTESIAN_POINT('Ctrl Pts',(12.8210010441111,53.5195453796293,4.9570408908587));
#56702=CARTESIAN_POINT('Ctrl Pts',(12.9901349854012,53.9581157815362,4.93087238739977));
#56703=CARTESIAN_POINT('Ctrl Pts',(13.3042575537142,54.227817360156,4.90470388394084));
#56704=CARTESIAN_POINT('Ctrl Pts',(13.6183801220271,54.4975189387757,4.87853538048192));
#56705=CARTESIAN_POINT('Ctrl Pts',(14.0774913173628,54.5983516941084,4.85236687702299));
#56706=CARTESIAN_POINT('Ctrl Pts',(14.4757201786558,54.4851010127079,4.82619837356406));
#56707=CARTESIAN_POINT('Ctrl Pts',(14.5752351369457,54.4568003596631,4.81965902450291));
#56708=CARTESIAN_POINT('Ctrl Pts',(14.6709481788587,54.4151308478692,4.81311967544175));
#56709=CARTESIAN_POINT('Ctrl Pts',(14.7604987163791,54.3623830037273,4.80658032638059));
#56710=CARTESIAN_POINT('Origin',(14.1292828945603,53.2669068454841,4.5));
#56711=CARTESIAN_POINT('',(14.7614006096927,54.3603381104062,4.30658032638059));
#56712=CARTESIAN_POINT('',(14.7627659331487,54.3621523730593,4.44341967361941));
#56713=CARTESIAN_POINT('',(14.7615328945603,54.3619959685696,4.5));
#56714=CARTESIAN_POINT('Ctrl Pts',(14.7627659331487,54.3621523730593,4.44341967361941));
#56715=CARTESIAN_POINT('Ctrl Pts',(14.463761030489,54.5313718419492,4.46507821669334));
#56716=CARTESIAN_POINT('Ctrl Pts',(14.0916672421201,54.5784026588885,4.48673675976726));
#56717=CARTESIAN_POINT('Ctrl Pts',(13.7635961371407,54.4794617725194,4.50839530284119));
#56718=CARTESIAN_POINT('Ctrl Pts',(13.3672107562715,54.3599184164247,4.53456380630012));
#56719=CARTESIAN_POINT('Ctrl Pts',(13.0350905669399,54.0272826554628,4.56073230975904));
#56720=CARTESIAN_POINT('Ctrl Pts',(12.9161621999348,53.6307123234038,4.58690081321797));
#56721=CARTESIAN_POINT('Ctrl Pts',(12.7972338329298,53.2341419913447,4.61306931667689));
#56722=CARTESIAN_POINT('Ctrl Pts',(12.8914972882514,52.7736370881886,4.63923782013582));
#56723=CARTESIAN_POINT('Ctrl Pts',(13.1566837320242,52.4556934772733,4.66540632359475));
#56724=CARTESIAN_POINT('Ctrl Pts',(13.421870175797,52.1377498663579,4.69157482705367));
#56725=CARTESIAN_POINT('Ctrl Pts',(13.8579796080209,51.9623675476834,4.7177433305126));
#56726=CARTESIAN_POINT('Ctrl Pts',(14.2694553352381,52.0081900560918,4.74391183397153));
#56727=CARTESIAN_POINT('Ctrl Pts',(14.6809310624553,52.0540125645002,4.77008033743045));
#56728=CARTESIAN_POINT('Ctrl Pts',(15.0677730846659,52.3210398999916,4.79624884088938));
#56729=CARTESIAN_POINT('Ctrl Pts',(15.2565169212345,52.6895337942872,4.82241734434831));
#56730=CARTESIAN_POINT('Ctrl Pts',(15.4452607578031,53.0580276885828,4.84858584780723));
#56731=CARTESIAN_POINT('Ctrl Pts',(15.4359064087297,53.5279881416827,4.87475435126616));
#56732=CARTESIAN_POINT('Ctrl Pts',(15.2326483139276,53.888679374195,4.90092285472508));
#56733=CARTESIAN_POINT('Ctrl Pts',(15.1226200827607,54.0839297446631,4.91508846102319));
#56734=CARTESIAN_POINT('Ctrl Pts',(14.9557721746585,54.2471609203011,4.9292540673213));
#56735=CARTESIAN_POINT('Ctrl Pts',(14.7603543171395,54.3604895118786,4.94341967361941));
#56736=CARTESIAN_POINT('Ctrl Pts',(14.7604987163791,54.3623830037273,4.80658032638059));
#56737=CARTESIAN_POINT('Ctrl Pts',(15.0293024323073,54.2040498780404,4.78695117198282));
#56738=CARTESIAN_POINT('Ctrl Pts',(15.242580788107,53.945898828656,4.76732201758505));
#56739=CARTESIAN_POINT('Ctrl Pts',(15.3364895893995,53.649879171516,4.74769286318729));
#56740=CARTESIAN_POINT('Ctrl Pts',(15.4616836115997,53.2552421298582,4.72152435972836));
#56741=CARTESIAN_POINT('Ctrl Pts',(15.3747251287497,52.7933021646762,4.69535585626943));
#56742=CARTESIAN_POINT('Ctrl Pts',(15.1146073473565,52.471198645522,4.66918735281051));
#56743=CARTESIAN_POINT('Ctrl Pts',(14.8544895659633,52.1490951263678,4.64301884935158));
#56744=CARTESIAN_POINT('Ctrl Pts',(14.4212124860269,51.9668280532413,4.61685034589265));
#56745=CARTESIAN_POINT('Ctrl Pts',(14.0090627058929,52.0061281492218,4.59068184243372));
#56746=CARTESIAN_POINT('Ctrl Pts',(13.596912925759,52.0454282452023,4.5645133389748));
#56747=CARTESIAN_POINT('Ctrl Pts',(13.2058904454275,52.3062955102899,4.53834483551587));
#56748=CARTESIAN_POINT('Ctrl Pts',(13.0113343903925,52.6717539614819,4.51217633205695));
#56749=CARTESIAN_POINT('Ctrl Pts',(12.8167783353574,53.0372124126739,4.48600782859802));
#56750=CARTESIAN_POINT('Ctrl Pts',(12.8186887056188,53.5072620499704,4.45983932513909));
#56751=CARTESIAN_POINT('Ctrl Pts',(13.0162088697902,53.8711270288388,4.43367082168017));
#56752=CARTESIAN_POINT('Ctrl Pts',(13.2137290339615,54.2349920077072,4.40750231822124));
#56753=CARTESIAN_POINT('Ctrl Pts',(13.606858992043,54.4926723281474,4.38133381476231));
#56754=CARTESIAN_POINT('Ctrl Pts',(14.0193145970927,54.5286210713629,4.35516531130339));
#56755=CARTESIAN_POINT('Ctrl Pts',(14.2745724669733,54.5508687981624,4.33897031632912));
#56756=CARTESIAN_POINT('Ctrl Pts',(14.5372321463568,54.4881923359769,4.32277532135485));
#56757=CARTESIAN_POINT('Ctrl Pts',(14.7614006096927,54.3603381104062,4.30658032638059));
#56758=CARTESIAN_POINT('Origin',(14.1292828945603,53.2669068454841,4.5));
#56759=CARTESIAN_POINT('',(14.7626048989925,54.3636737206204,3.80658032638058));
#56760=CARTESIAN_POINT('',(14.7608564829457,54.3629211099724,3.94341967361941));
#56761=CARTESIAN_POINT('',(14.7615328945603,54.3619959685696,4.5));
#56762=CARTESIAN_POINT('Ctrl Pts',(14.7608564829457,54.3629211099724,3.94341967361941));
#56763=CARTESIAN_POINT('Ctrl Pts',(14.6904886508112,54.4043824600063,3.94856535914752));
#56764=CARTESIAN_POINT('Ctrl Pts',(14.6162453479771,54.4388759703619,3.95371104467562));
#56765=CARTESIAN_POINT('Ctrl Pts',(14.5392165090643,54.465226788063,3.95885673020373));
#56766=CARTESIAN_POINT('Ctrl Pts',(14.1474845568267,54.5992344844895,3.98502523366266));
#56767=CARTESIAN_POINT('Ctrl Pts',(13.6837115472212,54.5226514105579,4.01119373712158));
#56768=CARTESIAN_POINT('Ctrl Pts',(13.3558588106244,54.2698183268938,4.03736224058051));
#56769=CARTESIAN_POINT('Ctrl Pts',(13.0280060740275,54.0169852432297,4.06353074403944));
#56770=CARTESIAN_POINT('Ctrl Pts',(12.8360736104392,53.5879021498331,4.08969924749836));
#56771=CARTESIAN_POINT('Ctrl Pts',(12.8661262178428,53.1749750062962,4.11586775095729));
#56772=CARTESIAN_POINT('Ctrl Pts',(12.8961788252464,52.7620478627593,4.14203625441622));
#56773=CARTESIAN_POINT('Ctrl Pts',(13.1482165036419,52.3652766690821,4.16820475787515));
#56774=CARTESIAN_POINT('Ctrl Pts',(13.5092225624184,52.1625783447115,4.19437326133407));
#56775=CARTESIAN_POINT('Ctrl Pts',(13.8702286211949,51.959880020341,4.220541764793));
#56776=CARTESIAN_POINT('Ctrl Pts',(14.3402030603525,51.951254565277,4.24671026825192));
#56777=CARTESIAN_POINT('Ctrl Pts',(14.708403754256,52.1405697363842,4.27287877171085));
#56778=CARTESIAN_POINT('Ctrl Pts',(15.0766044481595,52.3298849074914,4.29904727516978));
#56779=CARTESIAN_POINT('Ctrl Pts',(15.343031396809,52.7171407047698,4.3252157786287));
#56780=CARTESIAN_POINT('Ctrl Pts',(15.3882155906945,53.1286870249125,4.35138428208763));
#56781=CARTESIAN_POINT('Ctrl Pts',(15.43339978458,53.5402333450552,4.37755278554656));
#56782=CARTESIAN_POINT('Ctrl Pts',(15.2573412237015,53.9760701880622,4.40372128900548));
#56783=CARTESIAN_POINT('Ctrl Pts',(14.938986657059,54.2407631339519,4.42988979246441));
#56784=CARTESIAN_POINT('Ctrl Pts',(14.8841204517295,54.2863811304883,4.43439975284941));
#56785=CARTESIAN_POINT('Ctrl Pts',(14.825027751098,54.3269157877332,4.43890971323441));
#56786=CARTESIAN_POINT('Ctrl Pts',(14.7627659331487,54.3621523730593,4.44341967361941));
#56787=CARTESIAN_POINT('Ctrl Pts',(14.7614006096927,54.3603381104062,4.30658032638059));
#56788=CARTESIAN_POINT('Ctrl Pts',(14.899452277793,54.2816005000793,4.29660681789593));
#56789=CARTESIAN_POINT('Ctrl Pts',(15.0229058598302,54.178143727902,4.28663330941127));
#56790=CARTESIAN_POINT('Ctrl Pts',(15.1210425075748,54.0545798005254,4.27665980092661));
#56791=CARTESIAN_POINT('Ctrl Pts',(15.3785335609892,53.7303726204816,4.25049129746768));
#56792=CARTESIAN_POINT('Ctrl Pts',(15.4617344158,53.2677410944033,4.22432279400875));
#56793=CARTESIAN_POINT('Ctrl Pts',(15.3333368195411,52.8741346977794,4.19815429054983));
#56794=CARTESIAN_POINT('Ctrl Pts',(15.2049392232822,52.4805283011554,4.1719857870909));
#56795=CARTESIAN_POINT('Ctrl Pts',(14.8649431759537,52.1559470339858,4.14581728363197));
#56796=CARTESIAN_POINT('Ctrl Pts',(14.4658069467496,52.0459369947103,4.11964878017305));
#56797=CARTESIAN_POINT('Ctrl Pts',(14.0666707175455,51.9359269554348,4.09348027671412));
#56798=CARTESIAN_POINT('Ctrl Pts',(13.6083943064658,52.0404881440534,4.06731177325519));
#56799=CARTESIAN_POINT('Ctrl Pts',(13.2964743036118,52.3127340807067,4.04114326979627));
#56800=CARTESIAN_POINT('Ctrl Pts',(12.9845543007579,52.5849800173601,4.01497476633734));
#56801=CARTESIAN_POINT('Ctrl Pts',(12.8189907061297,53.0249107020483,3.98880626287841));
#56802=CARTESIAN_POINT('Ctrl Pts',(12.8740242036727,53.4352559863353,3.96263775941949));
#56803=CARTESIAN_POINT('Ctrl Pts',(12.9290577012157,53.8456012706222,3.93646925596056));
#56804=CARTESIAN_POINT('Ctrl Pts',(13.2046882909297,54.2263611545079,3.91030075250164));
#56805=CARTESIAN_POINT('Ctrl Pts',(13.5773199398677,54.4067983801299,3.88413224904271));
#56806=CARTESIAN_POINT('Ctrl Pts',(13.9454253210212,54.5850438777981,3.85828160815533));
#56807=CARTESIAN_POINT('Ctrl Pts',(14.4081895758327,54.5678037039579,3.83243096726796));
#56808=CARTESIAN_POINT('Ctrl Pts',(14.7626048989925,54.3636737206204,3.80658032638058));
#56809=CARTESIAN_POINT('Origin',(14.1292828945603,53.2669068454841,4.5));
#56810=CARTESIAN_POINT('',(14.7601616123225,54.3612756103012,3.30658032638059));
#56811=CARTESIAN_POINT('',(14.7609899830458,54.3602193411782,3.44341967361941));
#56812=CARTESIAN_POINT('',(14.7615328945603,54.3619959685696,4.5));
#56813=CARTESIAN_POINT('Ctrl Pts',(14.7609899830458,54.3602193411782,3.44341967361941));
#56814=CARTESIAN_POINT('Ctrl Pts',(14.5562500775904,54.4775990222049,3.45822100506063));
#56815=CARTESIAN_POINT('Ctrl Pts',(14.3197636804793,54.5407089292625,3.47302233650184));
#56816=CARTESIAN_POINT('Ctrl Pts',(14.0857261531979,54.532655265383,3.48782366794306));
#56817=CARTESIAN_POINT('Ctrl Pts',(13.671951766312,54.5184165239613,3.51399217140198));
#56818=CARTESIAN_POINT('Ctrl Pts',(13.2658319689464,54.2817372437526,3.54016067486091));
#56819=CARTESIAN_POINT('Ctrl Pts',(13.0494757061861,53.9287472260938,3.56632917831983));
#56820=CARTESIAN_POINT('Ctrl Pts',(12.8331194434257,53.575757208435,3.59249768177876));
#56821=CARTESIAN_POINT('Ctrl Pts',(12.8065267152706,53.1064564533261,3.61866618523769));
#56822=CARTESIAN_POINT('Ctrl Pts',(12.9816220168908,52.7312849984863,3.64483468869661));
#56823=CARTESIAN_POINT('Ctrl Pts',(13.1567173185109,52.3561135436466,3.67100319215554));
#56824=CARTESIAN_POINT('Ctrl Pts',(13.5335006499062,52.0750713890761,3.69717169561447));
#56825=CARTESIAN_POINT('Ctrl Pts',(13.9430178866457,52.0141811772634,3.72334019907339));
#56826=CARTESIAN_POINT('Ctrl Pts',(14.3525351233851,51.9532909654507,3.74950870253232));
#56827=CARTESIAN_POINT('Ctrl Pts',(14.7947862654686,52.1125526963959,3.77567720599125));
#56828=CARTESIAN_POINT('Ctrl Pts',(15.0714606437586,52.4205515169895,3.80184570945017));
#56829=CARTESIAN_POINT('Ctrl Pts',(15.3481350220485,52.7285503375831,3.8280142129091));
#56830=CARTESIAN_POINT('Ctrl Pts',(15.4592326365448,53.185286247825,3.85418271636802));
#56831=CARTESIAN_POINT('Ctrl Pts',(15.3549359963582,53.5859534363384,3.88035121982695));
#56832=CARTESIAN_POINT('Ctrl Pts',(15.271147892813,53.907834791464,3.90137403775777));
#56833=CARTESIAN_POINT('Ctrl Pts',(15.0483458981207,54.1935297998804,3.92239685568859));
#56834=CARTESIAN_POINT('Ctrl Pts',(14.7608564829457,54.3629211099724,3.94341967361941));
#56835=CARTESIAN_POINT('Ctrl Pts',(14.7626048989925,54.3636737206204,3.80658032638058));
#56836=CARTESIAN_POINT('Ctrl Pts',(14.7669628321868,54.3611637139356,3.80626246380903));
#56837=CARTESIAN_POINT('Ctrl Pts',(14.7713043836124,54.3586254505289,3.80594460123748));
#56838=CARTESIAN_POINT('Ctrl Pts',(14.7756291758562,54.3560589463809,3.80562673866593));
#56839=CARTESIAN_POINT('Ctrl Pts',(15.131674054745,54.1447677196515,3.779458235207));
#56840=CARTESIAN_POINT('Ctrl Pts',(15.3741311043607,53.7420706988344,3.75328973174808));
#56841=CARTESIAN_POINT('Ctrl Pts',(15.3942797010543,53.3285420152435,3.72712122828915));
#56842=CARTESIAN_POINT('Ctrl Pts',(15.414428297748,52.9150133316526,3.70095272483022));
#56843=CARTESIAN_POINT('Ctrl Pts',(15.2122684415196,52.4906529852878,3.6747842213713));
#56844=CARTESIAN_POINT('Ctrl Pts',(14.8784510160553,52.2457491989657,3.64861571791237));
#56845=CARTESIAN_POINT('Ctrl Pts',(14.544633590591,52.0008454126437,3.62244721445344));
#56846=CARTESIAN_POINT('Ctrl Pts',(14.0791585958908,51.9353981863644,3.59627871099452));
#56847=CARTESIAN_POINT('Ctrl Pts',(13.6907505503598,52.0787548359323,3.57011020753559));
#56848=CARTESIAN_POINT('Ctrl Pts',(13.3023425048288,52.2221114855002,3.54394170407667));
#56849=CARTESIAN_POINT('Ctrl Pts',(12.9910014084669,52.5742720109151,3.51777320061774));
#56850=CARTESIAN_POINT('Ctrl Pts',(12.896336314222,52.9773234433404,3.49160469715881));
#56851=CARTESIAN_POINT('Ctrl Pts',(12.801671219977,53.3803748757656,3.46543619369988));
#56852=CARTESIAN_POINT('Ctrl Pts',(12.9236821278488,53.8343172152012,3.43926769024096));
#56853=CARTESIAN_POINT('Ctrl Pts',(13.2076578874333,54.1355973270763,3.41309918678203));
#56854=CARTESIAN_POINT('Ctrl Pts',(13.4916336470178,54.4368774389515,3.38693068332311));
#56855=CARTESIAN_POINT('Ctrl Pts',(13.9375742583148,54.5854953232664,3.36076217986418));
#56856=CARTESIAN_POINT('Ctrl Pts',(14.3455146684413,54.5148089413369,3.33459367640525));
#56857=CARTESIAN_POINT('Ctrl Pts',(14.4910812336828,54.4895857137002,3.32525589306369));
#56858=CARTESIAN_POINT('Ctrl Pts',(14.6318092436286,54.436438533397,3.31591810972214));
#56859=CARTESIAN_POINT('Ctrl Pts',(14.7601616123225,54.3612756103012,3.30658032638059));
#56860=CARTESIAN_POINT('Origin',(14.1292828945603,53.2669068454841,4.5));
#56861=CARTESIAN_POINT('',(14.7622249872189,54.3610567043162,2.80658032638059));
#56862=CARTESIAN_POINT('',(14.7628222445741,54.3633003878638,2.94341967361941));
#56863=CARTESIAN_POINT('',(14.7615328945603,54.3619959685696,4.5));
#56864=CARTESIAN_POINT('Ctrl Pts',(14.7628222445741,54.3633003878638,2.94341967361941));
#56865=CARTESIAN_POINT('Ctrl Pts',(14.4266363996141,54.5552567541312,2.96787665097373));
#56866=CARTESIAN_POINT('Ctrl Pts',(13.9945792873817,54.5843264233177,2.99233362832806));
#56867=CARTESIAN_POINT('Ctrl Pts',(13.6379437474727,54.4342123040851,3.01679060568238));
#56868=CARTESIAN_POINT('Ctrl Pts',(13.256350461251,54.2735930341132,3.04295910914131));
#56869=CARTESIAN_POINT('Ctrl Pts',(12.9611042822246,53.9078334931332,3.06912761260023));
#56870=CARTESIAN_POINT('Ctrl Pts',(12.8845971374177,53.5009445240528,3.09529611605916));
#56871=CARTESIAN_POINT('Ctrl Pts',(12.8080899926107,53.0940555549725,3.12146461951808));
#56872=CARTESIAN_POINT('Ctrl Pts',(12.9503218820233,52.6460371577917,3.14763312297701));
#56873=CARTESIAN_POINT('Ctrl Pts',(13.2475143204016,52.3577861486808,3.17380162643594));
#56874=CARTESIAN_POINT('Ctrl Pts',(13.54470675878,52.0695351395699,3.19997012989486));
#56875=CARTESIAN_POINT('Ctrl Pts',(13.9968597461241,51.9410515185289,3.22613863335379));
#56876=CARTESIAN_POINT('Ctrl Pts',(14.4012225159017,52.0299488478797,3.25230713681272));
#56877=CARTESIAN_POINT('Ctrl Pts',(14.8055852856792,52.1188461772305,3.27847564027164));
#56878=CARTESIAN_POINT('Ctrl Pts',(15.1621578378903,52.4251244569731,3.30464414373057));
#56879=CARTESIAN_POINT('Ctrl Pts',(15.3110487977949,52.8114448760708,3.3308126471895));
#56880=CARTESIAN_POINT('Ctrl Pts',(15.4599397576996,53.1977652951685,3.35698115064842));
#56881=CARTESIAN_POINT('Ctrl Pts',(15.4011491252979,53.6641278536213,3.38314965410735));
#56882=CARTESIAN_POINT('Ctrl Pts',(15.1610393208939,54.0014100315303,3.40931815756628));
#56883=CARTESIAN_POINT('Ctrl Pts',(15.0567395295787,54.1479199204438,3.42068532958399));
#56884=CARTESIAN_POINT('Ctrl Pts',(14.918226764983,54.2700737329326,3.4320525016017));
#56885=CARTESIAN_POINT('Ctrl Pts',(14.7609899830458,54.3602193411782,3.44341967361941));
#56886=CARTESIAN_POINT('Ctrl Pts',(14.7601616123225,54.3612756103012,3.30658032638059));
#56887=CARTESIAN_POINT('Ctrl Pts',(14.9915080373649,54.2257995475618,3.28974960626321));
#56888=CARTESIAN_POINT('Ctrl Pts',(15.1826489574086,54.0187995905144,3.27291888614585));
#56889=CARTESIAN_POINT('Ctrl Pts',(15.2894496720194,53.7748722761244,3.25608816602848));
#56890=CARTESIAN_POINT('Ctrl Pts',(15.455504056515,53.395612641015,3.22991966256955));
#56891=CARTESIAN_POINT('Ctrl Pts',(15.4176726165505,52.9270840189701,3.20375115911062));
#56892=CARTESIAN_POINT('Ctrl Pts',(15.1929194920754,52.5793801620778,3.17758265565169));
#56893=CARTESIAN_POINT('Ctrl Pts',(14.9681663676002,52.2316763051856,3.15141415219277));
#56894=CARTESIAN_POINT('Ctrl Pts',(14.5564915586145,52.004797213446,3.12524564873384));
#56895=CARTESIAN_POINT('Ctrl Pts',(14.1424947973993,52.00047827147,3.09907714527492));
#56896=CARTESIAN_POINT('Ctrl Pts',(13.7284980361841,51.9961593294939,3.07290864181599));
#56897=CARTESIAN_POINT('Ctrl Pts',(13.3121793227393,52.2144005372813,3.04674013835706));
#56898=CARTESIAN_POINT('Ctrl Pts',(13.0802212088747,52.5573397364563,3.02057163489813));
#56899=CARTESIAN_POINT('Ctrl Pts',(12.8482630950101,52.9002789356314,2.99440313143921));
#56900=CARTESIAN_POINT('Ctrl Pts',(12.8006655807257,53.3679161261941,2.96823462798028));
#56901=CARTESIAN_POINT('Ctrl Pts',(12.9587713715113,53.7505576476053,2.94206612452136));
#56902=CARTESIAN_POINT('Ctrl Pts',(13.116877162297,54.1331991690165,2.91589762106243));
#56903=CARTESIAN_POINT('Ctrl Pts',(13.4806862581528,54.4308450212763,2.8897291176035));
#56904=CARTESIAN_POINT('Ctrl Pts',(13.8870635107844,54.5100264348898,2.86356061414458));
#56905=CARTESIAN_POINT('Ctrl Pts',(14.1820172367656,54.5674973017321,2.84456718488991));
#56906=CARTESIAN_POINT('Ctrl Pts',(14.499396034384,54.5098802470415,2.82557375563525));
#56907=CARTESIAN_POINT('Ctrl Pts',(14.7622249872189,54.3610567043162,2.80658032638059));
#56908=CARTESIAN_POINT('Origin',(14.1292828945603,53.2669068454841,4.5));
#56909=CARTESIAN_POINT('',(14.7617771735939,54.3636459375188,2.30658032638059));
#56910=CARTESIAN_POINT('',(14.7602610286104,54.3618122024717,2.44341967361941));
#56911=CARTESIAN_POINT('',(14.7615328945603,54.3619959685696,4.5));
#56912=CARTESIAN_POINT('',(12.9355708698302,52.8497595669186,2.));
#56913=CARTESIAN_POINT('Ctrl Pts',(14.7617771735939,54.3636459375188,2.30658032638059));
#56914=CARTESIAN_POINT('Ctrl Pts',(15.0854028058299,54.1740757700734,2.2828923946305));
#56915=CARTESIAN_POINT('Ctrl Pts',(15.3230378955527,53.8318500257242,2.25920446288042));
#56916=CARTESIAN_POINT('Ctrl Pts',(15.3806718879601,53.4614673043247,2.23551653113034));
#56917=CARTESIAN_POINT('Ctrl Pts',(15.4443412427006,53.0522985500271,2.20934802767141));
#56918=CARTESIAN_POINT('Ctrl Pts',(15.2883366067183,52.6087669190161,2.18317952421249));
#56919=CARTESIAN_POINT('Ctrl Pts',(14.981978171922,52.3301976113127,2.15701102075356));
#56920=CARTESIAN_POINT('Ctrl Pts',(14.6756197371256,52.0516283036092,2.13084251729463));
#56921=CARTESIAN_POINT('Ctrl Pts',(14.2189075035153,51.9380213192133,2.10467401383571));
#56922=CARTESIAN_POINT('Ctrl Pts',(13.8181892890955,52.0394181405146,2.07850551037678));
#56923=CARTESIAN_POINT('Ctrl Pts',(13.4174710746757,52.140814961816,2.05233700691785));
#56924=CARTESIAN_POINT('Ctrl Pts',(13.0727468794464,52.4572155888145,2.02616850345893));
#56925=CARTESIAN_POINT('Ctrl Pts',(12.9355708698302,52.8497595669186,2.));
#56926=CARTESIAN_POINT('',(13.8936035762985,54.5113733504501,2.));
#56927=CARTESIAN_POINT('Origin',(14.1292828945603,53.2669068454841,2.));
#56928=CARTESIAN_POINT('Ctrl Pts',(13.8936031194075,54.5113848919291,2.));
#56929=CARTESIAN_POINT('Ctrl Pts',(13.5065360962338,54.4366467486623,2.02490816038701));
#56930=CARTESIAN_POINT('Ctrl Pts',(13.1551959025419,54.1671648587472,2.04981632077402));
#56931=CARTESIAN_POINT('Ctrl Pts',(12.9858211468817,53.8112635997049,2.07472448116103));
#56932=CARTESIAN_POINT('Ctrl Pts',(12.8078760955218,53.4373538776067,2.10089298461995));
#56933=CARTESIAN_POINT('Ctrl Pts',(12.830777130449,52.9680579532916,2.12706148807888));
#56934=CARTESIAN_POINT('Ctrl Pts',(13.0443872879449,52.6134595791442,2.15322999153781));
#56935=CARTESIAN_POINT('Ctrl Pts',(13.2579974454408,52.2588612049968,2.17939849499673));
#56936=CARTESIAN_POINT('Ctrl Pts',(13.6623167255053,52.0189603810172,2.20556699845566));
#56937=CARTESIAN_POINT('Ctrl Pts',(14.0759781319804,52.0015075823912,2.23173550191458));
#56938=CARTESIAN_POINT('Ctrl Pts',(14.4896395384554,51.9840547837652,2.25790400537351));
#56939=CARTESIAN_POINT('Ctrl Pts',(14.9126430713409,52.1890500104929,2.28407250883244));
#56940=CARTESIAN_POINT('Ctrl Pts',(15.1553414968488,52.5244832283522,2.31024101229136));
#56941=CARTESIAN_POINT('Ctrl Pts',(15.3980399223566,52.8599164462115,2.33640951575029));
#56942=CARTESIAN_POINT('Ctrl Pts',(15.4604332404868,53.3257876552024,2.36257801920922));
#56943=CARTESIAN_POINT('Ctrl Pts',(15.3145273105893,53.7132383944998,2.38874652266814));
#56944=CARTESIAN_POINT('Ctrl Pts',(15.2129148646388,53.9830685332266,2.40697090631857));
#56945=CARTESIAN_POINT('Ctrl Pts',(15.010275844201,54.2148642023246,2.42519528996899));
#56946=CARTESIAN_POINT('Ctrl Pts',(14.7602610286104,54.3618122024717,2.44341967361941));
#56947=CARTESIAN_POINT('Origin',(14.1292828945603,53.2669068454841,0.895788276411274));
#56948=CARTESIAN_POINT('',(14.9010968564111,54.6052515498159,5.60421172358873));
#56949=CARTESIAN_POINT('',(14.89962934498,54.6010727330809,5.64578827641128));
#56950=CARTESIAN_POINT('',(14.9007828945603,54.6031840435236,0.895788276411274));
#56951=CARTESIAN_POINT('',(15.2209662466057,52.1764590205668,6.));
#56952=CARTESIAN_POINT('Ctrl Pts',(14.89962934498,54.6010727330809,5.64578827641128));
#56953=CARTESIAN_POINT('Ctrl Pts',(14.6737409652706,54.7312989825202,5.65918483710515));
#56954=CARTESIAN_POINT('Ctrl Pts',(13.9138866474417,54.955646298412,5.69874990125794));
#56955=CARTESIAN_POINT('Ctrl Pts',(12.6330342875793,54.2971998857928,5.76448346886966));
#56956=CARTESIAN_POINT('Ctrl Pts',(12.4433594214855,52.5865231455987,5.84298897924644));
#56957=CARTESIAN_POINT('Ctrl Pts',(13.7694165995699,51.486617996264,5.92149448962322));
#56958=CARTESIAN_POINT('Ctrl Pts',(14.8623799894179,51.8174664687921,5.97383149654107));
#56959=CARTESIAN_POINT('Ctrl Pts',(15.2209662466057,52.1764590205668,6.));
#56960=CARTESIAN_POINT('',(15.6220374293776,52.8664110852719,6.));
#56961=CARTESIAN_POINT('Origin',(14.1292828945603,53.2669068454841,6.));
#56962=CARTESIAN_POINT('Ctrl Pts',(14.9010968564111,54.6052515498159,5.60421172358873));
#56963=CARTESIAN_POINT('Ctrl Pts',(14.8619571740658,54.628166857787,5.60655897483644));
#56964=CARTESIAN_POINT('Ctrl Pts',(14.3739271072306,54.8842868995419,5.63507472954308));
#56965=CARTESIAN_POINT('Ctrl Pts',(13.1774033105245,54.8145932898247,5.68975898770864));
#56966=CARTESIAN_POINT('Ctrl Pts',(12.3131175991141,53.326633245717,5.76826449808541));
#56967=CARTESIAN_POINT('Ctrl Pts',(13.0780276880699,51.7849182946399,5.8467700084622));
#56968=CARTESIAN_POINT('Ctrl Pts',(14.7574918726583,51.5760767532103,5.92401517576705));
#56969=CARTESIAN_POINT('Ctrl Pts',(15.4957392820493,52.402248403584,5.97509183961299));
#56970=CARTESIAN_POINT('Ctrl Pts',(15.6220514315181,52.8664094746825,6.));
#56971=CARTESIAN_POINT('Origin',(14.1292828945603,53.2669068454841,0.895788276411274));
#56972=CARTESIAN_POINT('',(14.8993447411713,54.6013457970434,5.10421172358873));
#56973=CARTESIAN_POINT('',(14.9024169355128,54.6041163881961,5.14578827641128));
#56974=CARTESIAN_POINT('',(14.9007828945603,54.6031840435236,0.895788276411274));
#56975=CARTESIAN_POINT('Ctrl Pts',(14.9024169355127,54.6041163881961,5.14578827641128));
#56976=CARTESIAN_POINT('Ctrl Pts',(14.5148361321472,54.8241371380329,5.16884048301826));
#56977=CARTESIAN_POINT('Ctrl Pts',(13.4683417470894,54.9257881846255,5.21806119308415));
#56978=CARTESIAN_POINT('Ctrl Pts',(12.3638311119676,53.696734568805,5.29345040660898));
#56979=CARTESIAN_POINT('Ctrl Pts',(12.7969355370903,52.0313922294383,5.37195591698577));
#56980=CARTESIAN_POINT('Ctrl Pts',(14.424976702367,51.4740982114769,5.45046142736254));
#56981=CARTESIAN_POINT('Ctrl Pts',(15.7877203932888,52.5246186608361,5.52896693773932));
#56982=CARTESIAN_POINT('Ctrl Pts',(15.6845839838159,53.9480078415062,5.59407588742224));
#56983=CARTESIAN_POINT('Ctrl Pts',(15.1149856235702,54.4769183144689,5.63301633364622));
#56984=CARTESIAN_POINT('Ctrl Pts',(14.89962934498,54.6010727330809,5.64578827641128));
#56985=CARTESIAN_POINT('Ctrl Pts',(14.8993447411713,54.6013457970434,5.10421172358873));
#56986=CARTESIAN_POINT('Ctrl Pts',(14.6972931579988,54.7185214822016,5.11621462074955));
#56987=CARTESIAN_POINT('Ctrl Pts',(13.9751327847045,54.9521265711601,5.15438602136929));
#56988=CARTESIAN_POINT('Ctrl Pts',(12.6886982319545,54.374296277089,5.21872592544795));
#56989=CARTESIAN_POINT('Ctrl Pts',(12.4109789893207,52.6761143673659,5.29723143582474));
#56990=CARTESIAN_POINT('Ctrl Pts',(13.6742819091468,51.5077662723951,5.37573694620152));
#56991=CARTESIAN_POINT('Ctrl Pts',(15.3456277491901,51.9170631330653,5.4542424565783));
#56992=CARTESIAN_POINT('Ctrl Pts',(15.9087950365255,53.4884877368246,5.53040071570737));
#56993=CARTESIAN_POINT('Ctrl Pts',(15.2983088061438,54.3726938586823,5.58039047137751));
#56994=CARTESIAN_POINT('Ctrl Pts',(14.9010968564111,54.6052515498159,5.60421172358873));
#56995=CARTESIAN_POINT('Origin',(14.1292828945603,53.2669068454841,0.895788276411274));
#56996=CARTESIAN_POINT('',(14.9022875039252,54.6033748953446,4.60421172358873));
#56997=CARTESIAN_POINT('',(14.899520943644,54.6036563213,4.64578827641127));
#56998=CARTESIAN_POINT('',(14.9007828945603,54.6031840435236,0.895788276411274));
#56999=CARTESIAN_POINT('Ctrl Pts',(14.899520943644,54.6036563213,4.64578827641127));
#57000=CARTESIAN_POINT('Ctrl Pts',(14.7902473340007,54.6680216226135,4.65232762547243));
#57001=CARTESIAN_POINT('Ctrl Pts',(14.20608207924,54.9223430869235,4.68503547799252));
#57002=CARTESIAN_POINT('Ctrl Pts',(12.9456280488333,54.6455146101901,4.74391183397153));
#57003=CARTESIAN_POINT('Ctrl Pts',(12.3264734310144,53.0400243844668,4.8224173443483));
#57004=CARTESIAN_POINT('Ctrl Pts',(13.3241207711359,51.6380076713391,4.90092285472509));
#57005=CARTESIAN_POINT('Ctrl Pts',(15.0438575043004,51.6968266074015,4.97942836510187));
#57006=CARTESIAN_POINT('Ctrl Pts',(15.9433802614164,53.1637305367386,5.05793387547864));
#57007=CARTESIAN_POINT('Ctrl Pts',(15.4295729948612,54.265256390372,5.11338717924845));
#57008=CARTESIAN_POINT('Ctrl Pts',(14.9548117824789,54.5743730329603,5.14267197955933));
#57009=CARTESIAN_POINT('Ctrl Pts',(14.9024169355127,54.6041163881961,5.14578827641128));
#57010=CARTESIAN_POINT('Ctrl Pts',(14.9022875039252,54.6033748953446,4.60421172358873));
#57011=CARTESIAN_POINT('Ctrl Pts',(14.5374282197781,54.8098641325902,4.62587026666265));
#57012=CARTESIAN_POINT('Ctrl Pts',(13.5347909686423,54.9365925287331,4.6736973131955));
#57013=CARTESIAN_POINT('Ctrl Pts',(12.3888319545388,53.7888545684046,4.74769286318728));
#57014=CARTESIAN_POINT('Ctrl Pts',(12.7339055288242,52.1030679359729,4.82619837356406));
#57015=CARTESIAN_POINT('Ctrl Pts',(14.3303867955418,51.461039661442,4.90470388394084));
#57016=CARTESIAN_POINT('Ctrl Pts',(15.7465131069793,52.4385560995514,4.98320939431762));
#57017=CARTESIAN_POINT('Ctrl Pts',(15.7175049264688,53.8959207488069,5.04971200753358));
#57018=CARTESIAN_POINT('Ctrl Pts',(15.1378024352416,54.4630571321133,5.09004611729062));
#57019=CARTESIAN_POINT('Ctrl Pts',(14.8993447411713,54.6013457970434,5.10421172358873));
#57020=CARTESIAN_POINT('Origin',(14.1292828945603,53.2669068454841,0.895788276411274));
#57021=CARTESIAN_POINT('',(14.899957506564,54.6043129428392,4.10421172358873));
#57022=CARTESIAN_POINT('',(14.9006214745914,54.60116105013,4.14578827641127));
#57023=CARTESIAN_POINT('',(14.9007828945603,54.6031840435236,0.895788276411274));
#57024=CARTESIAN_POINT('Ctrl Pts',(14.9006214745914,54.60116105013,4.14578827641127));
#57025=CARTESIAN_POINT('Ctrl Pts',(14.6270809930356,54.7571745495808,4.16198327138554));
#57026=CARTESIAN_POINT('Ctrl Pts',(13.7886805442009,54.9572356101558,4.20434676981873));
#57027=CARTESIAN_POINT('Ctrl Pts',(12.5323678038339,54.1337749126023,4.27287877171085));
#57028=CARTESIAN_POINT('Ctrl Pts',(12.5253744436601,52.413047533365,4.35138428208763));
#57029=CARTESIAN_POINT('Ctrl Pts',(13.9568043064156,51.4580814834716,4.42988979246441));
#57030=CARTESIAN_POINT('Ctrl Pts',(15.5429170806551,52.1253130228171,4.50839530284119));
#57031=CARTESIAN_POINT('Ctrl Pts',(15.8347326759058,53.6754928499224,4.58036146415681));
#57032=CARTESIAN_POINT('Ctrl Pts',(15.2275273759708,54.4104510916165,4.62615912201351));
#57033=CARTESIAN_POINT('Ctrl Pts',(14.899520943644,54.6036563213,4.64578827641127));
#57034=CARTESIAN_POINT('Ctrl Pts',(14.899957506564,54.6043129428392,4.10421172358873));
#57035=CARTESIAN_POINT('Ctrl Pts',(14.8140915002504,54.654905954387,4.10935740911683));
#57036=CARTESIAN_POINT('Ctrl Pts',(14.2627733336105,54.9110489082196,4.14067159810387));
#57037=CARTESIAN_POINT('Ctrl Pts',(13.0196598476916,54.705772943414,4.19815429054983));
#57038=CARTESIAN_POINT('Ctrl Pts',(12.317045870665,53.1350132444558,4.2766598009266));
#57039=CARTESIAN_POINT('Ctrl Pts',(13.239689139382,51.6825388628568,4.35516531130338));
#57040=CARTESIAN_POINT('Ctrl Pts',(14.9601412381249,51.6509633535716,4.43367082168016));
#57041=CARTESIAN_POINT('Ctrl Pts',(15.9354598188275,53.0686043860759,4.51217633205695));
#57042=CARTESIAN_POINT('Ctrl Pts',(15.4687653497055,54.223916817667,4.5690232993598));
#57043=CARTESIAN_POINT('Ctrl Pts',(14.9782621856933,54.5603776227797,4.59970176320372));
#57044=CARTESIAN_POINT('Ctrl Pts',(14.9022875039252,54.6033748953446,4.60421172358873));
#57045=CARTESIAN_POINT('Origin',(14.1292828945603,53.2669068454841,0.895788276411274));
#57046=CARTESIAN_POINT('',(14.9001204094145,54.6010161225549,3.60421172358873));
#57047=CARTESIAN_POINT('',(14.9020910027761,54.6052313123369,3.64578827641127));
#57048=CARTESIAN_POINT('',(14.9007828945603,54.6031840435236,0.895788276411274));
#57049=CARTESIAN_POINT('Ctrl Pts',(14.9020910027761,54.6052313123369,3.64578827641127));
#57050=CARTESIAN_POINT('Ctrl Pts',(14.4696174214114,54.8543199357372,3.67163891729864));
#57051=CARTESIAN_POINT('Ctrl Pts',(13.3333022960118,54.8966530893797,3.72365806164495));
#57052=CARTESIAN_POINT('Ctrl Pts',(12.3283770240505,53.5084355106896,3.80184570945017));
#57053=CARTESIAN_POINT('Ctrl Pts',(12.9344615472089,51.8979656495417,3.88035121982696));
#57054=CARTESIAN_POINT('Ctrl Pts',(14.6120902596549,51.5151947977303,3.95885673020373));
#57055=CARTESIAN_POINT('Ctrl Pts',(15.8567258492822,52.7034009548899,4.03736224058051));
#57056=CARTESIAN_POINT('Ctrl Pts',(15.614980939896,54.0476036870055,4.09967275598302));
#57057=CARTESIAN_POINT('Ctrl Pts',(15.0690783538945,54.5050818625188,4.13581476792661));
#57058=CARTESIAN_POINT('Ctrl Pts',(14.9006214745914,54.60116105013,4.14578827641127));
#57059=CARTESIAN_POINT('Ctrl Pts',(14.9001204094145,54.6010161225549,3.60421172358873));
#57060=CARTESIAN_POINT('Ctrl Pts',(14.6502875315041,54.7442481097626,3.61901305502994));
#57061=CARTESIAN_POINT('Ctrl Pts',(13.8515268344552,54.9574092639254,3.65998288993008));
#57062=CARTESIAN_POINT('Ctrl Pts',(12.5800953694062,54.216441978079,3.72712122828915));
#57063=CARTESIAN_POINT('Ctrl Pts',(12.482746426243,52.4984560584277,3.80562673866593));
#57064=CARTESIAN_POINT('Ctrl Pts',(13.8620505314459,51.4696350750293,3.88413224904271));
#57065=CARTESIAN_POINT('Ctrl Pts',(15.4810149732843,52.0526501422855,3.96263775941949));
#57066=CARTESIAN_POINT('Ctrl Pts',(15.8610566498332,53.6150480556463,4.03599758426816));
#57067=CARTESIAN_POINT('Ctrl Pts',(15.2507650728867,54.3976140171991,4.08318890565791));
#57068=CARTESIAN_POINT('Ctrl Pts',(14.899957506564,54.6043129428392,4.10421172358873));
#57069=CARTESIAN_POINT('Origin',(14.1292828945603,53.2669068454841,0.895788276411274));
#57070=CARTESIAN_POINT('',(14.9023562176693,54.604775754849,3.10421172358873));
#57071=CARTESIAN_POINT('',(14.8991095940519,54.6023050298359,3.14578827641127));
#57072=CARTESIAN_POINT('',(14.9007828945603,54.6031840435236,0.895788276411274));
#57073=CARTESIAN_POINT('Ctrl Pts',(14.8991095940519,54.6023050298359,3.14578827641127));
#57074=CARTESIAN_POINT('Ctrl Pts',(14.7424882378679,54.6940222226684,3.15512605975283));
#57075=CARTESIAN_POINT('Ctrl Pts',(14.0895244416362,54.9406197878808,3.19063234655331));
#57076=CARTESIAN_POINT('Ctrl Pts',(12.8070376180166,54.5132075415872,3.25230713681272));
#57077=CARTESIAN_POINT('Ctrl Pts',(12.3603879600183,52.8514447189324,3.3308126471895));
#57078=CARTESIAN_POINT('Ctrl Pts',(13.5001253542918,51.5622781929174,3.40931815756628));
#57079=CARTESIAN_POINT('Ctrl Pts',(15.2041061771209,51.8018631754771,3.48782366794306));
#57080=CARTESIAN_POINT('Ctrl Pts',(15.944159933136,53.3553341468671,3.56632917831984));
#57081=CARTESIAN_POINT('Ctrl Pts',(15.3488521474601,54.3440811110856,3.61898404780924));
#57082=CARTESIAN_POINT('Ctrl Pts',(14.9074087496474,54.6021684888377,3.64547041383972));
#57083=CARTESIAN_POINT('Ctrl Pts',(14.9020910027761,54.6052313123369,3.64578827641127));
#57084=CARTESIAN_POINT('Ctrl Pts',(14.9023562176693,54.604775754849,3.10421172358873));
#57085=CARTESIAN_POINT('Ctrl Pts',(14.4921270687778,54.8390095809862,3.12866870094305));
#57086=CARTESIAN_POINT('Ctrl Pts',(13.4008007460488,54.9124362051017,3.1792941817563));
#57087=CARTESIAN_POINT('Ctrl Pts',(12.3435458814549,53.6026781745395,3.25608816602847));
#57088=CARTESIAN_POINT('Ctrl Pts',(12.8642192037884,51.9626013374103,3.33459367640525));
#57089=CARTESIAN_POINT('Ctrl Pts',(14.5194316817765,51.4922567887357,3.41309918678203));
#57090=CARTESIAN_POINT('Ctrl Pts',(15.824749470772,52.6134605506407,3.49160469715881));
#57091=CARTESIAN_POINT('Ctrl Pts',(15.6501092546376,53.9988114930956,3.55530887609437));
#57092=CARTESIAN_POINT('Ctrl Pts',(15.091987830948,54.4910163807415,3.59284455157101));
#57093=CARTESIAN_POINT('Ctrl Pts',(14.9001204094145,54.6010161225549,3.60421172358873));
#57094=CARTESIAN_POINT('Origin',(14.1292828945603,53.2669068454841,0.895788276411274));
#57095=CARTESIAN_POINT('',(14.8992309062956,54.6029598038327,2.60421172358873));
#57096=CARTESIAN_POINT('',(14.9016274172746,54.6020379108679,2.64578827641127));
#57097=CARTESIAN_POINT('',(14.9007828945603,54.6031840435236,0.895788276411274));
#57098=CARTESIAN_POINT('Ctrl Pts',(14.9016274172746,54.6020379108679,2.64578827641127));
#57099=CARTESIAN_POINT('Ctrl Pts',(14.5809116606718,54.7836391180053,2.66478170566594));
#57100=CARTESIAN_POINT('Ctrl Pts',(13.6600505366298,54.9508125591569,2.70994363837953));
#57101=CARTESIAN_POINT('Ctrl Pts',(12.4499634166736,53.9607949476381,2.78127407455204));
#57102=CARTESIAN_POINT('Ctrl Pts',(12.6242053254301,52.2488988977253,2.85977958492882));
#57103=CARTESIAN_POINT('Ctrl Pts',(14.1482380059646,51.4499755676755,2.9382850953056));
#57104=CARTESIAN_POINT('Ctrl Pts',(15.6552705807332,52.2805199058823,3.01679060568238));
#57105=CARTESIAN_POINT('Ctrl Pts',(15.777288771741,53.7916708150444,3.08595833271761));
#57106=CARTESIAN_POINT('Ctrl Pts',(15.1814089486113,54.4369910204986,3.1289575562939));
#57107=CARTESIAN_POINT('Ctrl Pts',(14.8991095940519,54.6023050298359,3.14578827641127));
#57108=CARTESIAN_POINT('Ctrl Pts',(14.8992309062956,54.6029598038327,2.60421172358873));
#57109=CARTESIAN_POINT('Ctrl Pts',(14.7662449521696,54.681123251708,2.61215584339723));
#57110=CARTESIAN_POINT('Ctrl Pts',(14.1480244437874,54.9322850073565,2.64626846666466));
#57111=CARTESIAN_POINT('Ctrl Pts',(12.8743150895914,54.5809192738243,2.70654959339101));
#57112=CARTESIAN_POINT('Ctrl Pts',(12.3410089780029,52.9449163922479,2.78505510376779));
#57113=CARTESIAN_POINT('Ctrl Pts',(13.4114743235374,51.5976690199096,2.86356061414457));
#57114=CARTESIAN_POINT('Ctrl Pts',(15.125685020798,51.7474403844543,2.94206612452135));
#57115=CARTESIAN_POINT('Ctrl Pts',(15.9462998191018,53.2599021194416,3.02057163489813));
#57116=CARTESIAN_POINT('Ctrl Pts',(15.3893775359764,54.3055097335425,3.07462016792059));
#57117=CARTESIAN_POINT('Ctrl Pts',(14.9310645035309,54.588383814741,3.10250019748412));
#57118=CARTESIAN_POINT('Ctrl Pts',(14.9023562176693,54.604775754849,3.10421172358873));
#57119=CARTESIAN_POINT('Origin',(14.1292828945603,53.2669068454841,0.895788276411274));
#57120=CARTESIAN_POINT('',(14.9013089558621,54.600969116598,2.10421172358873));
#57121=CARTESIAN_POINT('',(14.9010809748678,54.6051974101417,2.14578827641127));
#57122=CARTESIAN_POINT('',(14.9007828945603,54.6031840435236,0.895788276411274));
#57123=CARTESIAN_POINT('',(15.6194800884629,52.866705242183,2.));
#57124=CARTESIAN_POINT('Ctrl Pts',(15.6194800884629,52.866705242183,2.));
#57125=CARTESIAN_POINT('Ctrl Pts',(15.7510836294753,53.3567463262429,2.02616850345893));
#57126=CARTESIAN_POINT('Ctrl Pts',(15.5785415188313,54.0947786094125,2.06090574465517));
#57127=CARTESIAN_POINT('Ctrl Pts',(15.0460508163988,54.5187167298269,2.09564298585141));
#57128=CARTESIAN_POINT('Ctrl Pts',(14.9013089558621,54.600969116598,2.10421172358873));
#57129=CARTESIAN_POINT('',(15.2224998162609,52.1743915631094,2.));
#57130=CARTESIAN_POINT('Origin',(14.1292828945603,53.2669068454841,2.));
#57131=CARTESIAN_POINT('Ctrl Pts',(15.2225082026616,52.1743802571171,2.));
#57132=CARTESIAN_POINT('Ctrl Pts',(15.5613276195564,52.5158503863372,2.02490816038701));
#57133=CARTESIAN_POINT('Ctrl Pts',(15.8908670066042,53.5171650620887,2.0735042525241));
#57134=CARTESIAN_POINT('Ctrl Pts',(15.2959835850222,54.3738753315586,2.12210034466119));
#57135=CARTESIAN_POINT('Ctrl Pts',(14.9010809748678,54.6051974101417,2.14578827641127));
#57136=CARTESIAN_POINT('Origin',(-39.0658530619283,38.8697713466882,4.5));
#57137=CARTESIAN_POINT('',(-39.6970780592613,39.9631802546368,5.80658032638059));
#57138=CARTESIAN_POINT('',(-39.6962628554159,39.9650155589839,5.94341967361941));
#57139=CARTESIAN_POINT('',(-39.6981030619283,39.9648604697737,4.5));
#57140=CARTESIAN_POINT('',(-40.2595650866585,39.2869186252538,6.));
#57141=CARTESIAN_POINT('Ctrl Pts',(-39.6962628554159,39.9650155589839,5.94341967361941));
#57142=CARTESIAN_POINT('Ctrl Pts',(-39.9540142218038,39.8131911161898,5.96227978241294));
#57143=CARTESIAN_POINT('Ctrl Pts',(-40.160699881421,39.5698320958276,5.98113989120647));
#57144=CARTESIAN_POINT('Ctrl Pts',(-40.2595650866585,39.2869186252538,6.));
#57145=CARTESIAN_POINT('',(-39.6981030619283,39.9648604697737,6.));
#57146=CARTESIAN_POINT('Origin',(-39.0658530619283,38.8697713466882,6.));
#57147=CARTESIAN_POINT('',(-39.6981030619283,39.9648604697737,7.));
#57148=CARTESIAN_POINT('',(-39.6981030619283,39.9648604697737,4.5));
#57149=CARTESIAN_POINT('',(-39.7608672580762,37.8134023216061,7.));
#57150=CARTESIAN_POINT('Origin',(-39.0658530619283,38.8697713466882,7.));
#57151=CARTESIAN_POINT('',(-38.3708388657805,39.9261403717704,7.));
#57152=CARTESIAN_POINT('Origin',(-39.0658530619283,38.8697713466882,7.));
#57153=CARTESIAN_POINT('Origin',(-39.0658530619283,38.8697713466882,7.));
#57154=CARTESIAN_POINT('',(-39.3015291113282,37.6253036020567,6.));
#57155=CARTESIAN_POINT('Origin',(-39.0658530619283,38.8697713466882,6.));
#57156=CARTESIAN_POINT('Ctrl Pts',(-39.3015295597333,37.6252918061955,6.));
#57157=CARTESIAN_POINT('Ctrl Pts',(-39.6885932560667,37.7000310216234,5.97509183961299));
#57158=CARTESIAN_POINT('Ctrl Pts',(-40.0399430624791,37.9695097738977,5.95018367922598));
#57159=CARTESIAN_POINT('Ctrl Pts',(-40.2093203959796,38.3254113926459,5.92527551883898));
#57160=CARTESIAN_POINT('Ctrl Pts',(-40.3872681556177,38.6993214926512,5.89910701538005));
#57161=CARTESIAN_POINT('Ctrl Pts',(-40.3643620641528,39.1686216551033,5.87293851192112));
#57162=CARTESIAN_POINT('Ctrl Pts',(-40.1507501683313,39.5232214807692,5.8467700084622));
#57163=CARTESIAN_POINT('Ctrl Pts',(-40.0413948614145,39.7047533782285,5.83337344776833));
#57164=CARTESIAN_POINT('Ctrl Pts',(-39.8820599551598,39.8562249589825,5.81997688707446));
#57165=CARTESIAN_POINT('Ctrl Pts',(-39.6970780592613,39.9631802546368,5.80658032638059));
#57166=CARTESIAN_POINT('Origin',(-39.0658530619283,38.8697713466882,4.5));
#57167=CARTESIAN_POINT('',(-39.6980969738519,39.9664052404927,5.30658032638059));
#57168=CARTESIAN_POINT('',(-39.6994431549996,39.9659335873643,5.44341967361941));
#57169=CARTESIAN_POINT('',(-39.6981030619283,39.9648604697737,4.5));
#57170=CARTESIAN_POINT('Ctrl Pts',(-39.6994431549996,39.9659335873643,5.44341967361941));
#57171=CARTESIAN_POINT('Ctrl Pts',(-39.7317442057588,39.9475451778338,5.44576692486712));
#57172=CARTESIAN_POINT('Ctrl Pts',(-39.7631672715511,39.9276731785137,5.44811417611483));
#57173=CARTESIAN_POINT('Ctrl Pts',(-39.7935612952929,39.9063356334612,5.45046142736254));
#57174=CARTESIAN_POINT('Ctrl Pts',(-40.1324113081289,39.6684524404899,5.47662993082147));
#57175=CARTESIAN_POINT('Ctrl Pts',(-40.3433609694206,39.2484155500404,5.50279843428039));
#57176=CARTESIAN_POINT('Ctrl Pts',(-40.3318541433896,38.8345478072092,5.52896693773932));
#57177=CARTESIAN_POINT('Ctrl Pts',(-40.3203473173587,38.420680064378,5.55513544119825));
#57178=CARTESIAN_POINT('Ctrl Pts',(-40.086384004005,38.0129814691651,5.58130394465717));
#57179=CARTESIAN_POINT('Ctrl Pts',(-39.7348031115542,37.7943227533549,5.6074724481161));
#57180=CARTESIAN_POINT('Ctrl Pts',(-39.3832222191033,37.5756640375447,5.63364095157503));
#57181=CARTESIAN_POINT('Ctrl Pts',(-38.9140237475553,37.5460452011372,5.65980945503395));
#57182=CARTESIAN_POINT('Ctrl Pts',(-38.5377492251912,37.7186390805662,5.68597795849288));
#57183=CARTESIAN_POINT('Ctrl Pts',(-38.1614747028271,37.8912329599952,5.7121464619518));
#57184=CARTESIAN_POINT('Ctrl Pts',(-37.8781241296468,38.2660395552607,5.73831496541073));
#57185=CARTESIAN_POINT('Ctrl Pts',(-37.814457003614,38.6752103329024,5.76448346886966));
#57186=CARTESIAN_POINT('Ctrl Pts',(-37.7507898775812,39.0843811105442,5.79065197232858));
#57187=CARTESIAN_POINT('Ctrl Pts',(-37.9068061986959,39.5279160705621,5.81682047578751));
#57188=CARTESIAN_POINT('Ctrl Pts',(-38.2131591663055,39.8064837741936,5.84298897924644));
#57189=CARTESIAN_POINT('Ctrl Pts',(-38.5195121339152,40.0850514778251,5.86915748270536));
#57190=CARTESIAN_POINT('Ctrl Pts',(-38.9762017480197,40.1986519250703,5.89532598616429));
#57191=CARTESIAN_POINT('Ctrl Pts',(-39.3769209838015,40.0972547064535,5.92149448962322));
#57192=CARTESIAN_POINT('Ctrl Pts',(-39.4888346944845,40.0689362780501,5.92880288428861));
#57193=CARTESIAN_POINT('Ctrl Pts',(-39.5963828000181,40.0238483557584,5.93611127895401));
#57194=CARTESIAN_POINT('Ctrl Pts',(-39.6962628554159,39.9650155589839,5.94341967361941));
#57195=CARTESIAN_POINT('Ctrl Pts',(-39.6970780592613,39.9631802546368,5.80658032638059));
#57196=CARTESIAN_POINT('Ctrl Pts',(-39.520720989639,40.0651487333929,5.79380838361554));
#57197=CARTESIAN_POINT('Ctrl Pts',(-39.3210527704035,40.1266553179232,5.78103644085048));
#57198=CARTESIAN_POINT('Ctrl Pts',(-39.1191586941911,40.1351732662231,5.76826449808542));
#57199=CARTESIAN_POINT('Ctrl Pts',(-38.7054968160504,40.1526257371314,5.7420959946265));
#57200=CARTESIAN_POINT('Ctrl Pts',(-38.2824907599468,39.9476311900682,5.71592749116757));
#57201=CARTESIAN_POINT('Ctrl Pts',(-38.0397913612151,39.6121973316471,5.68975898770864));
#57202=CARTESIAN_POINT('Ctrl Pts',(-37.7970919624834,39.2767634732261,5.66359048424972));
#57203=CARTESIAN_POINT('Ctrl Pts',(-37.7346992211236,38.8108903034471,5.63742198079079));
#57204=CARTESIAN_POINT('Ctrl Pts',(-37.8806057126089,38.4234383862029,5.61125347733186));
#57205=CARTESIAN_POINT('Ctrl Pts',(-38.0265122040943,38.0359864689587,5.58508497387294));
#57206=CARTESIAN_POINT('Ctrl Pts',(-38.3807179284248,37.7269558042492,5.55891647041401));
#57207=CARTESIAN_POINT('Ctrl Pts',(-38.7843854256714,37.6349404921318,5.53274796695508));
#57208=CARTESIAN_POINT('Ctrl Pts',(-39.188052922918,37.5429251800145,5.50657946349616));
#57209=CARTESIAN_POINT('Ctrl Pts',(-39.6411821930806,37.6679252204893,5.48041096003723));
#57210=CARTESIAN_POINT('Ctrl Pts',(-39.9405883560671,37.9538786579723,5.4542424565783));
#57211=CARTESIAN_POINT('Ctrl Pts',(-40.2399945190536,38.2398320954553,5.42807395311938));
#57212=CARTESIAN_POINT('Ctrl Pts',(-40.3856775748639,38.6867389299465,5.40190544966045));
#57213=CARTESIAN_POINT('Ctrl Pts',(-40.312309689211,39.0942060073491,5.37573694620152));
#57214=CARTESIAN_POINT('Ctrl Pts',(-40.2476788760258,39.4531495468055,5.35268473959455));
#57215=CARTESIAN_POINT('Ctrl Pts',(-40.0130623748058,39.7814874463141,5.32963253298757));
#57216=CARTESIAN_POINT('Ctrl Pts',(-39.6980969738519,39.9664052404927,5.30658032638059));
#57217=CARTESIAN_POINT('Origin',(-39.0658530619283,38.8697713466882,4.5));
#57218=CARTESIAN_POINT('',(-39.6989570949589,39.9641614067485,4.80658032638059));
#57219=CARTESIAN_POINT('',(-39.697389467188,39.9630895992609,4.94341967361941));
#57220=CARTESIAN_POINT('',(-39.6981030619283,39.9648604697737,4.5));
#57221=CARTESIAN_POINT('Ctrl Pts',(-39.697389467188,39.9630895992609,4.94341967361941));
#57222=CARTESIAN_POINT('Ctrl Pts',(-39.8633425703643,39.8677036169061,4.95542257078023));
#57223=CARTESIAN_POINT('Ctrl Pts',(-40.0085235722312,39.7366393919841,4.96742546794105));
#57224=CARTESIAN_POINT('Ctrl Pts',(-40.1149177943607,39.5793405247057,4.97942836510186));
#57225=CARTESIAN_POINT('Ctrl Pts',(-40.3468765900167,39.2364003247431,5.00559686856079));
#57226=CARTESIAN_POINT('Ctrl Pts',(-40.3944742703016,38.7687617621182,5.03176537201971));
#57227=CARTESIAN_POINT('Ctrl Pts',(-40.2363680070802,38.3861191307629,5.05793387547864));
#57228=CARTESIAN_POINT('Ctrl Pts',(-40.0782617438588,38.0034764994076,5.08410237893757));
#57229=CARTESIAN_POINT('Ctrl Pts',(-39.7144515371312,37.705829799322,5.1102708823965));
#57230=CARTESIAN_POINT('Ctrl Pts',(-39.3080731239833,37.626648148232,5.13643938585542));
#57231=CARTESIAN_POINT('Ctrl Pts',(-38.9016947108354,37.5474664971421,5.16260788931435));
#57232=CARTESIAN_POINT('Ctrl Pts',(-38.4527480912673,37.6867498950478,5.18877639277327));
#57233=CARTESIAN_POINT('Ctrl Pts',(-38.1625484528667,37.982040398373,5.2149448962322));
#57234=CARTESIAN_POINT('Ctrl Pts',(-37.8723488144662,38.2773309016981,5.24111339969112));
#57235=CARTESIAN_POINT('Ctrl Pts',(-37.7408961572331,38.7286285104427,5.26728190315005));
#57236=CARTESIAN_POINT('Ctrl Pts',(-37.8271310042327,39.1335692645202,5.29345040660898));
#57237=CARTESIAN_POINT('Ctrl Pts',(-37.9133658512322,39.5385100185978,5.31961891006791));
#57238=CARTESIAN_POINT('Ctrl Pts',(-38.2172882024643,39.8970939180084,5.34578741352683));
#57239=CARTESIAN_POINT('Ctrl Pts',(-38.6026245602705,40.0485211199671,5.37195591698576));
#57240=CARTESIAN_POINT('Ctrl Pts',(-38.9533971820163,40.1863656694332,5.39577716919697));
#57241=CARTESIAN_POINT('Ctrl Pts',(-39.3716335617261,40.1525497161724,5.41959842140819));
#57242=CARTESIAN_POINT('Ctrl Pts',(-39.6994431549996,39.9659335873643,5.44341967361941));
#57243=CARTESIAN_POINT('Ctrl Pts',(-39.6980969738519,39.9664052404927,5.30658032638059));
#57244=CARTESIAN_POINT('Ctrl Pts',(-39.6555185906107,39.9914032265725,5.30346402952864));
#57245=CARTESIAN_POINT('Ctrl Pts',(-39.6114718472881,40.0137802388959,5.30034773267669));
#57246=CARTESIAN_POINT('Ctrl Pts',(-39.5661781885584,40.033257573116,5.29723143582475));
#57247=CARTESIAN_POINT('Ctrl Pts',(-39.1858334006749,40.1968147411666,5.27106293236582));
#57248=CARTESIAN_POINT('Ctrl Pts',(-38.7175626520242,40.1559017569539,5.24489442890689));
#57249=CARTESIAN_POINT('Ctrl Pts',(-38.3713436649215,39.928865763386,5.21872592544796));
#57250=CARTESIAN_POINT('Ctrl Pts',(-38.0251246778187,39.701829769818,5.19255742198904));
#57251=CARTESIAN_POINT('Ctrl Pts',(-37.8009574522638,39.2886707668948,5.16638891853011));
#57252=CARTESIAN_POINT('Ctrl Pts',(-37.7993614588042,38.8746535306862,5.14022041507118));
#57253=CARTESIAN_POINT('Ctrl Pts',(-37.7977654653446,38.4606362944776,5.11405191161226));
#57254=CARTESIAN_POINT('Ctrl Pts',(-38.0187407039802,38.0457608249837,5.08788340815333));
#57255=CARTESIAN_POINT('Ctrl Pts',(-38.3631991409408,37.8160625276688,5.06171490469441));
#57256=CARTESIAN_POINT('Ctrl Pts',(-38.7076575779013,37.5863642303539,5.03554640123548));
#57257=CARTESIAN_POINT('Ctrl Pts',(-39.1755992131868,37.5418431052181,5.00937789777655));
#57258=CARTESIAN_POINT('Ctrl Pts',(-39.5571935097812,37.7024627985795,4.98320939431763));
#57259=CARTESIAN_POINT('Ctrl Pts',(-39.9387878063755,37.863082491941,4.9570408908587));
#57260=CARTESIAN_POINT('Ctrl Pts',(-40.2340347642788,38.2288430037995,4.93087238739978));
#57261=CARTESIAN_POINT('Ctrl Pts',(-40.3105421109526,38.635733049973,4.90470388394085));
#57262=CARTESIAN_POINT('Ctrl Pts',(-40.3870494576263,39.0426230961465,4.87853538048192));
#57263=CARTESIAN_POINT('Ctrl Pts',(-40.2448171930705,39.4906426766349,4.85236687702299));
#57264=CARTESIAN_POINT('Ctrl Pts',(-39.9476239688235,39.7788944478041,4.82619837356406));
#57265=CARTESIAN_POINT('Ctrl Pts',(-39.8733571986579,39.8509268034996,4.81965902450291));
#57266=CARTESIAN_POINT('Ctrl Pts',(-39.789413588409,39.9129821459892,4.81311967544175));
#57267=CARTESIAN_POINT('Ctrl Pts',(-39.6989570949589,39.9641614067485,4.80658032638059));
#57268=CARTESIAN_POINT('Origin',(-39.0658530619283,38.8697713466882,4.5));
#57269=CARTESIAN_POINT('',(-39.6967352121902,39.9639200225483,4.30658032638059));
#57270=CARTESIAN_POINT('',(-39.6976237458347,39.9660095563765,4.44341967361941));
#57271=CARTESIAN_POINT('',(-39.6981030619283,39.9648604697737,4.5));
#57272=CARTESIAN_POINT('Ctrl Pts',(-39.6976237458347,39.9660095563765,4.44341967361941));
#57273=CARTESIAN_POINT('Ctrl Pts',(-39.9936753773632,39.7916729655961,4.46507821669334));
#57274=CARTESIAN_POINT('Ctrl Pts',(-40.2204527828214,39.4929448719807,4.48673675976726));
#57275=CARTESIAN_POINT('Ctrl Pts',(-40.2988032317419,39.159355592007,4.50839530284118));
#57276=CARTESIAN_POINT('Ctrl Pts',(-40.3934686017341,38.756302986065,4.53456380630011));
#57277=CARTESIAN_POINT('Ctrl Pts',(-40.2714573392084,38.3023593247386,4.56073230975904));
#57278=CARTESIAN_POINT('Ctrl Pts',(-39.9874807525881,38.0010783358291,4.58690081321797));
#57279=CARTESIAN_POINT('Ctrl Pts',(-39.7035041659678,37.6997973469195,4.61306931667689));
#57280=CARTESIAN_POINT('Ctrl Pts',(-39.2575622552529,37.5511790304267,4.63923782013582));
#57281=CARTESIAN_POINT('Ctrl Pts',(-38.8496206579413,37.6218656179337,4.66540632359474));
#57282=CARTESIAN_POINT('Ctrl Pts',(-38.4416790606296,37.6925522054406,4.69157482705367));
#57283=CARTESIAN_POINT('Ctrl Pts',(-38.0717377767213,37.9825436969474,4.7177433305126));
#57284=CARTESIAN_POINT('Ctrl Pts',(-37.9056829078162,38.361804436646,4.74391183397152));
#57285=CARTESIAN_POINT('Ctrl Pts',(-37.739628038911,38.7410651763447,4.77008033743045));
#57286=CARTESIAN_POINT('Ctrl Pts',(-37.777459585009,39.2095951642353,4.79624884088937));
#57287=CARTESIAN_POINT('Ctrl Pts',(-38.0022133656486,39.5573000327044,4.8224173443483));
#57288=CARTESIAN_POINT('Ctrl Pts',(-38.2269671462881,39.9050049011735,4.84858584780723));
#57289=CARTESIAN_POINT('Ctrl Pts',(-38.6386431614694,40.1318846502211,4.87475435126616));
#57290=CARTESIAN_POINT('Ctrl Pts',(-39.0526411245735,40.1362036060948,4.90092285472508));
#57291=CARTESIAN_POINT('Ctrl Pts',(-39.2767476411253,40.1385415551724,4.91508846102319));
#57292=CARTESIAN_POINT('Ctrl Pts',(-39.5015345588232,40.0756624434911,4.9292540673213));
#57293=CARTESIAN_POINT('Ctrl Pts',(-39.697389467188,39.9630895992609,4.94341967361941));
#57294=CARTESIAN_POINT('Ctrl Pts',(-39.6989570949589,39.9641614067485,4.80658032638059));
#57295=CARTESIAN_POINT('Ctrl Pts',(-39.4274339724573,40.1177861180174,4.78695117198282));
#57296=CARTESIAN_POINT('Ctrl Pts',(-39.0972285087862,40.1734152228909,4.76732201758506));
#57297=CARTESIAN_POINT('Ctrl Pts',(-38.7939127211062,40.1067326165456,4.74769286318729));
#57298=CARTESIAN_POINT('Ctrl Pts',(-38.389548881574,40.0178350522677,4.72152435972836));
#57299=CARTESIAN_POINT('Ctrl Pts',(-38.0329753864478,39.7115559618618,4.69535585626944));
#57300=CARTESIAN_POINT('Ctrl Pts',(-37.8840840327676,39.3252345207529,4.66918735281051));
#57301=CARTESIAN_POINT('Ctrl Pts',(-37.7351926790873,38.9389130796439,4.64301884935158));
#57302=CARTESIAN_POINT('Ctrl Pts',(-37.7939834668531,38.472549287832,4.61685034589266));
#57303=CARTESIAN_POINT('Ctrl Pts',(-38.0340939063583,38.1352662178079,4.59068184243373));
#57304=CARTESIAN_POINT('Ctrl Pts',(-38.2742043458636,37.7979831477837,4.5645133389748));
#57305=CARTESIAN_POINT('Ctrl Pts',(-38.6956344371082,37.5897807995474,4.53834483551588));
#57306=CARTESIAN_POINT('Ctrl Pts',(-39.1094099185268,37.6040195786007,4.51217633205695));
#57307=CARTESIAN_POINT('Ctrl Pts',(-39.5231853999454,37.618258357654,4.48600782859802));
#57308=CARTESIAN_POINT('Ctrl Pts',(-39.929306271538,37.854938263997,4.4598393251391));
#57309=CARTESIAN_POINT('Ctrl Pts',(-40.1456631065935,38.2079292154005,4.43367082168017));
#57310=CARTESIAN_POINT('Ctrl Pts',(-40.3620199416489,38.560920166804,4.40750231822124));
#57311=CARTESIAN_POINT('Ctrl Pts',(-40.3886127401672,39.0302221632679,4.38133381476232));
#57312=CARTESIAN_POINT('Ctrl Pts',(-40.2135169753906,39.4053946105006,4.35516531130339));
#57313=CARTESIAN_POINT('Ctrl Pts',(-40.1051548355753,39.6375789196628,4.33897031632912));
#57314=CARTESIAN_POINT('Ctrl Pts',(-39.919545071043,39.8337111891107,4.32277532135486));
#57315=CARTESIAN_POINT('Ctrl Pts',(-39.6967352121902,39.9639200225483,4.30658032638059));
#57316=CARTESIAN_POINT('Origin',(-39.0658530619283,38.8697713466882,4.5));
#57317=CARTESIAN_POINT('',(-39.6990217970716,39.9666307803347,3.80658032638059));
#57318=CARTESIAN_POINT('',(-39.6992442211058,39.9647402889406,3.94341967361941));
#57319=CARTESIAN_POINT('',(-39.6981030619283,39.9648604697737,4.5));
#57320=CARTESIAN_POINT('Ctrl Pts',(-39.6992442211058,39.9647402889406,3.94341967361941));
#57321=CARTESIAN_POINT('Ctrl Pts',(-39.7703349168266,39.9245305221536,3.94856535914752));
#57322=CARTESIAN_POINT('Ctrl Pts',(-39.8373290103598,39.877480560471,3.95371104467563));
#57323=CARTESIAN_POINT('Ctrl Pts',(-39.8986640775364,39.8239468894644,3.95885673020373));
#57324=CARTESIAN_POINT('Ctrl Pts',(-40.2105849885205,39.551700160189,3.98502523366266));
#57325=CARTESIAN_POINT('Ctrl Pts',(-40.3761490651667,39.1117681946799,4.01119373712159));
#57326=CARTESIAN_POINT('Ctrl Pts',(-40.3211154074003,38.7014217157033,4.03736224058051));
#57327=CARTESIAN_POINT('Ctrl Pts',(-40.2660817496338,38.2910752367267,4.06353074403944));
#57328=CARTESIAN_POINT('Ctrl Pts',(-39.9904503574547,37.9103142442825,4.08969924749836));
#57329=CARTESIAN_POINT('Ctrl Pts',(-39.6178176236238,37.7298764933343,4.11586775095729));
#57330=CARTESIAN_POINT('Ctrl Pts',(-39.245184889793,37.5494387423861,4.14203625441622));
#57331=CARTESIAN_POINT('Ctrl Pts',(-38.7755508143104,37.5693242329338,4.16820475787514));
#57332=CARTESIAN_POINT('Ctrl Pts',(-38.4195048988347,37.780616074816,4.19437326133407));
#57333=CARTESIAN_POINT('Ctrl Pts',(-38.0634589833589,37.9919079166982,4.220541764793));
#57334=CARTESIAN_POINT('Ctrl Pts',(-37.82100122789,38.3946061099149,4.24671026825192));
#57335=CARTESIAN_POINT('Ctrl Pts',(-37.8008525725161,38.8081359974719,4.27287877171085));
#57336=CARTESIAN_POINT('Ctrl Pts',(-37.7807039171422,39.221665885029,4.29904727516978));
#57337=CARTESIAN_POINT('Ctrl Pts',(-37.9828643618632,39.6460274669263,4.3252157786287));
#57338=CARTESIAN_POINT('Ctrl Pts',(-38.3166827592479,39.8909319662484,4.35138428208763));
#57339=CARTESIAN_POINT('Ctrl Pts',(-38.6505011566327,40.1358364655705,4.37755278554655));
#57340=CARTESIAN_POINT('Ctrl Pts',(-39.1159775066813,40.2012838823174,4.40372128900548));
#57341=CARTESIAN_POINT('Ctrl Pts',(-39.5043866829606,40.057926815412,4.42988979246441));
#57342=CARTESIAN_POINT('Ctrl Pts',(-39.571326315215,40.0332202175102,4.43439975284941));
#57343=CARTESIAN_POINT('Ctrl Pts',(-39.6359768878004,40.0023116804572,4.43890971323441));
#57344=CARTESIAN_POINT('Ctrl Pts',(-39.6976237458347,39.9660095563765,4.44341967361941));
#57345=CARTESIAN_POINT('Ctrl Pts',(-39.6967352121902,39.9639200225483,4.30658032638059));
#57346=CARTESIAN_POINT('Ctrl Pts',(-39.5595202256302,40.0441076920801,4.29660681789593));
#57347=CARTESIAN_POINT('Ctrl Pts',(-39.4081968207293,40.0992933977544,4.28663330941127));
#57348=CARTESIAN_POINT('Ctrl Pts',(-39.2521185625475,40.1225003286185,4.27665980092661));
#57349=CARTESIAN_POINT('Ctrl Pts',(-38.8426002425525,40.1833907015023,4.25049129746768));
#57350=CARTESIAN_POINT('Ctrl Pts',(-38.4003479306342,40.0241285492682,4.22432279400876));
#57351=CARTESIAN_POINT('Ctrl Pts',(-38.1236728204874,39.7161289139554,4.19815429054983));
#57352=CARTESIAN_POINT('Ctrl Pts',(-37.8469977103406,39.4081292786425,4.17198578709091));
#57353=CARTESIAN_POINT('Ctrl Pts',(-37.7358998019654,38.9513921602507,4.14581728363198));
#57354=CARTESIAN_POINT('Ctrl Pts',(-37.840196718037,38.5507239118952,4.11964878017305));
#57355=CARTESIAN_POINT('Ctrl Pts',(-37.9444936341086,38.1500556635396,4.09348027671412));
#57356=CARTESIAN_POINT('Ctrl Pts',(-38.2641853746271,37.8054562852203,4.0673117732552));
#57357=CARTESIAN_POINT('Ctrl Pts',(-38.6559183630715,37.6714482343173,4.04114326979627));
#57358=CARTESIAN_POINT('Ctrl Pts',(-39.0476513515158,37.5374401834144,4.01497476633735));
#57359=CARTESIAN_POINT('Ctrl Pts',(-39.5114255878859,37.6140234599276,3.98880626287842));
#57360=CARTESIAN_POINT('Ctrl Pts',(-39.8392791917195,37.8668572123835,3.9626377594195));
#57361=CARTESIAN_POINT('Ctrl Pts',(-40.1671327955531,38.1196909648394,3.93646925596057));
#57362=CARTESIAN_POINT('Ctrl Pts',(-40.3590657668502,38.548775193238,3.91030075250164));
#57363=CARTESIAN_POINT('Ctrl Pts',(-40.3290130799472,38.9617034290506,3.88413224904271));
#57364=CARTESIAN_POINT('Ctrl Pts',(-40.2993254358659,39.3696159240468,3.85828160815534));
#57365=CARTESIAN_POINT('Ctrl Pts',(-40.0530121946873,39.7617625287194,3.83243096726797));
#57366=CARTESIAN_POINT('Ctrl Pts',(-39.6990217970716,39.9666307803347,3.80658032638059));
#57367=CARTESIAN_POINT('Origin',(-39.0658530619283,38.8697713466882,4.5));
#57368=CARTESIAN_POINT('',(-39.6981666138854,39.9633157673857,3.30658032638059));
#57369=CARTESIAN_POINT('',(-39.6968376638892,39.9635050155947,3.44341967361941));
#57370=CARTESIAN_POINT('',(-39.6981030619283,39.9648604697737,4.5));
#57371=CARTESIAN_POINT('Ctrl Pts',(-39.6968376638892,39.9635050155947,3.44341967361941));
#57372=CARTESIAN_POINT('Ctrl Pts',(-39.9008619683973,39.8448845676908,3.45822100506062));
#57373=CARTESIAN_POINT('Ctrl Pts',(-40.0737604294823,39.6716358129756,3.47302233650184));
#57374=CARTESIAN_POINT('Ctrl Pts',(-40.1838048209619,39.4649259634328,3.48782366794305));
#57375=CARTESIAN_POINT('Ctrl Pts',(-40.3783614424731,39.0994664482373,3.51399217140198));
#57376=CARTESIAN_POINT('Ctrl Pts',(-40.3764510665601,38.6294154424261,3.54016067486091));
#57377=CARTESIAN_POINT('Ctrl Pts',(-40.1789303273027,38.265549404193,3.56632917831983));
#57378=CARTESIAN_POINT('Ctrl Pts',(-39.9814095880453,37.9016833659598,3.59249768177876));
#57379=CARTESIAN_POINT('Ctrl Pts',(-39.5882784854434,37.6440022953046,3.61866618523768));
#57380=CARTESIAN_POINT('Ctrl Pts',(-39.1758216795725,37.6080534474274,3.64483468869661));
#57381=CARTESIAN_POINT('Ctrl Pts',(-38.7633648737016,37.5721045995503,3.67100319215554));
#57382=CARTESIAN_POINT('Ctrl Pts',(-38.3315823645617,37.7578879744511,3.69717169561447));
#57383=CARTESIAN_POINT('Ctrl Pts',(-38.0740905614766,38.0820960983985,3.72334019907339));
#57384=CARTESIAN_POINT('Ctrl Pts',(-37.8165987583915,38.4063042223459,3.74950870253232));
#57385=CARTESIAN_POINT('Ctrl Pts',(-37.7333976613612,38.8689370953399,3.77567720599125));
#57386=CARTESIAN_POINT('Ctrl Pts',(-37.8617956314422,39.2625446379184,3.80184570945017));
#57387=CARTESIAN_POINT('Ctrl Pts',(-37.9901936015233,39.6561521804969,3.8280142129091));
#57388=CARTESIAN_POINT('Ctrl Pts',(-38.3301906387158,39.9807343926601,3.85418271636802));
#57389=CARTESIAN_POINT('Ctrl Pts',(-38.7293280299731,40.0907447522208,3.88035121982695));
#57390=CARTESIAN_POINT('Ctrl Pts',(-39.0499804019726,40.1791230487932,3.90137403775777));
#57391=CARTESIAN_POINT('Ctrl Pts',(-39.408801529933,40.1290182265619,3.92239685568859));
#57392=CARTESIAN_POINT('Ctrl Pts',(-39.6992442211058,39.9647402889406,3.94341967361941));
#57393=CARTESIAN_POINT('Ctrl Pts',(-39.6990217970716,39.9666307803347,3.80658032638059));
#57394=CARTESIAN_POINT('Ctrl Pts',(-39.6946690888126,39.9691498648546,3.80626246380904));
#57395=CARTESIAN_POINT('Ctrl Pts',(-39.6903001003537,39.9716406339069,3.80594460123749));
#57396=CARTESIAN_POINT('Ctrl Pts',(-39.6859150342415,39.9741027686317,3.80562673866594));
#57397=CARTESIAN_POINT('Ctrl Pts',(-39.3249080205419,40.1768016291735,3.77945823520701));
#57398=CARTESIAN_POINT('Ctrl Pts',(-38.8549323382457,40.1854271070305,3.75328973174808));
#57399=CARTESIAN_POINT('Ctrl Pts',(-38.486730670363,39.9961114351584,3.72712122828915));
#57400=CARTESIAN_POINT('Ctrl Pts',(-38.1185290024804,39.8067957632863,3.70095272483023));
#57401=CARTESIAN_POINT('Ctrl Pts',(-37.8521013490113,39.4195389416852,3.6747842213713));
#57402=CARTESIAN_POINT('Ctrl Pts',(-37.806917035636,39.007991532901,3.64861571791238));
#57403=CARTESIAN_POINT('Ctrl Pts',(-37.7617327222606,38.5964441241169,3.62244721445345));
#57404=CARTESIAN_POINT('Ctrl Pts',(-37.9377917489789,38.1606061281498,3.59627871099452));
#57405=CARTESIAN_POINT('Ctrl Pts',(-38.2561471576722,37.8959124821361,3.57011020753559));
#57406=CARTESIAN_POINT('Ctrl Pts',(-38.5745025663655,37.6312188361224,3.54394170407667));
#57407=CARTESIAN_POINT('Ctrl Pts',(-39.0351543570338,37.5376695400622,3.51777320061774));
#57408=CARTESIAN_POINT('Ctrl Pts',(-39.4315407865323,37.6572132122937,3.49160469715882));
#57409=CARTESIAN_POINT('Ctrl Pts',(-39.8279272160309,37.7767568845251,3.46543619369989));
#57410=CARTESIAN_POINT('Ctrl Pts',(-40.1600482843597,38.1093935250483,3.43926769024096));
#57411=CARTESIAN_POINT('Ctrl Pts',(-40.2789769657406,38.5059649062658,3.41309918678203));
#57412=CARTESIAN_POINT('Ctrl Pts',(-40.3979056471215,38.9025362874833,3.38693068332311));
#57413=CARTESIAN_POINT('Ctrl Pts',(-40.3036419415545,39.3630424093952,3.36076217986418));
#57414=CARTESIAN_POINT('Ctrl Pts',(-40.0384547967127,39.6809868610392,3.33459367640526));
#57415=CARTESIAN_POINT('Ctrl Pts',(-39.943827295091,39.7944399061765,3.3252558930637));
#57416=CARTESIAN_POINT('Ctrl Pts',(-39.8274361583624,39.8897406125527,3.31591810972215));
#57417=CARTESIAN_POINT('Ctrl Pts',(-39.6981666138854,39.9633157673857,3.30658032638059));
#57418=CARTESIAN_POINT('Origin',(-39.0658530619283,38.8697713466882,4.5));
#57419=CARTESIAN_POINT('',(-39.696945388151,39.9649932150637,2.80658032638059));
#57420=CARTESIAN_POINT('',(-39.6985897981371,39.9666323328488,2.94341967361941));
#57421=CARTESIAN_POINT('',(-39.6981030619283,39.9648604697737,4.5));
#57422=CARTESIAN_POINT('Ctrl Pts',(-39.6985897981371,39.9666323328488,2.94341967361941));
#57423=CARTESIAN_POINT('Ctrl Pts',(-40.0329227359304,39.771464492525,2.96787665097373));
#57424=CARTESIAN_POINT('Ctrl Pts',(-40.2741270402692,39.4118258938478,2.99233362832805));
#57425=CARTESIAN_POINT('Ctrl Pts',(-40.3224423052902,39.0279123314598,3.01679060568238));
#57426=CARTESIAN_POINT('Ctrl Pts',(-40.3741387255592,38.617132076822,3.0429591091413));
#57427=CARTESIAN_POINT('Ctrl Pts',(-40.2050042874718,38.1785603982041,3.06912761260023));
#57428=CARTESIAN_POINT('Ctrl Pts',(-39.8908808035795,37.908858034419,3.09529611605915));
#57429=CARTESIAN_POINT('Ctrl Pts',(-39.5767573196872,37.6391556706339,3.12146461951808));
#57430=CARTESIAN_POINT('Ctrl Pts',(-39.11764478999,37.5383226216818,3.14763312297701));
#57431=CARTESIAN_POINT('Ctrl Pts',(-38.7194147698321,37.6515736327838,3.17380162643593));
#57432=CARTESIAN_POINT('Ctrl Pts',(-38.3211847496743,37.7648246438858,3.19997012989486));
#57433=CARTESIAN_POINT('Ctrl Pts',(-37.9838372390559,38.092159715042,3.22613863335379));
#57434=CARTESIAN_POINT('Ctrl Pts',(-37.8586428520748,38.4867979056613,3.25230713681271));
#57435=CARTESIAN_POINT('Ctrl Pts',(-37.7334484650937,38.8814360962806,3.27847564027164));
#57436=CARTESIAN_POINT('Ctrl Pts',(-37.8204072017499,39.343377406363,3.30464414373057));
#57437=CARTESIAN_POINT('Ctrl Pts',(-38.080525740607,39.6654818632946,3.33081264718949));
#57438=CARTESIAN_POINT('Ctrl Pts',(-38.3406442794642,39.9875863202263,3.35698115064842));
#57439=CARTESIAN_POINT('Ctrl Pts',(-38.7739226205222,40.1698539240071,3.38314965410735));
#57440=CARTESIAN_POINT('Ctrl Pts',(-39.1860736005189,40.1305537136076,3.40931815756627));
#57441=CARTESIAN_POINT('Ctrl Pts',(-39.3651052785911,40.1134823418097,3.42068532958398));
#57442=CARTESIAN_POINT('Ctrl Pts',(-39.5401504513672,40.0546035118007,3.4320525016017));
#57443=CARTESIAN_POINT('Ctrl Pts',(-39.6968376638892,39.9635050155947,3.44341967361941));
#57444=CARTESIAN_POINT('Ctrl Pts',(-39.6981666138854,39.9633157673857,3.30658032638059));
#57445=CARTESIAN_POINT('Ctrl Pts',(-39.4651670418018,40.0959299856956,3.28974960626322));
#57446=CARTESIAN_POINT('Ctrl Pts',(-39.1903285963568,40.157963071813,3.27291888614585));
#57447=CARTESIAN_POINT('Ctrl Pts',(-38.9256802513517,40.1284914650089,3.25608816602848));
#57448=CARTESIAN_POINT('Ctrl Pts',(-38.5142034349489,40.0826688359585,3.22991966256955));
#57449=CARTESIAN_POINT('Ctrl Pts',(-38.1273603862597,39.8156407964813,3.20375115911062));
#57450=CARTESIAN_POINT('Ctrl Pts',(-37.9386160518288,39.4471459263554,3.1775826556517));
#57451=CARTESIAN_POINT('Ctrl Pts',(-37.749871717398,39.0786510562295,3.15141415219277));
#57452=CARTESIAN_POINT('Ctrl Pts',(-37.7592260972255,38.6086893554548,3.12524564873384));
#57453=CARTESIAN_POINT('Ctrl Pts',(-37.9624847270864,38.2479971709405,3.09907714527492));
#57454=CARTESIAN_POINT('Ctrl Pts',(-38.1657433569474,37.8873049864262,3.07290864181599));
#57455=CARTESIAN_POINT('Ctrl Pts',(-38.5629062368417,37.6358823181722,3.04674013835707));
#57456=CARTESIAN_POINT('Ctrl Pts',(-38.9758805061506,37.6064702124723,3.02057163489814));
#57457=CARTESIAN_POINT('Ctrl Pts',(-39.3888547754595,37.5770581067724,2.99440313143921));
#57458=CARTESIAN_POINT('Ctrl Pts',(-39.817640434183,37.7696565636265,2.96823462798029));
#57459=CARTESIAN_POINT('Ctrl Pts',(-40.0699655096421,38.0979018769219,2.94206612452136));
#57460=CARTESIAN_POINT('Ctrl Pts',(-40.3222905851012,38.4261471902174,2.91589762106243));
#57461=CARTESIAN_POINT('Ctrl Pts',(-40.398155077296,38.8900393599541,2.88972911760351));
#57462=CARTESIAN_POINT('Ctrl Pts',(-40.2635392087761,39.2815641648304,2.86356061414458));
#57463=CARTESIAN_POINT('Ctrl Pts',(-40.1658333166795,39.5657377972484,2.84456718488992));
#57464=CARTESIAN_POINT('Ctrl Pts',(-39.9572455465607,39.811788018551,2.82557375563525));
#57465=CARTESIAN_POINT('Ctrl Pts',(-39.696945388151,39.9649932150637,2.80658032638059));
#57466=CARTESIAN_POINT('Origin',(-39.0658530619283,38.8697713466882,4.5));
#57467=CARTESIAN_POINT('',(-39.6994125047665,39.9658989902663,2.30658032638059));
#57468=CARTESIAN_POINT('',(-39.6985816414592,39.9636701304732,2.44341967361941));
#57469=CARTESIAN_POINT('',(-39.6981030619283,39.9648604697737,4.5));
#57470=CARTESIAN_POINT('',(-39.3014489339361,37.6274127691862,2.));
#57471=CARTESIAN_POINT('Ctrl Pts',(-39.6994125047665,39.9658989902663,2.30658032638059));
#57472=CARTESIAN_POINT('Ctrl Pts',(-39.3734254452085,40.1513842194032,2.28289239463051));
#57473=CARTESIAN_POINT('Ctrl Pts',(-38.9582283391778,40.1860737601752,2.25920446288042));
#57474=CARTESIAN_POINT('Ctrl Pts',(-38.6086499461796,40.0507923518177,2.23551653113034));
#57475=CARTESIAN_POINT('Ctrl Pts',(-38.2224641245192,39.9013444371629,2.20934802767141));
#57476=CARTESIAN_POINT('Ctrl Pts',(-37.9163596177671,39.5444633609379,2.18317952421249));
#57477=CARTESIAN_POINT('Ctrl Pts',(-37.8282894528998,39.1398698141335,2.15701102075356));
#57478=CARTESIAN_POINT('Ctrl Pts',(-37.7402192880325,38.7352762673292,2.13084251729463));
#57479=CARTESIAN_POINT('Ctrl Pts',(-37.8701834650499,38.2829702499457,2.10467401383571));
#57480=CARTESIAN_POINT('Ctrl Pts',(-38.1583556110386,37.9866358554263,2.07850551037678));
#57481=CARTESIAN_POINT('Ctrl Pts',(-38.4465277570273,37.6903014609068,2.05233700691785));
#57482=CARTESIAN_POINT('Ctrl Pts',(-38.8929078719872,37.5499386892516,2.02616850345893));
#57483=CARTESIAN_POINT('Ctrl Pts',(-39.3014489339361,37.6274127691862,2.));
#57484=CARTESIAN_POINT('',(-40.2614317556684,39.2879039300605,2.00000000000001));
#57485=CARTESIAN_POINT('Origin',(-39.0658530619283,38.8697713466882,2.));
#57486=CARTESIAN_POINT('Ctrl Pts',(-40.261442204914,39.2879094456028,2.00000000000001));
#57487=CARTESIAN_POINT('Ctrl Pts',(-40.3902478674696,38.9153329576354,2.02490816038701));
#57488=CARTESIAN_POINT('Ctrl Pts',(-40.3325476766157,38.4763154063561,2.04981632077402));
#57489=CARTESIAN_POINT('Ctrl Pts',(-40.1090165446371,38.1516794088468,2.07472448116103));
#57490=CARTESIAN_POINT('Ctrl Pts',(-39.8741748257196,37.8106169581592,2.10089298461995));
#57491=CARTESIAN_POINT('Ctrl Pts',(-39.4562956252315,37.5958042374567,2.12706148807888));
#57492=CARTESIAN_POINT('Ctrl Pts',(-39.042397118114,37.6034976893836,2.1532299915378));
#57493=CARTESIAN_POINT('Ctrl Pts',(-38.6284986109964,37.6111911413105,2.17939849499673));
#57494=CARTESIAN_POINT('Ctrl Pts',(-38.2185807972492,37.841390765867,2.20556699845566));
#57495=CARTESIAN_POINT('Ctrl Pts',(-37.996635575997,38.1909062543644,2.23173550191458));
#57496=CARTESIAN_POINT('Ctrl Pts',(-37.7746903547448,38.5404217428618,2.25790400537351));
#57497=CARTESIAN_POINT('Ctrl Pts',(-37.7407177259875,39.0092530953003,2.28407250883244));
#57498=CARTESIAN_POINT('Ctrl Pts',(-37.909862273516,39.3871539257345,2.31024101229136));
#57499=CARTESIAN_POINT('Ctrl Pts',(-38.0790068210445,39.7650547561687,2.33640951575029));
#57500=CARTESIAN_POINT('Ctrl Pts',(-38.4512685448588,40.0520250645987,2.36257801920921));
#57501=CARTESIAN_POINT('Ctrl Pts',(-38.8597650567826,40.1193923002797,2.38874652266814));
#57502=CARTESIAN_POINT('Ctrl Pts',(-39.1442519845446,40.1663084852441,2.40697090631856));
#57503=CARTESIAN_POINT('Ctrl Pts',(-39.4463130348953,40.1067156626302,2.42519528996899));
#57504=CARTESIAN_POINT('Ctrl Pts',(-39.6985816414592,39.9636701304732,2.44341967361941));
#57505=CARTESIAN_POINT('Origin',(-39.0658530619283,38.8697713466882,0.895788276411275));
#57506=CARTESIAN_POINT('',(-39.8389883040075,40.2073580112695,5.60421172358873));
#57507=CARTESIAN_POINT('',(-39.8361023073888,40.2039982703455,5.64578827641128));
#57508=CARTESIAN_POINT('',(-39.8373530619284,40.2060485447276,0.895788276411275));
#57509=CARTESIAN_POINT('',(-37.5756558680257,39.2699729499894,6.));
#57510=CARTESIAN_POINT('Ctrl Pts',(-39.8361023073888,40.2039982703455,5.64578827641127));
#57511=CARTESIAN_POINT('Ctrl Pts',(-40.0618255698415,40.0734865888946,5.65918483710514));
#57512=CARTESIAN_POINT('Ctrl Pts',(-40.6360432757834,39.5276070596663,5.69874990125794));
#57513=CARTESIAN_POINT('Ctrl Pts',(-40.7062544764741,38.0891194878961,5.76448346886966));
#57514=CARTESIAN_POINT('Ctrl Pts',(-39.3195619844849,37.0695313077001,5.84298897924644));
#57515=CARTESIAN_POINT('Ctrl Pts',(-37.7040659529861,37.6679522088103,5.92149448962322));
#57516=CARTESIAN_POINT('Ctrl Pts',(-37.4440523270134,38.7799318659295,5.97383149654107));
#57517=CARTESIAN_POINT('Ctrl Pts',(-37.5756558680257,39.2699729499894,6.));
#57518=CARTESIAN_POINT('',(-37.9726388313436,39.9622904787117,6.));
#57519=CARTESIAN_POINT('Origin',(-39.0658530619283,38.8697713466882,6.));
#57520=CARTESIAN_POINT('Ctrl Pts',(-39.8389883040075,40.2073580112695,5.60421172358873));
#57521=CARTESIAN_POINT('Ctrl Pts',(-39.8784035047362,40.18491964361,5.60655897483644));
#57522=CARTESIAN_POINT('Ctrl Pts',(-40.3442265162732,39.8903323926484,5.63507472954307));
#57523=CARTESIAN_POINT('Ctrl Pts',(-40.8821362004287,38.8192621207561,5.68975898770863));
#57524=CARTESIAN_POINT('Ctrl Pts',(-40.0256584008921,37.3267854127763,5.76826449808542));
#57525=CARTESIAN_POINT('Ctrl Pts',(-38.3080469142999,37.2183586878016,5.84677000846219));
#57526=CARTESIAN_POINT('Ctrl Pts',(-37.2874279838024,38.5683990357347,5.92401517576706));
#57527=CARTESIAN_POINT('Ctrl Pts',(-37.6338153475925,39.6208332722494,5.97509183961299));
#57528=CARTESIAN_POINT('Ctrl Pts',(-37.972630261787,39.962302073481,6.));
#57529=CARTESIAN_POINT('Origin',(-39.0658530619283,38.8697713466882,0.895788276411275));
#57530=CARTESIAN_POINT('',(-39.8364823014031,40.2038876485621,5.10421172358873));
#57531=CARTESIAN_POINT('',(-39.8373456329825,40.207933543715,5.14578827641127));
#57532=CARTESIAN_POINT('',(-39.8373530619284,40.2060485447276,0.895788276411275));
#57533=CARTESIAN_POINT('Ctrl Pts',(-39.8373456329825,40.207933543715,5.14578827641127));
#57534=CARTESIAN_POINT('Ctrl Pts',(-40.2216806378635,39.9822885010755,5.16884048301825));
#57535=CARTESIAN_POINT('Ctrl Pts',(-40.8329618074793,39.1268210714738,5.21806119308415));
#57536=CARTESIAN_POINT('Ctrl Pts',(-40.3208244444739,37.5557551266231,5.29345040660899));
#57537=CARTESIAN_POINT('Ctrl Pts',(-38.6620380533448,37.0981630448849,5.37195591698576));
#57538=CARTESIAN_POINT('Ctrl Pts',(-37.3653845951193,38.2294425600612,5.45046142736254));
#57539=CARTESIAN_POINT('Ctrl Pts',(-37.5937879163964,39.9348809965236,5.52896693773932));
#57540=CARTESIAN_POINT('Ctrl Pts',(-38.8780553810739,40.5572546562641,5.59407588742223));
#57541=CARTESIAN_POINT('Ctrl Pts',(-39.6209034474226,40.3284248126315,5.63301633364622));
#57542=CARTESIAN_POINT('Ctrl Pts',(-39.8361023073888,40.2039982703455,5.64578827641127));
#57543=CARTESIAN_POINT('Ctrl Pts',(-39.8364823014031,40.2038876485621,5.10421172358873));
#57544=CARTESIAN_POINT('Ctrl Pts',(-40.0389857717083,40.0874933656255,5.11621462074954));
#57545=CARTESIAN_POINT('Ctrl Pts',(-40.6023754577107,39.5788852724494,5.15438602136929));
#57546=CARTESIAN_POINT('Ctrl Pts',(-40.7451774946681,38.1758811994982,5.21872592544796));
#57547=CARTESIAN_POINT('Ctrl Pts',(-39.4133645670745,37.0862753673933,5.29723143582474));
#57548=CARTESIAN_POINT('Ctrl Pts',(-37.7698897533292,37.5961550422892,5.37573694620152));
#57549=CARTESIAN_POINT('Ctrl Pts',(-37.2886763485593,39.2482362054987,5.4542424565783));
#57550=CARTESIAN_POINT('Ctrl Pts',(-38.3679904575111,40.521668910622,5.53040071570737));
#57551=CARTESIAN_POINT('Ctrl Pts',(-39.4389802356634,40.4350754385143,5.58039047137751));
#57552=CARTESIAN_POINT('Ctrl Pts',(-39.8389883040075,40.2073580112695,5.60421172358873));
#57553=CARTESIAN_POINT('Origin',(-39.0658530619283,38.8697713466882,0.895788276411275));
#57554=CARTESIAN_POINT('',(-39.8367681787868,40.2074507120888,4.60421172358873));
#57555=CARTESIAN_POINT('',(-39.838395191597,40.2051955164573,4.64578827641127));
#57556=CARTESIAN_POINT('',(-39.8373530619284,40.2060485447276,0.895788276411275));
#57557=CARTESIAN_POINT('Ctrl Pts',(-39.838395191597,40.2051955164573,4.64578827641127));
#57558=CARTESIAN_POINT('Ctrl Pts',(-39.9487742895753,40.1427442714185,4.65232762547243));
#57559=CARTESIAN_POINT('Ctrl Pts',(-40.461107190991,39.7640019994127,4.68503547799252));
#57560=CARTESIAN_POINT('Ctrl Pts',(-40.8515947960302,38.533999133735,4.74391183397153));
#57561=CARTESIAN_POINT('Ctrl Pts',(-39.7707737852476,37.1950466549738,4.82241734434831));
#57562=CARTESIAN_POINT('Ctrl Pts',(-38.05776324374,37.3580267168588,4.90092285472509));
#57563=CARTESIAN_POINT('Ctrl Pts',(-37.248831349992,38.8767760630727,4.97942836510187));
#57564=CARTESIAN_POINT('Ctrl Pts',(-38.0694482634705,40.3892418792306,5.05793387547865));
#57565=CARTESIAN_POINT('Ctrl Pts',(-39.280304717179,40.4950348443414,5.11338717924845));
#57566=CARTESIAN_POINT('Ctrl Pts',(-39.7853895670742,40.2384372151433,5.14267197955933));
#57567=CARTESIAN_POINT('Ctrl Pts',(-39.8373456329825,40.207933543715,5.14578827641127));
#57568=CARTESIAN_POINT('Ctrl Pts',(-39.8367681787868,40.2074507120888,4.60421172358873));
#57569=CARTESIAN_POINT('Ctrl Pts',(-40.1980237481411,39.9947173316426,4.62587026666265));
#57570=CARTESIAN_POINT('Ctrl Pts',(-40.8090940791592,39.1897699662685,4.6736973131955));
#57571=CARTESIAN_POINT('Ctrl Pts',(-40.3881021894619,37.6234670214254,4.74769286318728));
#57572=CARTESIAN_POINT('Ctrl Pts',(-38.7556268199881,37.0794146789619,4.82619837356406));
#57573=CARTESIAN_POINT('Ctrl Pts',(-37.4013696406987,38.1409968175026,4.90470388394084));
#57574=CARTESIAN_POINT('Ctrl Pts',(-37.5398609233301,39.8561611622598,4.98320939431762));
#57575=CARTESIAN_POINT('Ctrl Pts',(-38.8164833870163,40.5597236082337,5.04971200753358));
#57576=CARTESIAN_POINT('Ctrl Pts',(-39.5974912981552,40.3412541164524,5.09004611729062));
#57577=CARTESIAN_POINT('Ctrl Pts',(-39.8364823014031,40.2038876485621,5.10421172358873));
#57578=CARTESIAN_POINT('Origin',(-39.0658530619283,38.8697713466882,0.895788276411275));
#57579=CARTESIAN_POINT('',(-39.8387455558871,40.2059018946482,4.10421172358873));
#57580=CARTESIAN_POINT('',(-39.835683949911,40.2049009685562,4.14578827641127));
#57581=CARTESIAN_POINT('',(-39.8373530619284,40.2060485447276,0.895788276411275));
#57582=CARTESIAN_POINT('Ctrl Pts',(-39.835683949911,40.2049009685562,4.14578827641127));
#57583=CARTESIAN_POINT('Ctrl Pts',(-40.1075666009271,40.0460142702611,4.16198327138554));
#57584=CARTESIAN_POINT('Ctrl Pts',(-40.7000264343407,39.4199669716347,4.20434676981873));
#57585=CARTESIAN_POINT('Ctrl Pts',(-40.6150446849375,37.9202337024768,4.27287877171085));
#57586=CARTESIAN_POINT('Ctrl Pts',(-39.1283436057741,37.0538111746305,4.35138428208763));
#57587=CARTESIAN_POINT('Ctrl Pts',(-37.5855995232345,37.8159848954577,4.42988979246441));
#57588=CARTESIAN_POINT('Ctrl Pts',(-37.3703820012353,39.5232193693979,4.50839530284119));
#57589=CARTESIAN_POINT('Ctrl Pts',(-38.5669726422018,40.5510318627906,4.58036146415681));
#57590=CARTESIAN_POINT('Ctrl Pts',(-39.5070704165714,40.3926553262541,4.6261591220135));
#57591=CARTESIAN_POINT('Ctrl Pts',(-39.838395191597,40.2051955164573,4.64578827641127));
#57592=CARTESIAN_POINT('Ctrl Pts',(-39.8387455558872,40.2059018946482,4.10421172358873));
#57593=CARTESIAN_POINT('Ctrl Pts',(-39.9254936329904,40.1568361214949,4.10935740911683));
#57594=CARTESIAN_POINT('Ctrl Pts',(-40.4229804016609,39.8074510911275,4.14067159810387));
#57595=CARTESIAN_POINT('Ctrl Pts',(-40.8667641756192,38.6282419782981,4.19815429054983));
#57596=CARTESIAN_POINT('Ctrl Pts',(-39.8577505620191,37.2343767082119,4.2766598009266));
#57597=CARTESIAN_POINT('Ctrl Pts',(-38.1385444446535,37.3071722287696,4.35516531130339));
#57598=CARTESIAN_POINT('Ctrl Pts',(-37.2509707395799,38.781343787805,4.43367082168017));
#57599=CARTESIAN_POINT('Ctrl Pts',(-37.9910266499109,40.3348192821528,4.51217633205694));
#57600=CARTESIAN_POINT('Ctrl Pts',(-39.2249072234587,40.508306713049,4.5690232993598));
#57601=CARTESIAN_POINT('Ctrl Pts',(-39.7615438988762,40.2517482031576,4.59970176320373));
#57602=CARTESIAN_POINT('Ctrl Pts',(-39.8367681787868,40.2074507120888,4.60421172358873));
#57603=CARTESIAN_POINT('Origin',(-39.0658530619283,38.8697713466882,0.895788276411275));
#57604=CARTESIAN_POINT('',(-39.8358089661004,40.2043945583313,3.60421172358873));
#57605=CARTESIAN_POINT('',(-39.8384741440368,40.2082087576148,3.64578827641127));
#57606=CARTESIAN_POINT('',(-39.8373530619284,40.2060485447276,0.895788276411275));
#57607=CARTESIAN_POINT('Ctrl Pts',(-39.8384741440368,40.2082087576148,3.64578827641127));
#57608=CARTESIAN_POINT('Ctrl Pts',(-40.2704292120645,39.9582192659243,3.67163891729865));
#57609=CARTESIAN_POINT('Ctrl Pts',(-40.875250043897,38.9953053985923,3.72365806164495));
#57610=CARTESIAN_POINT('Ctrl Pts',(-40.1754790439541,37.4309014426854,3.80184570945018));
#57611=CARTESIAN_POINT('Ctrl Pts',(-38.4777242474675,37.1505503260543,3.88035121982696));
#57612=CARTESIAN_POINT('Ctrl Pts',(-37.3074173539442,38.412037492713,3.95885673020373));
#57613=CARTESIAN_POINT('Ctrl Pts',(-37.7141174076169,40.0840312618198,4.03736224058051));
#57614=CARTESIAN_POINT('Ctrl Pts',(-38.9991071509758,40.5467766825012,4.09967275598303));
#57615=CARTESIAN_POINT('Ctrl Pts',(-39.6682480272047,40.3027495838885,4.13581476792661));
#57616=CARTESIAN_POINT('Ctrl Pts',(-39.835683949911,40.2049009685562,4.14578827641127));
#57617=CARTESIAN_POINT('Ctrl Pts',(-39.8358089661004,40.2043945583313,3.60421172358873));
#57618=CARTESIAN_POINT('Ctrl Pts',(-40.0847686354211,40.0596485313516,3.61901305502994));
#57619=CARTESIAN_POINT('Ctrl Pts',(-40.6687535790882,39.4744804296355,3.65998288993008));
#57620=CARTESIAN_POINT('Ctrl Pts',(-40.662772801836,38.0029007557487,3.72712122828915));
#57621=CARTESIAN_POINT('Ctrl Pts',(-39.2236238307452,37.0595985208235,3.80562673866593));
#57622=CARTESIAN_POINT('Ctrl Pts',(-37.642982284831,37.7397023107928,3.88413224904271));
#57623=CARTESIAN_POINT('Ctrl Pts',(-37.3384050779085,39.4332788778856,3.96263775941949));
#57624=CARTESIAN_POINT('Ctrl Pts',(-38.5014637504291,40.5436066616789,4.03599758426816));
#57625=CARTESIAN_POINT('Ctrl Pts',(-39.4843342688332,40.4063612522992,4.08318890565791));
#57626=CARTESIAN_POINT('Ctrl Pts',(-39.8387455558872,40.2059018946482,4.10421172358873));
#57627=CARTESIAN_POINT('Origin',(-39.0658530619283,38.8697713466882,0.895788276411275));
#57628=CARTESIAN_POINT('',(-39.8379469994295,40.2082106520625,3.10421172358873));
#57629=CARTESIAN_POINT('',(-39.8374306108962,40.204163629121,3.14578827641127));
#57630=CARTESIAN_POINT('',(-39.8373530619284,40.2060485447276,0.895788276411275));
#57631=CARTESIAN_POINT('Ctrl Pts',(-39.8374306108962,40.204163629121,3.14578827641127));
#57632=CARTESIAN_POINT('Ctrl Pts',(-39.9951711463869,40.1143839028202,3.15512605975283));
#57633=CARTESIAN_POINT('Ctrl Pts',(-40.5352143013727,39.6721982210719,3.19063234655331));
#57634=CARTESIAN_POINT('Ctrl Pts',(-40.8063086069208,38.3478222423284,3.25230713681272));
#57635=CARTESIAN_POINT('Ctrl Pts',(-39.590501232232,37.1301274942208,3.3308126471895));
#57636=CARTESIAN_POINT('Ctrl Pts',(-37.9041768834746,37.4725867203679,3.40931815756627));
#57637=CARTESIAN_POINT('Ctrl Pts',(-37.259671359806,39.0680743307528,3.48782366794306));
#57638=CARTESIAN_POINT('Ctrl Pts',(-38.2349925206666,40.4857191130317,3.56632917831984));
#57639=CARTESIAN_POINT('Ctrl Pts',(-39.3889296125877,40.4645408708171,3.61898404780924));
#57640=CARTESIAN_POINT('Ctrl Pts',(-39.8331627728674,40.2112826582981,3.64547041383972));
#57641=CARTESIAN_POINT('Ctrl Pts',(-39.8384741440368,40.2082087576148,3.64578827641127));
#57642=CARTESIAN_POINT('Ctrl Pts',(-39.8379469994295,40.2082106520625,3.10421172358873));
#57643=CARTESIAN_POINT('Ctrl Pts',(-40.2459151473258,39.9700580402636,3.12866870094305));
#57644=CARTESIAN_POINT('Ctrl Pts',(-40.855169338561,39.0616525117032,3.1792941817563));
#57645=CARTESIAN_POINT('Ctrl Pts',(-40.249511348243,37.4911595684212,3.25608816602847));
#57646=CARTESIAN_POINT('Ctrl Pts',(-38.5688218267178,37.1220364497186,3.33459367640525));
#57647=CARTESIAN_POINT('Ctrl Pts',(-37.333881829365,38.3203235548052,3.41309918678203));
#57648=CARTESIAN_POINT('Ctrl Pts',(-37.6522147609439,40.011368493019,3.49160469715881));
#57649=CARTESIAN_POINT('Ctrl Pts',(-38.9392875485226,40.5528026028124,3.55530887609438));
#57650=CARTESIAN_POINT('Ctrl Pts',(-39.6446121539839,40.3155570570627,3.59284455157102));
#57651=CARTESIAN_POINT('Ctrl Pts',(-39.8358089661004,40.2043945583313,3.60421172358873));
#57652=CARTESIAN_POINT('Origin',(-39.0658530619283,38.8697713466882,0.895788276411275));
#57653=CARTESIAN_POINT('',(-39.8379370462828,40.204596038962,2.60421172358873));
#57654=CARTESIAN_POINT('',(-39.8359404161091,40.2062105265248,2.64578827641127));
#57655=CARTESIAN_POINT('',(-39.8373530619284,40.2060485447276,0.895788276411275));
#57656=CARTESIAN_POINT('Ctrl Pts',(-39.8359404161091,40.2062105265248,2.64578827641127));
#57657=CARTESIAN_POINT('Ctrl Pts',(-40.1535704235636,40.0192626275773,2.66478170566594));
#57658=CARTESIAN_POINT('Ctrl Pts',(-40.7587789941875,39.3053583432972,2.70994363837953));
#57659=CARTESIAN_POINT('Ctrl Pts',(-40.5064415845058,37.7623789454716,2.78127407455204));
#57660=CARTESIAN_POINT('Ctrl Pts',(-38.936770715205,37.0573269432749,2.85977958492882));
#57661=CARTESIAN_POINT('Ctrl Pts',(-37.4828624739785,37.9777188225534,2.9382850953056));
#57662=CARTESIAN_POINT('Ctrl Pts',(-37.4486185639574,39.6981242894461,3.01679060568238));
#57663=CARTESIAN_POINT('Ctrl Pts',(-38.6963080267235,40.5593729851321,3.0859583327176));
#57664=CARTESIAN_POINT('Ctrl Pts',(-39.5531140116672,40.3659854866553,3.1289575562939));
#57665=CARTESIAN_POINT('Ctrl Pts',(-39.8374306108962,40.204163629121,3.14578827641127));
#57666=CARTESIAN_POINT('Ctrl Pts',(-39.8379370462828,40.204596038962,2.60421172358873));
#57667=CARTESIAN_POINT('Ctrl Pts',(-39.9721218195358,40.1285083617881,2.61215584339723));
#57668=CARTESIAN_POINT('Ctrl Pts',(-40.4987455670004,39.7186935414776,2.64626846666466));
#57669=CARTESIAN_POINT('Ctrl Pts',(-40.8313104277201,38.439942299895,2.70654959339101));
#57670=CARTESIAN_POINT('Ctrl Pts',(-39.6811395860238,37.1600807661057,2.78505510376779));
#57671=CARTESIAN_POINT('Ctrl Pts',(-37.9791520940816,37.4135079224236,2.86356061414458));
#57672=CARTESIAN_POINT('Ctrl Pts',(-37.2517503435483,38.9729479619195,2.94206612452135));
#57673=CARTESIAN_POINT('Ctrl Pts',(-38.1512758267995,40.4398561533634,3.02057163489813));
#57674=CARTESIAN_POINT('Ctrl Pts',(-39.3352629723092,40.4803512300078,3.07462016792059));
#57675=CARTESIAN_POINT('Ctrl Pts',(-39.8093969408979,40.2248768330901,3.10250019748412));
#57676=CARTESIAN_POINT('Ctrl Pts',(-39.8379469994295,40.2082106520625,3.10421172358873));
#57677=CARTESIAN_POINT('Origin',(-39.0658530619283,38.8697713466882,0.895788276411275));
#57678=CARTESIAN_POINT('',(-39.8351916364771,40.2053827942122,2.10421172358873));
#57679=CARTESIAN_POINT('',(-39.838950903209,40.2073157943284,2.14578827641127));
#57680=CARTESIAN_POINT('',(-39.8373530619284,40.2060485447276,0.895788276411275));
#57681=CARTESIAN_POINT('',(-37.9741697098829,39.9602191716056,2.));
#57682=CARTESIAN_POINT('Ctrl Pts',(-37.9741697098829,39.9602191716056,2.));
#57683=CARTESIAN_POINT('Ctrl Pts',(-38.3327559670707,40.3192117233802,2.02616850345893));
#57684=CARTESIAN_POINT('Ctrl Pts',(-39.0582121561479,40.5387775404138,2.06090574465517));
#57685=CARTESIAN_POINT('Ctrl Pts',(-39.6915909718076,40.2896039589219,2.09564298585141));
#57686=CARTESIAN_POINT('Ctrl Pts',(-39.8351916364771,40.2053827942122,2.10421172358873));
#57687=CARTESIAN_POINT('',(-37.5730967199607,39.2702632425652,2.));
#57688=CARTESIAN_POINT('Origin',(-39.0658530619283,38.8697713466882,2.));
#57689=CARTESIAN_POINT('Ctrl Pts',(-37.5730824075077,39.2702648660737,2.));
#57690=CARTESIAN_POINT('Ctrl Pts',(-37.6993955576028,39.7344217910383,2.02490816038701));
#57691=CARTESIAN_POINT('Ctrl Pts',(-38.4017837618403,40.520493253107,2.0735042525241));
#57692=CARTESIAN_POINT('Ctrl Pts',(-39.4411667728032,40.4336532467271,2.12210034466119));
#57693=CARTESIAN_POINT('Ctrl Pts',(-39.838950903209,40.2073157943283,2.14578827641127));
#57694=CARTESIAN_POINT('Origin',(-53.1951359564886,-14.3971354987959,4.5));
#57695=CARTESIAN_POINT('',(-54.457664959728,-14.3970890371748,5.80658032638058));
#57696=CARTESIAN_POINT('',(-54.4588632108481,-14.3954785432618,5.94341967361942));
#57697=CARTESIAN_POINT('',(-54.4596359564886,-14.3971354987959,4.5));
#57698=CARTESIAN_POINT('',(-54.153252109211,-15.2223467977324,6.));
#57699=CARTESIAN_POINT('Ctrl Pts',(-54.4588632108481,-14.3954785432618,
5.94341967361942));
#57700=CARTESIAN_POINT('Ctrl Pts',(-54.4562503558692,-14.6946046444958,
5.96227978241294));
#57701=CARTESIAN_POINT('Ctrl Pts',(-54.348829759182,-14.9952702831595,5.98113989120647));
#57702=CARTESIAN_POINT('Ctrl Pts',(-54.153252109211,-15.2223467977324,6.));
#57703=CARTESIAN_POINT('',(-54.4596359564886,-14.3971354987959,6.));
#57704=CARTESIAN_POINT('Origin',(-53.1951359564886,-14.3971354987959,6.));
#57705=CARTESIAN_POINT('',(-54.4596359564886,-14.3971354987959,7.));
#57706=CARTESIAN_POINT('',(-54.4596359564886,-14.3971354987959,4.5));
#57707=CARTESIAN_POINT('',(-52.6278006430704,-15.5272199611918,7.));
#57708=CARTESIAN_POINT('Origin',(-53.1951359564886,-14.3971354987959,7.));
#57709=CARTESIAN_POINT('',(-53.7624712699068,-13.2670510364,7.));
#57710=CARTESIAN_POINT('Origin',(-53.1951359564886,-14.3971354987959,7.));
#57711=CARTESIAN_POINT('Origin',(-53.1951359564886,-14.3971354987959,7.));
#57712=CARTESIAN_POINT('',(-52.2352360662266,-15.2234730828751,6.));
#57713=CARTESIAN_POINT('Origin',(-53.1951359564886,-14.3971354987959,6.));
#57714=CARTESIAN_POINT('Ctrl Pts',(-52.2352263046383,-15.223479246524,6.));
#57715=CARTESIAN_POINT('Ctrl Pts',(-52.4934849626836,-15.5213201221341,
5.97509183961299));
#57716=CARTESIAN_POINT('Ctrl Pts',(-52.9025331767738,-15.6908484929834,
5.95018367922598));
#57717=CARTESIAN_POINT('Ctrl Pts',(-53.2954400519545,-15.6595806594193,
5.92527551883898));
#57718=CARTESIAN_POINT('Ctrl Pts',(-53.7082278597432,-15.6267306858339,
5.89910701538005));
#57719=CARTESIAN_POINT('Ctrl Pts',(-54.1031995108901,-15.3722499881178,
5.87293851192112));
#57720=CARTESIAN_POINT('Ctrl Pts',(-54.3034856243485,-15.009959026203,5.84677000846219));
#57721=CARTESIAN_POINT('Ctrl Pts',(-54.4060190030454,-14.8244897704715,
5.83337344776832));
#57722=CARTESIAN_POINT('Ctrl Pts',(-54.457529785952,-14.6107659273806,5.81997688707445));
#57723=CARTESIAN_POINT('Ctrl Pts',(-54.457664959728,-14.3970890371748,5.80658032638058));
#57724=CARTESIAN_POINT('Origin',(-53.1951359564886,-14.3971354987959,4.5));
#57725=CARTESIAN_POINT('',(-54.4609673117159,-14.396357828719,5.30658032638058));
#57726=CARTESIAN_POINT('',(-54.4612320294125,-14.3977598345137,5.44341967361941));
#57727=CARTESIAN_POINT('',(-54.4596359564886,-14.3971354987959,4.5));
#57728=CARTESIAN_POINT('Ctrl Pts',(-54.4612320294125,-14.3977598345137,
5.44341967361941));
#57729=CARTESIAN_POINT('Ctrl Pts',(-54.4614577199909,-14.4349274614079,
5.44576692486712));
#57730=CARTESIAN_POINT('Ctrl Pts',(-54.4599595944507,-14.4720765205797,
5.44811417611483));
#57731=CARTESIAN_POINT('Ctrl Pts',(-54.4566777507412,-14.5090671702315,
5.45046142736254));
#57732=CARTESIAN_POINT('Ctrl Pts',(-54.4200898743707,-14.9214601530044,
5.47662993082147));
#57733=CARTESIAN_POINT('Ctrl Pts',(-54.1618024272562,-15.3141643064504,
5.5027984342804));
#57734=CARTESIAN_POINT('Ctrl Pts',(-53.7976302145161,-15.5111328144605,
5.52896693773933));
#57735=CARTESIAN_POINT('Ctrl Pts',(-53.4334580017759,-15.7081013224707,
5.55513544119825));
#57736=CARTESIAN_POINT('Ctrl Pts',(-52.9634010234101,-15.709334185045,5.58130394465718));
#57737=CARTESIAN_POINT('Ctrl Pts',(-52.598247155701,-15.5141854678805,5.60747244811611));
#57738=CARTESIAN_POINT('Ctrl Pts',(-52.2330932879918,-15.3190367507161,
5.63364095157503));
#57739=CARTESIAN_POINT('Ctrl Pts',(-51.9728425309394,-14.9275064538129,
5.65980945503395));
#57740=CARTESIAN_POINT('Ctrl Pts',(-51.9341769083662,-14.5153483233265,
5.68597795849288));
#57741=CARTESIAN_POINT('Ctrl Pts',(-51.8955112857929,-14.1031901928401,
5.71214646195181));
#57742=CARTESIAN_POINT('Ctrl Pts',(-52.0784307976988,-13.6704042287704,
5.73831496541074));
#57743=CARTESIAN_POINT('Ctrl Pts',(-52.4009468670997,-13.4106806439539,
5.76448346886967));
#57744=CARTESIAN_POINT('Ctrl Pts',(-52.7234629365007,-13.1509570591374,
5.79065197232859));
#57745=CARTESIAN_POINT('Ctrl Pts',(-53.1855755633968,-13.0642958535739,
5.81682047578752));
#57746=CARTESIAN_POINT('Ctrl Pts',(-53.5800025789138,-13.1903251026302,
5.84298897924644));
#57747=CARTESIAN_POINT('Ctrl Pts',(-53.9744295944308,-13.3163543516866,
5.86915748270537));
#57748=CARTESIAN_POINT('Ctrl Pts',(-54.3011709985689,-13.6550740553627,
5.89532598616429));
#57749=CARTESIAN_POINT('Ctrl Pts',(-54.4137178903471,-14.0528046923317,
5.92149448962322));
#57750=CARTESIAN_POINT('Ctrl Pts',(-54.4451502229132,-14.1638837408548,
5.92880288428862));
#57751=CARTESIAN_POINT('Ctrl Pts',(-54.4598757063537,-14.2795655532322,
5.93611127895402));
#57752=CARTESIAN_POINT('Ctrl Pts',(-54.4588632108481,-14.3954785432618,
5.94341967361942));
#57753=CARTESIAN_POINT('Ctrl Pts',(-54.457664959728,-14.3970890371748,5.80658032638058));
#57754=CARTESIAN_POINT('Ctrl Pts',(-54.4577938309935,-14.1933748843943,
5.79380838361553));
#57755=CARTESIAN_POINT('Ctrl Pts',(-54.4112262077565,-13.989703408191,5.78103644085047));
#57756=CARTESIAN_POINT('Ctrl Pts',(-54.3176561881973,-13.8105991567173,
5.76826449808541));
#57757=CARTESIAN_POINT('Ctrl Pts',(-54.1259400628177,-13.4436314752601,
5.74209599462649));
#57758=CARTESIAN_POINT('Ctrl Pts',(-53.7369072362884,-13.1797973384592,
5.71592749116756));
#57759=CARTESIAN_POINT('Ctrl Pts',(-53.3250643574771,-13.1373309568652,
5.68975898770863));
#57760=CARTESIAN_POINT('Ctrl Pts',(-52.9132214786657,-13.0948645752712,
5.66359048424971));
#57761=CARTESIAN_POINT('Ctrl Pts',(-52.4785685475723,-13.2737659488842,
5.63742198079078));
#57762=CARTESIAN_POINT('Ctrl Pts',(-52.2159793451473,-13.5938495375153,
5.61125347733185));
#57763=CARTESIAN_POINT('Ctrl Pts',(-51.9533901427223,-13.9139331261463,
5.58508497387293));
#57764=CARTESIAN_POINT('Ctrl Pts',(-51.8628646689658,-14.3751989297955,
5.558916470414));
#57765=CARTESIAN_POINT('Ctrl Pts',(-51.9850104565428,-14.7707919534968,
5.53274796695507));
#57766=CARTESIAN_POINT('Ctrl Pts',(-52.1071562441199,-15.1663849771981,
5.50657946349615));
#57767=CARTESIAN_POINT('Ctrl Pts',(-52.4419732930306,-15.4963052209516,
5.48041096003722));
#57768=CARTESIAN_POINT('Ctrl Pts',(-52.8393182643656,-15.6126214609836,
5.4542424565783));
#57769=CARTESIAN_POINT('Ctrl Pts',(-53.2366632357006,-15.7289377010156,
5.42807395311937));
#57770=CARTESIAN_POINT('Ctrl Pts',(-53.69653612946,-15.6316499373263,5.40190544966044));
#57771=CARTESIAN_POINT('Ctrl Pts',(-54.0127281594173,-15.3643787057253,
5.37573694620152));
#57772=CARTESIAN_POINT('Ctrl Pts',(-54.291266212367,-15.1289356793162,5.35268473959454));
#57773=CARTESIAN_POINT('Ctrl Pts',(-54.4583064998761,-14.7615838076199,
5.32963253298756));
#57774=CARTESIAN_POINT('Ctrl Pts',(-54.4609673117159,-14.396357828719,5.30658032638058));
#57775=CARTESIAN_POINT('Origin',(-53.1951359564886,-14.3971354987959,4.5));
#57776=CARTESIAN_POINT('',(-54.4594541523146,-14.3982246410602,4.80658032638058));
#57777=CARTESIAN_POINT('',(-54.4577421278041,-14.3974029482829,4.94341967361941));
#57778=CARTESIAN_POINT('',(-54.4596359564886,-14.3971354987959,4.5));
#57779=CARTESIAN_POINT('Ctrl Pts',(-54.4577421278041,-14.3974029482829,
4.94341967361941));
#57780=CARTESIAN_POINT('Ctrl Pts',(-54.4581119948619,-14.5888150279108,
4.95542257078023));
#57781=CARTESIAN_POINT('Ctrl Pts',(-54.4171976582397,-14.7800770605195,
4.96742546794105));
#57782=CARTESIAN_POINT('Ctrl Pts',(-54.3341701782111,-14.9508661287461,
4.97942836510187));
#57783=CARTESIAN_POINT('Ctrl Pts',(-54.1531551391583,-15.3232174255002,
5.00559686856079));
#57784=CARTESIAN_POINT('Ctrl Pts',(-53.7719681306167,-15.5982567367276,
5.03176537201972));
#57785=CARTESIAN_POINT('Ctrl Pts',(-53.3615378715941,-15.6526538764831,
5.05793387547865));
#57786=CARTESIAN_POINT('Ctrl Pts',(-52.9511076125715,-15.7070510162386,
5.08410237893757));
#57787=CARTESIAN_POINT('Ctrl Pts',(-52.5114341030678,-15.5408059845222,
5.1102708823965));
#57788=CARTESIAN_POINT('Ctrl Pts',(-52.239672304957,-15.2284636038326,5.13643938585543));
#57789=CARTESIAN_POINT('Ctrl Pts',(-51.9679105068461,-14.9161212231431,
5.16260788931435));
#57790=CARTESIAN_POINT('Ctrl Pts',(-51.8640604201282,-14.4576814934805,
5.18877639277328));
#57791=CARTESIAN_POINT('Ctrl Pts',(-51.974689389455,-14.0587171002307,5.21494489623221));
#57792=CARTESIAN_POINT('Ctrl Pts',(-52.0853183587818,-13.659752706981,5.24111339969114));
#57793=CARTESIAN_POINT('Ctrl Pts',(-52.4104263841535,-13.3202636501442,
5.26728190315006));
#57794=CARTESIAN_POINT('Ctrl Pts',(-52.804231701646,-13.1924751167177,5.29345040660898));
#57795=CARTESIAN_POINT('Ctrl Pts',(-53.1980370191385,-13.0646865832913,
5.31961891006791));
#57796=CARTESIAN_POINT('Ctrl Pts',(-53.6605396287519,-13.1485985732751,
5.34578741352684));
#57797=CARTESIAN_POINT('Ctrl Pts',(-53.9843467807452,-13.406595474317,5.37195591698577));
#57798=CARTESIAN_POINT('Ctrl Pts',(-54.2791092171045,-13.6414506795096,
5.39577716919699));
#57799=CARTESIAN_POINT('Ctrl Pts',(-54.4589415919507,-14.0205614348097,
5.4195984214082));
#57800=CARTESIAN_POINT('Ctrl Pts',(-54.4612320294125,-14.3977598345137,
5.44341967361941));
#57801=CARTESIAN_POINT('Ctrl Pts',(-54.4609673117159,-14.396357828719,5.30658032638058));
#57802=CARTESIAN_POINT('Ctrl Pts',(-54.4613270117525,-14.3469850034748,
5.30346402952863));
#57803=CARTESIAN_POINT('Ctrl Pts',(-54.4586827097295,-14.2976510284966,
5.30034773267668));
#57804=CARTESIAN_POINT('Ctrl Pts',(-54.4529037631581,-14.2486870321021,
5.29723143582474));
#57805=CARTESIAN_POINT('Ctrl Pts',(-54.4043761707862,-13.8375212895923,
5.27106293236581));
#57806=CARTESIAN_POINT('Ctrl Pts',(-54.134809819887,-13.4524445040854,5.24489442890688));
#57807=CARTESIAN_POINT('Ctrl Pts',(-53.7650823822708,-13.2661285769126,
5.21872592544796));
#57808=CARTESIAN_POINT('Ctrl Pts',(-53.3953549446545,-13.0798126497399,
5.19255742198903));
#57809=CARTESIAN_POINT('Ctrl Pts',(-52.9254664203213,-13.0922575809014,
5.1663889185301));
#57810=CARTESIAN_POINT('Ctrl Pts',(-52.5661199525803,-13.2978834669457,
5.14022041507118));
#57811=CARTESIAN_POINT('Ctrl Pts',(-52.2067734848394,-13.5035093529901,
5.11405191161225));
#57812=CARTESIAN_POINT('Ctrl Pts',(-51.9579690736908,-13.9023161939173,
5.08788340815333));
#57813=CARTESIAN_POINT('Ctrl Pts',(-51.9312738021255,-14.315473986753,5.0617149046944));
#57814=CARTESIAN_POINT('Ctrl Pts',(-51.9045785305602,-14.7286317795886,
5.03554640123547));
#57815=CARTESIAN_POINT('Ctrl Pts',(-52.0999923985782,-15.1561405243328,
5.00937789777654));
#57816=CARTESIAN_POINT('Ctrl Pts',(-52.4298893914915,-15.4063003551787,
4.98320939431762));
#57817=CARTESIAN_POINT('Ctrl Pts',(-52.7597863844047,-15.6564601860247,
4.95704089085869));
#57818=CARTESIAN_POINT('Ctrl Pts',(-53.2241665022132,-15.7292711029725,
4.93087238739976));
#57819=CARTESIAN_POINT('Ctrl Pts',(-53.6147962366241,-15.5920837570553,
4.90470388394084));
#57820=CARTESIAN_POINT('Ctrl Pts',(-54.0054259710351,-15.4548964111382,
4.87853538048191));
#57821=CARTESIAN_POINT('Ctrl Pts',(-54.3223053220485,-15.107710802356,4.85236687702299));
#57822=CARTESIAN_POINT('Ctrl Pts',(-54.4233417938017,-14.706209118673,4.82619837356406));
#57823=CARTESIAN_POINT('Ctrl Pts',(-54.4485901905141,-14.6058763020728,
4.8196590245029));
#57824=CARTESIAN_POINT('Ctrl Pts',(-54.460359856649,-14.5021516119852,4.81311967544174));
#57825=CARTESIAN_POINT('Ctrl Pts',(-54.4594541523146,-14.3982246410602,
4.80658032638058));
#57826=CARTESIAN_POINT('Origin',(-53.1951359564886,-14.3971354987959,4.5));
#57827=CARTESIAN_POINT('',(-54.458134169311,-14.3964211317122,4.30658032638058));
#57828=CARTESIAN_POINT('',(-54.4603880160508,-14.3961458582298,4.44341967361942));
#57829=CARTESIAN_POINT('',(-54.4596359564886,-14.3971354987959,4.5));
#57830=CARTESIAN_POINT('Ctrl Pts',(-54.4603880160508,-14.3961458582298,
4.44341967361942));
#57831=CARTESIAN_POINT('Ctrl Pts',(-54.4574339233842,-14.7397014586706,
4.46507821669334));
#57832=CARTESIAN_POINT('Ctrl Pts',(-54.312116901092,-15.0854595650489,4.48673675976727));
#57833=CARTESIAN_POINT('Ctrl Pts',(-54.0623960097695,-15.3201070497197,
4.50839530284119));
#57834=CARTESIAN_POINT('Ctrl Pts',(-53.7606757146401,-15.6036152013657,
4.53456380630012));
#57835=CARTESIAN_POINT('Ctrl Pts',(-53.3065445684699,-15.7249218506019,
4.56073230975904));
#57836=CARTESIAN_POINT('Ctrl Pts',(-52.9036403743547,-15.6296316648431,
4.58690081321797));
#57837=CARTESIAN_POINT('Ctrl Pts',(-52.5007361802396,-15.5343414790842,
4.6130693166769));
#57838=CARTESIAN_POINT('Ctrl Pts',(-52.1490589381795,-15.2224544583304,
4.63923782013582));
#57839=CARTESIAN_POINT('Ctrl Pts',(-52.0063049058888,-14.8338244281946,
4.66540632359475));
#57840=CARTESIAN_POINT('Ctrl Pts',(-51.8635508735981,-14.4451943980587,
4.69157482705368));
#57841=CARTESIAN_POINT('Ctrl Pts',(-51.9297200510767,-13.9798213585407,
4.7177433305126));
#57842=CARTESIAN_POINT('Ctrl Pts',(-52.1751413884873,-13.6463841561873,
4.74391183397153));
#57843=CARTESIAN_POINT('Ctrl Pts',(-52.4205627258978,-13.3129469538339,
4.77008033743046));
#57844=CARTESIAN_POINT('Ctrl Pts',(-52.8452362232402,-13.111445588645,4.79624884088938));
#57845=CARTESIAN_POINT('Ctrl Pts',(-53.2587332445463,-13.1322355800464,
4.82241734434831));
#57846=CARTESIAN_POINT('Ctrl Pts',(-53.6722302658525,-13.1530255714477,
4.84858584780724));
#57847=CARTESIAN_POINT('Ctrl Pts',(-54.0745508111225,-13.3961069194393,
4.87475435126616));
#57848=CARTESIAN_POINT('Ctrl Pts',(-54.2852895489753,-13.7524792345754,
4.90092285472509));
#57849=CARTESIAN_POINT('Ctrl Pts',(-54.3993672224223,-13.9453916768054,
4.9150884610232));
#57850=CARTESIAN_POINT('Ctrl Pts',(-54.4573056172638,-14.1715018075515,
4.92925406732131));
#57851=CARTESIAN_POINT('Ctrl Pts',(-54.4577421278041,-14.3974029482829,
4.94341967361941));
#57852=CARTESIAN_POINT('Ctrl Pts',(-54.4594541523146,-14.3982246410602,
4.80658032638058));
#57853=CARTESIAN_POINT('Ctrl Pts',(-54.4567355009545,-14.0862672062605,
4.78695117198282));
#57854=CARTESIAN_POINT('Ctrl Pts',(-54.3398093025916,-13.7724871818732,
4.76732201758505));
#57855=CARTESIAN_POINT('Ctrl Pts',(-54.1304031431366,-13.5431499271195,
4.74769286318728));
#57856=CARTESIAN_POINT('Ctrl Pts',(-53.8512344282254,-13.2374101778329,
4.72152435972836));
#57857=CARTESIAN_POINT('Ctrl Pts',(-53.4077034059102,-13.0817484378433,
4.69535585626943));
#57858=CARTESIAN_POINT('Ctrl Pts',(-52.9986946517684,-13.1459652901465,
4.6691873528105));
#57859=CARTESIAN_POINT('Ctrl Pts',(-52.5896858976267,-13.2101821424497,
4.64301884935157));
#57860=CARTESIAN_POINT('Ctrl Pts',(-52.2151994116584,-13.4942775870456,
4.61685034589265));
#57861=CARTESIAN_POINT('Ctrl Pts',(-52.0431593891151,-13.8708598453683,
4.59068184243372));
#57862=CARTESIAN_POINT('Ctrl Pts',(-51.8711193665719,-14.247442103691,4.56451333897479));
#57863=CARTESIAN_POINT('Ctrl Pts',(-51.9015258074537,-14.7165111757404,
4.53834483551587));
#57864=CARTESIAN_POINT('Ctrl Pts',(-52.1207441004937,-15.0677309159732,
4.51217633205694));
#57865=CARTESIAN_POINT('Ctrl Pts',(-52.3399623935336,-15.4189506562059,
4.48600782859801));
#57866=CARTESIAN_POINT('Ctrl Pts',(-52.7479925387317,-15.6523210646219,
4.45983932513909));
#57867=CARTESIAN_POINT('Ctrl Pts',(-53.1618689696675,-15.6631960750064,
4.43367082168017));
#57868=CARTESIAN_POINT('Ctrl Pts',(-53.5757454006032,-15.6740710853908,
4.40750231822124));
#57869=CARTESIAN_POINT('Ctrl Pts',(-53.9954681172766,-15.4624506977437,
4.38133381476231));
#57870=CARTESIAN_POINT('Ctrl Pts',(-54.2328284639311,-15.1232280099042,
4.35516531130338));
#57871=CARTESIAN_POINT('Ctrl Pts',(-54.3797245073824,-14.9132920564272,
4.33897031632912));
#57872=CARTESIAN_POINT('Ctrl Pts',(-54.4567749448579,-14.6544838494259,
4.32277532135485));
#57873=CARTESIAN_POINT('Ctrl Pts',(-54.458134169311,-14.3964211317122,4.30658032638058));
#57874=CARTESIAN_POINT('Origin',(-53.1951359564886,-14.3971354987959,4.5));
#57875=CARTESIAN_POINT('',(-54.4616250374271,-14.3970459917425,3.80658032638058));
#57876=CARTESIAN_POINT('',(-54.4600990366243,-14.3981838592136,3.94341967361941));
#57877=CARTESIAN_POINT('',(-54.4596359564886,-14.3971354987959,4.5));
#57878=CARTESIAN_POINT('Ctrl Pts',(-54.4600990366243,-14.3981838592136,
3.94341967361941));
#57879=CARTESIAN_POINT('Ctrl Pts',(-54.460821703013,-14.4798548702781,3.94856535914752));
#57880=CARTESIAN_POINT('Ctrl Pts',(-54.4535723073139,-14.561398217572,3.95371104467563));
#57881=CARTESIAN_POINT('Ctrl Pts',(-54.4378783642807,-14.6412825634277,
3.95885673020373));
#57882=CARTESIAN_POINT('Ctrl Pts',(-54.3580664518923,-15.0475362626526,
3.98502523366266));
#57883=CARTESIAN_POINT('Ctrl Pts',(-54.0598570383511,-15.410883959442,4.01119373712159));
#57884=CARTESIAN_POINT('Ctrl Pts',(-53.6769707694449,-15.5683962274082,
4.03736224058052));
#57885=CARTESIAN_POINT('Ctrl Pts',(-53.2940845005388,-15.7259084953743,
4.06353074403944));
#57886=CARTESIAN_POINT('Ctrl Pts',(-52.8265213762676,-15.6775853345172,
4.08969924749837));
#57887=CARTESIAN_POINT('Ctrl Pts',(-52.4839422593842,-15.4450954247484,
4.11586775095729));
#57888=CARTESIAN_POINT('Ctrl Pts',(-52.1413631425007,-15.2126055149797,
4.14203625441622));
#57889=CARTESIAN_POINT('Ctrl Pts',(-51.9237680330049,-14.7959488562993,
4.16820475787515));
#57890=CARTESIAN_POINT('Ctrl Pts',(-51.9287291645367,-14.3819592468436,
4.19437326133407));
#57891=CARTESIAN_POINT('Ctrl Pts',(-51.9336902960684,-13.967969637388,4.220541764793));
#57892=CARTESIAN_POINT('Ctrl Pts',(-52.1612076686276,-13.5566470771571,
4.24671026825193));
#57893=CARTESIAN_POINT('Ctrl Pts',(-52.5092597878395,-13.3324334921486,
4.27287877171085));
#57894=CARTESIAN_POINT('Ctrl Pts',(-52.8573119070513,-13.1082199071402,
4.29904727516978));
#57895=CARTESIAN_POINT('Ctrl Pts',(-53.3258987729158,-13.0711152973543,
4.3252157786287));
#57896=CARTESIAN_POINT('Ctrl Pts',(-53.7049004648973,-13.2377578095269,
4.35138428208763));
#57897=CARTESIAN_POINT('Ctrl Pts',(-54.0839021568789,-13.4044003216995,
4.37755278554656));
#57898=CARTESIAN_POINT('Ctrl Pts',(-54.3733186749775,-13.7747899558306,
4.40372128900549));
#57899=CARTESIAN_POINT('Ctrl Pts',(-54.4433722119826,-14.1828395999241,
4.42988979246441));
#57900=CARTESIAN_POINT('Ctrl Pts',(-54.4554454540469,-14.2531641308192,
4.43439975284941));
#57901=CARTESIAN_POINT('Ctrl Pts',(-54.4610031470342,-14.3246072444484,
4.43890971323442));
#57902=CARTESIAN_POINT('Ctrl Pts',(-54.4603880160508,-14.3961458582298,
4.44341967361942));
#57903=CARTESIAN_POINT('Ctrl Pts',(-54.458134169311,-14.3964211317122,4.30658032638058));
#57904=CARTESIAN_POINT('Ctrl Pts',(-54.4589712326528,-14.237496062036,4.29660681789592));
#57905=CARTESIAN_POINT('Ctrl Pts',(-54.4311018285097,-14.0788537248348,
4.28663330941126));
#57906=CARTESIAN_POINT('Ctrl Pts',(-54.3731606475783,-13.9320829192412,
4.27665980092661));
#57907=CARTESIAN_POINT('Ctrl Pts',(-54.2211345079355,-13.5469855044494,
4.25049129746768));
#57908=CARTESIAN_POINT('Ctrl Pts',(-53.8620842520144,-13.2436156628976,
4.22432279400875));
#57909=CARTESIAN_POINT('Ctrl Pts',(-53.4570122824291,-13.1580080377804,
4.19815429054982));
#57910=CARTESIAN_POINT('Ctrl Pts',(-53.0519403128439,-13.0724004126631,
4.1719857870909));
#57911=CARTESIAN_POINT('Ctrl Pts',(-52.6008466295945,-13.2045550039804,
4.14581728363197));
#57912=CARTESIAN_POINT('Ctrl Pts',(-52.3060070023708,-13.4952121220022,
4.11964878017305));
#57913=CARTESIAN_POINT('Ctrl Pts',(-52.0111673751472,-13.7858692400241,
4.09348027671412));
#57914=CARTESIAN_POINT('Ctrl Pts',(-51.8725818039491,-14.2350288847506,
4.06731177325519));
#57915=CARTESIAN_POINT('Ctrl Pts',(-51.9523937062209,-14.6412825324806,
4.04114326979627));
#57916=CARTESIAN_POINT('Ctrl Pts',(-52.0322056084927,-15.0475361802107,
4.01497476633734));
#57917=CARTESIAN_POINT('Ctrl Pts',(-52.3304149842342,-15.4108838309442,
3.98880626287841));
#57918=CARTESIAN_POINT('Ctrl Pts',(-52.7133012046075,-15.5683960789447,
3.96263775941949));
#57919=CARTESIAN_POINT('Ctrl Pts',(-53.0961874249808,-15.7259083269452,
3.93646925596056));
#57920=CARTESIAN_POINT('Ctrl Pts',(-53.5637504899858,-15.6775851722127,
3.91030075250163));
#57921=CARTESIAN_POINT('Ctrl Pts',(-53.9063295634455,-15.4450952919135,
3.88413224904271));
#57922=CARTESIAN_POINT('Ctrl Pts',(-54.2447474105889,-15.2154294107524,
3.85828160815533));
#57923=CARTESIAN_POINT('Ctrl Pts',(-54.4611991270569,-14.8060436899639,
3.83243096726796));
#57924=CARTESIAN_POINT('Ctrl Pts',(-54.4616250374271,-14.3970459917425,
3.80658032638058));
#57925=CARTESIAN_POINT('Origin',(-53.1951359564886,-14.3971354987959,4.5));
#57926=CARTESIAN_POINT('',(-54.458326569365,-14.3979628849946,3.30658032638058));
#57927=CARTESIAN_POINT('',(-54.4578259861007,-14.3967173602322,3.44341967361941));
#57928=CARTESIAN_POINT('',(-54.4596359564886,-14.3971354987959,4.5));
#57929=CARTESIAN_POINT('Ctrl Pts',(-54.4578259861007,-14.3967173602322,
3.44341967361941));
#57930=CARTESIAN_POINT('Ctrl Pts',(-54.4571098189797,-14.6327171768276,
3.45822100506063));
#57931=CARTESIAN_POINT('Ctrl Pts',(-54.3935213986439,-14.8690753747194,
3.47302233650184));
#57932=CARTESIAN_POINT('Ctrl Pts',(-54.2695279486697,-15.0677310009766,
3.48782366794306));
#57933=CARTESIAN_POINT('Ctrl Pts',(-54.0503096278436,-15.4189507857301,
3.51399217140198));
#57934=CARTESIAN_POINT('Ctrl Pts',(-53.6422794309233,-15.6523212237234,
3.54016067486091));
#57935=CARTESIAN_POINT('Ctrl Pts',(-53.228402947526,-15.6631962354854,3.56632917831984));
#57936=CARTESIAN_POINT('Ctrl Pts',(-52.8145264641287,-15.6740712472475,
3.59249768177877));
#57937=CARTESIAN_POINT('Ctrl Pts',(-52.3948036942543,-15.4624508327782,
3.61866618523769));
#57938=CARTESIAN_POINT('Ctrl Pts',(-52.1574433175134,-15.1232281019409,
3.64483468869661));
#57939=CARTESIAN_POINT('Ctrl Pts',(-51.9200829407725,-14.7840053711036,
3.67100319215554));
#57940=CARTESIAN_POINT('Ctrl Pts',(-51.865084957165,-14.3171803238982,3.69717169561447));
#57941=CARTESIAN_POINT('Ctrl Pts',(-52.0171111160778,-13.932082860293,3.7233401990734));
#57942=CARTESIAN_POINT('Ctrl Pts',(-52.1691372749906,-13.5469853966878,
3.74950870253232));
#57943=CARTESIAN_POINT('Ctrl Pts',(-52.5281875764236,-13.2436155166828,
3.77567720599125));
#57944=CARTESIAN_POINT('Ctrl Pts',(-52.933259597354,-13.1580078807144,3.80184570945017));
#57945=CARTESIAN_POINT('Ctrl Pts',(-53.3383316182844,-13.072400244746,3.8280142129091));
#57946=CARTESIAN_POINT('Ctrl Pts',(-53.7894253587122,-13.2045548528142,
3.85418271636803));
#57947=CARTESIAN_POINT('Ctrl Pts',(-54.0842650233083,-13.4952120076785,
3.88035121982696));
#57948=CARTESIAN_POINT('Ctrl Pts',(-54.3211284189289,-13.7287153280572,
3.90137403775778));
#57949=CARTESIAN_POINT('Ctrl Pts',(-54.4571465662818,-14.0645150435707,
3.9223968556886));
#57950=CARTESIAN_POINT('Ctrl Pts',(-54.4600990366243,-14.3981838592136,
3.94341967361941));
#57951=CARTESIAN_POINT('Ctrl Pts',(-54.4616250374271,-14.3970459917425,
3.80658032638058));
#57952=CARTESIAN_POINT('Ctrl Pts',(-54.4616302744719,-14.3920169071375,
3.80626246380903));
#57953=CARTESIAN_POINT('Ctrl Pts',(-54.4616028495907,-14.3869878811994,
3.80594460123748));
#57954=CARTESIAN_POINT('Ctrl Pts',(-54.4615425879167,-14.3819592487679,
3.80562673866593));
#57955=CARTESIAN_POINT('Ctrl Pts',(-54.4565814570138,-13.9679696917871,
3.779458235207));
#57956=CARTESIAN_POINT('Ctrl Pts',(-54.2290641132938,-13.5566471836914,
3.75328973174807));
#57957=CARTESIAN_POINT('Ctrl Pts',(-53.8810120381994,-13.3324336271042,
3.72712122828915));
#57958=CARTESIAN_POINT('Ctrl Pts',(-53.532959963105,-13.1082200705171,3.70095272483022));
#57959=CARTESIAN_POINT('Ctrl Pts',(-53.0643731566361,-13.0711154654387,
3.67478422137129));
#57960=CARTESIAN_POINT('Ctrl Pts',(-52.6853715126953,-13.2377579564864,
3.64861571791237));
#57961=CARTESIAN_POINT('Ctrl Pts',(-52.3063698687544,-13.4044004475342,
3.62244721445344));
#57962=CARTESIAN_POINT('Ctrl Pts',(-52.0169533873414,-13.7747900347082,
3.59627871099452));
#57963=CARTESIAN_POINT('Ctrl Pts',(-51.9468998592157,-14.182839627083,3.57011020753559));
#57964=CARTESIAN_POINT('Ctrl Pts',(-51.87684633109,-14.5908892194578,3.54394170407666));
#57965=CARTESIAN_POINT('Ctrl Pts',(-52.0261557562516,-15.0365988170333,
3.51777320061773));
#57966=CARTESIAN_POINT('Ctrl Pts',(-52.327876013137,-15.3201069327361,3.49160469715881));
#57967=CARTESIAN_POINT('Ctrl Pts',(-52.6295962700224,-15.6036150484389,
3.46543619369988));
#57968=CARTESIAN_POINT('Ctrl Pts',(-53.0837273586317,-15.7249216822689,
3.43926769024096));
#57969=CARTESIAN_POINT('Ctrl Pts',(-53.4866315016752,-15.6296315086021,
3.41309918678203));
#57970=CARTESIAN_POINT('Ctrl Pts',(-53.8895356447186,-15.5343413349353,
3.38693068332311));
#57971=CARTESIAN_POINT('Ctrl Pts',(-54.2412128421963,-15.2224543537718,
3.36076217986418));
#57972=CARTESIAN_POINT('Ctrl Pts',(-54.3839668563951,-14.8338243728713,
3.33459367640525));
#57973=CARTESIAN_POINT('Ctrl Pts',(-54.4349061872521,-14.6951484043591,
3.32525589306369));
#57974=CARTESIAN_POINT('Ctrl Pts',(-54.4592433859174,-14.5467007705307,
3.31591810972214));
#57975=CARTESIAN_POINT('Ctrl Pts',(-54.458326569365,-14.3979628849946,3.30658032638058));
#57976=CARTESIAN_POINT('Origin',(-53.1951359564886,-14.3971354987959,4.5));
#57977=CARTESIAN_POINT('',(-54.4591686783466,-14.3960664985434,2.80658032638058));
#57978=CARTESIAN_POINT('',(-54.4614103817624,-14.3966710984295,2.94341967361941));
#57979=CARTESIAN_POINT('',(-54.4596359564886,-14.3971354987959,4.5));
#57980=CARTESIAN_POINT('Ctrl Pts',(-54.4614103817624,-14.3966710984295,
2.94341967361941));
#57981=CARTESIAN_POINT('Ctrl Pts',(-54.4595565487343,-14.7837947911815,
2.96787665097374));
#57982=CARTESIAN_POINT('Ctrl Pts',(-54.2687030511239,-15.172502088678,2.99233362832806));
#57983=CARTESIAN_POINT('Ctrl Pts',(-53.9603826185353,-15.4063004831901,
3.01679060568238));
#57984=CARTESIAN_POINT('Ctrl Pts',(-53.6304855838459,-15.6564603458274,
3.04295910914131));
#57985=CARTESIAN_POINT('Ctrl Pts',(-53.1661054070793,-15.729271271822,3.06912761260023));
#57986=CARTESIAN_POINT('Ctrl Pts',(-52.7754756231319,-15.5920839084722,
3.09529611605916));
#57987=CARTESIAN_POINT('Ctrl Pts',(-52.3848458391845,-15.4548965451224,
3.12146461951809));
#57988=CARTESIAN_POINT('Ctrl Pts',(-52.0679664480565,-15.1077108924282,
3.14763312297701));
#57989=CARTESIAN_POINT('Ctrl Pts',(-51.9669299635083,-14.7062091578755,
3.17380162643594));
#57990=CARTESIAN_POINT('Ctrl Pts',(-51.8658934789602,-14.3047074233228,
3.19997012989487));
#57991=CARTESIAN_POINT('Ctrl Pts',(-51.980699900992,-13.8488896069116,3.22613863335379));
#57992=CARTESIAN_POINT('Ctrl Pts',(-52.2598686512828,-13.5431498188588,
3.25230713681272));
#57993=CARTESIAN_POINT('Ctrl Pts',(-52.5390374015737,-13.237410030806,3.27847564027165));
#57994=CARTESIAN_POINT('Ctrl Pts',(-52.9825684801236,-13.0817482711116,
3.30464414373057));
#57995=CARTESIAN_POINT('Ctrl Pts',(-53.3915772861129,-13.1459651315609,
3.3308126471895));
#57996=CARTESIAN_POINT('Ctrl Pts',(-53.8005860921022,-13.2101819920102,
3.35698115064842));
#57997=CARTESIAN_POINT('Ctrl Pts',(-54.1750726255309,-13.4942774726031,
3.38314965410735));
#57998=CARTESIAN_POINT('Ctrl Pts',(-54.3471126698793,-13.8708597786564,
3.40931815756628));
#57999=CARTESIAN_POINT('Ctrl Pts',(-54.4218440652422,-14.0344410036375,
3.42068532958399));
#58000=CARTESIAN_POINT('Ctrl Pts',(-54.4583759903277,-14.2154734956486,
3.4320525016017));
#58001=CARTESIAN_POINT('Ctrl Pts',(-54.4578259861007,-14.3967173602322,
3.44341967361941));
#58002=CARTESIAN_POINT('Ctrl Pts',(-54.458326569365,-14.3979628849946,3.30658032638058));
#58003=CARTESIAN_POINT('Ctrl Pts',(-54.4566740698126,-14.1298729507199,
3.28974960626321));
#58004=CARTESIAN_POINT('Ctrl Pts',(-54.3729773016518,-13.8608400579149,
3.27291888614584));
#58005=CARTESIAN_POINT('Ctrl Pts',(-54.2151303952057,-13.6463842512931,
3.25608816602847));
#58006=CARTESIAN_POINT('Ctrl Pts',(-53.9697090888974,-13.3129470912529,
3.22991966256955));
#58007=CARTESIAN_POINT('Ctrl Pts',(-53.5450356453608,-13.1114457518099,
3.20375115911062));
#58008=CARTESIAN_POINT('Ctrl Pts',(-53.1315386764808,-13.1322357404855,
3.17758265565169));
#58009=CARTESIAN_POINT('Ctrl Pts',(-52.7180417076007,-13.153025729161,3.15141415219276));
#58010=CARTESIAN_POINT('Ctrl Pts',(-52.3157212133773,-13.396107045955,3.12524564873384));
#58011=CARTESIAN_POINT('Ctrl Pts',(-52.1049825022091,-13.7524793160883,
3.09907714527491));
#58012=CARTESIAN_POINT('Ctrl Pts',(-51.8942437910409,-14.1088515862216,
3.07290864181599));
#58013=CARTESIAN_POINT('Ctrl Pts',(-51.8750868629279,-14.5785148096942,
3.04674013835706));
#58014=CARTESIAN_POINT('Ctrl Pts',(-52.0561018790939,-14.9508660589359,
3.02057163489813));
#58015=CARTESIAN_POINT('Ctrl Pts',(-52.2371168952598,-15.3232173081776,
2.99440313143921));
#58016=CARTESIAN_POINT('Ctrl Pts',(-52.6183038557047,-15.5982565831885,
2.96823462798028));
#58017=CARTESIAN_POINT('Ctrl Pts',(-53.0287340625826,-15.6526537166303,
2.94206612452135));
#58018=CARTESIAN_POINT('Ctrl Pts',(-53.4391642694604,-15.7070508500722,
2.91589762106243));
#58019=CARTESIAN_POINT('Ctrl Pts',(-53.8788377227712,-15.5408058419451,
2.8897291176035));
#58020=CARTESIAN_POINT('Ctrl Pts',(-54.150599486686,-15.2284634997803,2.86356061414457));
#58021=CARTESIAN_POINT('Ctrl Pts',(-54.3478475962364,-15.0017614956533,
2.84456718488991));
#58022=CARTESIAN_POINT('Ctrl Pts',(-54.4566391704649,-14.6980948440071,
2.82557375563525));
#58023=CARTESIAN_POINT('Ctrl Pts',(-54.4591686783466,-14.3960664985434,
2.80658032638058));
#58024=CARTESIAN_POINT('Origin',(-53.1951359564886,-14.3971354987959,4.5));
#58025=CARTESIAN_POINT('',(-54.4611870990995,-14.3977489718831,2.30658032638058));
#58026=CARTESIAN_POINT('',(-54.4588409672492,-14.3981450852038,2.44341967361942));
#58027=CARTESIAN_POINT('',(-54.4596359564886,-14.3971354987959,4.5));
#58028=CARTESIAN_POINT('',(-52.2370198037663,-15.2223467977324,2.));
#58029=CARTESIAN_POINT('Ctrl Pts',(-54.4611870990995,-14.3977489718831,
2.30658032638058));
#58030=CARTESIAN_POINT('Ctrl Pts',(-54.4588273697935,-14.0226957918939,
2.2828923946305));
#58031=CARTESIAN_POINT('Ctrl Pts',(-54.2812687919142,-13.6457847405029,
2.25920446288042));
#58032=CARTESIAN_POINT('Ctrl Pts',(-53.9893248675415,-13.4106809034345,
2.23551653113034));
#58033=CARTESIAN_POINT('Ctrl Pts',(-53.6668089267087,-13.1509572754522,
2.20934802767141));
#58034=CARTESIAN_POINT('Ctrl Pts',(-53.2046966949687,-13.064295685136,2.18317952421249));
#58035=CARTESIAN_POINT('Ctrl Pts',(-52.8102694972366,-13.190325107422,2.15701102075356));
#58036=CARTESIAN_POINT('Ctrl Pts',(-52.4158422995045,-13.316354529708,2.13084251729463));
#58037=CARTESIAN_POINT('Ctrl Pts',(-52.0891001357801,-13.6550749645962,
2.10467401383571));
#58038=CARTESIAN_POINT('Ctrl Pts',(-51.9765532487624,-14.05280555706,2.07850551037678));
#58039=CARTESIAN_POINT('Ctrl Pts',(-51.8640063617447,-14.4505361495237,
2.05233700691785));
#58040=CARTESIAN_POINT('Ctrl Pts',(-51.9656547514336,-14.9072768995629,
2.02616850345893));
#58041=CARTESIAN_POINT('Ctrl Pts',(-52.2370198037663,-15.2223467977324,
2.));
#58042=CARTESIAN_POINT('',(-54.1550359790162,-15.2234729584201,2.));
#58043=CARTESIAN_POINT('Origin',(-53.1951359564886,-14.3971354987959,2.));
#58044=CARTESIAN_POINT('Ctrl Pts',(-54.1550457523822,-15.2234791283661,
2.));
#58045=CARTESIAN_POINT('Ctrl Pts',(-53.8967871302308,-15.5213198394326,
2.02490816038701));
#58046=CARTESIAN_POINT('Ctrl Pts',(-53.4877388130256,-15.6908487049404,
2.04981632077402));
#58047=CARTESIAN_POINT('Ctrl Pts',(-53.0948318598941,-15.6595809742728,
2.07472448116103));
#58048=CARTESIAN_POINT('Ctrl Pts',(-52.6820439702103,-15.6267311087904,
2.10089298461995));
#58049=CARTESIAN_POINT('Ctrl Pts',(-52.2870722649439,-15.3722500867662,
2.12706148807888));
#58050=CARTESIAN_POINT('Ctrl Pts',(-52.0867861333632,-15.0099590154002,
2.15322999153781));
#58051=CARTESIAN_POINT('Ctrl Pts',(-51.8865000017826,-14.6476679440343,
2.17939849499673));
#58052=CARTESIAN_POINT('Ctrl Pts',(-51.8808994438879,-14.1775668233264,
2.20556699845566));
#58053=CARTESIAN_POINT('Ctrl Pts',(-52.0726155940678,-13.8105991317322,
2.23173550191459));
#58054=CARTESIAN_POINT('Ctrl Pts',(-52.2643317442477,-13.4436314401379,
2.25790400537351));
#58055=CARTESIAN_POINT('Ctrl Pts',(-52.6533646025024,-13.1797971776571,
2.28407250883244));
#58056=CARTESIAN_POINT('Ctrl Pts',(-53.065207531184,-13.1373307700534,2.31024101229137));
#58057=CARTESIAN_POINT('Ctrl Pts',(-53.4770504598656,-13.0948643624498,
2.33640951575029));
#58058=CARTESIAN_POINT('Ctrl Pts',(-53.9117034589741,-13.2737658097233,
2.36257801920922));
#58059=CARTESIAN_POINT('Ctrl Pts',(-54.1742926968884,-13.5938494504631,
2.38874652266814));
#58060=CARTESIAN_POINT('Ctrl Pts',(-54.3571662426276,-13.8167634997217,
2.40697090631857));
#58061=CARTESIAN_POINT('Ctrl Pts',(-54.456587675354,-14.108151888276,2.42519528996899));
#58062=CARTESIAN_POINT('Ctrl Pts',(-54.4588409672492,-14.3981450852038,
2.44341967361942));
#58063=CARTESIAN_POINT('Origin',(-53.1951359564886,-14.3971354987959,0.895788276411275));
#58064=CARTESIAN_POINT('',(-54.7400835567429,-14.3978973414314,5.60421172358873));
#58065=CARTESIAN_POINT('',(-54.7357308572386,-14.3970788042278,5.64578827641128));
#58066=CARTESIAN_POINT('',(-54.7381359564886,-14.3971354987959,0.895788276411275));
#58067=CARTESIAN_POINT('',(-52.7966221146314,-12.9064860705774,6.));
#58068=CARTESIAN_POINT('Ctrl Pts',(-54.7357308572386,-14.3970788042278,
5.64578827641128));
#58069=CARTESIAN_POINT('Ctrl Pts',(-54.7355659120932,-14.6578169944908,
5.65918483710515));
#58070=CARTESIAN_POINT('Ctrl Pts',(-54.5499292284113,-15.4280437939379,
5.69874990125794));
#58071=CARTESIAN_POINT('Ctrl Pts',(-53.3392716219708,-16.2080719085829,
5.76448346886966));
#58072=CARTESIAN_POINT('Ctrl Pts',(-51.7629444164752,-15.5169955192796,
5.84298897924644));
#58073=CARTESIAN_POINT('Ctrl Pts',(-51.4734277108623,-13.8186461670281,
5.92149448962322));
#58074=CARTESIAN_POINT('Ctrl Pts',(-52.3064323164313,-13.0375346028627,
5.97383149654107));
#58075=CARTESIAN_POINT('Ctrl Pts',(-52.7966221146314,-12.9064860705774,
6.));
#58076=CARTESIAN_POINT('',(-53.5946738441133,-12.904124289093,6.));
#58077=CARTESIAN_POINT('Origin',(-53.1951359564886,-14.3971354987959,6.));
#58078=CARTESIAN_POINT('Ctrl Pts',(-54.7400835567429,-14.3978973414314,
5.60421172358873));
#58079=CARTESIAN_POINT('Ctrl Pts',(-54.740358954578,-14.4432509581161,5.60655897483644));
#58080=CARTESIAN_POINT('Ctrl Pts',(-54.7181503847516,-14.9939574593074,
5.63507472954307));
#58081=CARTESIAN_POINT('Ctrl Pts',(-54.0595320288467,-15.9953308004788,
5.68975898770864));
#58082=CARTESIAN_POINT('Ctrl Pts',(-52.3387777758965,-15.9998439842325,
5.76826449808541));
#58083=CARTESIAN_POINT('Ctrl Pts',(-51.386068598834,-14.5665551393412,5.8467700084622));
#58084=CARTESIAN_POINT('Ctrl Pts',(-52.0449383322286,-13.007675117235,5.92401517576705));
#58085=CARTESIAN_POINT('Ctrl Pts',(-53.1295481846289,-12.781420423434,5.97509183961299));
#58086=CARTESIAN_POINT('Ctrl Pts',(-53.5946794545979,-12.9041113494969,
6.));
#58087=CARTESIAN_POINT('Origin',(-53.1951359564886,-14.3971354987959,0.895788276411275));
#58088=CARTESIAN_POINT('',(-54.7358250212096,-14.397461852737,5.10421172358873));
#58089=CARTESIAN_POINT('',(-54.7397605362559,-14.3961865506515,5.14578827641127));
#58090=CARTESIAN_POINT('',(-54.7381359564886,-14.3971354987959,0.895788276411275));
#58091=CARTESIAN_POINT('Ctrl Pts',(-54.7397605362559,-14.3961865506515,
5.14578827641127));
#58092=CARTESIAN_POINT('Ctrl Pts',(-54.7365136934968,-14.8418517823194,
5.16884048301825));
#58093=CARTESIAN_POINT('Ctrl Pts',(-54.3012988565586,-15.7989681003252,
5.21806119308415));
#58094=CARTESIAN_POINT('Ctrl Pts',(-52.6846517467245,-16.1409756074536,
5.29345040660899));
#58095=CARTESIAN_POINT('Ctrl Pts',(-51.4589751002972,-14.933224869348,5.37195591698576));
#58096=CARTESIAN_POINT('Ctrl Pts',(-51.7903649128864,-13.2446527814935,
5.45046142736255));
#58097=CARTESIAN_POINT('Ctrl Pts',(-53.3815143142557,-12.5897421777335,
5.52896693773931));
#58098=CARTESIAN_POINT('Ctrl Pts',(-54.5626373610633,-13.3907557638884,
5.59407588742224));
#58099=CARTESIAN_POINT('Ctrl Pts',(-54.7358881117761,-14.1484975960505,
5.63301633364622));
#58100=CARTESIAN_POINT('Ctrl Pts',(-54.7357308572386,-14.3970788042278,
5.64578827641128));
#58101=CARTESIAN_POINT('Ctrl Pts',(-54.7358250212096,-14.397461852737,5.10421172358873));
#58102=CARTESIAN_POINT('Ctrl Pts',(-54.7362763496954,-14.6310315157388,
5.11621462074955));
#58103=CARTESIAN_POINT('Ctrl Pts',(-54.5775040932279,-15.3732433417349,
5.15438602136928));
#58104=CARTESIAN_POINT('Ctrl Pts',(-53.4338710221273,-16.1984132586634,
5.21872592544796));
#58105=CARTESIAN_POINT('Ctrl Pts',(-51.8243426112988,-15.5898341745865,
5.29723143582474));
#58106=CARTESIAN_POINT('Ctrl Pts',(-51.4441749154368,-13.9116075960113,
5.37573694620152));
#58107=CARTESIAN_POINT('Ctrl Pts',(-52.6343093950298,-12.6688279644592,
5.45424245657829));
#58108=CARTESIAN_POINT('Ctrl Pts',(-54.2767867908486,-12.9668231409662,
5.53040071570738));
#58109=CARTESIAN_POINT('Ctrl Pts',(-54.7372886615245,-13.9376228212707,
5.58039047137751));
#58110=CARTESIAN_POINT('Ctrl Pts',(-54.7400835567429,-14.3978973414314,
5.60421172358873));
#58111=CARTESIAN_POINT('Origin',(-53.1951359564886,-14.3971354987959,0.895788276411275));
#58112=CARTESIAN_POINT('',(-54.7390536535266,-14.3959278946888,4.60421172358873));
#58113=CARTESIAN_POINT('',(-54.7379141108259,-14.3984645193683,4.64578827641127));
#58114=CARTESIAN_POINT('',(-54.7381359564886,-14.3971354987959,0.895788276411275));
#58115=CARTESIAN_POINT('Ctrl Pts',(-54.7379141108259,-14.3984645193683,
4.64578827641127));
#58116=CARTESIAN_POINT('Ctrl Pts',(-54.7390192921529,-14.5252809022368,
4.65232762547243));
#58117=CARTESIAN_POINT('Ctrl Pts',(-54.6671855077626,-15.158343636416,4.68503547799252));
#58118=CARTESIAN_POINT('Ctrl Pts',(-53.7972179286764,-16.1115146859015,
4.74391183397153));
#58119=CARTESIAN_POINT('Ctrl Pts',(-52.0972451605187,-15.8449731797319,
4.8224173443483));
#58120=CARTESIAN_POINT('Ctrl Pts',(-51.3818866828157,-14.2799767547255,
4.90092285472509));
#58121=CARTESIAN_POINT('Ctrl Pts',(-52.2926938154427,-12.820050407037,4.97942836510186));
#58122=CARTESIAN_POINT('Ctrl Pts',(-54.0128314027411,-12.7744928061304,
5.05793387547865));
#58123=CARTESIAN_POINT('Ctrl Pts',(-54.7098771965036,-13.7702259631725,
5.11338717924845));
#58124=CARTESIAN_POINT('Ctrl Pts',(-54.7401994584832,-14.3359395997999,
5.14267197955932));
#58125=CARTESIAN_POINT('Ctrl Pts',(-54.7397605362559,-14.3961865506515,
5.14578827641127));
#58126=CARTESIAN_POINT('Ctrl Pts',(-54.7390536535266,-14.3959278946888,
4.60421172358873));
#58127=CARTESIAN_POINT('Ctrl Pts',(-54.7354489362591,-14.815149952008,4.62587026666265));
#58128=CARTESIAN_POINT('Ctrl Pts',(-54.3438802932755,-15.7468235466057,
4.6736973131955));
#58129=CARTESIAN_POINT('Ctrl Pts',(-52.7769304442279,-16.1653842141838,
4.74769286318728));
#58130=CARTESIAN_POINT('Ctrl Pts',(-51.4895330907316,-15.0236483351254,
4.82619837356406));
#58131=CARTESIAN_POINT('Ctrl Pts',(-51.7317609456535,-13.3200407432483,
4.90470388394085));
#58132=CARTESIAN_POINT('Ctrl Pts',(-53.2863782799341,-12.5823975487372,
4.98320939431761));
#58133=CARTESIAN_POINT('Ctrl Pts',(-54.5339890873504,-13.3362017488983,
5.04971200753359));
#58134=CARTESIAN_POINT('Ctrl Pts',(-54.7352923713373,-14.1218070799821,
5.09004611729062));
#58135=CARTESIAN_POINT('Ctrl Pts',(-54.7358250212096,-14.397461852737,5.10421172358873));
#58136=CARTESIAN_POINT('Origin',(-53.1951359564886,-14.3971354987959,0.895788276411275));
#58137=CARTESIAN_POINT('',(-54.7387010277811,-14.3984147555176,4.10421172358873));
#58138=CARTESIAN_POINT('',(-54.7363034079594,-14.3962637958223,4.14578827641127));
#58139=CARTESIAN_POINT('',(-54.7381359564886,-14.3971354987959,0.895788276411275));
#58140=CARTESIAN_POINT('Ctrl Pts',(-54.7363034079594,-14.3962637958223,
4.14578827641127));
#58141=CARTESIAN_POINT('Ctrl Pts',(-54.7346448209045,-14.7111635771051,
4.16198327138554));
#58142=CARTESIAN_POINT('Ctrl Pts',(-54.488702537285,-15.5372702616991,4.20434676981873));
#58143=CARTESIAN_POINT('Ctrl Pts',(-53.147408175106,-16.2135387160798,4.27287877171085));
#58144=CARTESIAN_POINT('Ctrl Pts',(-51.6537177503358,-15.3592313846778,
4.35138428208763));
#58145=CARTESIAN_POINT('Ctrl Pts',(-51.5424078137269,-13.6420935954197,
4.42988979246441));
#58146=CARTESIAN_POINT('Ctrl Pts',(-52.9133037754093,-12.6020953249298,
4.50839530284119));
#58147=CARTESIAN_POINT('Ctrl Pts',(-54.4017068046157,-13.124465562129,4.58036146415681));
#58148=CARTESIAN_POINT('Ctrl Pts',(-54.7345966896724,-14.0177999706171,
4.62615912201351));
#58149=CARTESIAN_POINT('Ctrl Pts',(-54.7379141108259,-14.3984645193683,
4.64578827641127));
#58150=CARTESIAN_POINT('Ctrl Pts',(-54.7387010277811,-14.3984147555176,
4.10421172358873));
#58151=CARTESIAN_POINT('Ctrl Pts',(-54.7395828579414,-14.49807341117,4.10935740911683));
#58152=CARTESIAN_POINT('Ctrl Pts',(-54.6857500758113,-15.1036004690399,
4.14067159810387));
#58153=CARTESIAN_POINT('Ctrl Pts',(-53.8864190756817,-16.0775304145121,
4.19815429054983));
#58154=CARTESIAN_POINT('Ctrl Pts',(-52.1747941628695,-15.9006321056092,
4.2766598009266));
#58155=CARTESIAN_POINT('Ctrl Pts',(-51.3782360277521,-14.3753622969642,
4.35516531130339));
#58156=CARTESIAN_POINT('Ctrl Pts',(-52.2111169431944,-12.8696192117061,
4.43367082168016));
#58157=CARTESIAN_POINT('Ctrl Pts',(-53.9264895031678,-12.7337890506155,
4.51217633205695));
#58158=CARTESIAN_POINT('Ctrl Pts',(-54.6936722382488,-13.7156146023329,
4.5690232993598));
#58159=CARTESIAN_POINT('Ctrl Pts',(-54.7398042641295,-14.3086332477416,
4.59970176320373));
#58160=CARTESIAN_POINT('Ctrl Pts',(-54.7390536535266,-14.3959278946888,
4.60421172358873));
#58161=CARTESIAN_POINT('Origin',(-53.1951359564886,-14.3971354987959,0.895788276411275));
#58162=CARTESIAN_POINT('',(-54.7359273488899,-14.3966252672389,3.60421172358873));
#58163=CARTESIAN_POINT('',(-54.740563122869,-14.3970262782475,3.64578827641127));
#58164=CARTESIAN_POINT('',(-54.7381359564886,-14.3971354987959,0.895788276411275));
#58165=CARTESIAN_POINT('Ctrl Pts',(-54.740563122869,-14.3970262782475,3.64578827641127));
#58166=CARTESIAN_POINT('Ctrl Pts',(-54.7400434078029,-14.8961037383943,
3.67163891729865));
#58167=CARTESIAN_POINT('Ctrl Pts',(-54.208547388428,-15.9013481621327,3.72365806164495));
#58168=CARTESIAN_POINT('Ctrl Pts',(-52.5038529249194,-16.0775302015137,
3.80184570945018));
#58169=CARTESIAN_POINT('Ctrl Pts',(-51.4121872860838,-14.7474105690538,
3.88035121982695));
#58170=CARTESIAN_POINT('Ctrl Pts',(-51.9195124019995,-13.1031559265556,
3.95885673020374));
#58171=CARTESIAN_POINT('Ctrl Pts',(-53.5708470479161,-12.6193729267869,
4.03736224058051));
#58172=CARTESIAN_POINT('Ctrl Pts',(-54.6140883917719,-13.5008315971724,
4.09967275598302));
#58173=CARTESIAN_POINT('Ctrl Pts',(-54.7373248304478,-14.202336249353,4.13581476792661));
#58174=CARTESIAN_POINT('Ctrl Pts',(-54.7363034079594,-14.3962637958223,
4.14578827641127));
#58175=CARTESIAN_POINT('Ctrl Pts',(-54.7359273488899,-14.3966252672389,
3.60421172358873));
#58176=CARTESIAN_POINT('Ctrl Pts',(-54.7350534494295,-14.6846029003008,
3.61901305502994));
#58177=CARTESIAN_POINT('Ctrl Pts',(-54.5202760602344,-15.482930589367,3.65998288993008));
#58178=CARTESIAN_POINT('Ctrl Pts',(-53.2428637439183,-16.2135389463141,
3.72712122828915));
#58179=CARTESIAN_POINT('Ctrl Pts',(-51.7063697132749,-15.4388525891942,
3.80562673866593));
#58180=CARTESIAN_POINT('Ctrl Pts',(-51.5050366439836,-13.7299295812751,
3.88413224904271));
#58181=CARTESIAN_POINT('Ctrl Pts',(-52.8194248174382,-12.6193727014466,
3.96263775941949));
#58182=CARTESIAN_POINT('Ctrl Pts',(-54.3625220492744,-13.0714459438974,
4.03599758426816));
#58183=CARTESIAN_POINT('Ctrl Pts',(-54.7350982901468,-13.9912569994582,
4.0831889056579));
#58184=CARTESIAN_POINT('Ctrl Pts',(-54.7387010277811,-14.3984147555176,
4.10421172358873));
#58185=CARTESIAN_POINT('Origin',(-53.1951359564886,-14.3971354987959,0.895788276411275));
#58186=CARTESIAN_POINT('',(-54.740301190334,-14.3965688164983,3.10421172358873));
#58187=CARTESIAN_POINT('',(-54.7365381831935,-14.3981451127971,3.14578827641127));
#58188=CARTESIAN_POINT('',(-54.7381359564886,-14.3971354987959,0.895788276411275));
#58189=CARTESIAN_POINT('Ctrl Pts',(-54.7365381831935,-14.3981451127971,
3.14578827641127));
#58190=CARTESIAN_POINT('Ctrl Pts',(-54.7376569241507,-14.5796417971643,
3.15512605975283));
#58191=CARTESIAN_POINT('Ctrl Pts',(-54.6247347728585,-15.2684238709215,
3.19063234655331));
#58192=CARTESIAN_POINT('Ctrl Pts',(-53.6133414157459,-16.165383989977,3.25230713681272));
#58193=CARTESIAN_POINT('Ctrl Pts',(-51.9508876322962,-15.7213124929433,
3.3308126471895));
#58194=CARTESIAN_POINT('Ctrl Pts',(-51.4043053238161,-14.0896875604189,
3.40931815756628));
#58195=CARTESIAN_POINT('Ctrl Pts',(-52.4637825025118,-12.7337892614639,
3.48782366794306));
#58196=CARTESIAN_POINT('Ctrl Pts',(-54.1791548450535,-12.8696194053218,
3.56632917831984));
#58197=CARTESIAN_POINT('Ctrl Pts',(-54.7377809864981,-13.8795446348882,
3.61898404780924));
#58198=CARTESIAN_POINT('Ctrl Pts',(-54.7405695133476,-14.3908895621182,
3.64547041383972));
#58199=CARTESIAN_POINT('Ctrl Pts',(-54.740563122869,-14.3970262782475,3.64578827641127));
#58200=CARTESIAN_POINT('Ctrl Pts',(-54.740301190334,-14.3965688164983,3.10421172358873));
#58201=CARTESIAN_POINT('Ctrl Pts',(-54.7380390595611,-14.8689546274246,
3.12866870094305));
#58202=CARTESIAN_POINT('Ctrl Pts',(-54.2559651859222,-15.850784329065,3.17929418175629));
#58203=CARTESIAN_POINT('Ctrl Pts',(-52.5930539078611,-16.1115149029785,
3.25608816602847));
#58204=CARTESIAN_POINT('Ctrl Pts',(-51.4330422815012,-14.8405600699842,
3.33459367640525));
#58205=CARTESIAN_POINT('Ctrl Pts',(-51.8533182226522,-13.1719316222439,
3.41309918678203));
#58206=CARTESIAN_POINT('Ctrl Pts',(-53.4769681733105,-12.6020950974316,
3.49160469715881));
#58207=CARTESIAN_POINT('Ctrl Pts',(-54.5893972536881,-13.4460134923652,
3.55530887609438));
#58208=CARTESIAN_POINT('Ctrl Pts',(-54.7365984888838,-14.175463319392,3.59284455157102));
#58209=CARTESIAN_POINT('Ctrl Pts',(-54.7359273488899,-14.3966252672389,
3.60421172358873));
#58210=CARTESIAN_POINT('Origin',(-53.1951359564886,-14.3971354987959,0.895788276411275));
#58211=CARTESIAN_POINT('',(-54.73716587472,-14.3983674417199,2.60421172358873));
#58212=CARTESIAN_POINT('',(-54.7375657625992,-14.3958310564158,2.64578827641127));
#58213=CARTESIAN_POINT('',(-54.7381359564886,-14.3971354987959,0.895788276411275));
#58214=CARTESIAN_POINT('Ctrl Pts',(-54.7375657625992,-14.3958310564158,
2.64578827641127));
#58215=CARTESIAN_POINT('Ctrl Pts',(-54.734479142859,-14.7643796819994,2.66478170566594));
#58216=CARTESIAN_POINT('Ctrl Pts',(-54.4188250031304,-15.6454555959149,
2.70994363837953));
#58217=CARTESIAN_POINT('Ctrl Pts',(-52.9564009216581,-16.198413027115,2.78127407455204));
#58218=CARTESIAN_POINT('Ctrl Pts',(-51.5609762954032,-15.1915669978344,
2.85977958492882));
#58219=CARTESIAN_POINT('Ctrl Pts',(-51.6311047416152,-13.472254177388,2.9382850953056));
#58220=CARTESIAN_POINT('Ctrl Pts',(-53.1038936445493,-12.5823977792547,
3.01679060568238));
#58221=CARTESIAN_POINT('Ctrl Pts',(-54.4735979274945,-13.2323024338895,
3.0859583327176));
#58222=CARTESIAN_POINT('Ctrl Pts',(-54.7345217286191,-14.0710096690757,
3.1289575562939));
#58223=CARTESIAN_POINT('Ctrl Pts',(-54.7365381831935,-14.3981451127971,
3.14578827641127));
#58224=CARTESIAN_POINT('Ctrl Pts',(-54.73716587472,-14.3983674417199,2.60421172358873));
#58225=CARTESIAN_POINT('Ctrl Pts',(-54.7383644283813,-14.5526183883782,
2.61215584339723));
#58226=CARTESIAN_POINT('Ctrl Pts',(-54.6467666252149,-15.2135939671077,
2.64626846666466));
#58227=CARTESIAN_POINT('Ctrl Pts',(-53.7056202382209,-16.1409758479641,
2.70654959339102));
#58228=CARTESIAN_POINT('Ctrl Pts',(-52.0221470001079,-15.7848310056966,
2.78505510376779));
#58229=CARTESIAN_POINT('Ctrl Pts',(-51.3906291820653,-14.1841570315506,
2.86356061414457));
#58230=CARTESIAN_POINT('Ctrl Pts',(-52.377440405223,-12.7744925974775,2.94206612452135));
#58231=CARTESIAN_POINT('Ctrl Pts',(-54.0975782126822,-12.8200502087089,
3.02057163489813));
#58232=CARTESIAN_POINT('Ctrl Pts',(-54.7246398714755,-13.8251629314517,
3.07462016792059));
#58233=CARTESIAN_POINT('Ctrl Pts',(-54.7404594967271,-14.3635107392415,
3.10250019748412));
#58234=CARTESIAN_POINT('Ctrl Pts',(-54.740301190334,-14.3965688164983,3.10421172358873));
#58235=CARTESIAN_POINT('Origin',(-53.1951359564886,-14.3971354987959,0.895788276411275));
#58236=CARTESIAN_POINT('',(-54.7364807484814,-14.3955730757723,2.10421172358873));
#58237=CARTESIAN_POINT('',(-54.7400287307462,-14.397884086359,2.14578827641127));
#58238=CARTESIAN_POINT('',(-54.7381359564886,-14.3971354987959,0.895788276411275));
#58239=CARTESIAN_POINT('',(-53.5936497983459,-12.9064860705774,2.));
#58240=CARTESIAN_POINT('Ctrl Pts',(-53.5936497983459,-12.9064860705774,
2.));
#58241=CARTESIAN_POINT('Ctrl Pts',(-54.083839596546,-13.0375346028627,2.02616850345893));
#58242=CARTESIAN_POINT('Ctrl Pts',(-54.6367230898564,-13.5559776050111,
2.06090574465517));
#58243=CARTESIAN_POINT('Ctrl Pts',(-54.737618997593,-14.2290968579424,2.09564298585141));
#58244=CARTESIAN_POINT('Ctrl Pts',(-54.7364807484814,-14.3955730757723,
2.10421172358873));
#58245=CARTESIAN_POINT('',(-52.7955982877703,-12.9041242545674,2.));
#58246=CARTESIAN_POINT('Origin',(-53.1951359564886,-14.3971354987959,2.));
#58247=CARTESIAN_POINT('Ctrl Pts',(-52.7955926848293,-12.9041113294173,
2.));
#58248=CARTESIAN_POINT('Ctrl Pts',(-53.2607241041144,-12.7814202621555,
2.02490816038701));
#58249=CARTESIAN_POINT('Ctrl Pts',(-54.2926583006945,-12.9966875828164,
2.0735042525241));
#58250=CARTESIAN_POINT('Ctrl Pts',(-54.7371492824905,-13.9402272601641,
2.12210034466119));
#58251=CARTESIAN_POINT('Ctrl Pts',(-54.7400287307462,-14.397884086359,2.14578827641127));
#58252=CARTESIAN_POINT('Origin',(-14.1292828945604,-53.2669068454841,4.5));
#58253=CARTESIAN_POINT('',(-14.7605875520818,-54.3602657339262,5.80658032638058));
#58254=CARTESIAN_POINT('',(-14.7625813317604,-54.3604987677495,5.94341967361942));
#58255=CARTESIAN_POINT('',(-14.7615328945604,-54.3619959685696,4.5));
#58256=CARTESIAN_POINT('',(-13.8936870225526,-54.5092654229862,6.));
#58257=CARTESIAN_POINT('Ctrl Pts',(-14.7625813317604,-54.3604987677495,
5.94341967361942));
#58258=CARTESIAN_POINT('Ctrl Pts',(-14.5022241622972,-54.5077988388626,
5.96227978241295));
#58259=CARTESIAN_POINT('Ctrl Pts',(-14.1881298777611,-54.5651023789871,
5.98113989120648));
#58260=CARTESIAN_POINT('Ctrl Pts',(-13.8936870225526,-54.5092654229862,
6.00000000000001));
#58261=CARTESIAN_POINT('',(-14.7615328945604,-54.3619959685696,6.));
#58262=CARTESIAN_POINT('Origin',(-14.1292828945604,-53.2669068454841,6.));
#58263=CARTESIAN_POINT('',(-14.7615328945604,-54.3619959685696,7.));
#58264=CARTESIAN_POINT('',(-14.7615328945604,-54.3619959685696,4.5));
#58265=CARTESIAN_POINT('',(-12.8669333849943,-53.3406222827979,7.));
#58266=CARTESIAN_POINT('Origin',(-14.1292828945604,-53.2669068454841,7.));
#58267=CARTESIAN_POINT('',(-15.3916324041264,-53.1931914081703,7.));
#58268=CARTESIAN_POINT('Origin',(-14.1292828945604,-53.2669068454841,7.));
#58269=CARTESIAN_POINT('Origin',(-14.1292828945604,-53.2669068454841,7.));
#58270=CARTESIAN_POINT('',(-12.9337035820667,-52.8487780612892,6.));
#58271=CARTESIAN_POINT('Origin',(-14.1292828945604,-53.2669068454841,6.));
#58272=CARTESIAN_POINT('Ctrl Pts',(-12.9336933707122,-52.8487726938777,
6.));
#58273=CARTESIAN_POINT('Ctrl Pts',(-12.8048848553781,-53.2213517629531,
5.97509183961299));
#58274=CARTESIAN_POINT('Ctrl Pts',(-12.8625933288288,-53.6603618768577,
5.95018367922598));
#58275=CARTESIAN_POINT('Ctrl Pts',(-13.0861255368911,-53.9849952189361,
5.92527551883897));
#58276=CARTESIAN_POINT('Ctrl Pts',(-13.3209683863418,-54.3260548798291,
5.89910701538004));
#58277=CARTESIAN_POINT('Ctrl Pts',(-13.7388407631054,-54.540870088853,5.87293851192112));
#58278=CARTESIAN_POINT('Ctrl Pts',(-14.1527369297938,-54.5331774952646,
5.84677000846219));
#58279=CARTESIAN_POINT('Ctrl Pts',(-14.3646246721213,-54.5292393909301,
5.83337344776832));
#58280=CARTESIAN_POINT('Ctrl Pts',(-14.5754703413608,-54.4669871159197,
5.81997688707445));
#58281=CARTESIAN_POINT('Ctrl Pts',(-14.7605875520818,-54.3602657339262,
5.80658032638058));
#58282=CARTESIAN_POINT('Origin',(-14.1292828945604,-53.2669068454841,4.5));
#58283=CARTESIAN_POINT('',(-14.7628720032994,-54.3627600319775,5.30658032638058));
#58284=CARTESIAN_POINT('',(-14.761790188637,-54.3636903053853,5.44341967361943));
#58285=CARTESIAN_POINT('',(-14.7615328945604,-54.3619959685696,4.5));
#58286=CARTESIAN_POINT('Ctrl Pts',(-14.761790188637,-54.3636903053853,5.44341967361943));
#58287=CARTESIAN_POINT('Ctrl Pts',(-14.7297149272464,-54.3824695710557,
5.44576692486714));
#58288=CARTESIAN_POINT('Ctrl Pts',(-14.6967938380796,-54.3997466843014,
5.44811417611484));
#58289=CARTESIAN_POINT('Ctrl Pts',(-14.6631180766711,-54.4153998475156,
5.45046142736255));
#58290=CARTESIAN_POINT('Ctrl Pts',(-14.2876813696889,-54.5899102907896,
5.47662993082148));
#58291=CARTESIAN_POINT('Ctrl Pts',(-13.8184459253802,-54.5625788561695,
5.5027984342804));
#58292=CARTESIAN_POINT('Ctrl Pts',(-13.4657801062202,-54.3456807478706,
5.52896693773933));
#58293=CARTESIAN_POINT('Ctrl Pts',(-13.1131142870602,-54.1287826395717,
5.55513544119826));
#58294=CARTESIAN_POINT('Ctrl Pts',(-12.8770180930488,-53.7223178575942,
5.58130394465719));
#58295=CARTESIAN_POINT('Ctrl Pts',(-12.8634449158406,-53.308510984467,5.60747244811611));
#58296=CARTESIAN_POINT('Ctrl Pts',(-12.8498717386324,-52.8947041113399,
5.63364095157504));
#58297=CARTESIAN_POINT('Ctrl Pts',(-13.0588215782272,-52.4735551470632,
5.65980945503396));
#58298=CARTESIAN_POINT('Ctrl Pts',(-13.3964281425195,-52.2339907213231,
5.68597795849289));
#58299=CARTESIAN_POINT('Ctrl Pts',(-13.7340347068117,-51.994426295583,5.71214646195181));
#58300=CARTESIAN_POINT('Ctrl Pts',(-14.2002979958014,-51.9364464083796,
5.73831496541074));
#58301=CARTESIAN_POINT('Ctrl Pts',(-14.5864832378068,-52.0858916506601,
5.76448346886967));
#58302=CARTESIAN_POINT('Ctrl Pts',(-14.9726684798122,-52.2353368929406,
5.7906519723286));
#58303=CARTESIAN_POINT('Ctrl Pts',(-15.2787756748334,-52.5922072647049,
5.81682047578752));
#58304=CARTESIAN_POINT('Ctrl Pts',(-15.3668446182304,-52.9968058417406,
5.84298897924645));
#58305=CARTESIAN_POINT('Ctrl Pts',(-15.4549135616273,-53.4014044187763,
5.86915748270538));
#58306=CARTESIAN_POINT('Ctrl Pts',(-15.3249442534001,-53.8537312010833,
5.8953259861643));
#58307=CARTESIAN_POINT('Ctrl Pts',(-15.0367728841186,-54.1500649721194,
5.92149448962323));
#58308=CARTESIAN_POINT('Ctrl Pts',(-14.9562917782242,-54.2328256907374,
5.92880288428863));
#58309=CARTESIAN_POINT('Ctrl Pts',(-14.8634711500129,-54.3034191895921,
5.93611127895402));
#58310=CARTESIAN_POINT('Ctrl Pts',(-14.7625813317604,-54.3604987677495,
5.94341967361942));
#58311=CARTESIAN_POINT('Ctrl Pts',(-14.7605875520818,-54.3602657339262,
5.80658032638058));
#58312=CARTESIAN_POINT('Ctrl Pts',(-14.9370736274398,-54.2585202625491,
5.79380838361552));
#58313=CARTESIAN_POINT('Ctrl Pts',(-15.0901745042163,-54.1163557782414,
5.78103644085047));
#58314=CARTESIAN_POINT('Ctrl Pts',(-15.1984983273049,-53.9457696468095,
5.76826449808541));
#58315=CARTESIAN_POINT('Ctrl Pts',(-15.4204436015143,-53.5962547881436,
5.74209599462648));
#58316=CARTESIAN_POINT('Ctrl Pts',(-15.4544141933199,-53.1274254670123,
5.71592749116756));
#58317=CARTESIAN_POINT('Ctrl Pts',(-15.2852697206798,-52.7495259168145,
5.68975898770863));
#58318=CARTESIAN_POINT('Ctrl Pts',(-15.1161252480397,-52.3716263666168,
5.6635904842497));
#58319=CARTESIAN_POINT('Ctrl Pts',(-14.7438657109538,-52.0846565873524,
5.63742198079078));
#58320=CARTESIAN_POINT('Ctrl Pts',(-14.3353706309513,-52.0172894645935,
5.61125347733185));
#58321=CARTESIAN_POINT('Ctrl Pts',(-13.9268755509488,-51.9499223418345,
5.58508497387292));
#58322=CARTESIAN_POINT('Ctrl Pts',(-13.4821449280297,-52.1021578755809,
5.558916470414));
#58323=CARTESIAN_POINT('Ctrl Pts',(-13.2006242325167,-52.4057357189425,
5.53274796695507));
#58324=CARTESIAN_POINT('Ctrl Pts',(-12.9191035370036,-52.7093135623041,
5.50657946349614));
#58325=CARTESIAN_POINT('Ctrl Pts',(-12.8007927688965,-53.1642337152808,
5.48041096003722));
#58326=CARTESIAN_POINT('Ctrl Pts',(-12.8987324301598,-53.5665026413488,
5.45424245657829));
#58327=CARTESIAN_POINT('Ctrl Pts',(-12.9966720914232,-53.9687715674168,
5.42807395311936));
#58328=CARTESIAN_POINT('Ctrl Pts',(-13.3108621820569,-54.3183892665762,
5.40190544966044));
#58329=CARTESIAN_POINT('Ctrl Pts',(-13.7004218404059,-54.4585839700533,
5.37573694620151));
#58330=CARTESIAN_POINT('Ctrl Pts',(-14.0435904799156,-54.5820834768108,
5.35268473959454));
#58331=CARTESIAN_POINT('Ctrl Pts',(-14.4452466462963,-54.5430686762864,
5.32963253298756));
#58332=CARTESIAN_POINT('Ctrl Pts',(-14.7628720032994,-54.3627600319775,
5.30658032638058));
#58333=CARTESIAN_POINT('Origin',(-14.1292828945604,-53.2669068454841,4.5));
#58334=CARTESIAN_POINT('',(-14.7604987163791,-54.3623830037273,4.80658032638058));
#58335=CARTESIAN_POINT('',(-14.7603543171395,-54.3604895118786,4.94341967361942));
#58336=CARTESIAN_POINT('',(-14.7615328945604,-54.3619959685696,4.5));
#58337=CARTESIAN_POINT('Ctrl Pts',(-14.7603543171395,-54.3604895118786,
4.94341967361942));
#58338=CARTESIAN_POINT('Ctrl Pts',(-14.5947715388364,-54.4565158591777,
4.95542257078024));
#58339=CARTESIAN_POINT('Ctrl Pts',(-14.4086766047112,-54.5167140163305,
4.96742546794106));
#58340=CARTESIAN_POINT('Ctrl Pts',(-14.2192552064615,-54.5302046425139,
4.97942836510188));
#58341=CARTESIAN_POINT('Ctrl Pts',(-13.8062820343284,-54.5596166663956,
5.00559686856081));
#58342=CARTESIAN_POINT('Ctrl Pts',(-13.3774975305931,-54.3670187022342,
5.03176537201973));
#58343=CARTESIAN_POINT('Ctrl Pts',(-13.1251731138615,-54.0387742648884,
5.05793387547866));
#58344=CARTESIAN_POINT('Ctrl Pts',(-12.8728486971299,-53.7105298275425,
5.08410237893758));
#58345=CARTESIAN_POINT('Ctrl Pts',(-12.796984367402,-53.2466389170122,5.11027088239651));
#58346=CARTESIAN_POINT('Ctrl Pts',(-12.9315998955733,-52.8551151331565,
5.13643938585543));
#58347=CARTESIAN_POINT('Ctrl Pts',(-13.0662154237446,-52.4635913493009,
5.16260788931436));
#58348=CARTESIAN_POINT('Ctrl Pts',(-13.411310809815,-52.14443469212,5.18877639277329));
#58349=CARTESIAN_POINT('Ctrl Pts',(-13.81213856493,-52.0407600014986,5.21494489623221));
#58350=CARTESIAN_POINT('Ctrl Pts',(-14.212966320045,-51.9370853108772,5.24111339969114));
#58351=CARTESIAN_POINT('Ctrl Pts',(-14.6695264442046,-52.0488925868152,
5.26728190315007));
#58352=CARTESIAN_POINT('Ctrl Pts',(-14.9770971987178,-52.3260437079763,
5.29345040660899));
#58353=CARTESIAN_POINT('Ctrl Pts',(-15.2846679532311,-52.6031948291373,
5.31961891006792));
#58354=CARTESIAN_POINT('Ctrl Pts',(-15.4432493380979,-53.0456897955214,
5.34578741352684));
#58355=CARTESIAN_POINT('Ctrl Pts',(-15.3817210457035,-53.4551134392974,
5.37195591698577));
#58356=CARTESIAN_POINT('Ctrl Pts',(-15.3257116918039,-53.827812775923,5.39577716919699));
#58357=CARTESIAN_POINT('Ctrl Pts',(-15.087308341869,-54.1731075442456,5.41959842140821));
#58358=CARTESIAN_POINT('Ctrl Pts',(-14.761790188637,-54.3636903053853,5.44341967361943));
#58359=CARTESIAN_POINT('Ctrl Pts',(-14.7628720032994,-54.3627600319775,
5.30658032638058));
#58360=CARTESIAN_POINT('Ctrl Pts',(-14.8058099708877,-54.3383851306842,
5.30346402952863));
#58361=CARTESIAN_POINT('Ctrl Pts',(-14.8472122922316,-54.3114281126392,
5.30034773267668));
#58362=CARTESIAN_POINT('Ctrl Pts',(-14.8867268805692,-54.281941402285,5.29723143582473));
#58363=CARTESIAN_POINT('Ctrl Pts',(-15.2185430363193,-54.0343324232445,
5.27106293236581));
#58364=CARTESIAN_POINT('Ctrl Pts',(-15.4172461217553,-53.6083427573686,
5.24489442890688));
#58365=CARTESIAN_POINT('Ctrl Pts',(-15.393736730538,-53.1949914739396,5.21872592544795));
#58366=CARTESIAN_POINT('Ctrl Pts',(-15.3702273393206,-52.7816401905105,
5.19255742198903));
#58367=CARTESIAN_POINT('Ctrl Pts',(-15.12450547145,-52.3809272895283,5.1663889185301));
#58368=CARTESIAN_POINT('Ctrl Pts',(-14.7667550258398,-52.1725370796236,
5.14022041507117));
#58369=CARTESIAN_POINT('Ctrl Pts',(-14.4090045802295,-51.9641468697189,
5.11405191161225));
#58370=CARTESIAN_POINT('Ctrl Pts',(-13.9392255568797,-51.9480793508917,
5.08788340815332));
#58371=CARTESIAN_POINT('Ctrl Pts',(-13.5680728067533,-52.1315394490878,
5.0617149046944));
#58372=CARTESIAN_POINT('Ctrl Pts',(-13.1969200566269,-52.3149995472838,
5.03554640123547));
#58373=CARTESIAN_POINT('Ctrl Pts',(-12.9243935797239,-52.6979872625031,
5.00937789777654));
#58374=CARTESIAN_POINT('Ctrl Pts',(-12.8726973119175,-53.1087663210662,
4.98320939431761));
#58375=CARTESIAN_POINT('Ctrl Pts',(-12.8210010441111,-53.5195453796293,
4.95704089085869));
#58376=CARTESIAN_POINT('Ctrl Pts',(-12.9901349854012,-53.9581157815361,
4.93087238739976));
#58377=CARTESIAN_POINT('Ctrl Pts',(-13.3042575537142,-54.2278173601559,
4.90470388394083));
#58378=CARTESIAN_POINT('Ctrl Pts',(-13.6183801220271,-54.4975189387757,
4.87853538048191));
#58379=CARTESIAN_POINT('Ctrl Pts',(-14.0774913173628,-54.5983516941084,
4.85236687702298));
#58380=CARTESIAN_POINT('Ctrl Pts',(-14.4757201786558,-54.4851010127079,
4.82619837356405));
#58381=CARTESIAN_POINT('Ctrl Pts',(-14.5752351369457,-54.4568003596631,
4.8196590245029));
#58382=CARTESIAN_POINT('Ctrl Pts',(-14.6709481788587,-54.4151308478692,
4.81311967544174));
#58383=CARTESIAN_POINT('Ctrl Pts',(-14.7604987163791,-54.3623830037273,
4.80658032638058));
#58384=CARTESIAN_POINT('Origin',(-14.1292828945604,-53.2669068454841,4.5));
#58385=CARTESIAN_POINT('',(-14.7614006096927,-54.3603381104062,4.30658032638058));
#58386=CARTESIAN_POINT('',(-14.7627659331487,-54.3621523730593,4.44341967361942));
#58387=CARTESIAN_POINT('',(-14.7615328945604,-54.3619959685696,4.5));
#58388=CARTESIAN_POINT('Ctrl Pts',(-14.7627659331487,-54.3621523730593,
4.44341967361942));
#58389=CARTESIAN_POINT('Ctrl Pts',(-14.463761030489,-54.5313718419493,4.46507821669335));
#58390=CARTESIAN_POINT('Ctrl Pts',(-14.0916672421201,-54.5784026588885,
4.48673675976727));
#58391=CARTESIAN_POINT('Ctrl Pts',(-13.7635961371407,-54.4794617725194,
4.5083953028412));
#58392=CARTESIAN_POINT('Ctrl Pts',(-13.3672107562715,-54.3599184164247,
4.53456380630013));
#58393=CARTESIAN_POINT('Ctrl Pts',(-13.0350905669399,-54.0272826554628,
4.56073230975905));
#58394=CARTESIAN_POINT('Ctrl Pts',(-12.9161621999348,-53.6307123234038,
4.58690081321798));
#58395=CARTESIAN_POINT('Ctrl Pts',(-12.7972338329298,-53.2341419913447,
4.61306931667691));
#58396=CARTESIAN_POINT('Ctrl Pts',(-12.8914972882515,-52.7736370881886,
4.63923782013583));
#58397=CARTESIAN_POINT('Ctrl Pts',(-13.1566837320242,-52.4556934772733,
4.66540632359475));
#58398=CARTESIAN_POINT('Ctrl Pts',(-13.421870175797,-52.1377498663579,4.69157482705368));
#58399=CARTESIAN_POINT('Ctrl Pts',(-13.8579796080209,-51.9623675476834,
4.71774333051261));
#58400=CARTESIAN_POINT('Ctrl Pts',(-14.2694553352381,-52.0081900560918,
4.74391183397154));
#58401=CARTESIAN_POINT('Ctrl Pts',(-14.6809310624553,-52.0540125645002,
4.77008033743047));
#58402=CARTESIAN_POINT('Ctrl Pts',(-15.0677730846659,-52.3210398999916,
4.79624884088939));
#58403=CARTESIAN_POINT('Ctrl Pts',(-15.2565169212345,-52.6895337942872,
4.82241734434832));
#58404=CARTESIAN_POINT('Ctrl Pts',(-15.4452607578031,-53.0580276885828,
4.84858584780724));
#58405=CARTESIAN_POINT('Ctrl Pts',(-15.4359064087297,-53.5279881416827,
4.87475435126617));
#58406=CARTESIAN_POINT('Ctrl Pts',(-15.2326483139276,-53.888679374195,4.90092285472509));
#58407=CARTESIAN_POINT('Ctrl Pts',(-15.1226200827607,-54.0839297446631,
4.9150884610232));
#58408=CARTESIAN_POINT('Ctrl Pts',(-14.9557721746586,-54.2471609203011,
4.92925406732131));
#58409=CARTESIAN_POINT('Ctrl Pts',(-14.7603543171395,-54.3604895118786,
4.94341967361942));
#58410=CARTESIAN_POINT('Ctrl Pts',(-14.7604987163791,-54.3623830037273,
4.80658032638058));
#58411=CARTESIAN_POINT('Ctrl Pts',(-15.0293024323073,-54.2040498780404,
4.78695117198281));
#58412=CARTESIAN_POINT('Ctrl Pts',(-15.2425807881071,-53.945898828656,4.76732201758504));
#58413=CARTESIAN_POINT('Ctrl Pts',(-15.3364895893995,-53.6498791715159,
4.74769286318727));
#58414=CARTESIAN_POINT('Ctrl Pts',(-15.4616836115997,-53.2552421298581,
4.72152435972835));
#58415=CARTESIAN_POINT('Ctrl Pts',(-15.3747251287498,-52.7933021646762,
4.69535585626942));
#58416=CARTESIAN_POINT('Ctrl Pts',(-15.1146073473566,-52.471198645522,4.6691873528105));
#58417=CARTESIAN_POINT('Ctrl Pts',(-14.8544895659634,-52.1490951263678,
4.64301884935157));
#58418=CARTESIAN_POINT('Ctrl Pts',(-14.4212124860269,-51.9668280532413,
4.61685034589264));
#58419=CARTESIAN_POINT('Ctrl Pts',(-14.009062705893,-52.0061281492218,4.59068184243372));
#58420=CARTESIAN_POINT('Ctrl Pts',(-13.596912925759,-52.0454282452023,4.56451333897479));
#58421=CARTESIAN_POINT('Ctrl Pts',(-13.2058904454275,-52.3062955102899,
4.53834483551586));
#58422=CARTESIAN_POINT('Ctrl Pts',(-13.0113343903925,-52.6717539614819,
4.51217633205694));
#58423=CARTESIAN_POINT('Ctrl Pts',(-12.8167783353574,-53.037212412674,4.48600782859801));
#58424=CARTESIAN_POINT('Ctrl Pts',(-12.8186887056188,-53.5072620499705,
4.45983932513909));
#58425=CARTESIAN_POINT('Ctrl Pts',(-13.0162088697902,-53.8711270288388,
4.43367082168016));
#58426=CARTESIAN_POINT('Ctrl Pts',(-13.2137290339616,-54.2349920077072,
4.40750231822123));
#58427=CARTESIAN_POINT('Ctrl Pts',(-13.606858992043,-54.4926723281474,4.38133381476231));
#58428=CARTESIAN_POINT('Ctrl Pts',(-14.0193145970927,-54.5286210713629,
4.35516531130338));
#58429=CARTESIAN_POINT('Ctrl Pts',(-14.2745724669733,-54.5508687981624,
4.33897031632911));
#58430=CARTESIAN_POINT('Ctrl Pts',(-14.5372321463568,-54.4881923359769,
4.32277532135484));
#58431=CARTESIAN_POINT('Ctrl Pts',(-14.7614006096927,-54.3603381104062,
4.30658032638058));
#58432=CARTESIAN_POINT('Origin',(-14.1292828945604,-53.2669068454841,4.5));
#58433=CARTESIAN_POINT('',(-14.7626048989925,-54.3636737206204,3.80658032638058));
#58434=CARTESIAN_POINT('',(-14.7608564829457,-54.3629211099724,3.94341967361942));
#58435=CARTESIAN_POINT('',(-14.7615328945604,-54.3619959685696,4.5));
#58436=CARTESIAN_POINT('Ctrl Pts',(-14.7608564829457,-54.3629211099724,
3.94341967361942));
#58437=CARTESIAN_POINT('Ctrl Pts',(-14.6904886508113,-54.4043824600063,
3.94856535914753));
#58438=CARTESIAN_POINT('Ctrl Pts',(-14.6162453479771,-54.4388759703619,
3.95371104467564));
#58439=CARTESIAN_POINT('Ctrl Pts',(-14.5392165090643,-54.465226788063,3.95885673020374));
#58440=CARTESIAN_POINT('Ctrl Pts',(-14.1474845568268,-54.5992344844895,
3.98502523366267));
#58441=CARTESIAN_POINT('Ctrl Pts',(-13.6837115472213,-54.5226514105579,
4.0111937371216));
#58442=CARTESIAN_POINT('Ctrl Pts',(-13.3558588106244,-54.2698183268938,
4.03736224058052));
#58443=CARTESIAN_POINT('Ctrl Pts',(-13.0280060740275,-54.0169852432297,
4.06353074403945));
#58444=CARTESIAN_POINT('Ctrl Pts',(-12.8360736104392,-53.5879021498332,
4.08969924749838));
#58445=CARTESIAN_POINT('Ctrl Pts',(-12.8661262178428,-53.1749750062963,
4.1158677509573));
#58446=CARTESIAN_POINT('Ctrl Pts',(-12.8961788252464,-52.7620478627593,
4.14203625441623));
#58447=CARTESIAN_POINT('Ctrl Pts',(-13.1482165036419,-52.3652766690821,
4.16820475787516));
#58448=CARTESIAN_POINT('Ctrl Pts',(-13.5092225624184,-52.1625783447115,
4.19437326133408));
#58449=CARTESIAN_POINT('Ctrl Pts',(-13.8702286211949,-51.959880020341,4.22054176479301));
#58450=CARTESIAN_POINT('Ctrl Pts',(-14.3402030603525,-51.951254565277,4.24671026825193));
#58451=CARTESIAN_POINT('Ctrl Pts',(-14.708403754256,-52.1405697363842,4.27287877171086));
#58452=CARTESIAN_POINT('Ctrl Pts',(-15.0766044481595,-52.3298849074914,
4.29904727516979));
#58453=CARTESIAN_POINT('Ctrl Pts',(-15.343031396809,-52.7171407047698,4.32521577862871));
#58454=CARTESIAN_POINT('Ctrl Pts',(-15.3882155906945,-53.1286870249125,
4.35138428208764));
#58455=CARTESIAN_POINT('Ctrl Pts',(-15.43339978458,-53.5402333450552,4.37755278554657));
#58456=CARTESIAN_POINT('Ctrl Pts',(-15.2573412237015,-53.9760701880622,
4.40372128900549));
#58457=CARTESIAN_POINT('Ctrl Pts',(-14.938986657059,-54.2407631339519,4.42988979246442));
#58458=CARTESIAN_POINT('Ctrl Pts',(-14.8841204517295,-54.2863811304883,
4.43439975284942));
#58459=CARTESIAN_POINT('Ctrl Pts',(-14.8250277510981,-54.3269157877332,
4.43890971323442));
#58460=CARTESIAN_POINT('Ctrl Pts',(-14.7627659331487,-54.3621523730593,
4.44341967361942));
#58461=CARTESIAN_POINT('Ctrl Pts',(-14.7614006096927,-54.3603381104062,
4.30658032638058));
#58462=CARTESIAN_POINT('Ctrl Pts',(-14.8994522777931,-54.2816005000793,
4.29660681789592));
#58463=CARTESIAN_POINT('Ctrl Pts',(-15.0229058598302,-54.178143727902,4.28663330941126));
#58464=CARTESIAN_POINT('Ctrl Pts',(-15.1210425075748,-54.0545798005254,
4.2766598009266));
#58465=CARTESIAN_POINT('Ctrl Pts',(-15.3785335609892,-53.7303726204816,
4.25049129746767));
#58466=CARTESIAN_POINT('Ctrl Pts',(-15.4617344158,-53.2677410944033,4.22432279400875));
#58467=CARTESIAN_POINT('Ctrl Pts',(-15.3333368195411,-52.8741346977794,
4.19815429054982));
#58468=CARTESIAN_POINT('Ctrl Pts',(-15.2049392232823,-52.4805283011554,
4.17198578709089));
#58469=CARTESIAN_POINT('Ctrl Pts',(-14.8649431759538,-52.1559470339858,
4.14581728363197));
#58470=CARTESIAN_POINT('Ctrl Pts',(-14.4658069467496,-52.0459369947103,
4.11964878017304));
#58471=CARTESIAN_POINT('Ctrl Pts',(-14.0666707175455,-51.9359269554348,
4.09348027671411));
#58472=CARTESIAN_POINT('Ctrl Pts',(-13.6083943064658,-52.0404881440534,
4.06731177325519));
#58473=CARTESIAN_POINT('Ctrl Pts',(-13.2964743036119,-52.3127340807067,
4.04114326979626));
#58474=CARTESIAN_POINT('Ctrl Pts',(-12.9845543007579,-52.5849800173601,
4.01497476633733));
#58475=CARTESIAN_POINT('Ctrl Pts',(-12.8189907061298,-53.0249107020483,
3.98880626287841));
#58476=CARTESIAN_POINT('Ctrl Pts',(-12.8740242036727,-53.4352559863353,
3.96263775941948));
#58477=CARTESIAN_POINT('Ctrl Pts',(-12.9290577012157,-53.8456012706222,
3.93646925596056));
#58478=CARTESIAN_POINT('Ctrl Pts',(-13.2046882909298,-54.2263611545079,
3.91030075250163));
#58479=CARTESIAN_POINT('Ctrl Pts',(-13.5773199398677,-54.4067983801299,
3.8841322490427));
#58480=CARTESIAN_POINT('Ctrl Pts',(-13.9454253210212,-54.5850438777981,
3.85828160815533));
#58481=CARTESIAN_POINT('Ctrl Pts',(-14.4081895758327,-54.5678037039579,
3.83243096726795));
#58482=CARTESIAN_POINT('Ctrl Pts',(-14.7626048989925,-54.3636737206204,
3.80658032638058));
#58483=CARTESIAN_POINT('Origin',(-14.1292828945604,-53.2669068454841,4.5));
#58484=CARTESIAN_POINT('',(-14.7601616123226,-54.3612756103012,3.30658032638058));
#58485=CARTESIAN_POINT('',(-14.7609899830459,-54.3602193411783,3.44341967361942));
#58486=CARTESIAN_POINT('',(-14.7615328945604,-54.3619959685696,4.5));
#58487=CARTESIAN_POINT('Ctrl Pts',(-14.7609899830459,-54.3602193411783,
3.44341967361942));
#58488=CARTESIAN_POINT('Ctrl Pts',(-14.5562500775905,-54.4775990222049,
3.45822100506064));
#58489=CARTESIAN_POINT('Ctrl Pts',(-14.3197636804794,-54.5407089292625,
3.47302233650185));
#58490=CARTESIAN_POINT('Ctrl Pts',(-14.0857261531979,-54.532655265383,3.48782366794307));
#58491=CARTESIAN_POINT('Ctrl Pts',(-13.671951766312,-54.5184165239613,3.51399217140199));
#58492=CARTESIAN_POINT('Ctrl Pts',(-13.2658319689464,-54.2817372437526,
3.54016067486092));
#58493=CARTESIAN_POINT('Ctrl Pts',(-13.0494757061861,-53.9287472260938,
3.56632917831984));
#58494=CARTESIAN_POINT('Ctrl Pts',(-12.8331194434257,-53.575757208435,3.59249768177877));
#58495=CARTESIAN_POINT('Ctrl Pts',(-12.8065267152706,-53.1064564533261,
3.6186661852377));
#58496=CARTESIAN_POINT('Ctrl Pts',(-12.9816220168908,-52.7312849984863,
3.64483468869663));
#58497=CARTESIAN_POINT('Ctrl Pts',(-13.1567173185109,-52.3561135436466,
3.67100319215555));
#58498=CARTESIAN_POINT('Ctrl Pts',(-13.5335006499063,-52.075071389076,3.69717169561448));
#58499=CARTESIAN_POINT('Ctrl Pts',(-13.9430178866457,-52.0141811772634,
3.72334019907341));
#58500=CARTESIAN_POINT('Ctrl Pts',(-14.3525351233851,-51.9532909654507,
3.74950870253233));
#58501=CARTESIAN_POINT('Ctrl Pts',(-14.7947862654687,-52.1125526963959,
3.77567720599126));
#58502=CARTESIAN_POINT('Ctrl Pts',(-15.0714606437586,-52.4205515169895,
3.80184570945019));
#58503=CARTESIAN_POINT('Ctrl Pts',(-15.3481350220485,-52.7285503375831,
3.82801421290911));
#58504=CARTESIAN_POINT('Ctrl Pts',(-15.4592326365449,-53.185286247825,3.85418271636804));
#58505=CARTESIAN_POINT('Ctrl Pts',(-15.3549359963582,-53.5859534363384,
3.88035121982696));
#58506=CARTESIAN_POINT('Ctrl Pts',(-15.271147892813,-53.907834791464,3.90137403775778));
#58507=CARTESIAN_POINT('Ctrl Pts',(-15.0483458981207,-54.1935297998804,
3.9223968556886));
#58508=CARTESIAN_POINT('Ctrl Pts',(-14.7608564829457,-54.3629211099724,
3.94341967361942));
#58509=CARTESIAN_POINT('Ctrl Pts',(-14.7626048989925,-54.3636737206204,
3.80658032638058));
#58510=CARTESIAN_POINT('Ctrl Pts',(-14.7669628321868,-54.3611637139356,
3.80626246380903));
#58511=CARTESIAN_POINT('Ctrl Pts',(-14.7713043836124,-54.3586254505289,
3.80594460123748));
#58512=CARTESIAN_POINT('Ctrl Pts',(-14.7756291758562,-54.3560589463809,
3.80562673866593));
#58513=CARTESIAN_POINT('Ctrl Pts',(-15.131674054745,-54.1447677196515,3.779458235207));
#58514=CARTESIAN_POINT('Ctrl Pts',(-15.3741311043607,-53.7420706988344,
3.75328973174807));
#58515=CARTESIAN_POINT('Ctrl Pts',(-15.3942797010543,-53.3285420152435,
3.72712122828914));
#58516=CARTESIAN_POINT('Ctrl Pts',(-15.414428297748,-52.9150133316526,3.70095272483022));
#58517=CARTESIAN_POINT('Ctrl Pts',(-15.2122684415196,-52.4906529852878,
3.67478422137129));
#58518=CARTESIAN_POINT('Ctrl Pts',(-14.8784510160553,-52.2457491989657,
3.64861571791236));
#58519=CARTESIAN_POINT('Ctrl Pts',(-14.544633590591,-52.0008454126437,3.62244721445344));
#58520=CARTESIAN_POINT('Ctrl Pts',(-14.0791585958908,-51.9353981863644,
3.59627871099451));
#58521=CARTESIAN_POINT('Ctrl Pts',(-13.6907505503598,-52.0787548359323,
3.57011020753558));
#58522=CARTESIAN_POINT('Ctrl Pts',(-13.3023425048288,-52.2221114855001,
3.54394170407666));
#58523=CARTESIAN_POINT('Ctrl Pts',(-12.991001408467,-52.5742720109151,3.51777320061773));
#58524=CARTESIAN_POINT('Ctrl Pts',(-12.896336314222,-52.9773234433404,3.49160469715881));
#58525=CARTESIAN_POINT('Ctrl Pts',(-12.801671219977,-53.3803748757656,3.46543619369988));
#58526=CARTESIAN_POINT('Ctrl Pts',(-12.9236821278489,-53.8343172152012,
3.43926769024095));
#58527=CARTESIAN_POINT('Ctrl Pts',(-13.2076578874333,-54.1355973270763,
3.41309918678203));
#58528=CARTESIAN_POINT('Ctrl Pts',(-13.4916336470178,-54.4368774389515,
3.3869306833231));
#58529=CARTESIAN_POINT('Ctrl Pts',(-13.9375742583148,-54.5854953232663,
3.36076217986417));
#58530=CARTESIAN_POINT('Ctrl Pts',(-14.3455146684413,-54.5148089413369,
3.33459367640524));
#58531=CARTESIAN_POINT('Ctrl Pts',(-14.4910812336828,-54.4895857137002,
3.32525589306369));
#58532=CARTESIAN_POINT('Ctrl Pts',(-14.6318092436287,-54.436438533397,3.31591810972213));
#58533=CARTESIAN_POINT('Ctrl Pts',(-14.7601616123226,-54.3612756103012,
3.30658032638058));
#58534=CARTESIAN_POINT('Origin',(-14.1292828945604,-53.2669068454841,4.5));
#58535=CARTESIAN_POINT('',(-14.7622249872189,-54.3610567043161,2.80658032638058));
#58536=CARTESIAN_POINT('',(-14.7628222445742,-54.3633003878638,2.94341967361942));
#58537=CARTESIAN_POINT('',(-14.7615328945604,-54.3619959685696,4.5));
#58538=CARTESIAN_POINT('Ctrl Pts',(-14.7628222445742,-54.3633003878638,
2.94341967361942));
#58539=CARTESIAN_POINT('Ctrl Pts',(-14.4266363996141,-54.5552567541312,
2.96787665097375));
#58540=CARTESIAN_POINT('Ctrl Pts',(-13.9945792873817,-54.5843264233178,
2.99233362832807));
#58541=CARTESIAN_POINT('Ctrl Pts',(-13.6379437474727,-54.4342123040852,
3.01679060568239));
#58542=CARTESIAN_POINT('Ctrl Pts',(-13.256350461251,-54.2735930341132,3.04295910914132));
#58543=CARTESIAN_POINT('Ctrl Pts',(-12.9611042822246,-53.9078334931332,
3.06912761260024));
#58544=CARTESIAN_POINT('Ctrl Pts',(-12.8845971374177,-53.5009445240528,
3.09529611605917));
#58545=CARTESIAN_POINT('Ctrl Pts',(-12.8080899926108,-53.0940555549725,
3.12146461951809));
#58546=CARTESIAN_POINT('Ctrl Pts',(-12.9503218820233,-52.6460371577917,
3.14763312297702));
#58547=CARTESIAN_POINT('Ctrl Pts',(-13.2475143204017,-52.3577861486808,
3.17380162643595));
#58548=CARTESIAN_POINT('Ctrl Pts',(-13.54470675878,-52.0695351395699,3.19997012989488));
#58549=CARTESIAN_POINT('Ctrl Pts',(-13.9968597461241,-51.9410515185288,
3.2261386333538));
#58550=CARTESIAN_POINT('Ctrl Pts',(-14.4012225159017,-52.0299488478796,
3.25230713681273));
#58551=CARTESIAN_POINT('Ctrl Pts',(-14.8055852856793,-52.1188461772304,
3.27847564027165));
#58552=CARTESIAN_POINT('Ctrl Pts',(-15.1621578378903,-52.4251244569732,
3.30464414373058));
#58553=CARTESIAN_POINT('Ctrl Pts',(-15.3110487977949,-52.8114448760709,
3.33081264718951));
#58554=CARTESIAN_POINT('Ctrl Pts',(-15.4599397576996,-53.1977652951686,
3.35698115064843));
#58555=CARTESIAN_POINT('Ctrl Pts',(-15.4011491252979,-53.6641278536213,
3.38314965410736));
#58556=CARTESIAN_POINT('Ctrl Pts',(-15.161039320894,-54.0014100315303,3.40931815756629));
#58557=CARTESIAN_POINT('Ctrl Pts',(-15.0567395295787,-54.1479199204438,
3.420685329584));
#58558=CARTESIAN_POINT('Ctrl Pts',(-14.918226764983,-54.2700737329326,3.43205250160171));
#58559=CARTESIAN_POINT('Ctrl Pts',(-14.7609899830459,-54.3602193411783,
3.44341967361942));
#58560=CARTESIAN_POINT('Ctrl Pts',(-14.7601616123226,-54.3612756103012,
3.30658032638058));
#58561=CARTESIAN_POINT('Ctrl Pts',(-14.9915080373649,-54.2257995475618,
3.28974960626321));
#58562=CARTESIAN_POINT('Ctrl Pts',(-15.1826489574086,-54.0187995905144,
3.27291888614584));
#58563=CARTESIAN_POINT('Ctrl Pts',(-15.2894496720194,-53.7748722761244,
3.25608816602847));
#58564=CARTESIAN_POINT('Ctrl Pts',(-15.4555040565151,-53.395612641015,3.22991966256954));
#58565=CARTESIAN_POINT('Ctrl Pts',(-15.4176726165505,-52.9270840189701,
3.20375115911061));
#58566=CARTESIAN_POINT('Ctrl Pts',(-15.1929194920754,-52.5793801620778,
3.17758265565168));
#58567=CARTESIAN_POINT('Ctrl Pts',(-14.9681663676002,-52.2316763051856,
3.15141415219276));
#58568=CARTESIAN_POINT('Ctrl Pts',(-14.5564915586145,-52.004797213446,3.12524564873383));
#58569=CARTESIAN_POINT('Ctrl Pts',(-14.1424947973993,-52.0004782714699,
3.09907714527491));
#58570=CARTESIAN_POINT('Ctrl Pts',(-13.7284980361841,-51.9961593294939,
3.07290864181598));
#58571=CARTESIAN_POINT('Ctrl Pts',(-13.3121793227393,-52.2144005372813,
3.04674013835705));
#58572=CARTESIAN_POINT('Ctrl Pts',(-13.0802212088747,-52.5573397364563,
3.02057163489813));
#58573=CARTESIAN_POINT('Ctrl Pts',(-12.8482630950101,-52.9002789356314,
2.9944031314392));
#58574=CARTESIAN_POINT('Ctrl Pts',(-12.8006655807257,-53.3679161261941,
2.96823462798027));
#58575=CARTESIAN_POINT('Ctrl Pts',(-12.9587713715114,-53.7505576476053,
2.94206612452135));
#58576=CARTESIAN_POINT('Ctrl Pts',(-13.116877162297,-54.1331991690165,2.91589762106242));
#58577=CARTESIAN_POINT('Ctrl Pts',(-13.4806862581528,-54.4308450212763,
2.88972911760349));
#58578=CARTESIAN_POINT('Ctrl Pts',(-13.8870635107844,-54.5100264348898,
2.86356061414457));
#58579=CARTESIAN_POINT('Ctrl Pts',(-14.1820172367656,-54.5674973017321,
2.8445671848899));
#58580=CARTESIAN_POINT('Ctrl Pts',(-14.4993960343841,-54.5098802470415,
2.82557375563524));
#58581=CARTESIAN_POINT('Ctrl Pts',(-14.7622249872189,-54.3610567043161,
2.80658032638058));
#58582=CARTESIAN_POINT('Origin',(-14.1292828945604,-53.2669068454841,4.5));
#58583=CARTESIAN_POINT('',(-14.7617771735939,-54.3636459375188,2.30658032638058));
#58584=CARTESIAN_POINT('',(-14.7602610286104,-54.3618122024717,2.44341967361942));
#58585=CARTESIAN_POINT('',(-14.7615328945604,-54.3619959685696,4.5));
#58586=CARTESIAN_POINT('',(-12.9355708698302,-52.8497595669186,2.));
#58587=CARTESIAN_POINT('Ctrl Pts',(-14.7617771735939,-54.3636459375188,
2.30658032638058));
#58588=CARTESIAN_POINT('Ctrl Pts',(-15.08540280583,-54.1740757700734,2.28289239463049));
#58589=CARTESIAN_POINT('Ctrl Pts',(-15.3230378955527,-53.8318500257242,
2.25920446288041));
#58590=CARTESIAN_POINT('Ctrl Pts',(-15.3806718879601,-53.4614673043247,
2.23551653113033));
#58591=CARTESIAN_POINT('Ctrl Pts',(-15.4443412427006,-53.0522985500271,
2.2093480276714));
#58592=CARTESIAN_POINT('Ctrl Pts',(-15.2883366067183,-52.6087669190161,
2.18317952421248));
#58593=CARTESIAN_POINT('Ctrl Pts',(-14.981978171922,-52.3301976113127,2.15701102075355));
#58594=CARTESIAN_POINT('Ctrl Pts',(-14.6756197371256,-52.0516283036092,
2.13084251729463));
#58595=CARTESIAN_POINT('Ctrl Pts',(-14.2189075035153,-51.9380213192134,
2.1046740138357));
#58596=CARTESIAN_POINT('Ctrl Pts',(-13.8181892890955,-52.0394181405147,
2.07850551037677));
#58597=CARTESIAN_POINT('Ctrl Pts',(-13.4174710746757,-52.140814961816,2.05233700691785));
#58598=CARTESIAN_POINT('Ctrl Pts',(-13.0727468794465,-52.4572155888145,
2.02616850345892));
#58599=CARTESIAN_POINT('Ctrl Pts',(-12.9355708698302,-52.8497595669186,
1.99999999999999));
#58600=CARTESIAN_POINT('',(-13.8936035762987,-54.5113733504501,2.));
#58601=CARTESIAN_POINT('Origin',(-14.1292828945604,-53.2669068454841,2.));
#58602=CARTESIAN_POINT('Ctrl Pts',(-13.8936031194076,-54.5113848919291,
2.));
#58603=CARTESIAN_POINT('Ctrl Pts',(-13.5065360962339,-54.4366467486624,
2.02490816038701));
#58604=CARTESIAN_POINT('Ctrl Pts',(-13.1551959025419,-54.1671648587472,
2.04981632077402));
#58605=CARTESIAN_POINT('Ctrl Pts',(-12.9858211468817,-53.8112635997049,
2.07472448116103));
#58606=CARTESIAN_POINT('Ctrl Pts',(-12.8078760955218,-53.4373538776067,
2.10089298461996));
#58607=CARTESIAN_POINT('Ctrl Pts',(-12.830777130449,-52.9680579532915,2.12706148807889));
#58608=CARTESIAN_POINT('Ctrl Pts',(-13.0443872879449,-52.6134595791442,
2.15322999153781));
#58609=CARTESIAN_POINT('Ctrl Pts',(-13.2579974454408,-52.2588612049968,
2.17939849499674));
#58610=CARTESIAN_POINT('Ctrl Pts',(-13.6623167255054,-52.0189603810172,
2.20556699845567));
#58611=CARTESIAN_POINT('Ctrl Pts',(-14.0759781319804,-52.0015075823912,
2.23173550191459));
#58612=CARTESIAN_POINT('Ctrl Pts',(-14.4896395384555,-51.9840547837653,
2.25790400537352));
#58613=CARTESIAN_POINT('Ctrl Pts',(-14.9126430713409,-52.1890500104929,
2.28407250883245));
#58614=CARTESIAN_POINT('Ctrl Pts',(-15.1553414968488,-52.5244832283522,
2.31024101229137));
#58615=CARTESIAN_POINT('Ctrl Pts',(-15.3980399223566,-52.8599164462115,
2.3364095157503));
#58616=CARTESIAN_POINT('Ctrl Pts',(-15.4604332404868,-53.3257876552024,
2.36257801920923));
#58617=CARTESIAN_POINT('Ctrl Pts',(-15.3145273105893,-53.7132383944998,
2.38874652266815));
#58618=CARTESIAN_POINT('Ctrl Pts',(-15.2129148646389,-53.9830685332266,
2.40697090631858));
#58619=CARTESIAN_POINT('Ctrl Pts',(-15.010275844201,-54.2148642023245,2.425195289969));
#58620=CARTESIAN_POINT('Ctrl Pts',(-14.7602610286104,-54.3618122024717,
2.44341967361942));
#58621=CARTESIAN_POINT('Origin',(-14.1292828945604,-53.2669068454841,0.895788276411274));
#58622=CARTESIAN_POINT('',(-14.9010968564111,-54.6052515498159,5.60421172358873));
#58623=CARTESIAN_POINT('',(-14.89962934498,-54.6010727330809,5.64578827641128));
#58624=CARTESIAN_POINT('',(-14.9007828945603,-54.6031840435235,0.895788276411274));
#58625=CARTESIAN_POINT('',(-15.2209662466057,-52.1764590205668,6.));
#58626=CARTESIAN_POINT('Ctrl Pts',(-14.89962934498,-54.6010727330809,5.64578827641128));
#58627=CARTESIAN_POINT('Ctrl Pts',(-14.6737409652706,-54.7312989825202,
5.65918483710515));
#58628=CARTESIAN_POINT('Ctrl Pts',(-13.9138866474417,-54.955646298412,5.69874990125794));
#58629=CARTESIAN_POINT('Ctrl Pts',(-12.6330342875793,-54.2971998857928,
5.76448346886966));
#58630=CARTESIAN_POINT('Ctrl Pts',(-12.4433594214856,-52.5865231455987,
5.84298897924644));
#58631=CARTESIAN_POINT('Ctrl Pts',(-13.76941659957,-51.486617996264,5.92149448962323));
#58632=CARTESIAN_POINT('Ctrl Pts',(-14.8623799894179,-51.8174664687922,
5.97383149654107));
#58633=CARTESIAN_POINT('Ctrl Pts',(-15.2209662466057,-52.1764590205668,
6.));
#58634=CARTESIAN_POINT('',(-15.6220374293776,-52.8664110852719,6.));
#58635=CARTESIAN_POINT('Origin',(-14.1292828945604,-53.2669068454841,6.));
#58636=CARTESIAN_POINT('Ctrl Pts',(-14.9010968564111,-54.6052515498159,
5.60421172358873));
#58637=CARTESIAN_POINT('Ctrl Pts',(-14.8619571740658,-54.628166857787,5.60655897483644));
#58638=CARTESIAN_POINT('Ctrl Pts',(-14.3739271072306,-54.8842868995418,
5.63507472954307));
#58639=CARTESIAN_POINT('Ctrl Pts',(-13.1774033105245,-54.8145932898247,
5.68975898770864));
#58640=CARTESIAN_POINT('Ctrl Pts',(-12.3131175991141,-53.3266332457169,
5.76826449808541));
#58641=CARTESIAN_POINT('Ctrl Pts',(-13.07802768807,-51.78491829464,5.84677000846219));
#58642=CARTESIAN_POINT('Ctrl Pts',(-14.7574918726583,-51.5760767532103,
5.92401517576706));
#58643=CARTESIAN_POINT('Ctrl Pts',(-15.4957392820493,-52.402248403584,5.97509183961299));
#58644=CARTESIAN_POINT('Ctrl Pts',(-15.6220514315181,-52.8664094746825,
6.));
#58645=CARTESIAN_POINT('Origin',(-14.1292828945604,-53.2669068454841,0.895788276411274));
#58646=CARTESIAN_POINT('',(-14.8993447411713,-54.6013457970434,5.10421172358873));
#58647=CARTESIAN_POINT('',(-14.9024169355128,-54.6041163881961,5.14578827641127));
#58648=CARTESIAN_POINT('',(-14.9007828945603,-54.6031840435235,0.895788276411274));
#58649=CARTESIAN_POINT('Ctrl Pts',(-14.9024169355128,-54.6041163881961,
5.14578827641127));
#58650=CARTESIAN_POINT('Ctrl Pts',(-14.5148361321472,-54.8241371380329,
5.16884048301825));
#58651=CARTESIAN_POINT('Ctrl Pts',(-13.4683417470894,-54.9257881846255,
5.21806119308415));
#58652=CARTESIAN_POINT('Ctrl Pts',(-12.3638311119676,-53.696734568805,5.29345040660899));
#58653=CARTESIAN_POINT('Ctrl Pts',(-12.7969355370903,-52.0313922294383,
5.37195591698576));
#58654=CARTESIAN_POINT('Ctrl Pts',(-14.424976702367,-51.4740982114769,5.45046142736254));
#58655=CARTESIAN_POINT('Ctrl Pts',(-15.7877203932888,-52.5246186608361,
5.52896693773933));
#58656=CARTESIAN_POINT('Ctrl Pts',(-15.6845839838159,-53.9480078415062,
5.59407588742224));
#58657=CARTESIAN_POINT('Ctrl Pts',(-15.1149856235702,-54.4769183144689,
5.63301633364622));
#58658=CARTESIAN_POINT('Ctrl Pts',(-14.89962934498,-54.6010727330809,5.64578827641128));
#58659=CARTESIAN_POINT('Ctrl Pts',(-14.8993447411713,-54.6013457970434,
5.10421172358873));
#58660=CARTESIAN_POINT('Ctrl Pts',(-14.6972931579988,-54.7185214822016,
5.11621462074955));
#58661=CARTESIAN_POINT('Ctrl Pts',(-13.9751327847045,-54.9521265711601,
5.15438602136929));
#58662=CARTESIAN_POINT('Ctrl Pts',(-12.6886982319545,-54.374296277089,5.21872592544796));
#58663=CARTESIAN_POINT('Ctrl Pts',(-12.4109789893208,-52.6761143673659,
5.29723143582474));
#58664=CARTESIAN_POINT('Ctrl Pts',(-13.6742819091468,-51.5077662723951,
5.37573694620152));
#58665=CARTESIAN_POINT('Ctrl Pts',(-15.3456277491901,-51.9170631330653,
5.4542424565783));
#58666=CARTESIAN_POINT('Ctrl Pts',(-15.9087950365254,-53.4884877368246,
5.53040071570737));
#58667=CARTESIAN_POINT('Ctrl Pts',(-15.2983088061438,-54.3726938586823,
5.58039047137751));
#58668=CARTESIAN_POINT('Ctrl Pts',(-14.9010968564111,-54.6052515498159,
5.60421172358873));
#58669=CARTESIAN_POINT('Origin',(-14.1292828945604,-53.2669068454841,0.895788276411274));
#58670=CARTESIAN_POINT('',(-14.9022875039252,-54.6033748953446,4.60421172358873));
#58671=CARTESIAN_POINT('',(-14.899520943644,-54.6036563213,4.64578827641127));
#58672=CARTESIAN_POINT('',(-14.9007828945603,-54.6031840435235,0.895788276411274));
#58673=CARTESIAN_POINT('Ctrl Pts',(-14.899520943644,-54.6036563213,4.64578827641127));
#58674=CARTESIAN_POINT('Ctrl Pts',(-14.7902473340007,-54.6680216226135,
4.65232762547243));
#58675=CARTESIAN_POINT('Ctrl Pts',(-14.20608207924,-54.9223430869235,4.68503547799252));
#58676=CARTESIAN_POINT('Ctrl Pts',(-12.9456280488333,-54.64551461019,4.74391183397153));
#58677=CARTESIAN_POINT('Ctrl Pts',(-12.3264734310144,-53.0400243844669,
4.82241734434831));
#58678=CARTESIAN_POINT('Ctrl Pts',(-13.324120771136,-51.638007671339,4.90092285472508));
#58679=CARTESIAN_POINT('Ctrl Pts',(-15.0438575043005,-51.6968266074015,
4.97942836510187));
#58680=CARTESIAN_POINT('Ctrl Pts',(-15.9433802614164,-53.1637305367386,
5.05793387547864));
#58681=CARTESIAN_POINT('Ctrl Pts',(-15.4295729948612,-54.2652563903719,
5.11338717924845));
#58682=CARTESIAN_POINT('Ctrl Pts',(-14.9548117824789,-54.5743730329603,
5.14267197955932));
#58683=CARTESIAN_POINT('Ctrl Pts',(-14.9024169355128,-54.6041163881961,
5.14578827641127));
#58684=CARTESIAN_POINT('Ctrl Pts',(-14.9022875039252,-54.6033748953446,
4.60421172358873));
#58685=CARTESIAN_POINT('Ctrl Pts',(-14.5374282197782,-54.8098641325902,
4.62587026666265));
#58686=CARTESIAN_POINT('Ctrl Pts',(-13.5347909686423,-54.936592528733,4.6736973131955));
#58687=CARTESIAN_POINT('Ctrl Pts',(-12.3888319545389,-53.7888545684045,
4.74769286318728));
#58688=CARTESIAN_POINT('Ctrl Pts',(-12.7339055288242,-52.1030679359729,
4.82619837356406));
#58689=CARTESIAN_POINT('Ctrl Pts',(-14.3303867955418,-51.461039661442,4.90470388394084));
#58690=CARTESIAN_POINT('Ctrl Pts',(-15.7465131069793,-52.4385560995515,
4.98320939431762));
#58691=CARTESIAN_POINT('Ctrl Pts',(-15.7175049264688,-53.8959207488069,
5.04971200753358));
#58692=CARTESIAN_POINT('Ctrl Pts',(-15.1378024352416,-54.4630571321133,
5.09004611729062));
#58693=CARTESIAN_POINT('Ctrl Pts',(-14.8993447411713,-54.6013457970434,
5.10421172358873));
#58694=CARTESIAN_POINT('Origin',(-14.1292828945604,-53.2669068454841,0.895788276411274));
#58695=CARTESIAN_POINT('',(-14.899957506564,-54.6043129428392,4.10421172358872));
#58696=CARTESIAN_POINT('',(-14.9006214745914,-54.60116105013,4.14578827641127));
#58697=CARTESIAN_POINT('',(-14.9007828945603,-54.6031840435235,0.895788276411274));
#58698=CARTESIAN_POINT('Ctrl Pts',(-14.9006214745914,-54.60116105013,4.14578827641127));
#58699=CARTESIAN_POINT('Ctrl Pts',(-14.6270809930356,-54.7571745495808,
4.16198327138554));
#58700=CARTESIAN_POINT('Ctrl Pts',(-13.7886805442009,-54.9572356101558,
4.20434676981873));
#58701=CARTESIAN_POINT('Ctrl Pts',(-12.5323678038339,-54.1337749126023,
4.27287877171085));
#58702=CARTESIAN_POINT('Ctrl Pts',(-12.5253744436601,-52.413047533365,4.35138428208763));
#58703=CARTESIAN_POINT('Ctrl Pts',(-13.9568043064156,-51.4580814834715,
4.42988979246441));
#58704=CARTESIAN_POINT('Ctrl Pts',(-15.5429170806551,-52.1253130228172,
4.50839530284119));
#58705=CARTESIAN_POINT('Ctrl Pts',(-15.8347326759058,-53.6754928499223,
4.58036146415681));
#58706=CARTESIAN_POINT('Ctrl Pts',(-15.2275273759708,-54.4104510916165,
4.62615912201351));
#58707=CARTESIAN_POINT('Ctrl Pts',(-14.899520943644,-54.6036563213,4.64578827641127));
#58708=CARTESIAN_POINT('Ctrl Pts',(-14.899957506564,-54.6043129428392,4.10421172358873));
#58709=CARTESIAN_POINT('Ctrl Pts',(-14.8140915002505,-54.654905954387,4.10935740911683));
#58710=CARTESIAN_POINT('Ctrl Pts',(-14.2627733336105,-54.9110489082195,
4.14067159810386));
#58711=CARTESIAN_POINT('Ctrl Pts',(-13.0196598476917,-54.705772943414,4.19815429054983));
#58712=CARTESIAN_POINT('Ctrl Pts',(-12.3170458706651,-53.1350132444558,
4.2766598009266));
#58713=CARTESIAN_POINT('Ctrl Pts',(-13.239689139382,-51.6825388628568,4.35516531130339));
#58714=CARTESIAN_POINT('Ctrl Pts',(-14.9601412381249,-51.6509633535717,
4.43367082168016));
#58715=CARTESIAN_POINT('Ctrl Pts',(-15.9354598188275,-53.0686043860759,
4.51217633205695));
#58716=CARTESIAN_POINT('Ctrl Pts',(-15.4687653497055,-54.223916817667,4.5690232993598));
#58717=CARTESIAN_POINT('Ctrl Pts',(-14.9782621856933,-54.5603776227797,
4.59970176320373));
#58718=CARTESIAN_POINT('Ctrl Pts',(-14.9022875039252,-54.6033748953446,
4.60421172358873));
#58719=CARTESIAN_POINT('Origin',(-14.1292828945604,-53.2669068454841,0.895788276411274));
#58720=CARTESIAN_POINT('',(-14.9001204094146,-54.6010161225549,3.60421172358873));
#58721=CARTESIAN_POINT('',(-14.9020910027761,-54.6052313123369,3.64578827641127));
#58722=CARTESIAN_POINT('',(-14.9007828945603,-54.6031840435235,0.895788276411274));
#58723=CARTESIAN_POINT('Ctrl Pts',(-14.9020910027761,-54.6052313123369,
3.64578827641127));
#58724=CARTESIAN_POINT('Ctrl Pts',(-14.4696174214115,-54.8543199357372,
3.67163891729865));
#58725=CARTESIAN_POINT('Ctrl Pts',(-13.3333022960118,-54.8966530893797,
3.72365806164495));
#58726=CARTESIAN_POINT('Ctrl Pts',(-12.3283770240505,-53.5084355106897,
3.80184570945017));
#58727=CARTESIAN_POINT('Ctrl Pts',(-12.9344615472089,-51.8979656495417,
3.88035121982696));
#58728=CARTESIAN_POINT('Ctrl Pts',(-14.612090259655,-51.5151947977304,3.95885673020373));
#58729=CARTESIAN_POINT('Ctrl Pts',(-15.8567258492822,-52.7034009548898,
4.03736224058051));
#58730=CARTESIAN_POINT('Ctrl Pts',(-15.614980939896,-54.0476036870055,4.09967275598303));
#58731=CARTESIAN_POINT('Ctrl Pts',(-15.0690783538945,-54.5050818625188,
4.13581476792661));
#58732=CARTESIAN_POINT('Ctrl Pts',(-14.9006214745914,-54.60116105013,4.14578827641127));
#58733=CARTESIAN_POINT('Ctrl Pts',(-14.9001204094146,-54.6010161225549,
3.60421172358873));
#58734=CARTESIAN_POINT('Ctrl Pts',(-14.6502875315042,-54.7442481097626,
3.61901305502994));
#58735=CARTESIAN_POINT('Ctrl Pts',(-13.8515268344553,-54.9574092639254,
3.65998288993008));
#58736=CARTESIAN_POINT('Ctrl Pts',(-12.5800953694062,-54.216441978079,3.72712122828915));
#58737=CARTESIAN_POINT('Ctrl Pts',(-12.482746426243,-52.4984560584276,3.80562673866593));
#58738=CARTESIAN_POINT('Ctrl Pts',(-13.8620505314459,-51.4696350750294,
3.88413224904271));
#58739=CARTESIAN_POINT('Ctrl Pts',(-15.4810149732843,-52.0526501422855,
3.96263775941948));
#58740=CARTESIAN_POINT('Ctrl Pts',(-15.8610566498332,-53.6150480556464,
4.03599758426816));
#58741=CARTESIAN_POINT('Ctrl Pts',(-15.2507650728867,-54.397614017199,4.0831889056579));
#58742=CARTESIAN_POINT('Ctrl Pts',(-14.899957506564,-54.6043129428392,4.10421172358873));
#58743=CARTESIAN_POINT('Origin',(-14.1292828945604,-53.2669068454841,0.895788276411274));
#58744=CARTESIAN_POINT('',(-14.9023562176693,-54.604775754849,3.10421172358873));
#58745=CARTESIAN_POINT('',(-14.8991095940519,-54.6023050298359,3.14578827641127));
#58746=CARTESIAN_POINT('',(-14.9007828945603,-54.6031840435235,0.895788276411274));
#58747=CARTESIAN_POINT('Ctrl Pts',(-14.8991095940519,-54.6023050298359,
3.14578827641127));
#58748=CARTESIAN_POINT('Ctrl Pts',(-14.7424882378679,-54.6940222226685,
3.15512605975283));
#58749=CARTESIAN_POINT('Ctrl Pts',(-14.0895244416362,-54.9406197878808,
3.19063234655331));
#58750=CARTESIAN_POINT('Ctrl Pts',(-12.8070376180166,-54.5132075415871,
3.25230713681272));
#58751=CARTESIAN_POINT('Ctrl Pts',(-12.3603879600184,-52.8514447189325,
3.3308126471895));
#58752=CARTESIAN_POINT('Ctrl Pts',(-13.5001253542918,-51.5622781929174,
3.40931815756628));
#58753=CARTESIAN_POINT('Ctrl Pts',(-15.2041061771209,-51.8018631754771,
3.48782366794306));
#58754=CARTESIAN_POINT('Ctrl Pts',(-15.944159933136,-53.3553341468671,3.56632917831984));
#58755=CARTESIAN_POINT('Ctrl Pts',(-15.3488521474601,-54.3440811110855,
3.61898404780924));
#58756=CARTESIAN_POINT('Ctrl Pts',(-14.9074087496474,-54.6021684888377,
3.64547041383972));
#58757=CARTESIAN_POINT('Ctrl Pts',(-14.9020910027761,-54.6052313123369,
3.64578827641127));
#58758=CARTESIAN_POINT('Ctrl Pts',(-14.9023562176693,-54.604775754849,3.10421172358873));
#58759=CARTESIAN_POINT('Ctrl Pts',(-14.4921270687778,-54.8390095809862,
3.12866870094305));
#58760=CARTESIAN_POINT('Ctrl Pts',(-13.4008007460488,-54.9124362051017,
3.1792941817563));
#58761=CARTESIAN_POINT('Ctrl Pts',(-12.3435458814549,-53.6026781745395,
3.25608816602847));
#58762=CARTESIAN_POINT('Ctrl Pts',(-12.8642192037885,-51.9626013374103,
3.33459367640525));
#58763=CARTESIAN_POINT('Ctrl Pts',(-14.5194316817766,-51.4922567887358,
3.41309918678203));
#58764=CARTESIAN_POINT('Ctrl Pts',(-15.824749470772,-52.6134605506407,3.49160469715881));
#58765=CARTESIAN_POINT('Ctrl Pts',(-15.6501092546376,-53.9988114930956,
3.55530887609438));
#58766=CARTESIAN_POINT('Ctrl Pts',(-15.091987830948,-54.4910163807415,3.59284455157101));
#58767=CARTESIAN_POINT('Ctrl Pts',(-14.9001204094146,-54.6010161225549,
3.60421172358873));
#58768=CARTESIAN_POINT('Origin',(-14.1292828945604,-53.2669068454841,0.895788276411274));
#58769=CARTESIAN_POINT('',(-14.8992309062956,-54.6029598038327,2.60421172358873));
#58770=CARTESIAN_POINT('',(-14.9016274172746,-54.6020379108679,2.64578827641127));
#58771=CARTESIAN_POINT('',(-14.9007828945603,-54.6031840435235,0.895788276411274));
#58772=CARTESIAN_POINT('Ctrl Pts',(-14.9016274172746,-54.6020379108679,
2.64578827641127));
#58773=CARTESIAN_POINT('Ctrl Pts',(-14.5809116606719,-54.7836391180053,
2.66478170566594));
#58774=CARTESIAN_POINT('Ctrl Pts',(-13.6600505366298,-54.9508125591569,
2.70994363837953));
#58775=CARTESIAN_POINT('Ctrl Pts',(-12.4499634166736,-53.960794947638,2.78127407455204));
#58776=CARTESIAN_POINT('Ctrl Pts',(-12.6242053254302,-52.2488988977254,
2.85977958492882));
#58777=CARTESIAN_POINT('Ctrl Pts',(-14.1482380059646,-51.4499755676755,
2.93828509530561));
#58778=CARTESIAN_POINT('Ctrl Pts',(-15.6552705807332,-52.2805199058824,
3.01679060568238));
#58779=CARTESIAN_POINT('Ctrl Pts',(-15.777288771741,-53.7916708150444,3.08595833271761));
#58780=CARTESIAN_POINT('Ctrl Pts',(-15.1814089486113,-54.4369910204986,
3.1289575562939));
#58781=CARTESIAN_POINT('Ctrl Pts',(-14.8991095940519,-54.6023050298359,
3.14578827641127));
#58782=CARTESIAN_POINT('Ctrl Pts',(-14.8992309062956,-54.6029598038327,
2.60421172358873));
#58783=CARTESIAN_POINT('Ctrl Pts',(-14.7662449521696,-54.681123251708,2.61215584339723));
#58784=CARTESIAN_POINT('Ctrl Pts',(-14.1480244437874,-54.9322850073565,
2.64626846666466));
#58785=CARTESIAN_POINT('Ctrl Pts',(-12.8743150895914,-54.5809192738243,
2.70654959339101));
#58786=CARTESIAN_POINT('Ctrl Pts',(-12.3410089780029,-52.9449163922479,
2.7850551037678));
#58787=CARTESIAN_POINT('Ctrl Pts',(-13.4114743235374,-51.5976690199096,
2.86356061414457));
#58788=CARTESIAN_POINT('Ctrl Pts',(-15.125685020798,-51.7474403844543,2.94206612452135));
#58789=CARTESIAN_POINT('Ctrl Pts',(-15.9462998191018,-53.2599021194416,
3.02057163489813));
#58790=CARTESIAN_POINT('Ctrl Pts',(-15.3893775359764,-54.3055097335425,
3.07462016792059));
#58791=CARTESIAN_POINT('Ctrl Pts',(-14.9310645035309,-54.5883838147409,
3.10250019748412));
#58792=CARTESIAN_POINT('Ctrl Pts',(-14.9023562176693,-54.604775754849,3.10421172358873));
#58793=CARTESIAN_POINT('Origin',(-14.1292828945604,-53.2669068454841,0.895788276411274));
#58794=CARTESIAN_POINT('',(-14.9013089558621,-54.6009691165979,2.10421172358873));
#58795=CARTESIAN_POINT('',(-14.9010809748678,-54.6051974101417,2.14578827641127));
#58796=CARTESIAN_POINT('',(-14.9007828945603,-54.6031840435235,0.895788276411274));
#58797=CARTESIAN_POINT('',(-15.6194800884629,-52.866705242183,2.));
#58798=CARTESIAN_POINT('Ctrl Pts',(-15.6194800884629,-52.866705242183,2.));
#58799=CARTESIAN_POINT('Ctrl Pts',(-15.7510836294753,-53.3567463262429,
2.02616850345893));
#58800=CARTESIAN_POINT('Ctrl Pts',(-15.5785415188313,-54.0947786094125,
2.06090574465517));
#58801=CARTESIAN_POINT('Ctrl Pts',(-15.0460508163988,-54.5187167298269,
2.09564298585141));
#58802=CARTESIAN_POINT('Ctrl Pts',(-14.9013089558621,-54.6009691165979,
2.10421172358873));
#58803=CARTESIAN_POINT('',(-15.2224998162609,-52.1743915631094,2.));
#58804=CARTESIAN_POINT('Origin',(-14.1292828945604,-53.2669068454841,2.));
#58805=CARTESIAN_POINT('Ctrl Pts',(-15.2225082026616,-52.1743802571171,
2.));
#58806=CARTESIAN_POINT('Ctrl Pts',(-15.5613276195564,-52.5158503863372,
2.02490816038701));
#58807=CARTESIAN_POINT('Ctrl Pts',(-15.8908670066042,-53.5171650620887,
2.0735042525241));
#58808=CARTESIAN_POINT('Ctrl Pts',(-15.2959835850222,-54.3738753315586,
2.12210034466119));
#58809=CARTESIAN_POINT('Ctrl Pts',(-14.9010809748678,-54.6051974101417,
2.14578827641127));
#58810=CARTESIAN_POINT('Origin',(39.0658530619283,-38.8697713466883,4.5));
#58811=CARTESIAN_POINT('',(39.6970780592612,-39.9631802546368,5.80658032638059));
#58812=CARTESIAN_POINT('',(39.6962628554159,-39.965015558984,5.94341967361942));
#58813=CARTESIAN_POINT('',(39.6981030619283,-39.9648604697737,4.5));
#58814=CARTESIAN_POINT('',(40.2595650866584,-39.2869186252538,6.));
#58815=CARTESIAN_POINT('Ctrl Pts',(39.6962628554159,-39.965015558984,5.94341967361942));
#58816=CARTESIAN_POINT('Ctrl Pts',(39.9540142218037,-39.8131911161898,5.96227978241295));
#58817=CARTESIAN_POINT('Ctrl Pts',(40.160699881421,-39.5698320958276,5.98113989120648));
#58818=CARTESIAN_POINT('Ctrl Pts',(40.2595650866584,-39.2869186252538,6.00000000000001));
#58819=CARTESIAN_POINT('',(39.6981030619283,-39.9648604697737,6.));
#58820=CARTESIAN_POINT('Origin',(39.0658530619283,-38.8697713466883,6.));
#58821=CARTESIAN_POINT('',(39.6981030619283,-39.9648604697737,7.));
#58822=CARTESIAN_POINT('',(39.6981030619283,-39.9648604697737,4.5));
#58823=CARTESIAN_POINT('',(39.7608672580761,-37.8134023216062,7.));
#58824=CARTESIAN_POINT('Origin',(39.0658530619283,-38.8697713466883,7.));
#58825=CARTESIAN_POINT('',(38.3708388657804,-39.9261403717704,7.));
#58826=CARTESIAN_POINT('Origin',(39.0658530619283,-38.8697713466883,7.));
#58827=CARTESIAN_POINT('Origin',(39.0658530619283,-38.8697713466883,7.));
#58828=CARTESIAN_POINT('',(39.3015291113281,-37.6253036020567,6.));
#58829=CARTESIAN_POINT('Origin',(39.0658530619283,-38.8697713466883,6.));
#58830=CARTESIAN_POINT('Ctrl Pts',(39.3015295597332,-37.6252918061955,6.));
#58831=CARTESIAN_POINT('Ctrl Pts',(39.6885932560667,-37.7000310216234,5.97509183961299));
#58832=CARTESIAN_POINT('Ctrl Pts',(40.039943062479,-37.9695097738977,5.95018367922598));
#58833=CARTESIAN_POINT('Ctrl Pts',(40.2093203959796,-38.325411392646,5.92527551883897));
#58834=CARTESIAN_POINT('Ctrl Pts',(40.3872681556176,-38.6993214926512,5.89910701538004));
#58835=CARTESIAN_POINT('Ctrl Pts',(40.3643620641527,-39.1686216551033,5.87293851192112));
#58836=CARTESIAN_POINT('Ctrl Pts',(40.1507501683313,-39.5232214807692,5.84677000846219));
#58837=CARTESIAN_POINT('Ctrl Pts',(40.0413948614145,-39.7047533782285,5.83337344776832));
#58838=CARTESIAN_POINT('Ctrl Pts',(39.8820599551598,-39.8562249589825,5.81997688707446));
#58839=CARTESIAN_POINT('Ctrl Pts',(39.6970780592612,-39.9631802546368,5.80658032638059));
#58840=CARTESIAN_POINT('Origin',(39.0658530619283,-38.8697713466883,4.5));
#58841=CARTESIAN_POINT('',(39.6980969738518,-39.9664052404928,5.30658032638059));
#58842=CARTESIAN_POINT('',(39.6994431549996,-39.9659335873643,5.44341967361942));
#58843=CARTESIAN_POINT('',(39.6981030619283,-39.9648604697737,4.5));
#58844=CARTESIAN_POINT('Ctrl Pts',(39.6994431549996,-39.9659335873643,5.44341967361942));
#58845=CARTESIAN_POINT('Ctrl Pts',(39.7317442057588,-39.9475451778339,5.44576692486713));
#58846=CARTESIAN_POINT('Ctrl Pts',(39.7631672715511,-39.9276731785138,5.44811417611484));
#58847=CARTESIAN_POINT('Ctrl Pts',(39.7935612952928,-39.9063356334613,5.45046142736255));
#58848=CARTESIAN_POINT('Ctrl Pts',(40.1324113081288,-39.6684524404899,5.47662993082147));
#58849=CARTESIAN_POINT('Ctrl Pts',(40.3433609694206,-39.2484155500404,5.5027984342804));
#58850=CARTESIAN_POINT('Ctrl Pts',(40.3318541433896,-38.8345478072092,5.52896693773932));
#58851=CARTESIAN_POINT('Ctrl Pts',(40.3203473173586,-38.420680064378,5.55513544119825));
#58852=CARTESIAN_POINT('Ctrl Pts',(40.086384004005,-38.0129814691652,5.58130394465718));
#58853=CARTESIAN_POINT('Ctrl Pts',(39.7348031115542,-37.794322753355,5.60747244811611));
#58854=CARTESIAN_POINT('Ctrl Pts',(39.3832222191033,-37.5756640375447,5.63364095157504));
#58855=CARTESIAN_POINT('Ctrl Pts',(38.9140237475553,-37.5460452011372,5.65980945503396));
#58856=CARTESIAN_POINT('Ctrl Pts',(38.5377492251912,-37.7186390805662,5.68597795849288));
#58857=CARTESIAN_POINT('Ctrl Pts',(38.161474702827,-37.8912329599952,5.71214646195181));
#58858=CARTESIAN_POINT('Ctrl Pts',(37.8781241296467,-38.2660395552607,5.73831496541074));
#58859=CARTESIAN_POINT('Ctrl Pts',(37.814457003614,-38.6752103329025,5.76448346886967));
#58860=CARTESIAN_POINT('Ctrl Pts',(37.7507898775812,-39.0843811105442,5.79065197232859));
#58861=CARTESIAN_POINT('Ctrl Pts',(37.9068061986959,-39.5279160705621,5.81682047578752));
#58862=CARTESIAN_POINT('Ctrl Pts',(38.2131591663055,-39.8064837741936,5.84298897924645));
#58863=CARTESIAN_POINT('Ctrl Pts',(38.5195121339151,-40.0850514778251,5.86915748270537));
#58864=CARTESIAN_POINT('Ctrl Pts',(38.9762017480197,-40.1986519250703,5.8953259861643));
#58865=CARTESIAN_POINT('Ctrl Pts',(39.3769209838014,-40.0972547064535,5.92149448962322));
#58866=CARTESIAN_POINT('Ctrl Pts',(39.4888346944845,-40.0689362780501,5.92880288428862));
#58867=CARTESIAN_POINT('Ctrl Pts',(39.596382800018,-40.0238483557585,5.93611127895402));
#58868=CARTESIAN_POINT('Ctrl Pts',(39.6962628554159,-39.965015558984,5.94341967361942));
#58869=CARTESIAN_POINT('Ctrl Pts',(39.6970780592612,-39.9631802546368,5.80658032638059));
#58870=CARTESIAN_POINT('Ctrl Pts',(39.5207209896389,-40.0651487333929,5.79380838361553));
#58871=CARTESIAN_POINT('Ctrl Pts',(39.3210527704035,-40.1266553179232,5.78103644085048));
#58872=CARTESIAN_POINT('Ctrl Pts',(39.1191586941911,-40.1351732662231,5.76826449808542));
#58873=CARTESIAN_POINT('Ctrl Pts',(38.7054968160504,-40.1526257371314,5.74209599462649));
#58874=CARTESIAN_POINT('Ctrl Pts',(38.2824907599468,-39.9476311900682,5.71592749116756));
#58875=CARTESIAN_POINT('Ctrl Pts',(38.0397913612151,-39.6121973316472,5.68975898770864));
#58876=CARTESIAN_POINT('Ctrl Pts',(37.7970919624834,-39.2767634732261,5.66359048424971));
#58877=CARTESIAN_POINT('Ctrl Pts',(37.7346992211236,-38.8108903034472,5.63742198079078));
#58878=CARTESIAN_POINT('Ctrl Pts',(37.8806057126089,-38.4234383862029,5.61125347733185));
#58879=CARTESIAN_POINT('Ctrl Pts',(38.0265122040942,-38.0359864689587,5.58508497387293));
#58880=CARTESIAN_POINT('Ctrl Pts',(38.3807179284248,-37.7269558042492,5.558916470414));
#58881=CARTESIAN_POINT('Ctrl Pts',(38.7843854256713,-37.6349404921319,5.53274796695507));
#58882=CARTESIAN_POINT('Ctrl Pts',(39.1880529229179,-37.5429251800145,5.50657946349615));
#58883=CARTESIAN_POINT('Ctrl Pts',(39.6411821930806,-37.6679252204893,5.48041096003722));
#58884=CARTESIAN_POINT('Ctrl Pts',(39.9405883560671,-37.9538786579723,5.4542424565783));
#58885=CARTESIAN_POINT('Ctrl Pts',(40.2399945190535,-38.2398320954553,5.42807395311937));
#58886=CARTESIAN_POINT('Ctrl Pts',(40.3856775748639,-38.6867389299466,5.40190544966044));
#58887=CARTESIAN_POINT('Ctrl Pts',(40.3123096892109,-39.0942060073491,5.37573694620152));
#58888=CARTESIAN_POINT('Ctrl Pts',(40.2476788760258,-39.4531495468055,5.35268473959454));
#58889=CARTESIAN_POINT('Ctrl Pts',(40.0130623748058,-39.7814874463141,5.32963253298756));
#58890=CARTESIAN_POINT('Ctrl Pts',(39.6980969738518,-39.9664052404928,5.30658032638059));
#58891=CARTESIAN_POINT('Origin',(39.0658530619283,-38.8697713466883,4.5));
#58892=CARTESIAN_POINT('',(39.6989570949588,-39.9641614067485,4.80658032638058));
#58893=CARTESIAN_POINT('',(39.697389467188,-39.9630895992609,4.94341967361942));
#58894=CARTESIAN_POINT('',(39.6981030619283,-39.9648604697737,4.5));
#58895=CARTESIAN_POINT('Ctrl Pts',(39.697389467188,-39.9630895992609,4.94341967361942));
#58896=CARTESIAN_POINT('Ctrl Pts',(39.8633425703643,-39.8677036169061,4.95542257078024));
#58897=CARTESIAN_POINT('Ctrl Pts',(40.0085235722312,-39.7366393919842,4.96742546794105));
#58898=CARTESIAN_POINT('Ctrl Pts',(40.1149177943607,-39.5793405247057,4.97942836510187));
#58899=CARTESIAN_POINT('Ctrl Pts',(40.3468765900167,-39.2364003247431,5.0055968685608));
#58900=CARTESIAN_POINT('Ctrl Pts',(40.3944742703015,-38.7687617621182,5.03176537201972));
#58901=CARTESIAN_POINT('Ctrl Pts',(40.2363680070802,-38.3861191307629,5.05793387547865));
#58902=CARTESIAN_POINT('Ctrl Pts',(40.0782617438588,-38.0034764994076,5.08410237893758));
#58903=CARTESIAN_POINT('Ctrl Pts',(39.7144515371312,-37.705829799322,5.11027088239651));
#58904=CARTESIAN_POINT('Ctrl Pts',(39.3080731239833,-37.626648148232,5.13643938585543));
#58905=CARTESIAN_POINT('Ctrl Pts',(38.9016947108354,-37.5474664971421,5.16260788931436));
#58906=CARTESIAN_POINT('Ctrl Pts',(38.4527480912673,-37.6867498950479,5.18877639277328));
#58907=CARTESIAN_POINT('Ctrl Pts',(38.1625484528667,-37.982040398373,5.21494489623221));
#58908=CARTESIAN_POINT('Ctrl Pts',(37.8723488144661,-38.2773309016981,5.24111339969114));
#58909=CARTESIAN_POINT('Ctrl Pts',(37.7408961572331,-38.7286285104427,5.26728190315006));
#58910=CARTESIAN_POINT('Ctrl Pts',(37.8271310042327,-39.1335692645202,5.29345040660899));
#58911=CARTESIAN_POINT('Ctrl Pts',(37.9133658512322,-39.5385100185978,5.31961891006792));
#58912=CARTESIAN_POINT('Ctrl Pts',(38.2172882024643,-39.8970939180085,5.34578741352684));
#58913=CARTESIAN_POINT('Ctrl Pts',(38.6026245602704,-40.0485211199672,5.37195591698577));
#58914=CARTESIAN_POINT('Ctrl Pts',(38.9533971820163,-40.1863656694333,5.39577716919699));
#58915=CARTESIAN_POINT('Ctrl Pts',(39.3716335617261,-40.1525497161724,5.4195984214082));
#58916=CARTESIAN_POINT('Ctrl Pts',(39.6994431549996,-39.9659335873643,5.44341967361942));
#58917=CARTESIAN_POINT('Ctrl Pts',(39.6980969738518,-39.9664052404928,5.30658032638059));
#58918=CARTESIAN_POINT('Ctrl Pts',(39.6555185906107,-39.9914032265725,5.30346402952864));
#58919=CARTESIAN_POINT('Ctrl Pts',(39.6114718472881,-40.0137802388959,5.30034773267669));
#58920=CARTESIAN_POINT('Ctrl Pts',(39.5661781885583,-40.0332575731161,5.29723143582474));
#58921=CARTESIAN_POINT('Ctrl Pts',(39.1858334006749,-40.1968147411666,5.27106293236581));
#58922=CARTESIAN_POINT('Ctrl Pts',(38.7175626520242,-40.1559017569539,5.24489442890688));
#58923=CARTESIAN_POINT('Ctrl Pts',(38.3713436649214,-39.928865763386,5.21872592544795));
#58924=CARTESIAN_POINT('Ctrl Pts',(38.0251246778187,-39.701829769818,5.19255742198903));
#58925=CARTESIAN_POINT('Ctrl Pts',(37.8009574522638,-39.2886707668948,5.1663889185301));
#58926=CARTESIAN_POINT('Ctrl Pts',(37.7993614588042,-38.8746535306862,5.14022041507118));
#58927=CARTESIAN_POINT('Ctrl Pts',(37.7977654653446,-38.4606362944777,5.11405191161225));
#58928=CARTESIAN_POINT('Ctrl Pts',(38.0187407039802,-38.0457608249837,5.08788340815333));
#58929=CARTESIAN_POINT('Ctrl Pts',(38.3631991409407,-37.8160625276688,5.0617149046944));
#58930=CARTESIAN_POINT('Ctrl Pts',(38.7076575779013,-37.5863642303539,5.03554640123547));
#58931=CARTESIAN_POINT('Ctrl Pts',(39.1755992131867,-37.5418431052182,5.00937789777654));
#58932=CARTESIAN_POINT('Ctrl Pts',(39.5571935097811,-37.7024627985796,4.98320939431762));
#58933=CARTESIAN_POINT('Ctrl Pts',(39.9387878063755,-37.863082491941,4.95704089085869));
#58934=CARTESIAN_POINT('Ctrl Pts',(40.2340347642788,-38.2288430037996,4.93087238739977));
#58935=CARTESIAN_POINT('Ctrl Pts',(40.3105421109525,-38.635733049973,4.90470388394084));
#58936=CARTESIAN_POINT('Ctrl Pts',(40.3870494576263,-39.0426230961465,4.87853538048192));
#58937=CARTESIAN_POINT('Ctrl Pts',(40.2448171930704,-39.4906426766349,4.85236687702299));
#58938=CARTESIAN_POINT('Ctrl Pts',(39.9476239688235,-39.7788944478041,4.82619837356406));
#58939=CARTESIAN_POINT('Ctrl Pts',(39.8733571986578,-39.8509268034997,4.8196590245029));
#58940=CARTESIAN_POINT('Ctrl Pts',(39.7894135884089,-39.9129821459893,4.81311967544174));
#58941=CARTESIAN_POINT('Ctrl Pts',(39.6989570949588,-39.9641614067485,4.80658032638058));
#58942=CARTESIAN_POINT('Origin',(39.0658530619283,-38.8697713466883,4.5));
#58943=CARTESIAN_POINT('',(39.6967352121902,-39.9639200225483,4.30658032638058));
#58944=CARTESIAN_POINT('',(39.6976237458347,-39.9660095563765,4.44341967361942));
#58945=CARTESIAN_POINT('',(39.6981030619283,-39.9648604697737,4.5));
#58946=CARTESIAN_POINT('Ctrl Pts',(39.6976237458347,-39.9660095563765,4.44341967361942));
#58947=CARTESIAN_POINT('Ctrl Pts',(39.9936753773632,-39.7916729655961,4.46507821669334));
#58948=CARTESIAN_POINT('Ctrl Pts',(40.2204527828214,-39.4929448719807,4.48673675976727));
#58949=CARTESIAN_POINT('Ctrl Pts',(40.2988032317419,-39.159355592007,4.50839530284119));
#58950=CARTESIAN_POINT('Ctrl Pts',(40.393468601734,-38.756302986065,4.53456380630012));
#58951=CARTESIAN_POINT('Ctrl Pts',(40.2714573392084,-38.3023593247387,4.56073230975905));
#58952=CARTESIAN_POINT('Ctrl Pts',(39.9874807525881,-38.0010783358291,4.58690081321797));
#58953=CARTESIAN_POINT('Ctrl Pts',(39.7035041659678,-37.6997973469195,4.6130693166769));
#58954=CARTESIAN_POINT('Ctrl Pts',(39.2575622552528,-37.5511790304267,4.63923782013583));
#58955=CARTESIAN_POINT('Ctrl Pts',(38.8496206579412,-37.6218656179337,4.66540632359475));
#58956=CARTESIAN_POINT('Ctrl Pts',(38.4416790606296,-37.6925522054406,4.69157482705368));
#58957=CARTESIAN_POINT('Ctrl Pts',(38.0717377767213,-37.9825436969474,4.71774333051261));
#58958=CARTESIAN_POINT('Ctrl Pts',(37.9056829078162,-38.3618044366461,4.74391183397153));
#58959=CARTESIAN_POINT('Ctrl Pts',(37.739628038911,-38.7410651763447,4.77008033743046));
#58960=CARTESIAN_POINT('Ctrl Pts',(37.7774595850089,-39.2095951642353,4.79624884088938));
#58961=CARTESIAN_POINT('Ctrl Pts',(38.0022133656485,-39.5573000327044,4.82241734434831));
#58962=CARTESIAN_POINT('Ctrl Pts',(38.2269671462881,-39.9050049011735,4.84858584780724));
#58963=CARTESIAN_POINT('Ctrl Pts',(38.6386431614693,-40.1318846502211,4.87475435126617));
#58964=CARTESIAN_POINT('Ctrl Pts',(39.0526411245735,-40.1362036060948,4.90092285472509));
#58965=CARTESIAN_POINT('Ctrl Pts',(39.2767476411253,-40.1385415551725,4.9150884610232));
#58966=CARTESIAN_POINT('Ctrl Pts',(39.5015345588232,-40.0756624434911,4.92925406732131));
#58967=CARTESIAN_POINT('Ctrl Pts',(39.697389467188,-39.9630895992609,4.94341967361942));
#58968=CARTESIAN_POINT('Ctrl Pts',(39.6989570949588,-39.9641614067485,4.80658032638058));
#58969=CARTESIAN_POINT('Ctrl Pts',(39.4274339724573,-40.1177861180175,4.78695117198281));
#58970=CARTESIAN_POINT('Ctrl Pts',(39.0972285087862,-40.1734152228909,4.76732201758505));
#58971=CARTESIAN_POINT('Ctrl Pts',(38.7939127211062,-40.1067326165456,4.74769286318728));
#58972=CARTESIAN_POINT('Ctrl Pts',(38.389548881574,-40.0178350522677,4.72152435972836));
#58973=CARTESIAN_POINT('Ctrl Pts',(38.0329753864477,-39.7115559618618,4.69535585626943));
#58974=CARTESIAN_POINT('Ctrl Pts',(37.8840840327675,-39.3252345207529,4.6691873528105));
#58975=CARTESIAN_POINT('Ctrl Pts',(37.7351926790873,-38.938913079644,4.64301884935158));
#58976=CARTESIAN_POINT('Ctrl Pts',(37.7939834668531,-38.472549287832,4.61685034589265));
#58977=CARTESIAN_POINT('Ctrl Pts',(38.0340939063583,-38.1352662178079,4.59068184243372));
#58978=CARTESIAN_POINT('Ctrl Pts',(38.2742043458635,-37.7979831477838,4.56451333897479));
#58979=CARTESIAN_POINT('Ctrl Pts',(38.6956344371082,-37.5897807995474,4.53834483551587));
#58980=CARTESIAN_POINT('Ctrl Pts',(39.1094099185268,-37.6040195786007,4.51217633205694));
#58981=CARTESIAN_POINT('Ctrl Pts',(39.5231853999454,-37.6182583576541,4.48600782859802));
#58982=CARTESIAN_POINT('Ctrl Pts',(39.929306271538,-37.854938263997,4.45983932513909));
#58983=CARTESIAN_POINT('Ctrl Pts',(40.1456631065934,-38.2079292154005,4.43367082168016));
#58984=CARTESIAN_POINT('Ctrl Pts',(40.3620199416489,-38.560920166804,4.40750231822124));
#58985=CARTESIAN_POINT('Ctrl Pts',(40.3886127401672,-39.030222163268,4.38133381476231));
#58986=CARTESIAN_POINT('Ctrl Pts',(40.2135169753906,-39.4053946105007,4.35516531130339));
#58987=CARTESIAN_POINT('Ctrl Pts',(40.1051548355753,-39.6375789196628,4.33897031632912));
#58988=CARTESIAN_POINT('Ctrl Pts',(39.9195450710429,-39.8337111891107,4.32277532135485));
#58989=CARTESIAN_POINT('Ctrl Pts',(39.6967352121902,-39.9639200225483,4.30658032638058));
#58990=CARTESIAN_POINT('Origin',(39.0658530619283,-38.8697713466883,4.5));
#58991=CARTESIAN_POINT('',(39.6990217970716,-39.9666307803348,3.80658032638058));
#58992=CARTESIAN_POINT('',(39.6992442211058,-39.9647402889406,3.94341967361942));
#58993=CARTESIAN_POINT('',(39.6981030619283,-39.9648604697737,4.5));
#58994=CARTESIAN_POINT('Ctrl Pts',(39.6992442211058,-39.9647402889406,3.94341967361942));
#58995=CARTESIAN_POINT('Ctrl Pts',(39.7703349168266,-39.9245305221536,3.94856535914752));
#58996=CARTESIAN_POINT('Ctrl Pts',(39.8373290103597,-39.877480560471,3.95371104467563));
#58997=CARTESIAN_POINT('Ctrl Pts',(39.8986640775363,-39.8239468894644,3.95885673020374));
#58998=CARTESIAN_POINT('Ctrl Pts',(40.2105849885204,-39.551700160189,3.98502523366267));
#58999=CARTESIAN_POINT('Ctrl Pts',(40.3761490651667,-39.1117681946799,4.01119373712159));
#59000=CARTESIAN_POINT('Ctrl Pts',(40.3211154074002,-38.7014217157033,4.03736224058052));
#59001=CARTESIAN_POINT('Ctrl Pts',(40.2660817496338,-38.2910752367267,4.06353074403944));
#59002=CARTESIAN_POINT('Ctrl Pts',(39.9904503574547,-37.9103142442825,4.08969924749837));
#59003=CARTESIAN_POINT('Ctrl Pts',(39.6178176236238,-37.7298764933343,4.1158677509573));
#59004=CARTESIAN_POINT('Ctrl Pts',(39.245184889793,-37.5494387423861,4.14203625441622));
#59005=CARTESIAN_POINT('Ctrl Pts',(38.7755508143104,-37.5693242329338,4.16820475787515));
#59006=CARTESIAN_POINT('Ctrl Pts',(38.4195048988346,-37.780616074816,4.19437326133408));
#59007=CARTESIAN_POINT('Ctrl Pts',(38.0634589833589,-37.9919079166982,4.220541764793));
#59008=CARTESIAN_POINT('Ctrl Pts',(37.82100122789,-38.3946061099149,4.24671026825193));
#59009=CARTESIAN_POINT('Ctrl Pts',(37.8008525725161,-38.8081359974719,4.27287877171085));
#59010=CARTESIAN_POINT('Ctrl Pts',(37.7807039171421,-39.221665885029,4.29904727516978));
#59011=CARTESIAN_POINT('Ctrl Pts',(37.9828643618631,-39.6460274669263,4.32521577862871));
#59012=CARTESIAN_POINT('Ctrl Pts',(38.3166827592479,-39.8909319662484,4.35138428208763));
#59013=CARTESIAN_POINT('Ctrl Pts',(38.6505011566327,-40.1358364655705,4.37755278554656));
#59014=CARTESIAN_POINT('Ctrl Pts',(39.1159775066813,-40.2012838823174,4.40372128900549));
#59015=CARTESIAN_POINT('Ctrl Pts',(39.5043866829606,-40.057926815412,4.42988979246442));
#59016=CARTESIAN_POINT('Ctrl Pts',(39.571326315215,-40.0332202175102,4.43439975284942));
#59017=CARTESIAN_POINT('Ctrl Pts',(39.6359768878004,-40.0023116804572,4.43890971323442));
#59018=CARTESIAN_POINT('Ctrl Pts',(39.6976237458347,-39.9660095563765,4.44341967361942));
#59019=CARTESIAN_POINT('Ctrl Pts',(39.6967352121902,-39.9639200225483,4.30658032638058));
#59020=CARTESIAN_POINT('Ctrl Pts',(39.5595202256301,-40.0441076920802,4.29660681789592));
#59021=CARTESIAN_POINT('Ctrl Pts',(39.4081968207292,-40.0992933977544,4.28663330941126));
#59022=CARTESIAN_POINT('Ctrl Pts',(39.2521185625475,-40.1225003286186,4.2766598009266));
#59023=CARTESIAN_POINT('Ctrl Pts',(38.8426002425525,-40.1833907015023,4.25049129746768));
#59024=CARTESIAN_POINT('Ctrl Pts',(38.4003479306342,-40.0241285492683,4.22432279400875));
#59025=CARTESIAN_POINT('Ctrl Pts',(38.1236728204874,-39.7161289139554,4.19815429054983));
#59026=CARTESIAN_POINT('Ctrl Pts',(37.8469977103406,-39.4081292786425,4.1719857870909));
#59027=CARTESIAN_POINT('Ctrl Pts',(37.7358998019653,-38.9513921602507,4.14581728363197));
#59028=CARTESIAN_POINT('Ctrl Pts',(37.840196718037,-38.5507239118952,4.11964878017305));
#59029=CARTESIAN_POINT('Ctrl Pts',(37.9444936341086,-38.1500556635397,4.09348027671412));
#59030=CARTESIAN_POINT('Ctrl Pts',(38.2641853746271,-37.8054562852204,4.06731177325519));
#59031=CARTESIAN_POINT('Ctrl Pts',(38.6559183630714,-37.6714482343174,4.04114326979627));
#59032=CARTESIAN_POINT('Ctrl Pts',(39.0476513515157,-37.5374401834144,4.01497476633734));
#59033=CARTESIAN_POINT('Ctrl Pts',(39.5114255878859,-37.6140234599277,3.98880626287842));
#59034=CARTESIAN_POINT('Ctrl Pts',(39.8392791917195,-37.8668572123836,3.96263775941949));
#59035=CARTESIAN_POINT('Ctrl Pts',(40.1671327955531,-38.1196909648395,3.93646925596056));
#59036=CARTESIAN_POINT('Ctrl Pts',(40.3590657668502,-38.548775193238,3.91030075250163));
#59037=CARTESIAN_POINT('Ctrl Pts',(40.3290130799472,-38.9617034290506,3.88413224904271));
#59038=CARTESIAN_POINT('Ctrl Pts',(40.2993254358659,-39.3696159240468,3.85828160815533));
#59039=CARTESIAN_POINT('Ctrl Pts',(40.0530121946873,-39.7617625287194,3.83243096726796));
#59040=CARTESIAN_POINT('Ctrl Pts',(39.6990217970716,-39.9666307803348,3.80658032638058));
#59041=CARTESIAN_POINT('Origin',(39.0658530619283,-38.8697713466883,4.5));
#59042=CARTESIAN_POINT('',(39.6981666138854,-39.9633157673858,3.30658032638058));
#59043=CARTESIAN_POINT('',(39.6968376638891,-39.9635050155947,3.44341967361942));
#59044=CARTESIAN_POINT('',(39.6981030619283,-39.9648604697737,4.5));
#59045=CARTESIAN_POINT('Ctrl Pts',(39.6968376638891,-39.9635050155947,3.44341967361942));
#59046=CARTESIAN_POINT('Ctrl Pts',(39.9008619683972,-39.8448845676908,3.45822100506063));
#59047=CARTESIAN_POINT('Ctrl Pts',(40.0737604294822,-39.6716358129756,3.47302233650185));
#59048=CARTESIAN_POINT('Ctrl Pts',(40.1838048209619,-39.4649259634328,3.48782366794306));
#59049=CARTESIAN_POINT('Ctrl Pts',(40.378361442473,-39.0994664482373,3.51399217140199));
#59050=CARTESIAN_POINT('Ctrl Pts',(40.3764510665601,-38.6294154424262,3.54016067486091));
#59051=CARTESIAN_POINT('Ctrl Pts',(40.1789303273027,-38.265549404193,3.56632917831984));
#59052=CARTESIAN_POINT('Ctrl Pts',(39.9814095880453,-37.9016833659598,3.59249768177876));
#59053=CARTESIAN_POINT('Ctrl Pts',(39.5882784854434,-37.6440022953046,3.61866618523769));
#59054=CARTESIAN_POINT('Ctrl Pts',(39.1758216795725,-37.6080534474275,3.64483468869662));
#59055=CARTESIAN_POINT('Ctrl Pts',(38.7633648737015,-37.5721045995503,3.67100319215554));
#59056=CARTESIAN_POINT('Ctrl Pts',(38.3315823645617,-37.7578879744512,3.69717169561447));
#59057=CARTESIAN_POINT('Ctrl Pts',(38.0740905614766,-38.0820960983986,3.7233401990734));
#59058=CARTESIAN_POINT('Ctrl Pts',(37.8165987583915,-38.406304222346,3.74950870253232));
#59059=CARTESIAN_POINT('Ctrl Pts',(37.7333976613611,-38.8689370953399,3.77567720599125));
#59060=CARTESIAN_POINT('Ctrl Pts',(37.8617956314422,-39.2625446379184,3.80184570945018));
#59061=CARTESIAN_POINT('Ctrl Pts',(37.9901936015233,-39.6561521804969,3.82801421290911));
#59062=CARTESIAN_POINT('Ctrl Pts',(38.3301906387158,-39.9807343926601,3.85418271636803));
#59063=CARTESIAN_POINT('Ctrl Pts',(38.729328029973,-40.0907447522208,3.88035121982696));
#59064=CARTESIAN_POINT('Ctrl Pts',(39.0499804019726,-40.1791230487932,3.90137403775778));
#59065=CARTESIAN_POINT('Ctrl Pts',(39.4088015299329,-40.129018226562,3.9223968556886));
#59066=CARTESIAN_POINT('Ctrl Pts',(39.6992442211058,-39.9647402889406,3.94341967361942));
#59067=CARTESIAN_POINT('Ctrl Pts',(39.6990217970716,-39.9666307803348,3.80658032638058));
#59068=CARTESIAN_POINT('Ctrl Pts',(39.6946690888126,-39.9691498648546,3.80626246380903));
#59069=CARTESIAN_POINT('Ctrl Pts',(39.6903001003537,-39.9716406339069,3.80594460123748));
#59070=CARTESIAN_POINT('Ctrl Pts',(39.6859150342415,-39.9741027686317,3.80562673866593));
#59071=CARTESIAN_POINT('Ctrl Pts',(39.3249080205419,-40.1768016291736,3.779458235207));
#59072=CARTESIAN_POINT('Ctrl Pts',(38.8549323382456,-40.1854271070305,3.75328973174807));
#59073=CARTESIAN_POINT('Ctrl Pts',(38.486730670363,-39.9961114351584,3.72712122828915));
#59074=CARTESIAN_POINT('Ctrl Pts',(38.1185290024803,-39.8067957632863,3.70095272483022));
#59075=CARTESIAN_POINT('Ctrl Pts',(37.8521013490113,-39.4195389416852,3.6747842213713));
#59076=CARTESIAN_POINT('Ctrl Pts',(37.8069170356359,-39.007991532901,3.64861571791237));
#59077=CARTESIAN_POINT('Ctrl Pts',(37.7617327222606,-38.5964441241169,3.62244721445344));
#59078=CARTESIAN_POINT('Ctrl Pts',(37.9377917489788,-38.1606061281498,3.59627871099451));
#59079=CARTESIAN_POINT('Ctrl Pts',(38.2561471576721,-37.8959124821361,3.57011020753559));
#59080=CARTESIAN_POINT('Ctrl Pts',(38.5745025663654,-37.6312188361225,3.54394170407666));
#59081=CARTESIAN_POINT('Ctrl Pts',(39.0351543570337,-37.5376695400622,3.51777320061774));
#59082=CARTESIAN_POINT('Ctrl Pts',(39.4315407865323,-37.6572132122937,3.49160469715881));
#59083=CARTESIAN_POINT('Ctrl Pts',(39.8279272160309,-37.7767568845252,3.46543619369988));
#59084=CARTESIAN_POINT('Ctrl Pts',(40.1600482843597,-38.1093935250484,3.43926769024095));
#59085=CARTESIAN_POINT('Ctrl Pts',(40.2789769657405,-38.5059649062659,3.41309918678203));
#59086=CARTESIAN_POINT('Ctrl Pts',(40.3979056471214,-38.9025362874834,3.3869306833231));
#59087=CARTESIAN_POINT('Ctrl Pts',(40.3036419415544,-39.3630424093952,3.36076217986418));
#59088=CARTESIAN_POINT('Ctrl Pts',(40.0384547967127,-39.6809868610392,3.33459367640525));
#59089=CARTESIAN_POINT('Ctrl Pts',(39.943827295091,-39.7944399061765,3.32525589306369));
#59090=CARTESIAN_POINT('Ctrl Pts',(39.8274361583624,-39.8897406125527,3.31591810972214));
#59091=CARTESIAN_POINT('Ctrl Pts',(39.6981666138854,-39.9633157673858,3.30658032638058));
#59092=CARTESIAN_POINT('Origin',(39.0658530619283,-38.8697713466883,4.5));
#59093=CARTESIAN_POINT('',(39.696945388151,-39.9649932150637,2.80658032638058));
#59094=CARTESIAN_POINT('',(39.6985897981371,-39.9666323328489,2.94341967361942));
#59095=CARTESIAN_POINT('',(39.6981030619283,-39.9648604697737,4.5));
#59096=CARTESIAN_POINT('Ctrl Pts',(39.6985897981371,-39.9666323328489,2.94341967361942));
#59097=CARTESIAN_POINT('Ctrl Pts',(40.0329227359303,-39.771464492525,2.96787665097374));
#59098=CARTESIAN_POINT('Ctrl Pts',(40.2741270402692,-39.4118258938478,2.99233362832806));
#59099=CARTESIAN_POINT('Ctrl Pts',(40.3224423052901,-39.0279123314598,3.01679060568238));
#59100=CARTESIAN_POINT('Ctrl Pts',(40.3741387255592,-38.6171320768221,3.04295910914131));
#59101=CARTESIAN_POINT('Ctrl Pts',(40.2050042874718,-38.1785603982041,3.06912761260023));
#59102=CARTESIAN_POINT('Ctrl Pts',(39.8908808035795,-37.908858034419,3.09529611605916));
#59103=CARTESIAN_POINT('Ctrl Pts',(39.5767573196872,-37.6391556706339,3.12146461951809));
#59104=CARTESIAN_POINT('Ctrl Pts',(39.1176447899899,-37.5383226216818,3.14763312297702));
#59105=CARTESIAN_POINT('Ctrl Pts',(38.7194147698321,-37.6515736327838,3.17380162643594));
#59106=CARTESIAN_POINT('Ctrl Pts',(38.3211847496743,-37.7648246438858,3.19997012989487));
#59107=CARTESIAN_POINT('Ctrl Pts',(37.9838372390559,-38.092159715042,3.22613863335379));
#59108=CARTESIAN_POINT('Ctrl Pts',(37.8586428520748,-38.4867979056613,3.25230713681272));
#59109=CARTESIAN_POINT('Ctrl Pts',(37.7334484650937,-38.8814360962806,3.27847564027165));
#59110=CARTESIAN_POINT('Ctrl Pts',(37.8204072017498,-39.343377406363,3.30464414373057));
#59111=CARTESIAN_POINT('Ctrl Pts',(38.080525740607,-39.6654818632946,3.3308126471895));
#59112=CARTESIAN_POINT('Ctrl Pts',(38.3406442794641,-39.9875863202263,3.35698115064843));
#59113=CARTESIAN_POINT('Ctrl Pts',(38.7739226205222,-40.1698539240072,3.38314965410735));
#59114=CARTESIAN_POINT('Ctrl Pts',(39.1860736005189,-40.1305537136077,3.40931815756628));
#59115=CARTESIAN_POINT('Ctrl Pts',(39.3651052785911,-40.1134823418097,3.42068532958399));
#59116=CARTESIAN_POINT('Ctrl Pts',(39.5401504513672,-40.0546035118007,3.43205250160171));
#59117=CARTESIAN_POINT('Ctrl Pts',(39.6968376638891,-39.9635050155947,3.44341967361942));
#59118=CARTESIAN_POINT('Ctrl Pts',(39.6981666138854,-39.9633157673858,3.30658032638058));
#59119=CARTESIAN_POINT('Ctrl Pts',(39.4651670418018,-40.0959299856956,3.28974960626321));
#59120=CARTESIAN_POINT('Ctrl Pts',(39.1903285963567,-40.157963071813,3.27291888614584));
#59121=CARTESIAN_POINT('Ctrl Pts',(38.9256802513517,-40.128491465009,3.25608816602847));
#59122=CARTESIAN_POINT('Ctrl Pts',(38.5142034349489,-40.0826688359585,3.22991966256954));
#59123=CARTESIAN_POINT('Ctrl Pts',(38.1273603862596,-39.8156407964813,3.20375115911062));
#59124=CARTESIAN_POINT('Ctrl Pts',(37.9386160518288,-39.4471459263554,3.17758265565169));
#59125=CARTESIAN_POINT('Ctrl Pts',(37.7498717173979,-39.0786510562295,3.15141415219276));
#59126=CARTESIAN_POINT('Ctrl Pts',(37.7592260972255,-38.6086893554548,3.12524564873384));
#59127=CARTESIAN_POINT('Ctrl Pts',(37.9624847270864,-38.2479971709405,3.09907714527491));
#59128=CARTESIAN_POINT('Ctrl Pts',(38.1657433569474,-37.8873049864262,3.07290864181599));
#59129=CARTESIAN_POINT('Ctrl Pts',(38.5629062368417,-37.6358823181722,3.04674013835706));
#59130=CARTESIAN_POINT('Ctrl Pts',(38.9758805061506,-37.6064702124723,3.02057163489813));
#59131=CARTESIAN_POINT('Ctrl Pts',(39.3888547754595,-37.5770581067724,2.99440313143921));
#59132=CARTESIAN_POINT('Ctrl Pts',(39.8176404341829,-37.7696565636265,2.96823462798028));
#59133=CARTESIAN_POINT('Ctrl Pts',(40.069965509642,-38.0979018769219,2.94206612452135));
#59134=CARTESIAN_POINT('Ctrl Pts',(40.3222905851012,-38.4261471902174,2.91589762106243));
#59135=CARTESIAN_POINT('Ctrl Pts',(40.3981550772959,-38.8900393599541,2.8897291176035));
#59136=CARTESIAN_POINT('Ctrl Pts',(40.263539208776,-39.2815641648305,2.86356061414457));
#59137=CARTESIAN_POINT('Ctrl Pts',(40.1658333166794,-39.5657377972484,2.84456718488991));
#59138=CARTESIAN_POINT('Ctrl Pts',(39.9572455465606,-39.811788018551,2.82557375563525));
#59139=CARTESIAN_POINT('Ctrl Pts',(39.696945388151,-39.9649932150637,2.80658032638058));
#59140=CARTESIAN_POINT('Origin',(39.0658530619283,-38.8697713466883,4.5));
#59141=CARTESIAN_POINT('',(39.6994125047665,-39.9658989902663,2.30658032638058));
#59142=CARTESIAN_POINT('',(39.6985816414592,-39.9636701304733,2.44341967361942));
#59143=CARTESIAN_POINT('',(39.6981030619283,-39.9648604697737,4.5));
#59144=CARTESIAN_POINT('',(39.301448933936,-37.6274127691862,2.));
#59145=CARTESIAN_POINT('Ctrl Pts',(39.6994125047665,-39.9658989902663,2.30658032638058));
#59146=CARTESIAN_POINT('Ctrl Pts',(39.3734254452084,-40.1513842194032,2.2828923946305));
#59147=CARTESIAN_POINT('Ctrl Pts',(38.9582283391778,-40.1860737601753,2.25920446288042));
#59148=CARTESIAN_POINT('Ctrl Pts',(38.6086499461795,-40.0507923518177,2.23551653113034));
#59149=CARTESIAN_POINT('Ctrl Pts',(38.2224641245192,-39.901344437163,2.20934802767141));
#59150=CARTESIAN_POINT('Ctrl Pts',(37.9163596177671,-39.5444633609379,2.18317952421248));
#59151=CARTESIAN_POINT('Ctrl Pts',(37.8282894528998,-39.1398698141336,2.15701102075356));
#59152=CARTESIAN_POINT('Ctrl Pts',(37.7402192880324,-38.7352762673292,2.13084251729463));
#59153=CARTESIAN_POINT('Ctrl Pts',(37.8701834650499,-38.2829702499457,2.10467401383571));
#59154=CARTESIAN_POINT('Ctrl Pts',(38.1583556110386,-37.9866358554263,2.07850551037678));
#59155=CARTESIAN_POINT('Ctrl Pts',(38.4465277570273,-37.6903014609069,2.05233700691785));
#59156=CARTESIAN_POINT('Ctrl Pts',(38.8929078719872,-37.5499386892516,2.02616850345893));
#59157=CARTESIAN_POINT('Ctrl Pts',(39.301448933936,-37.6274127691862,2.));
#59158=CARTESIAN_POINT('',(40.2614317556683,-39.2879039300607,2.));
#59159=CARTESIAN_POINT('Origin',(39.0658530619283,-38.8697713466883,2.));
#59160=CARTESIAN_POINT('Ctrl Pts',(40.2614422049139,-39.287909445603,2.));
#59161=CARTESIAN_POINT('Ctrl Pts',(40.3902478674695,-38.9153329576355,2.02490816038701));
#59162=CARTESIAN_POINT('Ctrl Pts',(40.3325476766157,-38.4763154063562,2.04981632077402));
#59163=CARTESIAN_POINT('Ctrl Pts',(40.1090165446371,-38.1516794088469,2.07472448116103));
#59164=CARTESIAN_POINT('Ctrl Pts',(39.8741748257196,-37.8106169581592,2.10089298461995));
#59165=CARTESIAN_POINT('Ctrl Pts',(39.4562956252315,-37.5958042374567,2.12706148807888));
#59166=CARTESIAN_POINT('Ctrl Pts',(39.042397118114,-37.6034976893836,2.15322999153781));
#59167=CARTESIAN_POINT('Ctrl Pts',(38.6284986109964,-37.6111911413106,2.17939849499673));
#59168=CARTESIAN_POINT('Ctrl Pts',(38.2185807972492,-37.841390765867,2.20556699845566));
#59169=CARTESIAN_POINT('Ctrl Pts',(37.996635575997,-38.1909062543644,2.23173550191459));
#59170=CARTESIAN_POINT('Ctrl Pts',(37.7746903547448,-38.5404217428618,2.25790400537351));
#59171=CARTESIAN_POINT('Ctrl Pts',(37.7407177259875,-39.0092530953003,2.28407250883244));
#59172=CARTESIAN_POINT('Ctrl Pts',(37.909862273516,-39.3871539257345,2.31024101229137));
#59173=CARTESIAN_POINT('Ctrl Pts',(38.0790068210445,-39.7650547561687,2.33640951575029));
#59174=CARTESIAN_POINT('Ctrl Pts',(38.4512685448588,-40.0520250645987,2.36257801920922));
#59175=CARTESIAN_POINT('Ctrl Pts',(38.8597650567826,-40.1193923002797,2.38874652266815));
#59176=CARTESIAN_POINT('Ctrl Pts',(39.1442519845445,-40.1663084852441,2.40697090631857));
#59177=CARTESIAN_POINT('Ctrl Pts',(39.4463130348952,-40.1067156626302,2.42519528996899));
#59178=CARTESIAN_POINT('Ctrl Pts',(39.6985816414592,-39.9636701304733,2.44341967361942));
#59179=CARTESIAN_POINT('Origin',(39.0658530619283,-38.8697713466883,0.895788276411275));
#59180=CARTESIAN_POINT('',(39.8389883040074,-40.2073580112696,5.60421172358873));
#59181=CARTESIAN_POINT('',(39.8361023073888,-40.2039982703455,5.64578827641128));
#59182=CARTESIAN_POINT('',(39.8373530619283,-40.2060485447276,0.895788276411275));
#59183=CARTESIAN_POINT('',(37.5756558680257,-39.2699729499894,6.));
#59184=CARTESIAN_POINT('Ctrl Pts',(39.8361023073888,-40.2039982703455,5.64578827641128));
#59185=CARTESIAN_POINT('Ctrl Pts',(40.0618255698415,-40.0734865888946,5.65918483710515));
#59186=CARTESIAN_POINT('Ctrl Pts',(40.6360432757833,-39.5276070596663,5.69874990125794));
#59187=CARTESIAN_POINT('Ctrl Pts',(40.706254476474,-38.0891194878961,5.76448346886966));
#59188=CARTESIAN_POINT('Ctrl Pts',(39.3195619844849,-37.0695313077001,5.84298897924644));
#59189=CARTESIAN_POINT('Ctrl Pts',(37.7040659529861,-37.6679522088103,5.92149448962322));
#59190=CARTESIAN_POINT('Ctrl Pts',(37.4440523270134,-38.7799318659295,5.97383149654107));
#59191=CARTESIAN_POINT('Ctrl Pts',(37.5756558680257,-39.2699729499894,6.));
#59192=CARTESIAN_POINT('',(37.9726388313436,-39.9622904787117,6.));
#59193=CARTESIAN_POINT('Origin',(39.0658530619283,-38.8697713466883,6.));
#59194=CARTESIAN_POINT('Ctrl Pts',(39.8389883040074,-40.2073580112696,5.60421172358873));
#59195=CARTESIAN_POINT('Ctrl Pts',(39.8784035047361,-40.1849196436101,5.60655897483644));
#59196=CARTESIAN_POINT('Ctrl Pts',(40.3442265162732,-39.8903323926485,5.63507472954307));
#59197=CARTESIAN_POINT('Ctrl Pts',(40.8821362004287,-38.8192621207562,5.68975898770864));
#59198=CARTESIAN_POINT('Ctrl Pts',(40.025658400892,-37.3267854127763,5.76826449808541));
#59199=CARTESIAN_POINT('Ctrl Pts',(38.3080469143,-37.2183586878016,5.8467700084622));
#59200=CARTESIAN_POINT('Ctrl Pts',(37.2874279838023,-38.5683990357347,5.92401517576705));
#59201=CARTESIAN_POINT('Ctrl Pts',(37.6338153475925,-39.6208332722494,5.97509183961299));
#59202=CARTESIAN_POINT('Ctrl Pts',(37.972630261787,-39.9623020734811,6.));
#59203=CARTESIAN_POINT('Origin',(39.0658530619283,-38.8697713466883,0.895788276411275));
#59204=CARTESIAN_POINT('',(39.836482301403,-40.2038876485621,5.10421172358873));
#59205=CARTESIAN_POINT('',(39.8373456329824,-40.2079335437151,5.14578827641127));
#59206=CARTESIAN_POINT('',(39.8373530619283,-40.2060485447276,0.895788276411275));
#59207=CARTESIAN_POINT('Ctrl Pts',(39.8373456329825,-40.2079335437151,5.14578827641127));
#59208=CARTESIAN_POINT('Ctrl Pts',(40.2216806378634,-39.9822885010756,5.16884048301825));
#59209=CARTESIAN_POINT('Ctrl Pts',(40.8329618074792,-39.1268210714738,5.21806119308415));
#59210=CARTESIAN_POINT('Ctrl Pts',(40.3208244444739,-37.5557551266231,5.29345040660899));
#59211=CARTESIAN_POINT('Ctrl Pts',(38.6620380533447,-37.098163044885,5.37195591698576));
#59212=CARTESIAN_POINT('Ctrl Pts',(37.3653845951192,-38.2294425600612,5.45046142736254));
#59213=CARTESIAN_POINT('Ctrl Pts',(37.5937879163964,-39.9348809965236,5.52896693773932));
#59214=CARTESIAN_POINT('Ctrl Pts',(38.8780553810739,-40.5572546562641,5.59407588742224));
#59215=CARTESIAN_POINT('Ctrl Pts',(39.6209034474226,-40.3284248126315,5.63301633364622));
#59216=CARTESIAN_POINT('Ctrl Pts',(39.8361023073888,-40.2039982703455,5.64578827641128));
#59217=CARTESIAN_POINT('Ctrl Pts',(39.836482301403,-40.2038876485621,5.10421172358873));
#59218=CARTESIAN_POINT('Ctrl Pts',(40.0389857717083,-40.0874933656255,5.11621462074955));
#59219=CARTESIAN_POINT('Ctrl Pts',(40.6023754577107,-39.5788852724495,5.15438602136929));
#59220=CARTESIAN_POINT('Ctrl Pts',(40.745177494668,-38.1758811994982,5.21872592544796));
#59221=CARTESIAN_POINT('Ctrl Pts',(39.4133645670745,-37.0862753673934,5.29723143582474));
#59222=CARTESIAN_POINT('Ctrl Pts',(37.7698897533292,-37.5961550422893,5.37573694620152));
#59223=CARTESIAN_POINT('Ctrl Pts',(37.2886763485592,-39.2482362054987,5.4542424565783));
#59224=CARTESIAN_POINT('Ctrl Pts',(38.3679904575112,-40.5216689106221,5.53040071570737));
#59225=CARTESIAN_POINT('Ctrl Pts',(39.4389802356634,-40.4350754385143,5.58039047137751));
#59226=CARTESIAN_POINT('Ctrl Pts',(39.8389883040074,-40.2073580112696,5.60421172358873));
#59227=CARTESIAN_POINT('Origin',(39.0658530619283,-38.8697713466883,0.895788276411275));
#59228=CARTESIAN_POINT('',(39.8367681787868,-40.2074507120888,4.60421172358873));
#59229=CARTESIAN_POINT('',(39.838395191597,-40.2051955164573,4.64578827641127));
#59230=CARTESIAN_POINT('',(39.8373530619283,-40.2060485447276,0.895788276411275));
#59231=CARTESIAN_POINT('Ctrl Pts',(39.838395191597,-40.2051955164573,4.64578827641127));
#59232=CARTESIAN_POINT('Ctrl Pts',(39.9487742895753,-40.1427442714186,4.65232762547243));
#59233=CARTESIAN_POINT('Ctrl Pts',(40.461107190991,-39.7640019994127,4.68503547799252));
#59234=CARTESIAN_POINT('Ctrl Pts',(40.85159479603,-38.533999133735,4.74391183397153));
#59235=CARTESIAN_POINT('Ctrl Pts',(39.7707737852476,-37.1950466549739,4.82241734434831));
#59236=CARTESIAN_POINT('Ctrl Pts',(38.05776324374,-37.3580267168588,4.90092285472509));
#59237=CARTESIAN_POINT('Ctrl Pts',(37.248831349992,-38.8767760630728,4.97942836510187));
#59238=CARTESIAN_POINT('Ctrl Pts',(38.0694482634704,-40.3892418792306,5.05793387547864));
#59239=CARTESIAN_POINT('Ctrl Pts',(39.280304717179,-40.4950348443414,5.11338717924845));
#59240=CARTESIAN_POINT('Ctrl Pts',(39.7853895670741,-40.2384372151433,5.14267197955933));
#59241=CARTESIAN_POINT('Ctrl Pts',(39.8373456329825,-40.2079335437151,5.14578827641127));
#59242=CARTESIAN_POINT('Ctrl Pts',(39.8367681787868,-40.2074507120888,4.60421172358873));
#59243=CARTESIAN_POINT('Ctrl Pts',(40.1980237481411,-39.9947173316426,4.62587026666265));
#59244=CARTESIAN_POINT('Ctrl Pts',(40.8090940791592,-39.1897699662685,4.6736973131955));
#59245=CARTESIAN_POINT('Ctrl Pts',(40.3881021894618,-37.6234670214255,4.74769286318729));
#59246=CARTESIAN_POINT('Ctrl Pts',(38.7556268199881,-37.0794146789619,4.82619837356406));
#59247=CARTESIAN_POINT('Ctrl Pts',(37.4013696406987,-38.1409968175026,4.90470388394084));
#59248=CARTESIAN_POINT('Ctrl Pts',(37.5398609233301,-39.8561611622599,4.98320939431763));
#59249=CARTESIAN_POINT('Ctrl Pts',(38.8164833870163,-40.5597236082337,5.04971200753358));
#59250=CARTESIAN_POINT('Ctrl Pts',(39.5974912981551,-40.3412541164524,5.09004611729062));
#59251=CARTESIAN_POINT('Ctrl Pts',(39.836482301403,-40.2038876485621,5.10421172358873));
#59252=CARTESIAN_POINT('Origin',(39.0658530619283,-38.8697713466883,0.895788276411275));
#59253=CARTESIAN_POINT('',(39.8387455558871,-40.2059018946483,4.10421172358873));
#59254=CARTESIAN_POINT('',(39.835683949911,-40.2049009685562,4.14578827641127));
#59255=CARTESIAN_POINT('',(39.8373530619283,-40.2060485447276,0.895788276411275));
#59256=CARTESIAN_POINT('Ctrl Pts',(39.8356839499109,-40.2049009685562,4.14578827641127));
#59257=CARTESIAN_POINT('Ctrl Pts',(40.107566600927,-40.0460142702611,4.16198327138554));
#59258=CARTESIAN_POINT('Ctrl Pts',(40.7000264343407,-39.4199669716347,4.20434676981874));
#59259=CARTESIAN_POINT('Ctrl Pts',(40.6150446849375,-37.9202337024769,4.27287877171085));
#59260=CARTESIAN_POINT('Ctrl Pts',(39.1283436057741,-37.0538111746305,4.35138428208763));
#59261=CARTESIAN_POINT('Ctrl Pts',(37.5855995232344,-37.8159848954578,4.42988979246441));
#59262=CARTESIAN_POINT('Ctrl Pts',(37.3703820012353,-39.5232193693979,4.50839530284119));
#59263=CARTESIAN_POINT('Ctrl Pts',(38.5669726422017,-40.5510318627907,4.58036146415681));
#59264=CARTESIAN_POINT('Ctrl Pts',(39.5070704165714,-40.3926553262541,4.6261591220135));
#59265=CARTESIAN_POINT('Ctrl Pts',(39.838395191597,-40.2051955164573,4.64578827641127));
#59266=CARTESIAN_POINT('Ctrl Pts',(39.8387455558871,-40.2059018946483,4.10421172358873));
#59267=CARTESIAN_POINT('Ctrl Pts',(39.9254936329904,-40.1568361214949,4.10935740911683));
#59268=CARTESIAN_POINT('Ctrl Pts',(40.4229804016609,-39.8074510911276,4.14067159810387));
#59269=CARTESIAN_POINT('Ctrl Pts',(40.8667641756191,-38.6282419782981,4.19815429054982));
#59270=CARTESIAN_POINT('Ctrl Pts',(39.8577505620191,-37.2343767082119,4.27665980092661));
#59271=CARTESIAN_POINT('Ctrl Pts',(38.1385444446534,-37.3071722287697,4.35516531130338));
#59272=CARTESIAN_POINT('Ctrl Pts',(37.2509707395799,-38.781343787805,4.43367082168017));
#59273=CARTESIAN_POINT('Ctrl Pts',(37.9910266499109,-40.3348192821528,4.51217633205694));
#59274=CARTESIAN_POINT('Ctrl Pts',(39.2249072234587,-40.508306713049,4.5690232993598));
#59275=CARTESIAN_POINT('Ctrl Pts',(39.7615438988762,-40.2517482031576,4.59970176320373));
#59276=CARTESIAN_POINT('Ctrl Pts',(39.8367681787868,-40.2074507120888,4.60421172358873));
#59277=CARTESIAN_POINT('Origin',(39.0658530619283,-38.8697713466883,0.895788276411275));
#59278=CARTESIAN_POINT('',(39.8358089661004,-40.2043945583313,3.60421172358873));
#59279=CARTESIAN_POINT('',(39.8384741440367,-40.2082087576147,3.64578827641127));
#59280=CARTESIAN_POINT('',(39.8373530619283,-40.2060485447276,0.895788276411275));
#59281=CARTESIAN_POINT('Ctrl Pts',(39.8384741440367,-40.2082087576148,3.64578827641127));
#59282=CARTESIAN_POINT('Ctrl Pts',(40.2704292120644,-39.9582192659243,3.67163891729865));
#59283=CARTESIAN_POINT('Ctrl Pts',(40.8752500438969,-38.9953053985924,3.72365806164495));
#59284=CARTESIAN_POINT('Ctrl Pts',(40.1754790439541,-37.4309014426854,3.80184570945018));
#59285=CARTESIAN_POINT('Ctrl Pts',(38.4777242474675,-37.1505503260543,3.88035121982696));
#59286=CARTESIAN_POINT('Ctrl Pts',(37.3074173539442,-38.4120374927131,3.95885673020373));
#59287=CARTESIAN_POINT('Ctrl Pts',(37.7141174076169,-40.0840312618198,4.03736224058051));
#59288=CARTESIAN_POINT('Ctrl Pts',(38.9991071509757,-40.5467766825013,4.09967275598303));
#59289=CARTESIAN_POINT('Ctrl Pts',(39.6682480272046,-40.3027495838885,4.13581476792661));
#59290=CARTESIAN_POINT('Ctrl Pts',(39.8356839499109,-40.2049009685562,4.14578827641127));
#59291=CARTESIAN_POINT('Ctrl Pts',(39.8358089661004,-40.2043945583313,3.60421172358873));
#59292=CARTESIAN_POINT('Ctrl Pts',(40.0847686354211,-40.0596485313517,3.61901305502994));
#59293=CARTESIAN_POINT('Ctrl Pts',(40.6687535790882,-39.4744804296356,3.65998288993008));
#59294=CARTESIAN_POINT('Ctrl Pts',(40.662772801836,-38.0029007557487,3.72712122828915));
#59295=CARTESIAN_POINT('Ctrl Pts',(39.2236238307452,-37.0595985208236,3.80562673866593));
#59296=CARTESIAN_POINT('Ctrl Pts',(37.642982284831,-37.7397023107928,3.88413224904271));
#59297=CARTESIAN_POINT('Ctrl Pts',(37.3384050779085,-39.4332788778856,3.96263775941949));
#59298=CARTESIAN_POINT('Ctrl Pts',(38.501463750429,-40.5436066616789,4.03599758426816));
#59299=CARTESIAN_POINT('Ctrl Pts',(39.4843342688331,-40.4063612522993,4.08318890565791));
#59300=CARTESIAN_POINT('Ctrl Pts',(39.8387455558871,-40.2059018946483,4.10421172358873));
#59301=CARTESIAN_POINT('Origin',(39.0658530619283,-38.8697713466883,0.895788276411275));
#59302=CARTESIAN_POINT('',(39.8379469994295,-40.2082106520626,3.10421172358873));
#59303=CARTESIAN_POINT('',(39.8374306108961,-40.204163629121,3.14578827641127));
#59304=CARTESIAN_POINT('',(39.8373530619283,-40.2060485447276,0.895788276411275));
#59305=CARTESIAN_POINT('Ctrl Pts',(39.8374306108961,-40.204163629121,3.14578827641127));
#59306=CARTESIAN_POINT('Ctrl Pts',(39.9951711463868,-40.1143839028202,3.15512605975283));
#59307=CARTESIAN_POINT('Ctrl Pts',(40.5352143013727,-39.6721982210719,3.19063234655331));
#59308=CARTESIAN_POINT('Ctrl Pts',(40.8063086069208,-38.3478222423284,3.25230713681272));
#59309=CARTESIAN_POINT('Ctrl Pts',(39.5905012322319,-37.1301274942209,3.3308126471895));
#59310=CARTESIAN_POINT('Ctrl Pts',(37.9041768834746,-37.472586720368,3.40931815756627));
#59311=CARTESIAN_POINT('Ctrl Pts',(37.259671359806,-39.0680743307528,3.48782366794306));
#59312=CARTESIAN_POINT('Ctrl Pts',(38.2349925206666,-40.4857191130318,3.56632917831984));
#59313=CARTESIAN_POINT('Ctrl Pts',(39.3889296125876,-40.4645408708171,3.61898404780924));
#59314=CARTESIAN_POINT('Ctrl Pts',(39.8331627728674,-40.2112826582981,3.64547041383972));
#59315=CARTESIAN_POINT('Ctrl Pts',(39.8384741440367,-40.2082087576148,3.64578827641127));
#59316=CARTESIAN_POINT('Ctrl Pts',(39.8379469994295,-40.2082106520626,3.10421172358873));
#59317=CARTESIAN_POINT('Ctrl Pts',(40.2459151473258,-39.9700580402637,3.12866870094305));
#59318=CARTESIAN_POINT('Ctrl Pts',(40.8551693385609,-39.0616525117033,3.1792941817563));
#59319=CARTESIAN_POINT('Ctrl Pts',(40.249511348243,-37.4911595684212,3.25608816602847));
#59320=CARTESIAN_POINT('Ctrl Pts',(38.5688218267177,-37.1220364497186,3.33459367640525));
#59321=CARTESIAN_POINT('Ctrl Pts',(37.333881829365,-38.3203235548052,3.41309918678203));
#59322=CARTESIAN_POINT('Ctrl Pts',(37.6522147609438,-40.0113684930191,3.49160469715881));
#59323=CARTESIAN_POINT('Ctrl Pts',(38.9392875485226,-40.5528026028124,3.55530887609437));
#59324=CARTESIAN_POINT('Ctrl Pts',(39.6446121539838,-40.3155570570627,3.59284455157101));
#59325=CARTESIAN_POINT('Ctrl Pts',(39.8358089661004,-40.2043945583313,3.60421172358873));
#59326=CARTESIAN_POINT('Origin',(39.0658530619283,-38.8697713466883,0.895788276411275));
#59327=CARTESIAN_POINT('',(39.8379370462827,-40.2045960389621,2.60421172358873));
#59328=CARTESIAN_POINT('',(39.8359404161091,-40.2062105265248,2.64578827641127));
#59329=CARTESIAN_POINT('',(39.8373530619283,-40.2060485447276,0.895788276411275));
#59330=CARTESIAN_POINT('Ctrl Pts',(39.8359404161091,-40.2062105265248,2.64578827641127));
#59331=CARTESIAN_POINT('Ctrl Pts',(40.1535704235635,-40.0192626275773,2.66478170566594));
#59332=CARTESIAN_POINT('Ctrl Pts',(40.7587789941875,-39.3053583432972,2.70994363837953));
#59333=CARTESIAN_POINT('Ctrl Pts',(40.5064415845057,-37.7623789454716,2.78127407455204));
#59334=CARTESIAN_POINT('Ctrl Pts',(38.936770715205,-37.057326943275,2.85977958492882));
#59335=CARTESIAN_POINT('Ctrl Pts',(37.4828624739785,-37.9777188225534,2.9382850953056));
#59336=CARTESIAN_POINT('Ctrl Pts',(37.4486185639574,-39.6981242894462,3.01679060568238));
#59337=CARTESIAN_POINT('Ctrl Pts',(38.6963080267235,-40.5593729851321,3.0859583327176));
#59338=CARTESIAN_POINT('Ctrl Pts',(39.5531140116671,-40.3659854866553,3.1289575562939));
#59339=CARTESIAN_POINT('Ctrl Pts',(39.8374306108961,-40.204163629121,3.14578827641127));
#59340=CARTESIAN_POINT('Ctrl Pts',(39.8379370462827,-40.2045960389621,2.60421172358873));
#59341=CARTESIAN_POINT('Ctrl Pts',(39.9721218195358,-40.1285083617881,2.61215584339723));
#59342=CARTESIAN_POINT('Ctrl Pts',(40.4987455670004,-39.7186935414777,2.64626846666466));
#59343=CARTESIAN_POINT('Ctrl Pts',(40.8313104277201,-38.439942299895,2.70654959339101));
#59344=CARTESIAN_POINT('Ctrl Pts',(39.6811395860237,-37.1600807661057,2.78505510376779));
#59345=CARTESIAN_POINT('Ctrl Pts',(37.9791520940816,-37.4135079224237,2.86356061414458));
#59346=CARTESIAN_POINT('Ctrl Pts',(37.2517503435483,-38.9729479619196,2.94206612452135));
#59347=CARTESIAN_POINT('Ctrl Pts',(38.1512758267994,-40.4398561533634,3.02057163489813));
#59348=CARTESIAN_POINT('Ctrl Pts',(39.3352629723092,-40.4803512300078,3.07462016792059));
#59349=CARTESIAN_POINT('Ctrl Pts',(39.8093969408979,-40.2248768330901,3.10250019748412));
#59350=CARTESIAN_POINT('Ctrl Pts',(39.8379469994295,-40.2082106520626,3.10421172358873));
#59351=CARTESIAN_POINT('Origin',(39.0658530619283,-38.8697713466883,0.895788276411275));
#59352=CARTESIAN_POINT('',(39.835191636477,-40.2053827942122,2.10421172358873));
#59353=CARTESIAN_POINT('',(39.8389509032089,-40.2073157943284,2.14578827641127));
#59354=CARTESIAN_POINT('',(39.8373530619283,-40.2060485447276,0.895788276411275));
#59355=CARTESIAN_POINT('',(37.9741697098829,-39.9602191716056,2.));
#59356=CARTESIAN_POINT('Ctrl Pts',(37.9741697098829,-39.9602191716056,2.));
#59357=CARTESIAN_POINT('Ctrl Pts',(38.3327559670707,-40.3192117233802,2.02616850345893));
#59358=CARTESIAN_POINT('Ctrl Pts',(39.0582121561479,-40.5387775404138,2.06090574465517));
#59359=CARTESIAN_POINT('Ctrl Pts',(39.6915909718076,-40.2896039589219,2.09564298585141));
#59360=CARTESIAN_POINT('Ctrl Pts',(39.835191636477,-40.2053827942122,2.10421172358873));
#59361=CARTESIAN_POINT('',(37.5730967199607,-39.2702632425652,2.));
#59362=CARTESIAN_POINT('Origin',(39.0658530619283,-38.8697713466883,2.));
#59363=CARTESIAN_POINT('Ctrl Pts',(37.5730824075077,-39.2702648660738,2.));
#59364=CARTESIAN_POINT('Ctrl Pts',(37.6993955576028,-39.7344217910383,2.02490816038701));
#59365=CARTESIAN_POINT('Ctrl Pts',(38.4017837618403,-40.520493253107,2.0735042525241));
#59366=CARTESIAN_POINT('Ctrl Pts',(39.4411667728031,-40.4336532467271,2.12210034466119));
#59367=CARTESIAN_POINT('Ctrl Pts',(39.8389509032089,-40.2073157943284,2.14578827641127));
#59368=CARTESIAN_POINT('Origin',(13.,-3.,18.));
#59369=CARTESIAN_POINT('',(9.53939201416946,-3.,18.));
#59370=CARTESIAN_POINT('',(9.53939201416946,-3.,2.));
#59371=CARTESIAN_POINT('',(9.53939201416946,-3.,0.));
#59372=CARTESIAN_POINT('',(13.,-3.,18.));
#59373=CARTESIAN_POINT('',(6.5,-3.,18.));
#59374=CARTESIAN_POINT('',(13.,-3.,2.));
#59375=CARTESIAN_POINT('',(13.,-3.,18.));
#59376=CARTESIAN_POINT('',(6.5,-3.,2.));
#59377=CARTESIAN_POINT('Origin',(13.,3.,18.));
#59378=CARTESIAN_POINT('',(13.,3.,18.));
#59379=CARTESIAN_POINT('',(13.,1.5,18.));
#59380=CARTESIAN_POINT('',(13.,3.,2.));
#59381=CARTESIAN_POINT('',(13.,3.,18.));
#59382=CARTESIAN_POINT('',(13.,1.5,2.));
#59383=CARTESIAN_POINT('Origin',(7.,3.,18.));
#59384=CARTESIAN_POINT('',(9.53939201416946,3.,2.));
#59385=CARTESIAN_POINT('',(9.53939201416946,3.,18.));
#59386=CARTESIAN_POINT('',(9.53939201416946,3.,0.));
#59387=CARTESIAN_POINT('',(3.5,3.,2.));
#59388=CARTESIAN_POINT('',(3.5,3.,18.));
#59389=CARTESIAN_POINT('Origin',(0.,0.,18.));
#59390=CARTESIAN_POINT('',(46.0449384185095,-16.7589870229578,18.));
#59391=CARTESIAN_POINT('',(34.5017338047181,-32.2758373034865,18.));
#59392=CARTESIAN_POINT('Ctrl Pts',(46.0449384185095,-16.7589870229578,18.));
#59393=CARTESIAN_POINT('Ctrl Pts',(45.8743956437238,-17.1218851168881,18.));
#59394=CARTESIAN_POINT('Ctrl Pts',(45.6995171721829,-17.4824839536868,18.));
#59395=CARTESIAN_POINT('Ctrl Pts',(45.5203598455,-17.8406806900323,18.));
#59396=CARTESIAN_POINT('Ctrl Pts',(45.1531768081802,-18.5748050936752,18.));
#59397=CARTESIAN_POINT('Ctrl Pts',(44.7680194870699,-19.2988348495882,18.));
#59398=CARTESIAN_POINT('Ctrl Pts',(44.3654220486085,-20.0118834338741,18.));
#59399=CARTESIAN_POINT('Ctrl Pts',(43.9631822808423,-20.7242985402524,18.));
#59400=CARTESIAN_POINT('Ctrl Pts',(43.5435334515142,-21.425751826585,18.));
#59401=CARTESIAN_POINT('Ctrl Pts',(43.1070531396035,-22.1153854338476,18.));
#59402=CARTESIAN_POINT('Ctrl Pts',(42.6709588293944,-22.8044091630961,18.));
#59403=CARTESIAN_POINT('Ctrl Pts',(42.2180628840101,-23.4816339600163,18.));
#59404=CARTESIAN_POINT('Ctrl Pts',(41.7489848299194,-24.1462327731379,18.));
#59405=CARTESIAN_POINT('Ctrl Pts',(41.2803227785336,-24.8102421856223,18.));
#59406=CARTESIAN_POINT('Ctrl Pts',(40.7955074062862,-25.4616478541608,18.));
#59407=CARTESIAN_POINT('Ctrl Pts',(40.295198597365,-26.0996556279412,18.));
#59408=CARTESIAN_POINT('Ctrl Pts',(39.7955319525129,-26.736844496156,18.));
#59409=CARTESIAN_POINT('Ctrl Pts',(39.2804117264143,-27.360669703197,18.));
#59410=CARTESIAN_POINT('Ctrl Pts',(38.7505356300951,-27.9703729038242,18.));
#59411=CARTESIAN_POINT('Ctrl Pts',(38.2210732096325,-28.5796001073353,18.));
#59412=CARTESIAN_POINT('Ctrl Pts',(37.6768780617941,-29.1747272108444,18.));
#59413=CARTESIAN_POINT('Ctrl Pts',(37.1186849480847,-29.7550324141308,18.));
#59414=CARTESIAN_POINT('Ctrl Pts',(36.5611161547233,-30.3346885654357,18.));
#59415=CARTESIAN_POINT('Ctrl Pts',(35.9895808113595,-30.899555826196,18.));
#59416=CARTESIAN_POINT('Ctrl Pts',(35.4048480816292,-31.4489514860585,18.));
#59417=CARTESIAN_POINT('Ctrl Pts',(35.107194183748,-31.7286173082753,18.));
#59418=CARTESIAN_POINT('Ctrl Pts',(34.8061210997365,-32.0042746598847,18.));
#59419=CARTESIAN_POINT('Ctrl Pts',(34.5017338047268,-32.2758373034788,18.));
#59420=CARTESIAN_POINT('',(44.1555553153094,-16.0713078122675,18.));
#59421=CARTESIAN_POINT('',(21.6129302780759,-7.86646329649042,18.));
#59422=CARTESIAN_POINT('',(43.5508185339833,-14.8096659320883,18.));
#59423=CARTESIAN_POINT('Origin',(44.4975754586351,-15.1316151914816,18.));
#59424=CARTESIAN_POINT('',(46.,0.,18.));
#59425=CARTESIAN_POINT('Origin',(1.83021655258307E-13,-3.27857114887026E-14,
18.));
#59426=CARTESIAN_POINT('',(46.0771487394572,7.40158428109252,18.));
#59427=CARTESIAN_POINT('Ctrl Pts',(46.0771487393634,7.40158428108604,18.));
#59428=CARTESIAN_POINT('Ctrl Pts',(46.2472869475148,4.94053945592452,18.));
#59429=CARTESIAN_POINT('Ctrl Pts',(46.2231469368338,2.46578847026075,18.));
#59430=CARTESIAN_POINT('Ctrl Pts',(46.,0.,18.));
#59431=CARTESIAN_POINT('',(46.4996348579608,6.56002729234549,18.));
#59432=CARTESIAN_POINT('',(43.358988599418,12.8159317895946,18.));
#59433=CARTESIAN_POINT('',(58.1177432099948,12.3926560582107,18.));
#59434=CARTESIAN_POINT('',(46.4996348579608,6.56002729234549,18.));
#59435=CARTESIAN_POINT('',(54.977096951452,18.6485605554598,18.));
#59436=CARTESIAN_POINT('',(58.1177432099948,12.3926560582107,18.));
#59437=CARTESIAN_POINT('',(45.2025619355918,13.741459297751,18.));
#59438=CARTESIAN_POINT('',(54.977096951452,18.6485605554598,18.));
#59439=CARTESIAN_POINT('',(37.5361777128299,31.4965928746404,18.));
#59440=CARTESIAN_POINT('Ctrl Pts',(37.5361777128299,31.4965928746404,18.));
#59441=CARTESIAN_POINT('Ctrl Pts',(37.7651853233442,31.1674494097669,18.));
#59442=CARTESIAN_POINT('Ctrl Pts',(37.9900338693208,30.8357007492528,18.));
#59443=CARTESIAN_POINT('Ctrl Pts',(38.2106627066136,30.5014475410796,18.));
#59444=CARTESIAN_POINT('Ctrl Pts',(38.6628417256667,29.8163952621406,18.));
#59445=CARTESIAN_POINT('Ctrl Pts',(39.0972913691121,29.1208241134464,18.));
#59446=CARTESIAN_POINT('Ctrl Pts',(39.5135109674438,28.4156399596004,18.));
#59447=CARTESIAN_POINT('Ctrl Pts',(39.9293606088442,27.7110826089289,18.));
#59448=CARTESIAN_POINT('Ctrl Pts',(40.327012508134,26.9969294809322,18.));
#59449=CARTESIAN_POINT('Ctrl Pts',(40.706012527242,26.2741097029318,18.));
#59450=CARTESIAN_POINT('Ctrl Pts',(41.0846776773738,25.5519285790389,18.));
#59451=CARTESIAN_POINT('Ctrl Pts',(41.444723808721,24.8210962666709,18.));
#59452=CARTESIAN_POINT('Ctrl Pts',(41.7857444361162,24.0825628192227,18.));
#59453=CARTESIAN_POINT('Ctrl Pts',(42.1264631259329,23.3446832647734,18.));
#59454=CARTESIAN_POINT('Ctrl Pts',(42.4481899106077,22.5991163638997,18.));
#59455=CARTESIAN_POINT('Ctrl Pts',(42.7505669752443,21.8468306747833,18.));
#59456=CARTESIAN_POINT('Ctrl Pts',(43.0525553238862,21.095512074491,18.));
#59457=CARTESIAN_POINT('Ctrl Pts',(43.3352436048344,20.3374921118706,18.));
#59458=CARTESIAN_POINT('Ctrl Pts',(43.5983239273765,19.573754195526,18.));
#59459=CARTESIAN_POINT('Ctrl Pts',(43.86119868316,18.8106130517806,18.));
#59460=CARTESIAN_POINT('Ctrl Pts',(44.104496050171,18.0417630511784,18.));
#59461=CARTESIAN_POINT('Ctrl Pts',(44.3279583123957,17.2682014144259,18.));
#59462=CARTESIAN_POINT('Ctrl Pts',(44.5511707711369,16.4955045249897,18.));
#59463=CARTESIAN_POINT('Ctrl Pts',(44.7545923968601,15.7181066959427,18.));
#59464=CARTESIAN_POINT('Ctrl Pts',(44.93801652698,14.9370153979336,18.));
#59465=CARTESIAN_POINT('Ctrl Pts',(45.0313867007029,14.539408877238,18.));
#59466=CARTESIAN_POINT('Ctrl Pts',(45.1195759021844,14.1408455013228,18.));
#59467=CARTESIAN_POINT('Ctrl Pts',(45.2025619355895,13.7414592977624,18.));
#59468=CARTESIAN_POINT('',(35.9959384951176,30.2041787151333,18.));
#59469=CARTESIAN_POINT('',(17.6190221917365,14.7841150227904,18.));
#59470=CARTESIAN_POINT('',(34.6009561857411,30.3112822399915,18.));
#59471=CARTESIAN_POINT('Origin',(35.3531508854311,30.9702231582522,18.));
#59472=CARTESIAN_POINT('',(23.,39.8371685740842,18.));
#59473=CARTESIAN_POINT('Origin',(1.19904086659517E-13,1.4210854715202E-13,
18.));
#59474=CARTESIAN_POINT('',(16.6286143540509,43.6047734828703,18.));
#59475=CARTESIAN_POINT('Ctrl Pts',(16.6286143540096,43.6047734827858,18.));
#59476=CARTESIAN_POINT('Ctrl Pts',(18.8450107965664,42.5215950805994,18.));
#59477=CARTESIAN_POINT('Ctrl Pts',(20.9761380121528,41.2633137257534,18.));
#59478=CARTESIAN_POINT('Ctrl Pts',(23.,39.8371685740842,18.));
#59479=CARTESIAN_POINT('',(17.56866714429,43.5498786998672,18.));
#59480=CARTESIAN_POINT('',(10.5805717967515,43.9579515042931,18.));
#59481=CARTESIAN_POINT('',(18.3265166382238,56.5277700595814,18.));
#59482=CARTESIAN_POINT('',(17.56866714429,43.5498786998672,18.));
#59483=CARTESIAN_POINT('',(11.3384212906854,56.9358428640073,18.));
#59484=CARTESIAN_POINT('',(18.3265166382238,56.5277700595814,18.));
#59485=CARTESIAN_POINT('',(10.7008281308737,46.0172966012375,18.));
#59486=CARTESIAN_POINT('',(11.3384212906854,56.9358428640073,18.));
#59487=CARTESIAN_POINT('',(-8.50876070567958,48.2555798975982,18.));
#59488=CARTESIAN_POINT('Ctrl Pts',(-8.50876070567958,48.2555798975982,18.));
#59489=CARTESIAN_POINT('Ctrl Pts',(-8.10921023867559,48.2893345785684,18.));
#59490=CARTESIAN_POINT('Ctrl Pts',(-7.70948313828089,48.3181848047075,18.));
#59491=CARTESIAN_POINT('Ctrl Pts',(-7.30969689033073,48.3421283806345,18.));
#59492=CARTESIAN_POINT('Ctrl Pts',(-6.49033472635619,48.3912007543976,18.));
#59493=CARTESIAN_POINT('Ctrl Pts',(-5.67072764184703,48.4196596047247,18.));
#59494=CARTESIAN_POINT('Ctrl Pts',(-4.85191047323153,48.4275242714055,18.));
#59495=CARTESIAN_POINT('Ctrl Pts',(-4.03382065662236,48.4353819519344,18.));
#59496=CARTESIAN_POINT('Ctrl Pts',(-3.21651952501596,48.4226820151353,18.));
#59497=CARTESIAN_POINT('Ctrl Pts',(-2.40103879694537,48.3894957296891,18.));
#59498=CARTESIAN_POINT('Ctrl Pts',(-1.58627997520921,48.3563388224843,18.));
#59499=CARTESIAN_POINT('Ctrl Pts',(-0.773338510221561,48.3027318255699,
18.));
#59500=CARTESIAN_POINT('Ctrl Pts',(0.0367595886500608,48.2287977387298,
18.));
#59501=CARTESIAN_POINT('Ctrl Pts',(0.846140753505449,48.1549290833008,18.));
#59502=CARTESIAN_POINT('Ctrl Pts',(1.65268340805356,48.0607693134724,18.));
#59503=CARTESIAN_POINT('Ctrl Pts',(2.4553698511975,47.9464928310905,18.));
#59504=CARTESIAN_POINT('Ctrl Pts',(3.25702489039038,47.8323631871365,18.));
#59505=CARTESIAN_POINT('Ctrl Pts',(4.05483344847245,47.6981685198292,18.));
#59506=CARTESIAN_POINT('Ctrl Pts',(4.84778992376607,47.5441338920999,18.));
#59507=CARTESIAN_POINT('Ctrl Pts',(5.64012898520712,47.3902191992169,18.));
#59508=CARTESIAN_POINT('Ctrl Pts',(6.42762334377131,47.2164954589048,18.));
#59509=CARTESIAN_POINT('Ctrl Pts',(7.20928051527433,47.023238095029,18.));
#59510=CARTESIAN_POINT('Ctrl Pts',(7.99006081195724,46.8301975301827,18.));
#59511=CARTESIAN_POINT('Ctrl Pts',(8.76501683998239,46.6176671844283,18.));
#59512=CARTESIAN_POINT('Ctrl Pts',(9.53317277684725,46.3859718167405,18.));
#59513=CARTESIAN_POINT('Ctrl Pts',(9.924195445201,46.2680294347701,18.));
#59514=CARTESIAN_POINT('Ctrl Pts',(10.3134562863487,46.145121765699,18.));
#59515=CARTESIAN_POINT('Ctrl Pts',(10.7008281308626,46.0172966012412,18.));
#59516=CARTESIAN_POINT('',(-8.1596168201918,46.2754865274007,18.));
#59517=CARTESIAN_POINT('',(-3.99390808633937,22.6505783192808,18.));
#59518=CARTESIAN_POINT('',(-8.94986234824223,45.1209481720799,18.));
#59519=CARTESIAN_POINT('Origin',(-9.14442457320401,46.1018383497338,18.));
#59520=CARTESIAN_POINT('',(-23.,39.8371685740842,18.));
#59521=CARTESIAN_POINT('Origin',(-6.31175685987896E-14,1.74894258640722E-13,
18.));
#59522=CARTESIAN_POINT('',(-29.4485343854063,36.2031892017778,18.));
#59523=CARTESIAN_POINT('Ctrl Pts',(-29.4485343853538,36.2031892016998,18.));
#59524=CARTESIAN_POINT('Ctrl Pts',(-27.4022761513372,37.5810556244599,18.));
#59525=CARTESIAN_POINT('Ctrl Pts',(-25.2470089259271,38.7975252541457,18.));
#59526=CARTESIAN_POINT('Ctrl Pts',(-23.,39.8371685740842,18.));
#59527=CARTESIAN_POINT('',(-28.9309677136708,36.9898514075217,18.));
#59528=CARTESIAN_POINT('',(-32.7784168026664,31.1420197146986,18.));
#59529=CARTESIAN_POINT('',(-39.791226571771,44.1351140013707,18.));
#59530=CARTESIAN_POINT('',(-28.9309677136708,36.9898514075217,18.));
#59531=CARTESIAN_POINT('',(-43.6386756607666,38.2872823085476,18.));
#59532=CARTESIAN_POINT('',(-39.791226571771,44.1351140013707,18.));
#59533=CARTESIAN_POINT('',(-34.5017338047182,32.2758373034865,18.));
#59534=CARTESIAN_POINT('',(-43.6386756607666,38.2872823085476,18.));
#59535=CARTESIAN_POINT('',(-46.0449384185095,16.7589870229578,18.));
#59536=CARTESIAN_POINT('Ctrl Pts',(-46.0449384185095,16.7589870229578,18.));
#59537=CARTESIAN_POINT('Ctrl Pts',(-43.6587293356143,21.8366030579606,18.));
#59538=CARTESIAN_POINT('Ctrl Pts',(-40.4224569853479,26.4671498428742,18.));
#59539=CARTESIAN_POINT('Ctrl Pts',(-35.8215879134419,31.0643477170003,18.));
#59540=CARTESIAN_POINT('Ctrl Pts',(-35.1697987101644,31.6798154760653,18.));
#59541=CARTESIAN_POINT('Ctrl Pts',(-34.5017338047181,32.2758373034865,18.));
#59542=CARTESIAN_POINT('',(-44.1555553153094,16.0713078122674,18.));
#59543=CARTESIAN_POINT('',(-21.6129302780759,7.86646329649041,18.));
#59544=CARTESIAN_POINT('',(-43.5508185339833,14.8096659320883,18.));
#59545=CARTESIAN_POINT('Origin',(-44.4975754586351,15.1316151914815,18.));
#59546=CARTESIAN_POINT('',(-46.,1.33226762955019E-14,18.));
#59547=CARTESIAN_POINT('Origin',(-1.83021655258307E-13,3.27857114887025E-14,
18.));
#59548=CARTESIAN_POINT('',(-46.0771487394572,-7.40158428109254,18.));
#59549=CARTESIAN_POINT('Ctrl Pts',(-46.0771487393634,-7.40158428108605,
18.));
#59550=CARTESIAN_POINT('Ctrl Pts',(-46.2472869474355,-4.94053945706959,
18.));
#59551=CARTESIAN_POINT('Ctrl Pts',(-46.2231469370949,-2.46578847314652,
18.));
#59552=CARTESIAN_POINT('Ctrl Pts',(-46.,6.66133814775094E-15,18.));
#59553=CARTESIAN_POINT('',(-46.4996348579608,-6.56002729234549,18.));
#59554=CARTESIAN_POINT('',(-43.358988599418,-12.8159317895946,18.));
#59555=CARTESIAN_POINT('',(-58.1177432099948,-12.3926560582107,18.));
#59556=CARTESIAN_POINT('',(-46.4996348579608,-6.56002729234549,18.));
#59557=CARTESIAN_POINT('',(-54.977096951452,-18.6485605554598,18.));
#59558=CARTESIAN_POINT('',(-58.1177432099948,-12.3926560582107,18.));
#59559=CARTESIAN_POINT('',(-45.2025619355918,-13.741459297751,18.));
#59560=CARTESIAN_POINT('',(-54.977096951452,-18.6485605554598,18.));
#59561=CARTESIAN_POINT('',(-37.5361777128299,-31.4965928746404,18.));
#59562=CARTESIAN_POINT('Ctrl Pts',(-37.5361777128299,-31.4965928746404,
18.));
#59563=CARTESIAN_POINT('Ctrl Pts',(-37.7651856275755,-31.1674489725069,
18.));
#59564=CARTESIAN_POINT('Ctrl Pts',(-37.9900344667344,-30.8356998678088,
18.));
#59565=CARTESIAN_POINT('Ctrl Pts',(-38.2106635859155,-30.5014462089352,
18.));
#59566=CARTESIAN_POINT('Ctrl Pts',(-38.6628429613237,-29.8163933416692,
18.));
#59567=CARTESIAN_POINT('Ctrl Pts',(-39.0972929310332,-29.1208215875746,
18.));
#59568=CARTESIAN_POINT('Ctrl Pts',(-39.5135128243241,-28.4156368135623,
18.));
#59569=CARTESIAN_POINT('Ctrl Pts',(-39.9293625109982,-27.7110792658639,
18.));
#59570=CARTESIAN_POINT('Ctrl Pts',(-40.3270144461478,-26.9969259376149,
18.));
#59571=CARTESIAN_POINT('Ctrl Pts',(-40.7060144914488,-26.274105956843,18.));
#59572=CARTESIAN_POINT('Ctrl Pts',(-41.0846796011326,-25.5519247574101,
18.));
#59573=CARTESIAN_POINT('Ctrl Pts',(-41.4447256889349,-24.8210923700318,
18.));
#59574=CARTESIAN_POINT('Ctrl Pts',(-41.7857462696941,-24.0825588483227,
18.));
#59575=CARTESIAN_POINT('Ctrl Pts',(-42.1264645145938,-23.3446800823079,
18.));
#59576=CARTESIAN_POINT('Ctrl Pts',(-42.448190895681,-22.5991139885945,18.));
#59577=CARTESIAN_POINT('Ctrl Pts',(-42.7505675993063,-21.8468291221756,
18.));
#59578=CARTESIAN_POINT('Ctrl Pts',(-43.0525558732906,-21.0955106322569,
18.));
#59579=CARTESIAN_POINT('Ctrl Pts',(-43.3352440854983,-20.3374907828153,
18.));
#59580=CARTESIAN_POINT('Ctrl Pts',(-43.598324345394,-19.5737529819962,18.));
#59581=CARTESIAN_POINT('Ctrl Pts',(-43.8611990228663,-18.810611999304,18.));
#59582=CARTESIAN_POINT('Ctrl Pts',(-44.1044963199916,-18.0417621627802,
18.));
#59583=CARTESIAN_POINT('Ctrl Pts',(-44.3279585209467,-17.2682006924827,
18.));
#59584=CARTESIAN_POINT('Ctrl Pts',(-44.5511707886356,-16.4955044188226,
18.));
#59585=CARTESIAN_POINT('Ctrl Pts',(-44.7545922549351,-15.7181072133933,
18.));
#59586=CARTESIAN_POINT('Ctrl Pts',(-44.9380162577493,-14.9370165444224,
18.));
#59587=CARTESIAN_POINT('Ctrl Pts',(-45.0313865311743,-14.5394096434031,
18.));
#59588=CARTESIAN_POINT('Ctrl Pts',(-45.1195758224217,-14.1408458851963,
18.));
#59589=CARTESIAN_POINT('Ctrl Pts',(-45.2025619355895,-13.7414592977624,
18.));
#59590=CARTESIAN_POINT('',(-35.9959384951176,-30.2041787151332,18.));
#59591=CARTESIAN_POINT('',(-17.6190221917365,-14.7841150227904,18.));
#59592=CARTESIAN_POINT('',(-34.6009561857411,-30.3112822399915,18.));
#59593=CARTESIAN_POINT('Origin',(-35.3531508854311,-30.9702231582522,18.));
#59594=CARTESIAN_POINT('',(-23.,-39.8371685740842,18.));
#59595=CARTESIAN_POINT('Origin',(-1.19904086659517E-13,-1.4210854715202E-13,
18.));
#59596=CARTESIAN_POINT('',(-16.6286143540509,-43.6047734828703,18.));
#59597=CARTESIAN_POINT('Ctrl Pts',(-16.6286143540096,-43.6047734827858,
18.));
#59598=CARTESIAN_POINT('Ctrl Pts',(-18.8450107961508,-42.5215950808033,
18.));
#59599=CARTESIAN_POINT('Ctrl Pts',(-20.976138011788,-41.2633137260105,18.));
#59600=CARTESIAN_POINT('Ctrl Pts',(-23.,-39.8371685740842,18.));
#59601=CARTESIAN_POINT('',(-17.56866714429,-43.5498786998672,18.));
#59602=CARTESIAN_POINT('',(-10.5805717967516,-43.9579515042931,18.));
#59603=CARTESIAN_POINT('',(-18.3265166382238,-56.5277700595814,18.));
#59604=CARTESIAN_POINT('',(-17.56866714429,-43.5498786998672,18.));
#59605=CARTESIAN_POINT('',(-11.3384212906854,-56.9358428640073,18.));
#59606=CARTESIAN_POINT('',(-18.3265166382238,-56.5277700595814,18.));
#59607=CARTESIAN_POINT('',(-10.7008281308737,-46.0172966012375,18.));
#59608=CARTESIAN_POINT('',(-11.3384212906854,-56.9358428640073,18.));
#59609=CARTESIAN_POINT('',(8.50876070567956,-48.2555798975982,18.));
#59610=CARTESIAN_POINT('Ctrl Pts',(8.50876070567956,-48.2555798975982,18.));
#59611=CARTESIAN_POINT('Ctrl Pts',(8.10921021903483,-48.2893345802281,18.));
#59612=CARTESIAN_POINT('Ctrl Pts',(7.70948309898196,-48.318184807544,18.));
#59613=CARTESIAN_POINT('Ctrl Pts',(7.30969683137374,-48.3421283841655,18.));
#59614=CARTESIAN_POINT('Ctrl Pts',(6.4903344600815,-48.3912007693555,18.));
#59615=CARTESIAN_POINT('Ctrl Pts',(5.67072716815546,-48.4196596206763,18.));
#59616=CARTESIAN_POINT('Ctrl Pts',(4.85190979280955,-48.4275242779409,18.));
#59617=CARTESIAN_POINT('Ctrl Pts',(4.0338208098616,-48.4353819390708,18.));
#59618=CARTESIAN_POINT('Ctrl Pts',(3.21652051059572,-48.4226820247691,18.));
#59619=CARTESIAN_POINT('Ctrl Pts',(2.40104061039322,-48.389495803488,18.));
#59620=CARTESIAN_POINT('Ctrl Pts',(1.58628269750797,-48.3563389637169,18.));
#59621=CARTESIAN_POINT('Ctrl Pts',(0.773342136541099,-48.3027320799326,
18.));
#59622=CARTESIAN_POINT('Ctrl Pts',(-0.0367550665778552,-48.2287981514392,
18.));
#59623=CARTESIAN_POINT('Ctrl Pts',(-0.846137205569798,-48.1549294836327,
18.));
#59624=CARTESIAN_POINT('Ctrl Pts',(-1.65268082939617,-48.0607696528264,
18.));
#59625=CARTESIAN_POINT('Ctrl Pts',(-2.45536823331685,-47.9464930614241,
18.));
#59626=CARTESIAN_POINT('Ctrl Pts',(-3.25702327991691,-47.832363444143,18.));
#59627=CARTESIAN_POINT('Ctrl Pts',(-4.0548318460644,-47.6981688032625,18.));
#59628=CARTESIAN_POINT('Ctrl Pts',(-4.8477883300669,-47.5441342016816,18.));
#59629=CARTESIAN_POINT('Ctrl Pts',(-5.64012748982834,-47.390219517518,18.));
#59630=CARTESIAN_POINT('Ctrl Pts',(-6.42762194625921,-47.2164957811652,
18.));
#59631=CARTESIAN_POINT('Ctrl Pts',(-7.20927921482277,-47.0232384165534,
18.));
#59632=CARTESIAN_POINT('Ctrl Pts',(-7.99005956714217,-46.8301978611867,
18.));
#59633=CARTESIAN_POINT('Ctrl Pts',(-8.76501565061606,-46.6176675222901,
18.));
#59634=CARTESIAN_POINT('Ctrl Pts',(-9.53317164254934,-46.3859721588735,
18.));
#59635=CARTESIAN_POINT('Ctrl Pts',(-9.92419469240932,-46.2680296724606,
18.));
#59636=CARTESIAN_POINT('Ctrl Pts',(-10.3134559117797,-46.1451218892995,
18.));
#59637=CARTESIAN_POINT('Ctrl Pts',(-10.7008281308626,-46.0172966012412,
18.));
#59638=CARTESIAN_POINT('',(8.15961682019179,-46.2754865274007,18.));
#59639=CARTESIAN_POINT('',(3.99390808633936,-22.6505783192808,18.));
#59640=CARTESIAN_POINT('',(8.94986234824221,-45.1209481720799,18.));
#59641=CARTESIAN_POINT('Origin',(9.144424573204,-46.1018383497338,18.));
#59642=CARTESIAN_POINT('',(23.,-39.8371685740842,18.));
#59643=CARTESIAN_POINT('Origin',(6.31175685987895E-14,-1.74894258640722E-13,
18.));
#59644=CARTESIAN_POINT('',(29.4485343854062,-36.2031892017778,18.));
#59645=CARTESIAN_POINT('Ctrl Pts',(29.4485343853537,-36.2031892016999,18.));
#59646=CARTESIAN_POINT('Ctrl Pts',(27.40227615007,-37.5810556253112,18.));
#59647=CARTESIAN_POINT('Ctrl Pts',(25.2470089248039,-38.797525254667,18.));
#59648=CARTESIAN_POINT('Ctrl Pts',(23.,-39.8371685740842,18.));
#59649=CARTESIAN_POINT('',(28.9309677136708,-36.9898514075217,18.));
#59650=CARTESIAN_POINT('',(32.7784168026664,-31.1420197146986,18.));
#59651=CARTESIAN_POINT('',(39.7912265717709,-44.1351140013707,18.));
#59652=CARTESIAN_POINT('',(28.9309677136708,-36.9898514075217,18.));
#59653=CARTESIAN_POINT('',(43.6386756607666,-38.2872823085476,18.));
#59654=CARTESIAN_POINT('',(39.7912265717709,-44.1351140013707,18.));
#59655=CARTESIAN_POINT('',(43.6386756607666,-38.2872823085476,18.));
#59656=CARTESIAN_POINT('Ctrl Pts',(52.7966221146313,12.9064860705774,18.));
#59657=CARTESIAN_POINT('Ctrl Pts',(52.7391846522721,12.9274734829174,18.));
#59658=CARTESIAN_POINT('Ctrl Pts',(52.6833098509988,12.9520735040296,18.));
#59659=CARTESIAN_POINT('Ctrl Pts',(52.6291956963058,12.9799861915281,18.));
#59660=CARTESIAN_POINT('Ctrl Pts',(52.575396618885,13.0077363586382,18.));
#59661=CARTESIAN_POINT('Ctrl Pts',(52.5233370565323,13.0387617569737,18.));
#59662=CARTESIAN_POINT('Ctrl Pts',(52.4732434855936,13.0728123808106,18.));
#59663=CARTESIAN_POINT('Ctrl Pts',(52.4354166035921,13.0985248406297,18.));
#59664=CARTESIAN_POINT('Ctrl Pts',(52.3987113360342,13.1259633238972,18.));
#59665=CARTESIAN_POINT('Ctrl Pts',(52.3632409515082,13.1550320009626,18.));
#59666=CARTESIAN_POINT('Ctrl Pts',(52.34482728488,13.1701223625688,18.));
#59667=CARTESIAN_POINT('Ctrl Pts',(52.3267466539926,13.1856521912727,18.));
#59668=CARTESIAN_POINT('Ctrl Pts',(52.3090166072819,13.2016088137114,18.));
#59669=CARTESIAN_POINT('Ctrl Pts',(52.2996792306519,13.2100122316992,18.));
#59670=CARTESIAN_POINT('Ctrl Pts',(52.290437736064,13.2185355104073,18.));
#59671=CARTESIAN_POINT('Ctrl Pts',(52.2813109131323,13.227161085094,18.));
#59672=CARTESIAN_POINT('Ctrl Pts',(52.2382824916349,13.2678263709279,18.));
#59673=CARTESIAN_POINT('Ctrl Pts',(52.1977162889855,13.3108358032842,18.));
#59674=CARTESIAN_POINT('Ctrl Pts',(52.1598201080567,13.3559496827387,18.));
#59675=CARTESIAN_POINT('Ctrl Pts',(52.1226978380937,13.4001422523101,18.));
#59676=CARTESIAN_POINT('Ctrl Pts',(52.0881372055927,13.4463551316942,18.));
#59677=CARTESIAN_POINT('Ctrl Pts',(52.0563765963043,13.4943859943979,18.));
#59678=CARTESIAN_POINT('Ctrl Pts',(52.0333851347596,13.5291554700963,18.));
#59679=CARTESIAN_POINT('Ctrl Pts',(52.0118618266788,13.5648781300802,18.));
#59680=CARTESIAN_POINT('Ctrl Pts',(51.9919136247933,13.6014809507274,18.));
#59681=CARTESIAN_POINT('Ctrl Pts',(51.9814876879778,13.6206114316362,18.));
#59682=CARTESIAN_POINT('Ctrl Pts',(51.9714922558871,13.6399823727779,18.));
#59683=CARTESIAN_POINT('Ctrl Pts',(51.9619442850847,13.6595834362837,18.));
#59684=CARTESIAN_POINT('Ctrl Pts',(51.9575038197887,13.6686992834163,18.));
#59685=CARTESIAN_POINT('Ctrl Pts',(51.9531624130337,13.6778603944405,18.));
#59686=CARTESIAN_POINT('Ctrl Pts',(51.948924721729,13.6870583249534,18.));
#59687=CARTESIAN_POINT('Ctrl Pts',(51.9255871022594,13.7377127466136,18.));
#59688=CARTESIAN_POINT('Ctrl Pts',(51.9053583908605,13.7895496677192,18.));
#59689=CARTESIAN_POINT('Ctrl Pts',(51.8884515319674,13.8423787830974,18.));
#59690=CARTESIAN_POINT('Ctrl Pts',(51.8771391871495,13.877726636496,18.));
#59691=CARTESIAN_POINT('Ctrl Pts',(51.8673149503303,13.9135190517323,18.));
#59692=CARTESIAN_POINT('Ctrl Pts',(51.8590555816082,13.9497009999509,18.));
#59693=CARTESIAN_POINT('Ctrl Pts',(51.8468310253394,14.0032533084619,18.));
#59694=CARTESIAN_POINT('Ctrl Pts',(51.8380328718691,14.0576598787871,18.));
#59695=CARTESIAN_POINT('Ctrl Pts',(51.8326065611663,14.1126100767572,18.));
#59696=CARTESIAN_POINT('Ctrl Pts',(51.830930637981,14.1295815175501,18.));
#59697=CARTESIAN_POINT('Ctrl Pts',(51.8295766661961,14.1466047249362,18.));
#59698=CARTESIAN_POINT('Ctrl Pts',(51.828543856078,14.1636702346734,18.));
#59699=CARTESIAN_POINT('Ctrl Pts',(51.8276375355829,14.1786457088329,18.));
#59700=CARTESIAN_POINT('Ctrl Pts',(51.8269785320498,14.1936603247014,18.));
#59701=CARTESIAN_POINT('Ctrl Pts',(51.826566991848,14.2086715965765,18.));
#59702=CARTESIAN_POINT('Ctrl Pts',(51.8250409572498,14.2643349804729,18.));
#59703=CARTESIAN_POINT('Ctrl Pts',(51.8269058844663,14.3200271043436,18.));
#59704=CARTESIAN_POINT('Ctrl Pts',(51.8320579502604,14.3754301634831,18.));
#59705=CARTESIAN_POINT('Ctrl Pts',(51.8372038210242,14.4307666039798,18.));
#59706=CARTESIAN_POINT('Ctrl Pts',(51.8456293850989,14.4858158153881,18.));
#59707=CARTESIAN_POINT('Ctrl Pts',(51.8572803743357,14.5402457976327,18.));
#59708=CARTESIAN_POINT('Ctrl Pts',(51.8647273765295,14.5750359934649,18.));
#59709=CARTESIAN_POINT('Ctrl Pts',(51.8734930706666,14.6095728457467,18.));
#59710=CARTESIAN_POINT('Ctrl Pts',(51.8835725601024,14.6437631510401,18.));
#59711=CARTESIAN_POINT('Ctrl Pts',(51.8887663989076,14.6613810011831,18.));
#59712=CARTESIAN_POINT('Ctrl Pts',(51.8943091902133,14.6789067372084,18.));
#59713=CARTESIAN_POINT('Ctrl Pts',(51.9002009421238,14.6963268927931,18.));
#59714=CARTESIAN_POINT('Ctrl Pts',(51.9037544840207,14.7068336577858,18.));
#59715=CARTESIAN_POINT('Ctrl Pts',(51.9074348703348,14.7173013531614,18.));
#59716=CARTESIAN_POINT('Ctrl Pts',(51.9112372618813,14.7277145312037,18.));
#59717=CARTESIAN_POINT('Ctrl Pts',(51.9296249995619,14.7780709408272,18.));
#59718=CARTESIAN_POINT('Ctrl Pts',(51.950888554962,14.827232989418,18.));
#59719=CARTESIAN_POINT('Ctrl Pts',(51.9749870630625,14.8748868070182,18.));
#59720=CARTESIAN_POINT('Ctrl Pts',(51.9901200745184,14.9048117204051,18.));
#59721=CARTESIAN_POINT('Ctrl Pts',(52.006371831386,14.9341413324084,18.));
#59722=CARTESIAN_POINT('Ctrl Pts',(52.0237395591854,14.9627903220902,18.));
#59723=CARTESIAN_POINT('Ctrl Pts',(52.0300897392709,14.9732652815005,18.));
#59724=CARTESIAN_POINT('Ctrl Pts',(52.036590534633,14.9836512987207,18.));
#59725=CARTESIAN_POINT('Ctrl Pts',(52.0432374284802,14.9939369612961,18.));
#59726=CARTESIAN_POINT('Ctrl Pts',(52.071139405187,15.0371135674213,18.));
#59727=CARTESIAN_POINT('Ctrl Pts',(52.1015680157944,15.078457457165,18.));
#59728=CARTESIAN_POINT('Ctrl Pts',(52.1344986678541,15.1176697568719,18.));
#59729=CARTESIAN_POINT('Ctrl Pts',(52.1528947874596,15.1395750065495,18.));
#59730=CARTESIAN_POINT('Ctrl Pts',(52.1720723161451,15.160814400533,18.));
#59731=CARTESIAN_POINT('Ctrl Pts',(52.1920310817112,15.1813299718051,18.));
#59732=CARTESIAN_POINT('Ctrl Pts',(52.2060486090393,15.1957385573463,18.));
#59733=CARTESIAN_POINT('Ctrl Pts',(52.2204515743704,15.2097900005096,18.));
#59734=CARTESIAN_POINT('Ctrl Pts',(52.2352228301846,15.2234768233201,18.));
#59735=CARTESIAN_POINT('Ctrl Pts',(54.1532521092111,15.2223467977324,18.));
#59736=CARTESIAN_POINT('Ctrl Pts',(54.1901305933404,15.1879071947037,18.));
#59737=CARTESIAN_POINT('Ctrl Pts',(54.2246310285467,15.1512289528612,18.));
#59738=CARTESIAN_POINT('Ctrl Pts',(54.2567513295154,15.1126319834755,18.));
#59739=CARTESIAN_POINT('Ctrl Pts',(54.2903114638431,15.0723048558287,18.));
#59740=CARTESIAN_POINT('Ctrl Pts',(54.3212739167588,15.0298826695218,18.));
#59741=CARTESIAN_POINT('Ctrl Pts',(54.3496082931449,14.9856806062947,18.));
#59742=CARTESIAN_POINT('Ctrl Pts',(54.3723325448347,14.9502304239334,18.));
#59743=CARTESIAN_POINT('Ctrl Pts',(54.393365943357,14.9136342530605,18.));
#59744=CARTESIAN_POINT('Ctrl Pts',(54.4126765683611,14.8760367445277,18.));
#59745=CARTESIAN_POINT('Ctrl Pts',(54.4208393026161,14.8601440185936,18.));
#59746=CARTESIAN_POINT('Ctrl Pts',(54.4286940175273,14.8440722071043,18.));
#59747=CARTESIAN_POINT('Ctrl Pts',(54.4362374127529,14.8278315944995,18.));
#59748=CARTESIAN_POINT('Ctrl Pts',(54.4405190389662,14.8186134333707,18.));
#59749=CARTESIAN_POINT('Ctrl Pts',(54.4447005519148,14.8093401785886,18.));
#59750=CARTESIAN_POINT('Ctrl Pts',(54.4487750435515,14.8000286716828,18.));
#59751=CARTESIAN_POINT('Ctrl Pts',(54.4705983254202,14.7501555444453,18.));
#59752=CARTESIAN_POINT('Ctrl Pts',(54.4894011486138,14.6990895949691,18.));
#59753=CARTESIAN_POINT('Ctrl Pts',(54.5051559559802,14.6471623387574,18.));
#59754=CARTESIAN_POINT('Ctrl Pts',(54.5211994761642,14.5942834958898,18.));
#59755=CARTESIAN_POINT('Ctrl Pts',(54.5340828409905,14.540510565072,18.));
#59756=CARTESIAN_POINT('Ctrl Pts',(54.5437362577265,14.4861590282357,18.));
#59757=CARTESIAN_POINT('Ctrl Pts',(54.5506403107398,14.4472872067934,18.));
#59758=CARTESIAN_POINT('Ctrl Pts',(54.5558914111236,14.4081186550579,18.));
#59759=CARTESIAN_POINT('Ctrl Pts',(54.559449023704,14.3687624021492,18.));
#59760=CARTESIAN_POINT('Ctrl Pts',(54.5609614737352,14.3520308540687,18.));
#59761=CARTESIAN_POINT('Ctrl Pts',(54.5621676846347,14.3352653382879,18.));
#59762=CARTESIAN_POINT('Ctrl Pts',(54.5630637815993,14.3184741004755,18.));
#59763=CARTESIAN_POINT('Ctrl Pts',(54.5635976657008,14.3084700771749,18.));
#59764=CARTESIAN_POINT('Ctrl Pts',(54.5640211036069,14.2984625720653,18.));
#59765=CARTESIAN_POINT('Ctrl Pts',(54.5643335016801,14.2884609518038,18.));
#59766=CARTESIAN_POINT('Ctrl Pts',(54.5661075110382,14.2316649294805,18.));
#59767=CARTESIAN_POINT('Ctrl Pts',(54.5643085969182,14.1749865267886,18.));
#59768=CARTESIAN_POINT('Ctrl Pts',(54.5588768122569,14.1187579548823,18.));
#59769=CARTESIAN_POINT('Ctrl Pts',(54.555541323331,14.0842297490327,18.));
#59770=CARTESIAN_POINT('Ctrl Pts',(54.5508350741444,14.0498706203909,18.));
#59771=CARTESIAN_POINT('Ctrl Pts',(54.5447349150617,14.0157544413133,18.));
#59772=CARTESIAN_POINT('Ctrl Pts',(54.5350624849657,13.9616597279126,18.));
#59773=CARTESIAN_POINT('Ctrl Pts',(54.5218884030871,13.908175336948,18.));
#59774=CARTESIAN_POINT('Ctrl Pts',(54.5054388352982,13.8555057819067,18.));
#59775=CARTESIAN_POINT('Ctrl Pts',(54.5005174069387,13.8397479550029,18.));
#59776=CARTESIAN_POINT('Ctrl Pts',(54.4953024361436,13.8240630966687,18.));
#59777=CARTESIAN_POINT('Ctrl Pts',(54.4897991057291,13.8084568180236,18.));
#59778=CARTESIAN_POINT('Ctrl Pts',(54.4847109304732,13.7940278314178,18.));
#59779=CARTESIAN_POINT('Ctrl Pts',(54.4793736286687,13.7796597824156,18.));
#59780=CARTESIAN_POINT('Ctrl Pts',(54.4738049082136,13.765391301815,18.));
#59781=CARTESIAN_POINT('Ctrl Pts',(54.4531741179316,13.712529960814,18.));
#59782=CARTESIAN_POINT('Ctrl Pts',(54.4293497755018,13.6609649910116,18.));
#59783=CARTESIAN_POINT('Ctrl Pts',(54.4026149607928,13.6109069383257,18.));
#59784=CARTESIAN_POINT('Ctrl Pts',(54.3752481593716,13.5596655587876,18.));
#59785=CARTESIAN_POINT('Ctrl Pts',(54.3448313135357,13.5100022755867,18.));
#59786=CARTESIAN_POINT('Ctrl Pts',(54.3116127229013,13.4621485545139,18.));
#59787=CARTESIAN_POINT('Ctrl Pts',(54.2914450604171,13.4330956152779,18.));
#59788=CARTESIAN_POINT('Ctrl Pts',(54.270243640872,13.404709837219,18.));
#59789=CARTESIAN_POINT('Ctrl Pts',(54.248055329197,13.3770462315215,18.));
#59790=CARTESIAN_POINT('Ctrl Pts',(54.2358385422418,13.3618147717255,18.));
#59791=CARTESIAN_POINT('Ctrl Pts',(54.2233224644031,13.3468022959008,18.));
#59792=CARTESIAN_POINT('Ctrl Pts',(54.210514166911,13.3320184620734,18.));
#59793=CARTESIAN_POINT('Ctrl Pts',(54.2028017059937,13.3231164404993,18.));
#59794=CARTESIAN_POINT('Ctrl Pts',(54.1949819266705,13.3142958366262,18.));
#59795=CARTESIAN_POINT('Ctrl Pts',(54.1870606016122,13.3055635742289,18.));
#59796=CARTESIAN_POINT('Ctrl Pts',(54.146465975084,13.2608131154156,18.));
#59797=CARTESIAN_POINT('Ctrl Pts',(54.10333569294,13.2185196121713,18.));
#59798=CARTESIAN_POINT('Ctrl Pts',(54.0579299117865,13.1789337623729,18.));
#59799=CARTESIAN_POINT('Ctrl Pts',(54.0284074581576,13.1531953787278,18.));
#59800=CARTESIAN_POINT('Ctrl Pts',(53.9979219697629,13.1286019537641,18.));
#59801=CARTESIAN_POINT('Ctrl Pts',(53.966534783368,13.1052284206224,18.));
#59802=CARTESIAN_POINT('Ctrl Pts',(53.9535624126213,13.0955681046655,18.));
#59803=CARTESIAN_POINT('Ctrl Pts',(53.940435929729,13.0861162377761,18.));
#59804=CARTESIAN_POINT('Ctrl Pts',(53.9271593222801,13.0768784342968,18.));
#59805=CARTESIAN_POINT('Ctrl Pts',(53.9174397053042,13.0701155687181,18.));
#59806=CARTESIAN_POINT('Ctrl Pts',(53.9076405168284,13.0634681523302,18.));
#59807=CARTESIAN_POINT('Ctrl Pts',(53.897771829427,13.0569437429014,18.));
#59808=CARTESIAN_POINT('Ctrl Pts',(53.8470357673058,13.0234010002221,18.));
#59809=CARTESIAN_POINT('Ctrl Pts',(53.7944075338674,12.9930657400092,18.));
#59810=CARTESIAN_POINT('Ctrl Pts',(53.740123223725,12.9662046863981,18.));
#59811=CARTESIAN_POINT('Ctrl Pts',(53.7146984023412,12.9536239335351,18.));
#59812=CARTESIAN_POINT('Ctrl Pts',(53.6889097287653,12.941805763883,18.));
#59813=CARTESIAN_POINT('Ctrl Pts',(53.6627787780123,12.9307804983812,18.));
#59814=CARTESIAN_POINT('Ctrl Pts',(53.6403263881356,12.9213073046241,18.));
#59815=CARTESIAN_POINT('Ctrl Pts',(53.6176212739246,12.9124195098708,18.));
#59816=CARTESIAN_POINT('Ctrl Pts',(53.5946845822246,12.9041113672218,18.));
#59817=CARTESIAN_POINT('Origin',(0.,0.,18.));
#59818=CARTESIAN_POINT('Ctrl Pts',(15.2209662466057,52.1764590205668,18.));
#59819=CARTESIAN_POINT('Ctrl Pts',(15.1740718831799,52.1372104252047,18.));
#59820=CARTESIAN_POINT('Ctrl Pts',(15.1248302485577,52.1011214310192,18.));
#59821=CARTESIAN_POINT('Ctrl Pts',(15.0736000909597,52.0682135291378,18.));
#59822=CARTESIAN_POINT('Ctrl Pts',(15.0226682165857,52.0354972307088,18.));
#59823=CARTESIAN_POINT('Ctrl Pts',(14.9697696730429,52.0059250068959,18.));
#59824=CARTESIAN_POINT('Ctrl Pts',(14.9152342077278,51.9795679908667,18.));
#59825=CARTESIAN_POINT('Ctrl Pts',(14.8740531445005,51.9596651636458,18.));
#59826=CARTESIAN_POINT('Ctrl Pts',(14.831938111089,51.9415966925909,18.));
#59827=CARTESIAN_POINT('Ctrl Pts',(14.7890287317841,51.9254127571039,18.));
#59828=CARTESIAN_POINT('Ctrl Pts',(14.7667532709537,51.9170112228272,18.));
#59829=CARTESIAN_POINT('Ctrl Pts',(14.7442637387324,51.9091178393319,18.));
#59830=CARTESIAN_POINT('Ctrl Pts',(14.7215798846744,51.9017414674401,18.));
#59831=CARTESIAN_POINT('Ctrl Pts',(14.7096336326145,51.8978567661154,18.));
#59832=CARTESIAN_POINT('Ctrl Pts',(14.6976315192819,51.8941150313084,18.));
#59833=CARTESIAN_POINT('Ctrl Pts',(14.6855981509457,51.8905237529518,18.));
#59834=CARTESIAN_POINT('Ctrl Pts',(14.6288668056565,51.8735926621063,18.));
#59835=CARTESIAN_POINT('Ctrl Pts',(14.5713364809609,51.8599659874371,18.));
#59836=CARTESIAN_POINT('Ctrl Pts',(14.5133186620421,51.8497038434798,18.));
#59837=CARTESIAN_POINT('Ctrl Pts',(14.4564856885499,51.8396512740043,18.));
#59838=CARTESIAN_POINT('Ctrl Pts',(14.3991838939685,51.8328273015831,18.));
#59839=CARTESIAN_POINT('Ctrl Pts',(14.3417076889049,51.8293372126129,18.));
#59840=CARTESIAN_POINT('Ctrl Pts',(14.3001007306979,51.8268107412538,18.));
#59841=CARTESIAN_POINT('Ctrl Pts',(14.2584023661317,51.8260323215432,18.));
#59842=CARTESIAN_POINT('Ctrl Pts',(14.2167293111348,51.8270580660935,18.));
#59843=CARTESIAN_POINT('Ctrl Pts',(14.1949488647985,51.827594172077,18.));
#59844=CARTESIAN_POINT('Ctrl Pts',(14.1731754256014,51.8286233369707,18.));
#59845=CARTESIAN_POINT('Ctrl Pts',(14.1514264245833,51.8301550767572,18.));
#59846=CARTESIAN_POINT('Ctrl Pts',(14.1413116392164,51.8308674413925,18.));
#59847=CARTESIAN_POINT('Ctrl Pts',(14.1312071832961,51.8316882253561,18.));
#59848=CARTESIAN_POINT('Ctrl Pts',(14.1211226983366,51.8326172394596,18.));
#59849=CARTESIAN_POINT('Ctrl Pts',(14.0655859083915,51.8377334611929,18.));
#59850=CARTESIAN_POINT('Ctrl Pts',(14.010579492857,51.8461333286653,18.));
#59851=CARTESIAN_POINT('Ctrl Pts',(13.9563747310531,51.8579061060214,18.));
#59852=CARTESIAN_POINT('Ctrl Pts',(13.9201064161194,51.8657832515449,18.));
#59853=CARTESIAN_POINT('Ctrl Pts',(13.8841971505527,51.8751714207574,18.));
#59854=CARTESIAN_POINT('Ctrl Pts',(13.8487329702921,51.8861095759353,18.));
#59855=CARTESIAN_POINT('Ctrl Pts',(13.7962430344238,51.902298955179,18.));
#59856=CARTESIAN_POINT('Ctrl Pts',(13.7447264797303,51.9218828237725,18.));
#59857=CARTESIAN_POINT('Ctrl Pts',(13.6944250448181,51.9446586129267,18.));
#59858=CARTESIAN_POINT('Ctrl Pts',(13.6788893969321,51.9516929379165,18.));
#59859=CARTESIAN_POINT('Ctrl Pts',(13.6634698927207,51.9590319641544,18.));
#59860=CARTESIAN_POINT('Ctrl Pts',(13.6481743336116,51.9666702755676,18.));
#59861=CARTESIAN_POINT('Ctrl Pts',(13.6347520070389,51.9733731302669,18.));
#59862=CARTESIAN_POINT('Ctrl Pts',(13.6214194410696,51.9803097396806,18.));
#59863=CARTESIAN_POINT('Ctrl Pts',(13.6082135027491,51.9874589876079,18.));
#59864=CARTESIAN_POINT('Ctrl Pts',(13.5592445611088,52.0139691147967,18.));
#59865=CARTESIAN_POINT('Ctrl Pts',(13.5119462056412,52.0434302755537,18.));
#59866=CARTESIAN_POINT('Ctrl Pts',(13.4665417533877,52.0755936524918,18.));
#59867=CARTESIAN_POINT('Ctrl Pts',(13.4211918994935,52.1077183533193,18.));
#59868=CARTESIAN_POINT('Ctrl Pts',(13.3777306362705,52.1425397400705,18.));
#59869=CARTESIAN_POINT('Ctrl Pts',(13.336418351779,52.1798448137035,18.));
#59870=CARTESIAN_POINT('Ctrl Pts',(13.310012629919,52.2036892321482,18.));
#59871=CARTESIAN_POINT('Ctrl Pts',(13.284485655765,52.2285490007982,18.));
#59872=CARTESIAN_POINT('Ctrl Pts',(13.2599156980565,52.2543732768879,18.));
#59873=CARTESIAN_POINT('Ctrl Pts',(13.2472551099776,52.2676801993451,18.));
#59874=CARTESIAN_POINT('Ctrl Pts',(13.2348487708532,52.2812432661479,18.));
#59875=CARTESIAN_POINT('Ctrl Pts',(13.2227083469491,52.2950557511153,18.));
#59876=CARTESIAN_POINT('Ctrl Pts',(13.2153859887604,52.3033865938607,18.));
#59877=CARTESIAN_POINT('Ctrl Pts',(13.2081608879655,52.311807752205,18.));
#59878=CARTESIAN_POINT('Ctrl Pts',(13.2010440030961,52.3203073114271,18.));
#59879=CARTESIAN_POINT('Ctrl Pts',(13.1666279154686,52.3614097853814,18.));
#59880=CARTESIAN_POINT('Ctrl Pts',(13.1346840827622,52.4044056088251,18.));
#59881=CARTESIAN_POINT('Ctrl Pts',(13.1054638931938,52.4491024554233,18.));
#59882=CARTESIAN_POINT('Ctrl Pts',(13.087114648167,52.4771704933884,18.));
#59883=CARTESIAN_POINT('Ctrl Pts',(13.0698403219756,52.5059097415566,18.));
#59884=CARTESIAN_POINT('Ctrl Pts',(13.0537134178051,52.5352751363851,18.));
#59885=CARTESIAN_POINT('Ctrl Pts',(13.0478169296962,52.5460120205131,18.));
#59886=CARTESIAN_POINT('Ctrl Pts',(13.0420727750503,52.5568348697425,18.));
#59887=CARTESIAN_POINT('Ctrl Pts',(13.0364885788728,52.5677340663375,18.));
#59888=CARTESIAN_POINT('Ctrl Pts',(13.0130475064211,52.6134861941154,18.));
#59889=CARTESIAN_POINT('Ctrl Pts',(12.9924569304889,52.6605100892665,18.));
#59890=CARTESIAN_POINT('Ctrl Pts',(12.9749633881428,52.7086350162103,18.));
#59891=CARTESIAN_POINT('Ctrl Pts',(12.9651909077076,52.7355192171171,18.));
#59892=CARTESIAN_POINT('Ctrl Pts',(12.9563857854424,52.7627472106675,18.));
#59893=CARTESIAN_POINT('Ctrl Pts',(12.948598136759,52.7902898637941,18.));
#59894=CARTESIAN_POINT('Ctrl Pts',(12.9431286937976,52.8096336961118,18.));
#59895=CARTESIAN_POINT('Ctrl Pts',(12.9381612650277,52.82913275561,18.));
#59896=CARTESIAN_POINT('Ctrl Pts',(12.9336937527446,52.8487684531621,18.));
#59897=CARTESIAN_POINT('Ctrl Pts',(13.8936870225526,54.5092654229862,18.));
#59898=CARTESIAN_POINT('Ctrl Pts',(13.9419518764864,54.5239833380073,18.));
#59899=CARTESIAN_POINT('Ctrl Pts',(13.9909664228046,54.5355224856699,18.));
#59900=CARTESIAN_POINT('Ctrl Pts',(14.0404525674476,54.5440410140802,18.));
#59901=CARTESIAN_POINT('Ctrl Pts',(14.0921569775487,54.5529413939656,18.));
#59902=CARTESIAN_POINT('Ctrl Pts',(14.1443769192153,54.5585445895535,18.));
#59903=CARTESIAN_POINT('Ctrl Pts',(14.1968242396273,54.5609818668625,18.));
#59904=CARTESIAN_POINT('Ctrl Pts',(14.2388871088231,54.5629365687584,18.));
#59905=CARTESIAN_POINT('Ctrl Pts',(14.2810970053263,54.5628539586051,18.));
#59906=CARTESIAN_POINT('Ctrl Pts',(14.3233126980424,54.5607787169104,18.));
#59907=CARTESIAN_POINT('Ctrl Pts',(14.3411576908209,54.5599014916259,18.));
#59908=CARTESIAN_POINT('Ctrl Pts',(14.359003766426,54.5586679663763,18.));
#59909=CARTESIAN_POINT('Ctrl Pts',(14.3768403679013,54.5570804251692,18.));
#59910=CARTESIAN_POINT('Ctrl Pts',(14.3869641761631,54.5561793587407,18.));
#59911=CARTESIAN_POINT('Ctrl Pts',(14.3970856400397,54.5551640486899,18.));
#59912=CARTESIAN_POINT('Ctrl Pts',(14.4071867211758,54.554036933109,18.));
#59913=CARTESIAN_POINT('Ctrl Pts',(14.46128977502,54.5479999164633,18.));
#59914=CARTESIAN_POINT('Ctrl Pts',(14.5149156125182,54.53875069329,18.));
#59915=CARTESIAN_POINT('Ctrl Pts',(14.5677633543885,54.5264311541972,18.));
#59916=CARTESIAN_POINT('Ctrl Pts',(14.6215795301015,54.51388585979,18.));
#59917=CARTESIAN_POINT('Ctrl Pts',(14.6745899303726,54.498156745542,18.));
#59918=CARTESIAN_POINT('Ctrl Pts',(14.7264864439584,54.4793411079432,18.));
#59919=CARTESIAN_POINT('Ctrl Pts',(14.7636024302316,54.4658843090452,18.));
#59920=CARTESIAN_POINT('Ctrl Pts',(14.8001489167129,54.4508476461193,18.));
#59921=CARTESIAN_POINT('Ctrl Pts',(14.8360112141901,54.4342505283932,18.));
#59922=CARTESIAN_POINT('Ctrl Pts',(14.8512574582442,54.4271945468959,18.));
#59923=CARTESIAN_POINT('Ctrl Pts',(14.8663799984359,54.4198563674573,18.));
#59924=CARTESIAN_POINT('Ctrl Pts',(14.8813697562834,54.4122367571808,18.));
#59925=CARTESIAN_POINT('Ctrl Pts',(14.8903005158295,54.4076970636177,18.));
#59926=CARTESIAN_POINT('Ctrl Pts',(14.8991790662204,54.4030599782254,18.));
#59927=CARTESIAN_POINT('Ctrl Pts',(14.9079969993248,54.3983296699863,18.));
#59928=CARTESIAN_POINT('Ctrl Pts',(14.9580707729375,54.3714680028497,18.));
#59929=CARTESIAN_POINT('Ctrl Pts',(15.0062562237396,54.3415708986464,18.));
#59930=CARTESIAN_POINT('Ctrl Pts',(15.052235675618,54.3087525448002,18.));
#59931=CARTESIAN_POINT('Ctrl Pts',(15.080470042487,54.288599946092,18.));
#59932=CARTESIAN_POINT('Ctrl Pts',(15.1078726148529,54.2673447838712,18.));
#59933=CARTESIAN_POINT('Ctrl Pts',(15.1343678441299,54.245003945279,18.));
#59934=CARTESIAN_POINT('Ctrl Pts',(15.1763790053575,54.209580036988,18.));
#59935=CARTESIAN_POINT('Ctrl Pts',(15.2161107900716,54.1714287640077,18.));
#59936=CARTESIAN_POINT('Ctrl Pts',(15.2534991669625,54.1308482498305,18.));
#59937=CARTESIAN_POINT('Ctrl Pts',(15.2646851435514,54.1187072391929,18.));
#59938=CARTESIAN_POINT('Ctrl Pts',(15.2756611560254,54.1063484965527,18.));
#59939=CARTESIAN_POINT('Ctrl Pts',(15.2864249364023,54.0937793159867,18.));
#59940=CARTESIAN_POINT('Ctrl Pts',(15.296376721656,54.0821583258301,18.));
#59941=CARTESIAN_POINT('Ctrl Pts',(15.3061511701423,54.0703520539335,18.));
#59942=CARTESIAN_POINT('Ctrl Pts',(15.3157236805298,54.0583951512571,18.));
#59943=CARTESIAN_POINT('Ctrl Pts',(15.3511875377787,54.014097691919,18.));
#59944=CARTESIAN_POINT('Ctrl Pts',(15.3839319325097,53.9676827164785,18.));
#59945=CARTESIAN_POINT('Ctrl Pts',(15.4139160661048,53.9195006536869,18.));
#59946=CARTESIAN_POINT('Ctrl Pts',(15.4446090042121,53.8701795997215,18.));
#59947=CARTESIAN_POINT('Ctrl Pts',(15.4724102509795,53.8190061740294,18.));
#59948=CARTESIAN_POINT('Ctrl Pts',(15.497243500525,53.7663111449781,18.));
#59949=CARTESIAN_POINT('Ctrl Pts',(15.5123202613396,53.7343189424406,18.));
#59950=CARTESIAN_POINT('Ctrl Pts',(15.5263023651589,53.7017650594462,18.));
#59951=CARTESIAN_POINT('Ctrl Pts',(15.5391656032547,53.668717588239,18.));
#59952=CARTESIAN_POINT('Ctrl Pts',(15.5462480435936,53.6505218010325,18.));
#59953=CARTESIAN_POINT('Ctrl Pts',(15.5529911929917,53.6321763121665,18.));
#59954=CARTESIAN_POINT('Ctrl Pts',(15.5593902229536,53.6136920745805,18.));
#59955=CARTESIAN_POINT('Ctrl Pts',(15.5632433723038,53.6025618675853,18.));
#59956=CARTESIAN_POINT('Ctrl Pts',(15.5669723526287,53.5913794289557,18.));
#59957=CARTESIAN_POINT('Ctrl Pts',(15.5705740541365,53.5801532197423,18.));
#59958=CARTESIAN_POINT('Ctrl Pts',(15.5890317873762,53.5226219738838,18.));
#59959=CARTESIAN_POINT('Ctrl Pts',(15.6040939073564,53.4641232630989,18.));
#59960=CARTESIAN_POINT('Ctrl Pts',(15.6156733811598,53.4050077405015,18.));
#59961=CARTESIAN_POINT('Ctrl Pts',(15.6232022585969,53.3665713200026,18.));
#59962=CARTESIAN_POINT('Ctrl Pts',(15.6292580546325,53.3278733667412,18.));
#59963=CARTESIAN_POINT('Ctrl Pts',(15.6338065434899,53.2890044670766,18.));
#59964=CARTESIAN_POINT('Ctrl Pts',(15.6356864328875,53.2729399597947,18.));
#59965=CARTESIAN_POINT('Ctrl Pts',(15.6373087460133,53.2568462124372,18.));
#59966=CARTESIAN_POINT('Ctrl Pts',(15.6386706145235,53.2407294854927,18.));
#59967=CARTESIAN_POINT('Ctrl Pts',(15.6396676228531,53.2289306143917,18.));
#59968=CARTESIAN_POINT('Ctrl Pts',(15.6405248635805,53.2171205569137,18.));
#59969=CARTESIAN_POINT('Ctrl Pts',(15.6412408277512,53.205311815233,18.));
#59970=CARTESIAN_POINT('Ctrl Pts',(15.6449216835252,53.1446016892555,18.));
#59971=CARTESIAN_POINT('Ctrl Pts',(15.6448786914156,53.0838566394801,18.));
#59972=CARTESIAN_POINT('Ctrl Pts',(15.6409989084031,53.0234144938957,18.));
#59973=CARTESIAN_POINT('Ctrl Pts',(15.6391817516166,52.9951054738585,18.));
#59974=CARTESIAN_POINT('Ctrl Pts',(15.6365222466638,52.9668626417859,18.));
#59975=CARTESIAN_POINT('Ctrl Pts',(15.6330049221515,52.9387198431847,18.));
#59976=CARTESIAN_POINT('Ctrl Pts',(15.6299827554381,52.91453889859,18.));
#59977=CARTESIAN_POINT('Ctrl Pts',(15.6263272558779,52.8904317889029,18.));
#59978=CARTESIAN_POINT('Ctrl Pts',(15.6220539738783,52.8664139542998,18.));
#59979=CARTESIAN_POINT('Ctrl Pts',(-37.5756558680257,39.2699729499893,18.));
#59980=CARTESIAN_POINT('Ctrl Pts',(-37.5651127690922,39.2097369422873,18.));
#59981=CARTESIAN_POINT('Ctrl Pts',(-37.5584799714475,39.1490477940627,18.));
#59982=CARTESIAN_POINT('Ctrl Pts',(-37.5555966212126,39.0882269703887,18.));
#59983=CARTESIAN_POINT('Ctrl Pts',(-37.5527300631013,39.0277603564721,18.));
#59984=CARTESIAN_POINT('Ctrl Pts',(-37.553569953746,38.9671624857772,18.));
#59985=CARTESIAN_POINT('Ctrl Pts',(-37.5580129364599,38.9067545255738,18.));
#59986=CARTESIAN_POINT('Ctrl Pts',(-37.5613679468783,38.8611389225246,18.));
#59987=CARTESIAN_POINT('Ctrl Pts',(-37.5667786506927,38.8156316117443,18.));
#59988=CARTESIAN_POINT('Ctrl Pts',(-37.5742186551894,38.7703786151083,18.));
#59989=CARTESIAN_POINT('Ctrl Pts',(-37.5780809441846,38.7468866735401,18.));
#59990=CARTESIAN_POINT('Ctrl Pts',(-37.5824903524789,38.7234634071241,18.));
#59991=CARTESIAN_POINT('Ctrl Pts',(-37.5874446737534,38.7001303514373,18.));
#59992=CARTESIAN_POINT('Ctrl Pts',(-37.5900538576765,38.6878420418179,18.));
#59993=CARTESIAN_POINT('Ctrl Pts',(-37.5928147908849,38.6755768363574,18.));
#59994=CARTESIAN_POINT('Ctrl Pts',(-37.5957216552661,38.6633597908174,18.));
#59995=CARTESIAN_POINT('Ctrl Pts',(-37.6094259854369,38.605762874059,18.));
#59996=CARTESIAN_POINT('Ctrl Pts',(-37.6263915747065,38.5491262011484,18.));
#59997=CARTESIAN_POINT('Ctrl Pts',(-37.6465146580723,38.4937496146526,18.));
#59998=CARTESIAN_POINT('Ctrl Pts',(-37.6662269366984,38.439503519135,18.));
#59999=CARTESIAN_POINT('Ctrl Pts',(-37.6889696982612,38.3864657328387,18.));
#60000=CARTESIAN_POINT('Ctrl Pts',(-37.7146868377003,38.3349439029342,18.));
#60001=CARTESIAN_POINT('Ctrl Pts',(-37.7333032641332,38.2976476725983,18.));
#60002=CARTESIAN_POINT('Ctrl Pts',(-37.7534791916943,38.2611463231356,18.));
#60003=CARTESIAN_POINT('Ctrl Pts',(-37.7752048261667,38.2255690008542,18.));
#60004=CARTESIAN_POINT('Ctrl Pts',(-37.7865596505648,38.2069746418461,18.));
#60005=CARTESIAN_POINT('Ctrl Pts',(-37.7983379414309,38.188632883801,18.));
#60006=CARTESIAN_POINT('Ctrl Pts',(-37.8105392196984,38.1705635815837,18.));
#60007=CARTESIAN_POINT('Ctrl Pts',(-37.8162136717173,38.1621600859665,18.));
#60008=CARTESIAN_POINT('Ctrl Pts',(-37.8219768455385,38.1538197468508,18.));
#60009=CARTESIAN_POINT('Ctrl Pts',(-37.8278237560891,38.1455508194946,18.));
#60010=CARTESIAN_POINT('Ctrl Pts',(-37.8600240522425,38.1000119135318,18.));
#60011=CARTESIAN_POINT('Ctrl Pts',(-37.8948027203391,38.0565742506206,18.));
#60012=CARTESIAN_POINT('Ctrl Pts',(-37.932101350128,38.0155174319281,18.));
#60013=CARTESIAN_POINT('Ctrl Pts',(-37.9570573615923,37.9880468668221,18.));
#60014=CARTESIAN_POINT('Ctrl Pts',(-37.9831422874089,37.9616427832137,18.));
#60015=CARTESIAN_POINT('Ctrl Pts',(-38.0103468288125,37.9363991775294,18.));
#60016=CARTESIAN_POINT('Ctrl Pts',(-38.050612215002,37.8990361682947,18.));
#60017=CARTESIAN_POINT('Ctrl Pts',(-38.0933303033917,37.8642134925913,18.));
#60018=CARTESIAN_POINT('Ctrl Pts',(-38.1382048591451,37.8320391955257,18.));
#60019=CARTESIAN_POINT('Ctrl Pts',(-38.1520648967442,37.8221017831198,18.));
#60020=CARTESIAN_POINT('Ctrl Pts',(-38.1661307314527,37.8124173314208,18.));
#60021=CARTESIAN_POINT('Ctrl Pts',(-38.1803937730742,37.8029898884102,18.));
#60022=CARTESIAN_POINT('Ctrl Pts',(-38.1929089479187,37.7947177329509,18.));
#60023=CARTESIAN_POINT('Ctrl Pts',(-38.2055816457065,37.7866401763901,18.));
#60024=CARTESIAN_POINT('Ctrl Pts',(-38.2183751516207,37.7787785855269,18.));
#60025=CARTESIAN_POINT('Ctrl Pts',(-38.2658171634217,37.7496255379568,18.));
#60026=CARTESIAN_POINT('Ctrl Pts',(-38.3149793341025,37.723394852447,18.));
#60027=CARTESIAN_POINT('Ctrl Pts',(-38.365534594144,37.700155493664,18.));
#60028=CARTESIAN_POINT('Ctrl Pts',(-38.4160291498247,37.6769440396019,18.));
#60029=CARTESIAN_POINT('Ctrl Pts',(-38.4679146667789,37.6567165566507,18.));
#60030=CARTESIAN_POINT('Ctrl Pts',(-38.5208765564485,37.6395920241963,18.));
#60031=CARTESIAN_POINT('Ctrl Pts',(-38.5547280084067,37.6286466011514,18.));
#60032=CARTESIAN_POINT('Ctrl Pts',(-38.5890193652551,37.6189698569052,18.));
#60033=CARTESIAN_POINT('Ctrl Pts',(-38.6236674824541,37.6106041450253,18.));
#60034=CARTESIAN_POINT('Ctrl Pts',(-38.641521850756,37.6062932469711,18.));
#60035=CARTESIAN_POINT('Ctrl Pts',(-38.6594709236641,37.6023306259802,18.));
#60036=CARTESIAN_POINT('Ctrl Pts',(-38.677503044697,37.5987230218509,18.));
#60037=CARTESIAN_POINT('Ctrl Pts',(-38.6883788046389,37.5965471582126,18.));
#60038=CARTESIAN_POINT('Ctrl Pts',(-38.6992841521561,37.5945006838765,18.));
#60039=CARTESIAN_POINT('Ctrl Pts',(-38.7102032898677,37.5925871316739,18.));
#60040=CARTESIAN_POINT('Ctrl Pts',(-38.763006061038,37.583333575052,18.));
#60041=CARTESIAN_POINT('Ctrl Pts',(-38.8162124112958,37.5771677759252,18.));
#60042=CARTESIAN_POINT('Ctrl Pts',(-38.8695301449481,37.5742112603263,18.));
#60043=CARTESIAN_POINT('Ctrl Pts',(-38.9030118817427,37.5723546683385,18.));
#60044=CARTESIAN_POINT('Ctrl Pts',(-38.9365374743059,37.5717646060231,18.));
#60045=CARTESIAN_POINT('Ctrl Pts',(-38.970031659091,37.5724813268559,18.));
#60046=CARTESIAN_POINT('Ctrl Pts',(-38.9822787358886,37.5727433942905,18.));
#60047=CARTESIAN_POINT('Ctrl Pts',(-38.9945241009328,37.5731803873939,18.));
#60048=CARTESIAN_POINT('Ctrl Pts',(-39.006755607008,37.5737941004355,18.));
#60049=CARTESIAN_POINT('Ctrl Pts',(-39.05809813714,37.5763702002338,18.));
#60050=CARTESIAN_POINT('Ctrl Pts',(-39.109116914763,37.5820508279815,18.));
#60051=CARTESIAN_POINT('Ctrl Pts',(-39.1595408594659,37.5909641089067,18.));
#60052=CARTESIAN_POINT('Ctrl Pts',(-39.187706877111,37.5959429265953,18.));
#60053=CARTESIAN_POINT('Ctrl Pts',(-39.2156870323819,37.6019312274164,18.));
#60054=CARTESIAN_POINT('Ctrl Pts',(-39.2434310600143,37.6089578358496,18.));
#60055=CARTESIAN_POINT('Ctrl Pts',(-39.2629177980487,37.6138931566914,18.));
#60056=CARTESIAN_POINT('Ctrl Pts',(-39.2822879943277,37.6193408368567,18.));
#60057=CARTESIAN_POINT('Ctrl Pts',(-39.3015265966439,37.6252897660473,18.));
#60058=CARTESIAN_POINT('Ctrl Pts',(-40.2595650866584,39.2869186252538,18.));
#60059=CARTESIAN_POINT('Ctrl Pts',(-40.2481791157548,39.3360745846547,18.));
#60060=CARTESIAN_POINT('Ctrl Pts',(-40.233665287806,39.3842904001651,18.));
#60061=CARTESIAN_POINT('Ctrl Pts',(-40.2162996606326,39.4314043435469,18.));
#60062=CARTESIAN_POINT('Ctrl Pts',(-40.1981554153043,39.4806307226793,18.));
#60063=CARTESIAN_POINT('Ctrl Pts',(-40.1768978215462,39.5286549715329,18.));
#60064=CARTESIAN_POINT('Ctrl Pts',(-40.1527847010642,39.5752932074852,18.));
#60065=CARTESIAN_POINT('Ctrl Pts',(-40.1334453389403,39.6126983095988,18.));
#60066=CARTESIAN_POINT('Ctrl Pts',(-40.1122679418623,39.6492120507124,18.));
#60067=CARTESIAN_POINT('Ctrl Pts',(-40.089361863191,39.6847344690018,18.));
#60068=CARTESIAN_POINT('Ctrl Pts',(-40.0796819049363,39.6997460094353,18.));
#60069=CARTESIAN_POINT('Ctrl Pts',(-40.0696929904195,39.7145804305273,18.));
#60070=CARTESIAN_POINT('Ctrl Pts',(-40.0594023733884,39.7292297389137,18.));
#60071=CARTESIAN_POINT('Ctrl Pts',(-40.0535563601133,39.7375518882114,18.));
#60072=CARTESIAN_POINT('Ctrl Pts',(-40.0476124487805,39.7458148202868,18.));
#60073=CARTESIAN_POINT('Ctrl Pts',(-40.0415817907732,39.7540041063919,18.));
#60074=CARTESIAN_POINT('Ctrl Pts',(-40.0093013797014,39.7978390447242,18.));
#60075=CARTESIAN_POINT('Ctrl Pts',(-39.9744777462107,39.8396546716854,18.));
#60076=CARTESIAN_POINT('Ctrl Pts',(-39.9373842779719,39.8792613960026,18.));
#60077=CARTESIAN_POINT('Ctrl Pts',(-39.8996105080951,39.9195945155777,18.));
#60078=CARTESIAN_POINT('Ctrl Pts',(-39.8594823789697,39.9576379445105,18.));
#60079=CARTESIAN_POINT('Ctrl Pts',(-39.817238289424,39.9931735245898,18.));
#60080=CARTESIAN_POINT('Ctrl Pts',(-39.7870250053652,40.0185888332561,18.));
#60081=CARTESIAN_POINT('Ctrl Pts',(-39.7557282762375,40.0427209888158,18.));
#60082=CARTESIAN_POINT('Ctrl Pts',(-39.7234222902936,40.0654803762021,18.));
#60083=CARTESIAN_POINT('Ctrl Pts',(-39.7096908088931,40.0751541284635,18.));
#60084=CARTESIAN_POINT('Ctrl Pts',(-39.6957768723929,40.0845797514891,18.));
#60085=CARTESIAN_POINT('Ctrl Pts',(-39.6816856838153,40.0937497716388,18.));
#60086=CARTESIAN_POINT('Ctrl Pts',(-39.6732915903904,40.0992123346739,18.));
#60087=CARTESIAN_POINT('Ctrl Pts',(-39.6648392875157,40.104581065436,18.));
#60088=CARTESIAN_POINT('Ctrl Pts',(-39.6563366062018,40.1098507565136,18.));
#60089=CARTESIAN_POINT('Ctrl Pts',(-39.6080360371336,40.1397859109041,18.));
#60090=CARTESIAN_POINT('Ctrl Pts',(-39.5580510184926,40.1665680778016,18.));
#60091=CARTESIAN_POINT('Ctrl Pts',(-39.5066393729943,40.1899792587996,18.));
#60092=CARTESIAN_POINT('Ctrl Pts',(-39.4750618486744,40.2043586300522,18.));
#60093=CARTESIAN_POINT('Ctrl Pts',(-39.4429452140606,40.217465799326,18.));
#60094=CARTESIAN_POINT('Ctrl Pts',(-39.4103419265004,40.2292437480239,18.));
#60095=CARTESIAN_POINT('Ctrl Pts',(-39.3586573390136,40.2479148227972,18.));
#60096=CARTESIAN_POINT('Ctrl Pts',(-39.3057507659291,40.2632482055135,18.));
#60097=CARTESIAN_POINT('Ctrl Pts',(-39.2519123537495,40.2753374915748,18.));
#60098=CARTESIAN_POINT('Ctrl Pts',(-39.2358056778285,40.2789542069425,18.));
#60099=CARTESIAN_POINT('Ctrl Pts',(-39.2196154532535,40.2822802513834,18.));
#60100=CARTESIAN_POINT('Ctrl Pts',(-39.2033491283307,40.2853173071474,18.));
#60101=CARTESIAN_POINT('Ctrl Pts',(-39.1883094890373,40.2881253306819,18.));
#60102=CARTESIAN_POINT('Ctrl Pts',(-39.1731980803203,40.2906871462819,18.));
#60103=CARTESIAN_POINT('Ctrl Pts',(-39.1580572086001,40.2929987736051,18.));
#60104=CARTESIAN_POINT('Ctrl Pts',(-39.1019623295839,40.3015630397466,18.));
#60105=CARTESIAN_POINT('Ctrl Pts',(-39.0453935804777,40.3067133780786,18.));
#60106=CARTESIAN_POINT('Ctrl Pts',(-38.988674785285,40.3085896575269,18.));
#60107=CARTESIAN_POINT('Ctrl Pts',(-38.9306156897047,40.3105102746249,18.));
#60108=CARTESIAN_POINT('Ctrl Pts',(-38.8723984153787,40.3090004242116,18.));
#60109=CARTESIAN_POINT('Ctrl Pts',(-38.8143475050087,40.3041593897172,18.));
#60110=CARTESIAN_POINT('Ctrl Pts',(-38.7791040438476,40.3012203348411,18.));
#60111=CARTESIAN_POINT('Ctrl Pts',(-38.7439215217934,40.297052459211,18.));
#60112=CARTESIAN_POINT('Ctrl Pts',(-38.7088709965466,40.2916688390196,18.));
#60113=CARTESIAN_POINT('Ctrl Pts',(-38.6895721262637,40.2887046098962,18.));
#60114=CARTESIAN_POINT('Ctrl Pts',(-38.6703132641282,40.2853716920803,18.));
#60115=CARTESIAN_POINT('Ctrl Pts',(-38.6511063076066,40.2816713797398,18.));
#60116=CARTESIAN_POINT('Ctrl Pts',(-38.6395410469613,40.2794432767793,18.));
#60117=CARTESIAN_POINT('Ctrl Pts',(-38.627992637109,40.2770815256585,18.));
#60118=CARTESIAN_POINT('Ctrl Pts',(-38.6164699649865,40.2745876647122,18.));
#60119=CARTESIAN_POINT('Ctrl Pts',(-38.557419079826,40.2618072354178,18.));
#60120=CARTESIAN_POINT('Ctrl Pts',(-38.4992281803323,40.2456023804861,18.));
#60121=CARTESIAN_POINT('Ctrl Pts',(-38.4422443841854,40.2260730329326,18.));
#60122=CARTESIAN_POINT('Ctrl Pts',(-38.4051943363965,40.2133753309704,18.));
#60123=CARTESIAN_POINT('Ctrl Pts',(-38.368654306916,40.1992711514025,18.));
#60124=CARTESIAN_POINT('Ctrl Pts',(-38.3327198362902,40.183776140909,18.));
#60125=CARTESIAN_POINT('Ctrl Pts',(-38.3178657816824,40.1773710449659,18.));
#60126=CARTESIAN_POINT('Ctrl Pts',(-38.3031152165708,40.170728187765,18.));
#60127=CARTESIAN_POINT('Ctrl Pts',(-38.2884749985355,40.1638482153583,18.));
#60128=CARTESIAN_POINT('Ctrl Pts',(-38.2777585350481,40.1588121583192,18.));
#60129=CARTESIAN_POINT('Ctrl Pts',(-38.2671022703707,40.1536494636781,18.));
#60130=CARTESIAN_POINT('Ctrl Pts',(-38.2565177796711,40.148365072953,18.));
#60131=CARTESIAN_POINT('Ctrl Pts',(-38.2021024002753,40.121197764261,18.));
#60132=CARTESIAN_POINT('Ctrl Pts',(-38.149518572045,40.0907880130311,18.));
#60133=CARTESIAN_POINT('Ctrl Pts',(-38.0991152601742,40.0572068987011,18.));
#60134=CARTESIAN_POINT('Ctrl Pts',(-38.0755109333516,40.0414805591354,18.));
#60135=CARTESIAN_POINT('Ctrl Pts',(-38.0523849413559,40.0250579742236,18.));
#60136=CARTESIAN_POINT('Ctrl Pts',(-38.0297743098615,40.0079426645895,18.));
#60137=CARTESIAN_POINT('Ctrl Pts',(-38.0103443715311,39.9932350076725,18.));
#60138=CARTESIAN_POINT('Ctrl Pts',(-37.9912950014703,39.9780157739289,18.));
#60139=CARTESIAN_POINT('Ctrl Pts',(-37.9726317990811,39.9623061512025,18.));
#60140=CARTESIAN_POINT('Ctrl Pts',(-52.7966221146314,-12.9064860705774,
18.));
#60141=CARTESIAN_POINT('Ctrl Pts',(-52.7391846522721,-12.9274734829173,
18.));
#60142=CARTESIAN_POINT('Ctrl Pts',(-52.6833098509988,-12.9520735040296,
18.));
#60143=CARTESIAN_POINT('Ctrl Pts',(-52.6291956963058,-12.9799861915281,
18.));
#60144=CARTESIAN_POINT('Ctrl Pts',(-52.5753966188852,-13.0077363586381,
18.));
#60145=CARTESIAN_POINT('Ctrl Pts',(-52.5233370565326,-13.0387617569735,
18.));
#60146=CARTESIAN_POINT('Ctrl Pts',(-52.4732434855941,-13.0728123808102,
18.));
#60147=CARTESIAN_POINT('Ctrl Pts',(-52.4354166035925,-13.0985248406294,
18.));
#60148=CARTESIAN_POINT('Ctrl Pts',(-52.3987113360346,-13.1259633238969,
18.));
#60149=CARTESIAN_POINT('Ctrl Pts',(-52.3632409515086,-13.1550320009623,
18.));
#60150=CARTESIAN_POINT('Ctrl Pts',(-52.3448272848805,-13.1701223625684,
18.));
#60151=CARTESIAN_POINT('Ctrl Pts',(-52.3267466539931,-13.1856521912722,
18.));
#60152=CARTESIAN_POINT('Ctrl Pts',(-52.3090166072825,-13.2016088137109,
18.));
#60153=CARTESIAN_POINT('Ctrl Pts',(-52.2996792306588,-13.210012231693,18.));
#60154=CARTESIAN_POINT('Ctrl Pts',(-52.2904377360769,-13.2185355103954,
18.));
#60155=CARTESIAN_POINT('Ctrl Pts',(-52.2813109131512,-13.2271610850761,
18.));
#60156=CARTESIAN_POINT('Ctrl Pts',(-52.2382824916528,-13.2678263709096,
18.));
#60157=CARTESIAN_POINT('Ctrl Pts',(-52.1977162890024,-13.3108358032656,
18.));
#60158=CARTESIAN_POINT('Ctrl Pts',(-52.1598201080725,-13.3559496827199,
18.));
#60159=CARTESIAN_POINT('Ctrl Pts',(-52.1226978381087,-13.4001422522907,
18.));
#60160=CARTESIAN_POINT('Ctrl Pts',(-52.088137205607,-13.4463551316742,18.));
#60161=CARTESIAN_POINT('Ctrl Pts',(-52.0563765963178,-13.4943859943775,
18.));
#60162=CARTESIAN_POINT('Ctrl Pts',(-52.0333851347714,-13.5291554700772,
18.));
#60163=CARTESIAN_POINT('Ctrl Pts',(-52.0118618266889,-13.5648781300626,
18.));
#60164=CARTESIAN_POINT('Ctrl Pts',(-51.991913624802,-13.6014809507113,18.));
#60165=CARTESIAN_POINT('Ctrl Pts',(-51.9814876879865,-13.6206114316197,
18.));
#60166=CARTESIAN_POINT('Ctrl Pts',(-51.9714922558957,-13.6399823727608,
18.));
#60167=CARTESIAN_POINT('Ctrl Pts',(-51.9619442850932,-13.6595834362661,
18.));
#60168=CARTESIAN_POINT('Ctrl Pts',(-51.9575038197999,-13.6686992833929,
18.));
#60169=CARTESIAN_POINT('Ctrl Pts',(-51.9531624130475,-13.6778603944113,
18.));
#60170=CARTESIAN_POINT('Ctrl Pts',(-51.9489247217451,-13.6870583249183,
18.));
#60171=CARTESIAN_POINT('Ctrl Pts',(-51.925587102274,-13.7377127465782,18.));
#60172=CARTESIAN_POINT('Ctrl Pts',(-51.9053583908736,-13.7895496676836,
18.));
#60173=CARTESIAN_POINT('Ctrl Pts',(-51.8884515319789,-13.8423787830615,
18.));
#60174=CARTESIAN_POINT('Ctrl Pts',(-51.8771391871561,-13.8777266364718,
18.));
#60175=CARTESIAN_POINT('Ctrl Pts',(-51.867314950333,-13.91351905172,18.));
#60176=CARTESIAN_POINT('Ctrl Pts',(-51.8590555816082,-13.9497009999509,
18.));
#60177=CARTESIAN_POINT('Ctrl Pts',(-51.8468310253394,-14.0032533084619,
18.));
#60178=CARTESIAN_POINT('Ctrl Pts',(-51.8380328718691,-14.0576598787871,
18.));
#60179=CARTESIAN_POINT('Ctrl Pts',(-51.8326065611663,-14.1126100767572,
18.));
#60180=CARTESIAN_POINT('Ctrl Pts',(-51.830930637981,-14.1295815175498,18.));
#60181=CARTESIAN_POINT('Ctrl Pts',(-51.8295766661961,-14.1466047249358,
18.));
#60182=CARTESIAN_POINT('Ctrl Pts',(-51.828543856078,-14.1636702346728,18.));
#60183=CARTESIAN_POINT('Ctrl Pts',(-51.8276375355831,-14.1786457088294,
18.));
#60184=CARTESIAN_POINT('Ctrl Pts',(-51.8269785320501,-14.193660324695,18.));
#60185=CARTESIAN_POINT('Ctrl Pts',(-51.8265669918482,-14.2086715965672,
18.));
#60186=CARTESIAN_POINT('Ctrl Pts',(-51.8250409572497,-14.2643349804636,
18.));
#60187=CARTESIAN_POINT('Ctrl Pts',(-51.8269058844658,-14.3200271043344,
18.));
#60188=CARTESIAN_POINT('Ctrl Pts',(-51.8320579502595,-14.3754301634739,
18.));
#60189=CARTESIAN_POINT('Ctrl Pts',(-51.837203821023,-14.4307666039711,18.));
#60190=CARTESIAN_POINT('Ctrl Pts',(-51.8456293850974,-14.4858158153797,
18.));
#60191=CARTESIAN_POINT('Ctrl Pts',(-51.857280374334,-14.5402457976247,18.));
#60192=CARTESIAN_POINT('Ctrl Pts',(-51.8647273765276,-14.5750359934568,
18.));
#60193=CARTESIAN_POINT('Ctrl Pts',(-51.8734930706644,-14.6095728457385,
18.));
#60194=CARTESIAN_POINT('Ctrl Pts',(-51.8835725600999,-14.6437631510318,
18.));
#60195=CARTESIAN_POINT('Ctrl Pts',(-51.8887663989049,-14.6613810011742,
18.));
#60196=CARTESIAN_POINT('Ctrl Pts',(-51.8943091902103,-14.678906737199,18.));
#60197=CARTESIAN_POINT('Ctrl Pts',(-51.9002009421205,-14.6963268927831,
18.));
#60198=CARTESIAN_POINT('Ctrl Pts',(-51.9037544840212,-14.7068336577877,
18.));
#60199=CARTESIAN_POINT('Ctrl Pts',(-51.9074348703396,-14.7173013531751,
18.));
#60200=CARTESIAN_POINT('Ctrl Pts',(-51.9112372618906,-14.7277145312291,
18.));
#60201=CARTESIAN_POINT('Ctrl Pts',(-51.9296249995719,-14.7780709408516,
18.));
#60202=CARTESIAN_POINT('Ctrl Pts',(-51.9508885549727,-14.8272329894413,
18.));
#60203=CARTESIAN_POINT('Ctrl Pts',(-51.9749870630737,-14.8748868070404,
18.));
#60204=CARTESIAN_POINT('Ctrl Pts',(-51.9901200745311,-14.9048117204289,
18.));
#60205=CARTESIAN_POINT('Ctrl Pts',(-52.0063718314004,-14.9341413324336,
18.));
#60206=CARTESIAN_POINT('Ctrl Pts',(-52.0237395592016,-14.9627903221168,
18.));
#60207=CARTESIAN_POINT('Ctrl Pts',(-52.0300897392816,-14.9732652815175,
18.));
#60208=CARTESIAN_POINT('Ctrl Pts',(-52.0365905346379,-14.9836512987282,
18.));
#60209=CARTESIAN_POINT('Ctrl Pts',(-52.043237428479,-14.9939369612944,18.));
#60210=CARTESIAN_POINT('Ctrl Pts',(-52.0711394051858,-15.0371135674196,
18.));
#60211=CARTESIAN_POINT('Ctrl Pts',(-52.1015680157931,-15.0784574571633,
18.));
#60212=CARTESIAN_POINT('Ctrl Pts',(-52.1344986678528,-15.1176697568703,
18.));
#60213=CARTESIAN_POINT('Ctrl Pts',(-52.1528947874586,-15.1395750065485,
18.));
#60214=CARTESIAN_POINT('Ctrl Pts',(-52.1720723161447,-15.1608144005325,
18.));
#60215=CARTESIAN_POINT('Ctrl Pts',(-52.1920310817112,-15.1813299718051,
18.));
#60216=CARTESIAN_POINT('Ctrl Pts',(-52.2060486090393,-15.1957385573463,
18.));
#60217=CARTESIAN_POINT('Ctrl Pts',(-52.2204515743704,-15.2097900005096,
18.));
#60218=CARTESIAN_POINT('Ctrl Pts',(-52.2352228301845,-15.2234768233201,
18.));
#60219=CARTESIAN_POINT('Ctrl Pts',(-54.153252109211,-15.2223467977324,18.));
#60220=CARTESIAN_POINT('Ctrl Pts',(-54.1901305933404,-15.1879071947038,
18.));
#60221=CARTESIAN_POINT('Ctrl Pts',(-54.2246310285466,-15.1512289528613,
18.));
#60222=CARTESIAN_POINT('Ctrl Pts',(-54.2567513295153,-15.1126319834757,
18.));
#60223=CARTESIAN_POINT('Ctrl Pts',(-54.290311463843,-15.0723048558288,18.));
#60224=CARTESIAN_POINT('Ctrl Pts',(-54.3212739167588,-15.0298826695219,
18.));
#60225=CARTESIAN_POINT('Ctrl Pts',(-54.3496082931449,-14.9856806062948,
18.));
#60226=CARTESIAN_POINT('Ctrl Pts',(-54.3723325448346,-14.9502304239335,
18.));
#60227=CARTESIAN_POINT('Ctrl Pts',(-54.393365943357,-14.9136342530605,18.));
#60228=CARTESIAN_POINT('Ctrl Pts',(-54.412676568361,-14.8760367445278,18.));
#60229=CARTESIAN_POINT('Ctrl Pts',(-54.4208393026161,-14.8601440185936,
18.));
#60230=CARTESIAN_POINT('Ctrl Pts',(-54.4286940175272,-14.8440722071043,
18.));
#60231=CARTESIAN_POINT('Ctrl Pts',(-54.4362374127529,-14.8278315944995,
18.));
#60232=CARTESIAN_POINT('Ctrl Pts',(-54.4405190389689,-14.8186134333647,
18.));
#60233=CARTESIAN_POINT('Ctrl Pts',(-54.4447005519202,-14.8093401785766,
18.));
#60234=CARTESIAN_POINT('Ctrl Pts',(-54.4487750435594,-14.8000286716647,
18.));
#60235=CARTESIAN_POINT('Ctrl Pts',(-54.4705983254274,-14.7501555444271,
18.));
#60236=CARTESIAN_POINT('Ctrl Pts',(-54.4894011486202,-14.6990895949508,
18.));
#60237=CARTESIAN_POINT('Ctrl Pts',(-54.5051559559858,-14.647162338739,18.));
#60238=CARTESIAN_POINT('Ctrl Pts',(-54.521199476169,-14.5942834958713,18.));
#60239=CARTESIAN_POINT('Ctrl Pts',(-54.5340828409945,-14.5405105650536,
18.));
#60240=CARTESIAN_POINT('Ctrl Pts',(-54.5437362577297,-14.4861590282174,
18.));
#60241=CARTESIAN_POINT('Ctrl Pts',(-54.5506403107422,-14.4472872067766,
18.));
#60242=CARTESIAN_POINT('Ctrl Pts',(-54.5558914111254,-14.4081186550425,
18.));
#60243=CARTESIAN_POINT('Ctrl Pts',(-54.5594490237053,-14.3687624021353,
18.));
#60244=CARTESIAN_POINT('Ctrl Pts',(-54.560961473737,-14.3520308540468,18.));
#60245=CARTESIAN_POINT('Ctrl Pts',(-54.5621676846368,-14.3352653382578,
18.));
#60246=CARTESIAN_POINT('Ctrl Pts',(-54.5630637816013,-14.3184741004373,
18.));
#60247=CARTESIAN_POINT('Ctrl Pts',(-54.5635976657032,-14.3084700771252,
18.));
#60248=CARTESIAN_POINT('Ctrl Pts',(-54.5640211036094,-14.2984625720042,
18.));
#60249=CARTESIAN_POINT('Ctrl Pts',(-54.5643335016824,-14.2884609517312,
18.));
#60250=CARTESIAN_POINT('Ctrl Pts',(-54.5661075110375,-14.2316649294083,
18.));
#60251=CARTESIAN_POINT('Ctrl Pts',(-54.5643085969144,-14.1749865267171,
18.));
#60252=CARTESIAN_POINT('Ctrl Pts',(-54.5588768122501,-14.1187579548114,
18.));
#60253=CARTESIAN_POINT('Ctrl Pts',(-54.5555413233245,-14.0842297489857,
18.));
#60254=CARTESIAN_POINT('Ctrl Pts',(-54.5508350741402,-14.0498706203676,
18.));
#60255=CARTESIAN_POINT('Ctrl Pts',(-54.5447349150618,-14.0157544413133,
18.));
#60256=CARTESIAN_POINT('Ctrl Pts',(-54.5350624849658,-13.9616597279133,
18.));
#60257=CARTESIAN_POINT('Ctrl Pts',(-54.5218884030874,-13.9081753369494,
18.));
#60258=CARTESIAN_POINT('Ctrl Pts',(-54.5054388352989,-13.8555057819088,
18.));
#60259=CARTESIAN_POINT('Ctrl Pts',(-54.5005174069393,-13.8397479550047,
18.));
#60260=CARTESIAN_POINT('Ctrl Pts',(-54.4953024361441,-13.8240630966703,
18.));
#60261=CARTESIAN_POINT('Ctrl Pts',(-54.4897991057295,-13.8084568180249,
18.));
#60262=CARTESIAN_POINT('Ctrl Pts',(-54.4847109304735,-13.7940278314187,
18.));
#60263=CARTESIAN_POINT('Ctrl Pts',(-54.4793736286689,-13.7796597824161,
18.));
#60264=CARTESIAN_POINT('Ctrl Pts',(-54.4738049082137,-13.765391301815,18.));
#60265=CARTESIAN_POINT('Ctrl Pts',(-54.4531741179316,-13.7125299608138,
18.));
#60266=CARTESIAN_POINT('Ctrl Pts',(-54.4293497755017,-13.6609649910114,
18.));
#60267=CARTESIAN_POINT('Ctrl Pts',(-54.4026149607926,-13.6109069383254,
18.));
#60268=CARTESIAN_POINT('Ctrl Pts',(-54.3752481593715,-13.5596655587874,
18.));
#60269=CARTESIAN_POINT('Ctrl Pts',(-54.3448313135357,-13.5100022755867,
18.));
#60270=CARTESIAN_POINT('Ctrl Pts',(-54.3116127229013,-13.462148554514,18.));
#60271=CARTESIAN_POINT('Ctrl Pts',(-54.2914450604172,-13.433095615278,18.));
#60272=CARTESIAN_POINT('Ctrl Pts',(-54.2702436408721,-13.4047098372191,
18.));
#60273=CARTESIAN_POINT('Ctrl Pts',(-54.2480553291971,-13.3770462315216,
18.));
#60274=CARTESIAN_POINT('Ctrl Pts',(-54.235838542242,-13.3618147717258,18.));
#60275=CARTESIAN_POINT('Ctrl Pts',(-54.2233224644036,-13.3468022959013,
18.));
#60276=CARTESIAN_POINT('Ctrl Pts',(-54.2105141669117,-13.3320184620741,
18.));
#60277=CARTESIAN_POINT('Ctrl Pts',(-54.2028017059965,-13.3231164405025,
18.));
#60278=CARTESIAN_POINT('Ctrl Pts',(-54.1949819266755,-13.3142958366318,
18.));
#60279=CARTESIAN_POINT('Ctrl Pts',(-54.1870606016195,-13.3055635742368,
18.));
#60280=CARTESIAN_POINT('Ctrl Pts',(-54.146465975092,-13.2608131154237,18.));
#60281=CARTESIAN_POINT('Ctrl Pts',(-54.1033356929487,-13.2185196121795,
18.));
#60282=CARTESIAN_POINT('Ctrl Pts',(-54.057929911796,-13.1789337623811,18.));
#60283=CARTESIAN_POINT('Ctrl Pts',(-54.0284074581666,-13.1531953787351,
18.));
#60284=CARTESIAN_POINT('Ctrl Pts',(-53.9979219697712,-13.1286019537706,
18.));
#60285=CARTESIAN_POINT('Ctrl Pts',(-53.9665347833756,-13.105228420628,18.));
#60286=CARTESIAN_POINT('Ctrl Pts',(-53.9535624126434,-13.0955681046817,
18.));
#60287=CARTESIAN_POINT('Ctrl Pts',(-53.9404359297659,-13.0861162378026,
18.));
#60288=CARTESIAN_POINT('Ctrl Pts',(-53.9271593223322,-13.076878434333,18.));
#60289=CARTESIAN_POINT('Ctrl Pts',(-53.9174397053675,-13.0701155687616,
18.));
#60290=CARTESIAN_POINT('Ctrl Pts',(-53.9076405169031,-13.0634681523805,
18.));
#60291=CARTESIAN_POINT('Ctrl Pts',(-53.8977718295133,-13.0569437429584,
18.));
#60292=CARTESIAN_POINT('Ctrl Pts',(-53.8470357673936,-13.023401000275,18.));
#60293=CARTESIAN_POINT('Ctrl Pts',(-53.7944075339565,-12.993065740058,18.));
#60294=CARTESIAN_POINT('Ctrl Pts',(-53.7401232238152,-12.9662046864427,
18.));
#60295=CARTESIAN_POINT('Ctrl Pts',(-53.7146984024022,-12.953623933563,18.));
#60296=CARTESIAN_POINT('Ctrl Pts',(-53.6889097287962,-12.9418057638961,
18.));
#60297=CARTESIAN_POINT('Ctrl Pts',(-53.6627787780123,-12.9307804983812,
18.));
#60298=CARTESIAN_POINT('Ctrl Pts',(-53.6403263881356,-12.9213073046241,
18.));
#60299=CARTESIAN_POINT('Ctrl Pts',(-53.6176212739247,-12.9124195098708,
18.));
#60300=CARTESIAN_POINT('Ctrl Pts',(-53.5946845822246,-12.9041113672218,
18.));
#60301=CARTESIAN_POINT('Ctrl Pts',(-15.2209662466057,-52.1764590205667,
18.));
#60302=CARTESIAN_POINT('Ctrl Pts',(-15.1740718831799,-52.1372104252047,
18.));
#60303=CARTESIAN_POINT('Ctrl Pts',(-15.1248302485577,-52.1011214310192,
18.));
#60304=CARTESIAN_POINT('Ctrl Pts',(-15.0736000909597,-52.0682135291378,
18.));
#60305=CARTESIAN_POINT('Ctrl Pts',(-15.0226682165858,-52.0354972307089,
18.));
#60306=CARTESIAN_POINT('Ctrl Pts',(-14.969769673043,-52.005925006896,18.));
#60307=CARTESIAN_POINT('Ctrl Pts',(-14.915234207728,-51.9795679908668,18.));
#60308=CARTESIAN_POINT('Ctrl Pts',(-14.8740531445008,-51.9596651636459,
18.));
#60309=CARTESIAN_POINT('Ctrl Pts',(-14.8319381110892,-51.941596692591,18.));
#60310=CARTESIAN_POINT('Ctrl Pts',(-14.7890287317843,-51.925412757104,18.));
#60311=CARTESIAN_POINT('Ctrl Pts',(-14.766753270954,-51.9170112228273,18.));
#60312=CARTESIAN_POINT('Ctrl Pts',(-14.7442637387328,-51.909117839332,18.));
#60313=CARTESIAN_POINT('Ctrl Pts',(-14.721579884675,-51.9017414674402,18.));
#60314=CARTESIAN_POINT('Ctrl Pts',(-14.7096336326171,-51.8978567661162,
18.));
#60315=CARTESIAN_POINT('Ctrl Pts',(-14.6976315192865,-51.8941150313098,
18.));
#60316=CARTESIAN_POINT('Ctrl Pts',(-14.6855981509523,-51.8905237529537,
18.));
#60317=CARTESIAN_POINT('Ctrl Pts',(-14.628866805663,-51.873592662108,18.));
#60318=CARTESIAN_POINT('Ctrl Pts',(-14.5713364809672,-51.8599659874384,
18.));
#60319=CARTESIAN_POINT('Ctrl Pts',(-14.5133186620481,-51.8497038434808,
18.));
#60320=CARTESIAN_POINT('Ctrl Pts',(-14.4564856885559,-51.8396512740051,
18.));
#60321=CARTESIAN_POINT('Ctrl Pts',(-14.3991838939743,-51.8328273015837,
18.));
#60322=CARTESIAN_POINT('Ctrl Pts',(-14.3417076889107,-51.8293372126133,
18.));
#60323=CARTESIAN_POINT('Ctrl Pts',(-14.3001007307031,-51.826810741254,18.));
#60324=CARTESIAN_POINT('Ctrl Pts',(-14.2584023661364,-51.8260323215432,
18.));
#60325=CARTESIAN_POINT('Ctrl Pts',(-14.2167293111391,-51.8270580660934,
18.));
#60326=CARTESIAN_POINT('Ctrl Pts',(-14.1949488648028,-51.8275941720769,
18.));
#60327=CARTESIAN_POINT('Ctrl Pts',(-14.1731754256056,-51.8286233369704,
18.));
#60328=CARTESIAN_POINT('Ctrl Pts',(-14.1514264245875,-51.8301550767569,
18.));
#60329=CARTESIAN_POINT('Ctrl Pts',(-14.1413116392116,-51.8308674413928,
18.));
#60330=CARTESIAN_POINT('Ctrl Pts',(-14.1312071832823,-51.8316882253572,
18.));
#60331=CARTESIAN_POINT('Ctrl Pts',(-14.1211226983139,-51.8326172394617,
18.));
#60332=CARTESIAN_POINT('Ctrl Pts',(-14.065585908369,-51.8377334611959,18.));
#60333=CARTESIAN_POINT('Ctrl Pts',(-14.0105794928347,-51.8461333286692,
18.));
#60334=CARTESIAN_POINT('Ctrl Pts',(-13.9563747310311,-51.8579061060262,
18.));
#60335=CARTESIAN_POINT('Ctrl Pts',(-13.9201064161049,-51.8657832515487,
18.));
#60336=CARTESIAN_POINT('Ctrl Pts',(-13.8841971505455,-51.8751714207596,
18.));
#60337=CARTESIAN_POINT('Ctrl Pts',(-13.8487329702921,-51.8861095759353,
18.));
#60338=CARTESIAN_POINT('Ctrl Pts',(-13.7962430344237,-51.902298955179,18.));
#60339=CARTESIAN_POINT('Ctrl Pts',(-13.7447264797303,-51.9218828237725,
18.));
#60340=CARTESIAN_POINT('Ctrl Pts',(-13.6944250448181,-51.9446586129267,
18.));
#60341=CARTESIAN_POINT('Ctrl Pts',(-13.6788893969317,-51.9516929379167,
18.));
#60342=CARTESIAN_POINT('Ctrl Pts',(-13.6634698927199,-51.9590319641548,
18.));
#60343=CARTESIAN_POINT('Ctrl Pts',(-13.6481743336104,-51.9666702755682,
18.));
#60344=CARTESIAN_POINT('Ctrl Pts',(-13.634752007033,-51.9733731302699,18.));
#60345=CARTESIAN_POINT('Ctrl Pts',(-13.6214194410592,-51.9803097396861,
18.));
#60346=CARTESIAN_POINT('Ctrl Pts',(-13.6082135027341,-51.987458987616,18.));
#60347=CARTESIAN_POINT('Ctrl Pts',(-13.559244561094,-52.0139691148055,18.));
#60348=CARTESIAN_POINT('Ctrl Pts',(-13.5119462056266,-52.0434302755632,
18.));
#60349=CARTESIAN_POINT('Ctrl Pts',(-13.4665417533732,-52.075593652502,18.));
#60350=CARTESIAN_POINT('Ctrl Pts',(-13.4211918994788,-52.1077183533306,
18.));
#60351=CARTESIAN_POINT('Ctrl Pts',(-13.3777306362556,-52.1425397400829,
18.));
#60352=CARTESIAN_POINT('Ctrl Pts',(-13.3364183517639,-52.1798448137172,
18.));
#60353=CARTESIAN_POINT('Ctrl Pts',(-13.3100126299148,-52.2036892321527,
18.));
#60354=CARTESIAN_POINT('Ctrl Pts',(-13.284485655771,-52.2285490007927,18.));
#60355=CARTESIAN_POINT('Ctrl Pts',(-13.2599156980719,-52.2543732768717,
18.));
#60356=CARTESIAN_POINT('Ctrl Pts',(-13.247255109996,-52.2676801993254,18.));
#60357=CARTESIAN_POINT('Ctrl Pts',(-13.2348487708744,-52.2812432661245,
18.));
#60358=CARTESIAN_POINT('Ctrl Pts',(-13.222708346973,-52.2950557510881,18.));
#60359=CARTESIAN_POINT('Ctrl Pts',(-13.215385988776,-52.3033865938424,18.));
#60360=CARTESIAN_POINT('Ctrl Pts',(-13.2081608879731,-52.3118077521959,
18.));
#60361=CARTESIAN_POINT('Ctrl Pts',(-13.2010440030959,-52.3203073114272,
18.));
#60362=CARTESIAN_POINT('Ctrl Pts',(-13.1666279154692,-52.3614097853807,
18.));
#60363=CARTESIAN_POINT('Ctrl Pts',(-13.1346840827633,-52.4044056088235,
18.));
#60364=CARTESIAN_POINT('Ctrl Pts',(-13.1054638931954,-52.4491024554207,
18.));
#60365=CARTESIAN_POINT('Ctrl Pts',(-13.0871146481686,-52.4771704933859,
18.));
#60366=CARTESIAN_POINT('Ctrl Pts',(-13.069840321977,-52.5059097415541,18.));
#60367=CARTESIAN_POINT('Ctrl Pts',(-13.0537134178065,-52.5352751363827,
18.));
#60368=CARTESIAN_POINT('Ctrl Pts',(-13.0478169297015,-52.5460120205034,
18.));
#60369=CARTESIAN_POINT('Ctrl Pts',(-13.0420727750593,-52.5568348697255,
18.));
#60370=CARTESIAN_POINT('Ctrl Pts',(-13.0364885788853,-52.5677340663131,
18.));
#60371=CARTESIAN_POINT('Ctrl Pts',(-13.0130475064328,-52.61348619409,18.));
#60372=CARTESIAN_POINT('Ctrl Pts',(-12.9924569304998,-52.6605100892402,
18.));
#60373=CARTESIAN_POINT('Ctrl Pts',(-12.9749633881527,-52.708635016183,18.));
#60374=CARTESIAN_POINT('Ctrl Pts',(-12.9651909077135,-52.7355192170987,
18.));
#60375=CARTESIAN_POINT('Ctrl Pts',(-12.956385785445,-52.7627472106582,18.));
#60376=CARTESIAN_POINT('Ctrl Pts',(-12.948598136759,-52.7902898637941,18.));
#60377=CARTESIAN_POINT('Ctrl Pts',(-12.9431286937976,-52.8096336961118,
18.));
#60378=CARTESIAN_POINT('Ctrl Pts',(-12.9381612650277,-52.82913275561,18.));
#60379=CARTESIAN_POINT('Ctrl Pts',(-12.9336937527446,-52.8487684531621,
18.));
#60380=CARTESIAN_POINT('Ctrl Pts',(-13.8936870225526,-54.5092654229862,
18.));
#60381=CARTESIAN_POINT('Ctrl Pts',(-13.9419518764876,-54.5239833380077,
18.));
#60382=CARTESIAN_POINT('Ctrl Pts',(-13.9909664228071,-54.5355224856705,
18.));
#60383=CARTESIAN_POINT('Ctrl Pts',(-14.0404525674513,-54.5440410140809,
18.));
#60384=CARTESIAN_POINT('Ctrl Pts',(-14.0921569775524,-54.5529413939661,
18.));
#60385=CARTESIAN_POINT('Ctrl Pts',(-14.1443769192189,-54.5585445895538,
18.));
#60386=CARTESIAN_POINT('Ctrl Pts',(-14.1968242396308,-54.5609818668627,
18.));
#60387=CARTESIAN_POINT('Ctrl Pts',(-14.2388871088265,-54.5629365687585,
18.));
#60388=CARTESIAN_POINT('Ctrl Pts',(-14.2810970053295,-54.562853958605,18.));
#60389=CARTESIAN_POINT('Ctrl Pts',(-14.3233126980455,-54.5607787169103,
18.));
#60390=CARTESIAN_POINT('Ctrl Pts',(-14.3411576908261,-54.5599014916257,
18.));
#60391=CARTESIAN_POINT('Ctrl Pts',(-14.3590037664332,-54.5586679663758,
18.));
#60392=CARTESIAN_POINT('Ctrl Pts',(-14.3768403679106,-54.5570804251684,
18.));
#60393=CARTESIAN_POINT('Ctrl Pts',(-14.3869641761715,-54.5561793587399,
18.));
#60394=CARTESIAN_POINT('Ctrl Pts',(-14.3970856400472,-54.5551640486891,
18.));
#60395=CARTESIAN_POINT('Ctrl Pts',(-14.4071867211825,-54.5540369331083,
18.));
#60396=CARTESIAN_POINT('Ctrl Pts',(-14.4612897750273,-54.5479999164622,
18.));
#60397=CARTESIAN_POINT('Ctrl Pts',(-14.5149156125263,-54.5387506932885,
18.));
#60398=CARTESIAN_POINT('Ctrl Pts',(-14.5677633543972,-54.5264311541952,
18.));
#60399=CARTESIAN_POINT('Ctrl Pts',(-14.6215795301098,-54.5138858597877,
18.));
#60400=CARTESIAN_POINT('Ctrl Pts',(-14.6745899303805,-54.4981567455395,
18.));
#60401=CARTESIAN_POINT('Ctrl Pts',(-14.7264864439659,-54.4793411079406,
18.));
#60402=CARTESIAN_POINT('Ctrl Pts',(-14.7636024302384,-54.4658843090425,
18.));
#60403=CARTESIAN_POINT('Ctrl Pts',(-14.800148916719,-54.4508476461167,18.));
#60404=CARTESIAN_POINT('Ctrl Pts',(-14.8360112141955,-54.4342505283907,
18.));
#60405=CARTESIAN_POINT('Ctrl Pts',(-14.8512574582524,-54.427194546892,18.));
#60406=CARTESIAN_POINT('Ctrl Pts',(-14.8663799984467,-54.419856367452,18.));
#60407=CARTESIAN_POINT('Ctrl Pts',(-14.8813697562969,-54.412236757174,18.));
#60408=CARTESIAN_POINT('Ctrl Pts',(-14.8903005158607,-54.4076970636017,
18.));
#60409=CARTESIAN_POINT('Ctrl Pts',(-14.8991790662691,-54.4030599781999,
18.));
#60410=CARTESIAN_POINT('Ctrl Pts',(-14.9079969993907,-54.3983296699509,
18.));
#60411=CARTESIAN_POINT('Ctrl Pts',(-14.9580707730014,-54.3714680028119,
18.));
#60412=CARTESIAN_POINT('Ctrl Pts',(-15.0062562238015,-54.3415708986061,
18.));
#60413=CARTESIAN_POINT('Ctrl Pts',(-15.0522356756777,-54.3087525447577,
18.));
#60414=CARTESIAN_POINT('Ctrl Pts',(-15.0804700425257,-54.2885999460621,
18.));
#60415=CARTESIAN_POINT('Ctrl Pts',(-15.1078726148715,-54.2673447838554,
18.));
#60416=CARTESIAN_POINT('Ctrl Pts',(-15.1343678441299,-54.245003945279,18.));
#60417=CARTESIAN_POINT('Ctrl Pts',(-15.1763790053575,-54.2095800369881,
18.));
#60418=CARTESIAN_POINT('Ctrl Pts',(-15.2161107900716,-54.1714287640079,
18.));
#60419=CARTESIAN_POINT('Ctrl Pts',(-15.2534991669623,-54.1308482498307,
18.));
#60420=CARTESIAN_POINT('Ctrl Pts',(-15.2646851435512,-54.1187072391932,
18.));
#60421=CARTESIAN_POINT('Ctrl Pts',(-15.2756611560252,-54.1063484965531,
18.));
#60422=CARTESIAN_POINT('Ctrl Pts',(-15.286424936402,-54.0937793159871,18.));
#60423=CARTESIAN_POINT('Ctrl Pts',(-15.2963767216443,-54.0821583258439,
18.));
#60424=CARTESIAN_POINT('Ctrl Pts',(-15.3061511701195,-54.0703520539612,
18.));
#60425=CARTESIAN_POINT('Ctrl Pts',(-15.3157236804964,-54.0583951512989,
18.));
#60426=CARTESIAN_POINT('Ctrl Pts',(-15.3511875377467,-54.0140976919625,
18.));
#60427=CARTESIAN_POINT('Ctrl Pts',(-15.3839319324792,-53.9676827165237,
18.));
#60428=CARTESIAN_POINT('Ctrl Pts',(-15.4139160660758,-53.9195006537336,
18.));
#60429=CARTESIAN_POINT('Ctrl Pts',(-15.4446090041847,-53.8701795997696,
18.));
#60430=CARTESIAN_POINT('Ctrl Pts',(-15.4724102509539,-53.8190061740789,
18.));
#60431=CARTESIAN_POINT('Ctrl Pts',(-15.4972435005011,-53.7663111450288,
18.));
#60432=CARTESIAN_POINT('Ctrl Pts',(-15.5123202613179,-53.7343189424898,
18.));
#60433=CARTESIAN_POINT('Ctrl Pts',(-15.5263023651392,-53.7017650594938,
18.));
#60434=CARTESIAN_POINT('Ctrl Pts',(-15.5391656032369,-53.6687175882849,
18.));
#60435=CARTESIAN_POINT('Ctrl Pts',(-15.5462480435773,-53.6505218010762,
18.));
#60436=CARTESIAN_POINT('Ctrl Pts',(-15.5529911929768,-53.6321763122081,
18.));
#60437=CARTESIAN_POINT('Ctrl Pts',(-15.5593902229399,-53.61369207462,18.));
#60438=CARTESIAN_POINT('Ctrl Pts',(-15.5632433722998,-53.6025618675981,
18.));
#60439=CARTESIAN_POINT('Ctrl Pts',(-15.5669723526336,-53.5913794289415,
18.));
#60440=CARTESIAN_POINT('Ctrl Pts',(-15.5705740541498,-53.5801532197009,
18.));
#60441=CARTESIAN_POINT('Ctrl Pts',(-15.5890317873878,-53.5226219738424,
18.));
#60442=CARTESIAN_POINT('Ctrl Pts',(-15.6040939073662,-53.4641232630576,
18.));
#60443=CARTESIAN_POINT('Ctrl Pts',(-15.6156733811679,-53.4050077404603,
18.));
#60444=CARTESIAN_POINT('Ctrl Pts',(-15.6232022586033,-53.3665713199646,
18.));
#60445=CARTESIAN_POINT('Ctrl Pts',(-15.6292580546374,-53.3278733667065,
18.));
#60446=CARTESIAN_POINT('Ctrl Pts',(-15.6338065434936,-53.2890044670453,
18.));
#60447=CARTESIAN_POINT('Ctrl Pts',(-15.635686432893,-53.2729399597453,18.));
#60448=CARTESIAN_POINT('Ctrl Pts',(-15.63730874602,-53.2568462123695,18.));
#60449=CARTESIAN_POINT('Ctrl Pts',(-15.6386706145308,-53.2407294854068,
18.));
#60450=CARTESIAN_POINT('Ctrl Pts',(-15.6396676228601,-53.2289306143017,
18.));
#60451=CARTESIAN_POINT('Ctrl Pts',(-15.6405248635871,-53.2171205568196,
18.));
#60452=CARTESIAN_POINT('Ctrl Pts',(-15.6412408277572,-53.2053118151348,
18.));
#60453=CARTESIAN_POINT('Ctrl Pts',(-15.6449216835272,-53.1446016891568,
18.));
#60454=CARTESIAN_POINT('Ctrl Pts',(-15.6448786914135,-53.0838566393811,
18.));
#60455=CARTESIAN_POINT('Ctrl Pts',(-15.6409989083968,-53.0234144937966,
18.));
#60456=CARTESIAN_POINT('Ctrl Pts',(-15.6391817516104,-52.9951054737926,
18.));
#60457=CARTESIAN_POINT('Ctrl Pts',(-15.6365222466597,-52.966862641753,18.));
#60458=CARTESIAN_POINT('Ctrl Pts',(-15.6330049221515,-52.9387198431847,
18.));
#60459=CARTESIAN_POINT('Ctrl Pts',(-15.6299827554382,-52.9145388985899,
18.));
#60460=CARTESIAN_POINT('Ctrl Pts',(-15.626327255878,-52.8904317889028,18.));
#60461=CARTESIAN_POINT('Ctrl Pts',(-15.6220539738783,-52.8664139542998,
18.));
#60462=CARTESIAN_POINT('Ctrl Pts',(37.5756558680257,-39.2699729499894,18.));
#60463=CARTESIAN_POINT('Ctrl Pts',(37.5651127690921,-39.2097369422873,18.));
#60464=CARTESIAN_POINT('Ctrl Pts',(37.5584799714474,-39.1490477940628,18.));
#60465=CARTESIAN_POINT('Ctrl Pts',(37.5555966212125,-39.0882269703887,18.));
#60466=CARTESIAN_POINT('Ctrl Pts',(37.5527300631012,-39.0277603564722,18.));
#60467=CARTESIAN_POINT('Ctrl Pts',(37.5535699537459,-38.9671624857774,18.));
#60468=CARTESIAN_POINT('Ctrl Pts',(37.5580129364599,-38.906754525574,18.));
#60469=CARTESIAN_POINT('Ctrl Pts',(37.5613679468783,-38.8611389225248,18.));
#60470=CARTESIAN_POINT('Ctrl Pts',(37.5667786506926,-38.8156316117445,18.));
#60471=CARTESIAN_POINT('Ctrl Pts',(37.5742186551894,-38.7703786151086,18.));
#60472=CARTESIAN_POINT('Ctrl Pts',(37.5780809441845,-38.7468866735407,18.));
#60473=CARTESIAN_POINT('Ctrl Pts',(37.5824903524787,-38.7234634071251,18.));
#60474=CARTESIAN_POINT('Ctrl Pts',(37.5874446737531,-38.7001303514386,18.));
#60475=CARTESIAN_POINT('Ctrl Pts',(37.5900538576758,-38.6878420418208,18.));
#60476=CARTESIAN_POINT('Ctrl Pts',(37.5928147908839,-38.6755768363618,18.));
#60477=CARTESIAN_POINT('Ctrl Pts',(37.5957216552647,-38.6633597908234,18.));
#60478=CARTESIAN_POINT('Ctrl Pts',(37.6094259854351,-38.6057628740656,18.));
#60479=CARTESIAN_POINT('Ctrl Pts',(37.6263915747042,-38.5491262011556,18.));
#60480=CARTESIAN_POINT('Ctrl Pts',(37.6465146580695,-38.4937496146603,18.));
#60481=CARTESIAN_POINT('Ctrl Pts',(37.6662269366953,-38.4395035191427,18.));
#60482=CARTESIAN_POINT('Ctrl Pts',(37.6889696982578,-38.3864657328463,18.));
#60483=CARTESIAN_POINT('Ctrl Pts',(37.7146868376966,-38.3349439029418,18.));
#60484=CARTESIAN_POINT('Ctrl Pts',(37.7333032641295,-38.2976476726051,18.));
#60485=CARTESIAN_POINT('Ctrl Pts',(37.7534791916908,-38.2611463231416,18.));
#60486=CARTESIAN_POINT('Ctrl Pts',(37.7752048261634,-38.2255690008596,18.));
#60487=CARTESIAN_POINT('Ctrl Pts',(37.7865596505613,-38.2069746418515,18.));
#60488=CARTESIAN_POINT('Ctrl Pts',(37.7983379414274,-38.1886328838064,18.));
#60489=CARTESIAN_POINT('Ctrl Pts',(37.8105392196947,-38.1705635815892,18.));
#60490=CARTESIAN_POINT('Ctrl Pts',(37.816213671722,-38.1621600859593,18.));
#60491=CARTESIAN_POINT('Ctrl Pts',(37.821976845552,-38.1538197468311,18.));
#60492=CARTESIAN_POINT('Ctrl Pts',(37.8278237561117,-38.1455508194627,18.));
#60493=CARTESIAN_POINT('Ctrl Pts',(37.8600240522662,-38.1000119135009,18.));
#60494=CARTESIAN_POINT('Ctrl Pts',(37.8948027203639,-38.0565742505908,18.));
#60495=CARTESIAN_POINT('Ctrl Pts',(37.9321013501539,-38.0155174318995,18.));
#60496=CARTESIAN_POINT('Ctrl Pts',(37.9570573616103,-37.9880468668039,18.));
#60497=CARTESIAN_POINT('Ctrl Pts',(37.9831422874183,-37.961642783205,18.));
#60498=CARTESIAN_POINT('Ctrl Pts',(38.0103468288125,-37.9363991775295,18.));
#60499=CARTESIAN_POINT('Ctrl Pts',(38.0506122150019,-37.8990361682947,18.));
#60500=CARTESIAN_POINT('Ctrl Pts',(38.0933303033916,-37.8642134925913,18.));
#60501=CARTESIAN_POINT('Ctrl Pts',(38.1382048591451,-37.8320391955257,18.));
#60502=CARTESIAN_POINT('Ctrl Pts',(38.1520648967439,-37.82210178312,18.));
#60503=CARTESIAN_POINT('Ctrl Pts',(38.1661307314521,-37.8124173314212,18.));
#60504=CARTESIAN_POINT('Ctrl Pts',(38.1803937730732,-37.8029898884108,18.));
#60505=CARTESIAN_POINT('Ctrl Pts',(38.1929089479265,-37.7947177329458,18.));
#60506=CARTESIAN_POINT('Ctrl Pts',(38.2055816457233,-37.7866401763794,18.));
#60507=CARTESIAN_POINT('Ctrl Pts',(38.2183751516466,-37.778778585511,18.));
#60508=CARTESIAN_POINT('Ctrl Pts',(38.2658171634483,-37.7496255379419,18.));
#60509=CARTESIAN_POINT('Ctrl Pts',(38.3149793341298,-37.7233948524332,18.));
#60510=CARTESIAN_POINT('Ctrl Pts',(38.3655345941719,-37.7001554936512,18.));
#60511=CARTESIAN_POINT('Ctrl Pts',(38.4160291498531,-37.6769440395902,18.));
#60512=CARTESIAN_POINT('Ctrl Pts',(38.4679146668078,-37.6567165566401,18.));
#60513=CARTESIAN_POINT('Ctrl Pts',(38.5208765564778,-37.6395920241868,18.));
#60514=CARTESIAN_POINT('Ctrl Pts',(38.5547280084195,-37.6286466011481,18.));
#60515=CARTESIAN_POINT('Ctrl Pts',(38.5890193652508,-37.6189698569069,18.));
#60516=CARTESIAN_POINT('Ctrl Pts',(38.6236674824325,-37.6106041450305,18.));
#60517=CARTESIAN_POINT('Ctrl Pts',(38.641521850732,-37.6062932469766,18.));
#60518=CARTESIAN_POINT('Ctrl Pts',(38.6594709236377,-37.6023306259858,18.));
#60519=CARTESIAN_POINT('Ctrl Pts',(38.6775030446682,-37.5987230218566,18.));
#60520=CARTESIAN_POINT('Ctrl Pts',(38.6883788045946,-37.5965471582212,18.));
#60521=CARTESIAN_POINT('Ctrl Pts',(38.6992841520963,-37.5945006838876,18.));
#60522=CARTESIAN_POINT('Ctrl Pts',(38.7102032897924,-37.5925871316871,18.));
#60523=CARTESIAN_POINT('Ctrl Pts',(38.7630060609621,-37.5833335750623,18.));
#60524=CARTESIAN_POINT('Ctrl Pts',(38.8162124112195,-37.5771677759325,18.));
#60525=CARTESIAN_POINT('Ctrl Pts',(38.8695301448715,-37.5742112603306,18.));
#60526=CARTESIAN_POINT('Ctrl Pts',(38.9030118816576,-37.5723546683413,18.));
#60527=CARTESIAN_POINT('Ctrl Pts',(38.9365374742123,-37.5717646060238,18.));
#60528=CARTESIAN_POINT('Ctrl Pts',(38.9700316589891,-37.5724813268537,18.));
#60529=CARTESIAN_POINT('Ctrl Pts',(38.9822787357142,-37.5727433942858,18.));
#60530=CARTESIAN_POINT('Ctrl Pts',(38.994524100686,-37.5731803873846,18.));
#60531=CARTESIAN_POINT('Ctrl Pts',(39.0067556066892,-37.5737941004195,18.));
#60532=CARTESIAN_POINT('Ctrl Pts',(39.0580981368241,-37.576370200205,18.));
#60533=CARTESIAN_POINT('Ctrl Pts',(39.1091169144504,-37.5820508279399,18.));
#60534=CARTESIAN_POINT('Ctrl Pts',(39.1595408591573,-37.5909641088522,18.));
#60535=CARTESIAN_POINT('Ctrl Pts',(39.1877068769066,-37.5959429265516,18.));
#60536=CARTESIAN_POINT('Ctrl Pts',(39.2156870322805,-37.6019312273908,18.));
#60537=CARTESIAN_POINT('Ctrl Pts',(39.2434310600143,-37.6089578358496,18.));
#60538=CARTESIAN_POINT('Ctrl Pts',(39.2629177980487,-37.6138931566914,18.));
#60539=CARTESIAN_POINT('Ctrl Pts',(39.2822879943277,-37.6193408368567,18.));
#60540=CARTESIAN_POINT('Ctrl Pts',(39.3015265966439,-37.6252897660473,18.));
#60541=CARTESIAN_POINT('Ctrl Pts',(40.2595650866584,-39.2869186252539,18.));
#60542=CARTESIAN_POINT('Ctrl Pts',(40.248179115755,-39.3360745846542,18.));
#60543=CARTESIAN_POINT('Ctrl Pts',(40.2336652878063,-39.384290400164,18.));
#60544=CARTESIAN_POINT('Ctrl Pts',(40.2162996606332,-39.4314043435453,18.));
#60545=CARTESIAN_POINT('Ctrl Pts',(40.1981554153049,-39.4806307226778,18.));
#60546=CARTESIAN_POINT('Ctrl Pts',(40.1768978215469,-39.5286549715316,18.));
#60547=CARTESIAN_POINT('Ctrl Pts',(40.1527847010649,-39.575293207484,18.));
#60548=CARTESIAN_POINT('Ctrl Pts',(40.1334453389409,-39.6126983095976,18.));
#60549=CARTESIAN_POINT('Ctrl Pts',(40.112267941863,-39.6492120507113,18.));
#60550=CARTESIAN_POINT('Ctrl Pts',(40.0893618631916,-39.6847344690008,18.));
#60551=CARTESIAN_POINT('Ctrl Pts',(40.0796819049373,-39.6997460094337,18.));
#60552=CARTESIAN_POINT('Ctrl Pts',(40.0696929904209,-39.7145804305253,18.));
#60553=CARTESIAN_POINT('Ctrl Pts',(40.0594023733901,-39.7292297389113,18.));
#60554=CARTESIAN_POINT('Ctrl Pts',(40.0535563601261,-39.7375518881931,18.));
#60555=CARTESIAN_POINT('Ctrl Pts',(40.0476124488049,-39.7458148202529,18.));
#60556=CARTESIAN_POINT('Ctrl Pts',(40.0415817908095,-39.7540041063426,18.));
#60557=CARTESIAN_POINT('Ctrl Pts',(40.0093013797404,-39.7978390446753,18.));
#60558=CARTESIAN_POINT('Ctrl Pts',(39.9744777462525,-39.8396546716371,18.));
#60559=CARTESIAN_POINT('Ctrl Pts',(39.9373842780164,-39.8792613959551,18.));
#60560=CARTESIAN_POINT('Ctrl Pts',(39.899610508142,-39.9195945155313,18.));
#60561=CARTESIAN_POINT('Ctrl Pts',(39.8594823790191,-39.9576379444654,18.));
#60562=CARTESIAN_POINT('Ctrl Pts',(39.8172382894759,-39.9931735245461,18.));
#60563=CARTESIAN_POINT('Ctrl Pts',(39.787025005414,-40.0185888332176,18.));
#60564=CARTESIAN_POINT('Ctrl Pts',(39.7557282762828,-40.042720988782,18.));
#60565=CARTESIAN_POINT('Ctrl Pts',(39.7234222903352,-40.0654803761728,18.));
#60566=CARTESIAN_POINT('Ctrl Pts',(39.7096908089594,-40.0751541284175,18.));
#60567=CARTESIAN_POINT('Ctrl Pts',(39.6957768724846,-40.0845797514274,18.));
#60568=CARTESIAN_POINT('Ctrl Pts',(39.681685683933,-40.0937497715622,18.));
#60569=CARTESIAN_POINT('Ctrl Pts',(39.6732915905444,-40.0992123345749,18.));
#60570=CARTESIAN_POINT('Ctrl Pts',(39.6648392877063,-40.1045810653156,18.));
#60571=CARTESIAN_POINT('Ctrl Pts',(39.6563366064296,-40.1098507563725,18.));
#60572=CARTESIAN_POINT('Ctrl Pts',(39.6080360373664,-40.139785910773,18.));
#60573=CARTESIAN_POINT('Ctrl Pts',(39.55805101873,-40.1665680776809,18.));
#60574=CARTESIAN_POINT('Ctrl Pts',(39.5066393732359,-40.1899792586896,18.));
#60575=CARTESIAN_POINT('Ctrl Pts',(39.4750618488382,-40.2043586299853,18.));
#60576=CARTESIAN_POINT('Ctrl Pts',(39.4429452141437,-40.2174657992959,18.));
#60577=CARTESIAN_POINT('Ctrl Pts',(39.4103419265004,-40.2292437480239,18.));
#60578=CARTESIAN_POINT('Ctrl Pts',(39.3586573390129,-40.2479148227975,18.));
#60579=CARTESIAN_POINT('Ctrl Pts',(39.3057507659274,-40.263248205514,18.));
#60580=CARTESIAN_POINT('Ctrl Pts',(39.251912353747,-40.2753374915754,18.));
#60581=CARTESIAN_POINT('Ctrl Pts',(39.2358056778267,-40.2789542069429,18.));
#60582=CARTESIAN_POINT('Ctrl Pts',(39.2196154532522,-40.2822802513836,18.));
#60583=CARTESIAN_POINT('Ctrl Pts',(39.2033491283299,-40.2853173071475,18.));
#60584=CARTESIAN_POINT('Ctrl Pts',(39.1883094890343,-40.2881253306825,18.));
#60585=CARTESIAN_POINT('Ctrl Pts',(39.173198080315,-40.2906871462828,18.));
#60586=CARTESIAN_POINT('Ctrl Pts',(39.1580572085924,-40.2929987736063,18.));
#60587=CARTESIAN_POINT('Ctrl Pts',(39.101962329576,-40.3015630397475,18.));
#60588=CARTESIAN_POINT('Ctrl Pts',(39.0453935804695,-40.3067133780792,18.));
#60589=CARTESIAN_POINT('Ctrl Pts',(38.9886747852766,-40.3085896575272,18.));
#60590=CARTESIAN_POINT('Ctrl Pts',(38.9306156896966,-40.3105102746249,18.));
#60591=CARTESIAN_POINT('Ctrl Pts',(38.8723984153708,-40.3090004242113,18.));
#60592=CARTESIAN_POINT('Ctrl Pts',(38.8143475050011,-40.3041593897166,18.));
#60593=CARTESIAN_POINT('Ctrl Pts',(38.7791040438403,-40.3012203348404,18.));
#60594=CARTESIAN_POINT('Ctrl Pts',(38.7439215217865,-40.2970524592101,18.));
#60595=CARTESIAN_POINT('Ctrl Pts',(38.70887099654,-40.2916688390186,18.));
#60596=CARTESIAN_POINT('Ctrl Pts',(38.6895721262573,-40.2887046098952,18.));
#60597=CARTESIAN_POINT('Ctrl Pts',(38.670313264122,-40.2853716920792,18.));
#60598=CARTESIAN_POINT('Ctrl Pts',(38.6511063076007,-40.2816713797387,18.));
#60599=CARTESIAN_POINT('Ctrl Pts',(38.6395410469802,-40.279443276783,18.));
#60600=CARTESIAN_POINT('Ctrl Pts',(38.6279926371529,-40.2770815256674,18.));
#60601=CARTESIAN_POINT('Ctrl Pts',(38.6164699650551,-40.2745876647271,18.));
#60602=CARTESIAN_POINT('Ctrl Pts',(38.5574190798941,-40.2618072354354,18.));
#60603=CARTESIAN_POINT('Ctrl Pts',(38.4992281803999,-40.2456023805064,18.));
#60604=CARTESIAN_POINT('Ctrl Pts',(38.4422443842522,-40.2260730329555,18.));
#60605=CARTESIAN_POINT('Ctrl Pts',(38.4051943364571,-40.2133753309932,18.));
#60606=CARTESIAN_POINT('Ctrl Pts',(38.3686543069706,-40.1992711514246,18.));
#60607=CARTESIAN_POINT('Ctrl Pts',(38.3327198363388,-40.18377614093,18.));
#60608=CARTESIAN_POINT('Ctrl Pts',(38.317865781759,-40.1773710449996,18.));
#60609=CARTESIAN_POINT('Ctrl Pts',(38.3031152166749,-40.1707281878123,18.));
#60610=CARTESIAN_POINT('Ctrl Pts',(38.2884749986667,-40.16384821542,18.));
#60611=CARTESIAN_POINT('Ctrl Pts',(38.2777585351888,-40.1588121583866,18.));
#60612=CARTESIAN_POINT('Ctrl Pts',(38.2671022705206,-40.1536494637514,18.));
#60613=CARTESIAN_POINT('Ctrl Pts',(38.2565177798301,-40.1483650730324,18.));
#60614=CARTESIAN_POINT('Ctrl Pts',(38.2021024004308,-40.1211977643468,18.));
#60615=CARTESIAN_POINT('Ctrl Pts',(38.1495185721966,-40.0907880131231,18.));
#60616=CARTESIAN_POINT('Ctrl Pts',(38.0991152603216,-40.0572068987993,18.));
#60617=CARTESIAN_POINT('Ctrl Pts',(38.0755109334479,-40.0414805592038,18.));
#60618=CARTESIAN_POINT('Ctrl Pts',(38.052384941403,-40.0250579742592,18.));
#60619=CARTESIAN_POINT('Ctrl Pts',(38.0297743098615,-40.0079426645895,18.));
#60620=CARTESIAN_POINT('Ctrl Pts',(38.0103443715311,-39.9932350076725,18.));
#60621=CARTESIAN_POINT('Ctrl Pts',(37.9912950014703,-39.9780157739289,18.));
#60622=CARTESIAN_POINT('Ctrl Pts',(37.9726317990811,-39.9623061512026,18.));
#60623=CARTESIAN_POINT('Origin',(39.0658530619283,-38.8697713466883,6.));
#60624=CARTESIAN_POINT('Ctrl Pts',(40.2595650866584,-39.2869186252538,6.));
#60625=CARTESIAN_POINT('Ctrl Pts',(40.2480819791948,-39.3364939464152,6.));
#60626=CARTESIAN_POINT('Ctrl Pts',(40.2334065100538,-39.3851618422783,6.));
#60627=CARTESIAN_POINT('Ctrl Pts',(40.2158026351627,-39.4327533922897,6.));
#60628=CARTESIAN_POINT('Ctrl Pts',(40.2039391979306,-39.4648258405338,6.));
#60629=CARTESIAN_POINT('Ctrl Pts',(40.1907446643154,-39.4964096047557,6.));
#60630=CARTESIAN_POINT('Ctrl Pts',(40.1762870855587,-39.5274524412394,6.));
#60631=CARTESIAN_POINT('Ctrl Pts',(40.1696136376125,-39.5417814486659,6.));
#60632=CARTESIAN_POINT('Ctrl Pts',(40.1626709449276,-39.5559951858299,6.));
#60633=CARTESIAN_POINT('Ctrl Pts',(40.1554650290736,-39.570088378074,6.));
#60634=CARTESIAN_POINT('Ctrl Pts',(40.1494095391052,-39.5819315894,6.));
#60635=CARTESIAN_POINT('Ctrl Pts',(40.1431714820681,-39.5936830081332,6.));
#60636=CARTESIAN_POINT('Ctrl Pts',(40.1367585398276,-39.605333444489,6.));
#60637=CARTESIAN_POINT('Ctrl Pts',(40.1108375205575,-39.6524243388018,6.));
#60638=CARTESIAN_POINT('Ctrl Pts',(40.0820470672629,-39.6978983470909,6.));
#60639=CARTESIAN_POINT('Ctrl Pts',(40.0506487799103,-39.7415597566453,6.));
#60640=CARTESIAN_POINT('Ctrl Pts',(40.0386313329833,-39.7582708169074,6.));
#60641=CARTESIAN_POINT('Ctrl Pts',(40.0262313128012,-39.7747162396004,6.));
#60642=CARTESIAN_POINT('Ctrl Pts',(40.0134614554023,-39.7908844940545,6.));
#60643=CARTESIAN_POINT('Ctrl Pts',(40.0042845094336,-39.8025036682472,6.));
#60644=CARTESIAN_POINT('Ctrl Pts',(39.9949165410699,-39.8139796930435,6.));
#60645=CARTESIAN_POINT('Ctrl Pts',(39.9853619687249,-39.8253081417496,6.));
#60646=CARTESIAN_POINT('Ctrl Pts',(39.9779669485161,-39.8340761016426,6.));
#60647=CARTESIAN_POINT('Ctrl Pts',(39.9704598011529,-39.8427558568352,6.));
#60648=CARTESIAN_POINT('Ctrl Pts',(39.9628530938026,-39.8513338610346,6.));
#60649=CARTESIAN_POINT('Ctrl Pts',(39.9252574597059,-39.8937300637949,6.));
#60650=CARTESIAN_POINT('Ctrl Pts',(39.8851758120027,-39.9337126571768,6.));
#60651=CARTESIAN_POINT('Ctrl Pts',(39.8429000971153,-39.9710687869798,6.));
#60652=CARTESIAN_POINT('Ctrl Pts',(39.8012367830184,-40.0078837804949,6.));
#60653=CARTESIAN_POINT('Ctrl Pts',(39.7574416833394,-40.0421487782558,6.));
#60654=CARTESIAN_POINT('Ctrl Pts',(39.7117463596985,-40.0736370674475,6.));
#60655=CARTESIAN_POINT('Ctrl Pts',(39.6878846430625,-40.0900799892649,6.));
#60656=CARTESIAN_POINT('Ctrl Pts',(39.6635040440747,-40.1057652810295,6.));
#60657=CARTESIAN_POINT('Ctrl Pts',(39.6386333596699,-40.1206568258712,6.));
#60658=CARTESIAN_POINT('Ctrl Pts',(39.6252910649894,-40.1286456442042,6.));
#60659=CARTESIAN_POINT('Ctrl Pts',(39.6118076808574,-40.1364059738163,6.));
#60660=CARTESIAN_POINT('Ctrl Pts',(39.5981873691663,-40.143931847729,6.));
#60661=CARTESIAN_POINT('Ctrl Pts',(39.5885046151473,-40.1492820326239,6.));
#60662=CARTESIAN_POINT('Ctrl Pts',(39.578752655703,-40.1545137209881,6.));
#60663=CARTESIAN_POINT('Ctrl Pts',(39.5689329318771,-40.1596246754951,6.));
#60664=CARTESIAN_POINT('Ctrl Pts',(39.5602883880088,-40.1641239741748,6.));
#60665=CARTESIAN_POINT('Ctrl Pts',(39.5516000265252,-40.1685251724648,6.));
#60666=CARTESIAN_POINT('Ctrl Pts',(39.5428697391371,-40.1728269741578,6.));
#60667=CARTESIAN_POINT('Ctrl Pts',(39.4996812011881,-40.1941078916592,6.));
#60668=CARTESIAN_POINT('Ctrl Pts',(39.4554640760098,-40.2129597963733,6.));
#60669=CARTESIAN_POINT('Ctrl Pts',(39.4103710639643,-40.2292497271408,6.));
#60670=CARTESIAN_POINT('Ctrl Pts',(39.3590466351121,-40.2477907683078,6.));
#60671=CARTESIAN_POINT('Ctrl Pts',(39.3065877413209,-40.2630147095086,6.));
#60672=CARTESIAN_POINT('Ctrl Pts',(39.2532910929843,-40.2750393024531,6.));
#60673=CARTESIAN_POINT('Ctrl Pts',(39.2011942210274,-40.2867932062822,6.));
#60674=CARTESIAN_POINT('Ctrl Pts',(39.1482960037837,-40.2954900228406,6.));
#60675=CARTESIAN_POINT('Ctrl Pts',(39.0948540754971,-40.3011985092878,6.));
#60676=CARTESIAN_POINT('Ctrl Pts',(39.0817639227308,-40.3025967552354,6.));
#60677=CARTESIAN_POINT('Ctrl Pts',(39.068641090622,-40.3038155206653,6.));
#60678=CARTESIAN_POINT('Ctrl Pts',(39.0554892737728,-40.3048554432515,6.));
#60679=CARTESIAN_POINT('Ctrl Pts',(39.0455592029516,-40.3056406203147,6.));
#60680=CARTESIAN_POINT('Ctrl Pts',(39.0356145767473,-40.3063236056235,6.));
#60681=CARTESIAN_POINT('Ctrl Pts',(39.025668518601,-40.3069043036963,6.));
#60682=CARTESIAN_POINT('Ctrl Pts',(38.9681511418141,-40.3102624410974,6.));
#60683=CARTESIAN_POINT('Ctrl Pts',(38.9104821863231,-40.310212548994,6.));
#60684=CARTESIAN_POINT('Ctrl Pts',(38.8529878287072,-40.3068889012164,6.));
#60685=CARTESIAN_POINT('Ctrl Pts',(38.7942601300285,-40.3034939561593,6.));
#60686=CARTESIAN_POINT('Ctrl Pts',(38.7357135777964,-40.2966834251873,6.));
#60687=CARTESIAN_POINT('Ctrl Pts',(38.6776775931017,-40.286548962706,6.));
#60688=CARTESIAN_POINT('Ctrl Pts',(38.6191308062327,-40.2763253020229,6.));
#60689=CARTESIAN_POINT('Ctrl Pts',(38.5611024280606,-40.2627189747631,6.));
#60690=CARTESIAN_POINT('Ctrl Pts',(38.5039291822238,-40.2457711880671,6.));
#60691=CARTESIAN_POINT('Ctrl Pts',(38.4909781935321,-40.2419321442865,6.));
#60692=CARTESIAN_POINT('Ctrl Pts',(38.4780675596638,-40.2379201261483,6.));
#60693=CARTESIAN_POINT('Ctrl Pts',(38.4652269235143,-40.2337440112463,6.));
#60694=CARTESIAN_POINT('Ctrl Pts',(38.4073726900059,-40.2149282825016,6.));
#60695=CARTESIAN_POINT('Ctrl Pts',(38.350840226895,-40.1927581041523,6.));
#60696=CARTESIAN_POINT('Ctrl Pts',(38.2959735970115,-40.1673423639825,6.));
#60697=CARTESIAN_POINT('Ctrl Pts',(38.2415891997282,-40.1421500072882,6.));
#60698=CARTESIAN_POINT('Ctrl Pts',(38.188840316281,-40.1137687286488,6.));
#60699=CARTESIAN_POINT('Ctrl Pts',(38.1380651653058,-40.0822545047403,6.));
#60700=CARTESIAN_POINT('Ctrl Pts',(38.1008618421232,-40.0591638031984,6.));
#60701=CARTESIAN_POINT('Ctrl Pts',(38.0647181228192,-40.0343901126825,6.));
#60702=CARTESIAN_POINT('Ctrl Pts',(38.0297736279237,-40.0079388493487,6.));
#60703=CARTESIAN_POINT('Ctrl Pts',(38.0103531401622,-39.9932384956196,6.));
#60704=CARTESIAN_POINT('Ctrl Pts',(37.9913031820638,-39.978019748027,6.));
#60705=CARTESIAN_POINT('Ctrl Pts',(37.972630261787,-39.9623020734811,6.));
#60706=CARTESIAN_POINT('Ctrl Pts',(37.5756558680257,-39.2699729499894,6.));
#60707=CARTESIAN_POINT('Ctrl Pts',(37.5651290682188,-39.2098300642739,6.));
#60708=CARTESIAN_POINT('Ctrl Pts',(37.5584870272447,-39.1491583710679,6.));
#60709=CARTESIAN_POINT('Ctrl Pts',(37.5555980370803,-39.0882817362079,6.));
#60710=CARTESIAN_POINT('Ctrl Pts',(37.5529191835608,-39.0318330886643,6.));
#60711=CARTESIAN_POINT('Ctrl Pts',(37.5534681438704,-38.9752074993234,6.));
#60712=CARTESIAN_POINT('Ctrl Pts',(37.5571795337599,-38.9186719371964,6.));
#60713=CARTESIAN_POINT('Ctrl Pts',(37.5580753630152,-38.9050257798197,6.));
#60714=CARTESIAN_POINT('Ctrl Pts',(37.5591557658531,-38.8913844979576,6.));
#60715=CARTESIAN_POINT('Ctrl Pts',(37.5604183353149,-38.8777672141046,6.));
#60716=CARTESIAN_POINT('Ctrl Pts',(37.5659749115671,-38.8178374610373,6.));
#60717=CARTESIAN_POINT('Ctrl Pts',(37.5750599728567,-38.7582987523151,6.));
#60718=CARTESIAN_POINT('Ctrl Pts',(37.5875760422342,-38.6994723222252,6.));
#60719=CARTESIAN_POINT('Ctrl Pts',(37.5953014146649,-38.6631625138097,6.));
#60720=CARTESIAN_POINT('Ctrl Pts',(37.6043349305656,-38.6271243505865,6.));
#60721=CARTESIAN_POINT('Ctrl Pts',(37.6146623853249,-38.5914381458253,6.));
#60722=CARTESIAN_POINT('Ctrl Pts',(37.618196224716,-38.5792270716504,6.));
#60723=CARTESIAN_POINT('Ctrl Pts',(37.6218816204035,-38.5670572471734,6.));
#60724=CARTESIAN_POINT('Ctrl Pts',(37.6257181655967,-38.554932025581,6.));
#60725=CARTESIAN_POINT('Ctrl Pts',(37.6293072146005,-38.5435890041159,6.));
#60726=CARTESIAN_POINT('Ctrl Pts',(37.6330262982645,-38.5322922610371,6.));
#60727=CARTESIAN_POINT('Ctrl Pts',(37.6368725792164,-38.5210500434224,6.));
#60728=CARTESIAN_POINT('Ctrl Pts',(37.6559105737014,-38.4654042703705,6.));
#60729=CARTESIAN_POINT('Ctrl Pts',(37.6780754632223,-38.4110469589617,6.));
#60730=CARTESIAN_POINT('Ctrl Pts',(37.7032762357148,-38.3582791322986,6.));
#60731=CARTESIAN_POINT('Ctrl Pts',(37.7278335946554,-38.3068585474627,6.));
#60732=CARTESIAN_POINT('Ctrl Pts',(37.755274401204,-38.2569465430554,6.));
#60733=CARTESIAN_POINT('Ctrl Pts',(37.7855529342812,-38.2088521686951,6.));
#60734=CARTESIAN_POINT('Ctrl Pts',(37.8019690565572,-38.182776825868,6.));
#60735=CARTESIAN_POINT('Ctrl Pts',(37.8192199432064,-38.1572363736107,6.));
#60736=CARTESIAN_POINT('Ctrl Pts',(37.8373023126868,-38.1322851555329,6.));
#60737=CARTESIAN_POINT('Ctrl Pts',(37.8523464601752,-38.1115262718488,6.));
#60738=CARTESIAN_POINT('Ctrl Pts',(37.8679662045799,-38.0911753045124,6.));
#60739=CARTESIAN_POINT('Ctrl Pts',(37.8841609617823,-38.0712658190579,6.));
#60740=CARTESIAN_POINT('Ctrl Pts',(37.8910830994432,-38.0627558922124,6.));
#60741=CARTESIAN_POINT('Ctrl Pts',(37.8981112327975,-38.0543257382742,6.));
#60742=CARTESIAN_POINT('Ctrl Pts',(37.9052335275508,-38.045991446363,6.));
#60743=CARTESIAN_POINT('Ctrl Pts',(37.9382051680335,-38.0074090391343,6.));
#60744=CARTESIAN_POINT('Ctrl Pts',(37.9732473043207,-37.9708103555609,6.));
#60745=CARTESIAN_POINT('Ctrl Pts',(38.0103191942679,-37.9364107324676,6.));
#60746=CARTESIAN_POINT('Ctrl Pts',(38.051746090584,-37.8979700265518,6.));
#60747=CARTESIAN_POINT('Ctrl Pts',(38.0957081060154,-37.8622743231266,6.));
#60748=CARTESIAN_POINT('Ctrl Pts',(38.1418690155718,-37.8294138953185,6.));
#60749=CARTESIAN_POINT('Ctrl Pts',(38.1810411655061,-37.8015285347964,6.));
#60750=CARTESIAN_POINT('Ctrl Pts',(38.2217977223915,-37.7756856343115,6.));
#60751=CARTESIAN_POINT('Ctrl Pts',(38.2639408148781,-37.7519688192021,6.));
#60752=CARTESIAN_POINT('Ctrl Pts',(38.2755270772485,-37.7454484329125,6.));
#60753=CARTESIAN_POINT('Ctrl Pts',(38.2872181519006,-37.739088903714,6.));
#60754=CARTESIAN_POINT('Ctrl Pts',(38.2990099288398,-37.7328923323595,6.));
#60755=CARTESIAN_POINT('Ctrl Pts',(38.3081902154278,-37.7280680975397,6.));
#60756=CARTESIAN_POINT('Ctrl Pts',(38.3174331791898,-37.7233419166124,6.));
#60757=CARTESIAN_POINT('Ctrl Pts',(38.326721624664,-37.7187221448981,6.));
#60758=CARTESIAN_POINT('Ctrl Pts',(38.3764239790722,-37.6940018048084,6.));
#60759=CARTESIAN_POINT('Ctrl Pts',(38.4275178409774,-37.6722751485944,6.));
#60760=CARTESIAN_POINT('Ctrl Pts',(38.4796831985246,-37.6536175540612,6.));
#60761=CARTESIAN_POINT('Ctrl Pts',(38.5315566487786,-37.6350643638333,6.));
#60762=CARTESIAN_POINT('Ctrl Pts',(38.5844908269661,-37.6195458589746,6.));
#60763=CARTESIAN_POINT('Ctrl Pts',(38.638177242684,-37.6071867479532,6.));
#60764=CARTESIAN_POINT('Ctrl Pts',(38.687988216704,-37.5957197995686,6.));
#60765=CARTESIAN_POINT('Ctrl Pts',(38.7384475153595,-37.5869729725659,6.));
#60766=CARTESIAN_POINT('Ctrl Pts',(38.7893004136634,-37.5810866485362,6.));
#60767=CARTESIAN_POINT('Ctrl Pts',(38.802362818863,-37.5795746491778,6.));
#60768=CARTESIAN_POINT('Ctrl Pts',(38.8154556556125,-37.5782513512197,6.));
#60769=CARTESIAN_POINT('Ctrl Pts',(38.8285456601,-37.5771216020813,6.));
#60770=CARTESIAN_POINT('Ctrl Pts',(38.8814582148971,-37.572554918147,6.));
#60771=CARTESIAN_POINT('Ctrl Pts',(38.9344079183622,-37.5711349247241,6.));
#60772=CARTESIAN_POINT('Ctrl Pts',(38.9871128327977,-37.5729646742369,6.));
#60773=CARTESIAN_POINT('Ctrl Pts',(39.0380304487623,-37.5747323743462,6.));
#60774=CARTESIAN_POINT('Ctrl Pts',(39.0887204479042,-37.5795333200091,6.));
#60775=CARTESIAN_POINT('Ctrl Pts',(39.1389156304819,-37.5875063462533,6.));
#60776=CARTESIAN_POINT('Ctrl Pts',(39.174030172766,-37.5930839565499,6.));
#60777=CARTESIAN_POINT('Ctrl Pts',(39.2089023015724,-37.6002148717552,6.));
#60778=CARTESIAN_POINT('Ctrl Pts',(39.2434333426904,-37.6089601149436,6.));
#60779=CARTESIAN_POINT('Ctrl Pts',(39.2629126135314,-37.6138933852743,6.));
#60780=CARTESIAN_POINT('Ctrl Pts',(39.2822832137846,-37.6193406085393,6.));
#60781=CARTESIAN_POINT('Ctrl Pts',(39.3015295597332,-37.6252918061955,6.));
#60782=CARTESIAN_POINT('Origin',(39.0658530619283,-38.8697713466883,0.895788276411275));
#60783=CARTESIAN_POINT('Ctrl Pts',(39.8389509032089,-40.2073157943284,2.14578827641127));
#60784=CARTESIAN_POINT('Ctrl Pts',(39.8806063786858,-40.1836140086682,2.14826884812012));
#60785=CARTESIAN_POINT('Ctrl Pts',(40.3479144857801,-39.8865682523885,2.17691792328789));
#60786=CARTESIAN_POINT('Ctrl Pts',(40.8820206309179,-38.8100483503822,2.23173550191459));
#60787=CARTESIAN_POINT('Ctrl Pts',(40.0177367088944,-37.3220789090571,2.31024101229137));
#60788=CARTESIAN_POINT('Ctrl Pts',(38.2999828751462,-37.2220283999295,2.38874652266815));
#60789=CARTESIAN_POINT('Ctrl Pts',(37.2689794778045,-38.599756793647,2.46725203304492));
#60790=CARTESIAN_POINT('Ctrl Pts',(37.8495046941263,-40.2196189105814,2.5457575434217));
#60791=CARTESIAN_POINT('Ctrl Pts',(39.1164929505456,-40.5298919958252,2.60526962454382));
#60792=CARTESIAN_POINT('Ctrl Pts',(39.7159505584363,-40.2768331102243,2.63861320220701));
#60793=CARTESIAN_POINT('Ctrl Pts',(39.8359404161091,-40.2062105265248,2.64578827641127));
#60794=CARTESIAN_POINT('Ctrl Pts',(39.835191636477,-40.2053827942122,2.10421172358873));
#60795=CARTESIAN_POINT('Ctrl Pts',(40.1301403364055,-40.0323966656676,2.12181148931034));
#60796=CARTESIAN_POINT('Ctrl Pts',(40.7310614116501,-39.3634532239961,2.16557975849087));
#60797=CARTESIAN_POINT('Ctrl Pts',(40.5621188491035,-37.8394675163551,2.23551653113034));
#60798=CARTESIAN_POINT('Ctrl Pts',(39.0323736383015,-37.0530949705805,2.31402204150712));
#60799=CARTESIAN_POINT('Ctrl Pts',(37.5317729583208,-37.8957949010443,2.3925275518839));
#60800=CARTESIAN_POINT('Ctrl Pts',(37.4074081512686,-39.612062461691,2.47103306226068));
#60801=CARTESIAN_POINT('Ctrl Pts',(38.6322604476798,-40.5562805179572,2.54159445282895));
#60802=CARTESIAN_POINT('Ctrl Pts',(39.5301075010647,-40.379146656691,2.5859873399383));
#60803=CARTESIAN_POINT('Ctrl Pts',(39.8379370462827,-40.2045960389621,2.60421172358873));
#60804=CARTESIAN_POINT('Ctrl Pts',(39.301448933936,-37.6274127691862,2.));
#60805=CARTESIAN_POINT('Ctrl Pts',(38.8929078719872,-37.5499386892516,2.02616850345893));
#60806=CARTESIAN_POINT('Ctrl Pts',(38.0001476420674,-37.8306642325621,2.07850551037678));
#60807=CARTESIAN_POINT('Ctrl Pts',(37.6102551110149,-39.1875822847128,2.15701102075356));
#60808=CARTESIAN_POINT('Ctrl Pts',(38.5285686312713,-40.2582255133881,2.23551653113034));
#60809=CARTESIAN_POINT('Ctrl Pts',(39.927370040977,-40.0842697726412,2.31402204150712));
#60810=CARTESIAN_POINT('Ctrl Pts',(40.5542159206369,-38.8208279060992,2.3925275518839));
#60811=CARTESIAN_POINT('Ctrl Pts',(39.8459288050188,-37.6014258590767,2.47103306226067));
#60812=CARTESIAN_POINT('Ctrl Pts',(38.4382167358195,-37.5194337211688,2.54953857263746));
#60813=CARTESIAN_POINT('Ctrl Pts',(37.5933017676156,-38.6484924080488,2.62804408301423));
#60814=CARTESIAN_POINT('Ctrl Pts',(38.0690465090536,-39.975981485731,2.70654959339101));
#60815=CARTESIAN_POINT('Ctrl Pts',(39.4387308817871,-40.3114038497388,2.78505510376779));
#60816=CARTESIAN_POINT('Ctrl Pts',(40.4740195694907,-39.3539315296908,2.86356061414458));
#60817=CARTESIAN_POINT('Ctrl Pts',(40.2464260929064,-37.9622550204806,2.94206612452135));
#60818=CARTESIAN_POINT('Ctrl Pts',(38.9600691167361,-37.3844596499183,3.02057163489813));
#60819=CARTESIAN_POINT('Ctrl Pts',(37.768580477053,-38.1387276546802,3.09907714527491));
#60820=CARTESIAN_POINT('Ctrl Pts',(37.7405173375704,-39.5486127570041,3.17758265565169));
#60821=CARTESIAN_POINT('Ctrl Pts',(38.9010464836381,-40.3496968754357,3.25608816602847));
#60822=CARTESIAN_POINT('Ctrl Pts',(40.2093782359874,-39.823548531307,3.33459367640525));
#60823=CARTESIAN_POINT('Ctrl Pts',(40.4921693526885,-38.4420301655716,3.41309918678203));
#60824=CARTESIAN_POINT('Ctrl Pts',(39.4958061477021,-37.4441202440019,3.49160469715881));
#60825=CARTESIAN_POINT('Ctrl Pts',(38.1138507756971,-37.7247681321827,3.57011020753558));
#60826=CARTESIAN_POINT('Ctrl Pts',(37.5856736955423,-39.032282120084,3.64861571791237));
#60827=CARTESIAN_POINT('Ctrl Pts',(38.3849566559494,-40.1940525848875,3.72712122828914));
#60828=CARTESIAN_POINT('Ctrl Pts',(39.7948837028381,-40.1681761513166,3.80562673866593));
#60829=CARTESIAN_POINT('Ctrl Pts',(40.5509987381473,-38.9778594216365,3.8841322490427));
#60830=CARTESIAN_POINT('Ctrl Pts',(39.975199824256,-37.690606736441,3.96263775941949));
#60831=CARTESIAN_POINT('Ctrl Pts',(38.5838771151456,-37.4608569069011,4.04114326979626));
#60832=CARTESIAN_POINT('Ctrl Pts',(37.6248018935901,-38.4946550418589,4.11964878017305));
#60833=CARTESIAN_POINT('Ctrl Pts',(37.9580956187159,-39.8648663970343,4.19815429054983));
#60834=CARTESIAN_POINT('Ctrl Pts',(39.2848525544708,-40.3426528537363,4.2766598009266));
#60835=CARTESIAN_POINT('Ctrl Pts',(40.4152055386855,-39.4995241597319,4.35516531130339));
#60836=CARTESIAN_POINT('Ctrl Pts',(40.3354271431306,-38.09161817034,4.43367082168016));
#60837=CARTESIAN_POINT('Ctrl Pts',(39.1170645283528,-37.3815784513111,4.51217633205694));
#60838=CARTESIAN_POINT('Ctrl Pts',(37.8527742546189,-38.0061854960201,4.59068184243372));
#60839=CARTESIAN_POINT('Ctrl Pts',(37.6764018913215,-39.4052768714559,4.6691873528105));
#60840=CARTESIAN_POINT('Ctrl Pts',(38.7461223767003,-40.3241141426736,4.74769286318728));
#60841=CARTESIAN_POINT('Ctrl Pts',(40.1025849285146,-39.9386622571232,4.82619837356406));
#60842=CARTESIAN_POINT('Ctrl Pts',(40.5292817221821,-38.5946035156582,4.90470388394085));
#60843=CARTESIAN_POINT('Ctrl Pts',(39.6435408484722,-37.4973219800824,4.98320939431762));
#60844=CARTESIAN_POINT('Ctrl Pts',(38.2397159426158,-37.6308853554897,5.0617149046944));
#60845=CARTESIAN_POINT('Ctrl Pts',(37.5767902267089,-38.8755117639716,5.14022041507118));
#60846=CARTESIAN_POINT('Ctrl Pts',(38.2492919033735,-40.1149887727412,5.21872592544795));
#60847=CARTESIAN_POINT('Ctrl Pts',(39.6541041493255,-40.2377277253793,5.29723143582474));
#60848=CARTESIAN_POINT('Ctrl Pts',(40.5313606306742,-39.1336457644378,5.37573694620152));
#60849=CARTESIAN_POINT('Ctrl Pts',(40.0943114632432,-37.7929252609641,5.4542424565783));
#60850=CARTESIAN_POINT('Ctrl Pts',(38.7349236527553,-37.4179251395397,5.53274796695507));
#60851=CARTESIAN_POINT('Ctrl Pts',(37.6723064797637,-38.3450171336683,5.61125347733186));
#60852=CARTESIAN_POINT('Ctrl Pts',(37.8594847038433,-39.742636643005,5.68975898770863));
#60853=CARTESIAN_POINT('Ctrl Pts',(39.1285028721539,-40.3576202841946,5.76826449808542));
#60854=CARTESIAN_POINT('Ctrl Pts',(40.3414559726878,-39.6379218175554,5.84677000846219));
#60855=CARTESIAN_POINT('Ctrl Pts',(40.4101742470825,-38.2300213301991,5.92527551883897));
#60856=CARTESIAN_POINT('Ctrl Pts',(39.2737694148595,-37.394461217524,6.00378102921576));
#60857=CARTESIAN_POINT('Ctrl Pts',(37.9498583767322,-37.8848716060229,6.08228653959253));
#60858=CARTESIAN_POINT('Ctrl Pts',(37.7367752723626,-38.7961472226316,6.13462354651038));
#60859=CARTESIAN_POINT('Ctrl Pts',(37.8446253550651,-39.1977395433016,6.16079204996931));
#60860=CARTESIAN_POINT('Ctrl Pts',(39.3187452171453,-37.5362049495383,1.94640265001023));
#60861=CARTESIAN_POINT('Ctrl Pts',(38.8802110918636,-37.4530431059918,1.97257115346916));
#60862=CARTESIAN_POINT('Ctrl Pts',(37.9219088231848,-37.7543781296798,2.02490816038701));
#60863=CARTESIAN_POINT('Ctrl Pts',(37.5033923116662,-39.210914391274,2.10341367076379));
#60864=CARTESIAN_POINT('Ctrl Pts',(38.4891238668221,-40.360158948323,2.18191918114057));
#60865=CARTESIAN_POINT('Ctrl Pts',(39.9906183548468,-40.1734322378127,2.26042469151735));
#60866=CARTESIAN_POINT('Ctrl Pts',(40.6634841573972,-38.8172347208602,2.33893020189413));
#60867=CARTESIAN_POINT('Ctrl Pts',(39.9031981063107,-37.5083102090702,2.4174357122709));
#60868=CARTESIAN_POINT('Ctrl Pts',(38.3921387822617,-37.4202986140891,2.49594122264769));
#60869=CARTESIAN_POINT('Ctrl Pts',(37.4851943376786,-38.6322472032482,2.57444673302446));
#60870=CARTESIAN_POINT('Ctrl Pts',(37.9958659040779,-40.0571939606811,2.65295224340125));
#60871=CARTESIAN_POINT('Ctrl Pts',(39.4661057263451,-40.4172413750055,2.73145775377802));
#60872=CARTESIAN_POINT('Ctrl Pts',(40.5774001869564,-39.3894761747327,2.8099632641548));
#60873=CARTESIAN_POINT('Ctrl Pts',(40.3330979234395,-37.8956296621443,2.88846877453158));
#60874=CARTESIAN_POINT('Ctrl Pts',(38.9523029828924,-37.2754154143705,2.96697428490836));
#60875=CARTESIAN_POINT('Ctrl Pts',(37.6733411426948,-38.0850580439712,3.04547979528514));
#60876=CARTESIAN_POINT('Ctrl Pts',(37.6432177463661,-39.5984499344848,3.12398530566192));
#60877=CARTESIAN_POINT('Ctrl Pts',(38.8889472001127,-40.4583456851777,3.2024908160387));
#60878=CARTESIAN_POINT('Ctrl Pts',(40.293330196176,-39.893570132972,3.28099632641548));
#60879=CARTESIAN_POINT('Ctrl Pts',(40.5968824374325,-38.4106275244906,3.35950183679226));
#60880=CARTESIAN_POINT('Ctrl Pts',(39.5273711758787,-37.3394559940749,3.43800734716904));
#60881=CARTESIAN_POINT('Ctrl Pts',(38.0439594782896,-37.6407076615778,3.51651285754582));
#60882=CARTESIAN_POINT('Ctrl Pts',(37.4770062502969,-39.0442128569736,3.5950183679226));
#60883=CARTESIAN_POINT('Ctrl Pts',(38.3349686108551,-40.2912747609356,3.67352387829938));
#60884=CARTESIAN_POINT('Ctrl Pts',(39.8484055252959,-40.2634986076469,3.75202938867616));
#60885=CARTESIAN_POINT('Ctrl Pts',(40.6600307852876,-38.9857947132862,3.83053489905294));
#60886=CARTESIAN_POINT('Ctrl Pts',(40.0419595641553,-37.6040383051891,3.90904040942972));
#60887=CARTESIAN_POINT('Ctrl Pts',(38.5484928259196,-37.3574213799522,3.9875459198065));
#60888=CARTESIAN_POINT('Ctrl Pts',(37.5190070470414,-38.4671158588103,4.06605143018328));
#60889=CARTESIAN_POINT('Ctrl Pts',(37.8767695483495,-39.9379213519628,4.14455694056006));
#60890=CARTESIAN_POINT('Ctrl Pts',(39.3009304136176,-40.4507845262585,4.22306245093683));
#60891=CARTESIAN_POINT('Ctrl Pts',(40.5142683210176,-39.5457574952881,4.30156796131362));
#60892=CARTESIAN_POINT('Ctrl Pts',(40.4286329903996,-38.0344900143857,4.38007347169039));
#60893=CARTESIAN_POINT('Ctrl Pts',(39.1208242208265,-37.2723226924175,4.45857898206717));
#60894=CARTESIAN_POINT('Ctrl Pts',(37.7637160108241,-37.9427852958327,4.53708449244395));
#60895=CARTESIAN_POINT('Ctrl Pts',(37.5743952612927,-39.4445910374365,4.61559000282073));
#60896=CARTESIAN_POINT('Ctrl Pts',(38.7226493317982,-40.430884794758,4.69409551319751));
#60897=CARTESIAN_POINT('Ctrl Pts',(40.1786966524752,-40.0171349389622,4.77260102357429));
#60898=CARTESIAN_POINT('Ctrl Pts',(40.6367194134647,-38.5744020550171,4.85110653395107));
#60899=CARTESIAN_POINT('Ctrl Pts',(39.6859518273974,-37.3965635383795,4.92961204432785));
#60900=CARTESIAN_POINT('Ctrl Pts',(38.1790650429905,-37.5399324759461,5.00811755470463));
#60901=CARTESIAN_POINT('Ctrl Pts',(37.4674706011366,-38.8759331970053,5.08662306508141));
#60902=CARTESIAN_POINT('Ctrl Pts',(38.1893440234058,-40.2064064749044,5.16512857545819));
#60903=CARTESIAN_POINT('Ctrl Pts',(39.6972906335328,-40.3381563141405,5.24363408583496));
#60904=CARTESIAN_POINT('Ctrl Pts',(40.638950945132,-39.1530181185549,5.32213959621175));
#60905=CARTESIAN_POINT('Ctrl Pts',(40.1698157903201,-37.7138685495171,5.40064510658852));
#60906=CARTESIAN_POINT('Ctrl Pts',(38.7106284529518,-37.3113377746548,5.47915061696531));
#60907=CARTESIAN_POINT('Ctrl Pts',(37.5699991848822,-38.3064922757992,5.55765612734208));
#60908=CARTESIAN_POINT('Ctrl Pts',(37.7709191080277,-39.8067180941779,5.63616163771886));
#60909=CARTESIAN_POINT('Ctrl Pts',(39.1331023112333,-40.466850791403,5.71466714809565));
#60910=CARTESIAN_POINT('Ctrl Pts',(40.4351044267926,-39.6943156243661,5.79317265847242));
#60911=CARTESIAN_POINT('Ctrl Pts',(40.5088676568797,-38.1830540494315,5.8716781688492));
#60912=CARTESIAN_POINT('Ctrl Pts',(39.2890336047346,-37.2861512475827,5.95018367922599));
#60913=CARTESIAN_POINT('Ctrl Pts',(37.8679275688169,-37.8125651402854,6.02868918960276));
#60914=CARTESIAN_POINT('Ctrl Pts',(37.6392009572462,-38.7907421037309,6.08102619652061));
#60915=CARTESIAN_POINT('Ctrl Pts',(37.7549688593853,-39.2218173455308,6.10719469997954));
#60916=CARTESIAN_POINT('Ctrl Pts',(39.3360415003545,-37.4449971298904,1.89280530002046));
#60917=CARTESIAN_POINT('Ctrl Pts',(38.8675143117401,-37.356147522732,1.91897380347939));
#60918=CARTESIAN_POINT('Ctrl Pts',(37.8436700043021,-37.6780920267975,1.97131081039724));
#60919=CARTESIAN_POINT('Ctrl Pts',(37.3965295123176,-39.2342464978351,2.04981632077402));
#60920=CARTESIAN_POINT('Ctrl Pts',(38.4496791023729,-40.4620923832581,2.1283218311508));
#60921=CARTESIAN_POINT('Ctrl Pts',(40.0538666687167,-40.2625947029841,2.20682734152758));
#60922=CARTESIAN_POINT('Ctrl Pts',(40.7727523941575,-38.8136415356213,2.28533285190436));
#60923=CARTESIAN_POINT('Ctrl Pts',(39.9604674076026,-37.4151945590636,2.36383836228113));
#60924=CARTESIAN_POINT('Ctrl Pts',(38.3460608287039,-37.3211635070092,2.44234387265792));
#60925=CARTESIAN_POINT('Ctrl Pts',(37.3770869077416,-38.6160019984476,2.52084938303469));
#60926=CARTESIAN_POINT('Ctrl Pts',(37.9226852991021,-40.1384064356313,2.59935489341147));
#60927=CARTESIAN_POINT('Ctrl Pts',(39.4934805709031,-40.5230789002723,2.67786040378825));
#60928=CARTESIAN_POINT('Ctrl Pts',(40.6807808044221,-39.4250208197745,2.75636591416503));
#60929=CARTESIAN_POINT('Ctrl Pts',(40.4197697539726,-37.829004303808,2.83487142454181));
#60930=CARTESIAN_POINT('Ctrl Pts',(38.9445368490487,-37.1663711788227,2.91337693491859));
#60931=CARTESIAN_POINT('Ctrl Pts',(37.5781018083366,-38.0313884332623,2.99188244529537));
#60932=CARTESIAN_POINT('Ctrl Pts',(37.5459181551617,-39.6482871119655,3.07038795567215));
#60933=CARTESIAN_POINT('Ctrl Pts',(38.8768479165872,-40.5669944949197,3.14889346604893));
#60934=CARTESIAN_POINT('Ctrl Pts',(40.3772821563646,-39.963591734637,3.22739897642571));
#60935=CARTESIAN_POINT('Ctrl Pts',(40.7015955221767,-38.3792248834095,3.30590448680249));
#60936=CARTESIAN_POINT('Ctrl Pts',(39.5589362040553,-37.2347917441479,3.38440999717927));
#60937=CARTESIAN_POINT('Ctrl Pts',(37.9740681808821,-37.5566471909729,3.46291550755605));
#60938=CARTESIAN_POINT('Ctrl Pts',(37.3683388050514,-39.0561435938632,3.54142101793282));
#60939=CARTESIAN_POINT('Ctrl Pts',(38.2849805657608,-40.3884969369837,3.61992652830961));
#60940=CARTESIAN_POINT('Ctrl Pts',(39.9019273477536,-40.3588210639772,3.69843203868639));
#60941=CARTESIAN_POINT('Ctrl Pts',(40.769062832428,-38.9937300049359,3.77693754906317));
#60942=CARTESIAN_POINT('Ctrl Pts',(40.1087193040547,-37.5174698739373,3.85544305943995));
#60943=CARTESIAN_POINT('Ctrl Pts',(38.5131085366936,-37.2539858530032,3.93394856981672));
#60944=CARTESIAN_POINT('Ctrl Pts',(37.4132122004928,-38.4395766757617,4.01245408019351));
#60945=CARTESIAN_POINT('Ctrl Pts',(37.7954434779832,-40.0109763068913,4.09095959057028));
#60946=CARTESIAN_POINT('Ctrl Pts',(39.3170082727643,-40.5589161987807,4.16946510094707));
#60947=CARTESIAN_POINT('Ctrl Pts',(40.6133311033497,-39.5919908308444,4.24797061132384));
#60948=CARTESIAN_POINT('Ctrl Pts',(40.5218388376685,-37.9773618584313,4.32647612170062));
#60949=CARTESIAN_POINT('Ctrl Pts',(39.1245839133003,-37.163066933524,4.4049816320774));
#60950=CARTESIAN_POINT('Ctrl Pts',(37.6746577670293,-37.8793850956453,4.48348714245418));
#60951=CARTESIAN_POINT('Ctrl Pts',(37.472388631264,-39.4839052034172,4.56199265283096));
#60952=CARTESIAN_POINT('Ctrl Pts',(38.6991762868961,-40.5376554468423,4.64049816320774));
#60953=CARTESIAN_POINT('Ctrl Pts',(40.2548083764357,-40.0956076208012,4.71900367358451));
#60954=CARTESIAN_POINT('Ctrl Pts',(40.7441571047474,-38.554200594376,4.79750918396131));
#60955=CARTESIAN_POINT('Ctrl Pts',(39.7283628063224,-37.2958050966767,4.87601469433807));
#60956=CARTESIAN_POINT('Ctrl Pts',(38.1184141433653,-37.4489795964024,4.95452020471486));
#60957=CARTESIAN_POINT('Ctrl Pts',(37.3581509755643,-38.876354630039,5.03302571509164));
#60958=CARTESIAN_POINT('Ctrl Pts',(38.1293961434381,-40.2978241770675,5.11153122546842));
#60959=CARTESIAN_POINT('Ctrl Pts',(39.74047711774,-40.4385849029016,5.1900367358452));
#60960=CARTESIAN_POINT('Ctrl Pts',(40.7465412595899,-39.172390472672,5.26854224622198));
#60961=CARTESIAN_POINT('Ctrl Pts',(40.245320117397,-37.6348118380701,5.34704775659875));
#60962=CARTESIAN_POINT('Ctrl Pts',(38.6863332531482,-37.2047504097699,5.42555326697554));
#60963=CARTESIAN_POINT('Ctrl Pts',(37.4676918900007,-38.2679674179302,5.50405877735231));
#60964=CARTESIAN_POINT('Ctrl Pts',(37.682353512212,-39.8707995453507,5.5825642877291));
#60965=CARTESIAN_POINT('Ctrl Pts',(39.1377017503128,-40.5760812986116,5.66106979810587));
#60966=CARTESIAN_POINT('Ctrl Pts',(40.5287528808974,-39.7507094311768,5.73957530848265));
#60967=CARTESIAN_POINT('Ctrl Pts',(40.6075610666769,-38.1360867686638,5.81808081885943));
#60968=CARTESIAN_POINT('Ctrl Pts',(39.3042977946098,-37.1778412776414,5.89658632923621));
#60969=CARTESIAN_POINT('Ctrl Pts',(37.7859967609014,-37.7402586745479,5.97509183961299));
#60970=CARTESIAN_POINT('Ctrl Pts',(37.5416266421298,-38.7853369848302,6.02742884653084));
#60971=CARTESIAN_POINT('Ctrl Pts',(37.6653123637055,-39.2458951477601,6.05359734998977));
#60972=CARTESIAN_POINT('Ctrl Pts',(39.3533377835637,-37.3537893102425,1.83920795003069));
#60973=CARTESIAN_POINT('Ctrl Pts',(38.8548175316166,-37.2592519394722,1.86537645348962));
#60974=CARTESIAN_POINT('Ctrl Pts',(37.7654311854195,-37.6018059239151,1.91771346040747));
#60975=CARTESIAN_POINT('Ctrl Pts',(37.2896667129688,-39.2575786043963,1.99621897078425));
#60976=CARTESIAN_POINT('Ctrl Pts',(38.4102343379238,-40.564025818193,2.07472448116103));
#60977=CARTESIAN_POINT('Ctrl Pts',(40.1171149825864,-40.3517571681556,2.15322999153781));
#60978=CARTESIAN_POINT('Ctrl Pts',(40.8820206309179,-38.8100483503822,2.23173550191459));
#60979=CARTESIAN_POINT('Ctrl Pts',(40.0177367088944,-37.3220789090571,2.31024101229137));
#60980=CARTESIAN_POINT('Ctrl Pts',(38.2999828751462,-37.2220283999295,2.38874652266815));
#60981=CARTESIAN_POINT('Ctrl Pts',(37.2689794778045,-38.599756793647,2.46725203304492));
#60982=CARTESIAN_POINT('Ctrl Pts',(37.8495046941263,-40.2196189105814,2.5457575434217));
#60983=CARTESIAN_POINT('Ctrl Pts',(39.5208554154611,-40.6289164255391,2.62426305379848));
#60984=CARTESIAN_POINT('Ctrl Pts',(40.7841614218878,-39.4605654648164,2.70276856417526));
#60985=CARTESIAN_POINT('Ctrl Pts',(40.5064415845057,-37.7623789454716,2.78127407455204));
#60986=CARTESIAN_POINT('Ctrl Pts',(38.936770715205,-37.057326943275,2.85977958492882));
#60987=CARTESIAN_POINT('Ctrl Pts',(37.4828624739785,-37.9777188225534,2.9382850953056));
#60988=CARTESIAN_POINT('Ctrl Pts',(37.4486185639574,-39.6981242894462,3.01679060568238));
#60989=CARTESIAN_POINT('Ctrl Pts',(38.8647486330617,-40.6756433046616,3.09529611605916));
#60990=CARTESIAN_POINT('Ctrl Pts',(40.4612341165532,-40.033613336302,3.17380162643594));
#60991=CARTESIAN_POINT('Ctrl Pts',(40.8063086069208,-38.3478222423284,3.25230713681272));
#60992=CARTESIAN_POINT('Ctrl Pts',(39.5905012322319,-37.1301274942209,3.3308126471895));
#60993=CARTESIAN_POINT('Ctrl Pts',(37.9041768834746,-37.472586720368,3.40931815756627));
#60994=CARTESIAN_POINT('Ctrl Pts',(37.259671359806,-39.0680743307528,3.48782366794306));
#60995=CARTESIAN_POINT('Ctrl Pts',(38.2349925206666,-40.4857191130318,3.56632917831984));
#60996=CARTESIAN_POINT('Ctrl Pts',(39.9554491702113,-40.4541435203075,3.64483468869662));
#60997=CARTESIAN_POINT('Ctrl Pts',(40.8780948795684,-39.0016652965856,3.7233401990734));
#60998=CARTESIAN_POINT('Ctrl Pts',(40.1754790439541,-37.4309014426854,3.80184570945018));
#60999=CARTESIAN_POINT('Ctrl Pts',(38.4777242474675,-37.1505503260543,3.88035121982696));
#61000=CARTESIAN_POINT('Ctrl Pts',(37.3074173539442,-38.4120374927131,3.95885673020373));
#61001=CARTESIAN_POINT('Ctrl Pts',(37.7141174076169,-40.0840312618198,4.03736224058051));
#61002=CARTESIAN_POINT('Ctrl Pts',(39.333086131911,-40.6670478713029,4.11586775095729));
#61003=CARTESIAN_POINT('Ctrl Pts',(40.7123938856819,-39.6382241664006,4.19437326133408));
#61004=CARTESIAN_POINT('Ctrl Pts',(40.6150446849375,-37.9202337024769,4.27287877171085));
#61005=CARTESIAN_POINT('Ctrl Pts',(39.1283436057741,-37.0538111746305,4.35138428208763));
#61006=CARTESIAN_POINT('Ctrl Pts',(37.5855995232344,-37.8159848954578,4.42988979246441));
#61007=CARTESIAN_POINT('Ctrl Pts',(37.3703820012353,-39.5232193693979,4.50839530284119));
#61008=CARTESIAN_POINT('Ctrl Pts',(38.675703241994,-40.6444260989267,4.58690081321797));
#61009=CARTESIAN_POINT('Ctrl Pts',(40.3309201003962,-40.1740803026401,4.66540632359475));
#61010=CARTESIAN_POINT('Ctrl Pts',(40.85159479603,-38.533999133735,4.74391183397153));
#61011=CARTESIAN_POINT('Ctrl Pts',(39.7707737852476,-37.1950466549739,4.82241734434831));
#61012=CARTESIAN_POINT('Ctrl Pts',(38.05776324374,-37.3580267168588,4.90092285472509));
#61013=CARTESIAN_POINT('Ctrl Pts',(37.248831349992,-38.8767760630728,4.97942836510187));
#61014=CARTESIAN_POINT('Ctrl Pts',(38.0694482634704,-40.3892418792306,5.05793387547864));
#61015=CARTESIAN_POINT('Ctrl Pts',(39.7836636019472,-40.5390134916628,5.13643938585543));
#61016=CARTESIAN_POINT('Ctrl Pts',(40.8541315740477,-39.1917628267891,5.2149448962322));
#61017=CARTESIAN_POINT('Ctrl Pts',(40.3208244444739,-37.5557551266231,5.29345040660899));
#61018=CARTESIAN_POINT('Ctrl Pts',(38.6620380533447,-37.098163044885,5.37195591698576));
#61019=CARTESIAN_POINT('Ctrl Pts',(37.3653845951192,-38.2294425600612,5.45046142736254));
#61020=CARTESIAN_POINT('Ctrl Pts',(37.5937879163964,-39.9348809965236,5.52896693773932));
#61021=CARTESIAN_POINT('Ctrl Pts',(39.1423011893922,-40.6853118058201,5.6074724481161));
#61022=CARTESIAN_POINT('Ctrl Pts',(40.6224013350022,-39.8071032379875,5.68597795849288));
#61023=CARTESIAN_POINT('Ctrl Pts',(40.706254476474,-38.0891194878961,5.76448346886966));
#61024=CARTESIAN_POINT('Ctrl Pts',(39.3195619844849,-37.0695313077001,5.84298897924644));
#61025=CARTESIAN_POINT('Ctrl Pts',(37.7040659529861,-37.6679522088103,5.92149448962322));
#61026=CARTESIAN_POINT('Ctrl Pts',(37.4440523270134,-38.7799318659295,5.97383149654107));
#61027=CARTESIAN_POINT('Ctrl Pts',(37.5756558680257,-39.2699729499894,6.));
#61028=CARTESIAN_POINT('Ctrl Pts',(39.301448933936,-37.6274127691862,2.));
#61029=CARTESIAN_POINT('Ctrl Pts',(39.2531837869401,-37.6126947647985,2.));
#61030=CARTESIAN_POINT('Ctrl Pts',(39.2041689564388,-37.6011555074407,2.));
#61031=CARTESIAN_POINT('Ctrl Pts',(39.1546825373219,-37.5926368604753,2.));
#61032=CARTESIAN_POINT('Ctrl Pts',(39.1029779407392,-37.5837363739855,2.));
#61033=CARTESIAN_POINT('Ctrl Pts',(39.0507578251666,-37.5781330493143,2.));
#61034=CARTESIAN_POINT('Ctrl Pts',(38.9983103424736,-37.5756956341644,2.));
#61035=CARTESIAN_POINT('Ctrl Pts',(38.956247582128,-37.573740832827,2.));
#61036=CARTESIAN_POINT('Ctrl Pts',(38.9140378036175,-37.5738233147571,2.));
#61037=CARTESIAN_POINT('Ctrl Pts',(38.8718222352065,-37.5758984072385,2.));
#61038=CARTESIAN_POINT('Ctrl Pts',(38.8539763703747,-37.5767756148975,2.));
#61039=CARTESIAN_POINT('Ctrl Pts',(38.8361294237341,-37.5780091556835,2.));
#61040=CARTESIAN_POINT('Ctrl Pts',(38.8182919536747,-37.5795967458238,2.));
#61041=CARTESIAN_POINT('Ctrl Pts',(38.8081693423868,-37.5804976896136,2.));
#61042=CARTESIAN_POINT('Ctrl Pts',(38.7980490773275,-37.5815128494687,2.));
#61043=CARTESIAN_POINT('Ctrl Pts',(38.7879491906622,-37.5826397882183,2.));
#61044=CARTESIAN_POINT('Ctrl Pts',(38.7338460090748,-37.5886765858406,2.));
#61045=CARTESIAN_POINT('Ctrl Pts',(38.6802200536712,-37.5979256005399,2.));
#61046=CARTESIAN_POINT('Ctrl Pts',(38.6273722027161,-37.6102449557351,2.));
#61047=CARTESIAN_POINT('Ctrl Pts',(38.5735560674502,-37.6227900275514,2.));
#61048=CARTESIAN_POINT('Ctrl Pts',(38.5205457122249,-37.6385189267485,2.));
#61049=CARTESIAN_POINT('Ctrl Pts',(38.4686492447585,-37.6573343726379,2.));
#61050=CARTESIAN_POINT('Ctrl Pts',(38.4315334390211,-37.670790980931,2.));
#61051=CARTESIAN_POINT('Ctrl Pts',(38.3949871291052,-37.6858274526293,2.));
#61052=CARTESIAN_POINT('Ctrl Pts',(38.3591250016156,-37.7024243845644,2.));
#61053=CARTESIAN_POINT('Ctrl Pts',(38.3438782291838,-37.7094805650532,2.));
#61054=CARTESIAN_POINT('Ctrl Pts',(38.3287551691711,-37.7168189666978,2.));
#61055=CARTESIAN_POINT('Ctrl Pts',(38.3137649009327,-37.7244388227765,2.));
#61056=CARTESIAN_POINT('Ctrl Pts',(38.3048335703861,-37.7289787984644,2.));
#61057=CARTESIAN_POINT('Ctrl Pts',(38.2959544590328,-37.7336161783391,2.));
#61058=CARTESIAN_POINT('Ctrl Pts',(38.2871359717617,-37.7383467951532,2.));
#61059=CARTESIAN_POINT('Ctrl Pts',(38.2370624085326,-37.765208413578,2.));
#61060=CARTESIAN_POINT('Ctrl Pts',(38.1888771643904,-37.7951055006235,2.));
#61061=CARTESIAN_POINT('Ctrl Pts',(38.1428979102889,-37.8279238866627,2.));
#61062=CARTESIAN_POINT('Ctrl Pts',(38.1146649272205,-37.8480756041162,2.));
#61063=CARTESIAN_POINT('Ctrl Pts',(38.0872636609614,-37.869329805144,2.));
#61064=CARTESIAN_POINT('Ctrl Pts',(38.0607696487925,-37.891669608828,2.));
#61065=CARTESIAN_POINT('Ctrl Pts',(38.018758629417,-37.9270933838087,2.));
#61066=CARTESIAN_POINT('Ctrl Pts',(37.9790269569645,-37.9652445703221,2.));
#61067=CARTESIAN_POINT('Ctrl Pts',(37.941638665414,-38.0058250350943,2.));
#61068=CARTESIAN_POINT('Ctrl Pts',(37.9304525998642,-38.0179661552194,2.));
#61069=CARTESIAN_POINT('Ctrl Pts',(37.9194765003133,-38.030325015124,2.));
#61070=CARTESIAN_POINT('Ctrl Pts',(37.9087126348759,-38.0428943202534,2.));
#61071=CARTESIAN_POINT('Ctrl Pts',(37.8987608212084,-38.0545153669214,2.));
#61072=CARTESIAN_POINT('Ctrl Pts',(37.8889863441702,-38.0663216998073,2.));
#61073=CARTESIAN_POINT('Ctrl Pts',(37.8794138052933,-38.078278667435,2.));
#61074=CARTESIAN_POINT('Ctrl Pts',(37.8439500327395,-38.1225761297731,2.));
#61075=CARTESIAN_POINT('Ctrl Pts',(37.8112056943055,-38.1689911399599,2.));
#61076=CARTESIAN_POINT('Ctrl Pts',(37.7812215917711,-38.2171732589094,2.));
#61077=CARTESIAN_POINT('Ctrl Pts',(37.7505286360925,-38.2664944496879,2.));
#61078=CARTESIAN_POINT('Ctrl Pts',(37.7227273546034,-38.3176680405939,2.));
#61079=CARTESIAN_POINT('Ctrl Pts',(37.6978940563208,-38.3703632510374,2.));
#61080=CARTESIAN_POINT('Ctrl Pts',(37.6828172333397,-38.4023556328291,2.));
#61081=CARTESIAN_POINT('Ctrl Pts',(37.668835066908,-38.4349097034794,2.));
#61082=CARTESIAN_POINT('Ctrl Pts',(37.6559717665496,-38.4679573676399,2.));
#61083=CARTESIAN_POINT('Ctrl Pts',(37.6488893068041,-38.4861532228698,2.));
#61084=CARTESIAN_POINT('Ctrl Pts',(37.6421461366806,-38.5044987807375,2.));
#61085=CARTESIAN_POINT('Ctrl Pts',(37.6357470847774,-38.5229830878593,2.));
#61086=CARTESIAN_POINT('Ctrl Pts',(37.6318939139077,-38.5341133607227,2.));
#61087=CARTESIAN_POINT('Ctrl Pts',(37.6281649122475,-38.5452958653565,2.));
#61088=CARTESIAN_POINT('Ctrl Pts',(37.6245631893162,-38.556522141548,2.));
#61089=CARTESIAN_POINT('Ctrl Pts',(37.6061053671321,-38.6140536656795,2.));
#61090=CARTESIAN_POINT('Ctrl Pts',(37.5910431547266,-38.6725526585157,2.));
#61091=CARTESIAN_POINT('Ctrl Pts',(37.5794635885497,-38.7316684529324,2.));
#61092=CARTESIAN_POINT('Ctrl Pts',(37.5719346379231,-38.7701051171919,2.));
#61093=CARTESIAN_POINT('Ctrl Pts',(37.5658787738499,-38.8088033108132,2.));
#61094=CARTESIAN_POINT('Ctrl Pts',(37.5613302232313,-38.8476724431746,2.));
#61095=CARTESIAN_POINT('Ctrl Pts',(37.5594503644604,-38.8637365667855,2.));
#61096=CARTESIAN_POINT('Ctrl Pts',(37.557828067648,-38.8798299274171,2.));
#61097=CARTESIAN_POINT('Ctrl Pts',(37.5564662009589,-38.8959462648398,2.));
#61098=CARTESIAN_POINT('Ctrl Pts',(37.5554691679703,-38.9077451583699,2.));
#61099=CARTESIAN_POINT('Ctrl Pts',(37.5546119020137,-38.9195552385045,2.));
#61100=CARTESIAN_POINT('Ctrl Pts',(37.553895912205,-38.9313640017395,2.));
#61101=CARTESIAN_POINT('Ctrl Pts',(37.5502149156531,-38.9920743864676,2.));
#61102=CARTESIAN_POINT('Ctrl Pts',(37.5502577736837,-39.0528196704592,2.));
#61103=CARTESIAN_POINT('Ctrl Pts',(37.5541374325488,-39.1132620114035,2.));
#61104=CARTESIAN_POINT('Ctrl Pts',(37.5559545726128,-39.1415717682938,2.));
#61105=CARTESIAN_POINT('Ctrl Pts',(37.5586141014167,-39.1698153256793,2.));
#61106=CARTESIAN_POINT('Ctrl Pts',(37.5621314917739,-39.1979588342647,2.));
#61107=CARTESIAN_POINT('Ctrl Pts',(37.5651536457416,-39.2221398342386,2.));
#61108=CARTESIAN_POINT('Ctrl Pts',(37.5688091345127,-39.2462469913776,2.));
#61109=CARTESIAN_POINT('Ctrl Pts',(37.5730824075077,-39.2702648660738,2.));
#61110=CARTESIAN_POINT('Ctrl Pts',(39.696945388151,-39.9649932150637,2.80658032638058));
#61111=CARTESIAN_POINT('Ctrl Pts',(39.5986128055021,-40.0228689487565,2.79940525217632));
#61112=CARTESIAN_POINT('Ctrl Pts',(39.4929004903071,-40.0674950246048,2.79223017797206));
#61113=CARTESIAN_POINT('Ctrl Pts',(39.3829982676155,-40.0959214023961,2.78505510376779));
#61114=CARTESIAN_POINT('Ctrl Pts',(38.9821694242093,-40.1995963950695,2.75888660030887));
#61115=CARTESIAN_POINT('Ctrl Pts',(38.5256079666315,-40.0877889404002,2.73271809684994));
#61116=CARTESIAN_POINT('Ctrl Pts',(38.2180364476029,-39.8106370334519,2.70654959339101));
#61117=CARTESIAN_POINT('Ctrl Pts',(37.9104649285743,-39.5334851265036,2.68038108993209));
#61118=CARTESIAN_POINT('Ctrl Pts',(37.7518833480949,-39.0909887672762,2.65421258647316));
#61119=CARTESIAN_POINT('Ctrl Pts',(37.8134117192226,-38.6815641398492,2.62804408301423));
#61120=CARTESIAN_POINT('Ctrl Pts',(37.8749400903502,-38.2721395124221,2.60187557955531));
#61121=CARTESIAN_POINT('Ctrl Pts',(38.1565784130848,-37.8957866167955,2.57570707609638));
#61122=CARTESIAN_POINT('Ctrl Pts',(38.532016252652,-37.7212755253001,2.54953857263746));
#61123=CARTESIAN_POINT('Ctrl Pts',(38.9074540922192,-37.5467644338048,2.52337006917853));
#61124=CARTESIAN_POINT('Ctrl Pts',(39.376691448619,-37.5740951464408,2.4972015657196));
#61125=CARTESIAN_POINT('Ctrl Pts',(39.7293579794219,-37.7909941772625,2.47103306226067));
#61126=CARTESIAN_POINT('Ctrl Pts',(40.0820245102248,-38.0078932080842,2.44486455880175));
#61127=CARTESIAN_POINT('Ctrl Pts',(40.3181202154309,-38.4143605570917,2.41869605534282));
#61128=CARTESIAN_POINT('Ctrl Pts',(40.3316937547572,-38.8281678760191,2.3925275518839));
#61129=CARTESIAN_POINT('Ctrl Pts',(40.3452672940836,-39.2419751949465,2.36635904842497));
#61130=CARTESIAN_POINT('Ctrl Pts',(40.1363186675303,-39.6631224837939,2.34019054496604));
#61131=CARTESIAN_POINT('Ctrl Pts',(39.7987107859694,-39.9026887516754,2.31402204150712));
#61132=CARTESIAN_POINT('Ctrl Pts',(39.7667081702677,-39.9253977807734,2.31154146979827));
#61133=CARTESIAN_POINT('Ctrl Pts',(39.7335494773786,-39.9464752002681,2.30906089808943));
#61134=CARTESIAN_POINT('Ctrl Pts',(39.6994125047665,-39.9658989902663,2.30658032638058));
#61135=CARTESIAN_POINT('Ctrl Pts',(37.9741697098829,-39.9602191716056,2.));
#61136=CARTESIAN_POINT('Ctrl Pts',(38.3327559670707,-40.3192117233802,2.02616850345893));
#61137=CARTESIAN_POINT('Ctrl Pts',(39.4257675096925,-40.6500214621299,2.07850551037678));
#61138=CARTESIAN_POINT('Ctrl Pts',(40.7517604581817,-39.5501737910362,2.15701102075356));
#61139=CARTESIAN_POINT('Ctrl Pts',(40.5621188491035,-37.8394675163551,2.23551653113034));
#61140=CARTESIAN_POINT('Ctrl Pts',(39.0323736383015,-37.0530949705805,2.31402204150712));
#61141=CARTESIAN_POINT('Ctrl Pts',(37.5317729583208,-37.8957949010443,2.3925275518839));
#61142=CARTESIAN_POINT('Ctrl Pts',(37.4074081512686,-39.612062461691,2.47103306226068));
#61143=CARTESIAN_POINT('Ctrl Pts',(38.7701598472246,-40.6625848481854,2.54953857263746));
#61144=CARTESIAN_POINT('Ctrl Pts',(40.3982034912373,-40.1052897198446,2.62804408301424));
#61145=CARTESIAN_POINT('Ctrl Pts',(40.8313104277201,-38.439942299895,2.70654959339101));
#61146=CARTESIAN_POINT('Ctrl Pts',(39.6811395860237,-37.1600807661057,2.78505510376779));
#61147=CARTESIAN_POINT('Ctrl Pts',(37.9791520940816,-37.4135079224237,2.86356061414458));
#61148=CARTESIAN_POINT('Ctrl Pts',(37.2517503435483,-38.9729479619196,2.94206612452135));
#61149=CARTESIAN_POINT('Ctrl Pts',(38.1512758267994,-40.4398561533634,3.02057163489813));
#61150=CARTESIAN_POINT('Ctrl Pts',(39.8710175096896,-40.4986752642982,3.09907714527491));
#61151=CARTESIAN_POINT('Ctrl Pts',(40.868667784705,-39.0966544678461,3.17758265565169));
#61152=CARTESIAN_POINT('Ctrl Pts',(40.249511348243,-37.4911595684212,3.25608816602847));
#61153=CARTESIAN_POINT('Ctrl Pts',(38.5688218267177,-37.1220364497186,3.33459367640525));
#61154=CARTESIAN_POINT('Ctrl Pts',(37.333881829365,-38.3203235548052,3.41309918678203));
#61155=CARTESIAN_POINT('Ctrl Pts',(37.6522147609438,-40.0113684930191,3.49160469715881));
#61156=CARTESIAN_POINT('Ctrl Pts',(39.238332151816,-40.6786019749499,3.57011020753559));
#61157=CARTESIAN_POINT('Ctrl Pts',(40.6697661826987,-39.7236331447561,3.64861571791237));
#61158=CARTESIAN_POINT('Ctrl Pts',(40.662772801836,-38.0029007557487,3.72712122828915));
#61159=CARTESIAN_POINT('Ctrl Pts',(39.2236238307452,-37.0595985208236,3.80562673866593));
#61160=CARTESIAN_POINT('Ctrl Pts',(37.642982284831,-37.7397023107928,3.88413224904271));
#61161=CARTESIAN_POINT('Ctrl Pts',(37.3384050779085,-39.4332788778856,3.96263775941949));
#61162=CARTESIAN_POINT('Ctrl Pts',(38.5830442911661,-40.6214884944164,4.04114326979627));
#61163=CARTESIAN_POINT('Ctrl Pts',(40.26067788792,-40.2387165281926,4.11964878017305));
#61164=CARTESIAN_POINT('Ctrl Pts',(40.8667641756191,-38.6282419782981,4.19815429054982));
#61165=CARTESIAN_POINT('Ctrl Pts',(39.8577505620191,-37.2343767082119,4.27665980092661));
#61166=CARTESIAN_POINT('Ctrl Pts',(38.1385444446534,-37.3071722287697,4.35516531130338));
#61167=CARTESIAN_POINT('Ctrl Pts',(37.2509707395799,-38.781343787805,4.43367082168017));
#61168=CARTESIAN_POINT('Ctrl Pts',(37.9910266499109,-40.3348192821528,4.51217633205694));
#61169=CARTESIAN_POINT('Ctrl Pts',(39.6950124343117,-40.5744049619641,4.59068184243373));
#61170=CARTESIAN_POINT('Ctrl Pts',(40.8347531457538,-39.285234683173,4.6691873528105));
#61171=CARTESIAN_POINT('Ctrl Pts',(40.3881021894618,-37.6234670214255,4.74769286318729));
#61172=CARTESIAN_POINT('Ctrl Pts',(38.7556268199881,-37.0794146789619,4.82619837356406));
#61173=CARTESIAN_POINT('Ctrl Pts',(37.4013696406987,-38.1409968175026,4.90470388394084));
#61174=CARTESIAN_POINT('Ctrl Pts',(37.5398609233301,-39.8561611622599,4.98320939431763));
#61175=CARTESIAN_POINT('Ctrl Pts',(39.0468979136614,-40.6867079066975,5.0617149046944));
#61176=CARTESIAN_POINT('Ctrl Pts',(40.5709349782279,-39.8877822721679,5.14022041507118));
#61177=CARTESIAN_POINT('Ctrl Pts',(40.745177494668,-38.1758811994982,5.21872592544796));
#61178=CARTESIAN_POINT('Ctrl Pts',(39.4133645670745,-37.0862753673934,5.29723143582474));
#61179=CARTESIAN_POINT('Ctrl Pts',(37.7698897533292,-37.5961550422893,5.37573694620152));
#61180=CARTESIAN_POINT('Ctrl Pts',(37.2886763485592,-39.2482362054987,5.4542424565783));
#61181=CARTESIAN_POINT('Ctrl Pts',(38.4012556794041,-40.5609170045275,5.53274796695508));
#61182=CARTESIAN_POINT('Ctrl Pts',(40.1099052932563,-40.3569060637301,5.61125347733186));
#61183=CARTESIAN_POINT('Ctrl Pts',(40.8821362004287,-38.8192621207562,5.68975898770864));
#61184=CARTESIAN_POINT('Ctrl Pts',(40.025658400892,-37.3267854127763,5.76826449808541));
#61185=CARTESIAN_POINT('Ctrl Pts',(38.3080469143,-37.2183586878016,5.8467700084622));
#61186=CARTESIAN_POINT('Ctrl Pts',(37.2707754210207,-38.5904264849422,5.92527551883897));
#61187=CARTESIAN_POINT('Ctrl Pts',(37.8419099014003,-40.2140906446281,6.00378102921576));
#61188=CARTESIAN_POINT('Ctrl Pts',(39.5137297698779,-40.6299518311032,6.08228653959253));
#61189=CARTESIAN_POINT('Ctrl Pts',(40.3550860167094,-39.8577931806474,6.13462354651039));
#61190=CARTESIAN_POINT('Ctrl Pts',(40.5224743779889,-39.378793292775,6.16079204996931));
#61191=CARTESIAN_POINT('Ctrl Pts',(38.0398499461207,-39.8946132698472,1.94640265001023));
#61192=CARTESIAN_POINT('Ctrl Pts',(38.3768621543504,-40.2320073282822,1.97257115346916));
#61193=CARTESIAN_POINT('Ctrl Pts',(39.4041135512345,-40.5429141695936,2.02490816038701));
#61194=CARTESIAN_POINT('Ctrl Pts',(40.650329218204,-39.5092379343175,2.10341367076379));
#61195=CARTESIAN_POINT('Ctrl Pts',(40.4720972414715,-37.9014549038573,2.18191918114057));
#61196=CARTESIAN_POINT('Ctrl Pts',(39.0343879004488,-37.1623938193051,2.26042469151735));
#61197=CARTESIAN_POINT('Ctrl Pts',(37.6240696333812,-37.954393397504,2.33893020189413));
#61198=CARTESIAN_POINT('Ctrl Pts',(37.5071871332558,-39.567403123707,2.41743571227091));
#61199=CARTESIAN_POINT('Ctrl Pts',(38.7879499877074,-40.5547216897998,2.49594122264769));
#61200=CARTESIAN_POINT('Ctrl Pts',(40.3180437170825,-40.0309557671714,2.57444673302446));
#61201=CARTESIAN_POINT('Ctrl Pts',(40.7250931288709,-38.4658026130365,2.65295224340125));
#61202=CARTESIAN_POINT('Ctrl Pts',(39.6441213754036,-37.2629429019217,2.73145775377802));
#61203=CARTESIAN_POINT('Ctrl Pts',(38.044532569248,-37.5011228205998,2.80996326415481));
#61204=CARTESIAN_POINT('Ctrl Pts',(37.3608943502601,-38.9667404252288,2.88846877453158));
#61205=CARTESIAN_POINT('Ctrl Pts',(38.2063006183275,-40.3453932847829,2.96697428490837));
#61206=CARTESIAN_POINT('Ctrl Pts',(39.8225754490498,-40.400673592003,3.04547979528514));
#61207=CARTESIAN_POINT('Ctrl Pts',(40.7602029110188,-39.0830042303774,3.12398530566192));
#61208=CARTESIAN_POINT('Ctrl Pts',(40.1782975152901,-37.5741026188095,3.2024908160387));
#61209=CARTESIAN_POINT('Ctrl Pts',(38.598725304576,-37.2271874907223,3.28099632641548));
#61210=CARTESIAN_POINT('Ctrl Pts',(37.4380844623892,-38.3533806319362,3.35950183679226));
#61211=CARTESIAN_POINT('Ctrl Pts',(37.7372651534312,-39.9426852341612,3.43800734716904));
#61212=CARTESIAN_POINT('Ctrl Pts',(39.2279550884041,-40.5697751592293,3.51651285754582));
#61213=CARTESIAN_POINT('Ctrl Pts',(40.5732680612611,-39.6722612478536,3.5950183679226));
#61214=CARTESIAN_POINT('Ctrl Pts',(40.5666954314397,-38.0550553160375,3.67352387829937));
#61215=CARTESIAN_POINT('Ctrl Pts',(39.214131681444,-37.1685060887655,3.75202938867616));
#61216=CARTESIAN_POINT('Ctrl Pts',(37.7285881416946,-37.8076919903125,3.83053489905293));
#61217=CARTESIAN_POINT('Ctrl Pts',(37.4423355733826,-39.399375908035,3.90904040942972));
#61218=CARTESIAN_POINT('Ctrl Pts',(38.6120920860802,-40.516097864552,3.98754591980649));
#61219=CARTESIAN_POINT('Ctrl Pts',(40.188792229238,-40.1563550606944,4.06605143018328));
#61220=CARTESIAN_POINT('Ctrl Pts',(40.758413831017,-38.6427733952556,4.14455694056005));
#61221=CARTESIAN_POINT('Ctrl Pts',(39.8101066964379,-37.3327688894207,4.22306245093684));
#61222=CARTESIAN_POINT('Ctrl Pts',(38.1943352093782,-37.401184727007,4.30156796131362));
#61223=CARTESIAN_POINT('Ctrl Pts',(37.360161650527,-38.7866639595805,4.38007347169039));
#61224=CARTESIAN_POINT('Ctrl Pts',(38.0556927021353,-40.2466758710431,4.45857898206717));
#61225=CARTESIAN_POINT('Ctrl Pts',(39.6571595751178,-40.4718470743308,4.53708449244395));
#61226=CARTESIAN_POINT('Ctrl Pts',(40.7283287185891,-39.2602386712458,4.61559000282073));
#61227=CARTESIAN_POINT('Ctrl Pts',(40.3085501518688,-37.6984499020877,4.69409551319751));
#61228=CARTESIAN_POINT('Ctrl Pts',(38.7742913281713,-37.1871300239526,4.77260102357429));
#61229=CARTESIAN_POINT('Ctrl Pts',(37.5015119247368,-38.1848429411531,4.85110653395107));
#61230=CARTESIAN_POINT('Ctrl Pts',(37.631670992589,-39.7968158255486,4.92961204432785));
#61231=CARTESIAN_POINT('Ctrl Pts',(39.0480383346578,-40.5773934042213,5.00811755470463));
#61232=CARTESIAN_POINT('Ctrl Pts',(40.4803829553959,-39.8265344772346,5.08662306508141));
#61233=CARTESIAN_POINT('Ctrl Pts',(40.6441423133075,-38.2176285328299,5.16512857545819));
#61234=CARTESIAN_POINT('Ctrl Pts',(39.3924568215175,-37.1935779446744,5.24363408583497));
#61235=CARTESIAN_POINT('Ctrl Pts',(37.8478603261192,-37.6727811258441,5.32213959621175));
#61236=CARTESIAN_POINT('Ctrl Pts',(37.3955987323729,-39.2254661767282,5.40064510658853));
#61237=CARTESIAN_POINT('Ctrl Pts',(38.4412406375015,-40.4591706088247,5.47915061696531));
#61238=CARTESIAN_POINT('Ctrl Pts',(40.04709074445,-40.2674338194666,5.55765612734208));
#61239=CARTESIAN_POINT('Ctrl Pts',(40.7728610105231,-38.8223009670344,5.63616163771887));
#61240=CARTESIAN_POINT('Ctrl Pts',(39.9679124974785,-37.419617899835,5.71466714809565));
#61241=CARTESIAN_POINT('Ctrl Pts',(38.3536397015357,-37.3177145801109,5.79317265847242));
#61242=CARTESIAN_POINT('Ctrl Pts',(37.3787747995027,-38.6072330401369,5.87167816884921));
#61243=CARTESIAN_POINT('Ctrl Pts',(37.9155474408704,-40.1332107732787,5.95018367922598));
#61244=CARTESIAN_POINT('Ctrl Pts',(39.4867836339601,-40.5240520115073,6.02868918960276));
#61245=CARTESIAN_POINT('Ctrl Pts',(40.2775203701537,-39.7983496548842,6.08102619652062));
#61246=CARTESIAN_POINT('Ctrl Pts',(40.4348379475454,-39.3481684036012,6.10719469997954));
#61247=CARTESIAN_POINT('Ctrl Pts',(38.1055301823584,-39.8290073680889,1.89280530002046));
#61248=CARTESIAN_POINT('Ctrl Pts',(38.4209683416301,-40.1448029331842,1.91897380347939));
#61249=CARTESIAN_POINT('Ctrl Pts',(39.3824595927764,-40.4358068770573,1.97131081039724));
#61250=CARTESIAN_POINT('Ctrl Pts',(40.5488979782264,-39.4683020775988,2.04981632077402));
#61251=CARTESIAN_POINT('Ctrl Pts',(40.3820756338396,-37.9634422913595,2.1283218311508));
#61252=CARTESIAN_POINT('Ctrl Pts',(39.0364021625962,-37.2716926680296,2.20682734152758));
#61253=CARTESIAN_POINT('Ctrl Pts',(37.7163663084416,-38.0129918939637,2.28533285190436));
#61254=CARTESIAN_POINT('Ctrl Pts',(37.606966115243,-39.5227437857229,2.36383836228114));
#61255=CARTESIAN_POINT('Ctrl Pts',(38.8057401281902,-40.4468585314142,2.44234387265792));
#61256=CARTESIAN_POINT('Ctrl Pts',(40.2378839429277,-39.9566218144982,2.5208493830347));
#61257=CARTESIAN_POINT('Ctrl Pts',(40.6188758300216,-38.491662926178,2.59935489341147));
#61258=CARTESIAN_POINT('Ctrl Pts',(39.6071031647834,-37.3658050377377,2.67786040378825));
#61259=CARTESIAN_POINT('Ctrl Pts',(38.1099130444145,-37.5887377187761,2.75636591416503));
#61260=CARTESIAN_POINT('Ctrl Pts',(37.4700383569718,-38.9605328885379,2.83487142454181));
#61261=CARTESIAN_POINT('Ctrl Pts',(38.2613254098556,-40.2509304162025,2.91337693491859));
#61262=CARTESIAN_POINT('Ctrl Pts',(39.77413338841,-40.3026719197079,2.99188244529537));
#61263=CARTESIAN_POINT('Ctrl Pts',(40.6517380373327,-39.0693539929087,3.07038795567215));
#61264=CARTESIAN_POINT('Ctrl Pts',(40.1070836823373,-37.6570456691978,3.14889346604893));
#61265=CARTESIAN_POINT('Ctrl Pts',(38.6286287824343,-37.3323385317259,3.22739897642571));
#61266=CARTESIAN_POINT('Ctrl Pts',(37.5422870954134,-38.3864377090672,3.30590448680249));
#61267=CARTESIAN_POINT('Ctrl Pts',(37.8223155459186,-39.8740019753033,3.38440999717927));
#61268=CARTESIAN_POINT('Ctrl Pts',(39.2175780249922,-40.4609483435087,3.46291550755605));
#61269=CARTESIAN_POINT('Ctrl Pts',(40.4767699398235,-39.620889350951,3.54142101793283));
#61270=CARTESIAN_POINT('Ctrl Pts',(40.4706180610435,-38.1072098763263,3.61992652830961));
#61271=CARTESIAN_POINT('Ctrl Pts',(39.2046395321427,-37.2774136567075,3.69843203868639));
#61272=CARTESIAN_POINT('Ctrl Pts',(37.8141939985582,-37.8756816698323,3.77693754906317));
#61273=CARTESIAN_POINT('Ctrl Pts',(37.5462660688567,-39.3654729381844,3.85544305943995));
#61274=CARTESIAN_POINT('Ctrl Pts',(38.6411398809942,-40.4107072346876,3.93394856981672));
#61275=CARTESIAN_POINT('Ctrl Pts',(40.1169065705561,-40.0739935931963,4.01245408019351));
#61276=CARTESIAN_POINT('Ctrl Pts',(40.650063486415,-38.6573048122132,4.09095959057028));
#61277=CARTESIAN_POINT('Ctrl Pts',(39.7624628308567,-37.4311610706296,4.16946510094707));
#61278=CARTESIAN_POINT('Ctrl Pts',(38.250125974103,-37.4951972252442,4.24797061132384));
#61279=CARTESIAN_POINT('Ctrl Pts',(37.4693525614741,-38.7919841313561,4.32647612170063));
#61280=CARTESIAN_POINT('Ctrl Pts',(38.1203587543597,-40.1585324599333,4.4049816320774));
#61281=CARTESIAN_POINT('Ctrl Pts',(39.6193067159238,-40.3692891866976,4.48348714245418));
#61282=CARTESIAN_POINT('Ctrl Pts',(40.6219042914244,-39.2352426593185,4.56199265283096));
#61283=CARTESIAN_POINT('Ctrl Pts',(40.2289981142758,-37.77343278275,4.64049816320774));
#61284=CARTESIAN_POINT('Ctrl Pts',(38.7929558363546,-37.2948453689432,4.71900367358452));
#61285=CARTESIAN_POINT('Ctrl Pts',(37.601654208775,-38.2286890648036,4.7975091839613));
#61286=CARTESIAN_POINT('Ctrl Pts',(37.7234810618479,-39.7374704888372,4.87601469433808));
#61287=CARTESIAN_POINT('Ctrl Pts',(39.0491787556542,-40.468078901745,4.95452020471486));
#61288=CARTESIAN_POINT('Ctrl Pts',(40.3898309325639,-39.7652866823013,5.03302571509164));
#61289=CARTESIAN_POINT('Ctrl Pts',(40.5431071319469,-38.2593758661616,5.11153122546842));
#61290=CARTESIAN_POINT('Ctrl Pts',(39.3715490759606,-37.3008805219554,5.1900367358452));
#61291=CARTESIAN_POINT('Ctrl Pts',(37.9258308989092,-37.7494072093988,5.26854224622198));
#61292=CARTESIAN_POINT('Ctrl Pts',(37.5025211161865,-39.2026961479577,5.34704775659876));
#61293=CARTESIAN_POINT('Ctrl Pts',(38.4812255955989,-40.3574242131219,5.42555326697554));
#61294=CARTESIAN_POINT('Ctrl Pts',(39.9842761956435,-40.1779615752029,5.50405877735232));
#61295=CARTESIAN_POINT('Ctrl Pts',(40.6635858206177,-38.8253398133127,5.58256428772909));
#61296=CARTESIAN_POINT('Ctrl Pts',(39.9101665940649,-37.5124503868936,5.66106979810588));
#61297=CARTESIAN_POINT('Ctrl Pts',(38.3992324887715,-37.4170704724203,5.73957530848265));
#61298=CARTESIAN_POINT('Ctrl Pts',(37.4867741779846,-38.6240395953316,5.81808081885943));
#61299=CARTESIAN_POINT('Ctrl Pts',(37.9891849803405,-40.0523309019293,5.89658632923621));
#61300=CARTESIAN_POINT('Ctrl Pts',(39.4598374980421,-40.4181521919114,5.97509183961299));
#61301=CARTESIAN_POINT('Ctrl Pts',(40.1999547235979,-39.7389061291211,6.02742884653085));
#61302=CARTESIAN_POINT('Ctrl Pts',(40.3472015171019,-39.3175435144275,6.05359734998977));
#61303=CARTESIAN_POINT('Ctrl Pts',(38.1712104185962,-39.7634014663305,1.83920795003069));
#61304=CARTESIAN_POINT('Ctrl Pts',(38.4650745289099,-40.0575985380862,1.86537645348962));
#61305=CARTESIAN_POINT('Ctrl Pts',(39.3608056343184,-40.328699584521,1.91771346040747));
#61306=CARTESIAN_POINT('Ctrl Pts',(40.4474667382487,-39.42736622088,1.99621897078425));
#61307=CARTESIAN_POINT('Ctrl Pts',(40.2920540262076,-38.0254296788618,2.07472448116103));
#61308=CARTESIAN_POINT('Ctrl Pts',(39.0384164247435,-37.3809915167542,2.15322999153781));
#61309=CARTESIAN_POINT('Ctrl Pts',(37.8086629835021,-38.0715903904234,2.23173550191459));
#61310=CARTESIAN_POINT('Ctrl Pts',(37.7067450972302,-39.4780844477388,2.31024101229137));
#61311=CARTESIAN_POINT('Ctrl Pts',(38.8235302686731,-40.3389953730286,2.38874652266814));
#61312=CARTESIAN_POINT('Ctrl Pts',(40.1577241687729,-39.8822878618251,2.46725203304493));
#61313=CARTESIAN_POINT('Ctrl Pts',(40.5126585311724,-38.5175232393194,2.5457575434217));
#61314=CARTESIAN_POINT('Ctrl Pts',(39.5700849541633,-37.4686671735537,2.62426305379848));
#61315=CARTESIAN_POINT('Ctrl Pts',(38.1752935195809,-37.6763526169523,2.70276856417526));
#61316=CARTESIAN_POINT('Ctrl Pts',(37.5791823636836,-38.9543253518471,2.78127407455204));
#61317=CARTESIAN_POINT('Ctrl Pts',(38.3163502013836,-40.156467547622,2.85977958492882));
#61318=CARTESIAN_POINT('Ctrl Pts',(39.7256913277703,-40.2046702474127,2.9382850953056));
#61319=CARTESIAN_POINT('Ctrl Pts',(40.5432731636465,-39.05570375544,3.01679060568238));
#61320=CARTESIAN_POINT('Ctrl Pts',(40.0358698493845,-37.7399887195861,3.09529611605916));
#61321=CARTESIAN_POINT('Ctrl Pts',(38.6585322602926,-37.4374895727296,3.17380162643594));
#61322=CARTESIAN_POINT('Ctrl Pts',(37.6464897284375,-38.4194947861982,3.25230713681272));
#61323=CARTESIAN_POINT('Ctrl Pts',(37.907365938406,-39.8053187164454,3.3308126471895));
#61324=CARTESIAN_POINT('Ctrl Pts',(39.2072009615803,-40.3521215277881,3.40931815756628));
#61325=CARTESIAN_POINT('Ctrl Pts',(40.3802718183859,-39.5695174540484,3.48782366794306));
#61326=CARTESIAN_POINT('Ctrl Pts',(40.3745406906472,-38.159364436615,3.56632917831984));
#61327=CARTESIAN_POINT('Ctrl Pts',(39.1951473828414,-37.3863212246494,3.64483468869662));
#61328=CARTESIAN_POINT('Ctrl Pts',(37.8997998554218,-37.943671349352,3.7233401990734));
#61329=CARTESIAN_POINT('Ctrl Pts',(37.6501965643308,-39.3315699683338,3.80184570945018));
#61330=CARTESIAN_POINT('Ctrl Pts',(38.6701876759083,-40.3053166048232,3.88035121982695));
#61331=CARTESIAN_POINT('Ctrl Pts',(40.0450209118742,-39.9916321256981,3.95885673020374));
#61332=CARTESIAN_POINT('Ctrl Pts',(40.5417131418129,-38.6718362291708,4.03736224058051));
#61333=CARTESIAN_POINT('Ctrl Pts',(39.7148189652755,-37.5295532518384,4.11586775095729));
#61334=CARTESIAN_POINT('Ctrl Pts',(38.3059167388278,-37.5892097234815,4.19437326133407));
#61335=CARTESIAN_POINT('Ctrl Pts',(37.5785434724212,-38.7973043031316,4.27287877171085));
#61336=CARTESIAN_POINT('Ctrl Pts',(38.1850248065841,-40.0703890488237,4.35138428208763));
#61337=CARTESIAN_POINT('Ctrl Pts',(39.5814538567299,-40.2667312990643,4.42988979246441));
#61338=CARTESIAN_POINT('Ctrl Pts',(40.5154798642596,-39.2102466473914,4.50839530284119));
#61339=CARTESIAN_POINT('Ctrl Pts',(40.1494460766828,-37.8484156634123,4.58690081321798));
#61340=CARTESIAN_POINT('Ctrl Pts',(38.8116203445378,-37.4025607139339,4.66540632359475));
#61341=CARTESIAN_POINT('Ctrl Pts',(37.7017964928131,-38.2725351884542,4.74391183397153));
#61342=CARTESIAN_POINT('Ctrl Pts',(37.8152911311068,-39.6781251521259,4.82241734434831));
#61343=CARTESIAN_POINT('Ctrl Pts',(39.0503191766506,-40.3587643992688,4.90092285472509));
#61344=CARTESIAN_POINT('Ctrl Pts',(40.2992789097318,-39.7040388873681,4.97942836510187));
#61345=CARTESIAN_POINT('Ctrl Pts',(40.4420719505864,-38.3011231994933,5.05793387547865));
#61346=CARTESIAN_POINT('Ctrl Pts',(39.3506413304036,-37.4081830992363,5.13643938585543));
#61347=CARTESIAN_POINT('Ctrl Pts',(38.0038014716991,-37.8260332929536,5.21494489623221));
#61348=CARTESIAN_POINT('Ctrl Pts',(37.6094435000001,-39.1799261191872,5.29345040660899));
#61349=CARTESIAN_POINT('Ctrl Pts',(38.5212105536963,-40.2556778174191,5.37195591698577));
#61350=CARTESIAN_POINT('Ctrl Pts',(39.9214616468371,-40.0884893309394,5.45046142736255));
#61351=CARTESIAN_POINT('Ctrl Pts',(40.5543106307123,-38.8283786595909,5.52896693773932));
#61352=CARTESIAN_POINT('Ctrl Pts',(39.8524206906513,-37.6052828739523,5.60747244811611));
#61353=CARTESIAN_POINT('Ctrl Pts',(38.4448252760073,-37.5164263647296,5.68597795849288));
#61354=CARTESIAN_POINT('Ctrl Pts',(37.5947735564665,-38.6408461505263,5.76448346886966));
#61355=CARTESIAN_POINT('Ctrl Pts',(38.0628225198106,-39.97145103058,5.84298897924644));
#61356=CARTESIAN_POINT('Ctrl Pts',(39.4328913621242,-40.3122523723155,5.92149448962322));
#61357=CARTESIAN_POINT('Ctrl Pts',(40.1223890770422,-39.6794626033579,5.97383149654108));
#61358=CARTESIAN_POINT('Ctrl Pts',(40.2595650866584,-39.2869186252538,6.));
#61359=CARTESIAN_POINT('Ctrl Pts',(39.6985816414592,-39.9636701304733,2.44341967361942));
#61360=CARTESIAN_POINT('Ctrl Pts',(39.808547063221,-39.9013157119468,2.45136379342792));
#61361=CARTESIAN_POINT('Ctrl Pts',(39.9090512176556,-39.8231041003581,2.45930791323642));
#61362=CARTESIAN_POINT('Ctrl Pts',(39.9945142458228,-39.7309450099414,2.46725203304493));
#61363=CARTESIAN_POINT('Ctrl Pts',(40.2760356229061,-39.4273663209899,2.49342053650385));
#61364=CARTESIAN_POINT('Ctrl Pts',(40.3943470770392,-38.9724447801547,2.51958903996278));
#61365=CARTESIAN_POINT('Ctrl Pts',(40.2964072079376,-38.5701746654428,2.54575754342171));
#61366=CARTESIAN_POINT('Ctrl Pts',(40.1984673388361,-38.1679045507309,2.57192604688063));
#61367=CARTESIAN_POINT('Ctrl Pts',(39.8842761464997,-37.8182858621423,2.59809455033956));
#61368=CARTESIAN_POINT('Ctrl Pts',(39.4947153112344,-37.6780907584144,2.62426305379849));
#61369=CARTESIAN_POINT('Ctrl Pts',(39.1051544759692,-37.5378956546866,2.65043155725741));
#61370=CARTESIAN_POINT('Ctrl Pts',(38.640223997775,-37.6071241358194,2.67660006071634));
#61371=CARTESIAN_POINT('Ctrl Pts',(38.3084068993617,-37.8547338322017,2.70276856417527));
#61372=CARTESIAN_POINT('Ctrl Pts',(37.9765898009484,-38.1023435285839,2.72893706763419));
#61373=CARTESIAN_POINT('Ctrl Pts',(37.777886082316,-38.5283344402155,2.75510557109312));
#61374=CARTESIAN_POINT('Ctrl Pts',(37.8013955292832,-38.9416869286604,2.78127407455204));
#61375=CARTESIAN_POINT('Ctrl Pts',(37.8249049762503,-39.3550394171054,2.80744257801097));
#61376=CARTESIAN_POINT('Ctrl Pts',(38.0706275888169,-39.7557534823637,2.8336110814699));
#61377=CARTESIAN_POINT('Ctrl Pts',(38.4283790828314,-39.9641442982913,2.85977958492882));
#61378=CARTESIAN_POINT('Ctrl Pts',(38.7861305768458,-40.1725351142189,2.88594808838775));
#61379=CARTESIAN_POINT('Ctrl Pts',(39.2559109523081,-40.1886026808158,2.91211659184668));
#61380=CARTESIAN_POINT('Ctrl Pts',(39.6270647793519,-40.0051420487855,2.9382850953056));
#61381=CARTESIAN_POINT('Ctrl Pts',(39.6513397427561,-39.9931429804635,2.93999662141021));
#61382=CARTESIAN_POINT('Ctrl Pts',(39.6751928123865,-39.9802903924142,2.94170814751481));
#61383=CARTESIAN_POINT('Ctrl Pts',(39.6985897981371,-39.9666323328489,2.94341967361942));
#61384=CARTESIAN_POINT('Ctrl Pts',(37.9741697098829,-39.9602191716056,2.));
#61385=CARTESIAN_POINT('Ctrl Pts',(38.0210640733086,-39.9994677669677,2.));
#61386=CARTESIAN_POINT('Ctrl Pts',(38.0703056805301,-40.0355567831455,2.));
#61387=CARTESIAN_POINT('Ctrl Pts',(38.1215357900136,-40.0684647235096,2.));
#61388=CARTESIAN_POINT('Ctrl Pts',(38.1724676227797,-40.1011810641969,2.));
#61389=CARTESIAN_POINT('Ctrl Pts',(38.2253661047044,-40.1307533458139,2.));
#61390=CARTESIAN_POINT('Ctrl Pts',(38.2799014945801,-40.1571104299646,2.));
#61391=CARTESIAN_POINT('Ctrl Pts',(38.3210824949734,-40.1770133057898,2.));
#61392=CARTESIAN_POINT('Ctrl Pts',(38.3631974573972,-40.1950818318595,2.));
#61393=CARTESIAN_POINT('Ctrl Pts',(38.4061067602768,-40.2112658265379,2.));
#61394=CARTESIAN_POINT('Ctrl Pts',(38.4283821944254,-40.2196673964429,2.));
#61395=CARTESIAN_POINT('Ctrl Pts',(38.4508716987496,-40.2275608160991,2.));
#61396=CARTESIAN_POINT('Ctrl Pts',(38.4735555240459,-40.2349372243514,2.));
#61397=CARTESIAN_POINT('Ctrl Pts',(38.4855017473433,-40.2388219403974,2.));
#61398=CARTESIAN_POINT('Ctrl Pts',(38.4975038315133,-40.2425636903004,2.));
#61399=CARTESIAN_POINT('Ctrl Pts',(38.5095371704371,-40.2461549840666,2.));
#61400=CARTESIAN_POINT('Ctrl Pts',(38.5662684087361,-40.2630861570139,2.));
#61401=CARTESIAN_POINT('Ctrl Pts',(38.6237986216725,-40.2767129172189,2.));
#61402=CARTESIAN_POINT('Ctrl Pts',(38.6818163301316,-40.286975145154,2.));
#61403=CARTESIAN_POINT('Ctrl Pts',(38.7386491570057,-40.2970277900975,2.));
#61404=CARTESIAN_POINT('Ctrl Pts',(38.7959508055663,-40.3038518408626,2.));
#61405=CARTESIAN_POINT('Ctrl Pts',(38.8534268715921,-40.3073420065174,2.));
#61406=CARTESIAN_POINT('Ctrl Pts',(38.8950337651378,-40.3098685355737,2.));
#61407=CARTESIAN_POINT('Ctrl Pts',(38.936732068862,-40.3106470090916,2.));
#61408=CARTESIAN_POINT('Ctrl Pts',(38.9784050690609,-40.3096213125542,2.));
#61409=CARTESIAN_POINT('Ctrl Pts',(39.0001855019757,-40.3090852312902,2.));
#61410=CARTESIAN_POINT('Ctrl Pts',(39.0219589293942,-40.3080560888428,2.));
#61411=CARTESIAN_POINT('Ctrl Pts',(39.0437079205698,-40.3065243689253,2.));
#61412=CARTESIAN_POINT('Ctrl Pts',(39.0538226985479,-40.3058120137285,2.));
#61413=CARTESIAN_POINT('Ctrl Pts',(39.0639271475071,-40.304991238701,2.));
#61414=CARTESIAN_POINT('Ctrl Pts',(39.0740116259566,-40.3040622329977,2.));
#61415=CARTESIAN_POINT('Ctrl Pts',(39.1295483097952,-40.2989460639973,2.));
#61416=CARTESIAN_POINT('Ctrl Pts',(39.1845546342683,-40.290546241389,2.));
#61417=CARTESIAN_POINT('Ctrl Pts',(39.2387593260286,-40.2787734967498,2.));
#61418=CARTESIAN_POINT('Ctrl Pts',(39.2750276515461,-40.2708963606396,2.));
#61419=CARTESIAN_POINT('Ctrl Pts',(39.3109369359741,-40.2615081906175,2.));
#61420=CARTESIAN_POINT('Ctrl Pts',(39.3464011448467,-40.2505700228958,2.));
#61421=CARTESIAN_POINT('Ctrl Pts',(39.3988910752724,-40.2343806398264,2.));
#61422=CARTESIAN_POINT('Ctrl Pts',(39.4504076476632,-40.2147967478769,2.));
#61423=CARTESIAN_POINT('Ctrl Pts',(39.5007091188364,-40.1920209197932,2.));
#61424=CARTESIAN_POINT('Ctrl Pts',(39.5162447294003,-40.1849866047498,2.));
#61425=CARTESIAN_POINT('Ctrl Pts',(39.5316641987863,-40.1776475888755,2.));
#61426=CARTESIAN_POINT('Ctrl Pts',(39.5469597255065,-40.1700092883085,2.));
#61427=CARTESIAN_POINT('Ctrl Pts',(39.5603821271819,-40.1633063914287,2.));
#61428=CARTESIAN_POINT('Ctrl Pts',(39.5737147687383,-40.1563697366024,2.));
#61429=CARTESIAN_POINT('Ctrl Pts',(39.5869207826454,-40.1492204403541,2.));
#61430=CARTESIAN_POINT('Ctrl Pts',(39.6358897832549,-40.1227102537983,2.));
#61431=CARTESIAN_POINT('Ctrl Pts',(39.6831882130913,-40.0932490202941,2.));
#61432=CARTESIAN_POINT('Ctrl Pts',(39.7285927500286,-40.0610855616068,2.));
#61433=CARTESIAN_POINT('Ctrl Pts',(39.7739426813493,-40.0289607841969,2.));
#61434=CARTESIAN_POINT('Ctrl Pts',(39.8174040328982,-39.9941393127207,2.));
#61435=CARTESIAN_POINT('Ctrl Pts',(39.8587164117551,-39.9568341504056,2.));
#61436=CARTESIAN_POINT('Ctrl Pts',(39.8851222214917,-39.9329896503903,2.));
#61437=CARTESIAN_POINT('Ctrl Pts',(39.9106492841583,-39.9081297964333,2.));
#61438=CARTESIAN_POINT('Ctrl Pts',(39.9352193294799,-39.8823054325727,2.));
#61439=CARTESIAN_POINT('Ctrl Pts',(39.9478799225961,-39.8689985070443,2.));
#61440=CARTESIAN_POINT('Ctrl Pts',(39.9602862681286,-39.8554354381392,2.));
#61441=CARTESIAN_POINT('Ctrl Pts',(39.9724266997057,-39.8416229521515,2.));
#61442=CARTESIAN_POINT('Ctrl Pts',(39.9797490690336,-39.8332921013825,2.));
#61443=CARTESIAN_POINT('Ctrl Pts',(39.9869741812514,-39.8248709352525,2.));
#61444=CARTESIAN_POINT('Ctrl Pts',(39.9940910777987,-39.8163713685009,2.));
#61445=CARTESIAN_POINT('Ctrl Pts',(40.0285072441014,-39.7752688316186,2.));
#61446=CARTESIAN_POINT('Ctrl Pts',(40.0604511582512,-39.7322729488107,2.));
#61447=CARTESIAN_POINT('Ctrl Pts',(40.0896714279617,-39.6875760500101,2.));
#61448=CARTESIAN_POINT('Ctrl Pts',(40.1080207191928,-39.6595079855692,2.));
#61449=CARTESIAN_POINT('Ctrl Pts',(40.1252950915591,-39.6307687140534,2.));
#61450=CARTESIAN_POINT('Ctrl Pts',(40.1414220409055,-39.6014032999083,2.));
#61451=CARTESIAN_POINT('Ctrl Pts',(40.1473185206864,-39.5906664539592,2.));
#61452=CARTESIAN_POINT('Ctrl Pts',(40.1530626681065,-39.5798436442736,2.));
#61453=CARTESIAN_POINT('Ctrl Pts',(40.1586468583821,-39.568944488148,2.));
#61454=CARTESIAN_POINT('Ctrl Pts',(40.1820879992589,-39.5231923483445,2.));
#61455=CARTESIAN_POINT('Ctrl Pts',(40.2026786417518,-39.4761684518135,2.));
#61456=CARTESIAN_POINT('Ctrl Pts',(40.2201722454891,-39.4280435373081,2.));
#61457=CARTESIAN_POINT('Ctrl Pts',(40.2299448374458,-39.4011591309003,2.));
#61458=CARTESIAN_POINT('Ctrl Pts',(40.238750054338,-39.3739309307312,2.));
#61459=CARTESIAN_POINT('Ctrl Pts',(40.2465377789655,-39.3463880711444,2.));
#61460=CARTESIAN_POINT('Ctrl Pts',(40.2520072382766,-39.3270442246388,2.));
#61461=CARTESIAN_POINT('Ctrl Pts',(40.2569746809644,-39.3075451531312,2.));
#61462=CARTESIAN_POINT('Ctrl Pts',(40.2614422049139,-39.2879094456029,2.));
#61463=CARTESIAN_POINT('Origin',(39.0658530619283,-38.8697713466883,4.5));
#61464=CARTESIAN_POINT('Origin',(-14.1292828945604,-53.2669068454841,6.));
#61465=CARTESIAN_POINT('Ctrl Pts',(-13.8936870225526,-54.5092654229862,
6.));
#61466=CARTESIAN_POINT('Ctrl Pts',(-13.9423636521357,-54.5241089051337,
6.));
#61467=CARTESIAN_POINT('Ctrl Pts',(-13.9918505584128,-54.5357341393499,
6.));
#61468=CARTESIAN_POINT('Ctrl Pts',(-14.0418694708007,-54.5442851897484,
6.));
#61469=CARTESIAN_POINT('Ctrl Pts',(-14.0755804158032,-54.5500482896627,
6.));
#61470=CARTESIAN_POINT('Ctrl Pts',(-14.1095337101414,-54.5544140915419,
6.));
#61471=CARTESIAN_POINT('Ctrl Pts',(-14.1436500643641,-54.5574153942333,
6.));
#61472=CARTESIAN_POINT('Ctrl Pts',(-14.1594122637946,-54.5588020351172,
6.));
#61473=CARTESIAN_POINT('Ctrl Pts',(-14.175209321514,-54.5598972886034,6.));
#61474=CARTESIAN_POINT('Ctrl Pts',(-14.1910336359969,-54.5607037375781,
6.));
#61475=CARTESIAN_POINT('Ctrl Pts',(-14.2042983435535,-54.561379742205,6.));
#61476=CARTESIAN_POINT('Ctrl Pts',(-14.2175747324108,-54.5618523554147,
6.));
#61477=CARTESIAN_POINT('Ctrl Pts',(-14.23085113108,-54.5621236288021,6.));
#61478=CARTESIAN_POINT('Ctrl Pts',(-14.2845943079494,-54.5632217499118,
6.));
#61479=CARTESIAN_POINT('Ctrl Pts',(-14.3383718685971,-54.5610264739157,
6.));
#61480=CARTESIAN_POINT('Ctrl Pts',(-14.3918835284745,-54.5556664140613,
6.));
#61481=CARTESIAN_POINT('Ctrl Pts',(-14.4123675638329,-54.5536146059913,
6.));
#61482=CARTESIAN_POINT('Ctrl Pts',(-14.4328128170871,-54.5510985259743,
6.));
#61483=CARTESIAN_POINT('Ctrl Pts',(-14.4532029278842,-54.5481234358992,
6.));
#61484=CARTESIAN_POINT('Ctrl Pts',(-14.4678705661439,-54.5459833030943,
6.));
#61485=CARTESIAN_POINT('Ctrl Pts',(-14.4825096747515,-54.5436056260969,
6.));
#61486=CARTESIAN_POINT('Ctrl Pts',(-14.4971141905477,-54.5409920215199,
6.));
#61487=CARTESIAN_POINT('Ctrl Pts',(-14.5083899394825,-54.5389741285999,
6.));
#61488=CARTESIAN_POINT('Ctrl Pts',(-14.5196453771421,-54.5368154090892,
6.));
#61489=CARTESIAN_POINT('Ctrl Pts',(-14.530862572558,-54.5345199552341,6.));
#61490=CARTESIAN_POINT('Ctrl Pts',(-14.5863736835655,-54.5231603248594,
6.));
#61491=CARTESIAN_POINT('Ctrl Pts',(-14.6410375587487,-54.50844123275,6.));
#61492=CARTESIAN_POINT('Ctrl Pts',(-14.6945239554116,-54.4905089639425,
6.));
#61493=CARTESIAN_POINT('Ctrl Pts',(-14.7472373377701,-54.4728358619729,
6.));
#61494=CARTESIAN_POINT('Ctrl Pts',(-14.7988082442548,-54.4520415391379,
6.));
#61495=CARTESIAN_POINT('Ctrl Pts',(-14.8489245845884,-54.428213079953,6.));
#61496=CARTESIAN_POINT('Ctrl Pts',(-14.8750932856906,-54.4157708341309,
6.));
#61497=CARTESIAN_POINT('Ctrl Pts',(-14.9008653565699,-54.4025004732343,
6.));
#61498=CARTESIAN_POINT('Ctrl Pts',(-14.9261951332699,-54.3884088626685,
6.));
#61499=CARTESIAN_POINT('Ctrl Pts',(-14.9397870442971,-54.3808473306696,
6.));
#61500=CARTESIAN_POINT('Ctrl Pts',(-14.9532515802469,-54.3730492659014,
6.));
#61501=CARTESIAN_POINT('Ctrl Pts',(-14.9665814892698,-54.365015287363,6.));
#61502=CARTESIAN_POINT('Ctrl Pts',(-14.9760605318105,-54.3593022382938,
6.));
#61503=CARTESIAN_POINT('Ctrl Pts',(-14.9854714934371,-54.3534698862629,
6.));
#61504=CARTESIAN_POINT('Ctrl Pts',(-14.9948117124905,-54.3475183599598,
6.));
#61505=CARTESIAN_POINT('Ctrl Pts',(-15.0030222328171,-54.3422866702739,
6.));
#61506=CARTESIAN_POINT('Ctrl Pts',(-15.0111697862519,-54.3369681733363,
6.));
#61507=CARTESIAN_POINT('Ctrl Pts',(-15.0192523731614,-54.331563816082,6.));
#61508=CARTESIAN_POINT('Ctrl Pts',(-15.0592738168887,-54.3048037970243,
6.));
#61509=CARTESIAN_POINT('Ctrl Pts',(-15.0977061906147,-54.2759385109371,
6.));
#61510=CARTESIAN_POINT('Ctrl Pts',(-15.1343580440251,-54.2450336527683,
6.));
#61511=CARTESIAN_POINT('Ctrl Pts',(-15.1760762697673,-54.2098568273243,
6.));
#61512=CARTESIAN_POINT('Ctrl Pts',(-15.2154892262361,-54.17203873631,6.));
#61513=CARTESIAN_POINT('Ctrl Pts',(-15.2525505184471,-54.1318952661582,
6.));
#61514=CARTESIAN_POINT('Ctrl Pts',(-15.2887783562999,-54.0926545640469,
6.));
#61515=CARTESIAN_POINT('Ctrl Pts',(-15.3227594146245,-54.0511910495941,
6.));
#61516=CARTESIAN_POINT('Ctrl Pts',(-15.3544244053254,-54.0077622836715,
6.));
#61517=CARTESIAN_POINT('Ctrl Pts',(-15.3621778074591,-53.9971284360401,
6.));
#61518=CARTESIAN_POINT('Ctrl Pts',(-15.3697922131958,-53.9863766151879,
6.));
#61519=CARTESIAN_POINT('Ctrl Pts',(-15.3772663285991,-53.975510336868,6.));
#61520=CARTESIAN_POINT('Ctrl Pts',(-15.3829111783894,-53.9673035450824,
6.));
#61521=CARTESIAN_POINT('Ctrl Pts',(-15.3884748239273,-53.9590330393209,
6.));
#61522=CARTESIAN_POINT('Ctrl Pts',(-15.3939506112134,-53.9507101506706,
6.));
#61523=CARTESIAN_POINT('Ctrl Pts',(-15.4256178027139,-53.9025778009366,
6.));
#61524=CARTESIAN_POINT('Ctrl Pts',(-15.4544095035981,-53.852609994368,6.));
#61525=CARTESIAN_POINT('Ctrl Pts',(-15.4802788953647,-53.8011564089965,
6.));
#61526=CARTESIAN_POINT('Ctrl Pts',(-15.5067035063538,-53.7485985062167,
6.));
#61527=CARTESIAN_POINT('Ctrl Pts',(-15.5300796467437,-53.6944895430076,
6.));
#61528=CARTESIAN_POINT('Ctrl Pts',(-15.5503219669977,-53.6391607087766,
6.));
#61529=CARTESIAN_POINT('Ctrl Pts',(-15.5707432288232,-53.5833427691257,
6.));
#61530=CARTESIAN_POINT('Ctrl Pts',(-15.5879756421218,-53.5262822854476,
6.));
#61531=CARTESIAN_POINT('Ctrl Pts',(-15.6018865037253,-53.4682915822501,
6.));
#61532=CARTESIAN_POINT('Ctrl Pts',(-15.6050386064326,-53.4551512996596,
6.));
#61533=CARTESIAN_POINT('Ctrl Pts',(-15.6080206160618,-53.4419594370913,
6.));
#61534=CARTESIAN_POINT('Ctrl Pts',(-15.6108253927011,-53.4287461304568,
6.));
#61535=CARTESIAN_POINT('Ctrl Pts',(-15.6234580838913,-53.3692335047533,
6.));
#61536=CARTESIAN_POINT('Ctrl Pts',(-15.6325248597527,-53.3091883987973,
6.));
#61537=CARTESIAN_POINT('Ctrl Pts',(-15.6379479683267,-53.2489633020354,
6.));
#61538=CARTESIAN_POINT('Ctrl Pts',(-15.6433234244293,-53.1892673989372,
6.));
#61539=CARTESIAN_POINT('Ctrl Pts',(-15.6451194085378,-53.1293935642286,
6.));
#61540=CARTESIAN_POINT('Ctrl Pts',(-15.6432152689538,-53.0696627698792,
6.));
#61541=CARTESIAN_POINT('Ctrl Pts',(-15.6418200559649,-53.0258964510577,
6.));
#61542=CARTESIAN_POINT('Ctrl Pts',(-15.6384374018706,-52.9822063985564,
6.));
#61543=CARTESIAN_POINT('Ctrl Pts',(-15.6330021738796,-52.9387162761377,
6.));
#61544=CARTESIAN_POINT('Ctrl Pts',(-15.6299816095937,-52.9145471500616,
6.));
#61545=CARTESIAN_POINT('Ctrl Pts',(-15.626326826898,-52.8904397607359,6.));
#61546=CARTESIAN_POINT('Ctrl Pts',(-15.6220514315181,-52.8664094746825,
6.));
#61547=CARTESIAN_POINT('Ctrl Pts',(-15.2209662466057,-52.1764590205668,
6.));
#61548=CARTESIAN_POINT('Ctrl Pts',(-15.1741443796226,-52.1372711016556,
6.));
#61549=CARTESIAN_POINT('Ctrl Pts',(-15.1249225029807,-52.1011828129763,
6.));
#61550=CARTESIAN_POINT('Ctrl Pts',(-15.0736468678487,-52.0682420900143,
6.));
#61551=CARTESIAN_POINT('Ctrl Pts',(-15.0261004125905,-52.0376970834737,
6.));
#61552=CARTESIAN_POINT('Ctrl Pts',(-14.9767869967238,-52.0098588542083,
6.));
#61553=CARTESIAN_POINT('Ctrl Pts',(-14.9259704605544,-51.9848043154143,
6.));
#61554=CARTESIAN_POINT('Ctrl Pts',(-14.9137051793402,-51.9787570523153,
6.));
#61555=CARTESIAN_POINT('Ctrl Pts',(-14.9013518482974,-51.9728720566067,
6.));
#61556=CARTESIAN_POINT('Ctrl Pts',(-14.8889282287138,-51.9671568052641,
6.));
#61557=CARTESIAN_POINT('Ctrl Pts',(-14.8342503521426,-51.9420032817374,
6.));
#61558=CARTESIAN_POINT('Ctrl Pts',(-14.7781470458952,-51.9201009097871,
6.));
#61559=CARTESIAN_POINT('Ctrl Pts',(-14.7209451681374,-51.9015259517645,
6.));
#61560=CARTESIAN_POINT('Ctrl Pts',(-14.6856380616414,-51.8900608032978,
6.));
#61561=CARTESIAN_POINT('Ctrl Pts',(-14.6499121652624,-51.8798643401128,
6.));
#61562=CARTESIAN_POINT('Ctrl Pts',(-14.6138441165377,-51.8709644321812,
6.));
#61563=CARTESIAN_POINT('Ctrl Pts',(-14.6015017900197,-51.8679189231072,
6.));
#61564=CARTESIAN_POINT('Ctrl Pts',(-14.5891194062045,-51.8650253041639,
6.));
#61565=CARTESIAN_POINT('Ctrl Pts',(-14.5767000721463,-51.8622849004515,
6.));
#61566=CARTESIAN_POINT('Ctrl Pts',(-14.5650829788742,-51.8597215161847,
6.));
#61567=CARTESIAN_POINT('Ctrl Pts',(-14.5534409513892,-51.8572938728812,
6.));
#61568=CARTESIAN_POINT('Ctrl Pts',(-14.5417825459458,-51.8550036366081,
6.));
#61569=CARTESIAN_POINT('Ctrl Pts',(-14.4840742559295,-51.843667127538,6.));
#61570=CARTESIAN_POINT('Ctrl Pts',(-14.4259183529299,-51.8356828275257,
6.));
#61571=CARTESIAN_POINT('Ctrl Pts',(-14.367620963232,-51.8311224894044,6.));
#61572=CARTESIAN_POINT('Ctrl Pts',(-14.3108124222532,-51.8266786171078,
6.));
#61573=CARTESIAN_POINT('Ctrl Pts',(-14.2538685532984,-51.8254861890658,
6.));
#61574=CARTESIAN_POINT('Ctrl Pts',(-14.1970797852011,-51.8276601888203,
6.));
#61575=CARTESIAN_POINT('Ctrl Pts',(-14.1662905485282,-51.8288388689574,
6.));
#61576=CARTESIAN_POINT('Ctrl Pts',(-14.1355471145905,-51.8310079452929,
6.));
#61577=CARTESIAN_POINT('Ctrl Pts',(-14.1048981745618,-51.8341917567471,
6.));
#61578=CARTESIAN_POINT('Ctrl Pts',(-14.0793989212455,-51.8368406188189,
6.));
#61579=CARTESIAN_POINT('Ctrl Pts',(-14.0539650962438,-51.8401919425301,
6.));
#61580=CARTESIAN_POINT('Ctrl Pts',(-14.0286260526481,-51.8442620101075,
6.));
#61581=CARTESIAN_POINT('Ctrl Pts',(-14.0177944478155,-51.846001829666,6.));
#61582=CARTESIAN_POINT('Ctrl Pts',(-14.0069789239642,-51.8478733580626,
6.));
#61583=CARTESIAN_POINT('Ctrl Pts',(-13.996199334982,-51.8498743912714,6.));
#61584=CARTESIAN_POINT('Ctrl Pts',(-13.9463007654824,-51.8591371465399,
6.));
#61585=CARTESIAN_POINT('Ctrl Pts',(-13.8970847123908,-51.8711850123186,
6.));
#61586=CARTESIAN_POINT('Ctrl Pts',(-13.8487579820866,-51.8860904144816,
6.));
#61587=CARTESIAN_POINT('Ctrl Pts',(-13.7947539043117,-51.9027468796016,
6.));
#61588=CARTESIAN_POINT('Ctrl Pts',(-13.7418592133642,-51.9229715823675,
6.));
#61589=CARTESIAN_POINT('Ctrl Pts',(-13.6903202642367,-51.9465184249238,
6.));
#61590=CARTESIAN_POINT('Ctrl Pts',(-13.6465843618314,-51.9665002527537,
6.));
#61591=CARTESIAN_POINT('Ctrl Pts',(-13.6038249088342,-51.9888755884466,
6.));
#61592=CARTESIAN_POINT('Ctrl Pts',(-13.562213300163,-52.0135148505948,6.));
#61593=CARTESIAN_POINT('Ctrl Pts',(-13.5507734482976,-52.0202886696816,
6.));
#61594=CARTESIAN_POINT('Ctrl Pts',(-13.5394204822292,-52.0272336869077,
6.));
#61595=CARTESIAN_POINT('Ctrl Pts',(-13.5281582767465,-52.0343473928026,
6.));
#61596=CARTESIAN_POINT('Ctrl Pts',(-13.519389840783,-52.0398859238388,6.));
#61597=CARTESIAN_POINT('Ctrl Pts',(-13.5106749801112,-52.0455277717095,
6.));
#61598=CARTESIAN_POINT('Ctrl Pts',(-13.5020295300328,-52.0512622211197,
6.));
#61599=CARTESIAN_POINT('Ctrl Pts',(-13.4557689093827,-52.0819464754268,
6.));
#61600=CARTESIAN_POINT('Ctrl Pts',(-13.4114050031948,-52.1153327757811,
6.));
#61601=CARTESIAN_POINT('Ctrl Pts',(-13.3691631578584,-52.1511816195792,
6.));
#61602=CARTESIAN_POINT('Ctrl Pts',(-13.3271578443737,-52.1868297289317,
6.));
#61603=CARTESIAN_POINT('Ctrl Pts',(-13.2872501901036,-52.2249138499118,
6.));
#61604=CARTESIAN_POINT('Ctrl Pts',(-13.2497024980977,-52.2652291266103,
6.));
#61605=CARTESIAN_POINT('Ctrl Pts',(-13.2148651399623,-52.3026342947483,
6.));
#61606=CARTESIAN_POINT('Ctrl Pts',(-13.1820592966373,-52.3419610028466,
6.));
#61607=CARTESIAN_POINT('Ctrl Pts',(-13.1515339537958,-52.3830588008458,
6.));
#61608=CARTESIAN_POINT('Ctrl Pts',(-13.1436930287938,-52.3936154309067,
6.));
#61609=CARTESIAN_POINT('Ctrl Pts',(-13.1360003096902,-52.404292764071,6.));
#61610=CARTESIAN_POINT('Ctrl Pts',(-13.1284766278539,-52.415064415478,6.));
#61611=CARTESIAN_POINT('Ctrl Pts',(-13.09806445529,-52.4586055072624,6.));
#61612=CARTESIAN_POINT('Ctrl Pts',(-13.0703588458369,-52.5037520470482,
6.));
#61613=CARTESIAN_POINT('Ctrl Pts',(-13.0455900654096,-52.5503113513571,
6.));
#61614=CARTESIAN_POINT('Ctrl Pts',(-13.0216615115111,-52.595291233427,6.));
#61615=CARTESIAN_POINT('Ctrl Pts',(-13.0004736387158,-52.6415904794481,
6.));
#61616=CARTESIAN_POINT('Ctrl Pts',(-12.9822803194866,-52.6890470685693,
6.));
#61617=CARTESIAN_POINT('Ctrl Pts',(-12.9695523308543,-52.7222475483307,
6.));
#61618=CARTESIAN_POINT('Ctrl Pts',(-12.9582909257562,-52.7560147190405,
6.));
#61619=CARTESIAN_POINT('Ctrl Pts',(-12.9485983183411,-52.7902936156639,
6.));
#61620=CARTESIAN_POINT('Ctrl Pts',(-12.9431308250061,-52.8096299645733,
6.));
#61621=CARTESIAN_POINT('Ctrl Pts',(-12.9381627931205,-52.8291291517901,
6.));
#61622=CARTESIAN_POINT('Ctrl Pts',(-12.9336933707122,-52.8487726938777,
6.));
#61623=CARTESIAN_POINT('Origin',(-14.1292828945604,-53.2669068454841,0.895788276411274));
#61624=CARTESIAN_POINT('Ctrl Pts',(-14.9010809748678,-54.6051974101417,
2.14578827641127));
#61625=CARTESIAN_POINT('Ctrl Pts',(-14.8597272487244,-54.6294211798578,
2.14826884812012));
#61626=CARTESIAN_POINT('Ctrl Pts',(-14.3688277705329,-54.885598628679,2.17691792328789));
#61627=CARTESIAN_POINT('Ctrl Pts',(-13.1694755608909,-54.8098887390119,
2.23173550191459));
#61628=CARTESIAN_POINT('Ctrl Pts',(-12.3130077055018,-53.3174154968918,
2.31024101229136));
#61629=CARTESIAN_POINT('Ctrl Pts',(-13.0852322400692,-51.7797767714816,
2.38874652266815));
#61630=CARTESIAN_POINT('Ctrl Pts',(-14.7938791388703,-51.5757659053288,
2.46725203304492));
#61631=CARTESIAN_POINT('Ctrl Pts',(-15.9064540032169,-52.8884432158558,
2.5457575434217));
#61632=CARTESIAN_POINT('Ctrl Pts',(-15.5416657446855,-54.1408201433548,
2.60526962454382));
#61633=CARTESIAN_POINT('Ctrl Pts',(-15.0227829664514,-54.5334351262247,
2.63861320220701));
#61634=CARTESIAN_POINT('Ctrl Pts',(-14.9016274172746,-54.6020379108679,
2.64578827641127));
#61635=CARTESIAN_POINT('Ctrl Pts',(-14.9013089558621,-54.6009691165979,
2.10421172358873));
#61636=CARTESIAN_POINT('Ctrl Pts',(-14.6040162957702,-54.7699114721225,
2.12181148931034));
#61637=CARTESIAN_POINT('Ctrl Pts',(-13.7242010739632,-54.9558633776928,
2.16557975849087));
#61638=CARTESIAN_POINT('Ctrl Pts',(-12.4888977717378,-54.0475500892828,
2.23551653113034));
#61639=CARTESIAN_POINT('Ctrl Pts',(-12.5727324025626,-52.3295818538895,
2.31402204150712));
#61640=CARTESIAN_POINT('Ctrl Pts',(-14.0528383317196,-51.4513683986095,
2.3925275518839));
#61641=CARTESIAN_POINT('Ctrl Pts',(-15.6013423678816,-52.2018016959779,
2.47103306226067));
#61642=CARTESIAN_POINT('Ctrl Pts',(-15.8066350265236,-53.7346571674393,
2.54159445282895));
#61643=CARTESIAN_POINT('Ctrl Pts',(-15.2043102739953,-54.4236472184416,
2.5859873399383));
#61644=CARTESIAN_POINT('Ctrl Pts',(-14.8992309062956,-54.6029598038327,
2.60421172358873));
#61645=CARTESIAN_POINT('Ctrl Pts',(-12.9355708698302,-52.8497595669186,
2.));
#61646=CARTESIAN_POINT('Ctrl Pts',(-13.0727468794465,-52.4572155888145,
2.02616850345893));
#61647=CARTESIAN_POINT('Ctrl Pts',(-13.762195269905,-51.8244143348175,2.07850551037678));
#61648=CARTESIAN_POINT('Ctrl Pts',(-15.132331970736,-52.1652352880051,2.15701102075356));
#61649=CARTESIAN_POINT('Ctrl Pts',(-15.600345878683,-53.4958301810381,2.23551653113034));
#61650=CARTESIAN_POINT('Ctrl Pts',(-14.7503158422929,-54.6202478137908,
2.31402204150712));
#61651=CARTESIAN_POINT('Ctrl Pts',(-13.3427136311611,-54.5313920070952,
2.3925275518839));
#61652=CARTESIAN_POINT('Ctrl Pts',(-12.6408318404032,-53.3082990617544,
2.47103306226068));
#61653=CARTESIAN_POINT('Ctrl Pts',(-13.2736756018811,-52.0481926662385,
2.54953857263745));
#61654=CARTESIAN_POINT('Ctrl Pts',(-14.6739244700172,-51.8810042409304,
2.62804408301423));
#61655=CARTESIAN_POINT('Ctrl Pts',(-15.5856878633849,-52.9567530803092,
2.70654959339101));
#61656=CARTESIAN_POINT('Ctrl Pts',(-15.191331582231,-54.3106417984376,2.78505510376779));
#61657=CARTESIAN_POINT('Ctrl Pts',(-13.8444953540085,-54.7284908735361,
2.86356061414457));
#61658=CARTESIAN_POINT('Ctrl Pts',(-12.7530680664413,-53.8355533167568,
2.94206612452135));
#61659=CARTESIAN_POINT('Ctrl Pts',(-12.8958606092946,-52.4326417450687,
3.02057163489813));
#61660=CARTESIAN_POINT('Ctrl Pts',(-14.1448167496288,-51.7779181217065,
3.09907714527491));
#61661=CARTESIAN_POINT('Ctrl Pts',(-15.3798411765859,-52.4585553969251,
3.17758265565169));
#61662=CARTESIAN_POINT('Ctrl Pts',(-15.4933354964796,-53.86414126306,3.25608816602848));
#61663=CARTESIAN_POINT('Ctrl Pts',(-14.3835148696119,-54.7341132075812,
3.33459367640524));
#61664=CARTESIAN_POINT('Ctrl Pts',(-13.0456930357207,-54.2882595546367,
3.41309918678203));
#61665=CARTESIAN_POINT('Ctrl Pts',(-12.6796603121052,-52.9264325363301,
3.49160469715881));
#61666=CARTESIAN_POINT('Ctrl Pts',(-13.6136836011906,-51.8699509600852,
3.57011020753559));
#61667=CARTESIAN_POINT('Ctrl Pts',(-15.0101085852912,-52.066292638923,3.64861571791237));
#61668=CARTESIAN_POINT('Ctrl Pts',(-15.6165881539764,-53.3393736780174,
3.72712122828915));
#61669=CARTESIAN_POINT('Ctrl Pts',(-14.8892170051293,-54.5474647404685,
3.80562673866593));
#61670=CARTESIAN_POINT('Ctrl Pts',(-13.4803188806439,-54.6071210383936,
3.88413224904271));
#61671=CARTESIAN_POINT('Ctrl Pts',(-12.6534271115016,-53.4648413867365,
3.96263775941949));
#61672=CARTESIAN_POINT('Ctrl Pts',(-13.1501178953861,-52.1450493326719,
4.04114326979627));
#61673=CARTESIAN_POINT('Ctrl Pts',(-14.5249471286252,-51.8313657668163,
4.11964878017305));
#61674=CARTESIAN_POINT('Ctrl Pts',(-15.5449352706108,-52.805109568325,4.19815429054982));
#61675=CARTESIAN_POINT('Ctrl Pts',(-15.2953327061785,-54.1930041465599,
4.2766598009266));
#61676=CARTESIAN_POINT('Ctrl Pts',(-13.9999889501244,-54.7503526485876,
4.35516531130338));
#61677=CARTESIAN_POINT('Ctrl Pts',(-12.8205990758801,-53.977311687267,4.43367082168017));
#61678=CARTESIAN_POINT('Ctrl Pts',(-12.8148679650961,-52.5671627753774,
4.51217633205694));
#61679=CARTESIAN_POINT('Ctrl Pts',(-13.9879354060905,-51.7845609801147,
4.59068184243372));
#61680=CARTESIAN_POINT('Ctrl Pts',(-15.2877666458998,-52.3313621994943,
4.6691873528105));
#61681=CARTESIAN_POINT('Ctrl Pts',(-15.5486420944497,-53.7171820950401,
4.74769286318728));
#61682=CARTESIAN_POINT('Ctrl Pts',(-14.5366025126985,-54.6991844494411,
4.82619837356406));
#61683=CARTESIAN_POINT('Ctrl Pts',(-13.1592689266914,-54.396686183443,4.90470388394084));
#61684=CARTESIAN_POINT('Ctrl Pts',(-12.651867102821,-53.0809749777224,4.98320939431762));
#61685=CARTESIAN_POINT('Ctrl Pts',(-13.4694465335298,-51.9320118320645,
5.0617149046944));
#61686=CARTESIAN_POINT('Ctrl Pts',(-14.8787836035794,-51.9802143885461,
5.14022041507118));
#61687=CARTESIAN_POINT('Ctrl Pts',(-15.6159492071913,-53.1823530914927,
5.21872592544796));
#61688=CARTESIAN_POINT('Ctrl Pts',(-15.0198399508834,-54.4603220891204,
5.29723143582474));
#61689=CARTESIAN_POINT('Ctrl Pts',(-13.6250522726906,-54.6680069657355,
5.37573694620152));
#61690=CARTESIAN_POINT('Ctrl Pts',(-12.6824820007894,-53.6191538682575,
5.45424245657829));
#61691=CARTESIAN_POINT('Ctrl Pts',(-13.0374143051107,-52.2543934093274,
5.53274796695507));
#61692=CARTESIAN_POINT('Ctrl Pts',(-14.3716061738679,-51.7976868080881,
5.61125347733185));
#61693=CARTESIAN_POINT('Ctrl Pts',(-15.4883847851255,-52.6585961458811,
5.68975898770864));
#61694=CARTESIAN_POINT('Ctrl Pts',(-15.3864730097086,-54.0650841092748,
5.76826449808541));
#61695=CARTESIAN_POINT('Ctrl Pts',(-14.156713139869,-54.7556852978769,5.8467700084622));
#61696=CARTESIAN_POINT('Ctrl Pts',(-12.9030960095782,-54.1112396708051,
5.92527551883897));
#61697=CARTESIAN_POINT('Ctrl Pts',(-12.747656043165,-52.7093273325191,6.00378102921575));
#61698=CARTESIAN_POINT('Ctrl Pts',(-13.8343697837273,-51.8079468650312,
6.08228653959253));
#61699=CARTESIAN_POINT('Ctrl Pts',(-14.7300614275788,-52.0790796540862,
6.13462354651038));
#61700=CARTESIAN_POINT('Ctrl Pts',(-15.0239255378924,-52.3732767258419,
6.16079204996931));
#61701=CARTESIAN_POINT('Ctrl Pts',(-12.8479344393867,-52.8191346777449,
1.94640265001023));
#61702=CARTESIAN_POINT('Ctrl Pts',(-12.9951812328907,-52.3977720630513,
1.97257115346916));
#61703=CARTESIAN_POINT('Ctrl Pts',(-13.7352455128293,-51.7185136720468,
2.02490816038701));
#61704=CARTESIAN_POINT('Ctrl Pts',(-15.2059708708849,-52.0843560132568,
2.10341367076379));
#61705=CARTESIAN_POINT('Ctrl Pts',(-15.7083440442499,-53.5126365996361,
2.18191918114057));
#61706=CARTESIAN_POINT('Ctrl Pts',(-14.7959090084834,-54.7196034114377,
2.26042469151735));
#61707=CARTESIAN_POINT('Ctrl Pts',(-13.2849676077377,-54.6242242510674,
2.33893020189413));
#61708=CARTESIAN_POINT('Ctrl Pts',(-12.5315571287694,-53.3113378734669,
2.41743571227091));
#61709=CARTESIAN_POINT('Ctrl Pts',(-13.2108611479438,-51.9587207013195,
2.49594122264769));
#61710=CARTESIAN_POINT('Ctrl Pts',(-14.7139093596349,-51.7792581290633,
2.57444673302446));
#61711=CARTESIAN_POINT('Ctrl Pts',(-15.6926099099956,-52.9339831254913,
2.65295224340125));
#61712=CARTESIAN_POINT('Ctrl Pts',(-15.2693019419295,-54.3872676543484,
2.73145775377802));
#61713=CARTESIAN_POINT('Ctrl Pts',(-13.8235876618921,-54.8357931410496,
2.80996326415481));
#61714=CARTESIAN_POINT('Ctrl Pts',(-12.6520331831854,-53.8773005270505,
2.88846877453158));
#61715=CARTESIAN_POINT('Ctrl Pts',(-12.8053088480064,-52.3713941292876,
2.96697428490836));
#61716=CARTESIAN_POINT('Ctrl Pts',(-14.1459571684074,-51.6686039370295,
3.04547979528514));
#61717=CARTESIAN_POINT('Ctrl Pts',(-15.4716509779683,-52.3992102332442,
3.12398530566192));
#61718=CARTESIAN_POINT('Ctrl Pts',(-15.5934774892658,-53.90798725892,3.2024908160387));
#61719=CARTESIAN_POINT('Ctrl Pts',(-14.4021793232963,-54.8418282390413,
3.28099632641548));
#61720=CARTESIAN_POINT('Ctrl Pts',(-12.9661412298193,-54.3632422169535,
3.35950183679226));
#61721=CARTESIAN_POINT('Ctrl Pts',(-12.5732361947429,-52.9014365971976,
3.43800734716904));
#61722=CARTESIAN_POINT('Ctrl Pts',(-13.5758308522243,-51.7673933710292,
3.51651285754582));
#61723=CARTESIAN_POINT('Ctrl Pts',(-15.0747744492345,-51.9781494844411,
3.5950183679226));
#61724=CARTESIAN_POINT('Ctrl Pts',(-15.7257787470295,-53.3446938343006,
3.67352387829938));
#61725=CARTESIAN_POINT('Ctrl Pts',(-14.945007607421,-54.6414769649982,3.75202938867616));
#61726=CARTESIAN_POINT('Ctrl Pts',(-13.4326751537753,-54.7055129331413,
3.83053489905294));
#61727=CARTESIAN_POINT('Ctrl Pts',(-12.5450770823513,-53.4793727613876,
3.90904040942971));
#61728=CARTESIAN_POINT('Ctrl Pts',(-13.0782324459937,-52.0626881049618,
3.9875459198065));
#61729=CARTESIAN_POINT('Ctrl Pts',(-14.5539948389685,-51.7259754437876,
4.06605143018328));
#61730=CARTESIAN_POINT('Ctrl Pts',(-15.6488654635013,-52.77120669718,4.14455694056005));
#61731=CARTESIAN_POINT('Ctrl Pts',(-15.3809383138062,-54.2609936281335,
4.22306245093684));
#61732=CARTESIAN_POINT('Ctrl Pts',(-13.9904968284622,-54.8592598994547,
4.30156796131361));
#61733=CARTESIAN_POINT('Ctrl Pts',(-12.7245219851981,-54.0294660957121,
4.3800734716904));
#61734=CARTESIAN_POINT('Ctrl Pts',(-12.7183701246174,-52.5157910280399,
4.45857898206717));
#61735=CARTESIAN_POINT('Ctrl Pts',(-13.9775583728655,-51.6757344812337,
4.53708449244395));
#61736=CARTESIAN_POINT('Ctrl Pts',(-15.3728167908182,-52.2626791406019,
4.61559000282073));
#61737=CARTESIAN_POINT('Ctrl Pts',(-15.6528444240053,-53.7502390759288,
4.69409551319751));
#61738=CARTESIAN_POINT('Ctrl Pts',(-14.5665059036703,-54.8043351843038,
4.77260102357429));
#61739=CARTESIAN_POINT('Ctrl Pts',(-13.0880553007387,-54.4796289923587,
4.85110653395107));
#61740=CARTESIAN_POINT('Ctrl Pts',(-12.5434025455522,-53.0673247799705,
4.92961204432785));
#61741=CARTESIAN_POINT('Ctrl Pts',(-13.4210046127319,-51.8340104451561,
5.00811755470463));
#61742=CARTESIAN_POINT('Ctrl Pts',(-14.9338082371531,-51.8857517948312,
5.08662306508141));
#61743=CARTESIAN_POINT('Ctrl Pts',(-15.725092891933,-53.1761455732413,5.16512857545819));
#61744=CARTESIAN_POINT('Ctrl Pts',(-15.0852202435382,-54.5479367313644,
5.24363408583496));
#61745=CARTESIAN_POINT('Ctrl Pts',(-13.5880341553344,-54.7708688040089,
5.32213959621175));
#61746=CARTESIAN_POINT('Ctrl Pts',(-12.5762650378488,-53.6450141017733,
5.40064510658852));
#61747=CARTESIAN_POINT('Ctrl Pts',(-12.9572547157706,-52.1800596826976,
5.47915061696531));
#61748=CARTESIAN_POINT('Ctrl Pts',(-14.3893963500343,-51.689823942551,5.55765612734208));
#61749=CARTESIAN_POINT('Ctrl Pts',(-15.58816332118,-52.6139369841994,5.63616163771886));
#61750=CARTESIAN_POINT('Ctrl Pts',(-15.478769687465,-54.1236823346513,5.71466714809565));
#61751=CARTESIAN_POINT('Ctrl Pts',(-14.1587269327564,-54.8649840454692,
5.79317265847243));
#61752=CARTESIAN_POINT('Ctrl Pts',(-12.8130754355786,-54.1732264091344,
5.8716781688492));
#61753=CARTESIAN_POINT('Ctrl Pts',(-12.6462238359385,-52.6683926035455,
5.95018367922599));
#61754=CARTESIAN_POINT('Ctrl Pts',(-13.8127187223415,-51.7008372421089,
6.02868918960276));
#61755=CARTESIAN_POINT('Ctrl Pts',(-14.7741676148585,-51.9918752589882,
6.08102619652061));
#61756=CARTESIAN_POINT('Ctrl Pts',(-15.0896057741302,-52.3076708240835,
6.10719469997954));
#61757=CARTESIAN_POINT('Ctrl Pts',(-12.7602980089432,-52.7885097885712,
1.89280530002046));
#61758=CARTESIAN_POINT('Ctrl Pts',(-12.917615586335,-52.3383285372882,1.91897380347939));
#61759=CARTESIAN_POINT('Ctrl Pts',(-13.7082957557537,-51.6126130092761,
1.97131081039724));
#61760=CARTESIAN_POINT('Ctrl Pts',(-15.2796097710338,-52.0034767385084,
2.04981632077402));
#61761=CARTESIAN_POINT('Ctrl Pts',(-15.8163422098168,-53.5294430182342,
2.1283218311508));
#61762=CARTESIAN_POINT('Ctrl Pts',(-14.8415021746739,-54.8189590090846,
2.20682734152758));
#61763=CARTESIAN_POINT('Ctrl Pts',(-13.2272215843143,-54.7170564950396,
2.28533285190436));
#61764=CARTESIAN_POINT('Ctrl Pts',(-12.4222824171356,-53.3143766851794,
2.36383836228113));
#61765=CARTESIAN_POINT('Ctrl Pts',(-13.1480466940065,-51.8692487364006,
2.44234387265792));
#61766=CARTESIAN_POINT('Ctrl Pts',(-14.7538942492526,-51.677512017196,2.52084938303469));
#61767=CARTESIAN_POINT('Ctrl Pts',(-15.7995319566062,-52.9112131706736,
2.59935489341148));
#61768=CARTESIAN_POINT('Ctrl Pts',(-15.347272301628,-54.4638935102592,2.67786040378825));
#61769=CARTESIAN_POINT('Ctrl Pts',(-13.8026799697757,-54.9430954085631,
2.75636591416504));
#61770=CARTESIAN_POINT('Ctrl Pts',(-12.5509982999295,-53.9190477373443,
2.83487142454181));
#61771=CARTESIAN_POINT('Ctrl Pts',(-12.7147570867183,-52.3101465135064,
2.91337693491859));
#61772=CARTESIAN_POINT('Ctrl Pts',(-14.147097587186,-51.5592897523525,2.99188244529537));
#61773=CARTESIAN_POINT('Ctrl Pts',(-15.5634607793507,-52.3398650695632,
3.07038795567215));
#61774=CARTESIAN_POINT('Ctrl Pts',(-15.693619482052,-53.9518332547799,3.14889346604893));
#61775=CARTESIAN_POINT('Ctrl Pts',(-14.4208437769808,-54.9495432705015,
3.22739897642571));
#61776=CARTESIAN_POINT('Ctrl Pts',(-12.886589423918,-54.4382248792703,3.30590448680249));
#61777=CARTESIAN_POINT('Ctrl Pts',(-12.4668120773806,-52.876440658065,3.38440999717927));
#61778=CARTESIAN_POINT('Ctrl Pts',(-13.5379781032581,-51.6648357819733,
3.46291550755605));
#61779=CARTESIAN_POINT('Ctrl Pts',(-15.1394403131777,-51.8900063299591,
3.54142101793283));
#61780=CARTESIAN_POINT('Ctrl Pts',(-15.8349693400828,-53.3500139905838,
3.61992652830961));
#61781=CARTESIAN_POINT('Ctrl Pts',(-15.0007982097127,-54.7354891895279,
3.69843203868639));
#61782=CARTESIAN_POINT('Ctrl Pts',(-13.3850314269068,-54.8039048278889,
3.77693754906317));
#61783=CARTESIAN_POINT('Ctrl Pts',(-12.4367270532009,-53.4939041360386,
3.85544305943994));
#61784=CARTESIAN_POINT('Ctrl Pts',(-13.0063469966013,-51.9803268772517,
3.93394856981673));
#61785=CARTESIAN_POINT('Ctrl Pts',(-14.5830425493117,-51.6205851207591,
4.01245408019351));
#61786=CARTESIAN_POINT('Ctrl Pts',(-15.7527956563917,-52.7373038260349,
4.09095959057028));
#61787=CARTESIAN_POINT('Ctrl Pts',(-15.4665439214339,-54.3289831097072,
4.16946510094706));
#61788=CARTESIAN_POINT('Ctrl Pts',(-13.9810047068001,-54.9681671503218,
4.24797061132384));
#61789=CARTESIAN_POINT('Ctrl Pts',(-12.628444894516,-54.0816205041571,4.32647612170062));
#61790=CARTESIAN_POINT('Ctrl Pts',(-12.6218722841388,-52.4644192807025,
4.4049816320774));
#61791=CARTESIAN_POINT('Ctrl Pts',(-13.9671813396406,-51.5669079823526,
4.48348714245418));
#61792=CARTESIAN_POINT('Ctrl Pts',(-15.4578669357366,-52.1939960817095,
4.56199265283096));
#61793=CARTESIAN_POINT('Ctrl Pts',(-15.7570467535609,-53.7832960568175,
4.64049816320773));
#61794=CARTESIAN_POINT('Ctrl Pts',(-14.5964092946421,-54.9094859191667,
4.71900367358452));
#61795=CARTESIAN_POINT('Ctrl Pts',(-13.016841674786,-54.5625718012743,4.7975091839613));
#61796=CARTESIAN_POINT('Ctrl Pts',(-12.4349379882833,-53.0536745822187,
4.87601469433808));
#61797=CARTESIAN_POINT('Ctrl Pts',(-13.3725626919339,-51.7360090582476,
4.95452020471486));
#61798=CARTESIAN_POINT('Ctrl Pts',(-14.9888328707268,-51.7912892011163,
5.03302571509164));
#61799=CARTESIAN_POINT('Ctrl Pts',(-15.8342365766747,-53.16993805499,5.11153122546842));
#61800=CARTESIAN_POINT('Ctrl Pts',(-15.1506005361929,-54.6355513736084,
5.1900367358452));
#61801=CARTESIAN_POINT('Ctrl Pts',(-13.5510160379782,-54.8737306422823,
5.26854224622197));
#61802=CARTESIAN_POINT('Ctrl Pts',(-12.4700480749082,-53.6708743352892,
5.34704775659876));
#61803=CARTESIAN_POINT('Ctrl Pts',(-12.8770951264305,-52.105725956068,5.42555326697553));
#61804=CARTESIAN_POINT('Ctrl Pts',(-14.4071865262006,-51.581961077014,5.50405877735231));
#61805=CARTESIAN_POINT('Ctrl Pts',(-15.6879418572343,-52.5692778225178,
5.58256428772909));
#61806=CARTESIAN_POINT('Ctrl Pts',(-15.5710663652214,-54.1822805600277,
5.66106979810588));
#61807=CARTESIAN_POINT('Ctrl Pts',(-14.1607407256438,-54.9742827930615,
5.73957530848265));
#61808=CARTESIAN_POINT('Ctrl Pts',(-12.7230548615789,-54.2352131474636,
5.81808081885943));
#61809=CARTESIAN_POINT('Ctrl Pts',(-12.544791628712,-52.6274578745722,5.89658632923621));
#61810=CARTESIAN_POINT('Ctrl Pts',(-13.7910676609558,-51.5937276191864,
5.97509183961299));
#61811=CARTESIAN_POINT('Ctrl Pts',(-14.8182738021382,-51.9046708638902,
6.02742884653084));
#61812=CARTESIAN_POINT('Ctrl Pts',(-15.1552860103679,-52.2420649223251,
6.05359734998977));
#61813=CARTESIAN_POINT('Ctrl Pts',(-12.6726615784998,-52.7578848993974,
1.83920795003069));
#61814=CARTESIAN_POINT('Ctrl Pts',(-12.8400499397792,-52.278885011525,1.86537645348962));
#61815=CARTESIAN_POINT('Ctrl Pts',(-13.681345998678,-51.5067123465054,1.91771346040747));
#61816=CARTESIAN_POINT('Ctrl Pts',(-15.3532486711827,-51.92259746376,1.99621897078425));
#61817=CARTESIAN_POINT('Ctrl Pts',(-15.9243403753837,-53.5462494368323,
2.07472448116103));
#61818=CARTESIAN_POINT('Ctrl Pts',(-14.8870953408643,-54.9183146067314,
2.15322999153781));
#61819=CARTESIAN_POINT('Ctrl Pts',(-13.1694755608909,-54.8098887390119,
2.23173550191459));
#61820=CARTESIAN_POINT('Ctrl Pts',(-12.3130077055018,-53.3174154968918,
2.31024101229136));
#61821=CARTESIAN_POINT('Ctrl Pts',(-13.0852322400692,-51.7797767714816,
2.38874652266815));
#61822=CARTESIAN_POINT('Ctrl Pts',(-14.7938791388703,-51.5757659053288,
2.46725203304492));
#61823=CARTESIAN_POINT('Ctrl Pts',(-15.9064540032169,-52.8884432158558,
2.5457575434217));
#61824=CARTESIAN_POINT('Ctrl Pts',(-15.4252426613265,-54.5405193661699,
2.62426305379848));
#61825=CARTESIAN_POINT('Ctrl Pts',(-13.7817722776592,-55.0503976760766,
2.70276856417526));
#61826=CARTESIAN_POINT('Ctrl Pts',(-12.4499634166736,-53.960794947638,2.78127407455204));
#61827=CARTESIAN_POINT('Ctrl Pts',(-12.6242053254302,-52.2488988977254,
2.85977958492882));
#61828=CARTESIAN_POINT('Ctrl Pts',(-14.1482380059646,-51.4499755676755,
2.93828509530561));
#61829=CARTESIAN_POINT('Ctrl Pts',(-15.6552705807332,-52.2805199058824,
3.01679060568238));
#61830=CARTESIAN_POINT('Ctrl Pts',(-15.7937614748382,-53.9956792506399,
3.09529611605916));
#61831=CARTESIAN_POINT('Ctrl Pts',(-14.4395082306652,-55.0572583019617,
3.17380162643594));
#61832=CARTESIAN_POINT('Ctrl Pts',(-12.8070376180166,-54.5132075415871,
3.25230713681272));
#61833=CARTESIAN_POINT('Ctrl Pts',(-12.3603879600184,-52.8514447189325,
3.3308126471895));
#61834=CARTESIAN_POINT('Ctrl Pts',(-13.5001253542918,-51.5622781929174,
3.40931815756628));
#61835=CARTESIAN_POINT('Ctrl Pts',(-15.2041061771209,-51.8018631754771,
3.48782366794306));
#61836=CARTESIAN_POINT('Ctrl Pts',(-15.944159933136,-53.3553341468671,3.56632917831984));
#61837=CARTESIAN_POINT('Ctrl Pts',(-15.0565888120043,-54.8295014140574,
3.64483468869662));
#61838=CARTESIAN_POINT('Ctrl Pts',(-13.3373877000383,-54.9022967226366,
3.7233401990734));
#61839=CARTESIAN_POINT('Ctrl Pts',(-12.3283770240505,-53.5084355106897,
3.80184570945017));
#61840=CARTESIAN_POINT('Ctrl Pts',(-12.9344615472089,-51.8979656495417,
3.88035121982696));
#61841=CARTESIAN_POINT('Ctrl Pts',(-14.612090259655,-51.5151947977304,3.95885673020373));
#61842=CARTESIAN_POINT('Ctrl Pts',(-15.8567258492822,-52.7034009548898,
4.03736224058051));
#61843=CARTESIAN_POINT('Ctrl Pts',(-15.5521495290616,-54.3969725912808,
4.11586775095729));
#61844=CARTESIAN_POINT('Ctrl Pts',(-13.9715125851379,-55.0770744011889,
4.19437326133407));
#61845=CARTESIAN_POINT('Ctrl Pts',(-12.5323678038339,-54.1337749126023,
4.27287877171085));
#61846=CARTESIAN_POINT('Ctrl Pts',(-12.5253744436601,-52.413047533365,4.35138428208763));
#61847=CARTESIAN_POINT('Ctrl Pts',(-13.9568043064156,-51.4580814834715,
4.42988979246441));
#61848=CARTESIAN_POINT('Ctrl Pts',(-15.5429170806551,-52.1253130228172,
4.50839530284119));
#61849=CARTESIAN_POINT('Ctrl Pts',(-15.8612490831165,-53.8163530377063,
4.58690081321797));
#61850=CARTESIAN_POINT('Ctrl Pts',(-14.6263126856139,-55.0146366540294,
4.66540632359475));
#61851=CARTESIAN_POINT('Ctrl Pts',(-12.9456280488333,-54.64551461019,4.74391183397153));
#61852=CARTESIAN_POINT('Ctrl Pts',(-12.3264734310144,-53.0400243844669,
4.82241734434831));
#61853=CARTESIAN_POINT('Ctrl Pts',(-13.324120771136,-51.638007671339,4.90092285472508));
#61854=CARTESIAN_POINT('Ctrl Pts',(-15.0438575043005,-51.6968266074015,
4.97942836510187));
#61855=CARTESIAN_POINT('Ctrl Pts',(-15.9433802614164,-53.1637305367386,
5.05793387547864));
#61856=CARTESIAN_POINT('Ctrl Pts',(-15.2159808288477,-54.7231660158524,
5.13643938585543));
#61857=CARTESIAN_POINT('Ctrl Pts',(-13.513997920622,-54.9765924805557,5.2149448962322));
#61858=CARTESIAN_POINT('Ctrl Pts',(-12.3638311119676,-53.696734568805,5.29345040660899));
#61859=CARTESIAN_POINT('Ctrl Pts',(-12.7969355370903,-52.0313922294383,
5.37195591698576));
#61860=CARTESIAN_POINT('Ctrl Pts',(-14.424976702367,-51.4740982114769,5.45046142736254));
#61861=CARTESIAN_POINT('Ctrl Pts',(-15.7877203932888,-52.5246186608361,
5.52896693773933));
#61862=CARTESIAN_POINT('Ctrl Pts',(-15.6633630429778,-54.2408787854042,
5.60747244811611));
#61863=CARTESIAN_POINT('Ctrl Pts',(-14.1627545185313,-55.0835815406539,
5.68597795849288));
#61864=CARTESIAN_POINT('Ctrl Pts',(-12.6330342875793,-54.2971998857928,
5.76448346886966));
#61865=CARTESIAN_POINT('Ctrl Pts',(-12.4433594214856,-52.5865231455987,
5.84298897924644));
#61866=CARTESIAN_POINT('Ctrl Pts',(-13.76941659957,-51.486617996264,5.92149448962323));
#61867=CARTESIAN_POINT('Ctrl Pts',(-14.8623799894179,-51.8174664687922,
5.97383149654107));
#61868=CARTESIAN_POINT('Ctrl Pts',(-15.2209662466057,-52.1764590205668,
6.));
#61869=CARTESIAN_POINT('Ctrl Pts',(-12.9355708698302,-52.8497595669186,
2.));
#61870=CARTESIAN_POINT('Ctrl Pts',(-12.9469576730109,-52.8006000143783,
2.));
#61871=CARTESIAN_POINT('Ctrl Pts',(-12.9614720678986,-52.7523805759145,
2.));
#61872=CARTESIAN_POINT('Ctrl Pts',(-12.9788381112572,-52.7052630574535,
2.));
#61873=CARTESIAN_POINT('Ctrl Pts',(-12.9969823676714,-52.6560340926918,
2.));
#61874=CARTESIAN_POINT('Ctrl Pts',(-13.0182396625092,-52.608007253985,2.));
#61875=CARTESIAN_POINT('Ctrl Pts',(-13.0423523228529,-52.5613664966425,
2.));
#61876=CARTESIAN_POINT('Ctrl Pts',(-13.061689993281,-52.5239619306945,2.));
#61877=CARTESIAN_POINT('Ctrl Pts',(-13.0828653436285,-52.4874486478168,
2.));
#61878=CARTESIAN_POINT('Ctrl Pts',(-13.1057691188079,-52.4519266272348,
2.));
#61879=CARTESIAN_POINT('Ctrl Pts',(-13.1154541423153,-52.436905889314,2.));
#61880=CARTESIAN_POINT('Ctrl Pts',(-13.1254484616934,-52.4220624809487,
2.));
#61881=CARTESIAN_POINT('Ctrl Pts',(-13.1357448170118,-52.4074044118665,
2.));
#61882=CARTESIAN_POINT('Ctrl Pts',(-13.1415823490882,-52.3990940004831,
2.));
#61883=CARTESIAN_POINT('Ctrl Pts',(-13.1475174809115,-52.3908426597166,
2.));
#61884=CARTESIAN_POINT('Ctrl Pts',(-13.1535391079514,-52.3826647593396,
2.));
#61885=CARTESIAN_POINT('Ctrl Pts',(-13.185818005202,-52.3388271712184,2.));
#61886=CARTESIAN_POINT('Ctrl Pts',(-13.2206401757039,-52.2970090605309,
2.));
#61887=CARTESIAN_POINT('Ctrl Pts',(-13.2577323841666,-52.2574000923829,
2.));
#61888=CARTESIAN_POINT('Ctrl Pts',(-13.2955035907173,-52.2170660551502,
2.));
#61889=CARTESIAN_POINT('Ctrl Pts',(-13.3356292075146,-52.1790218018794,
2.));
#61890=CARTESIAN_POINT('Ctrl Pts',(-13.3778710217101,-52.1434855491502,
2.));
#61891=CARTESIAN_POINT('Ctrl Pts',(-13.4080812323503,-52.1180709759184,
2.));
#61892=CARTESIAN_POINT('Ctrl Pts',(-13.4393749054964,-52.0939395106298,
2.));
#61893=CARTESIAN_POINT('Ctrl Pts',(-13.4716779317663,-52.0711807776364,
2.));
#61894=CARTESIAN_POINT('Ctrl Pts',(-13.4854146711621,-52.0615027127549,
2.));
#61895=CARTESIAN_POINT('Ctrl Pts',(-13.4993340562618,-52.0520730061476,
2.));
#61896=CARTESIAN_POINT('Ctrl Pts',(-13.5134308827615,-52.0428991428661,
2.));
#61897=CARTESIAN_POINT('Ctrl Pts',(-13.52183136089,-52.0374323211065,2.));
#61898=CARTESIAN_POINT('Ctrl Pts',(-13.5302901169523,-52.0320595108122,
2.));
#61899=CARTESIAN_POINT('Ctrl Pts',(-13.538799357562,-52.0267858960231,2.));
#61900=CARTESIAN_POINT('Ctrl Pts',(-13.5870981541539,-51.9968526434936,
2.));
#61901=CARTESIAN_POINT('Ctrl Pts',(-13.6370817517559,-51.9700725295858,
2.));
#61902=CARTESIAN_POINT('Ctrl Pts',(-13.6884925442776,-51.9466636060488,
2.));
#61903=CARTESIAN_POINT('Ctrl Pts',(-13.7200525424512,-51.932293362996,2.));
#61904=CARTESIAN_POINT('Ctrl Pts',(-13.752151284848,-51.9191940299464,2.));
#61905=CARTESIAN_POINT('Ctrl Pts',(-13.7847364470979,-51.9074225450413,
2.));
#61906=CARTESIAN_POINT('Ctrl Pts',(-13.836418792392,-51.88875214706,2.));
#61907=CARTESIAN_POINT('Ctrl Pts',(-13.8893237899006,-51.8734194145919,
2.));
#61908=CARTESIAN_POINT('Ctrl Pts',(-13.9431611750089,-51.861330721175,2.));
#61909=CARTESIAN_POINT('Ctrl Pts',(-13.9592695284011,-51.8577137374523,
2.));
#61910=CARTESIAN_POINT('Ctrl Pts',(-13.9754615001947,-51.8543874911092,
2.));
#61911=CARTESIAN_POINT('Ctrl Pts',(-13.9917296362983,-51.8513502983977,
2.));
#61912=CARTESIAN_POINT('Ctrl Pts',(-14.0067700369073,-51.8485423187486,
2.));
#61913=CARTESIAN_POINT('Ctrl Pts',(-14.0218822544663,-51.8459805725654,
2.));
#61914=CARTESIAN_POINT('Ctrl Pts',(-14.0370239759629,-51.8436690391789,
2.));
#61915=CARTESIAN_POINT('Ctrl Pts',(-14.0931183782155,-51.8351056744626,
2.));
#61916=CARTESIAN_POINT('Ctrl Pts',(-14.149687152489,-51.8299561325424,2.));
#61917=CARTESIAN_POINT('Ctrl Pts',(-14.2064063479335,-51.828080515235,2.));
#61918=CARTESIAN_POINT('Ctrl Pts',(-14.2644669778174,-51.8261605387361,
2.));
#61919=CARTESIAN_POINT('Ctrl Pts',(-14.3226861857286,-51.8276710218953,
2.));
#61920=CARTESIAN_POINT('Ctrl Pts',(-14.3807392825943,-51.8325126403782,
2.));
#61921=CARTESIAN_POINT('Ctrl Pts',(-14.4159849881017,-51.8354521262703,
2.));
#61922=CARTESIAN_POINT('Ctrl Pts',(-14.4511698447364,-51.8396204788386,
2.));
#61923=CARTESIAN_POINT('Ctrl Pts',(-14.4862227576225,-51.8450046114987,
2.));
#61924=CARTESIAN_POINT('Ctrl Pts',(-14.5055224539648,-51.8479690477423,
2.));
#61925=CARTESIAN_POINT('Ctrl Pts',(-14.5247821602815,-51.8513021647932,
2.));
#61926=CARTESIAN_POINT('Ctrl Pts',(-14.5439899738547,-51.855002666883,2.));
#61927=CARTESIAN_POINT('Ctrl Pts',(-14.5555560513246,-51.8572309420422,
2.));
#61928=CARTESIAN_POINT('Ctrl Pts',(-14.5671052783022,-51.8595928681044,
2.));
#61929=CARTESIAN_POINT('Ctrl Pts',(-14.5786287782272,-51.8620869089405,
2.));
#61930=CARTESIAN_POINT('Ctrl Pts',(-14.6376831017684,-51.8748680861369,
2.));
#61931=CARTESIAN_POINT('Ctrl Pts',(-14.6958774997537,-51.8910736753997,
2.));
#61932=CARTESIAN_POINT('Ctrl Pts',(-14.7528646870875,-51.9106036961952,
2.));
#61933=CARTESIAN_POINT('Ctrl Pts',(-14.7899177177268,-51.9233021024998,
2.));
#61934=CARTESIAN_POINT('Ctrl Pts',(-14.8264606634567,-51.9374070196433,
2.));
#61935=CARTESIAN_POINT('Ctrl Pts',(-14.8623979324973,-51.9529027870108,
2.));
#61936=CARTESIAN_POINT('Ctrl Pts',(-14.8772478015739,-51.9593058922771,
2.));
#61937=CARTESIAN_POINT('Ctrl Pts',(-14.8919942354505,-51.9659465911414,
2.));
#61938=CARTESIAN_POINT('Ctrl Pts',(-14.9066303803289,-51.9728242372457,
2.));
#61939=CARTESIAN_POINT('Ctrl Pts',(-14.9173472276096,-51.9778601728396,
2.));
#61940=CARTESIAN_POINT('Ctrl Pts',(-14.9280038818557,-51.9830227414937,
2.));
#61941=CARTESIAN_POINT('Ctrl Pts',(-14.9385887530582,-51.988306995363,2.));
#61942=CARTESIAN_POINT('Ctrl Pts',(-14.9930076777083,-52.0154743937796,
2.));
#61943=CARTESIAN_POINT('Ctrl Pts',(-15.0455947546779,-52.0458841568081,
2.));
#61944=CARTESIAN_POINT('Ctrl Pts',(-15.0960008499165,-52.0794651524903,
2.));
#61945=CARTESIAN_POINT('Ctrl Pts',(-15.1196129598423,-52.095195753278,2.));
#61946=CARTESIAN_POINT('Ctrl Pts',(-15.1427463702698,-52.111622952968,2.));
#61947=CARTESIAN_POINT('Ctrl Pts',(-15.165364007469,-52.1287432229353,2.));
#61948=CARTESIAN_POINT('Ctrl Pts',(-15.1847945994588,-52.1434510802399,
2.));
#61949=CARTESIAN_POINT('Ctrl Pts',(-15.2038445286663,-52.1586704870383,
2.));
#61950=CARTESIAN_POINT('Ctrl Pts',(-15.2225082026616,-52.1743802571171,
2.));
#61951=CARTESIAN_POINT('Ctrl Pts',(-14.7622249872189,-54.3610567043161,
2.80658032638058));
#61952=CARTESIAN_POINT('Ctrl Pts',(-14.8615128627433,-54.3048362110035,
2.79940525217631));
#61953=CARTESIAN_POINT('Ctrl Pts',(-14.9530160801183,-54.235599890915,2.79223017797205));
#61954=CARTESIAN_POINT('Ctrl Pts',(-15.0325849243862,-54.1546351912659,
2.78505510376779));
#61955=CARTESIAN_POINT('Ctrl Pts',(-15.3227836759489,-53.8593455590615,
2.75888660030886));
#61956=CARTESIAN_POINT('Ctrl Pts',(-15.4542357696669,-53.4080493196853,
2.73271809684993));
#61957=CARTESIAN_POINT('Ctrl Pts',(-15.3680012509646,-53.0031097267674,
2.70654959339101));
#61958=CARTESIAN_POINT('Ctrl Pts',(-15.2817667322623,-52.5981701338496,
2.68038108993208));
#61959=CARTESIAN_POINT('Ctrl Pts',(-14.9778456011397,-52.23958718739,2.65421258647316));
#61960=CARTESIAN_POINT('Ctrl Pts',(-14.5925102242225,-52.0881604517115,
2.62804408301423));
#61961=CARTESIAN_POINT('Ctrl Pts',(-14.2071748473052,-51.9367337160331,
2.6018755795553));
#61962=CARTESIAN_POINT('Ctrl Pts',(-13.7404252245931,-51.9924631911358,
2.57570707609637));
#61963=CARTESIAN_POINT('Ctrl Pts',(-13.4015764529908,-52.2303456612731,
2.54953857263745));
#61964=CARTESIAN_POINT('Ctrl Pts',(-13.0627276813885,-52.4682281314104,
2.52337006917852));
#61965=CARTESIAN_POINT('Ctrl Pts',(-12.8517797608958,-52.8882635965824,
2.4972015657196));
#61966=CARTESIAN_POINT('Ctrl Pts',(-12.8632860991091,-53.3021301533919,
2.47103306226067));
#61967=CARTESIAN_POINT('Ctrl Pts',(-12.8747924373225,-53.7159967102013,
2.44486455880174));
#61968=CARTESIAN_POINT('Ctrl Pts',(-13.1087530342418,-54.1236943586483,
2.41869605534282));
#61969=CARTESIAN_POINT('Ctrl Pts',(-13.4603337012234,-54.3423524839877,
2.39252755188389));
#61970=CARTESIAN_POINT('Ctrl Pts',(-13.8119143682051,-54.5610106093271,
2.36635904842496));
#61971=CARTESIAN_POINT('Ctrl Pts',(-14.281115105249,-54.590629211559,2.34019054496604));
#61972=CARTESIAN_POINT('Ctrl Pts',(-14.6573871465026,-54.4180355738828,
2.31402204150711));
#61973=CARTESIAN_POINT('Ctrl Pts',(-14.6930548254675,-54.4016750320804,
2.31154146979827));
#61974=CARTESIAN_POINT('Ctrl Pts',(-14.7278874868095,-54.3834974973412,
2.30906089808942));
#61975=CARTESIAN_POINT('Ctrl Pts',(-14.7617771735939,-54.3636459375188,
2.30658032638058));
#61976=CARTESIAN_POINT('Ctrl Pts',(-15.6194800884629,-52.866705242183,2.));
#61977=CARTESIAN_POINT('Ctrl Pts',(-15.7510836294753,-53.3567463262429,
2.02616850345893));
#61978=CARTESIAN_POINT('Ctrl Pts',(-15.4911223508182,-54.468705692608,2.07850551037678));
#61979=CARTESIAN_POINT('Ctrl Pts',(-13.8755519245004,-55.0671510173417,
2.15701102075356));
#61980=CARTESIAN_POINT('Ctrl Pts',(-12.4888977717378,-54.0475500892828,
2.23551653113034));
#61981=CARTESIAN_POINT('Ctrl Pts',(-12.5727324025626,-52.3295818538895,
2.31402204150712));
#61982=CARTESIAN_POINT('Ctrl Pts',(-14.0528383317196,-51.4513683986095,
2.3925275518839));
#61983=CARTESIAN_POINT('Ctrl Pts',(-15.6013423678816,-52.2018016959779,
2.47103306226067));
#61984=CARTESIAN_POINT('Ctrl Pts',(-15.8297478005623,-53.907232954514,2.54953857263746));
#61985=CARTESIAN_POINT('Ctrl Pts',(-14.5330963425821,-55.0385110233129,
2.62804408301423));
#61986=CARTESIAN_POINT('Ctrl Pts',(-12.8743150895914,-54.5809192738243,
2.70654959339101));
#61987=CARTESIAN_POINT('Ctrl Pts',(-12.3410089780029,-52.9449163922479,
2.7850551037678));
#61988=CARTESIAN_POINT('Ctrl Pts',(-13.4114743235374,-51.5976690199096,
2.86356061414457));
#61989=CARTESIAN_POINT('Ctrl Pts',(-15.125685020798,-51.7474403844543,2.94206612452135));
#61990=CARTESIAN_POINT('Ctrl Pts',(-15.9462998191018,-53.2599021194416,
3.02057163489813));
#61991=CARTESIAN_POINT('Ctrl Pts',(-15.1373700363305,-54.7786474915821,
3.09907714527491));
#61992=CARTESIAN_POINT('Ctrl Pts',(-13.4243640409752,-54.9416270991707,
3.17758265565169));
#61993=CARTESIAN_POINT('Ctrl Pts',(-12.3435458814549,-53.6026781745395,
3.25608816602847));
#61994=CARTESIAN_POINT('Ctrl Pts',(-12.8642192037885,-51.9626013374103,
3.33459367640525));
#61995=CARTESIAN_POINT('Ctrl Pts',(-14.5194316817766,-51.4922567887358,
3.41309918678203));
#61996=CARTESIAN_POINT('Ctrl Pts',(-15.824749470772,-52.6134605506407,3.49160469715881));
#61997=CARTESIAN_POINT('Ctrl Pts',(-15.6095325175198,-54.3206905095792,
3.57011020753559));
#61998=CARTESIAN_POINT('Ctrl Pts',(-14.0667925161087,-55.0828622138133,
3.64861571791237));
#61999=CARTESIAN_POINT('Ctrl Pts',(-12.5800953694062,-54.216441978079,3.72712122828915));
#62000=CARTESIAN_POINT('Ctrl Pts',(-12.482746426243,-52.4984560584276,3.80562673866593));
#62001=CARTESIAN_POINT('Ctrl Pts',(-13.8620505314459,-51.4696350750294,
3.88413224904271));
#62002=CARTESIAN_POINT('Ctrl Pts',(-15.4810149732843,-52.0526501422855,
3.96263775941948));
#62003=CARTESIAN_POINT('Ctrl Pts',(-15.8877139511439,-53.7246394886754,
4.04114326979627));
#62004=CARTESIAN_POINT('Ctrl Pts',(-14.7174101533174,-54.9861233184472,
4.11964878017304));
#62005=CARTESIAN_POINT('Ctrl Pts',(-13.0196598476917,-54.705772943414,4.19815429054983));
#62006=CARTESIAN_POINT('Ctrl Pts',(-12.3170458706651,-53.1350132444558,
4.2766598009266));
#62007=CARTESIAN_POINT('Ctrl Pts',(-13.239689139382,-51.6825388628568,4.35516531130339));
#62008=CARTESIAN_POINT('Ctrl Pts',(-14.9601412381249,-51.6509633535717,
4.43367082168016));
#62009=CARTESIAN_POINT('Ctrl Pts',(-15.9354598188275,-53.0686043860759,
4.51217633205695));
#62010=CARTESIAN_POINT('Ctrl Pts',(-15.2909560004752,-54.6640877757789,
4.59068184243372));
#62011=CARTESIAN_POINT('Ctrl Pts',(-13.6046361114517,-55.0065460966708,
4.6691873528105));
#62012=CARTESIAN_POINT('Ctrl Pts',(-12.3888319545389,-53.7888545684045,
4.74769286318728));
#62013=CARTESIAN_POINT('Ctrl Pts',(-12.7339055288242,-52.1030679359729,
4.82619837356406));
#62014=CARTESIAN_POINT('Ctrl Pts',(-14.3303867955418,-51.461039661442,4.90470388394084));
#62015=CARTESIAN_POINT('Ctrl Pts',(-15.7465131069793,-52.4385560995515,
4.98320939431762));
#62016=CARTESIAN_POINT('Ctrl Pts',(-15.7122693095411,-54.1589569990369,
5.0617149046944));
#62017=CARTESIAN_POINT('Ctrl Pts',(-14.2583648731494,-55.0793464756679,
5.14022041507118));
#62018=CARTESIAN_POINT('Ctrl Pts',(-12.6886982319545,-54.374296277089,5.21872592544796));
#62019=CARTESIAN_POINT('Ctrl Pts',(-12.4109789893208,-52.6761143673659,
5.29723143582474));
#62020=CARTESIAN_POINT('Ctrl Pts',(-13.6742819091468,-51.5077662723951,
5.37573694620152));
#62021=CARTESIAN_POINT('Ctrl Pts',(-15.3456277491901,-51.9170631330653,
5.4542424565783));
#62022=CARTESIAN_POINT('Ctrl Pts',(-15.9261522494264,-53.5369201511686,
5.53274796695508));
#62023=CARTESIAN_POINT('Ctrl Pts',(-14.895150144613,-54.9146464419454,5.61125347733186));
#62024=CARTESIAN_POINT('Ctrl Pts',(-13.1774033105245,-54.8145932898247,
5.68975898770864));
#62025=CARTESIAN_POINT('Ctrl Pts',(-12.3131175991141,-53.3266332457169,
5.76826449808541));
#62026=CARTESIAN_POINT('Ctrl Pts',(-13.07802768807,-51.78491829464,5.84677000846219));
#62027=CARTESIAN_POINT('Ctrl Pts',(-14.7848942477639,-51.572669265091,5.92527551883898));
#62028=CARTESIAN_POINT('Ctrl Pts',(-15.9054717137608,-52.8790772926886,
6.00378102921575));
#62029=CARTESIAN_POINT('Ctrl Pts',(-15.4296884573085,-54.5349259880616,
6.08228653959253));
#62030=CARTESIAN_POINT('Ctrl Pts',(-14.340318424872,-54.8774262527002,6.13462354651039));
#62031=CARTESIAN_POINT('Ctrl Pts',(-13.8417981729249,-54.7828888819299,
6.16079204996931));
#62032=CARTESIAN_POINT('Ctrl Pts',(-15.5298235927831,-52.8907830444123,
1.94640265001023));
#62033=CARTESIAN_POINT('Ctrl Pts',(-15.6535093143589,-53.3513412073422,
1.97257115346916));
#62034=CARTESIAN_POINT('Ctrl Pts',(-15.4091883934694,-54.3964004476471,
2.02490816038701));
#62035=CARTESIAN_POINT('Ctrl Pts',(-13.8908174408455,-54.9588407987496,
2.10341367076379));
#62036=CARTESIAN_POINT('Ctrl Pts',(-12.5875902013567,-54.0005833268291,
2.18191918114057));
#62037=CARTESIAN_POINT('Ctrl Pts',(-12.6663809901671,-52.3859752455852,
2.26042469151735));
#62038=CARTESIAN_POINT('Ctrl Pts',(-14.0574375563364,-51.5605987847522,
2.33893020189413));
#62039=CARTESIAN_POINT('Ctrl Pts',(-15.5127771133299,-52.2658828763921,
2.41743571227091));
#62040=CARTESIAN_POINT('Ctrl Pts',(-15.7274407199139,-53.8687082577405,
2.49594122264768));
#62041=CARTESIAN_POINT('Ctrl Pts',(-14.5088012366685,-54.9319239065435,
2.57444673302446));
#62042=CARTESIAN_POINT('Ctrl Pts',(-12.9498192014264,-54.5018627905033,
2.65295224340125));
#62043=CARTESIAN_POINT('Ctrl Pts',(-12.4485990159725,-52.9642886845846,
2.73145775377802));
#62044=CARTESIAN_POINT('Ctrl Pts',(-13.4546606892816,-51.6980973487976,
2.8099632641548));
#62045=CARTESIAN_POINT('Ctrl Pts',(-15.0657373016022,-51.8388578416582,
2.88846877453159));
#62046=CARTESIAN_POINT('Ctrl Pts',(-15.8369804815592,-53.2603235530564,
2.96697428490836));
#62047=CARTESIAN_POINT('Ctrl Pts',(-15.0767192977297,-54.6876948517164,
3.04547979528514));
#62048=CARTESIAN_POINT('Ctrl Pts',(-13.4667749074093,-54.8408689244782,
3.12398530566192));
#62049=CARTESIAN_POINT('Ctrl Pts',(-12.4509832887027,-53.5824767670773,
3.2024908160387));
#62050=CARTESIAN_POINT('Ctrl Pts',(-12.9403307263376,-52.0410738118106,
3.28099632641548));
#62051=CARTESIAN_POINT('Ctrl Pts',(-14.4959586990071,-51.5990271583197,
3.35950183679226));
#62052=CARTESIAN_POINT('Ctrl Pts',(-15.7227431105485,-52.6527746126658,
3.43800734716904));
#62053=CARTESIAN_POINT('Ctrl Pts',(-15.5204745093119,-54.2572904770775,
3.51651285754582));
#62054=CARTESIAN_POINT('Ctrl Pts',(-14.0705521986317,-54.9736067439322,
3.5950183679226));
#62055=CARTESIAN_POINT('Ctrl Pts',(-12.6733009701311,-54.1593139732339,
3.67352387829938));
#62056=CARTESIAN_POINT('Ctrl Pts',(-12.5818089465339,-52.5446892716908,
3.75202938867616));
#62057=CARTESIAN_POINT('Ctrl Pts',(-13.8781283480645,-51.5777664615214,
3.83053489905294));
#62058=CARTESIAN_POINT('Ctrl Pts',(-15.3996891180402,-52.1257049039707,
3.90904040942972));
#62059=CARTESIAN_POINT('Ctrl Pts',(-15.781919384443,-53.6971003784726,3.9875459198065));
#62060=CARTESIAN_POINT('Ctrl Pts',(-14.682025957689,-54.8826880651052,4.06605143018327));
#62061=CARTESIAN_POINT('Ctrl Pts',(-13.0864194109997,-54.6192047411514,
4.14455694056006));
#62062=CARTESIAN_POINT('Ctrl Pts',(-12.4260776293937,-53.1429485151161,
4.22306245093684));
#62063=CARTESIAN_POINT('Ctrl Pts',(-13.2932108202671,-51.7778610670395,
4.30156796131361));
#62064=CARTESIAN_POINT('Ctrl Pts',(-14.9101533252533,-51.7481852724522,
4.38007347169039));
#62065=CARTESIAN_POINT('Ctrl Pts',(-15.8267926610378,-53.0805350913999,
4.45857898206717));
#62066=CARTESIAN_POINT('Ctrl Pts',(-15.2210648879245,-54.5800275275424,
4.53708449244395));
#62067=CARTESIAN_POINT('Ctrl Pts',(-13.6362010561689,-54.901882123576,4.61559000282073));
#62068=CARTESIAN_POINT('Ctrl Pts',(-12.4935447622286,-53.7574520104367,
4.69409551319751));
#62069=CARTESIAN_POINT('Ctrl Pts',(-12.8178572670739,-52.173089352326,4.77260102357429));
#62070=CARTESIAN_POINT('Ctrl Pts',(-14.3182875437761,-51.5696881839643,
4.85110653395107));
#62071=CARTESIAN_POINT('Ctrl Pts',(-15.6492137736117,-52.488393144862,4.92961204432785));
#62072=CARTESIAN_POINT('Ctrl Pts',(-15.6170302262462,-54.1052875309521,
5.00811755470463));
#62073=CARTESIAN_POINT('Ctrl Pts',(-14.2505987614542,-54.9703025272976,
5.08662306508141));
#62074=CARTESIAN_POINT('Ctrl Pts',(-12.7753698302556,-54.307671097417,5.16512857545819));
#62075=CARTESIAN_POINT('Ctrl Pts',(-12.5143593387719,-52.7116589137378,
5.24363408583497));
#62076=CARTESIAN_POINT('Ctrl Pts',(-13.7016566713931,-51.6136035265765,
5.32213959621175));
#62077=CARTESIAN_POINT('Ctrl Pts',(-15.2724473555814,-51.9982753762946,
5.40064510658853));
#62078=CARTESIAN_POINT('Ctrl Pts',(-15.8180450739392,-53.5206750214142,
5.4791506169653));
#62079=CARTESIAN_POINT('Ctrl Pts',(-14.8490723677412,-54.8155115364335,
5.55765612734209));
#62080=CARTESIAN_POINT('Ctrl Pts',(-13.2346723673735,-54.7214780003996,
5.63616163771886));
#62081=CARTESIAN_POINT('Ctrl Pts',(-12.4223856990886,-53.3230398556834,
5.71466714809565));
#62082=CARTESIAN_POINT('Ctrl Pts',(-13.1412755979873,-51.8740809240222,
5.79317265847242));
#62083=CARTESIAN_POINT('Ctrl Pts',(-14.745449926773,-51.674601683786,5.87167816884921));
#62084=CARTESIAN_POINT('Ctrl Pts',(-15.7986087657921,-52.9024107406155,
5.95018367922598));
#62085=CARTESIAN_POINT('Ctrl Pts',(-15.3514506199299,-54.4586366531711,
6.02868918960277));
#62086=CARTESIAN_POINT('Ctrl Pts',(-14.3276216447485,-54.7805306694404,
6.08102619652062));
#62087=CARTESIAN_POINT('Ctrl Pts',(-13.8590944561341,-54.691681062282,6.10719469997954));
#62088=CARTESIAN_POINT('Ctrl Pts',(-15.4401670971033,-52.9148608466415,
1.89280530002046));
#62089=CARTESIAN_POINT('Ctrl Pts',(-15.5559349992425,-53.3459360884415,
1.91897380347939));
#62090=CARTESIAN_POINT('Ctrl Pts',(-15.3272544361205,-54.3240952026862,
1.97131081039724));
#62091=CARTESIAN_POINT('Ctrl Pts',(-13.9060829571907,-54.8505305801576,
2.04981632077402));
#62092=CARTESIAN_POINT('Ctrl Pts',(-12.6862826309757,-53.9536165643755,
2.1283218311508));
#62093=CARTESIAN_POINT('Ctrl Pts',(-12.7600295777717,-52.4423686372808,
2.20682734152758));
#62094=CARTESIAN_POINT('Ctrl Pts',(-14.0620367809532,-51.6698291708949,
2.28533285190436));
#62095=CARTESIAN_POINT('Ctrl Pts',(-15.4242118587782,-52.3299640568063,
2.36383836228114));
#62096=CARTESIAN_POINT('Ctrl Pts',(-15.6251336392654,-53.8301835609669,
2.44234387265791));
#62097=CARTESIAN_POINT('Ctrl Pts',(-14.4845061307549,-54.8253367897741,
2.52084938303469));
#62098=CARTESIAN_POINT('Ctrl Pts',(-13.0253233132613,-54.4228063071824,
2.59935489341147));
#62099=CARTESIAN_POINT('Ctrl Pts',(-12.5561890539421,-52.9836609769212,
2.67786040378825));
#62100=CARTESIAN_POINT('Ctrl Pts',(-13.4978470550258,-51.7985256776856,
2.75636591416503));
#62101=CARTESIAN_POINT('Ctrl Pts',(-15.0057895824065,-51.9302752988621,
2.83487142454181));
#62102=CARTESIAN_POINT('Ctrl Pts',(-15.7276611440166,-53.2607449866711,
2.91337693491859));
#62103=CARTESIAN_POINT('Ctrl Pts',(-15.016068559129,-54.5967422118507,2.99188244529537));
#62104=CARTESIAN_POINT('Ctrl Pts',(-13.5091857738434,-54.7401107497856,
3.07038795567215));
#62105=CARTESIAN_POINT('Ctrl Pts',(-12.5584206959504,-53.5622753596153,
3.14889346604893));
#62106=CARTESIAN_POINT('Ctrl Pts',(-13.0164422488867,-52.1195462862107,
3.22739897642571));
#62107=CARTESIAN_POINT('Ctrl Pts',(-14.4724857162377,-51.7057975279038,
3.30590448680249));
#62108=CARTESIAN_POINT('Ctrl Pts',(-15.6207367503249,-52.6920886746908,
3.38440999717927));
#62109=CARTESIAN_POINT('Ctrl Pts',(-15.4314165011041,-54.1938904445758,
3.46291550755605));
#62110=CARTESIAN_POINT('Ctrl Pts',(-14.0743118811546,-54.864351274051,3.54142101793283));
#62111=CARTESIAN_POINT('Ctrl Pts',(-12.766506570856,-54.1021859683889,3.61992652830961));
#62112=CARTESIAN_POINT('Ctrl Pts',(-12.6808714668247,-52.5909224849539,
3.69843203868639));
#62113=CARTESIAN_POINT('Ctrl Pts',(-13.894206164683,-51.6858978480135,3.77693754906317));
#62114=CARTESIAN_POINT('Ctrl Pts',(-15.3183632627962,-52.1987596656559,
3.85544305943995));
#62115=CARTESIAN_POINT('Ctrl Pts',(-15.6761248177421,-53.6695612682698,
3.93394856981672));
#62116=CARTESIAN_POINT('Ctrl Pts',(-14.6466417620606,-54.7792528117632,
4.01245408019351));
#62117=CARTESIAN_POINT('Ctrl Pts',(-13.1531789743077,-54.5326365388889,
4.09095959057028));
#62118=CARTESIAN_POINT('Ctrl Pts',(-12.5351093881223,-53.1508837857763,
4.16946510094707));
#62119=CARTESIAN_POINT('Ctrl Pts',(-13.3467325011522,-51.8731832712222,
4.24797061132384));
#62120=CARTESIAN_POINT('Ctrl Pts',(-14.8601654123817,-51.8454071913326,
4.32647612170063));
#62121=CARTESIAN_POINT('Ctrl Pts',(-15.7181255032481,-53.092465796724,4.4049816320774));
#62122=CARTESIAN_POINT('Ctrl Pts',(-15.1511737753737,-54.4959672793058,
4.48348714245419));
#62123=CARTESIAN_POINT('Ctrl Pts',(-13.6677660008861,-54.7972181504813,
4.56199265283096));
#62124=CARTESIAN_POINT('Ctrl Pts',(-12.5982575699184,-53.7260494524687,
4.64049816320774));
#62125=CARTESIAN_POINT('Ctrl Pts',(-12.9018090053235,-52.2431107686793,
4.71900367358452));
#62126=CARTESIAN_POINT('Ctrl Pts',(-14.3061882920105,-51.6783367064866,
4.7975091839613));
#62127=CARTESIAN_POINT('Ctrl Pts',(-15.5519144402441,-52.5382301901725,
4.87601469433808));
#62128=CARTESIAN_POINT('Ctrl Pts',(-15.5217911429513,-54.0516180628673,
4.95452020471486));
#62129=CARTESIAN_POINT('Ctrl Pts',(-14.242832649759,-54.8612585789273,5.03302571509164));
#62130=CARTESIAN_POINT('Ctrl Pts',(-12.8620414285567,-54.2410459177449,
5.11153122546842));
#62131=CARTESIAN_POINT('Ctrl Pts',(-12.617739688223,-52.7472034601099,5.1900367358452));
#62132=CARTESIAN_POINT('Ctrl Pts',(-13.7290314336393,-51.7194407807578,
5.26854224622197));
#62133=CARTESIAN_POINT('Ctrl Pts',(-15.1992669619728,-52.079487619524,5.34704775659876));
#62134=CARTESIAN_POINT('Ctrl Pts',(-15.709937898452,-53.5044298916598,5.42555326697553));
#62135=CARTESIAN_POINT('Ctrl Pts',(-14.8029945908694,-54.7163766309217,
5.50405877735232));
#62136=CARTESIAN_POINT('Ctrl Pts',(-13.2919414242225,-54.6283627109744,
5.58256428772909));
#62137=CARTESIAN_POINT('Ctrl Pts',(-12.5316537990631,-53.31944646565,5.66106979810588));
#62138=CARTESIAN_POINT('Ctrl Pts',(-13.2045235079047,-51.9632435534043,
5.73957530848265));
#62139=CARTESIAN_POINT('Ctrl Pts',(-14.706005605782,-51.7765341024811,5.81808081885944));
#62140=CARTESIAN_POINT('Ctrl Pts',(-15.6917458178233,-52.9257441885424,
5.89658632923621));
#62141=CARTESIAN_POINT('Ctrl Pts',(-15.2732127825514,-54.3823473182807,
5.975091839613));
#62142=CARTESIAN_POINT('Ctrl Pts',(-14.314924864625,-54.6836350861806,6.02742884653085));
#62143=CARTESIAN_POINT('Ctrl Pts',(-13.8763907393433,-54.6004732426341,
6.05359734998977));
#62144=CARTESIAN_POINT('Ctrl Pts',(-15.3505106014235,-52.9389386488708,
1.83920795003069));
#62145=CARTESIAN_POINT('Ctrl Pts',(-15.4583606841261,-53.3405309695408,
1.86537645348962));
#62146=CARTESIAN_POINT('Ctrl Pts',(-15.2453204787717,-54.2517899577253,
1.91771346040747));
#62147=CARTESIAN_POINT('Ctrl Pts',(-13.9213484735358,-54.7422203615657,
1.99621897078425));
#62148=CARTESIAN_POINT('Ctrl Pts',(-12.7849750605946,-53.9066498019218,
2.07472448116103));
#62149=CARTESIAN_POINT('Ctrl Pts',(-12.8536781653762,-52.4987620289764,
2.15322999153781));
#62150=CARTESIAN_POINT('Ctrl Pts',(-14.06663600557,-51.7790595570376,2.23173550191459));
#62151=CARTESIAN_POINT('Ctrl Pts',(-15.3356466042264,-52.3940452372206,
2.31024101229137));
#62152=CARTESIAN_POINT('Ctrl Pts',(-15.522826558617,-53.7916588641933,2.38874652266814));
#62153=CARTESIAN_POINT('Ctrl Pts',(-14.4602110248413,-54.7187496730048,
2.46725203304492));
#62154=CARTESIAN_POINT('Ctrl Pts',(-13.1008274250962,-54.3437498238614,
2.5457575434217));
#62155=CARTESIAN_POINT('Ctrl Pts',(-12.6637790919117,-53.0030332692578,
2.62426305379848));
#62156=CARTESIAN_POINT('Ctrl Pts',(-13.54103342077,-51.8989540065736,2.70276856417526));
#62157=CARTESIAN_POINT('Ctrl Pts',(-14.9458418632107,-52.0216927560659,
2.78127407455204));
#62158=CARTESIAN_POINT('Ctrl Pts',(-15.618341806474,-53.2611664202859,2.85977958492882));
#62159=CARTESIAN_POINT('Ctrl Pts',(-14.9554178205282,-54.505789571985,2.9382850953056));
#62160=CARTESIAN_POINT('Ctrl Pts',(-13.5515966402775,-54.6393525750931,
3.01679060568238));
#62161=CARTESIAN_POINT('Ctrl Pts',(-12.6658581031982,-53.5420739521532,
3.09529611605916));
#62162=CARTESIAN_POINT('Ctrl Pts',(-13.0925537714359,-52.198018760611,3.17380162643594));
#62163=CARTESIAN_POINT('Ctrl Pts',(-14.4490127334682,-51.8125678974878,
3.25230713681272));
#62164=CARTESIAN_POINT('Ctrl Pts',(-15.5187303901013,-52.7314027367159,
3.3308126471895));
#62165=CARTESIAN_POINT('Ctrl Pts',(-15.3423584928962,-54.130490412074,3.40931815756628));
#62166=CARTESIAN_POINT('Ctrl Pts',(-14.0780715636776,-54.75509580417,3.48782366794306));
#62167=CARTESIAN_POINT('Ctrl Pts',(-12.8597121715808,-54.0450579635438,
3.56632917831983));
#62168=CARTESIAN_POINT('Ctrl Pts',(-12.7799339871156,-52.6371556982172,
3.64483468869662));
#62169=CARTESIAN_POINT('Ctrl Pts',(-13.9102839813016,-51.7940292345055,
3.7233401990734));
#62170=CARTESIAN_POINT('Ctrl Pts',(-15.2370374075522,-52.2718144273412,
3.80184570945018));
#62171=CARTESIAN_POINT('Ctrl Pts',(-15.5703302510412,-53.642022158067,3.88035121982695));
#62172=CARTESIAN_POINT('Ctrl Pts',(-14.6112575664322,-54.6758175584211,
3.95885673020374));
#62173=CARTESIAN_POINT('Ctrl Pts',(-13.2199385376158,-54.4460683366263,
4.03736224058051));
#62174=CARTESIAN_POINT('Ctrl Pts',(-12.644141146851,-53.1588190564366,4.1158677509573));
#62175=CARTESIAN_POINT('Ctrl Pts',(-13.4002541820374,-51.9685054754049,
4.19437326133407));
#62176=CARTESIAN_POINT('Ctrl Pts',(-14.8101774995101,-51.9426291102131,
4.27287877171085));
#62177=CARTESIAN_POINT('Ctrl Pts',(-15.6094583454585,-53.1043965020481,
4.35138428208763));
#62178=CARTESIAN_POINT('Ctrl Pts',(-15.081282662823,-54.4119070310692,4.42988979246441));
#62179=CARTESIAN_POINT('Ctrl Pts',(-13.6993309456032,-54.6925541773866,
4.50839530284119));
#62180=CARTESIAN_POINT('Ctrl Pts',(-12.7029703776082,-53.6946468945009,
4.58690081321797));
#62181=CARTESIAN_POINT('Ctrl Pts',(-12.9857607435731,-52.3131321850324,
4.66540632359475));
#62182=CARTESIAN_POINT('Ctrl Pts',(-14.2940890402448,-51.7869852290089,
4.74391183397153));
#62183=CARTESIAN_POINT('Ctrl Pts',(-15.4546151068764,-52.5880672354829,
4.82241734434831));
#62184=CARTESIAN_POINT('Ctrl Pts',(-15.4265520596564,-53.9979485947826,
4.90092285472509));
#62185=CARTESIAN_POINT('Ctrl Pts',(-14.2350665380638,-54.7522146305569,
4.97942836510187));
#62186=CARTESIAN_POINT('Ctrl Pts',(-12.9487130268578,-54.1744207380729,
5.05793387547865));
#62187=CARTESIAN_POINT('Ctrl Pts',(-12.7211200376741,-52.7827480064818,
5.13643938585543));
#62188=CARTESIAN_POINT('Ctrl Pts',(-13.7564061958854,-51.8252780349391,
5.2149448962322));
#62189=CARTESIAN_POINT('Ctrl Pts',(-15.1260865683642,-52.1606998627533,
5.29345040660899));
#62190=CARTESIAN_POINT('Ctrl Pts',(-15.6018307229648,-53.4881847619054,
5.37195591698576));
#62191=CARTESIAN_POINT('Ctrl Pts',(-14.7569168139975,-54.6172417254097,
5.45046142736255));
#62192=CARTESIAN_POINT('Ctrl Pts',(-13.3492104810715,-54.5352474215493,
5.52896693773932));
#62193=CARTESIAN_POINT('Ctrl Pts',(-12.6409218990375,-53.3158530756166,
5.60747244811611));
#62194=CARTESIAN_POINT('Ctrl Pts',(-13.2677714178221,-52.0524061827865,
5.68597795849288));
#62195=CARTESIAN_POINT('Ctrl Pts',(-14.666561284791,-51.8784665211762,5.76448346886966));
#62196=CARTESIAN_POINT('Ctrl Pts',(-15.5848828698546,-52.9490776364693,
5.84298897924644));
#62197=CARTESIAN_POINT('Ctrl Pts',(-15.1949749451728,-54.3060579833903,
5.92149448962322));
#62198=CARTESIAN_POINT('Ctrl Pts',(-14.3022280845015,-54.5867395029208,
5.97383149654108));
#62199=CARTESIAN_POINT('Ctrl Pts',(-13.8936870225526,-54.5092654229862,
6.));
#62200=CARTESIAN_POINT('Ctrl Pts',(-14.7602610286104,-54.3618122024717,
2.44341967361942));
#62201=CARTESIAN_POINT('Ctrl Pts',(-14.651278048058,-54.4258677305587,2.45136379342793));
#62202=CARTESIAN_POINT('Ctrl Pts',(-14.5332929975391,-54.473801003601,2.45930791323643));
#62203=CARTESIAN_POINT('Ctrl Pts',(-14.4107496805131,-54.5017345633457,
2.46725203304493));
#62204=CARTESIAN_POINT('Ctrl Pts',(-14.0070831582596,-54.5937497232903,
2.49342053650386));
#62205=CARTESIAN_POINT('Ctrl Pts',(-13.5539552916779,-54.4687497735759,
2.51958903996278));
#62206=CARTESIAN_POINT('Ctrl Pts',(-13.254549969523,-54.1827970396181,2.54575754342171));
#62207=CARTESIAN_POINT('Ctrl Pts',(-12.955144647368,-53.8968443056602,2.57192604688064));
#62208=CARTESIAN_POINT('Ctrl Pts',(-12.8094618696399,-53.449938787459,2.59809455033956));
#62209=CARTESIAN_POINT('Ctrl Pts',(-12.8828295355855,-53.042472817911,2.62426305379849));
#62210=CARTESIAN_POINT('Ctrl Pts',(-12.9561972015311,-52.6350068483631,
2.65043155725742));
#62211=CARTESIAN_POINT('Ctrl Pts',(-13.2486153111506,-52.2669804274683,
2.67660006071634));
#62212=CARTESIAN_POINT('Ctrl Pts',(-13.6289591063671,-52.1034236752697,
2.70276856417527));
#62213=CARTESIAN_POINT('Ctrl Pts',(-14.0093029015836,-51.939866923071,2.7289370676342));
#62214=CARTESIAN_POINT('Ctrl Pts',(-14.4775723823971,-51.9807798395685,
2.75510557109312));
#62215=CARTESIAN_POINT('Ctrl Pts',(-14.8237904466811,-52.2078152418539,
2.78127407455205));
#62216=CARTESIAN_POINT('Ctrl Pts',(-15.1700085109651,-52.4348506441393,
2.80744257801098));
#62217=CARTESIAN_POINT('Ctrl Pts',(-15.3941751587196,-52.8480085322126,
2.8336110814699));
#62218=CARTESIAN_POINT('Ctrl Pts',(-15.3957711516058,-53.2620246681991,
2.85977958492883));
#62219=CARTESIAN_POINT('Ctrl Pts',(-15.397367144492,-53.6760408041856,2.88594808838776));
#62220=CARTESIAN_POINT('Ctrl Pts',(-15.1763924825101,-54.0909151880853,
2.91211659184668));
#62221=CARTESIAN_POINT('Ctrl Pts',(-14.8319349548107,-54.3206128805532,
2.93828509530561));
#62222=CARTESIAN_POINT('Ctrl Pts',(-14.8094060374995,-54.3356360398807,
2.93999662141021));
#62223=CARTESIAN_POINT('Ctrl Pts',(-14.7863488988009,-54.3498670707759,
2.94170814751482));
#62224=CARTESIAN_POINT('Ctrl Pts',(-14.7628222445742,-54.3633003878638,
2.94341967361942));
#62225=CARTESIAN_POINT('Ctrl Pts',(-15.6194800884629,-52.866705242183,2.));
#62226=CARTESIAN_POINT('Ctrl Pts',(-15.6300231873965,-52.926941249885,2.));
#62227=CARTESIAN_POINT('Ctrl Pts',(-15.6366567833015,-52.987630087735,2.));
#62228=CARTESIAN_POINT('Ctrl Pts',(-15.6395415323775,-53.0484503647743,
2.));
#62229=CARTESIAN_POINT('Ctrl Pts',(-15.6424094897195,-53.1089166152119,
2.));
#62230=CARTESIAN_POINT('Ctrl Pts',(-15.6415715704011,-53.1695138895016,
2.));
#62231=CARTESIAN_POINT('Ctrl Pts',(-15.6371309452724,-53.2299210873137,
2.));
#62232=CARTESIAN_POINT('Ctrl Pts',(-15.6337777267599,-53.275535956418,2.));
#62233=CARTESIAN_POINT('Ctrl Pts',(-15.628369049543,-53.3210424392735,2.));
#62234=CARTESIAN_POINT('Ctrl Pts',(-15.6209312260544,-53.3662945441232,
2.));
#62235=CARTESIAN_POINT('Ctrl Pts',(-15.6170700144012,-53.3897863565925,
2.));
#62236=CARTESIAN_POINT('Ctrl Pts',(-15.6126617095028,-53.4132094747526,
2.));
#62237=CARTESIAN_POINT('Ctrl Pts',(-15.6077085063714,-53.4365423663737,
2.));
#62238=CARTESIAN_POINT('Ctrl Pts',(-15.6050999838096,-53.4488302480955,
2.));
#62239=CARTESIAN_POINT('Ctrl Pts',(-15.6023397247485,-53.4610950217813,
2.));
#62240=CARTESIAN_POINT('Ctrl Pts',(-15.5994335441816,-53.4733116340984,
2.));
#62241=CARTESIAN_POINT('Ctrl Pts',(-15.5857322512136,-53.5309072929295,
2.));
#62242=CARTESIAN_POINT('Ctrl Pts',(-15.5687698297262,-53.5875426491389,
2.));
#62243=CARTESIAN_POINT('Ctrl Pts',(-15.5486498653488,-53.6429179274305,
2.));
#62244=CARTESIAN_POINT('Ctrl Pts',(-15.5289409667849,-53.6971618476645,
2.));
#62245=CARTESIAN_POINT('Ctrl Pts',(-15.5062016386593,-53.750197506391,2.));
#62246=CARTESIAN_POINT('Ctrl Pts',(-15.4804878124321,-53.8017173359829,
2.));
#62247=CARTESIAN_POINT('Ctrl Pts',(-15.4618733917502,-53.8390129050285,
2.));
#62248=CARTESIAN_POINT('Ctrl Pts',(-15.4416993411965,-53.8755136264382,
2.));
#62249=CARTESIAN_POINT('Ctrl Pts',(-15.4199753876582,-53.9110903776553,
2.));
#62250=CARTESIAN_POINT('Ctrl Pts',(-15.4086212485557,-53.9296847546606,
2.));
#62251=CARTESIAN_POINT('Ctrl Pts',(-15.3968435749602,-53.9480265376898,
2.));
#62252=CARTESIAN_POINT('Ctrl Pts',(-15.3846428359465,-53.9660958743658,
2.));
#62253=CARTESIAN_POINT('Ctrl Pts',(-15.3789686731663,-53.9744993290676,
2.));
#62254=CARTESIAN_POINT('Ctrl Pts',(-15.373205772762,-53.9828396301787,2.));
#62255=CARTESIAN_POINT('Ctrl Pts',(-15.3673591188136,-53.9911085225216,
2.));
#62256=CARTESIAN_POINT('Ctrl Pts',(-15.3351612285807,-54.0366458316147,
2.));
#62257=CARTESIAN_POINT('Ctrl Pts',(-15.3003846168084,-54.0800821194251,
2.));
#62258=CARTESIAN_POINT('Ctrl Pts',(-15.2630875306082,-54.1211378587395,
2.));
#62259=CARTESIAN_POINT('Ctrl Pts',(-15.2381315874427,-54.1486087633418,
2.));
#62260=CARTESIAN_POINT('Ctrl Pts',(-15.212046413087,-54.1750132365444,2.));
#62261=CARTESIAN_POINT('Ctrl Pts',(-15.1848412564379,-54.2002572946035,
2.));
#62262=CARTESIAN_POINT('Ctrl Pts',(-15.1445758545731,-54.2376201429619,
2.));
#62263=CARTESIAN_POINT('Ctrl Pts',(-15.1018570560095,-54.2724429083026,
2.));
#62264=CARTESIAN_POINT('Ctrl Pts',(-15.0569812349608,-54.3046174971127,
2.));
#62265=CARTESIAN_POINT('Ctrl Pts',(-15.0431218621615,-54.3145542427936,
2.));
#62266=CARTESIAN_POINT('Ctrl Pts',(-15.0290566706306,-54.3242380855765,
2.));
#62267=CARTESIAN_POINT('Ctrl Pts',(-15.0147942526821,-54.3336649770066,
2.));
#62268=CARTESIAN_POINT('Ctrl Pts',(-15.0022772711832,-54.3419382043128,
2.));
#62269=CARTESIAN_POINT('Ctrl Pts',(-14.9896026925897,-54.3500168035422,
2.));
#62270=CARTESIAN_POINT('Ctrl Pts',(-14.9768072444657,-54.357879401603,2.));
#62271=CARTESIAN_POINT('Ctrl Pts',(-14.9293632591267,-54.3870329711781,
2.));
#62272=CARTESIAN_POINT('Ctrl Pts',(-14.8801986447078,-54.4132643407243,
2.));
#62273=CARTESIAN_POINT('Ctrl Pts',(-14.8296406252006,-54.4365044915624,
2.));
#62274=CARTESIAN_POINT('Ctrl Pts',(-14.779143507916,-54.4597166472999,2.));
#62275=CARTESIAN_POINT('Ctrl Pts',(-14.7272551246641,-54.4799449627967,
2.));
#62276=CARTESIAN_POINT('Ctrl Pts',(-14.6742902116631,-54.497070407063,2.));
#62277=CARTESIAN_POINT('Ctrl Pts',(-14.640435964457,-54.5080166918931,2.));
#62278=CARTESIAN_POINT('Ctrl Pts',(-14.6061417257406,-54.5176942656991,
2.));
#62279=CARTESIAN_POINT('Ctrl Pts',(-14.571490685658,-54.5260607579898,2.));
#62280=CARTESIAN_POINT('Ctrl Pts',(-14.5536361910117,-54.5303717250331,
2.));
#62281=CARTESIAN_POINT('Ctrl Pts',(-14.5356869955265,-54.5343344557627,
2.));
#62282=CARTESIAN_POINT('Ctrl Pts',(-14.5176547593652,-54.5379422095234,
2.));
#62283=CARTESIAN_POINT('Ctrl Pts',(-14.5067786943522,-54.540118210553,2.));
#62284=CARTESIAN_POINT('Ctrl Pts',(-14.4958730433407,-54.5421648311715,
2.));
#62285=CARTESIAN_POINT('Ctrl Pts',(-14.484953604442,-54.5440785381673,2.));
#62286=CARTESIAN_POINT('Ctrl Pts',(-14.432148545692,-54.5533329889941,2.));
#62287=CARTESIAN_POINT('Ctrl Pts',(-14.3789399495426,-54.5594997842154,
2.));
#62288=CARTESIAN_POINT('Ctrl Pts',(-14.3256201372965,-54.5624573557298,
2.));
#62289=CARTESIAN_POINT('Ctrl Pts',(-14.2921372782686,-54.5643146006433,
2.));
#62290=CARTESIAN_POINT('Ctrl Pts',(-14.2586106299683,-54.564905353366,2.));
#62291=CARTESIAN_POINT('Ctrl Pts',(-14.2251154868282,-54.5641893509547,
2.));
#62292=CARTESIAN_POINT('Ctrl Pts',(-14.2128693182197,-54.5639275731138,
2.));
#62293=CARTESIAN_POINT('Ctrl Pts',(-14.2006248767607,-54.5634909095273,
2.));
#62294=CARTESIAN_POINT('Ctrl Pts',(-14.1883942976858,-54.562877565248,2.));
#62295=CARTESIAN_POINT('Ctrl Pts',(-14.1370506806676,-54.5603027637126,
2.));
#62296=CARTESIAN_POINT('Ctrl Pts',(-14.0860310638802,-54.5546235246412,
2.));
#62297=CARTESIAN_POINT('Ctrl Pts',(-14.0356066350433,-54.5457116916821,
2.));
#62298=CARTESIAN_POINT('Ctrl Pts',(-14.0074349170479,-54.5407327231398,
2.));
#62299=CARTESIAN_POINT('Ctrl Pts',(-13.9794492438898,-54.5347439009261,
2.));
#62300=CARTESIAN_POINT('Ctrl Pts',(-13.9516999296066,-54.5277163783411,
2.));
#62301=CARTESIAN_POINT('Ctrl Pts',(-13.932212693117,-54.5227812295604,2.));
#62302=CARTESIAN_POINT('Ctrl Pts',(-13.9128420740716,-54.517333696643,2.));
#62303=CARTESIAN_POINT('Ctrl Pts',(-13.8936031194075,-54.5113848919291,
2.));
#62304=CARTESIAN_POINT('Origin',(-14.1292828945604,-53.2669068454841,4.5));
#62305=CARTESIAN_POINT('Origin',(-53.1951359564886,-14.3971354987959,6.));
#62306=CARTESIAN_POINT('Ctrl Pts',(-54.153252109211,-15.2223467977324,6.));
#62307=CARTESIAN_POINT('Ctrl Pts',(-54.1904452248526,-15.1876133706859,
6.));
#62308=CARTESIAN_POINT('Ctrl Pts',(-54.2252563920676,-15.1505690966151,
6.));
#62309=CARTESIAN_POINT('Ctrl Pts',(-54.2576712403365,-15.1115269977936,
6.));
#62310=CARTESIAN_POINT('Ctrl Pts',(-54.2795176350154,-15.0852140842524,
6.));
#62311=CARTESIAN_POINT('Ctrl Pts',(-54.3002751129523,-15.0579926438535,
6.));
#62312=CARTESIAN_POINT('Ctrl Pts',(-54.3199324346161,-15.0299477424349,
6.));
#62313=CARTESIAN_POINT('Ctrl Pts',(-54.3290141536918,-15.0169909459524,
6.));
#62314=CARTESIAN_POINT('Ctrl Pts',(-54.337860965377,-15.0038582766482,6.));
#62315=CARTESIAN_POINT('Ctrl Pts',(-54.3464713059304,-14.9905576084913,
6.));
#62316=CARTESIAN_POINT('Ctrl Pts',(-54.3536893846595,-14.9794076116576,
6.));
#62317=CARTESIAN_POINT('Ctrl Pts',(-54.360737149428,-14.9681457923566,6.));
#62318=CARTESIAN_POINT('Ctrl Pts',(-54.3676105396868,-14.9567832871792,
6.));
#62319=CARTESIAN_POINT('Ctrl Pts',(-54.3954330978975,-14.9107893962733,
6.));
#62320=CARTESIAN_POINT('Ctrl Pts',(-54.4204206822397,-14.8631190273978,
6.));
#62321=CARTESIAN_POINT('Ctrl Pts',(-54.4425345345564,-14.8140965424809,
6.));
#62322=CARTESIAN_POINT('Ctrl Pts',(-54.4509995916475,-14.7953310136339,
6.));
#62323=CARTESIAN_POINT('Ctrl Pts',(-54.4590431897372,-14.7763669364333,
6.));
#62324=CARTESIAN_POINT('Ctrl Pts',(-54.466661705721,-14.757221110189,6.));
#62325=CARTESIAN_POINT('Ctrl Pts',(-54.4721419467216,-14.7434489080701,
6.));
#62326=CARTESIAN_POINT('Ctrl Pts',(-54.4774022168759,-14.7295826467956,
6.));
#62327=CARTESIAN_POINT('Ctrl Pts',(-54.4824408848208,-14.7156283850094,
6.));
#62328=CARTESIAN_POINT('Ctrl Pts',(-54.4863313549552,-14.7048539820679,
6.));
#62329=CARTESIAN_POINT('Ctrl Pts',(-54.4900897012811,-14.6940267512127,
6.));
#62330=CARTESIAN_POINT('Ctrl Pts',(-54.4937105016092,-14.6831642693933,
6.));
#62331=CARTESIAN_POINT('Ctrl Pts',(-54.5116283442986,-14.6294103413058,
6.));
#62332=CARTESIAN_POINT('Ctrl Pts',(-54.5262131829608,-14.574710406265,6.));
#62333=CARTESIAN_POINT('Ctrl Pts',(-54.5374265846656,-14.5194236085091,
6.));
#62334=CARTESIAN_POINT('Ctrl Pts',(-54.5484779141294,-14.464935895228,6.));
#62335=CARTESIAN_POINT('Ctrl Pts',(-54.5562549501662,-14.4098769850162,
6.));
#62336=CARTESIAN_POINT('Ctrl Pts',(-54.5606770668673,-14.3545607001907,
6.));
#62337=CARTESIAN_POINT('Ctrl Pts',(-54.5629861190299,-14.3256767525837,
6.));
#62338=CARTESIAN_POINT('Ctrl Pts',(-54.5643796851133,-14.2967222396842,
6.));
#62339=CARTESIAN_POINT('Ctrl Pts',(-54.5648408789288,-14.2677401408304,
6.));
#62340=CARTESIAN_POINT('Ctrl Pts',(-54.565088353036,-14.2521885033312,6.));
#62341=CARTESIAN_POINT('Ctrl Pts',(-54.5650672991614,-14.2366289098601,
6.));
#62342=CARTESIAN_POINT('Ctrl Pts',(-54.564774627536,-14.2210679501474,6.));
#62343=CARTESIAN_POINT('Ctrl Pts',(-54.5645665072061,-14.2100024699717,
6.));
#62344=CARTESIAN_POINT('Ctrl Pts',(-54.5642210307075,-14.1989362982813,
6.));
#62345=CARTESIAN_POINT('Ctrl Pts',(-54.5637369787213,-14.1878718044098,
6.));
#62346=CARTESIAN_POINT('Ctrl Pts',(-54.5633114560902,-14.1781451785949,
6.));
#62347=CARTESIAN_POINT('Ctrl Pts',(-54.5627792671646,-14.1684296794191,
6.));
#62348=CARTESIAN_POINT('Ctrl Pts',(-54.5621402322801,-14.1587275142813,
6.));
#62349=CARTESIAN_POINT('Ctrl Pts',(-54.5589760897247,-14.1106878307941,
6.));
#62350=CARTESIAN_POINT('Ctrl Pts',(-54.553194193763,-14.0629716935933,6.));
#62351=CARTESIAN_POINT('Ctrl Pts',(-54.5447557136211,-14.0157777529758,
6.));
#62352=CARTESIAN_POINT('Ctrl Pts',(-54.5351507946184,-13.9620602624519,
6.));
#62353=CARTESIAN_POINT('Ctrl Pts',(-54.5221058408493,-13.9090185683991,
6.));
#62354=CARTESIAN_POINT('Ctrl Pts',(-54.5058712195205,-13.8568507922243,
6.));
#62355=CARTESIAN_POINT('Ctrl Pts',(-54.4900017008414,-13.8058562244003,
6.));
#62356=CARTESIAN_POINT('Ctrl Pts',(-54.4710837860606,-13.7556960237054,
6.));
#62357=CARTESIAN_POINT('Ctrl Pts',(-54.449305884132,-13.7065589746003,6.));
#62358=CARTESIAN_POINT('Ctrl Pts',(-54.4439733588473,-13.6945273033388,
6.));
#62359=CARTESIAN_POINT('Ctrl Pts',(-54.4384691647044,-13.6825570212273,
6.));
#62360=CARTESIAN_POINT('Ctrl Pts',(-54.4327956995134,-13.6706510067857,
6.));
#62361=CARTESIAN_POINT('Ctrl Pts',(-54.4285108294522,-13.6616590198587,
6.));
#62362=CARTESIAN_POINT('Ctrl Pts',(-54.4241301793919,-13.652705501481,6.));
#62363=CARTESIAN_POINT('Ctrl Pts',(-54.4196602351581,-13.6438018793311,
6.));
#62364=CARTESIAN_POINT('Ctrl Pts',(-54.3938099878638,-13.5923111173985,
6.));
#62365=CARTESIAN_POINT('Ctrl Pts',(-54.3649324447925,-13.5423928808473,
6.));
#62366=CARTESIAN_POINT('Ctrl Pts',(-54.3333070254867,-13.4942625535239,
6.));
#62367=CARTESIAN_POINT('Ctrl Pts',(-54.301002857855,-13.4450992476719,6.));
#62368=CARTESIAN_POINT('Ctrl Pts',(-54.2658311993318,-13.3978004684424,
6.));
#62369=CARTESIAN_POINT('Ctrl Pts',(-54.2280361920572,-13.3526057240926,
6.));
#62370=CARTESIAN_POINT('Ctrl Pts',(-54.1899071161637,-13.3070115051319,
6.));
#62371=CARTESIAN_POINT('Ctrl Pts',(-54.1491075472883,-13.2635576362936,
6.));
#62372=CARTESIAN_POINT('Ctrl Pts',(-54.1058416126673,-13.2225152020661,
6.));
#62373=CARTESIAN_POINT('Ctrl Pts',(-54.0960379392223,-13.2132153539042,
6.));
#62374=CARTESIAN_POINT('Ctrl Pts',(-54.0861045521206,-13.2040370185881,
6.));
#62375=CARTESIAN_POINT('Ctrl Pts',(-54.076063979376,-13.1950014469293,6.));
#62376=CARTESIAN_POINT('Ctrl Pts',(-54.0308409078756,-13.1543049335365,
6.));
#62377=CARTESIAN_POINT('Ctrl Pts',(-53.9833737358298,-13.1164303526698,
6.));
#62378=CARTESIAN_POINT('Ctrl Pts',(-53.9339288505494,-13.0816212827293,
6.));
#62379=CARTESIAN_POINT('Ctrl Pts',(-53.8849184368331,-13.0471180796338,
6.));
#62380=CARTESIAN_POINT('Ctrl Pts',(-53.8339641911266,-13.0156258219973,
6.));
#62381=CARTESIAN_POINT('Ctrl Pts',(-53.7812837559444,-12.9874094817676,
6.));
#62382=CARTESIAN_POINT('Ctrl Pts',(-53.7426834463104,-12.9667346436454,
6.));
#62383=CARTESIAN_POINT('Ctrl Pts',(-53.7031554636913,-12.9478191086954,
6.));
#62384=CARTESIAN_POINT('Ctrl Pts',(-53.6627743368928,-12.9307811146157,
6.));
#62385=CARTESIAN_POINT('Ctrl Pts',(-53.6403329837275,-12.921312442672,6.));
#62386=CARTESIAN_POINT('Ctrl Pts',(-53.6176279860555,-12.912423887492,6.));
#62387=CARTESIAN_POINT('Ctrl Pts',(-53.5946794545979,-12.9041113494969,
6.));
#62388=CARTESIAN_POINT('Ctrl Pts',(-52.7966221146314,-12.9064860705774,
6.));
#62389=CARTESIAN_POINT('Ctrl Pts',(-52.7392734478413,-12.9274410373818,
6.));
#62390=CARTESIAN_POINT('Ctrl Pts',(-52.6834091366923,-12.9520243011176,
6.));
#62391=CARTESIAN_POINT('Ctrl Pts',(-52.6292438196105,-12.9799599642101,
6.));
#62392=CARTESIAN_POINT('Ctrl Pts',(-52.579017857924,-13.0058639119715,6.));
#62393=CARTESIAN_POINT('Ctrl Pts',(-52.5302525542186,-13.0346514876413,
6.));
#62394=CARTESIAN_POINT('Ctrl Pts',(-52.4831464368575,-13.0661326532274,
6.));
#62395=CARTESIAN_POINT('Ctrl Pts',(-52.4717767044507,-13.0737310809607,
6.));
#62396=CARTESIAN_POINT('Ctrl Pts',(-52.4605034750011,-13.0814868963895,
6.));
#62397=CARTESIAN_POINT('Ctrl Pts',(-52.4493421044387,-13.0893884562007,
6.));
#62398=CARTESIAN_POINT('Ctrl Pts',(-52.4002195795838,-13.1241641646178,
6.));
#62399=CARTESIAN_POINT('Ctrl Pts',(-52.3531999207051,-13.1617999131249,
6.));
#62400=CARTESIAN_POINT('Ctrl Pts',(-52.308512601551,-13.2020507624865,6.));
#62401=CARTESIAN_POINT('Ctrl Pts',(-52.2809299424638,-13.2268950690355,
6.));
#62402=CARTESIAN_POINT('Ctrl Pts',(-52.2542366022566,-13.2527364020133,
6.));
#62403=CARTESIAN_POINT('Ctrl Pts',(-52.2284950356863,-13.2795223256619,
6.));
#62404=CARTESIAN_POINT('Ctrl Pts',(-52.2196863975423,-13.2886883376888,
6.));
#62405=CARTESIAN_POINT('Ctrl Pts',(-52.2109892711622,-13.2979649851678,
6.));
#62406=CARTESIAN_POINT('Ctrl Pts',(-52.2024063576282,-13.3073502398414,
6.));
#62407=CARTESIAN_POINT('Ctrl Pts',(-52.1943778462967,-13.3161292661239,
6.));
#62408=CARTESIAN_POINT('Ctrl Pts',(-52.1864544231925,-13.3249977568293,
6.));
#62409=CARTESIAN_POINT('Ctrl Pts',(-52.1786418093699,-13.3339491349468,
6.));
#62410=CARTESIAN_POINT('Ctrl Pts',(-52.1399699653664,-13.3782577755679,
6.));
#62411=CARTESIAN_POINT('Ctrl Pts',(-52.1039774129608,-13.4246301646367,
6.));
#62412=CARTESIAN_POINT('Ctrl Pts',(-52.0708793546133,-13.4728370626374,
6.));
#62413=CARTESIAN_POINT('Ctrl Pts',(-52.0386265755499,-13.5198128221889,
6.));
#62414=CARTESIAN_POINT('Ctrl Pts',(-52.009121966523,-13.5685314991956,6.));
#62415=CARTESIAN_POINT('Ctrl Pts',(-51.982610320354,-13.6187990638912,6.));
#62416=CARTESIAN_POINT('Ctrl Pts',(-51.968236469053,-13.6460526903011,6.));
#62417=CARTESIAN_POINT('Ctrl Pts',(-51.9547432274292,-13.6737618469832,
6.));
#62418=CARTESIAN_POINT('Ctrl Pts',(-51.9421760191472,-13.7018965351452,
6.));
#62419=CARTESIAN_POINT('Ctrl Pts',(-51.9317203742409,-13.7253039858987,
6.));
#62420=CARTESIAN_POINT('Ctrl Pts',(-51.9219057931392,-13.7490060035482,
6.));
#62421=CARTESIAN_POINT('Ctrl Pts',(-51.9127610531855,-13.7729853084091,
6.));
#62422=CARTESIAN_POINT('Ctrl Pts',(-51.9088519886743,-13.7832356435864,
6.));
#62423=CARTESIAN_POINT('Ctrl Pts',(-51.9050650272361,-13.7935379060622,
6.));
#62424=CARTESIAN_POINT('Ctrl Pts',(-51.9014081870189,-13.8038737999324,
6.));
#62425=CARTESIAN_POINT('Ctrl Pts',(-51.8844806830126,-13.8517186262041,
6.));
#62426=CARTESIAN_POINT('Ctrl Pts',(-51.8703064127133,-13.900364924046,6.));
#62427=CARTESIAN_POINT('Ctrl Pts',(-51.8590515016651,-13.9496698048621,
6.));
#62428=CARTESIAN_POINT('Ctrl Pts',(-51.8464743828166,-14.0047669391872,
6.));
#62429=CARTESIAN_POINT('Ctrl Pts',(-51.8375421395456,-14.0606874236398,
6.));
#62430=CARTESIAN_POINT('Ctrl Pts',(-51.8321648228283,-14.1170948620909,
6.));
#62431=CARTESIAN_POINT('Ctrl Pts',(-51.8276016369014,-14.1649621614985,
6.));
#62432=CARTESIAN_POINT('Ctrl Pts',(-51.8255995131662,-14.2131805783548,
6.));
#62433=CARTESIAN_POINT('Ctrl Pts',(-51.8261319285703,-14.2615368910676,
6.));
#62434=CARTESIAN_POINT('Ctrl Pts',(-51.826278300178,-14.2748310053593,6.));
#62435=CARTESIAN_POINT('Ctrl Pts',(-51.8266163768541,-14.2881354730497,
6.));
#62436=CARTESIAN_POINT('Ctrl Pts',(-51.8271459227333,-14.3014456837575,
6.));
#62437=CARTESIAN_POINT('Ctrl Pts',(-51.8275582116147,-14.3118086232139,
6.));
#62438=CARTESIAN_POINT('Ctrl Pts',(-51.8280867629368,-14.3221768232919,
6.));
#62439=CARTESIAN_POINT('Ctrl Pts',(-51.8287302146405,-14.3325312126322,
6.));
#62440=CARTESIAN_POINT('Ctrl Pts',(-51.8321732391036,-14.3879361724649,
6.));
#62441=CARTESIAN_POINT('Ctrl Pts',(-51.8389046601932,-14.4430495470179,
6.));
#62442=CARTESIAN_POINT('Ctrl Pts',(-51.8488297362242,-14.4975564316833,
6.));
#62443=CARTESIAN_POINT('Ctrl Pts',(-51.8586992382113,-14.5517581128431,
6.));
#62444=CARTESIAN_POINT('Ctrl Pts',(-51.8717272178035,-14.6053611705386,
6.));
#62445=CARTESIAN_POINT('Ctrl Pts',(-51.8878674165357,-14.65803601794,6.));
#62446=CARTESIAN_POINT('Ctrl Pts',(-51.9028425534804,-14.7069085917211,
6.));
#62447=CARTESIAN_POINT('Ctrl Pts',(-51.9204975501467,-14.7549825914389,
6.));
#62448=CARTESIAN_POINT('Ctrl Pts',(-51.9408266061655,-14.8019671660641,
6.));
#62449=CARTESIAN_POINT('Ctrl Pts',(-51.946048451174,-14.8140359097509,6.));
#62450=CARTESIAN_POINT('Ctrl Pts',(-51.9514489311129,-14.8260366549904,
6.));
#62451=CARTESIAN_POINT('Ctrl Pts',(-51.9570156117182,-14.8379381689157,
6.));
#62452=CARTESIAN_POINT('Ctrl Pts',(-51.9795172113314,-14.8860463899781,
6.));
#62453=CARTESIAN_POINT('Ctrl Pts',(-52.0047624527053,-14.9326133843135,
6.));
#62454=CARTESIAN_POINT('Ctrl Pts',(-52.0326996003995,-14.9773433960441,
6.));
#62455=CARTESIAN_POINT('Ctrl Pts',(-52.0596890512109,-15.0205560555688,
6.));
#62456=CARTESIAN_POINT('Ctrl Pts',(-52.0891914487675,-15.0620548998265,
6.));
#62457=CARTESIAN_POINT('Ctrl Pts',(-52.1211934155095,-15.1015390599239,
6.));
#62458=CARTESIAN_POINT('Ctrl Pts',(-52.1435818547289,-15.1291620096505,
6.));
#62459=CARTESIAN_POINT('Ctrl Pts',(-52.167194352484,-15.1557982112222,6.));
#62460=CARTESIAN_POINT('Ctrl Pts',(-52.1920344148669,-15.1813316631752,
6.));
#62461=CARTESIAN_POINT('Ctrl Pts',(-52.2060464360847,-15.1957348182485,
6.));
#62462=CARTESIAN_POINT('Ctrl Pts',(-52.2204492103834,-15.2097868473553,
6.));
#62463=CARTESIAN_POINT('Ctrl Pts',(-52.2352263046383,-15.223479246524,6.));
#62464=CARTESIAN_POINT('Origin',(-53.1951359564886,-14.3971354987959,0.895788276411275));
#62465=CARTESIAN_POINT('Ctrl Pts',(-54.7400287307462,-14.397884086359,2.14578827641127));
#62466=CARTESIAN_POINT('Ctrl Pts',(-54.7403302631026,-14.4458093584932,
2.14826884812012));
#62467=CARTESIAN_POINT('Ctrl Pts',(-54.7167366550282,-14.9990296040617,
2.17691792328789));
#62468=CARTESIAN_POINT('Ctrl Pts',(-54.0514939360651,-15.9998439808924,
2.23173550191459));
#62469=CARTESIAN_POINT('Ctrl Pts',(-52.3307400382945,-15.9953304824803,
2.31024101229136));
#62470=CARTESIAN_POINT('Ctrl Pts',(-51.3852180733225,-14.5577448223715,
2.38874652266815));
#62471=CARTESIAN_POINT('Ctrl Pts',(-52.0628629644955,-12.9760077060224,
2.46725203304492));
#62472=CARTESIAN_POINT('Ctrl Pts',(-53.7559624418889,-12.6688282037076,
2.54575754342171));
#62473=CARTESIAN_POINT('Ctrl Pts',(-54.658158616602,-13.6109326580654,2.60526962454382));
#62474=CARTESIAN_POINT('Ctrl Pts',(-54.7387317829834,-14.2566058695901,
2.63861320220701));
#62475=CARTESIAN_POINT('Ctrl Pts',(-54.7375657625992,-14.3958310564158,
2.64578827641127));
#62476=CARTESIAN_POINT('Ctrl Pts',(-54.7364807484814,-14.3955730757723,
2.10421172358873));
#62477=CARTESIAN_POINT('Ctrl Pts',(-54.7341428408094,-14.7375070363914,
2.12181148931034));
#62478=CARTESIAN_POINT('Ctrl Pts',(-54.4552744897983,-15.5924244351668,
2.16557975849088));
#62479=CARTESIAN_POINT('Ctrl Pts',(-53.0510002557363,-16.2080728204287,
2.23551653113034));
#62480=CARTESIAN_POINT('Ctrl Pts',(-51.605113325188,-15.2764851170283,2.31402204150712));
#62481=CARTESIAN_POINT('Ctrl Pts',(-51.5846111642588,-13.5555692706413,
2.3925275518839));
#62482=CARTESIAN_POINT('Ctrl Pts',(-53.0087575469087,-12.5897418281553,
2.47103306226068));
#62483=CARTESIAN_POINT('Ctrl Pts',(-54.4388957804213,-13.178381042198,2.54159445282895));
#62484=CARTESIAN_POINT('Ctrl Pts',(-54.7344163061994,-14.0445046478413,
2.5859873399383));
#62485=CARTESIAN_POINT('Ctrl Pts',(-54.73716587472,-14.3983674417199,2.60421172358873));
#62486=CARTESIAN_POINT('Ctrl Pts',(-52.2370198037663,-15.2223467977324,
2.));
#62487=CARTESIAN_POINT('Ctrl Pts',(-51.9656547514336,-14.9072768995629,
2.02616850345893));
#62488=CARTESIAN_POINT('Ctrl Pts',(-51.7623579720558,-13.9937953994845,
2.07850551037678));
#62489=CARTESIAN_POINT('Ctrl Pts',(-52.7425844632288,-12.9776340948197,
2.15701102075356));
#62490=CARTESIAN_POINT('Ctrl Pts',(-54.1289211584486,-13.2376188657684,
2.23551653113034));
#62491=CARTESIAN_POINT('Ctrl Pts',(-54.6776801082256,-14.5359758627139,
2.31402204150712));
#62492=CARTESIAN_POINT('Ctrl Pts',(-53.8969277031993,-15.7105670448821,
2.3925275518839));
#62493=CARTESIAN_POINT('Ctrl Pts',(-52.486757059174,-15.7068681992943,2.47103306226068));
#62494=CARTESIAN_POINT('Ctrl Pts',(-51.7118947618914,-14.5287560364896,
2.54953857263746));
#62495=CARTESIAN_POINT('Ctrl Pts',(-52.2672298007042,-13.2325106809332,
2.62804408301423));
#62496=CARTESIAN_POINT('Ctrl Pts',(-53.6547374411216,-12.9807747893732,
2.70654959339101));
#62497=CARTESIAN_POINT('Ctrl Pts',(-54.6300613996379,-13.9992418052107,
2.78505510376779));
#62498=CARTESIAN_POINT('Ctrl Pts',(-54.3185111760821,-15.374560833818,2.86356061414457));
#62499=CARTESIAN_POINT('Ctrl Pts',(-52.9994908161496,-15.8732958581993,
2.94206612452135));
#62500=CARTESIAN_POINT('Ctrl Pts',(-51.855929934815,-15.0481780331667,3.02057163489813));
#62501=CARTESIAN_POINT('Ctrl Pts',(-51.9134007191539,-13.639188362749,3.09907714527491));
#62502=CARTESIAN_POINT('Ctrl Pts',(-53.1203622018242,-12.909944412367,3.17758265565169));
#62503=CARTESIAN_POINT('Ctrl Pts',(-54.394382532434,-13.5144484306959,3.25608816602847));
#62504=CARTESIAN_POINT('Ctrl Pts',(-54.592890039674,-14.9105673726083,3.33459367640525));
#62505=CARTESIAN_POINT('Ctrl Pts',(-53.5378584472409,-15.8462283160989,
3.41309918678203));
#62506=CARTESIAN_POINT('Ctrl Pts',(-52.1754651814132,-15.4823084146089,
3.49160469715881));
#62507=CARTESIAN_POINT('Ctrl Pts',(-51.7275369059285,-14.1451796218823,
3.57011020753559));
#62508=CARTESIAN_POINT('Ctrl Pts',(-52.5957863501673,-13.0340108603602,
3.64861571791237));
#62509=CARTESIAN_POINT('Ctrl Pts',(-54.0015467695738,-13.1453246755956,
3.72712122828915));
#62510=CARTESIAN_POINT('Ctrl Pts',(-54.6840988007339,-14.3792921998829,
3.80562673866593));
#62511=CARTESIAN_POINT('Ctrl Pts',(-54.0313135549908,-15.6292620174801,
3.8841322490427));
#62512=CARTESIAN_POINT('Ctrl Pts',(-52.6286243599758,-15.7742314816778,
3.96263775941949));
#62513=CARTESIAN_POINT('Ctrl Pts',(-51.7339962327512,-14.6841885294771,
4.04114326979626));
#62514=CARTESIAN_POINT('Ctrl Pts',(-52.1497529463451,-13.3367095952976,
4.11964878017305));
#62515=CARTESIAN_POINT('Ctrl Pts',(-53.5030339960932,-12.9402458213458,
4.19815429054982));
#62516=CARTESIAN_POINT('Ctrl Pts',(-54.5801847638567,-13.8503553460012,
4.27665980092661));
#62517=CARTESIAN_POINT('Ctrl Pts',(-54.41519083395,-15.2508303100966,4.35516531130338));
#62518=CARTESIAN_POINT('Ctrl Pts',(-53.1560226839298,-15.8856914730379,
4.43367082168017));
#62519=CARTESIAN_POINT('Ctrl Pts',(-51.9319322483355,-15.1855802477899,
4.51217633205694));
#62520=CARTESIAN_POINT('Ctrl Pts',(-51.8407129256901,-13.7783730316415,
4.59068184243372));
#62521=CARTESIAN_POINT('Ctrl Pts',(-52.9641723835949,-12.9260866978538,
4.6691873528105));
#62522=CARTESIAN_POINT('Ctrl Pts',(-54.2947654505407,-13.3930719178224,
4.74769286318728));
#62523=CARTESIAN_POINT('Ctrl Pts',(-54.639184673062,-14.7605251935738,4.82619837356406));
#62524=CARTESIAN_POINT('Ctrl Pts',(-53.6885466200216,-15.8020820199203,
4.90470388394084));
#62525=CARTESIAN_POINT('Ctrl Pts',(-52.2954062665963,-15.5836492690769,
4.98320939431762));
#62526=CARTESIAN_POINT('Ctrl Pts',(-51.7091646625421,-14.3011230348445,
5.0617149046944));
#62527=CARTESIAN_POINT('Ctrl Pts',(-52.455577895988,-13.1047025120629,5.14022041507118));
#62528=CARTESIAN_POINT('Ctrl Pts',(-53.8652434689878,-13.0673677185784,
5.21872592544796));
#62529=CARTESIAN_POINT('Ctrl Pts',(-54.6739425216854,-14.2225980750992,
5.29723143582473));
#62530=CARTESIAN_POINT('Ctrl Pts',(-54.1564090232193,-15.5343621736369,
5.37573694620152));
#62531=CARTESIAN_POINT('Ctrl Pts',(-52.7767903419413,-15.826225464705,5.45424245657829));
#62532=CARTESIAN_POINT('Ctrl Pts',(-51.7723391952092,-14.8364647334447,
5.53274796695508));
#62533=CARTESIAN_POINT('Ctrl Pts',(-52.0439156164789,-13.4526673224972,
5.61125347733185));
#62534=CARTESIAN_POINT('Ctrl Pts',(-53.3478744097592,-12.9159632016583,
5.68975898770863));
#62535=CARTESIAN_POINT('Ctrl Pts',(-54.5149728893469,-13.707465612061,5.76826449808541));
#62536=CARTESIAN_POINT('Ctrl Pts',(-54.498171162037,-15.1177692904017,5.84677000846219));
#62537=CARTESIAN_POINT('Ctrl Pts',(-53.3132562085964,-15.88121138355,5.92527551883898));
#62538=CARTESIAN_POINT('Ctrl Pts',(-52.0214443153046,-15.3148691319142,
6.00378102921575));
#62539=CARTESIAN_POINT('Ctrl Pts',(-51.7841832172828,-13.9230591799233,
6.08228653959254));
#62540=CARTESIAN_POINT('Ctrl Pts',(-52.4668366999413,-13.2829324314546,
6.13462354651038));
#62541=CARTESIAN_POINT('Ctrl Pts',(-52.8685508929576,-13.1755371825403,
6.16079204996931));
#62542=CARTESIAN_POINT('Ctrl Pts',(-52.166679656532,-15.2829297282066,1.94640265001023));
#62543=CARTESIAN_POINT('Ctrl Pts',(-51.8753923247543,-14.9447289570595,
1.97257115346916));
#62544=CARTESIAN_POINT('Ctrl Pts',(-51.6571705017343,-13.9641841650946,
2.02490816038701));
#62545=CARTESIAN_POINT('Ctrl Pts',(-52.7093603717901,-12.8734213253437,
2.10341367076379));
#62546=CARTESIAN_POINT('Ctrl Pts',(-54.1974750476659,-13.152492891787,2.18191918114057));
#62547=CARTESIAN_POINT('Ctrl Pts',(-54.7865211643106,-14.5461688352594,
2.26042469151734));
#62548=CARTESIAN_POINT('Ctrl Pts',(-53.9484497808213,-15.8069926902189,
2.33893020189413));
#62549=CARTESIAN_POINT('Ctrl Pts',(-52.4347513855474,-15.8030222936896,
2.4174357122709));
#62550=CARTESIAN_POINT('Ctrl Pts',(-51.6030025323684,-14.5384189651169,
2.49594122264769));
#62551=CARTESIAN_POINT('Ctrl Pts',(-52.199107521968,-13.1470096892963,2.57444673302446));
#62552=CARTESIAN_POINT('Ctrl Pts',(-53.688479108044,-12.8767925941513,2.65295224340125));
#62553=CARTESIAN_POINT('Ctrl Pts',(-54.7354065257529,-13.9700304189807,
2.73145775377802));
#62554=CARTESIAN_POINT('Ctrl Pts',(-54.4009838263146,-15.4463185656761,
2.80996326415481));
#62555=CARTESIAN_POINT('Ctrl Pts',(-52.9851275179857,-15.9816682478379,
2.88846877453158));
#62556=CARTESIAN_POINT('Ctrl Pts',(-51.757612055011,-15.0959743547226,2.96697428490837));
#62557=CARTESIAN_POINT('Ctrl Pts',(-51.8193020599743,-13.5835436342954,
3.04547979528514));
#62558=CARTESIAN_POINT('Ctrl Pts',(-53.1148726827325,-12.8007622013296,
3.12398530566192));
#62559=CARTESIAN_POINT('Ctrl Pts',(-54.4824252822431,-13.4496459136362,
3.2024908160387));
#62560=CARTESIAN_POINT('Ctrl Pts',(-54.695506228462,-14.9482610003549,3.28099632641548));
#62561=CARTESIAN_POINT('Ctrl Pts',(-53.5630194367425,-15.9526135407249,
3.35950183679226));
#62562=CARTESIAN_POINT('Ctrl Pts',(-52.1006059983742,-15.5619764407204,
3.43800734716904));
#62563=CARTESIAN_POINT('Ctrl Pts',(-51.6197930452243,-14.1266822680611,
3.51651285754582));
#62564=CARTESIAN_POINT('Ctrl Pts',(-52.5517850676155,-12.9339369940614,
3.5950183679226));
#62565=CARTESIAN_POINT('Ctrl Pts',(-54.0607494614004,-13.0534229188377,
3.67352387829937));
#62566=CARTESIAN_POINT('Ctrl Pts',(-54.7934110854636,-14.3779822331642,
3.75202938867616));
#62567=CARTESIAN_POINT('Ctrl Pts',(-54.0927015769186,-15.7197186499972,
3.83053489905293));
#62568=CARTESIAN_POINT('Ctrl Pts',(-52.5870338816236,-15.8753310549564,
3.90904040942972));
#62569=CARTESIAN_POINT('Ctrl Pts',(-51.626726583862,-14.7052625426693,3.98754591980649));
#62570=CARTESIAN_POINT('Ctrl Pts',(-52.0730060982299,-13.2588583723836,
4.06605143018328));
#62571=CARTESIAN_POINT('Ctrl Pts',(-53.5256383467009,-12.8332881898262,
4.14455694056005));
#62572=CARTESIAN_POINT('Ctrl Pts',(-54.681868194159,-13.8102134526169,4.22306245093684));
#62573=CARTESIAN_POINT('Ctrl Pts',(-54.5047612262982,-15.3135043591139,
4.30156796131361));
#62574=CARTESIAN_POINT('Ctrl Pts',(-53.1531511809886,-15.9949738873852,
4.38007347169039));
#62575=CARTESIAN_POINT('Ctrl Pts',(-51.8391940823356,-15.2434639600858,
4.45857898206717));
#62576=CARTESIAN_POINT('Ctrl Pts',(-51.741277888369,-13.7329465529009,4.53708449244395));
#62577=CARTESIAN_POINT('Ctrl Pts',(-52.9472161808664,-12.8180895735458,
4.61559000282073));
#62578=CARTESIAN_POINT('Ctrl Pts',(-54.3754948070962,-13.3193585377509,
4.69409551319751));
#62579=CARTESIAN_POINT('Ctrl Pts',(-54.7451995847704,-14.787203466935,4.77260102357429));
#62580=CARTESIAN_POINT('Ctrl Pts',(-53.7247703895732,-15.905226241914,4.85110653395107));
#62581=CARTESIAN_POINT('Ctrl Pts',(-52.2293525645705,-15.6707572392952,
4.92961204432785));
#62582=CARTESIAN_POINT('Ctrl Pts',(-51.6000720026333,-14.2940742748049,
5.00811755470463));
#62583=CARTESIAN_POINT('Ctrl Pts',(-52.4012832024729,-13.0098184770542,
5.08662306508141));
#62584=CARTESIAN_POINT('Ctrl Pts',(-53.9144394469056,-12.9697427477624,
5.16512857545819));
#62585=CARTESIAN_POINT('Ctrl Pts',(-54.78250918266,-14.2097844010517,5.24363408583497));
#62586=CARTESIAN_POINT('Ctrl Pts',(-54.2269809354599,-15.6178517291775,
5.32213959621174));
#62587=CARTESIAN_POINT('Ctrl Pts',(-52.746077476869,-15.9311421789546,5.40064510658853));
#62588=CARTESIAN_POINT('Ctrl Pts',(-51.6678844969053,-14.8687181120791,
5.4791506169653));
#62589=CARTESIAN_POINT('Ctrl Pts',(-51.9593987152814,-13.3833291421626,
5.55765612734209));
#62590=CARTESIAN_POINT('Ctrl Pts',(-53.3590877112581,-12.80722286035,5.63616163771886));
#62591=CARTESIAN_POINT('Ctrl Pts',(-54.611868786487,-13.6568334614203,5.71466714809565));
#62592=CARTESIAN_POINT('Ctrl Pts',(-54.5938335594918,-15.1706746577306,
5.79317265847242));
#62593=CARTESIAN_POINT('Ctrl Pts',(-53.3219280130545,-15.9901648918943,
5.87167816884921));
#62594=CARTESIAN_POINT('Ctrl Pts',(-51.9352776823614,-15.3822445943693,
5.95018367922597));
#62595=CARTESIAN_POINT('Ctrl Pts',(-51.680598048476,-13.8882548422916,6.02868918960277));
#62596=CARTESIAN_POINT('Ctrl Pts',(-52.4133685721046,-13.2011331552573,
6.08102619652061));
#62597=CARTESIAN_POINT('Ctrl Pts',(-52.8445746335155,-13.0858534785527,
6.10719469997954));
#62598=CARTESIAN_POINT('Ctrl Pts',(-52.0963395092977,-15.3435126586808,
1.89280530002046));
#62599=CARTESIAN_POINT('Ctrl Pts',(-51.7851298980751,-14.9821810145562,
1.91897380347939));
#62600=CARTESIAN_POINT('Ctrl Pts',(-51.5519830314128,-13.9345729307046,
1.97131081039724));
#62601=CARTESIAN_POINT('Ctrl Pts',(-52.6761362803514,-12.7692085558677,
2.04981632077402));
#62602=CARTESIAN_POINT('Ctrl Pts',(-54.2660289368831,-13.0673669178057,
2.1283218311508));
#62603=CARTESIAN_POINT('Ctrl Pts',(-54.8953622203958,-14.5563618078048,
2.20682734152757));
#62604=CARTESIAN_POINT('Ctrl Pts',(-53.9999718584432,-15.9034183355557,
2.28533285190436));
#62605=CARTESIAN_POINT('Ctrl Pts',(-52.382745711921,-15.899176388085,2.36383836228113));
#62606=CARTESIAN_POINT('Ctrl Pts',(-51.4941103028454,-14.5480818937442,
2.44234387265792));
#62607=CARTESIAN_POINT('Ctrl Pts',(-52.1309852432317,-13.0615086976593,
2.52084938303469));
#62608=CARTESIAN_POINT('Ctrl Pts',(-53.7222207749664,-12.7728103989294,
2.59935489341148));
#62609=CARTESIAN_POINT('Ctrl Pts',(-54.8407516518678,-13.9408190327507,
2.67786040378825));
#62610=CARTESIAN_POINT('Ctrl Pts',(-54.483456476547,-15.5180762975342,2.75636591416503));
#62611=CARTESIAN_POINT('Ctrl Pts',(-52.9707642198219,-16.0900406374764,
2.83487142454181));
#62612=CARTESIAN_POINT('Ctrl Pts',(-51.6592941752071,-15.1437706762785,
2.91337693491859));
#62613=CARTESIAN_POINT('Ctrl Pts',(-51.7252034007948,-13.5278989058417,
2.99188244529537));
#62614=CARTESIAN_POINT('Ctrl Pts',(-53.1093831636409,-12.6915799902922,
3.07038795567215));
#62615=CARTESIAN_POINT('Ctrl Pts',(-54.5704680320522,-13.3848433965765,
3.14889346604893));
#62616=CARTESIAN_POINT('Ctrl Pts',(-54.7981224172499,-14.9859546281015,
3.22739897642571));
#62617=CARTESIAN_POINT('Ctrl Pts',(-53.5881804262442,-16.0589987653509,
3.30590448680249));
#62618=CARTESIAN_POINT('Ctrl Pts',(-52.0257468153352,-15.6416444668319,
3.38440999717927));
#62619=CARTESIAN_POINT('Ctrl Pts',(-51.5120491845202,-14.10818491424,3.46291550755605));
#62620=CARTESIAN_POINT('Ctrl Pts',(-52.5077837850636,-12.8338631277627,
3.54142101793282));
#62621=CARTESIAN_POINT('Ctrl Pts',(-54.1199521532269,-12.9615211620797,
3.61992652830961));
#62622=CARTESIAN_POINT('Ctrl Pts',(-54.9027233701933,-14.3766722664456,
3.69843203868638));
#62623=CARTESIAN_POINT('Ctrl Pts',(-54.1540895988463,-15.8101752825143,
3.77693754906317));
#62624=CARTESIAN_POINT('Ctrl Pts',(-52.5454434032715,-15.9764306282351,
3.85544305943994));
#62625=CARTESIAN_POINT('Ctrl Pts',(-51.5194569349729,-14.7263365558616,
3.93394856981673));
#62626=CARTESIAN_POINT('Ctrl Pts',(-51.9962592501148,-13.1810071494696,
4.0124540801935));
#62627=CARTESIAN_POINT('Ctrl Pts',(-53.5482426973085,-12.7263305583065,
4.09095959057029));
#62628=CARTESIAN_POINT('Ctrl Pts',(-54.7835516244614,-13.7700715592326,
4.16946510094706));
#62629=CARTESIAN_POINT('Ctrl Pts',(-54.5943316186465,-15.3761784081312,
4.24797061132385));
#62630=CARTESIAN_POINT('Ctrl Pts',(-53.1502796780473,-16.1042563017325,
4.32647612170062));
#62631=CARTESIAN_POINT('Ctrl Pts',(-51.7464559163358,-15.3013476723818,
4.4049816320774));
#62632=CARTESIAN_POINT('Ctrl Pts',(-51.6418428510479,-13.6875200741603,
4.48348714245418));
#62633=CARTESIAN_POINT('Ctrl Pts',(-52.9302599781378,-12.7100924492378,
4.56199265283096));
#62634=CARTESIAN_POINT('Ctrl Pts',(-54.4562241636517,-13.2456451576794,
4.64049816320774));
#62635=CARTESIAN_POINT('Ctrl Pts',(-54.8512144964788,-14.8138817402962,
4.71900367358453));
#62636=CARTESIAN_POINT('Ctrl Pts',(-53.7609941591247,-16.0083704639078,
4.79750918396129));
#62637=CARTESIAN_POINT('Ctrl Pts',(-52.1632988625446,-15.7578652095136,
4.87601469433808));
#62638=CARTESIAN_POINT('Ctrl Pts',(-51.4909793427245,-14.2870255147652,
4.95452020471486));
#62639=CARTESIAN_POINT('Ctrl Pts',(-52.3469885089578,-12.9149344420456,
5.03302571509164));
#62640=CARTESIAN_POINT('Ctrl Pts',(-53.9636354248233,-12.8721177769464,
5.11153122546841));
#62641=CARTESIAN_POINT('Ctrl Pts',(-54.8910758436347,-14.1969707270041,
5.1900367358452));
#62642=CARTESIAN_POINT('Ctrl Pts',(-54.2975528477005,-15.7013412847181,
5.26854224622197));
#62643=CARTESIAN_POINT('Ctrl Pts',(-52.7153646117968,-16.0360588932041,
5.34704775659876));
#62644=CARTESIAN_POINT('Ctrl Pts',(-51.5634297986012,-14.9009714907135,
5.42555326697554));
#62645=CARTESIAN_POINT('Ctrl Pts',(-51.8748818140839,-13.313990961828,5.50405877735231));
#62646=CARTESIAN_POINT('Ctrl Pts',(-53.3703010127568,-12.6984825190418,
5.58256428772909));
#62647=CARTESIAN_POINT('Ctrl Pts',(-54.7087646836272,-13.6062013107796,
5.66106979810588));
#62648=CARTESIAN_POINT('Ctrl Pts',(-54.6894959569467,-15.2235800250595,
5.73957530848265));
#62649=CARTESIAN_POINT('Ctrl Pts',(-53.3305998175127,-16.0991184002386,
5.81808081885943));
#62650=CARTESIAN_POINT('Ctrl Pts',(-51.8491110494183,-15.4496200568245,
5.89658632923621));
#62651=CARTESIAN_POINT('Ctrl Pts',(-51.5770128796692,-13.8534505046598,
5.97509183961299));
#62652=CARTESIAN_POINT('Ctrl Pts',(-52.359900444268,-13.11933387906,6.02742884653084));
#62653=CARTESIAN_POINT('Ctrl Pts',(-52.8205983740735,-12.996169774565,6.05359734998977));
#62654=CARTESIAN_POINT('Ctrl Pts',(-52.0259993620635,-15.4040955891549,
1.83920795003069));
#62655=CARTESIAN_POINT('Ctrl Pts',(-51.6948674713958,-15.0196330720529,
1.86537645348962));
#62656=CARTESIAN_POINT('Ctrl Pts',(-51.4467955610913,-13.9049616963147,
1.91771346040747));
#62657=CARTESIAN_POINT('Ctrl Pts',(-52.6429121889126,-12.6649957863916,
1.99621897078425));
#62658=CARTESIAN_POINT('Ctrl Pts',(-54.3345828261005,-12.9822409438244,
2.07472448116103));
#62659=CARTESIAN_POINT('Ctrl Pts',(-55.0042032764809,-14.5665547803503,
2.15322999153781));
#62660=CARTESIAN_POINT('Ctrl Pts',(-54.0514939360651,-15.9998439808924,
2.23173550191459));
#62661=CARTESIAN_POINT('Ctrl Pts',(-52.3307400382945,-15.9953304824803,
2.31024101229136));
#62662=CARTESIAN_POINT('Ctrl Pts',(-51.3852180733225,-14.5577448223715,
2.38874652266815));
#62663=CARTESIAN_POINT('Ctrl Pts',(-52.0628629644955,-12.9760077060224,
2.46725203304492));
#62664=CARTESIAN_POINT('Ctrl Pts',(-53.7559624418889,-12.6688282037076,
2.54575754342171));
#62665=CARTESIAN_POINT('Ctrl Pts',(-54.9460967779827,-13.9116076465207,
2.62426305379848));
#62666=CARTESIAN_POINT('Ctrl Pts',(-54.5659291267794,-15.5898340293922,
2.70276856417526));
#62667=CARTESIAN_POINT('Ctrl Pts',(-52.9564009216581,-16.198413027115,2.78127407455204));
#62668=CARTESIAN_POINT('Ctrl Pts',(-51.5609762954032,-15.1915669978344,
2.85977958492882));
#62669=CARTESIAN_POINT('Ctrl Pts',(-51.6311047416152,-13.472254177388,2.9382850953056));
#62670=CARTESIAN_POINT('Ctrl Pts',(-53.1038936445493,-12.5823977792547,
3.01679060568238));
#62671=CARTESIAN_POINT('Ctrl Pts',(-54.6585107818613,-13.3200408795168,
3.09529611605916));
#62672=CARTESIAN_POINT('Ctrl Pts',(-54.9007386060379,-15.0236482558481,
3.17380162643594));
#62673=CARTESIAN_POINT('Ctrl Pts',(-53.6133414157459,-16.165383989977,3.25230713681272));
#62674=CARTESIAN_POINT('Ctrl Pts',(-51.9508876322962,-15.7213124929433,
3.3308126471895));
#62675=CARTESIAN_POINT('Ctrl Pts',(-51.4043053238161,-14.0896875604189,
3.40931815756628));
#62676=CARTESIAN_POINT('Ctrl Pts',(-52.4637825025118,-12.7337892614639,
3.48782366794306));
#62677=CARTESIAN_POINT('Ctrl Pts',(-54.1791548450535,-12.8696194053218,
3.56632917831984));
#62678=CARTESIAN_POINT('Ctrl Pts',(-55.0120356549231,-14.3753622997269,
3.64483468869662));
#62679=CARTESIAN_POINT('Ctrl Pts',(-54.215477620774,-15.9006319150314,3.72334019907339));
#62680=CARTESIAN_POINT('Ctrl Pts',(-52.5038529249194,-16.0775302015137,
3.80184570945018));
#62681=CARTESIAN_POINT('Ctrl Pts',(-51.4121872860838,-14.7474105690538,
3.88035121982695));
#62682=CARTESIAN_POINT('Ctrl Pts',(-51.9195124019995,-13.1031559265556,
3.95885673020374));
#62683=CARTESIAN_POINT('Ctrl Pts',(-53.5708470479161,-12.6193729267869,
4.03736224058051));
#62684=CARTESIAN_POINT('Ctrl Pts',(-54.8852350547638,-13.7299296658483,
4.11586775095729));
#62685=CARTESIAN_POINT('Ctrl Pts',(-54.6839020109947,-15.4388524571486,
4.19437326133407));
#62686=CARTESIAN_POINT('Ctrl Pts',(-53.147408175106,-16.2135387160798,4.27287877171085));
#62687=CARTESIAN_POINT('Ctrl Pts',(-51.6537177503358,-15.3592313846778,
4.35138428208763));
#62688=CARTESIAN_POINT('Ctrl Pts',(-51.5424078137269,-13.6420935954197,
4.42988979246441));
#62689=CARTESIAN_POINT('Ctrl Pts',(-52.9133037754093,-12.6020953249298,
4.50839530284119));
#62690=CARTESIAN_POINT('Ctrl Pts',(-54.5369535202073,-13.171931777608,4.58690081321797));
#62691=CARTESIAN_POINT('Ctrl Pts',(-54.9572294081871,-14.8405600136574,
4.66540632359475));
#62692=CARTESIAN_POINT('Ctrl Pts',(-53.7972179286764,-16.1115146859015,
4.74391183397153));
#62693=CARTESIAN_POINT('Ctrl Pts',(-52.0972451605187,-15.8449731797319,
4.8224173443483));
#62694=CARTESIAN_POINT('Ctrl Pts',(-51.3818866828157,-14.2799767547255,
4.90092285472509));
#62695=CARTESIAN_POINT('Ctrl Pts',(-52.2926938154427,-12.820050407037,4.97942836510186));
#62696=CARTESIAN_POINT('Ctrl Pts',(-54.0128314027411,-12.7744928061304,
5.05793387547865));
#62697=CARTESIAN_POINT('Ctrl Pts',(-54.9996425046093,-14.1841570529565,
5.13643938585543));
#62698=CARTESIAN_POINT('Ctrl Pts',(-54.368124759941,-15.7848308402587,5.2149448962322));
#62699=CARTESIAN_POINT('Ctrl Pts',(-52.6846517467245,-16.1409756074536,
5.29345040660899));
#62700=CARTESIAN_POINT('Ctrl Pts',(-51.4589751002972,-14.933224869348,5.37195591698576));
#62701=CARTESIAN_POINT('Ctrl Pts',(-51.7903649128864,-13.2446527814935,
5.45046142736255));
#62702=CARTESIAN_POINT('Ctrl Pts',(-53.3815143142557,-12.5897421777335,
5.52896693773931));
#62703=CARTESIAN_POINT('Ctrl Pts',(-54.8056605807673,-13.5555691601388,
5.60747244811611));
#62704=CARTESIAN_POINT('Ctrl Pts',(-54.7851583544017,-15.2764853923884,
5.68597795849288));
#62705=CARTESIAN_POINT('Ctrl Pts',(-53.3392716219708,-16.2080719085829,
5.76448346886966));
#62706=CARTESIAN_POINT('Ctrl Pts',(-51.7629444164752,-15.5169955192796,
5.84298897924644));
#62707=CARTESIAN_POINT('Ctrl Pts',(-51.4734277108623,-13.8186461670281,
5.92149448962322));
#62708=CARTESIAN_POINT('Ctrl Pts',(-52.3064323164313,-13.0375346028627,
5.97383149654107));
#62709=CARTESIAN_POINT('Ctrl Pts',(-52.7966221146314,-12.9064860705774,
6.));
#62710=CARTESIAN_POINT('Ctrl Pts',(-52.2370198037663,-15.2223467977324,
2.));
#62711=CARTESIAN_POINT('Ctrl Pts',(-52.2001398221824,-15.1879057962803,
2.));
#62712=CARTESIAN_POINT('Ctrl Pts',(-52.1656378013748,-15.1512262749774,
2.));
#62713=CARTESIAN_POINT('Ctrl Pts',(-52.133515895996,-15.112628111497,2.));
#62714=CARTESIAN_POINT('Ctrl Pts',(-52.0999545216902,-15.0723002605552,
2.));
#62715=CARTESIAN_POINT('Ctrl Pts',(-52.0689907405509,-15.0298774985346,
2.));
#62716=CARTESIAN_POINT('Ctrl Pts',(-52.040655024137,-14.9856749556978,2.));
#62717=CARTESIAN_POINT('Ctrl Pts',(-52.0179305604283,-14.9502257344445,
2.));
#62718=CARTESIAN_POINT('Ctrl Pts',(-51.9968968139207,-14.9136306734534,
2.));
#62719=CARTESIAN_POINT('Ctrl Pts',(-51.9775857407058,-14.8760343811022,
2.));
#62720=CARTESIAN_POINT('Ctrl Pts',(-51.9694199887411,-14.8601366630044,
2.));
#62721=CARTESIAN_POINT('Ctrl Pts',(-51.9615624516271,-14.8440597542834,
2.));
#62722=CARTESIAN_POINT('Ctrl Pts',(-51.9540164358689,-14.8278139468956,
2.));
#62723=CARTESIAN_POINT('Ctrl Pts',(-51.9497380912329,-14.8186031043633,
2.));
#62724=CARTESIAN_POINT('Ctrl Pts',(-51.9455597070027,-14.809337270677,2.));
#62725=CARTESIAN_POINT('Ctrl Pts',(-51.9414881758912,-14.8000332485161,
2.));
#62726=CARTESIAN_POINT('Ctrl Pts',(-51.9196632025412,-14.750160109849,2.));
#62727=CARTESIAN_POINT('Ctrl Pts',(-51.9008587821636,-14.6990941701308,
2.));
#62728=CARTESIAN_POINT('Ctrl Pts',(-51.8851025499192,-14.6471668919688,
2.));
#62729=CARTESIAN_POINT('Ctrl Pts',(-51.8690578814023,-14.5942890242042,
2.));
#62730=CARTESIAN_POINT('Ctrl Pts',(-51.856173427568,-14.5405170693332,2.));
#62731=CARTESIAN_POINT('Ctrl Pts',(-51.8465190610514,-14.4861664358985,
2.));
#62732=CARTESIAN_POINT('Ctrl Pts',(-51.8396145127886,-14.4472962965663,
2.));
#62733=CARTESIAN_POINT('Ctrl Pts',(-51.8343629002831,-14.4081294057031,
2.));
#62734=CARTESIAN_POINT('Ctrl Pts',(-51.8308047851344,-14.368774756998,2.));
#62735=CARTESIAN_POINT('Ctrl Pts',(-51.8292917204625,-14.3520394558225,
2.));
#62736=CARTESIAN_POINT('Ctrl Pts',(-51.8280850590022,-14.3352701586909,
2.));
#62737=CARTESIAN_POINT('Ctrl Pts',(-51.8271886807144,-14.3184751150899,
2.));
#62738=CARTESIAN_POINT('Ctrl Pts',(-51.8266545203306,-14.3084667881852,
2.));
#62739=CARTESIAN_POINT('Ctrl Pts',(-51.8262309124811,-14.2984549964066,
2.));
#62740=CARTESIAN_POINT('Ctrl Pts',(-51.8259184500034,-14.2884490816797,
2.));
#62741=CARTESIAN_POINT('Ctrl Pts',(-51.8241448794411,-14.2316544356751,
2.));
#62742=CARTESIAN_POINT('Ctrl Pts',(-51.8259444031621,-14.1749772817713,
2.));
#62743=CARTESIAN_POINT('Ctrl Pts',(-51.831377054275,-14.1187497415498,2.));
#62744=CARTESIAN_POINT('Ctrl Pts',(-51.8347120697802,-14.0842325758864,
2.));
#62745=CARTESIAN_POINT('Ctrl Pts',(-51.8394171165311,-14.0498843037551,
2.));
#62746=CARTESIAN_POINT('Ctrl Pts',(-51.845515342272,-14.0157787106909,2.));
#62747=CARTESIAN_POINT('Ctrl Pts',(-51.8551874830705,-13.9616852559467,
2.));
#62748=CARTESIAN_POINT('Ctrl Pts',(-51.8683614486688,-13.9082017945064,
2.));
#62749=CARTESIAN_POINT('Ctrl Pts',(-51.8848110251026,-13.8555328884186,
2.));
#62750=CARTESIAN_POINT('Ctrl Pts',(-51.8897327932489,-13.8397741760089,
2.));
#62751=CARTESIAN_POINT('Ctrl Pts',(-51.8949481552399,-13.8240884170171,
2.));
#62752=CARTESIAN_POINT('Ctrl Pts',(-51.9004519259216,-13.8084812249409,
2.));
#62753=CARTESIAN_POINT('Ctrl Pts',(-51.9055403383158,-13.7940518756473,
2.));
#62754=CARTESIAN_POINT('Ctrl Pts',(-51.9108779029592,-13.7796834481853,
2.));
#62755=CARTESIAN_POINT('Ctrl Pts',(-51.9164469096078,-13.7654145762878,
2.));
#62756=CARTESIAN_POINT('Ctrl Pts',(-51.937078011076,-13.7125537049463,2.));
#62757=CARTESIAN_POINT('Ctrl Pts',(-51.9609027535564,-13.6609889337068,
2.));
#62758=CARTESIAN_POINT('Ctrl Pts',(-51.9876380075214,-13.6109308617714,
2.));
#62759=CARTESIAN_POINT('Ctrl Pts',(-52.0150055546465,-13.5596889081893,
2.));
#62760=CARTESIAN_POINT('Ctrl Pts',(-52.0454232532683,-13.5100248567806,
2.));
#62761=CARTESIAN_POINT('Ctrl Pts',(-52.078642743017,-13.4621702328318,2.));
#62762=CARTESIAN_POINT('Ctrl Pts',(-52.0988112436159,-13.4331163244463,
2.));
#62763=CARTESIAN_POINT('Ctrl Pts',(-52.1200135483417,-13.4047295468345,
2.));
#62764=CARTESIAN_POINT('Ctrl Pts',(-52.1422027768384,-13.3770649262843,
2.));
#62765=CARTESIAN_POINT('Ctrl Pts',(-52.1544198936712,-13.3618331257985,
2.));
#62766=CARTESIAN_POINT('Ctrl Pts',(-52.1669363024172,-13.3468202983724,
2.));
#62767=CARTESIAN_POINT('Ctrl Pts',(-52.1797449296066,-13.3320361041244,
2.));
#62768=CARTESIAN_POINT('Ctrl Pts',(-52.1874577031558,-13.3231337338192,
2.));
#62769=CARTESIAN_POINT('Ctrl Pts',(-52.1952777965008,-13.3143127818998,
2.));
#62770=CARTESIAN_POINT('Ctrl Pts',(-52.203199440933,-13.3055801677412,2.));
#62771=CARTESIAN_POINT('Ctrl Pts',(-52.2437953927146,-13.2608282495827,
2.));
#62772=CARTESIAN_POINT('Ctrl Pts',(-52.2869270093575,-13.2185332555895,
2.));
#62773=CARTESIAN_POINT('Ctrl Pts',(-52.3323340644277,-13.1789459514645,
2.));
#62774=CARTESIAN_POINT('Ctrl Pts',(-52.3618576920541,-13.1532063208296,
2.));
#62775=CARTESIAN_POINT('Ctrl Pts',(-52.3923443514376,-13.128611691001,2.));
#62776=CARTESIAN_POINT('Ctrl Pts',(-52.4237326847397,-13.1052370160425,
2.));
#62777=CARTESIAN_POINT('Ctrl Pts',(-52.4367029256792,-13.095578167222,2.));
#62778=CARTESIAN_POINT('Ctrl Pts',(-52.4498272128038,-13.0861276945749,
2.));
#62779=CARTESIAN_POINT('Ctrl Pts',(-52.4631015594291,-13.0768912105345,
2.));
#62780=CARTESIAN_POINT('Ctrl Pts',(-52.4728212296877,-13.0701281221689,
2.));
#62781=CARTESIAN_POINT('Ctrl Pts',(-52.4826204708896,-13.063480479123,2.));
#62782=CARTESIAN_POINT('Ctrl Pts',(-52.4924892032556,-13.0569558445777,
2.));
#62783=CARTESIAN_POINT('Ctrl Pts',(-52.5432262963862,-13.0234114157406,
2.));
#62784=CARTESIAN_POINT('Ctrl Pts',(-52.5958554389749,-12.9930745926173,
2.));
#62785=CARTESIAN_POINT('Ctrl Pts',(-52.6501404637806,-12.9662121664589,
2.));
#62786=CARTESIAN_POINT('Ctrl Pts',(-52.6755695105507,-12.9536288454861,
2.));
#62787=CARTESIAN_POINT('Ctrl Pts',(-52.7013624781742,-12.9418083828321,
2.));
#62788=CARTESIAN_POINT('Ctrl Pts',(-52.7274977743506,-12.930781120438,2.));
#62789=CARTESIAN_POINT('Ctrl Pts',(-52.7499504413758,-12.9213076693217,
2.));
#62790=CARTESIAN_POINT('Ctrl Pts',(-52.7726557928972,-12.9124196555961,
2.));
#62791=CARTESIAN_POINT('Ctrl Pts',(-52.7955926848293,-12.9041113294173,
2.));
#62792=CARTESIAN_POINT('Ctrl Pts',(-54.4591686783466,-14.3960664985434,
2.80658032638058));
#62793=CARTESIAN_POINT('Ctrl Pts',(-54.4601242407418,-14.2819704202925,
2.79940525217632));
#62794=CARTESIAN_POINT('Ctrl Pts',(-54.4459154362348,-14.1681081402059,
2.79223017797206));
#62795=CARTESIAN_POINT('Ctrl Pts',(-54.4155823692926,-14.0587171406723,
2.78505510376779));
#62796=CARTESIAN_POINT('Ctrl Pts',(-54.3049534134658,-13.6597527999316,
2.75888660030887));
#62797=CARTESIAN_POINT('Ctrl Pts',(-53.9798454272937,-13.3202637946524,
2.73271809684994));
#62798=CARTESIAN_POINT('Ctrl Pts',(-53.5860401608047,-13.1924752739395,
2.70654959339101));
#62799=CARTESIAN_POINT('Ctrl Pts',(-53.1922348943158,-13.0646867532265,
2.68038108993209));
#62800=CARTESIAN_POINT('Ctrl Pts',(-52.72973234751,-13.1485987170799,2.65421258647316));
#62801=CARTESIAN_POINT('Ctrl Pts',(-52.405925234305,-13.4065955915993,2.62804408301423));
#62802=CARTESIAN_POINT('Ctrl Pts',(-52.0821181210999,-13.6645924661187,
2.60187557955531));
#62803=CARTESIAN_POINT('Ctrl Pts',(-51.8970064414956,-14.0966742513041,
2.57570707609638));
#62804=CARTESIAN_POINT('Ctrl Pts',(-51.9335943179073,-14.509067171031,2.54953857263746));
#62805=CARTESIAN_POINT('Ctrl Pts',(-51.9701821943189,-14.9214600907578,
2.52337006917853));
#62806=CARTESIAN_POINT('Ctrl Pts',(-52.2284696267464,-15.314164145026,2.4972015657196));
#62807=CARTESIAN_POINT('Ctrl Pts',(-52.5926417836311,-15.5111326464248,
2.47103306226068));
#62808=CARTESIAN_POINT('Ctrl Pts',(-52.9568139405158,-15.7081011478235,
2.44486455880175));
#62809=CARTESIAN_POINT('Ctrl Pts',(-53.4268708218575,-15.7093340963528,
2.41869605534282));
#62810=CARTESIAN_POINT('Ctrl Pts',(-53.7920246633661,-15.5141853735895,
2.3925275518839));
#62811=CARTESIAN_POINT('Ctrl Pts',(-54.1571785048747,-15.3190366508261,
2.36635904842497));
#62812=CARTESIAN_POINT('Ctrl Pts',(-54.4174293065502,-14.92750625677,2.34019054496604));
#62813=CARTESIAN_POINT('Ctrl Pts',(-54.456094882425,-14.5153482269177,2.31402204150712));
#62814=CARTESIAN_POINT('Ctrl Pts',(-54.4597600799313,-14.4762788338196,
2.31154146979827));
#62815=CARTESIAN_POINT('Ctrl Pts',(-54.461434207113,-14.4370240895848,2.30906089808943));
#62816=CARTESIAN_POINT('Ctrl Pts',(-54.4611870990995,-14.3977489718831,
2.30658032638058));
#62817=CARTESIAN_POINT('Ctrl Pts',(-53.5936497983459,-12.9064860705774,
2.));
#62818=CARTESIAN_POINT('Ctrl Pts',(-54.083839596546,-13.0375346028627,2.02616850345893));
#62819=CARTESIAN_POINT('Ctrl Pts',(-54.9168437793101,-13.8186488783651,
2.07850551037678));
#62820=CARTESIAN_POINT('Ctrl Pts',(-54.6273278627067,-15.5169944524465,
2.15701102075356));
#62821=CARTESIAN_POINT('Ctrl Pts',(-53.0510002557363,-16.2080728204287,
2.23551653113034));
#62822=CARTESIAN_POINT('Ctrl Pts',(-51.605113325188,-15.2764851170283,2.31402204150712));
#62823=CARTESIAN_POINT('Ctrl Pts',(-51.5846111642588,-13.5555692706413,
2.3925275518839));
#62824=CARTESIAN_POINT('Ctrl Pts',(-53.0087575469087,-12.5897418281553,
2.47103306226068));
#62825=CARTESIAN_POINT('Ctrl Pts',(-54.5999071972633,-13.2446527015669,
2.54953857263746));
#62826=CARTESIAN_POINT('Ctrl Pts',(-54.9312970207009,-14.9332249012822,
2.62804408301423));
#62827=CARTESIAN_POINT('Ctrl Pts',(-53.7056202382209,-16.1409758479641,
2.70654959339102));
#62828=CARTESIAN_POINT('Ctrl Pts',(-52.0221470001079,-15.7848310056966,
2.78505510376779));
#62829=CARTESIAN_POINT('Ctrl Pts',(-51.3906291820653,-14.1841570315506,
2.86356061414457));
#62830=CARTESIAN_POINT('Ctrl Pts',(-52.377440405223,-12.7744925974775,2.94206612452135));
#62831=CARTESIAN_POINT('Ctrl Pts',(-54.0975782126822,-12.8200502087089,
3.02057163489813));
#62832=CARTESIAN_POINT('Ctrl Pts',(-55.0083854595842,-14.2799767390429,
3.09907714527492));
#62833=CARTESIAN_POINT('Ctrl Pts',(-54.293026891849,-15.8449733636912,3.17758265565169));
#62834=CARTESIAN_POINT('Ctrl Pts',(-52.5930539078611,-16.1115149029785,
3.25608816602847));
#62835=CARTESIAN_POINT('Ctrl Pts',(-51.4330422815012,-14.8405600699842,
3.33459367640525));
#62836=CARTESIAN_POINT('Ctrl Pts',(-51.8533182226522,-13.1719316222439,
3.41309918678203));
#62837=CARTESIAN_POINT('Ctrl Pts',(-53.4769681733105,-12.6020950974316,
3.49160469715881));
#62838=CARTESIAN_POINT('Ctrl Pts',(-54.8478643087328,-13.642093499697,3.57011020753559));
#62839=CARTESIAN_POINT('Ctrl Pts',(-54.7365543580298,-15.3592315066375,
3.64861571791237));
#62840=CARTESIAN_POINT('Ctrl Pts',(-53.2428637439183,-16.2135389463141,
3.72712122828915));
#62841=CARTESIAN_POINT('Ctrl Pts',(-51.7063697132749,-15.4388525891942,
3.80562673866593));
#62842=CARTESIAN_POINT('Ctrl Pts',(-51.5050366439836,-13.7299295812751,
3.88413224904271));
#62843=CARTESIAN_POINT('Ctrl Pts',(-52.8194248174382,-12.6193727014466,
3.96263775941949));
#62844=CARTESIAN_POINT('Ctrl Pts',(-54.4707596726698,-13.1031557625362,
4.04114326979626));
#62845=CARTESIAN_POINT('Ctrl Pts',(-54.978084852892,-14.7474106134536,4.11964878017304));
#62846=CARTESIAN_POINT('Ctrl Pts',(-53.8864190756817,-16.0775304145121,
4.19815429054983));
#62847=CARTESIAN_POINT('Ctrl Pts',(-52.1747941628695,-15.9006321056092,
4.2766598009266));
#62848=CARTESIAN_POINT('Ctrl Pts',(-51.3782360277521,-14.3753622969642,
4.35516531130339));
#62849=CARTESIAN_POINT('Ctrl Pts',(-52.2111169431944,-12.8696192117061,
4.43367082168016));
#62850=CARTESIAN_POINT('Ctrl Pts',(-53.9264895031678,-12.7337890506155,
4.51217633205695));
#62851=CARTESIAN_POINT('Ctrl Pts',(-54.9859668161601,-14.0896875214679,
4.59068184243372));
#62852=CARTESIAN_POINT('Ctrl Pts',(-54.4393844383933,-15.7213126607523,
4.6691873528105));
#62853=CARTESIAN_POINT('Ctrl Pts',(-52.7769304442279,-16.1653842141838,
4.74769286318728));
#62854=CARTESIAN_POINT('Ctrl Pts',(-51.4895330907316,-15.0236483351254,
4.82619837356406));
#62855=CARTESIAN_POINT('Ctrl Pts',(-51.7317609456535,-13.3200407432483,
4.90470388394085));
#62856=CARTESIAN_POINT('Ctrl Pts',(-53.2863782799341,-12.5823975487372,
4.98320939431761));
#62857=CARTESIAN_POINT('Ctrl Pts',(-54.7591673697362,-13.4722540610765,
5.06171490469441));
#62858=CARTESIAN_POINT('Ctrl Pts',(-54.8292958244512,-15.1915670968036,
5.14022041507117));
#62859=CARTESIAN_POINT('Ctrl Pts',(-53.4338710221273,-16.1984132586634,
5.21872592544796));
#62860=CARTESIAN_POINT('Ctrl Pts',(-51.8243426112988,-15.5898341745865,
5.29723143582474));
#62861=CARTESIAN_POINT('Ctrl Pts',(-51.4441749154368,-13.9116075960113,
5.37573694620152));
#62862=CARTESIAN_POINT('Ctrl Pts',(-52.6343093950298,-12.6688279644592,
5.45424245657829));
#62863=CARTESIAN_POINT('Ctrl Pts',(-54.3274091023452,-12.976007562431,5.53274796695508));
#62864=CARTESIAN_POINT('Ctrl Pts',(-55.0050540475836,-14.5577447773064,
5.61125347733185));
#62865=CARTESIAN_POINT('Ctrl Pts',(-54.0595320288467,-15.9953308004788,
5.68975898770864));
#62866=CARTESIAN_POINT('Ctrl Pts',(-52.3387777758965,-15.9998439842325,
5.76826449808541));
#62867=CARTESIAN_POINT('Ctrl Pts',(-51.386068598834,-14.5665551393412,5.8467700084622));
#62868=CARTESIAN_POINT('Ctrl Pts',(-52.0556885439603,-12.9822402103746,
5.92527551883896));
#62869=CARTESIAN_POINT('Ctrl Pts',(-53.7473606277104,-12.6649964614199,
6.00378102921576));
#62870=CARTESIAN_POINT('Ctrl Pts',(-54.943474474887,-13.9049596945687,6.08228653959253));
#62871=CARTESIAN_POINT('Ctrl Pts',(-54.6954044415815,-15.0196330720529,
6.13462354651039));
#62872=CARTESIAN_POINT('Ctrl Pts',(-54.3642725509138,-15.404095589155,6.16079204996931));
#62873=CARTESIAN_POINT('Ctrl Pts',(-53.5696735389038,-12.996169774565,1.94640265001023));
#62874=CARTESIAN_POINT('Ctrl Pts',(-54.0303714687093,-13.11933387906,1.97257115346916));
#62875=CARTESIAN_POINT('Ctrl Pts',(-54.813258635941,-13.8534530528714,2.02490816038701));
#62876=CARTESIAN_POINT('Ctrl Pts',(-54.5411612077312,-15.4496190541765,
2.10341367076379));
#62877=CARTESIAN_POINT('Ctrl Pts',(-53.0596720623164,-16.099119257224,2.18191918114057));
#62878=CARTESIAN_POINT('Ctrl Pts',(-51.7007757366844,-15.2235797662662,
2.26042469151735));
#62879=CARTESIAN_POINT('Ctrl Pts',(-51.6815070715035,-13.6062014146337,
2.33893020189412));
#62880=CARTESIAN_POINT('Ctrl Pts',(-53.0199708515249,-12.6984821904956,
2.41743571227091));
#62881=CARTESIAN_POINT('Ctrl Pts',(-54.5153902842031,-13.3139908867102,
2.49594122264768));
#62882=CARTESIAN_POINT('Ctrl Pts',(-54.8268423098815,-14.9009715207264,
2.57444673302447));
#62883=CARTESIAN_POINT('Ctrl Pts',(-53.6749073688187,-16.0360591192444,
2.65295224340125));
#62884=CARTESIAN_POINT('Ctrl Pts',(-52.0927189215492,-15.7013414402026,
2.73145775377802));
#62885=CARTESIAN_POINT('Ctrl Pts',(-51.4991958566553,-14.1969707068861,
2.8099632641548));
#62886=CARTESIAN_POINT('Ctrl Pts',(-52.4266363894587,-12.8721175808469,
2.88846877453159));
#62887=CARTESIAN_POINT('Ctrl Pts',(-54.0432835122394,-12.9149342556498,
2.96697428490836));
#62888=CARTESIAN_POINT('Ctrl Pts',(-54.8992927858724,-14.2870255000261,
3.04547979528514));
#62889=CARTESIAN_POINT('Ctrl Pts',(-54.2269731814369,-15.7578653824051,
3.12398530566192));
#62890=CARTESIAN_POINT('Ctrl Pts',(-52.6292776820116,-16.0083706679245,
3.2024908160387));
#62891=CARTESIAN_POINT('Ctrl Pts',(-51.5390572066436,-14.8138817932341,
3.28099632641548));
#62892=CARTESIAN_POINT('Ctrl Pts',(-51.9340475894427,-13.2456450116627,
3.35950183679226));
#62893=CARTESIAN_POINT('Ctrl Pts',(-53.4600119684315,-12.7100922354268,
3.43800734716904));
#62894=CARTESIAN_POINT('Ctrl Pts',(-54.7484292588084,-13.6875199841967,
3.51651285754582));
#62895=CARTESIAN_POINT('Ctrl Pts',(-54.6438161802745,-15.3013477870039,
3.5950183679226));
#62896=CARTESIAN_POINT('Ctrl Pts',(-53.2399922406132,-16.104256518115,3.67352387829938));
#62897=CARTESIAN_POINT('Ctrl Pts',(-51.7959401169765,-15.3761785322325,
3.75202938867615));
#62898=CARTESIAN_POINT('Ctrl Pts',(-51.6067200871749,-13.7700714797477,
3.83053489905294));
#62899=CARTESIAN_POINT('Ctrl Pts',(-52.8420291709109,-12.7263303465236,
3.90904040942972));
#62900=CARTESIAN_POINT('Ctrl Pts',(-54.3940128148265,-13.1810069953183,
3.9875459198065));
#62901=CARTESIAN_POINT('Ctrl Pts',(-54.8708151904059,-14.7263365975901,
4.06605143018327));
#62902=CARTESIAN_POINT('Ctrl Pts',(-53.8448285920578,-15.9764308284185,
4.14455694056006));
#62903=CARTESIAN_POINT('Ctrl Pts',(-52.2361821925785,-15.8101754616262,
4.22306245093683));
#62904=CARTESIAN_POINT('Ctrl Pts',(-51.4875483263378,-14.3766722638491,
4.30156796131362));
#62905=CARTESIAN_POINT('Ctrl Pts',(-52.2703196425253,-12.9615209801128,
4.38007347169039));
#62906=CARTESIAN_POINT('Ctrl Pts',(-53.8824882150386,-12.8338629295998,
4.45857898206717));
#62907=CARTESIAN_POINT('Ctrl Pts',(-54.8782229417988,-14.1081848776325,
4.53708449244395));
#62908=CARTESIAN_POINT('Ctrl Pts',(-54.3645252458656,-15.6416446245447,
4.61559000282073));
#62909=CARTESIAN_POINT('Ctrl Pts',(-52.8020914369185,-16.0589989760686,
4.69409551319751));
#62910=CARTESIAN_POINT('Ctrl Pts',(-51.5921492925276,-14.9859547026092,
4.77260102357429));
#62911=CARTESIAN_POINT('Ctrl Pts',(-51.8198037066208,-13.3848432685065,
4.85110653395107));
#62912=CARTESIAN_POINT('Ctrl Pts',(-53.2808887601503,-12.6915797736435,
4.92961204432785));
#62913=CARTESIAN_POINT('Ctrl Pts',(-54.6650686986216,-13.527898796528,5.00811755470463));
#62914=CARTESIAN_POINT('Ctrl Pts',(-54.7309779322007,-15.1437707692933,
5.08662306508141));
#62915=CARTESIAN_POINT('Ctrl Pts',(-53.41950772211,-16.090040855094,5.16512857545819));
#62916=CARTESIAN_POINT('Ctrl Pts',(-51.9068152720538,-15.5180764339929,
5.24363408583497));
#62917=CARTESIAN_POINT('Ctrl Pts',(-51.5495200547613,-13.9408189852801,
5.32213959621175));
#62918=CARTESIAN_POINT('Ctrl Pts',(-52.6680510665282,-12.7728101740752,
5.40064510658852));
#62919=CARTESIAN_POINT('Ctrl Pts',(-54.2592868143519,-13.061508562707,5.47915061696532));
#62920=CARTESIAN_POINT('Ctrl Pts',(-54.8961618055507,-14.5480818513904,
5.55765612734208));
#62921=CARTESIAN_POINT('Ctrl Pts',(-54.0075263459451,-15.8991766869513,
5.63616163771887));
#62922=CARTESIAN_POINT('Ctrl Pts',(-52.3902998656125,-15.9034183386947,
5.71466714809564));
#62923=CARTESIAN_POINT('Ctrl Pts',(-51.494909657185,-14.5563621451974,5.79317265847243));
#62924=CARTESIAN_POINT('Ctrl Pts',(-52.1242424658418,-13.0673662284834,
5.8716781688492));
#62925=CARTESIAN_POINT('Ctrl Pts',(-53.7141364819045,-12.7692091902835,
5.950183679226));
#62926=CARTESIAN_POINT('Ctrl Pts',(-54.8382871174937,-13.9345710493921,
6.02868918960275));
#62927=CARTESIAN_POINT('Ctrl Pts',(-54.6051420149022,-14.9821810145562,
6.08102619652062));
#62928=CARTESIAN_POINT('Ctrl Pts',(-54.2939324036795,-15.3435126586808,
6.10719469997954));
#62929=CARTESIAN_POINT('Ctrl Pts',(-53.5456972794618,-13.0858534785527,
1.89280530002046));
#62930=CARTESIAN_POINT('Ctrl Pts',(-53.9769033408726,-13.2011331552573,
1.91897380347939));
#62931=CARTESIAN_POINT('Ctrl Pts',(-54.7096734925719,-13.8882572273778,
1.97131081039724));
#62932=CARTESIAN_POINT('Ctrl Pts',(-54.4549945527556,-15.3822436559065,
2.04981632077402));
#62933=CARTESIAN_POINT('Ctrl Pts',(-53.0683438688966,-15.9901656940193,
2.1283218311508));
#62934=CARTESIAN_POINT('Ctrl Pts',(-51.7964381481809,-15.1706744155041,
2.20682734152758));
#62935=CARTESIAN_POINT('Ctrl Pts',(-51.7784029787483,-13.6568335586262,
2.28533285190436));
#62936=CARTESIAN_POINT('Ctrl Pts',(-53.0311841561409,-12.807222552836,2.36383836228114));
#62937=CARTESIAN_POINT('Ctrl Pts',(-54.4308733711429,-13.3833290718535,
2.44234387265792));
#62938=CARTESIAN_POINT('Ctrl Pts',(-54.722387599062,-14.8687181401707,2.5208493830347));
#62939=CARTESIAN_POINT('Ctrl Pts',(-53.6441944994167,-15.9311423905248,
2.59935489341147));
#62940=CARTESIAN_POINT('Ctrl Pts',(-52.1632908429905,-15.6178518747085,
2.67786040378825));
#62941=CARTESIAN_POINT('Ctrl Pts',(-51.6077625312453,-14.2097843822215,
2.75636591416503));
#62942=CARTESIAN_POINT('Ctrl Pts',(-52.4758323736945,-12.9697425642164,
2.83487142454181));
#62943=CARTESIAN_POINT('Ctrl Pts',(-53.9889888117967,-13.0098183025906,
2.91337693491859));
#62944=CARTESIAN_POINT('Ctrl Pts',(-54.7902001121605,-14.2940742610093,
2.99188244529538));
#62945=CARTESIAN_POINT('Ctrl Pts',(-54.1609194710247,-15.670757401119,3.07038795567215));
#62946=CARTESIAN_POINT('Ctrl Pts',(-52.6655014561621,-15.9052264328705,
3.14889346604893));
#62947=CARTESIAN_POINT('Ctrl Pts',(-51.645072131786,-14.7872035164841,3.22739897642571));
#62948=CARTESIAN_POINT('Ctrl Pts',(-52.0147769562333,-13.3193584010815,
3.30590448680249));
#62949=CARTESIAN_POINT('Ctrl Pts',(-53.4430557635525,-12.818089373422,3.38440999717927));
#62950=CARTESIAN_POINT('Ctrl Pts',(-54.648994208884,-13.7329464686964,3.46291550755605));
#62951=CARTESIAN_POINT('Ctrl Pts',(-54.5510780025192,-15.2434640673703,
3.54142101793283));
#62952=CARTESIAN_POINT('Ctrl Pts',(-53.2371207373081,-15.9949740899159,
3.61992652830961));
#62953=CARTESIAN_POINT('Ctrl Pts',(-51.8855105206782,-15.3135044752707,
3.69843203868638));
#62954=CARTESIAN_POINT('Ctrl Pts',(-51.7084035303663,-13.8102133782203,
3.77693754906317));
#62955=CARTESIAN_POINT('Ctrl Pts',(-52.8646335243837,-12.8332879916007,
3.85544305943994));
#62956=CARTESIAN_POINT('Ctrl Pts',(-54.3172659569833,-13.2588582281004,
3.93394856981673));
#62957=CARTESIAN_POINT('Ctrl Pts',(-54.7635455279197,-14.7052625817266,
4.0124540801935));
#62958=CARTESIAN_POINT('Ctrl Pts',(-53.8032381084339,-15.875331242325,4.09095959057029));
#62959=CARTESIAN_POINT('Ctrl Pts',(-52.2975702222875,-15.7197188176431,
4.16946510094706));
#62960=CARTESIAN_POINT('Ctrl Pts',(-51.5968606249236,-14.377982230734,4.24797061132384));
#62961=CARTESIAN_POINT('Ctrl Pts',(-52.329522341856,-13.0534227485195,4.32647612170062));
#62962=CARTESIAN_POINT('Ctrl Pts',(-53.8384869269094,-12.9339368085841,
4.4049816320774));
#62963=CARTESIAN_POINT('Ctrl Pts',(-54.7704790674375,-14.1266822337971,
4.48348714245418));
#62964=CARTESIAN_POINT('Ctrl Pts',(-54.289666053338,-15.5619765883372,4.56199265283096));
#62965=CARTESIAN_POINT('Ctrl Pts',(-52.827252429609,-15.9526137379533,4.64049816320774));
#62966=CARTESIAN_POINT('Ctrl Pts',(-51.6947654943235,-14.9482610700929,
4.71900367358452));
#62967=CARTESIAN_POINT('Ctrl Pts',(-51.9078464675881,-13.4496457937646,
4.7975091839613));
#62968=CARTESIAN_POINT('Ctrl Pts',(-53.2753992403664,-12.8007619985498,
4.87601469433808));
#62969=CARTESIAN_POINT('Ctrl Pts',(-54.570970027507,-13.5835435319795,4.95452020471486));
#62970=CARTESIAN_POINT('Ctrl Pts',(-54.6326600399502,-15.095974441783,5.03302571509164));
#62971=CARTESIAN_POINT('Ctrl Pts',(-53.4051444220927,-15.9816684515245,
5.11153122546842));
#62972=CARTESIAN_POINT('Ctrl Pts',(-51.9892879328089,-15.4463186933993,
5.19003673584519));
#62973=CARTESIAN_POINT('Ctrl Pts',(-51.6548651940858,-13.970030374549,5.26854224622198));
#62974=CARTESIAN_POINT('Ctrl Pts',(-52.7017927380266,-12.8767923836913,
5.34704775659875));
#62975=CARTESIAN_POINT('Ctrl Pts',(-54.1911645263586,-13.147009562983,5.42555326697554));
#62976=CARTESIAN_POINT('Ctrl Pts',(-54.7872695635179,-14.5384189254744,
5.50405877735231));
#62977=CARTESIAN_POINT('Ctrl Pts',(-53.9555206630435,-15.8030225734238,
5.5825642877291));
#62978=CARTESIAN_POINT('Ctrl Pts',(-52.4418219553284,-15.806992693157,5.66106979810587));
#62979=CARTESIAN_POINT('Ctrl Pts',(-51.603750715536,-14.5461691510535,5.73957530848265));
#62980=CARTESIAN_POINT('Ctrl Pts',(-52.1927963877232,-13.1524922465921,
5.81808081885944));
#62981=CARTESIAN_POINT('Ctrl Pts',(-53.6809123360987,-12.8734219191469,
5.89658632923621));
#62982=CARTESIAN_POINT('Ctrl Pts',(-54.7330997601003,-13.9641824042154,
5.97509183961299));
#62983=CARTESIAN_POINT('Ctrl Pts',(-54.5148795882229,-14.9447289570596,
6.02742884653085));
#62984=CARTESIAN_POINT('Ctrl Pts',(-54.2235922564453,-15.2829297282066,
6.05359734998977));
#62985=CARTESIAN_POINT('Ctrl Pts',(-53.5217210200197,-13.1755371825403,
1.83920795003069));
#62986=CARTESIAN_POINT('Ctrl Pts',(-53.923435213036,-13.2829324314546,1.86537645348962));
#62987=CARTESIAN_POINT('Ctrl Pts',(-54.6060883492027,-13.9230614018842,
1.91771346040747));
#62988=CARTESIAN_POINT('Ctrl Pts',(-54.36882789778,-15.3148682576366,1.99621897078425));
#62989=CARTESIAN_POINT('Ctrl Pts',(-53.0770156754767,-15.8812121308145,
2.07472448116103));
#62990=CARTESIAN_POINT('Ctrl Pts',(-51.8921005596774,-15.1177690647421,
2.15322999153781));
#62991=CARTESIAN_POINT('Ctrl Pts',(-51.8752988859931,-13.7074657026186,
2.23173550191459));
#62992=CARTESIAN_POINT('Ctrl Pts',(-53.042397460757,-12.9159629151763,2.31024101229137));
#62993=CARTESIAN_POINT('Ctrl Pts',(-54.3463564580827,-13.4526672569968,
2.38874652266814));
#62994=CARTESIAN_POINT('Ctrl Pts',(-54.6179328882426,-14.836464759615,2.46725203304492));
#62995=CARTESIAN_POINT('Ctrl Pts',(-53.6134816300145,-15.8262256618051,
2.5457575434217));
#62996=CARTESIAN_POINT('Ctrl Pts',(-52.2338627644319,-15.5343623092145,
2.62426305379848));
#62997=CARTESIAN_POINT('Ctrl Pts',(-51.7163292058353,-14.222598057557,2.70276856417526));
#62998=CARTESIAN_POINT('Ctrl Pts',(-52.5250283579302,-13.0673675475858,
2.78127407455204));
#62999=CARTESIAN_POINT('Ctrl Pts',(-53.9346941113538,-13.1047023495315,
2.85977958492882));
#63000=CARTESIAN_POINT('Ctrl Pts',(-54.6811074384486,-14.3011230219925,
2.9382850953056));
#63001=CARTESIAN_POINT('Ctrl Pts',(-54.0948657606126,-15.5836494198329,
3.01679060568238));
#63002=CARTESIAN_POINT('Ctrl Pts',(-52.7017252303126,-15.8020821978166,
3.09529611605916));
#63003=CARTESIAN_POINT('Ctrl Pts',(-51.7510870569284,-14.7605252397341,
3.17380162643594));
#63004=CARTESIAN_POINT('Ctrl Pts',(-52.0955063230238,-13.3930717905004,
3.25230713681272));
#63005=CARTESIAN_POINT('Ctrl Pts',(-53.4260995586735,-12.9260865114173,
3.33081264718949));
#63006=CARTESIAN_POINT('Ctrl Pts',(-54.5495591589596,-13.7783729531961,
3.40931815756628));
#63007=CARTESIAN_POINT('Ctrl Pts',(-54.4583398247639,-15.1855803477368,
3.48782366794305));
#63008=CARTESIAN_POINT('Ctrl Pts',(-53.234249234003,-15.8856916617167,3.56632917831984));
#63009=CARTESIAN_POINT('Ctrl Pts',(-51.9750809243799,-15.250830418309,3.64483468869661));
#63010=CARTESIAN_POINT('Ctrl Pts',(-51.8100869735576,-13.8503552766928,
3.7233401990734));
#63011=CARTESIAN_POINT('Ctrl Pts',(-52.8872378778566,-12.9402456366778,
3.80184570945017));
#63012=CARTESIAN_POINT('Ctrl Pts',(-54.24051909914,-13.3367094608825,3.88035121982696));
#63013=CARTESIAN_POINT('Ctrl Pts',(-54.6562758654336,-14.6841885658631,
3.95885673020373));
#63014=CARTESIAN_POINT('Ctrl Pts',(-53.7616476248099,-15.7742316562315,
4.03736224058052));
#63015=CARTESIAN_POINT('Ctrl Pts',(-52.3589582519965,-15.6292621736601,
4.11586775095729));
#63016=CARTESIAN_POINT('Ctrl Pts',(-51.7061729235092,-14.3792921976189,
4.19437326133407));
#63017=CARTESIAN_POINT('Ctrl Pts',(-52.3887250411869,-13.1453245169262,
4.27287877171085));
#63018=CARTESIAN_POINT('Ctrl Pts',(-53.7944856387802,-13.0340106875684,
4.35138428208763));
#63019=CARTESIAN_POINT('Ctrl Pts',(-54.6627351930762,-14.1451795899616,
4.42988979246442));
#63020=CARTESIAN_POINT('Ctrl Pts',(-54.2148068608104,-15.4823085521296,
4.50839530284119));
#63021=CARTESIAN_POINT('Ctrl Pts',(-52.8524134222996,-15.8462284998381,
4.58690081321797));
#63022=CARTESIAN_POINT('Ctrl Pts',(-51.7973816961194,-14.9105674375766,
4.66540632359475));
#63023=CARTESIAN_POINT('Ctrl Pts',(-51.9958892285554,-13.5144483190228,
4.74391183397153));
#63024=CARTESIAN_POINT('Ctrl Pts',(-53.2699097205826,-12.9099442234561,
4.82241734434831));
#63025=CARTESIAN_POINT('Ctrl Pts',(-54.4768713563924,-13.6391882674309,
4.90092285472509));
#63026=CARTESIAN_POINT('Ctrl Pts',(-54.5343421476998,-15.0481781142727,
4.97942836510187));
#63027=CARTESIAN_POINT('Ctrl Pts',(-53.3907811220752,-15.873296047955,5.05793387547865));
#63028=CARTESIAN_POINT('Ctrl Pts',(-52.0717605935641,-15.3745609528058,
5.13643938585542));
#63029=CARTESIAN_POINT('Ctrl Pts',(-51.7602103334102,-13.9992417638178,
5.21494489623221));
#63030=CARTESIAN_POINT('Ctrl Pts',(-52.7355344095251,-12.9807745933074,
5.29345040660898));
#63031=CARTESIAN_POINT('Ctrl Pts',(-54.1230422383652,-13.232510563259,5.37195591698577));
#63032=CARTESIAN_POINT('Ctrl Pts',(-54.6783773214851,-14.5287559995584,
5.45046142736254));
#63033=CARTESIAN_POINT('Ctrl Pts',(-53.9035149801418,-15.7068684598963,
5.52896693773933));
#63034=CARTESIAN_POINT('Ctrl Pts',(-52.4933440450442,-15.7105670476193,
5.60747244811611));
#63035=CARTESIAN_POINT('Ctrl Pts',(-51.712591773887,-14.5359761569097,5.68597795849288));
#63036=CARTESIAN_POINT('Ctrl Pts',(-52.2613503096046,-13.2376182647008,
5.76448346886967));
#63037=CARTESIAN_POINT('Ctrl Pts',(-53.6476881902928,-12.9776346480105,
5.84298897924644));
#63038=CARTESIAN_POINT('Ctrl Pts',(-54.6279124027069,-13.9937937590388,
5.92149448962322));
#63039=CARTESIAN_POINT('Ctrl Pts',(-54.4246171615437,-14.9072768995629,
5.97383149654108));
#63040=CARTESIAN_POINT('Ctrl Pts',(-54.153252109211,-15.2223467977324,6.));
#63041=CARTESIAN_POINT('Ctrl Pts',(-54.4588409672492,-14.3981450852038,
2.44341967361942));
#63042=CARTESIAN_POINT('Ctrl Pts',(-54.4598231909075,-14.5245548856247,
2.45136379342792));
#63043=CARTESIAN_POINT('Ctrl Pts',(-54.4423420959139,-14.6506995799382,
2.45930791323642));
#63044=CARTESIAN_POINT('Ctrl Pts',(-54.4052616068446,-14.770791992877,2.46725203304492));
#63045=CARTESIAN_POINT('Ctrl Pts',(-54.2831158021666,-15.166385060345,2.49342053650385));
#63046=CARTESIAN_POINT('Ctrl Pts',(-53.9482987160905,-15.4963053610751,
2.51958903996278));
#63047=CARTESIAN_POINT('Ctrl Pts',(-53.5509536954554,-15.6126216193417,
2.5457575434217));
#63048=CARTESIAN_POINT('Ctrl Pts',(-53.1536086748203,-15.7289378776082,
2.57192604688063));
#63049=CARTESIAN_POINT('Ctrl Pts',(-52.6937357196261,-15.6316500934114,
2.59809455033956));
#63050=CARTESIAN_POINT('Ctrl Pts',(-52.3775436489295,-15.3643788260367,
2.62426305379848));
#63051=CARTESIAN_POINT('Ctrl Pts',(-52.061351578233,-15.097107558662,2.65043155725741));
#63052=CARTESIAN_POINT('Ctrl Pts',(-51.8888403920341,-14.6598528081095,
2.67660006071634));
#63053=CARTESIAN_POINT('Ctrl Pts',(-51.9373679909505,-14.2486870145047,
2.70276856417526));
#63054=CARTESIAN_POINT('Ctrl Pts',(-51.9858955898669,-13.8375212208999,
2.72893706763419));
#63055=CARTESIAN_POINT('Ctrl Pts',(-52.2554619738986,-13.4524443842429,
2.75510557109312));
#63056=CARTESIAN_POINT('Ctrl Pts',(-52.6251894581517,-13.2661284329053,
2.78127407455204));
#63057=CARTESIAN_POINT('Ctrl Pts',(-52.9949169424048,-13.0798124815677,
2.80744257801097));
#63058=CARTESIAN_POINT('Ctrl Pts',(-53.4648055268793,-13.0922574155496,
2.8336110814699));
#63059=CARTESIAN_POINT('Ctrl Pts',(-53.824152040299,-13.2978833279507,2.85977958492882));
#63060=CARTESIAN_POINT('Ctrl Pts',(-54.1834985537188,-13.5035092403518,
2.88594808838775));
#63061=CARTESIAN_POINT('Ctrl Pts',(-54.4323029960837,-13.9023161311722,
2.91211659184667));
#63062=CARTESIAN_POINT('Ctrl Pts',(-54.4589982709601,-14.3154739762224,
2.9382850953056));
#63063=CARTESIAN_POINT('Ctrl Pts',(-54.4607442500488,-14.342496172514,2.93999662141021));
#63064=CARTESIAN_POINT('Ctrl Pts',(-54.4615401150314,-14.3695797577353,
2.94170814751481));
#63065=CARTESIAN_POINT('Ctrl Pts',(-54.4614103817624,-14.3966710984295,
2.94341967361941));
#63066=CARTESIAN_POINT('Ctrl Pts',(-53.5936497983459,-12.9064860705774,
2.));
#63067=CARTESIAN_POINT('Ctrl Pts',(-53.6510872607052,-12.9274734829173,
2.));
#63068=CARTESIAN_POINT('Ctrl Pts',(-53.7069621322555,-12.9520730502145,
2.));
#63069=CARTESIAN_POINT('Ctrl Pts',(-53.7610764088156,-12.9799849419358,
2.));
#63070=CARTESIAN_POINT('Ctrl Pts',(-53.8148756915178,-13.0077343612928,
2.));
#63071=CARTESIAN_POINT('Ctrl Pts',(-53.8669355047625,-13.0387586838187,
2.));
#63072=CARTESIAN_POINT('Ctrl Pts',(-53.9170293533882,-13.0728080082455,
2.));
#63073=CARTESIAN_POINT('Ctrl Pts',(-53.9548563761379,-13.098519439989,2.));
#63074=CARTESIAN_POINT('Ctrl Pts',(-53.9915618038204,-13.125956761284,2.));
#63075=CARTESIAN_POINT('Ctrl Pts',(-54.0270323602658,-13.1550241879182,
2.));
#63076=CARTESIAN_POINT('Ctrl Pts',(-54.0454462553227,-13.1701140144463,
2.));
#63077=CARTESIAN_POINT('Ctrl Pts',(-54.0635271127833,-13.1856432908818,
2.));
#63078=CARTESIAN_POINT('Ctrl Pts',(-54.0812573827313,-13.2015993500242,
2.));
#63079=CARTESIAN_POINT('Ctrl Pts',(-54.090594739605,-13.210002347776,2.));
#63080=CARTESIAN_POINT('Ctrl Pts',(-54.0998362160445,-13.2185251993375,
2.));
#63081=CARTESIAN_POINT('Ctrl Pts',(-54.1089630227178,-13.22715034206,2.));
#63082=CARTESIAN_POINT('Ctrl Pts',(-54.1519916743795,-13.2678138813483,
2.));
#63083=CARTESIAN_POINT('Ctrl Pts',(-54.1925581151182,-13.3108214912836,
2.));
#63084=CARTESIAN_POINT('Ctrl Pts',(-54.2304545251372,-13.3559335739759,
2.));
#63085=CARTESIAN_POINT('Ctrl Pts',(-54.2675766912808,-13.4001239927502,
2.));
#63086=CARTESIAN_POINT('Ctrl Pts',(-54.3021372565952,-13.4463347100088,
2.));
#63087=CARTESIAN_POINT('Ctrl Pts',(-54.3338978256666,-13.494363501403,2.));
#63088=CARTESIAN_POINT('Ctrl Pts',(-54.3568895198966,-13.5291318735784,
2.));
#63089=CARTESIAN_POINT('Ctrl Pts',(-54.3784130414151,-13.5648534993358,
2.));
#63090=CARTESIAN_POINT('Ctrl Pts',(-54.3983614304231,-13.6014553927541,
2.));
#63091=CARTESIAN_POINT('Ctrl Pts',(-54.4087875591048,-13.6205855616426,
2.));
#63092=CARTESIAN_POINT('Ctrl Pts',(-54.4187831681,-13.6399562243591,2.));
#63093=CARTESIAN_POINT('Ctrl Pts',(-54.4283312993198,-13.6595570483555,
2.));
#63094=CARTESIAN_POINT('Ctrl Pts',(-54.4327718218402,-13.6686727484199,
2.));
#63095=CARTESIAN_POINT('Ctrl Pts',(-54.4371132830006,-13.6778337205283,
2.));
#63096=CARTESIAN_POINT('Ctrl Pts',(-54.4413510256536,-13.6870315207414,
2.));
#63097=CARTESIAN_POINT('Ctrl Pts',(-54.4646885493226,-13.7376844031253,
2.));
#63098=CARTESIAN_POINT('Ctrl Pts',(-54.4849171741929,-13.7895200078225,
2.));
#63099=CARTESIAN_POINT('Ctrl Pts',(-54.5018239463819,-13.842348125432,2.));
#63100=CARTESIAN_POINT('Ctrl Pts',(-54.5131364715696,-13.877696056095,2.));
#63101=CARTESIAN_POINT('Ctrl Pts',(-54.5229608260229,-13.9134887100352,
2.));
#63102=CARTESIAN_POINT('Ctrl Pts',(-54.5312202420661,-13.9496710849604,
2.));
#63103=CARTESIAN_POINT('Ctrl Pts',(-54.5434447189016,-14.0032233702325,
2.));
#63104=CARTESIAN_POINT('Ctrl Pts',(-54.5522427226731,-14.0576303083872,
2.));
#63105=CARTESIAN_POINT('Ctrl Pts',(-54.5576688283951,-14.1125811869758,
2.));
#63106=CARTESIAN_POINT('Ctrl Pts',(-54.5593446193985,-14.1295521404892,
2.));
#63107=CARTESIAN_POINT('Ctrl Pts',(-54.5606984801866,-14.1465748861851,
2.));
#63108=CARTESIAN_POINT('Ctrl Pts',(-54.5617312008432,-14.1636399587011,
2.));
#63109=CARTESIAN_POINT('Ctrl Pts',(-54.5626375347856,-14.1786165686416,
2.));
#63110=CARTESIAN_POINT('Ctrl Pts',(-54.5632965181387,-14.1936323469849,
2.));
#63111=CARTESIAN_POINT('Ctrl Pts',(-54.563708005032,-14.2086448003678,2.));
#63112=CARTESIAN_POINT('Ctrl Pts',(-54.5652337512305,-14.264309255436,2.));
#63113=CARTESIAN_POINT('Ctrl Pts',(-54.5633684846619,-14.3200027126482,
2.));
#63114=CARTESIAN_POINT('Ctrl Pts',(-54.5582160449935,-14.3754072804874,
2.));
#63115=CARTESIAN_POINT('Ctrl Pts',(-54.553069811687,-14.4307451108539,2.));
#63116=CARTESIAN_POINT('Ctrl Pts',(-54.5446438644364,-14.4857958885223,
2.));
#63117=CARTESIAN_POINT('Ctrl Pts',(-54.5329924871079,-14.540227530455,2.));
#63118=CARTESIAN_POINT('Ctrl Pts',(-54.5255451328249,-14.5750192731178,
2.));
#63119=CARTESIAN_POINT('Ctrl Pts',(-54.5167790477671,-14.6095577033572,
2.));
#63120=CARTESIAN_POINT('Ctrl Pts',(-54.5066991329777,-14.6437495917827,
2.));
#63121=CARTESIAN_POINT('Ctrl Pts',(-54.501505292656,-14.6613675193633,2.));
#63122=CARTESIAN_POINT('Ctrl Pts',(-54.495962519931,-14.6788933419033,2.));
#63123=CARTESIAN_POINT('Ctrl Pts',(-54.4900708072911,-14.6963135911257,
2.));
#63124=CARTESIAN_POINT('Ctrl Pts',(-54.4865172473944,-14.706820535848,2.));
#63125=CARTESIAN_POINT('Ctrl Pts',(-54.4828368476645,-14.7172884125542,
2.));
#63126=CARTESIAN_POINT('Ctrl Pts',(-54.4790344473056,-14.7277017730835,
2.));
#63127=CARTESIAN_POINT('Ctrl Pts',(-54.4606465121879,-14.7780594891827,
2.));
#63128=CARTESIAN_POINT('Ctrl Pts',(-54.4393828187194,-14.8272228509927,
2.));
#63129=CARTESIAN_POINT('Ctrl Pts',(-54.4152842461416,-14.8748779184924,
2.));
#63130=CARTESIAN_POINT('Ctrl Pts',(-54.4001512378088,-14.9048035305279,
2.));
#63131=CARTESIAN_POINT('Ctrl Pts',(-54.3838995195653,-14.9341338196321,
2.));
#63132=CARTESIAN_POINT('Ctrl Pts',(-54.3665318698004,-14.9627834478566,
2.));
#63133=CARTESIAN_POINT('Ctrl Pts',(-54.3601820700066,-14.9732580604758,
2.));
#63134=CARTESIAN_POINT('Ctrl Pts',(-54.3536816777358,-14.9836437343855,
2.));
#63135=CARTESIAN_POINT('Ctrl Pts',(-54.347035206222,-14.9939290625586,2.));
#63136=CARTESIAN_POINT('Ctrl Pts',(-54.3191335463697,-15.0371065180788,
2.));
#63137=CARTESIAN_POINT('Ctrl Pts',(-54.2887053621836,-15.0784511646849,
2.));
#63138=CARTESIAN_POINT('Ctrl Pts',(-54.2557752605174,-15.1176640701704,
2.));
#63139=CARTESIAN_POINT('Ctrl Pts',(-54.2373775276085,-15.1395719454944,
2.));
#63140=CARTESIAN_POINT('Ctrl Pts',(-54.2181982612199,-15.1608137789775,
2.));
#63141=CARTESIAN_POINT('Ctrl Pts',(-54.1982376363281,-15.1813315747386,
2.));
#63142=CARTESIAN_POINT('Ctrl Pts',(-54.1842200551681,-15.1957404356268,
2.));
#63143=CARTESIAN_POINT('Ctrl Pts',(-54.1698170448365,-15.2097921118142,
2.));
#63144=CARTESIAN_POINT('Ctrl Pts',(-54.1550457523822,-15.2234791283661,
2.));
#63145=CARTESIAN_POINT('Origin',(-53.1951359564886,-14.3971354987959,4.5));
#63146=CARTESIAN_POINT('Origin',(-39.0658530619283,38.8697713466882,6.));
#63147=CARTESIAN_POINT('Ctrl Pts',(-40.2595650866585,39.2869186252538,6.));
#63148=CARTESIAN_POINT('Ctrl Pts',(-40.2480819791952,39.3364939464135,6.));
#63149=CARTESIAN_POINT('Ctrl Pts',(-40.2334065100549,39.3851618422748,6.));
#63150=CARTESIAN_POINT('Ctrl Pts',(-40.2158026351646,39.4327533922847,6.));
#63151=CARTESIAN_POINT('Ctrl Pts',(-40.2039391979396,39.46482584051,6.));
#63152=CARTESIAN_POINT('Ctrl Pts',(-40.1907446643331,39.4964096047136,6.));
#63153=CARTESIAN_POINT('Ctrl Pts',(-40.1762870855865,39.5274524411797,6.));
#63154=CARTESIAN_POINT('Ctrl Pts',(-40.1696136376379,39.5417814486133,6.));
#63155=CARTESIAN_POINT('Ctrl Pts',(-40.1626709449503,39.5559951857844,6.));
#63156=CARTESIAN_POINT('Ctrl Pts',(-40.1554650290934,39.5700883780353,6.));
#63157=CARTESIAN_POINT('Ctrl Pts',(-40.1494095391196,39.5819315893728,6.));
#63158=CARTESIAN_POINT('Ctrl Pts',(-40.1431714820768,39.5936830081174,6.));
#63159=CARTESIAN_POINT('Ctrl Pts',(-40.1367585398302,39.6053334444843,6.));
#63160=CARTESIAN_POINT('Ctrl Pts',(-40.1108375205617,39.6524243387947,6.));
#63161=CARTESIAN_POINT('Ctrl Pts',(-40.082047067269,39.6978983470816,6.));
#63162=CARTESIAN_POINT('Ctrl Pts',(-40.0506487799185,39.741559756634,6.));
#63163=CARTESIAN_POINT('Ctrl Pts',(-40.0386313329921,39.7582708168956,6.));
#63164=CARTESIAN_POINT('Ctrl Pts',(-40.0262313128106,39.7747162395881,6.));
#63165=CARTESIAN_POINT('Ctrl Pts',(-40.0134614554123,39.7908844940418,6.));
#63166=CARTESIAN_POINT('Ctrl Pts',(-40.0042845094518,39.8025036682244,6.));
#63167=CARTESIAN_POINT('Ctrl Pts',(-39.9949165410966,39.8139796930109,6.));
#63168=CARTESIAN_POINT('Ctrl Pts',(-39.9853619687604,39.8253081417074,6.));
#63169=CARTESIAN_POINT('Ctrl Pts',(-39.9779669485307,39.8340761016259,6.));
#63170=CARTESIAN_POINT('Ctrl Pts',(-39.970459801146,39.8427558568435,6.));
#63171=CARTESIAN_POINT('Ctrl Pts',(-39.9628530937736,39.8513338610673,6.));
#63172=CARTESIAN_POINT('Ctrl Pts',(-39.9252574596781,39.8937300638237,6.));
#63173=CARTESIAN_POINT('Ctrl Pts',(-39.8851758119764,39.9337126572018,6.));
#63174=CARTESIAN_POINT('Ctrl Pts',(-39.8429000970909,39.9710687870014,6.));
#63175=CARTESIAN_POINT('Ctrl Pts',(-39.8012367829931,40.0078837805156,6.));
#63176=CARTESIAN_POINT('Ctrl Pts',(-39.7574416833132,40.0421487782755,6.));
#63177=CARTESIAN_POINT('Ctrl Pts',(-39.7117463596714,40.0736370674662,6.));
#63178=CARTESIAN_POINT('Ctrl Pts',(-39.6878846430372,40.0900799892815,6.));
#63179=CARTESIAN_POINT('Ctrl Pts',(-39.6635040440514,40.1057652810441,6.));
#63180=CARTESIAN_POINT('Ctrl Pts',(-39.6386333596486,40.120656825884,6.));
#63181=CARTESIAN_POINT('Ctrl Pts',(-39.6252910649646,40.1286456442187,6.));
#63182=CARTESIAN_POINT('Ctrl Pts',(-39.6118076808291,40.1364059738324,6.));
#63183=CARTESIAN_POINT('Ctrl Pts',(-39.5981873691344,40.1439318477466,6.));
#63184=CARTESIAN_POINT('Ctrl Pts',(-39.5885046150635,40.1492820326699,6.));
#63185=CARTESIAN_POINT('Ctrl Pts',(-39.5787526555666,40.1545137210612,6.));
#63186=CARTESIAN_POINT('Ctrl Pts',(-39.5689329316873,40.1596246755939,6.));
#63187=CARTESIAN_POINT('Ctrl Pts',(-39.5602883878672,40.1641239742467,6.));
#63188=CARTESIAN_POINT('Ctrl Pts',(-39.5516000264324,40.1685251725109,6.));
#63189=CARTESIAN_POINT('Ctrl Pts',(-39.5428697390936,40.1728269741793,6.));
#63190=CARTESIAN_POINT('Ctrl Pts',(-39.4996812011584,40.1941078916718,6.));
#63191=CARTESIAN_POINT('Ctrl Pts',(-39.4554640759948,40.2129597963788,6.));
#63192=CARTESIAN_POINT('Ctrl Pts',(-39.4103710639644,40.2292497271407,6.));
#63193=CARTESIAN_POINT('Ctrl Pts',(-39.3590466351126,40.2477907683076,6.));
#63194=CARTESIAN_POINT('Ctrl Pts',(-39.3065877413218,40.2630147095083,6.));
#63195=CARTESIAN_POINT('Ctrl Pts',(-39.2532910929857,40.2750393024528,6.));
#63196=CARTESIAN_POINT('Ctrl Pts',(-39.2011942210287,40.286793206282,6.));
#63197=CARTESIAN_POINT('Ctrl Pts',(-39.148296003785,40.2954900228404,6.));
#63198=CARTESIAN_POINT('Ctrl Pts',(-39.0948540754983,40.3011985092876,6.));
#63199=CARTESIAN_POINT('Ctrl Pts',(-39.0817639227262,40.3025967552359,6.));
#63200=CARTESIAN_POINT('Ctrl Pts',(-39.0686410906115,40.3038155206662,6.));
#63201=CARTESIAN_POINT('Ctrl Pts',(-39.0554892737564,40.3048554432527,6.));
#63202=CARTESIAN_POINT('Ctrl Pts',(-39.0455592030118,40.3056406203098,6.));
#63203=CARTESIAN_POINT('Ctrl Pts',(-39.0356145768843,40.306323605614,6.));
#63204=CARTESIAN_POINT('Ctrl Pts',(-39.0256685188148,40.3069043036838,6.));
#63205=CARTESIAN_POINT('Ctrl Pts',(-38.9681511420326,40.3102624410931,6.));
#63206=CARTESIAN_POINT('Ctrl Pts',(-38.9104821865459,40.3102125489983,6.));
#63207=CARTESIAN_POINT('Ctrl Pts',(-38.8529878289339,40.3068889012295,6.));
#63208=CARTESIAN_POINT('Ctrl Pts',(-38.7942601302541,40.3034939561811,6.));
#63209=CARTESIAN_POINT('Ctrl Pts',(-38.7357135780205,40.2966834252177,6.));
#63210=CARTESIAN_POINT('Ctrl Pts',(-38.6776775933238,40.2865489627448,6.));
#63211=CARTESIAN_POINT('Ctrl Pts',(-38.6191308064349,40.276325302067,6.));
#63212=CARTESIAN_POINT('Ctrl Pts',(-38.561102428243,40.2627189748103,6.));
#63213=CARTESIAN_POINT('Ctrl Pts',(-38.5039291823866,40.2457711881153,6.));
#63214=CARTESIAN_POINT('Ctrl Pts',(-38.4909781937364,40.2419321443485,6.));
#63215=CARTESIAN_POINT('Ctrl Pts',(-38.4780675599091,40.2379201262253,6.));
#63216=CARTESIAN_POINT('Ctrl Pts',(-38.4652269238002,40.2337440113392,6.));
#63217=CARTESIAN_POINT('Ctrl Pts',(-38.4073726902873,40.2149282826056,6.));
#63218=CARTESIAN_POINT('Ctrl Pts',(-38.3508402271714,40.1927581042671,6.));
#63219=CARTESIAN_POINT('Ctrl Pts',(-38.2959735972823,40.1673423641079,6.));
#63220=CARTESIAN_POINT('Ctrl Pts',(-38.2415891999933,40.142150007424,6.));
#63221=CARTESIAN_POINT('Ctrl Pts',(-38.1888403165397,40.1137687287949,6.));
#63222=CARTESIAN_POINT('Ctrl Pts',(-38.1380651655577,40.0822545048966,6.));
#63223=CARTESIAN_POINT('Ctrl Pts',(-38.1008618422864,40.0591638033102,6.));
#63224=CARTESIAN_POINT('Ctrl Pts',(-38.0647181228981,40.0343901127421,6.));
#63225=CARTESIAN_POINT('Ctrl Pts',(-38.0297736279237,40.0079388493487,6.));
#63226=CARTESIAN_POINT('Ctrl Pts',(-38.0103531401622,39.9932384956196,6.));
#63227=CARTESIAN_POINT('Ctrl Pts',(-37.9913031820638,39.978019748027,6.));
#63228=CARTESIAN_POINT('Ctrl Pts',(-37.972630261787,39.9623020734811,6.));
#63229=CARTESIAN_POINT('Ctrl Pts',(-37.5756558680257,39.2699729499894,6.));
#63230=CARTESIAN_POINT('Ctrl Pts',(-37.5651290682188,39.2098300642739,6.));
#63231=CARTESIAN_POINT('Ctrl Pts',(-37.5584870272447,39.1491583710678,6.));
#63232=CARTESIAN_POINT('Ctrl Pts',(-37.5555980370803,39.0882817362078,6.));
#63233=CARTESIAN_POINT('Ctrl Pts',(-37.5529191835609,39.0318330886644,6.));
#63234=CARTESIAN_POINT('Ctrl Pts',(-37.5534681438705,38.9752074993239,6.));
#63235=CARTESIAN_POINT('Ctrl Pts',(-37.5571795337599,38.9186719371971,6.));
#63236=CARTESIAN_POINT('Ctrl Pts',(-37.5580753630163,38.9050257798038,6.));
#63237=CARTESIAN_POINT('Ctrl Pts',(-37.5591557658557,38.8913844979252,6.));
#63238=CARTESIAN_POINT('Ctrl Pts',(-37.5604183353195,38.8777672140557,6.));
#63239=CARTESIAN_POINT('Ctrl Pts',(-37.5659749115735,38.8178374609894,6.));
#63240=CARTESIAN_POINT('Ctrl Pts',(-37.5750599728648,38.7582987522682,6.));
#63241=CARTESIAN_POINT('Ctrl Pts',(-37.587576042244,38.6994723221795,6.));
#63242=CARTESIAN_POINT('Ctrl Pts',(-37.5953014146754,38.6631625137662,6.));
#63243=CARTESIAN_POINT('Ctrl Pts',(-37.6043349305766,38.6271243505451,6.));
#63244=CARTESIAN_POINT('Ctrl Pts',(-37.6146623853363,38.591438145786,6.));
#63245=CARTESIAN_POINT('Ctrl Pts',(-37.6181962247196,38.5792270716391,6.));
#63246=CARTESIAN_POINT('Ctrl Pts',(-37.6218816203987,38.56705724719,6.));
#63247=CARTESIAN_POINT('Ctrl Pts',(-37.6257181655827,38.5549320256251,6.));
#63248=CARTESIAN_POINT('Ctrl Pts',(-37.6293072145904,38.5435890041466,6.));
#63249=CARTESIAN_POINT('Ctrl Pts',(-37.6330262982585,38.5322922610546,6.));
#63250=CARTESIAN_POINT('Ctrl Pts',(-37.636872579215,38.5210500434267,6.));
#63251=CARTESIAN_POINT('Ctrl Pts',(-37.6559105736999,38.4654042703744,6.));
#63252=CARTESIAN_POINT('Ctrl Pts',(-37.6780754632208,38.4110469589651,6.));
#63253=CARTESIAN_POINT('Ctrl Pts',(-37.7032762357134,38.3582791323017,6.));
#63254=CARTESIAN_POINT('Ctrl Pts',(-37.7278335946531,38.3068585474672,6.));
#63255=CARTESIAN_POINT('Ctrl Pts',(-37.7552744012006,38.2569465430614,6.));
#63256=CARTESIAN_POINT('Ctrl Pts',(-37.7855529342765,38.2088521687025,6.));
#63257=CARTESIAN_POINT('Ctrl Pts',(-37.8019690565523,38.1827768258755,6.));
#63258=CARTESIAN_POINT('Ctrl Pts',(-37.8192199432012,38.1572363736183,6.));
#63259=CARTESIAN_POINT('Ctrl Pts',(-37.8373023126813,38.1322851555406,6.));
#63260=CARTESIAN_POINT('Ctrl Pts',(-37.8523464601685,38.1115262718578,6.));
#63261=CARTESIAN_POINT('Ctrl Pts',(-37.8679662045719,38.0911753045226,6.));
#63262=CARTESIAN_POINT('Ctrl Pts',(-37.884160961773,38.0712658190693,6.));
#63263=CARTESIAN_POINT('Ctrl Pts',(-37.8910830994387,38.0627558922177,6.));
#63264=CARTESIAN_POINT('Ctrl Pts',(-37.8981112327979,38.0543257382737,6.));
#63265=CARTESIAN_POINT('Ctrl Pts',(-37.9052335275561,38.0459914463568,6.));
#63266=CARTESIAN_POINT('Ctrl Pts',(-37.9382051680373,38.0074090391303,6.));
#63267=CARTESIAN_POINT('Ctrl Pts',(-37.9732473043227,37.970810355559,6.));
#63268=CARTESIAN_POINT('Ctrl Pts',(-38.0103191942679,37.9364107324676,6.));
#63269=CARTESIAN_POINT('Ctrl Pts',(-38.0517460905842,37.8979700265516,6.));
#63270=CARTESIAN_POINT('Ctrl Pts',(-38.0957081060159,37.8622743231261,6.));
#63271=CARTESIAN_POINT('Ctrl Pts',(-38.1418690155727,37.8294138953178,6.));
#63272=CARTESIAN_POINT('Ctrl Pts',(-38.181041165507,37.8015285347958,6.));
#63273=CARTESIAN_POINT('Ctrl Pts',(-38.2217977223924,37.775685634311,6.));
#63274=CARTESIAN_POINT('Ctrl Pts',(-38.2639408148789,37.7519688192016,6.));
#63275=CARTESIAN_POINT('Ctrl Pts',(-38.2755270772501,37.7454484329116,6.));
#63276=CARTESIAN_POINT('Ctrl Pts',(-38.287218151903,37.7390889037126,6.));
#63277=CARTESIAN_POINT('Ctrl Pts',(-38.299009928843,37.7328923323578,6.));
#63278=CARTESIAN_POINT('Ctrl Pts',(-38.3081902153401,37.7280680975859,6.));
#63279=CARTESIAN_POINT('Ctrl Pts',(-38.31743317901,37.7233419167043,6.));
#63280=CARTESIAN_POINT('Ctrl Pts',(-38.3267216243912,37.7187221450337,6.));
#63281=CARTESIAN_POINT('Ctrl Pts',(-38.3764239787938,37.6940018049334,6.));
#63282=CARTESIAN_POINT('Ctrl Pts',(-38.427517840694,37.6722751487084,6.));
#63283=CARTESIAN_POINT('Ctrl Pts',(-38.4796831982367,37.6536175541641,6.));
#63284=CARTESIAN_POINT('Ctrl Pts',(-38.5315566484918,37.6350643639232,6.));
#63285=CARTESIAN_POINT('Ctrl Pts',(-38.5844908266812,37.6195458590518,6.));
#63286=CARTESIAN_POINT('Ctrl Pts',(-38.6381772424017,37.6071867480182,6.));
#63287=CARTESIAN_POINT('Ctrl Pts',(-38.6879882164427,37.5957197996179,6.));
#63288=CARTESIAN_POINT('Ctrl Pts',(-38.7384475151204,37.5869729726017,6.));
#63289=CARTESIAN_POINT('Ctrl Pts',(-38.7893004134472,37.5810866485612,6.));
#63290=CARTESIAN_POINT('Ctrl Pts',(-38.8023628187198,37.5795746491922,6.));
#63291=CARTESIAN_POINT('Ctrl Pts',(-38.8154556555427,37.5782513512257,6.));
#63292=CARTESIAN_POINT('Ctrl Pts',(-38.8285456601036,37.577121602081,6.));
#63293=CARTESIAN_POINT('Ctrl Pts',(-38.8814582148995,37.5725549181469,6.));
#63294=CARTESIAN_POINT('Ctrl Pts',(-38.9344079183634,37.5711349247241,6.));
#63295=CARTESIAN_POINT('Ctrl Pts',(-38.9871128327976,37.5729646742369,6.));
#63296=CARTESIAN_POINT('Ctrl Pts',(-39.0380304487625,37.5747323743462,6.));
#63297=CARTESIAN_POINT('Ctrl Pts',(-39.0887204479045,37.5795333200091,6.));
#63298=CARTESIAN_POINT('Ctrl Pts',(-39.1389156304824,37.5875063462533,6.));
#63299=CARTESIAN_POINT('Ctrl Pts',(-39.1740301727663,37.5930839565499,6.));
#63300=CARTESIAN_POINT('Ctrl Pts',(-39.2089023015726,37.6002148717553,6.));
#63301=CARTESIAN_POINT('Ctrl Pts',(-39.2434333426905,37.6089601149435,6.));
#63302=CARTESIAN_POINT('Ctrl Pts',(-39.2629126135314,37.6138933852742,6.));
#63303=CARTESIAN_POINT('Ctrl Pts',(-39.2822832137847,37.6193406085392,6.));
#63304=CARTESIAN_POINT('Ctrl Pts',(-39.3015295597332,37.6252918061955,6.));
#63305=CARTESIAN_POINT('Origin',(-39.0658530619283,38.8697713466882,0.895788276411275));
#63306=CARTESIAN_POINT('Ctrl Pts',(-39.838950903209,40.2073157943283,2.14578827641127));
#63307=CARTESIAN_POINT('Ctrl Pts',(-39.8806063786858,40.1836140086682,2.14826884812012));
#63308=CARTESIAN_POINT('Ctrl Pts',(-40.3479144857802,39.8865682523885,2.17691792328789));
#63309=CARTESIAN_POINT('Ctrl Pts',(-40.8820206309179,38.8100483503822,2.23173550191459));
#63310=CARTESIAN_POINT('Ctrl Pts',(-40.0177367088945,37.3220789090571,2.31024101229137));
#63311=CARTESIAN_POINT('Ctrl Pts',(-38.2999828751462,37.2220283999294,2.38874652266815));
#63312=CARTESIAN_POINT('Ctrl Pts',(-37.2689794778046,38.599756793647,2.46725203304492));
#63313=CARTESIAN_POINT('Ctrl Pts',(-37.8495046941264,40.2196189105814,2.5457575434217));
#63314=CARTESIAN_POINT('Ctrl Pts',(-39.1164929505456,40.5298919958252,2.60526962454382));
#63315=CARTESIAN_POINT('Ctrl Pts',(-39.7159505584363,40.2768331102243,2.63861320220701));
#63316=CARTESIAN_POINT('Ctrl Pts',(-39.8359404161091,40.2062105265248,2.64578827641127));
#63317=CARTESIAN_POINT('Ctrl Pts',(-39.8351916364771,40.2053827942122,2.10421172358873));
#63318=CARTESIAN_POINT('Ctrl Pts',(-40.1301403364056,40.0323966656676,2.12181148931034));
#63319=CARTESIAN_POINT('Ctrl Pts',(-40.7310614116502,39.3634532239961,2.16557975849088));
#63320=CARTESIAN_POINT('Ctrl Pts',(-40.5621188491035,37.8394675163551,2.23551653113034));
#63321=CARTESIAN_POINT('Ctrl Pts',(-39.0323736383015,37.0530949705804,2.31402204150712));
#63322=CARTESIAN_POINT('Ctrl Pts',(-37.5317729583208,37.8957949010443,2.3925275518839));
#63323=CARTESIAN_POINT('Ctrl Pts',(-37.4074081512687,39.612062461691,2.47103306226068));
#63324=CARTESIAN_POINT('Ctrl Pts',(-38.6322604476799,40.5562805179572,2.54159445282895));
#63325=CARTESIAN_POINT('Ctrl Pts',(-39.5301075010648,40.379146656691,2.5859873399383));
#63326=CARTESIAN_POINT('Ctrl Pts',(-39.8379370462828,40.204596038962,2.60421172358873));
#63327=CARTESIAN_POINT('Ctrl Pts',(-39.3014489339361,37.6274127691862,2.));
#63328=CARTESIAN_POINT('Ctrl Pts',(-38.8929078719872,37.5499386892516,2.02616850345893));
#63329=CARTESIAN_POINT('Ctrl Pts',(-38.0001476420674,37.8306642325621,2.07850551037678));
#63330=CARTESIAN_POINT('Ctrl Pts',(-37.610255111015,39.1875822847128,2.15701102075356));
#63331=CARTESIAN_POINT('Ctrl Pts',(-38.5285686312713,40.258225513388,2.23551653113034));
#63332=CARTESIAN_POINT('Ctrl Pts',(-39.9273700409771,40.0842697726412,2.31402204150712));
#63333=CARTESIAN_POINT('Ctrl Pts',(-40.5542159206369,38.8208279060991,2.3925275518839));
#63334=CARTESIAN_POINT('Ctrl Pts',(-39.8459288050189,37.6014258590767,2.47103306226067));
#63335=CARTESIAN_POINT('Ctrl Pts',(-38.4382167358195,37.5194337211688,2.54953857263746));
#63336=CARTESIAN_POINT('Ctrl Pts',(-37.5933017676156,38.6484924080488,2.62804408301423));
#63337=CARTESIAN_POINT('Ctrl Pts',(-38.0690465090537,39.9759814857309,2.70654959339101));
#63338=CARTESIAN_POINT('Ctrl Pts',(-39.4387308817872,40.3114038497387,2.7850551037678));
#63339=CARTESIAN_POINT('Ctrl Pts',(-40.4740195694907,39.3539315296908,2.86356061414457));
#63340=CARTESIAN_POINT('Ctrl Pts',(-40.2464260929064,37.9622550204806,2.94206612452135));
#63341=CARTESIAN_POINT('Ctrl Pts',(-38.9600691167361,37.3844596499182,3.02057163489813));
#63342=CARTESIAN_POINT('Ctrl Pts',(-37.768580477053,38.1387276546801,3.09907714527491));
#63343=CARTESIAN_POINT('Ctrl Pts',(-37.7405173375704,39.5486127570041,3.17758265565169));
#63344=CARTESIAN_POINT('Ctrl Pts',(-38.9010464836382,40.3496968754357,3.25608816602847));
#63345=CARTESIAN_POINT('Ctrl Pts',(-40.2093782359874,39.823548531307,3.33459367640525));
#63346=CARTESIAN_POINT('Ctrl Pts',(-40.4921693526885,38.4420301655715,3.41309918678203));
#63347=CARTESIAN_POINT('Ctrl Pts',(-39.4958061477021,37.4441202440019,3.49160469715882));
#63348=CARTESIAN_POINT('Ctrl Pts',(-38.1138507756971,37.7247681321827,3.57011020753558));
#63349=CARTESIAN_POINT('Ctrl Pts',(-37.5856736955423,39.032282120084,3.64861571791237));
#63350=CARTESIAN_POINT('Ctrl Pts',(-38.3849566559494,40.1940525848875,3.72712122828914));
#63351=CARTESIAN_POINT('Ctrl Pts',(-39.7948837028381,40.1681761513166,3.80562673866593));
#63352=CARTESIAN_POINT('Ctrl Pts',(-40.5509987381473,38.9778594216365,3.8841322490427));
#63353=CARTESIAN_POINT('Ctrl Pts',(-39.975199824256,37.6906067364409,3.96263775941949));
#63354=CARTESIAN_POINT('Ctrl Pts',(-38.5838771151456,37.4608569069011,4.04114326979626));
#63355=CARTESIAN_POINT('Ctrl Pts',(-37.6248018935901,38.4946550418589,4.11964878017305));
#63356=CARTESIAN_POINT('Ctrl Pts',(-37.9580956187159,39.8648663970342,4.19815429054983));
#63357=CARTESIAN_POINT('Ctrl Pts',(-39.2848525544709,40.3426528537363,4.2766598009266));
#63358=CARTESIAN_POINT('Ctrl Pts',(-40.4152055386856,39.4995241597319,4.35516531130339));
#63359=CARTESIAN_POINT('Ctrl Pts',(-40.3354271431306,38.09161817034,4.43367082168016));
#63360=CARTESIAN_POINT('Ctrl Pts',(-39.1170645283528,37.381578451311,4.51217633205694));
#63361=CARTESIAN_POINT('Ctrl Pts',(-37.8527742546189,38.0061854960201,4.59068184243372));
#63362=CARTESIAN_POINT('Ctrl Pts',(-37.6764018913215,39.4052768714559,4.6691873528105));
#63363=CARTESIAN_POINT('Ctrl Pts',(-38.7461223767003,40.3241141426736,4.74769286318728));
#63364=CARTESIAN_POINT('Ctrl Pts',(-40.1025849285147,39.9386622571232,4.82619837356406));
#63365=CARTESIAN_POINT('Ctrl Pts',(-40.5292817221821,38.5946035156581,4.90470388394085));
#63366=CARTESIAN_POINT('Ctrl Pts',(-39.6435408484723,37.4973219800824,4.98320939431762));
#63367=CARTESIAN_POINT('Ctrl Pts',(-38.2397159426158,37.6308853554897,5.0617149046944));
#63368=CARTESIAN_POINT('Ctrl Pts',(-37.576790226709,38.8755117639716,5.14022041507117));
#63369=CARTESIAN_POINT('Ctrl Pts',(-38.2492919033736,40.1149887727412,5.21872592544796));
#63370=CARTESIAN_POINT('Ctrl Pts',(-39.6541041493256,40.2377277253793,5.29723143582474));
#63371=CARTESIAN_POINT('Ctrl Pts',(-40.5313606306742,39.1336457644378,5.37573694620152));
#63372=CARTESIAN_POINT('Ctrl Pts',(-40.0943114632433,37.792925260964,5.4542424565783));
#63373=CARTESIAN_POINT('Ctrl Pts',(-38.7349236527553,37.4179251395397,5.53274796695507));
#63374=CARTESIAN_POINT('Ctrl Pts',(-37.6723064797637,38.3450171336682,5.61125347733186));
#63375=CARTESIAN_POINT('Ctrl Pts',(-37.8594847038433,39.742636643005,5.68975898770863));
#63376=CARTESIAN_POINT('Ctrl Pts',(-39.1285028721539,40.3576202841945,5.76826449808542));
#63377=CARTESIAN_POINT('Ctrl Pts',(-40.3414559726879,39.6379218175554,5.84677000846219));
#63378=CARTESIAN_POINT('Ctrl Pts',(-40.4101742470826,38.2300213301991,5.92527551883897));
#63379=CARTESIAN_POINT('Ctrl Pts',(-39.2737694148596,37.3944612175239,6.00378102921576));
#63380=CARTESIAN_POINT('Ctrl Pts',(-37.9498583767322,37.8848716060229,6.08228653959253));
#63381=CARTESIAN_POINT('Ctrl Pts',(-37.7367752723626,38.7961472226316,6.13462354651038));
#63382=CARTESIAN_POINT('Ctrl Pts',(-37.8446253550652,39.1977395433015,6.16079204996931));
#63383=CARTESIAN_POINT('Ctrl Pts',(-39.3187452171453,37.5362049495383,1.94640265001023));
#63384=CARTESIAN_POINT('Ctrl Pts',(-38.8802110918637,37.4530431059918,1.97257115346916));
#63385=CARTESIAN_POINT('Ctrl Pts',(-37.9219088231848,37.7543781296798,2.02490816038701));
#63386=CARTESIAN_POINT('Ctrl Pts',(-37.5033923116663,39.2109143912739,2.10341367076379));
#63387=CARTESIAN_POINT('Ctrl Pts',(-38.4891238668221,40.3601589483231,2.18191918114057));
#63388=CARTESIAN_POINT('Ctrl Pts',(-39.9906183548469,40.1734322378127,2.26042469151735));
#63389=CARTESIAN_POINT('Ctrl Pts',(-40.6634841573972,38.8172347208602,2.33893020189413));
#63390=CARTESIAN_POINT('Ctrl Pts',(-39.9031981063108,37.5083102090701,2.4174357122709));
#63391=CARTESIAN_POINT('Ctrl Pts',(-38.3921387822617,37.420298614089,2.49594122264769));
#63392=CARTESIAN_POINT('Ctrl Pts',(-37.4851943376786,38.6322472032482,2.57444673302446));
#63393=CARTESIAN_POINT('Ctrl Pts',(-37.9958659040779,40.0571939606811,2.65295224340125));
#63394=CARTESIAN_POINT('Ctrl Pts',(-39.4661057263452,40.4172413750055,2.73145775377802));
#63395=CARTESIAN_POINT('Ctrl Pts',(-40.5774001869564,39.3894761747327,2.8099632641548));
#63396=CARTESIAN_POINT('Ctrl Pts',(-40.3330979234396,37.8956296621443,2.88846877453158));
#63397=CARTESIAN_POINT('Ctrl Pts',(-38.9523029828924,37.2754154143704,2.96697428490836));
#63398=CARTESIAN_POINT('Ctrl Pts',(-37.6733411426948,38.0850580439713,3.04547979528514));
#63399=CARTESIAN_POINT('Ctrl Pts',(-37.6432177463661,39.5984499344847,3.12398530566192));
#63400=CARTESIAN_POINT('Ctrl Pts',(-38.8889472001127,40.4583456851777,3.2024908160387));
#63401=CARTESIAN_POINT('Ctrl Pts',(-40.2933301961761,39.893570132972,3.28099632641548));
#63402=CARTESIAN_POINT('Ctrl Pts',(-40.5968824374326,38.4106275244905,3.35950183679226));
#63403=CARTESIAN_POINT('Ctrl Pts',(-39.5273711758787,37.3394559940749,3.43800734716904));
#63404=CARTESIAN_POINT('Ctrl Pts',(-38.0439594782896,37.6407076615778,3.51651285754582));
#63405=CARTESIAN_POINT('Ctrl Pts',(-37.4770062502969,39.0442128569736,3.5950183679226));
#63406=CARTESIAN_POINT('Ctrl Pts',(-38.3349686108551,40.2912747609356,3.67352387829938));
#63407=CARTESIAN_POINT('Ctrl Pts',(-39.8484055252959,40.2634986076469,3.75202938867616));
#63408=CARTESIAN_POINT('Ctrl Pts',(-40.6600307852877,38.9857947132862,3.83053489905294));
#63409=CARTESIAN_POINT('Ctrl Pts',(-40.0419595641554,37.6040383051891,3.90904040942972));
#63410=CARTESIAN_POINT('Ctrl Pts',(-38.5484928259196,37.3574213799521,3.9875459198065));
#63411=CARTESIAN_POINT('Ctrl Pts',(-37.5190070470414,38.4671158588103,4.06605143018328));
#63412=CARTESIAN_POINT('Ctrl Pts',(-37.8767695483496,39.9379213519627,4.14455694056006));
#63413=CARTESIAN_POINT('Ctrl Pts',(-39.3009304136176,40.4507845262585,4.22306245093683));
#63414=CARTESIAN_POINT('Ctrl Pts',(-40.5142683210177,39.5457574952881,4.30156796131362));
#63415=CARTESIAN_POINT('Ctrl Pts',(-40.4286329903996,38.0344900143857,4.38007347169039));
#63416=CARTESIAN_POINT('Ctrl Pts',(-39.1208242208266,37.2723226924175,4.45857898206717));
#63417=CARTESIAN_POINT('Ctrl Pts',(-37.7637160108241,37.9427852958327,4.53708449244395));
#63418=CARTESIAN_POINT('Ctrl Pts',(-37.5743952612928,39.4445910374365,4.61559000282073));
#63419=CARTESIAN_POINT('Ctrl Pts',(-38.7226493317982,40.430884794758,4.69409551319751));
#63420=CARTESIAN_POINT('Ctrl Pts',(-40.1786966524752,40.0171349389622,4.77260102357429));
#63421=CARTESIAN_POINT('Ctrl Pts',(-40.6367194134648,38.574402055017,4.85110653395107));
#63422=CARTESIAN_POINT('Ctrl Pts',(-39.6859518273974,37.3965635383795,4.92961204432785));
#63423=CARTESIAN_POINT('Ctrl Pts',(-38.1790650429906,37.539932475946,5.00811755470463));
#63424=CARTESIAN_POINT('Ctrl Pts',(-37.4674706011366,38.8759331970053,5.08662306508141));
#63425=CARTESIAN_POINT('Ctrl Pts',(-38.1893440234059,40.2064064749044,5.16512857545819));
#63426=CARTESIAN_POINT('Ctrl Pts',(-39.6972906335328,40.3381563141404,5.24363408583496));
#63427=CARTESIAN_POINT('Ctrl Pts',(-40.6389509451321,39.1530181185549,5.32213959621175));
#63428=CARTESIAN_POINT('Ctrl Pts',(-40.1698157903201,37.713868549517,5.40064510658852));
#63429=CARTESIAN_POINT('Ctrl Pts',(-38.7106284529518,37.3113377746548,5.47915061696531));
#63430=CARTESIAN_POINT('Ctrl Pts',(-37.5699991848822,38.3064922757992,5.55765612734208));
#63431=CARTESIAN_POINT('Ctrl Pts',(-37.7709191080277,39.8067180941779,5.63616163771886));
#63432=CARTESIAN_POINT('Ctrl Pts',(-39.1331023112333,40.4668507914031,5.71466714809565));
#63433=CARTESIAN_POINT('Ctrl Pts',(-40.4351044267927,39.694315624366,5.79317265847242));
#63434=CARTESIAN_POINT('Ctrl Pts',(-40.5088676568798,38.1830540494315,5.8716781688492));
#63435=CARTESIAN_POINT('Ctrl Pts',(-39.2890336047347,37.2861512475826,5.95018367922599));
#63436=CARTESIAN_POINT('Ctrl Pts',(-37.8679275688169,37.8125651402854,6.02868918960276));
#63437=CARTESIAN_POINT('Ctrl Pts',(-37.6392009572462,38.7907421037309,6.08102619652061));
#63438=CARTESIAN_POINT('Ctrl Pts',(-37.7549688593853,39.2218173455308,6.10719469997954));
#63439=CARTESIAN_POINT('Ctrl Pts',(-39.3360415003545,37.4449971298904,1.89280530002046));
#63440=CARTESIAN_POINT('Ctrl Pts',(-38.8675143117401,37.356147522732,1.91897380347939));
#63441=CARTESIAN_POINT('Ctrl Pts',(-37.8436700043022,37.6780920267975,1.97131081039724));
#63442=CARTESIAN_POINT('Ctrl Pts',(-37.3965295123175,39.2342464978351,2.04981632077402));
#63443=CARTESIAN_POINT('Ctrl Pts',(-38.449679102373,40.462092383258,2.1283218311508));
#63444=CARTESIAN_POINT('Ctrl Pts',(-40.0538666687167,40.2625947029841,2.20682734152758));
#63445=CARTESIAN_POINT('Ctrl Pts',(-40.7727523941575,38.8136415356212,2.28533285190436));
#63446=CARTESIAN_POINT('Ctrl Pts',(-39.9604674076027,37.4151945590636,2.36383836228113));
#63447=CARTESIAN_POINT('Ctrl Pts',(-38.3460608287039,37.3211635070092,2.44234387265792));
#63448=CARTESIAN_POINT('Ctrl Pts',(-37.3770869077416,38.6160019984476,2.52084938303469));
#63449=CARTESIAN_POINT('Ctrl Pts',(-37.9226852991021,40.1384064356312,2.59935489341147));
#63450=CARTESIAN_POINT('Ctrl Pts',(-39.4934805709032,40.5230789002723,2.67786040378825));
#63451=CARTESIAN_POINT('Ctrl Pts',(-40.6807808044221,39.4250208197745,2.75636591416503));
#63452=CARTESIAN_POINT('Ctrl Pts',(-40.4197697539727,37.829004303808,2.83487142454181));
#63453=CARTESIAN_POINT('Ctrl Pts',(-38.9445368490487,37.1663711788227,2.91337693491859));
#63454=CARTESIAN_POINT('Ctrl Pts',(-37.5781018083366,38.0313884332623,2.99188244529537));
#63455=CARTESIAN_POINT('Ctrl Pts',(-37.5459181551618,39.6482871119655,3.07038795567215));
#63456=CARTESIAN_POINT('Ctrl Pts',(-38.8768479165872,40.5669944949197,3.14889346604893));
#63457=CARTESIAN_POINT('Ctrl Pts',(-40.3772821563647,39.963591734637,3.22739897642571));
#63458=CARTESIAN_POINT('Ctrl Pts',(-40.7015955221767,38.3792248834095,3.30590448680249));
#63459=CARTESIAN_POINT('Ctrl Pts',(-39.5589362040553,37.2347917441478,3.38440999717927));
#63460=CARTESIAN_POINT('Ctrl Pts',(-37.9740681808821,37.5566471909729,3.46291550755605));
#63461=CARTESIAN_POINT('Ctrl Pts',(-37.3683388050514,39.0561435938632,3.54142101793282));
#63462=CARTESIAN_POINT('Ctrl Pts',(-38.2849805657609,40.3884969369837,3.61992652830961));
#63463=CARTESIAN_POINT('Ctrl Pts',(-39.9019273477536,40.3588210639771,3.69843203868638));
#63464=CARTESIAN_POINT('Ctrl Pts',(-40.7690628324281,38.9937300049359,3.77693754906317));
#63465=CARTESIAN_POINT('Ctrl Pts',(-40.1087193040547,37.5174698739372,3.85544305943995));
#63466=CARTESIAN_POINT('Ctrl Pts',(-38.5131085366936,37.2539858530032,3.93394856981672));
#63467=CARTESIAN_POINT('Ctrl Pts',(-37.4132122004928,38.4395766757617,4.01245408019351));
#63468=CARTESIAN_POINT('Ctrl Pts',(-37.7954434779833,40.0109763068912,4.09095959057028));
#63469=CARTESIAN_POINT('Ctrl Pts',(-39.3170082727643,40.5589161987807,4.16946510094707));
#63470=CARTESIAN_POINT('Ctrl Pts',(-40.6133311033498,39.5919908308443,4.24797061132384));
#63471=CARTESIAN_POINT('Ctrl Pts',(-40.5218388376685,37.9773618584313,4.32647612170062));
#63472=CARTESIAN_POINT('Ctrl Pts',(-39.1245839133004,37.163066933524,4.4049816320774));
#63473=CARTESIAN_POINT('Ctrl Pts',(-37.6746577670293,37.8793850956452,4.48348714245418));
#63474=CARTESIAN_POINT('Ctrl Pts',(-37.472388631264,39.4839052034172,4.56199265283096));
#63475=CARTESIAN_POINT('Ctrl Pts',(-38.6991762868962,40.5376554468423,4.64049816320775));
#63476=CARTESIAN_POINT('Ctrl Pts',(-40.2548083764357,40.0956076208012,4.71900367358451));
#63477=CARTESIAN_POINT('Ctrl Pts',(-40.7441571047475,38.554200594376,4.7975091839613));
#63478=CARTESIAN_POINT('Ctrl Pts',(-39.7283628063224,37.2958050966767,4.87601469433807));
#63479=CARTESIAN_POINT('Ctrl Pts',(-38.1184141433653,37.4489795964024,4.95452020471486));
#63480=CARTESIAN_POINT('Ctrl Pts',(-37.3581509755643,38.876354630039,5.03302571509164));
#63481=CARTESIAN_POINT('Ctrl Pts',(-38.1293961434382,40.2978241770675,5.11153122546842));
#63482=CARTESIAN_POINT('Ctrl Pts',(-39.7404771177401,40.4385849029016,5.1900367358452));
#63483=CARTESIAN_POINT('Ctrl Pts',(-40.7465412595899,39.172390472672,5.26854224622198));
#63484=CARTESIAN_POINT('Ctrl Pts',(-40.245320117397,37.63481183807,5.34704775659875));
#63485=CARTESIAN_POINT('Ctrl Pts',(-38.6863332531482,37.2047504097698,5.42555326697554));
#63486=CARTESIAN_POINT('Ctrl Pts',(-37.4676918900007,38.2679674179302,5.50405877735231));
#63487=CARTESIAN_POINT('Ctrl Pts',(-37.682353512212,39.8707995453507,5.5825642877291));
#63488=CARTESIAN_POINT('Ctrl Pts',(-39.1377017503128,40.5760812986115,5.66106979810587));
#63489=CARTESIAN_POINT('Ctrl Pts',(-40.5287528808974,39.7507094311768,5.73957530848266));
#63490=CARTESIAN_POINT('Ctrl Pts',(-40.6075610666769,38.1360867686637,5.81808081885943));
#63491=CARTESIAN_POINT('Ctrl Pts',(-39.3042977946098,37.1778412776413,5.89658632923621));
#63492=CARTESIAN_POINT('Ctrl Pts',(-37.7859967609015,37.7402586745478,5.97509183961299));
#63493=CARTESIAN_POINT('Ctrl Pts',(-37.5416266421298,38.7853369848302,6.02742884653084));
#63494=CARTESIAN_POINT('Ctrl Pts',(-37.6653123637055,39.2458951477601,6.05359734998977));
#63495=CARTESIAN_POINT('Ctrl Pts',(-39.3533377835637,37.3537893102425,1.83920795003069));
#63496=CARTESIAN_POINT('Ctrl Pts',(-38.8548175316166,37.2592519394721,1.86537645348962));
#63497=CARTESIAN_POINT('Ctrl Pts',(-37.7654311854196,37.6018059239151,1.91771346040747));
#63498=CARTESIAN_POINT('Ctrl Pts',(-37.2896667129688,39.2575786043963,1.99621897078425));
#63499=CARTESIAN_POINT('Ctrl Pts',(-38.4102343379238,40.564025818193,2.07472448116103));
#63500=CARTESIAN_POINT('Ctrl Pts',(-40.1171149825865,40.3517571681556,2.15322999153781));
#63501=CARTESIAN_POINT('Ctrl Pts',(-40.8820206309179,38.8100483503822,2.23173550191459));
#63502=CARTESIAN_POINT('Ctrl Pts',(-40.0177367088945,37.3220789090571,2.31024101229137));
#63503=CARTESIAN_POINT('Ctrl Pts',(-38.2999828751462,37.2220283999294,2.38874652266815));
#63504=CARTESIAN_POINT('Ctrl Pts',(-37.2689794778046,38.599756793647,2.46725203304492));
#63505=CARTESIAN_POINT('Ctrl Pts',(-37.8495046941264,40.2196189105814,2.5457575434217));
#63506=CARTESIAN_POINT('Ctrl Pts',(-39.5208554154611,40.6289164255391,2.62426305379848));
#63507=CARTESIAN_POINT('Ctrl Pts',(-40.7841614218878,39.4605654648164,2.70276856417526));
#63508=CARTESIAN_POINT('Ctrl Pts',(-40.5064415845058,37.7623789454716,2.78127407455204));
#63509=CARTESIAN_POINT('Ctrl Pts',(-38.936770715205,37.0573269432749,2.85977958492882));
#63510=CARTESIAN_POINT('Ctrl Pts',(-37.4828624739785,37.9777188225534,2.9382850953056));
#63511=CARTESIAN_POINT('Ctrl Pts',(-37.4486185639574,39.6981242894461,3.01679060568238));
#63512=CARTESIAN_POINT('Ctrl Pts',(-38.8647486330618,40.6756433046616,3.09529611605916));
#63513=CARTESIAN_POINT('Ctrl Pts',(-40.4612341165533,40.033613336302,3.17380162643594));
#63514=CARTESIAN_POINT('Ctrl Pts',(-40.8063086069208,38.3478222423284,3.25230713681272));
#63515=CARTESIAN_POINT('Ctrl Pts',(-39.590501232232,37.1301274942208,3.3308126471895));
#63516=CARTESIAN_POINT('Ctrl Pts',(-37.9041768834746,37.4725867203679,3.40931815756627));
#63517=CARTESIAN_POINT('Ctrl Pts',(-37.259671359806,39.0680743307528,3.48782366794306));
#63518=CARTESIAN_POINT('Ctrl Pts',(-38.2349925206666,40.4857191130317,3.56632917831984));
#63519=CARTESIAN_POINT('Ctrl Pts',(-39.9554491702114,40.4541435203075,3.64483468869662));
#63520=CARTESIAN_POINT('Ctrl Pts',(-40.8780948795684,39.0016652965855,3.7233401990734));
#63521=CARTESIAN_POINT('Ctrl Pts',(-40.1754790439541,37.4309014426854,3.80184570945018));
#63522=CARTESIAN_POINT('Ctrl Pts',(-38.4777242474675,37.1505503260543,3.88035121982696));
#63523=CARTESIAN_POINT('Ctrl Pts',(-37.3074173539442,38.412037492713,3.95885673020373));
#63524=CARTESIAN_POINT('Ctrl Pts',(-37.7141174076169,40.0840312618198,4.03736224058051));
#63525=CARTESIAN_POINT('Ctrl Pts',(-39.333086131911,40.6670478713028,4.11586775095729));
#63526=CARTESIAN_POINT('Ctrl Pts',(-40.7123938856819,39.6382241664006,4.19437326133407));
#63527=CARTESIAN_POINT('Ctrl Pts',(-40.6150446849375,37.9202337024768,4.27287877171085));
#63528=CARTESIAN_POINT('Ctrl Pts',(-39.1283436057741,37.0538111746305,4.35138428208763));
#63529=CARTESIAN_POINT('Ctrl Pts',(-37.5855995232345,37.8159848954577,4.42988979246441));
#63530=CARTESIAN_POINT('Ctrl Pts',(-37.3703820012353,39.5232193693979,4.50839530284119));
#63531=CARTESIAN_POINT('Ctrl Pts',(-38.6757032419941,40.6444260989267,4.58690081321797));
#63532=CARTESIAN_POINT('Ctrl Pts',(-40.3309201003962,40.1740803026401,4.66540632359475));
#63533=CARTESIAN_POINT('Ctrl Pts',(-40.8515947960302,38.533999133735,4.74391183397153));
#63534=CARTESIAN_POINT('Ctrl Pts',(-39.7707737852476,37.1950466549738,4.82241734434831));
#63535=CARTESIAN_POINT('Ctrl Pts',(-38.05776324374,37.3580267168588,4.90092285472509));
#63536=CARTESIAN_POINT('Ctrl Pts',(-37.248831349992,38.8767760630727,4.97942836510187));
#63537=CARTESIAN_POINT('Ctrl Pts',(-38.0694482634705,40.3892418792306,5.05793387547865));
#63538=CARTESIAN_POINT('Ctrl Pts',(-39.7836636019473,40.5390134916628,5.13643938585543));
#63539=CARTESIAN_POINT('Ctrl Pts',(-40.8541315740477,39.1917628267891,5.2149448962322));
#63540=CARTESIAN_POINT('Ctrl Pts',(-40.3208244444739,37.5557551266231,5.29345040660899));
#63541=CARTESIAN_POINT('Ctrl Pts',(-38.6620380533448,37.0981630448849,5.37195591698576));
#63542=CARTESIAN_POINT('Ctrl Pts',(-37.3653845951193,38.2294425600612,5.45046142736254));
#63543=CARTESIAN_POINT('Ctrl Pts',(-37.5937879163964,39.9348809965236,5.52896693773932));
#63544=CARTESIAN_POINT('Ctrl Pts',(-39.1423011893922,40.6853118058201,5.6074724481161));
#63545=CARTESIAN_POINT('Ctrl Pts',(-40.6224013350023,39.8071032379875,5.68597795849288));
#63546=CARTESIAN_POINT('Ctrl Pts',(-40.7062544764741,38.0891194878961,5.76448346886966));
#63547=CARTESIAN_POINT('Ctrl Pts',(-39.3195619844849,37.0695313077001,5.84298897924644));
#63548=CARTESIAN_POINT('Ctrl Pts',(-37.7040659529861,37.6679522088103,5.92149448962322));
#63549=CARTESIAN_POINT('Ctrl Pts',(-37.4440523270134,38.7799318659295,5.97383149654107));
#63550=CARTESIAN_POINT('Ctrl Pts',(-37.5756558680257,39.2699729499894,6.));
#63551=CARTESIAN_POINT('Ctrl Pts',(-39.3014489339361,37.6274127691862,2.));
#63552=CARTESIAN_POINT('Ctrl Pts',(-39.2531837869401,37.6126947647985,2.));
#63553=CARTESIAN_POINT('Ctrl Pts',(-39.204168956439,37.6011555074407,2.));
#63554=CARTESIAN_POINT('Ctrl Pts',(-39.1546825373221,37.5926368604753,2.));
#63555=CARTESIAN_POINT('Ctrl Pts',(-39.1029779407396,37.5837363739855,2.));
#63556=CARTESIAN_POINT('Ctrl Pts',(-39.0507578251671,37.5781330493143,2.));
#63557=CARTESIAN_POINT('Ctrl Pts',(-38.9983103424742,37.5756956341644,2.));
#63558=CARTESIAN_POINT('Ctrl Pts',(-38.9562475821286,37.573740832827,2.));
#63559=CARTESIAN_POINT('Ctrl Pts',(-38.914037803618,37.5738233147571,2.));
#63560=CARTESIAN_POINT('Ctrl Pts',(-38.871822235207,37.5758984072385,2.));
#63561=CARTESIAN_POINT('Ctrl Pts',(-38.8539763703757,37.5767756148974,2.));
#63562=CARTESIAN_POINT('Ctrl Pts',(-38.8361294237355,37.5780091556834,2.));
#63563=CARTESIAN_POINT('Ctrl Pts',(-38.8182919536766,37.5795967458236,2.));
#63564=CARTESIAN_POINT('Ctrl Pts',(-38.8081693423886,37.5804976896133,2.));
#63565=CARTESIAN_POINT('Ctrl Pts',(-38.7980490773292,37.5815128494685,2.));
#63566=CARTESIAN_POINT('Ctrl Pts',(-38.7879491906638,37.5826397882181,2.));
#63567=CARTESIAN_POINT('Ctrl Pts',(-38.7338460090771,37.5886765858403,2.));
#63568=CARTESIAN_POINT('Ctrl Pts',(-38.6802200536741,37.5979256005394,2.));
#63569=CARTESIAN_POINT('Ctrl Pts',(-38.6273722027196,37.6102449557342,2.));
#63570=CARTESIAN_POINT('Ctrl Pts',(-38.5735560674545,37.6227900275503,2.));
#63571=CARTESIAN_POINT('Ctrl Pts',(-38.5205457122299,37.6385189267469,2.));
#63572=CARTESIAN_POINT('Ctrl Pts',(-38.4686492447641,37.6573343726358,2.));
#63573=CARTESIAN_POINT('Ctrl Pts',(-38.4315334390262,37.6707909809289,2.));
#63574=CARTESIAN_POINT('Ctrl Pts',(-38.3949871291098,37.6858274526273,2.));
#63575=CARTESIAN_POINT('Ctrl Pts',(-38.3591250016197,37.7024243845625,2.));
#63576=CARTESIAN_POINT('Ctrl Pts',(-38.3438782291903,37.7094805650501,2.));
#63577=CARTESIAN_POINT('Ctrl Pts',(-38.32875516918,37.7168189666934,2.));
#63578=CARTESIAN_POINT('Ctrl Pts',(-38.3137649009439,37.7244388227708,2.));
#63579=CARTESIAN_POINT('Ctrl Pts',(-38.3048335703805,37.7289787984671,2.));
#63580=CARTESIAN_POINT('Ctrl Pts',(-38.2959544590106,37.7336161783506,2.));
#63581=CARTESIAN_POINT('Ctrl Pts',(-38.2871359717232,37.7383467951739,2.));
#63582=CARTESIAN_POINT('Ctrl Pts',(-38.2370624084947,37.7652084136004,2.));
#63583=CARTESIAN_POINT('Ctrl Pts',(-38.1888771643531,37.7951055006477,2.));
#63584=CARTESIAN_POINT('Ctrl Pts',(-38.1428979102524,37.8279238866887,2.));
#63585=CARTESIAN_POINT('Ctrl Pts',(-38.1146649271969,37.8480756041345,2.));
#63586=CARTESIAN_POINT('Ctrl Pts',(-38.0872636609501,37.8693298051536,2.));
#63587=CARTESIAN_POINT('Ctrl Pts',(-38.0607696487925,37.891669608828,2.));
#63588=CARTESIAN_POINT('Ctrl Pts',(-38.0187586294166,37.9270933838091,2.));
#63589=CARTESIAN_POINT('Ctrl Pts',(-37.9790269569637,37.9652445703229,2.));
#63590=CARTESIAN_POINT('Ctrl Pts',(-37.9416386654128,38.0058250350956,2.));
#63591=CARTESIAN_POINT('Ctrl Pts',(-37.9304525998634,38.0179661552202,2.));
#63592=CARTESIAN_POINT('Ctrl Pts',(-37.9194765003128,38.0303250151245,2.));
#63593=CARTESIAN_POINT('Ctrl Pts',(-37.9087126348758,38.0428943202534,2.));
#63594=CARTESIAN_POINT('Ctrl Pts',(-37.8987608212141,38.0545153669148,2.));
#63595=CARTESIAN_POINT('Ctrl Pts',(-37.8889863441815,38.0663216997937,2.));
#63596=CARTESIAN_POINT('Ctrl Pts',(-37.8794138053098,38.0782786674143,2.));
#63597=CARTESIAN_POINT('Ctrl Pts',(-37.8439500327557,38.1225761297512,2.));
#63598=CARTESIAN_POINT('Ctrl Pts',(-37.8112056943211,38.1689911399369,2.));
#63599=CARTESIAN_POINT('Ctrl Pts',(-37.7812215917862,38.2171732588852,2.));
#63600=CARTESIAN_POINT('Ctrl Pts',(-37.7505286361066,38.266494449663,2.));
#63601=CARTESIAN_POINT('Ctrl Pts',(-37.7227273546167,38.3176680405683,2.));
#63602=CARTESIAN_POINT('Ctrl Pts',(-37.6978940563331,38.3703632510113,2.));
#63603=CARTESIAN_POINT('Ctrl Pts',(-37.682817233351,38.4023556328038,2.));
#63604=CARTESIAN_POINT('Ctrl Pts',(-37.6688350669181,38.4349097034549,2.));
#63605=CARTESIAN_POINT('Ctrl Pts',(-37.6559717665588,38.4679573676163,2.));
#63606=CARTESIAN_POINT('Ctrl Pts',(-37.648889306812,38.4861532228486,2.));
#63607=CARTESIAN_POINT('Ctrl Pts',(-37.6421461366873,38.5044987807188,2.));
#63608=CARTESIAN_POINT('Ctrl Pts',(-37.635747084783,38.5229830878431,2.));
#63609=CARTESIAN_POINT('Ctrl Pts',(-37.6318939139123,38.534113360709,2.));
#63610=CARTESIAN_POINT('Ctrl Pts',(-37.6281649122512,38.5452958653453,2.));
#63611=CARTESIAN_POINT('Ctrl Pts',(-37.624563189319,38.5565221415394,2.));
#63612=CARTESIAN_POINT('Ctrl Pts',(-37.6061053671342,38.614053665672,2.));
#63613=CARTESIAN_POINT('Ctrl Pts',(-37.5910431547281,38.6725526585093,2.));
#63614=CARTESIAN_POINT('Ctrl Pts',(-37.5794635885507,38.7316684529271,2.));
#63615=CARTESIAN_POINT('Ctrl Pts',(-37.5719346379239,38.770105117187,2.));
#63616=CARTESIAN_POINT('Ctrl Pts',(-37.5658787738505,38.8088033108087,2.));
#63617=CARTESIAN_POINT('Ctrl Pts',(-37.5613302232318,38.8476724431706,2.));
#63618=CARTESIAN_POINT('Ctrl Pts',(-37.5594503644639,38.8637365667554,2.));
#63619=CARTESIAN_POINT('Ctrl Pts',(-37.5578280676537,38.8798299273607,2.));
#63620=CARTESIAN_POINT('Ctrl Pts',(-37.5564662009659,38.8959462647572,2.));
#63621=CARTESIAN_POINT('Ctrl Pts',(-37.5554691679745,38.9077451583122,2.));
#63622=CARTESIAN_POINT('Ctrl Pts',(-37.5546119020158,38.9195552384719,2.));
#63623=CARTESIAN_POINT('Ctrl Pts',(-37.5538959122054,38.931364001732,2.));
#63624=CARTESIAN_POINT('Ctrl Pts',(-37.5502149156534,38.9920743864587,2.));
#63625=CARTESIAN_POINT('Ctrl Pts',(-37.5502577736835,39.0528196704491,2.));
#63626=CARTESIAN_POINT('Ctrl Pts',(-37.5541374325481,39.1132620113921,2.));
#63627=CARTESIAN_POINT('Ctrl Pts',(-37.5559545726121,39.1415717682862,2.));
#63628=CARTESIAN_POINT('Ctrl Pts',(-37.5586141014162,39.1698153256755,2.));
#63629=CARTESIAN_POINT('Ctrl Pts',(-37.5621314917739,39.1979588342647,2.));
#63630=CARTESIAN_POINT('Ctrl Pts',(-37.5651536457416,39.2221398342386,2.));
#63631=CARTESIAN_POINT('Ctrl Pts',(-37.5688091345127,39.2462469913775,2.));
#63632=CARTESIAN_POINT('Ctrl Pts',(-37.5730824075077,39.2702648660737,2.));
#63633=CARTESIAN_POINT('Ctrl Pts',(-39.696945388151,39.9649932150637,2.80658032638059));
#63634=CARTESIAN_POINT('Ctrl Pts',(-39.5986128055021,40.0228689487565,2.79940525217633));
#63635=CARTESIAN_POINT('Ctrl Pts',(-39.4929004903071,40.0674950246048,2.79223017797206));
#63636=CARTESIAN_POINT('Ctrl Pts',(-39.3829982676155,40.0959214023961,2.7850551037678));
#63637=CARTESIAN_POINT('Ctrl Pts',(-38.9821694242093,40.1995963950695,2.75888660030887));
#63638=CARTESIAN_POINT('Ctrl Pts',(-38.5256079666315,40.0877889404002,2.73271809684995));
#63639=CARTESIAN_POINT('Ctrl Pts',(-38.2180364476029,39.8106370334519,2.70654959339102));
#63640=CARTESIAN_POINT('Ctrl Pts',(-37.9104649285743,39.5334851265035,2.68038108993209));
#63641=CARTESIAN_POINT('Ctrl Pts',(-37.751883348095,39.0909887672762,2.65421258647317));
#63642=CARTESIAN_POINT('Ctrl Pts',(-37.8134117192226,38.6815641398491,2.62804408301424));
#63643=CARTESIAN_POINT('Ctrl Pts',(-37.8749400903503,38.2721395124221,2.60187557955531));
#63644=CARTESIAN_POINT('Ctrl Pts',(-38.1565784130849,37.8957866167954,2.57570707609639));
#63645=CARTESIAN_POINT('Ctrl Pts',(-38.5320162526521,37.7212755253001,2.54953857263746));
#63646=CARTESIAN_POINT('Ctrl Pts',(-38.9074540922193,37.5467644338048,2.52337006917854));
#63647=CARTESIAN_POINT('Ctrl Pts',(-39.3766914486191,37.5740951464407,2.49720156571961));
#63648=CARTESIAN_POINT('Ctrl Pts',(-39.729357979422,37.7909941772624,2.47103306226068));
#63649=CARTESIAN_POINT('Ctrl Pts',(-40.0820245102249,38.0078932080842,2.44486455880175));
#63650=CARTESIAN_POINT('Ctrl Pts',(-40.3181202154309,38.4143605570917,2.41869605534283));
#63651=CARTESIAN_POINT('Ctrl Pts',(-40.3316937547573,38.8281678760191,2.3925275518839));
#63652=CARTESIAN_POINT('Ctrl Pts',(-40.3452672940836,39.2419751949465,2.36635904842498));
#63653=CARTESIAN_POINT('Ctrl Pts',(-40.1363186675303,39.6631224837939,2.34019054496605));
#63654=CARTESIAN_POINT('Ctrl Pts',(-39.7987107859694,39.9026887516753,2.31402204150712));
#63655=CARTESIAN_POINT('Ctrl Pts',(-39.7667081702678,39.9253977807734,2.31154146979828));
#63656=CARTESIAN_POINT('Ctrl Pts',(-39.7335494773786,39.9464752002681,2.30906089808943));
#63657=CARTESIAN_POINT('Ctrl Pts',(-39.6994125047665,39.9658989902663,2.30658032638059));
#63658=CARTESIAN_POINT('Ctrl Pts',(-37.9741697098829,39.9602191716056,2.));
#63659=CARTESIAN_POINT('Ctrl Pts',(-38.3327559670707,40.3192117233802,2.02616850345893));
#63660=CARTESIAN_POINT('Ctrl Pts',(-39.4257675096926,40.6500214621298,2.07850551037678));
#63661=CARTESIAN_POINT('Ctrl Pts',(-40.7517604581818,39.5501737910362,2.15701102075356));
#63662=CARTESIAN_POINT('Ctrl Pts',(-40.5621188491035,37.8394675163551,2.23551653113034));
#63663=CARTESIAN_POINT('Ctrl Pts',(-39.0323736383015,37.0530949705804,2.31402204150712));
#63664=CARTESIAN_POINT('Ctrl Pts',(-37.5317729583208,37.8957949010443,2.3925275518839));
#63665=CARTESIAN_POINT('Ctrl Pts',(-37.4074081512687,39.612062461691,2.47103306226068));
#63666=CARTESIAN_POINT('Ctrl Pts',(-38.7701598472246,40.6625848481854,2.54953857263746));
#63667=CARTESIAN_POINT('Ctrl Pts',(-40.3982034912373,40.1052897198445,2.62804408301424));
#63668=CARTESIAN_POINT('Ctrl Pts',(-40.8313104277201,38.439942299895,2.70654959339101));
#63669=CARTESIAN_POINT('Ctrl Pts',(-39.6811395860238,37.1600807661057,2.78505510376779));
#63670=CARTESIAN_POINT('Ctrl Pts',(-37.9791520940816,37.4135079224236,2.86356061414458));
#63671=CARTESIAN_POINT('Ctrl Pts',(-37.2517503435483,38.9729479619195,2.94206612452135));
#63672=CARTESIAN_POINT('Ctrl Pts',(-38.1512758267995,40.4398561533634,3.02057163489813));
#63673=CARTESIAN_POINT('Ctrl Pts',(-39.8710175096897,40.4986752642982,3.09907714527491));
#63674=CARTESIAN_POINT('Ctrl Pts',(-40.8686677847051,39.096654467846,3.17758265565169));
#63675=CARTESIAN_POINT('Ctrl Pts',(-40.249511348243,37.4911595684212,3.25608816602847));
#63676=CARTESIAN_POINT('Ctrl Pts',(-38.5688218267178,37.1220364497186,3.33459367640525));
#63677=CARTESIAN_POINT('Ctrl Pts',(-37.333881829365,38.3203235548052,3.41309918678203));
#63678=CARTESIAN_POINT('Ctrl Pts',(-37.6522147609439,40.011368493019,3.49160469715881));
#63679=CARTESIAN_POINT('Ctrl Pts',(-39.2383321518161,40.67860197495,3.57011020753559));
#63680=CARTESIAN_POINT('Ctrl Pts',(-40.6697661826987,39.7236331447561,3.64861571791237));
#63681=CARTESIAN_POINT('Ctrl Pts',(-40.662772801836,38.0029007557487,3.72712122828915));
#63682=CARTESIAN_POINT('Ctrl Pts',(-39.2236238307452,37.0595985208235,3.80562673866593));
#63683=CARTESIAN_POINT('Ctrl Pts',(-37.642982284831,37.7397023107928,3.88413224904271));
#63684=CARTESIAN_POINT('Ctrl Pts',(-37.3384050779085,39.4332788778856,3.96263775941949));
#63685=CARTESIAN_POINT('Ctrl Pts',(-38.5830442911661,40.6214884944165,4.04114326979627));
#63686=CARTESIAN_POINT('Ctrl Pts',(-40.26067788792,40.2387165281925,4.11964878017304));
#63687=CARTESIAN_POINT('Ctrl Pts',(-40.8667641756192,38.6282419782981,4.19815429054983));
#63688=CARTESIAN_POINT('Ctrl Pts',(-39.8577505620191,37.2343767082119,4.2766598009266));
#63689=CARTESIAN_POINT('Ctrl Pts',(-38.1385444446535,37.3071722287696,4.35516531130339));
#63690=CARTESIAN_POINT('Ctrl Pts',(-37.2509707395799,38.781343787805,4.43367082168017));
#63691=CARTESIAN_POINT('Ctrl Pts',(-37.9910266499109,40.3348192821528,4.51217633205694));
#63692=CARTESIAN_POINT('Ctrl Pts',(-39.6950124343118,40.5744049619641,4.59068184243373));
#63693=CARTESIAN_POINT('Ctrl Pts',(-40.8347531457538,39.2852346831729,4.6691873528105));
#63694=CARTESIAN_POINT('Ctrl Pts',(-40.3881021894619,37.6234670214254,4.74769286318728));
#63695=CARTESIAN_POINT('Ctrl Pts',(-38.7556268199881,37.0794146789619,4.82619837356406));
#63696=CARTESIAN_POINT('Ctrl Pts',(-37.4013696406987,38.1409968175026,4.90470388394084));
#63697=CARTESIAN_POINT('Ctrl Pts',(-37.5398609233301,39.8561611622598,4.98320939431762));
#63698=CARTESIAN_POINT('Ctrl Pts',(-39.0468979136614,40.6867079066975,5.0617149046944));
#63699=CARTESIAN_POINT('Ctrl Pts',(-40.570934978228,39.8877822721678,5.14022041507118));
#63700=CARTESIAN_POINT('Ctrl Pts',(-40.7451774946681,38.1758811994982,5.21872592544796));
#63701=CARTESIAN_POINT('Ctrl Pts',(-39.4133645670745,37.0862753673933,5.29723143582474));
#63702=CARTESIAN_POINT('Ctrl Pts',(-37.7698897533292,37.5961550422892,5.37573694620152));
#63703=CARTESIAN_POINT('Ctrl Pts',(-37.2886763485593,39.2482362054987,5.4542424565783));
#63704=CARTESIAN_POINT('Ctrl Pts',(-38.4012556794041,40.5609170045275,5.53274796695508));
#63705=CARTESIAN_POINT('Ctrl Pts',(-40.1099052932564,40.3569060637301,5.61125347733186));
#63706=CARTESIAN_POINT('Ctrl Pts',(-40.8821362004287,38.8192621207561,5.68975898770863));
#63707=CARTESIAN_POINT('Ctrl Pts',(-40.0256584008921,37.3267854127763,5.76826449808542));
#63708=CARTESIAN_POINT('Ctrl Pts',(-38.3080469142999,37.2183586878016,5.84677000846219));
#63709=CARTESIAN_POINT('Ctrl Pts',(-37.2707754210207,38.5904264849421,5.92527551883898));
#63710=CARTESIAN_POINT('Ctrl Pts',(-37.8419099014004,40.2140906446281,6.00378102921575));
#63711=CARTESIAN_POINT('Ctrl Pts',(-39.513729769878,40.6299518311032,6.08228653959253));
#63712=CARTESIAN_POINT('Ctrl Pts',(-40.3550860167095,39.8577931806473,6.13462354651039));
#63713=CARTESIAN_POINT('Ctrl Pts',(-40.5224743779889,39.3787932927749,6.16079204996931));
#63714=CARTESIAN_POINT('Ctrl Pts',(-38.0398499461207,39.8946132698472,1.94640265001023));
#63715=CARTESIAN_POINT('Ctrl Pts',(-38.3768621543504,40.2320073282822,1.97257115346916));
#63716=CARTESIAN_POINT('Ctrl Pts',(-39.4041135512345,40.5429141695936,2.02490816038701));
#63717=CARTESIAN_POINT('Ctrl Pts',(-40.6503292182041,39.5092379343174,2.10341367076379));
#63718=CARTESIAN_POINT('Ctrl Pts',(-40.4720972414715,37.9014549038573,2.18191918114057));
#63719=CARTESIAN_POINT('Ctrl Pts',(-39.0343879004488,37.162393819305,2.26042469151735));
#63720=CARTESIAN_POINT('Ctrl Pts',(-37.6240696333812,37.954393397504,2.33893020189413));
#63721=CARTESIAN_POINT('Ctrl Pts',(-37.5071871332559,39.5674031237069,2.41743571227091));
#63722=CARTESIAN_POINT('Ctrl Pts',(-38.7879499877075,40.5547216897998,2.49594122264769));
#63723=CARTESIAN_POINT('Ctrl Pts',(-40.3180437170825,40.0309557671714,2.57444673302447));
#63724=CARTESIAN_POINT('Ctrl Pts',(-40.7250931288709,38.4658026130364,2.65295224340124));
#63725=CARTESIAN_POINT('Ctrl Pts',(-39.6441213754037,37.2629429019217,2.73145775377803));
#63726=CARTESIAN_POINT('Ctrl Pts',(-38.044532569248,37.5011228205998,2.8099632641548));
#63727=CARTESIAN_POINT('Ctrl Pts',(-37.3608943502601,38.9667404252287,2.88846877453158));
#63728=CARTESIAN_POINT('Ctrl Pts',(-38.2063006183275,40.345393284783,2.96697428490836));
#63729=CARTESIAN_POINT('Ctrl Pts',(-39.8225754490499,40.400673592003,3.04547979528514));
#63730=CARTESIAN_POINT('Ctrl Pts',(-40.7602029110189,39.0830042303774,3.12398530566192));
#63731=CARTESIAN_POINT('Ctrl Pts',(-40.1782975152901,37.5741026188095,3.2024908160387));
#63732=CARTESIAN_POINT('Ctrl Pts',(-38.5987253045761,37.2271874907222,3.28099632641548));
#63733=CARTESIAN_POINT('Ctrl Pts',(-37.4380844623892,38.3533806319362,3.35950183679226));
#63734=CARTESIAN_POINT('Ctrl Pts',(-37.7372651534313,39.9426852341611,3.43800734716904));
#63735=CARTESIAN_POINT('Ctrl Pts',(-39.2279550884041,40.5697751592293,3.51651285754582));
#63736=CARTESIAN_POINT('Ctrl Pts',(-40.5732680612612,39.6722612478535,3.5950183679226));
#63737=CARTESIAN_POINT('Ctrl Pts',(-40.5666954314398,38.0550553160375,3.67352387829938));
#63738=CARTESIAN_POINT('Ctrl Pts',(-39.214131681444,37.1685060887655,3.75202938867616));
#63739=CARTESIAN_POINT('Ctrl Pts',(-37.7285881416946,37.8076919903125,3.83053489905294));
#63740=CARTESIAN_POINT('Ctrl Pts',(-37.4423355733826,39.399375908035,3.90904040942972));
#63741=CARTESIAN_POINT('Ctrl Pts',(-38.6120920860802,40.516097864552,3.9875459198065));
#63742=CARTESIAN_POINT('Ctrl Pts',(-40.1887922292381,40.1563550606944,4.06605143018328));
#63743=CARTESIAN_POINT('Ctrl Pts',(-40.7584138310171,38.6427733952556,4.14455694056006));
#63744=CARTESIAN_POINT('Ctrl Pts',(-39.8101066964379,37.3327688894207,4.22306245093684));
#63745=CARTESIAN_POINT('Ctrl Pts',(-38.1943352093783,37.4011847270069,4.30156796131362));
#63746=CARTESIAN_POINT('Ctrl Pts',(-37.360161650527,38.7866639595805,4.3800734716904));
#63747=CARTESIAN_POINT('Ctrl Pts',(-38.0556927021353,40.246675871043,4.45857898206717));
#63748=CARTESIAN_POINT('Ctrl Pts',(-39.6571595751178,40.4718470743308,4.53708449244396));
#63749=CARTESIAN_POINT('Ctrl Pts',(-40.7283287185891,39.2602386712457,4.61559000282073));
#63750=CARTESIAN_POINT('Ctrl Pts',(-40.3085501518689,37.6984499020877,4.69409551319751));
#63751=CARTESIAN_POINT('Ctrl Pts',(-38.7742913281713,37.1871300239525,4.77260102357429));
#63752=CARTESIAN_POINT('Ctrl Pts',(-37.5015119247369,38.1848429411531,4.85110653395107));
#63753=CARTESIAN_POINT('Ctrl Pts',(-37.631670992589,39.7968158255485,4.92961204432785));
#63754=CARTESIAN_POINT('Ctrl Pts',(-39.0480383346578,40.5773934042212,5.00811755470463));
#63755=CARTESIAN_POINT('Ctrl Pts',(-40.4803829553959,39.8265344772346,5.08662306508141));
#63756=CARTESIAN_POINT('Ctrl Pts',(-40.6441423133075,38.2176285328298,5.16512857545819));
#63757=CARTESIAN_POINT('Ctrl Pts',(-39.3924568215175,37.1935779446743,5.24363408583497));
#63758=CARTESIAN_POINT('Ctrl Pts',(-37.8478603261192,37.672781125844,5.32213959621175));
#63759=CARTESIAN_POINT('Ctrl Pts',(-37.3955987323729,39.2254661767282,5.40064510658853));
#63760=CARTESIAN_POINT('Ctrl Pts',(-38.4412406375015,40.4591706088247,5.47915061696531));
#63761=CARTESIAN_POINT('Ctrl Pts',(-40.04709074445,40.2674338194665,5.55765612734208));
#63762=CARTESIAN_POINT('Ctrl Pts',(-40.7728610105232,38.8223009670344,5.63616163771886));
#63763=CARTESIAN_POINT('Ctrl Pts',(-39.9679124974786,37.419617899835,5.71466714809565));
#63764=CARTESIAN_POINT('Ctrl Pts',(-38.3536397015357,37.3177145801109,5.79317265847242));
#63765=CARTESIAN_POINT('Ctrl Pts',(-37.3787747995027,38.6072330401369,5.87167816884921));
#63766=CARTESIAN_POINT('Ctrl Pts',(-37.9155474408704,40.1332107732787,5.95018367922598));
#63767=CARTESIAN_POINT('Ctrl Pts',(-39.4867836339601,40.5240520115073,6.02868918960276));
#63768=CARTESIAN_POINT('Ctrl Pts',(-40.2775203701537,39.7983496548842,6.08102619652062));
#63769=CARTESIAN_POINT('Ctrl Pts',(-40.4348379475454,39.3481684036012,6.10719469997954));
#63770=CARTESIAN_POINT('Ctrl Pts',(-38.1055301823585,39.8290073680889,1.89280530002046));
#63771=CARTESIAN_POINT('Ctrl Pts',(-38.4209683416302,40.1448029331842,1.91897380347939));
#63772=CARTESIAN_POINT('Ctrl Pts',(-39.3824595927765,40.4358068770573,1.97131081039724));
#63773=CARTESIAN_POINT('Ctrl Pts',(-40.5488979782264,39.4683020775987,2.04981632077402));
#63774=CARTESIAN_POINT('Ctrl Pts',(-40.3820756338396,37.9634422913595,2.12832183115079));
#63775=CARTESIAN_POINT('Ctrl Pts',(-39.0364021625962,37.2716926680296,2.20682734152758));
#63776=CARTESIAN_POINT('Ctrl Pts',(-37.7163663084416,38.0129918939637,2.28533285190435));
#63777=CARTESIAN_POINT('Ctrl Pts',(-37.6069661152431,39.5227437857229,2.36383836228114));
#63778=CARTESIAN_POINT('Ctrl Pts',(-38.8057401281902,40.4468585314142,2.44234387265791));
#63779=CARTESIAN_POINT('Ctrl Pts',(-40.2378839429278,39.9566218144982,2.5208493830347));
#63780=CARTESIAN_POINT('Ctrl Pts',(-40.6188758300216,38.4916629261779,2.59935489341147));
#63781=CARTESIAN_POINT('Ctrl Pts',(-39.6071031647836,37.3658050377377,2.67786040378825));
#63782=CARTESIAN_POINT('Ctrl Pts',(-38.1099130444144,37.588737718776,2.75636591416503));
#63783=CARTESIAN_POINT('Ctrl Pts',(-37.4700383569719,38.9605328885379,2.83487142454181));
#63784=CARTESIAN_POINT('Ctrl Pts',(-38.2613254098556,40.2509304162024,2.91337693491859));
#63785=CARTESIAN_POINT('Ctrl Pts',(-39.7741333884101,40.3026719197079,2.99188244529537));
#63786=CARTESIAN_POINT('Ctrl Pts',(-40.6517380373327,39.0693539929087,3.07038795567215));
#63787=CARTESIAN_POINT('Ctrl Pts',(-40.1070836823373,37.6570456691978,3.14889346604893));
#63788=CARTESIAN_POINT('Ctrl Pts',(-38.6286287824344,37.3323385317259,3.22739897642571));
#63789=CARTESIAN_POINT('Ctrl Pts',(-37.5422870954133,38.3864377090672,3.30590448680249));
#63790=CARTESIAN_POINT('Ctrl Pts',(-37.8223155459186,39.8740019753033,3.38440999717927));
#63791=CARTESIAN_POINT('Ctrl Pts',(-39.2175780249923,40.4609483435086,3.46291550755605));
#63792=CARTESIAN_POINT('Ctrl Pts',(-40.4767699398235,39.620889350951,3.54142101793282));
#63793=CARTESIAN_POINT('Ctrl Pts',(-40.4706180610436,38.1072098763262,3.61992652830961));
#63794=CARTESIAN_POINT('Ctrl Pts',(-39.2046395321427,37.2774136567074,3.69843203868638));
#63795=CARTESIAN_POINT('Ctrl Pts',(-37.8141939985582,37.8756816698323,3.77693754906317));
#63796=CARTESIAN_POINT('Ctrl Pts',(-37.5462660688567,39.3654729381844,3.85544305943995));
#63797=CARTESIAN_POINT('Ctrl Pts',(-38.6411398809943,40.4107072346876,3.93394856981673));
#63798=CARTESIAN_POINT('Ctrl Pts',(-40.1169065705561,40.0739935931962,4.01245408019351));
#63799=CARTESIAN_POINT('Ctrl Pts',(-40.6500634864151,38.6573048122132,4.09095959057029));
#63800=CARTESIAN_POINT('Ctrl Pts',(-39.7624628308567,37.4311610706295,4.16946510094706));
#63801=CARTESIAN_POINT('Ctrl Pts',(-38.2501259741031,37.4951972252442,4.24797061132385));
#63802=CARTESIAN_POINT('Ctrl Pts',(-37.4693525614741,38.7919841313561,4.32647612170062));
#63803=CARTESIAN_POINT('Ctrl Pts',(-38.1203587543597,40.1585324599333,4.40498163207741));
#63804=CARTESIAN_POINT('Ctrl Pts',(-39.6193067159239,40.3692891866976,4.48348714245418));
#63805=CARTESIAN_POINT('Ctrl Pts',(-40.6219042914244,39.2352426593185,4.56199265283096));
#63806=CARTESIAN_POINT('Ctrl Pts',(-40.2289981142758,37.77343278275,4.64049816320774));
#63807=CARTESIAN_POINT('Ctrl Pts',(-38.7929558363546,37.2948453689432,4.71900367358452));
#63808=CARTESIAN_POINT('Ctrl Pts',(-37.601654208775,38.2286890648036,4.7975091839613));
#63809=CARTESIAN_POINT('Ctrl Pts',(-37.7234810618479,39.7374704888372,4.87601469433808));
#63810=CARTESIAN_POINT('Ctrl Pts',(-39.0491787556542,40.468078901745,4.95452020471485));
#63811=CARTESIAN_POINT('Ctrl Pts',(-40.3898309325639,39.7652866823013,5.03302571509164));
#63812=CARTESIAN_POINT('Ctrl Pts',(-40.543107131947,38.2593758661615,5.11153122546841));
#63813=CARTESIAN_POINT('Ctrl Pts',(-39.3715490759605,37.3008805219553,5.1900367358452));
#63814=CARTESIAN_POINT('Ctrl Pts',(-37.9258308989092,37.7494072093988,5.26854224622198));
#63815=CARTESIAN_POINT('Ctrl Pts',(-37.5025211161865,39.2026961479577,5.34704775659876));
#63816=CARTESIAN_POINT('Ctrl Pts',(-38.4812255955989,40.3574242131219,5.42555326697554));
#63817=CARTESIAN_POINT('Ctrl Pts',(-39.9842761956436,40.1779615752029,5.50405877735232));
#63818=CARTESIAN_POINT('Ctrl Pts',(-40.6635858206177,38.8253398133127,5.58256428772909));
#63819=CARTESIAN_POINT('Ctrl Pts',(-39.910166594065,37.5124503868936,5.66106979810588));
#63820=CARTESIAN_POINT('Ctrl Pts',(-38.3992324887715,37.4170704724202,5.73957530848266));
#63821=CARTESIAN_POINT('Ctrl Pts',(-37.4867741779846,38.6240395953316,5.81808081885943));
#63822=CARTESIAN_POINT('Ctrl Pts',(-37.9891849803405,40.0523309019294,5.89658632923621));
#63823=CARTESIAN_POINT('Ctrl Pts',(-39.4598374980422,40.4181521919114,5.97509183961299));
#63824=CARTESIAN_POINT('Ctrl Pts',(-40.199954723598,39.738906129121,6.02742884653085));
#63825=CARTESIAN_POINT('Ctrl Pts',(-40.347201517102,39.3175435144275,6.05359734998977));
#63826=CARTESIAN_POINT('Ctrl Pts',(-38.1712104185962,39.7634014663305,1.83920795003069));
#63827=CARTESIAN_POINT('Ctrl Pts',(-38.4650745289099,40.0575985380862,1.86537645348962));
#63828=CARTESIAN_POINT('Ctrl Pts',(-39.3608056343184,40.328699584521,1.91771346040747));
#63829=CARTESIAN_POINT('Ctrl Pts',(-40.4474667382488,39.4273662208801,1.99621897078425));
#63830=CARTESIAN_POINT('Ctrl Pts',(-40.2920540262076,38.0254296788617,2.07472448116103));
#63831=CARTESIAN_POINT('Ctrl Pts',(-39.0384164247435,37.3809915167541,2.15322999153781));
#63832=CARTESIAN_POINT('Ctrl Pts',(-37.8086629835021,38.0715903904234,2.23173550191459));
#63833=CARTESIAN_POINT('Ctrl Pts',(-37.7067450972302,39.4780844477388,2.31024101229137));
#63834=CARTESIAN_POINT('Ctrl Pts',(-38.8235302686731,40.3389953730286,2.38874652266815));
#63835=CARTESIAN_POINT('Ctrl Pts',(-40.157724168773,39.882287861825,2.46725203304493));
#63836=CARTESIAN_POINT('Ctrl Pts',(-40.5126585311724,38.5175232393194,2.5457575434217));
#63837=CARTESIAN_POINT('Ctrl Pts',(-39.5700849541634,37.4686671735537,2.62426305379849));
#63838=CARTESIAN_POINT('Ctrl Pts',(-38.1752935195808,37.6763526169522,2.70276856417526));
#63839=CARTESIAN_POINT('Ctrl Pts',(-37.5791823636837,38.9543253518471,2.78127407455204));
#63840=CARTESIAN_POINT('Ctrl Pts',(-38.3163502013836,40.156467547622,2.85977958492882));
#63841=CARTESIAN_POINT('Ctrl Pts',(-39.7256913277703,40.2046702474127,2.9382850953056));
#63842=CARTESIAN_POINT('Ctrl Pts',(-40.5432731636466,39.05570375544,3.01679060568238));
#63843=CARTESIAN_POINT('Ctrl Pts',(-40.0358698493845,37.7399887195861,3.09529611605916));
#63844=CARTESIAN_POINT('Ctrl Pts',(-38.6585322602927,37.4374895727296,3.17380162643594));
#63845=CARTESIAN_POINT('Ctrl Pts',(-37.6464897284375,38.4194947861982,3.25230713681272));
#63846=CARTESIAN_POINT('Ctrl Pts',(-37.9073659384061,39.8053187164454,3.3308126471895));
#63847=CARTESIAN_POINT('Ctrl Pts',(-39.2072009615803,40.352121527788,3.40931815756628));
#63848=CARTESIAN_POINT('Ctrl Pts',(-40.380271818386,39.5695174540484,3.48782366794306));
#63849=CARTESIAN_POINT('Ctrl Pts',(-40.3745406906472,38.159364436615,3.56632917831983));
#63850=CARTESIAN_POINT('Ctrl Pts',(-39.1951473828414,37.3863212246494,3.64483468869662));
#63851=CARTESIAN_POINT('Ctrl Pts',(-37.8997998554218,37.943671349352,3.7233401990734));
#63852=CARTESIAN_POINT('Ctrl Pts',(-37.6501965643308,39.3315699683338,3.80184570945018));
#63853=CARTESIAN_POINT('Ctrl Pts',(-38.6701876759084,40.3053166048232,3.88035121982695));
#63854=CARTESIAN_POINT('Ctrl Pts',(-40.0450209118742,39.9916321256981,3.95885673020374));
#63855=CARTESIAN_POINT('Ctrl Pts',(-40.541713141813,38.6718362291708,4.03736224058052));
#63856=CARTESIAN_POINT('Ctrl Pts',(-39.7148189652756,37.5295532518384,4.11586775095729));
#63857=CARTESIAN_POINT('Ctrl Pts',(-38.3059167388278,37.5892097234815,4.19437326133407));
#63858=CARTESIAN_POINT('Ctrl Pts',(-37.5785434724212,38.7973043031316,4.27287877171086));
#63859=CARTESIAN_POINT('Ctrl Pts',(-38.1850248065841,40.0703890488236,4.35138428208763));
#63860=CARTESIAN_POINT('Ctrl Pts',(-39.5814538567299,40.2667312990643,4.42988979246442));
#63861=CARTESIAN_POINT('Ctrl Pts',(-40.5154798642597,39.2102466473913,4.50839530284119));
#63862=CARTESIAN_POINT('Ctrl Pts',(-40.1494460766828,37.8484156634123,4.58690081321797));
#63863=CARTESIAN_POINT('Ctrl Pts',(-38.8116203445379,37.4025607139339,4.66540632359475));
#63864=CARTESIAN_POINT('Ctrl Pts',(-37.701796492813,38.2725351884541,4.74391183397153));
#63865=CARTESIAN_POINT('Ctrl Pts',(-37.8152911311069,39.6781251521259,4.82241734434831));
#63866=CARTESIAN_POINT('Ctrl Pts',(-39.0503191766506,40.3587643992687,4.90092285472509));
#63867=CARTESIAN_POINT('Ctrl Pts',(-40.2992789097319,39.7040388873681,4.97942836510187));
#63868=CARTESIAN_POINT('Ctrl Pts',(-40.4420719505864,38.3011231994932,5.05793387547865));
#63869=CARTESIAN_POINT('Ctrl Pts',(-39.3506413304036,37.4081830992363,5.13643938585543));
#63870=CARTESIAN_POINT('Ctrl Pts',(-38.0038014716992,37.8260332929536,5.21494489623221));
#63871=CARTESIAN_POINT('Ctrl Pts',(-37.6094435000001,39.1799261191872,5.29345040660899));
#63872=CARTESIAN_POINT('Ctrl Pts',(-38.5212105536964,40.2556778174191,5.37195591698577));
#63873=CARTESIAN_POINT('Ctrl Pts',(-39.9214616468371,40.0884893309394,5.45046142736255));
#63874=CARTESIAN_POINT('Ctrl Pts',(-40.5543106307123,38.8283786595909,5.52896693773932));
#63875=CARTESIAN_POINT('Ctrl Pts',(-39.8524206906514,37.6052828739522,5.60747244811611));
#63876=CARTESIAN_POINT('Ctrl Pts',(-38.4448252760073,37.5164263647296,5.68597795849288));
#63877=CARTESIAN_POINT('Ctrl Pts',(-37.5947735564665,38.6408461505263,5.76448346886966));
#63878=CARTESIAN_POINT('Ctrl Pts',(-38.0628225198106,39.97145103058,5.84298897924644));
#63879=CARTESIAN_POINT('Ctrl Pts',(-39.4328913621243,40.3122523723154,5.92149448962322));
#63880=CARTESIAN_POINT('Ctrl Pts',(-40.1223890770422,39.6794626033579,5.97383149654108));
#63881=CARTESIAN_POINT('Ctrl Pts',(-40.2595650866585,39.2869186252538,6.));
#63882=CARTESIAN_POINT('Ctrl Pts',(-39.6985816414592,39.9636701304732,2.44341967361941));
#63883=CARTESIAN_POINT('Ctrl Pts',(-39.808547063221,39.9013157119467,2.45136379342791));
#63884=CARTESIAN_POINT('Ctrl Pts',(-39.9090512176557,39.823104100358,2.45930791323641));
#63885=CARTESIAN_POINT('Ctrl Pts',(-39.9945142458229,39.7309450099414,2.46725203304492));
#63886=CARTESIAN_POINT('Ctrl Pts',(-40.2760356229061,39.4273663209898,2.49342053650384));
#63887=CARTESIAN_POINT('Ctrl Pts',(-40.3943470770393,38.9724447801546,2.51958903996277));
#63888=CARTESIAN_POINT('Ctrl Pts',(-40.2964072079377,38.5701746654427,2.5457575434217));
#63889=CARTESIAN_POINT('Ctrl Pts',(-40.1984673388361,38.1679045507309,2.57192604688062));
#63890=CARTESIAN_POINT('Ctrl Pts',(-39.8842761464997,37.8182858621423,2.59809455033955));
#63891=CARTESIAN_POINT('Ctrl Pts',(-39.4947153112345,37.6780907584144,2.62426305379848));
#63892=CARTESIAN_POINT('Ctrl Pts',(-39.1051544759692,37.5378956546866,2.65043155725741));
#63893=CARTESIAN_POINT('Ctrl Pts',(-38.640223997775,37.6071241358194,2.67660006071633));
#63894=CARTESIAN_POINT('Ctrl Pts',(-38.3084068993617,37.8547338322016,2.70276856417526));
#63895=CARTESIAN_POINT('Ctrl Pts',(-37.9765898009484,38.1023435285838,2.72893706763418));
#63896=CARTESIAN_POINT('Ctrl Pts',(-37.7778860823161,38.5283344402155,2.75510557109311));
#63897=CARTESIAN_POINT('Ctrl Pts',(-37.8013955292832,38.9416869286604,2.78127407455204));
#63898=CARTESIAN_POINT('Ctrl Pts',(-37.8249049762503,39.3550394171054,2.80744257801096));
#63899=CARTESIAN_POINT('Ctrl Pts',(-38.070627588817,39.7557534823636,2.83361108146989));
#63900=CARTESIAN_POINT('Ctrl Pts',(-38.4283790828314,39.9641442982913,2.85977958492881));
#63901=CARTESIAN_POINT('Ctrl Pts',(-38.7861305768459,40.1725351142189,2.88594808838774));
#63902=CARTESIAN_POINT('Ctrl Pts',(-39.2559109523081,40.1886026808158,2.91211659184667));
#63903=CARTESIAN_POINT('Ctrl Pts',(-39.6270647793519,40.0051420487854,2.93828509530559));
#63904=CARTESIAN_POINT('Ctrl Pts',(-39.6513397427562,39.9931429804635,2.9399966214102));
#63905=CARTESIAN_POINT('Ctrl Pts',(-39.6751928123865,39.9802903924142,2.9417081475148));
#63906=CARTESIAN_POINT('Ctrl Pts',(-39.6985897981371,39.9666323328488,2.94341967361941));
#63907=CARTESIAN_POINT('Ctrl Pts',(-37.9741697098829,39.9602191716056,2.));
#63908=CARTESIAN_POINT('Ctrl Pts',(-38.0210640733087,39.9994677669677,2.));
#63909=CARTESIAN_POINT('Ctrl Pts',(-38.0703056805302,40.0355567831455,2.));
#63910=CARTESIAN_POINT('Ctrl Pts',(-38.1215357900136,40.0684647235096,2.));
#63911=CARTESIAN_POINT('Ctrl Pts',(-38.1724676227795,40.1011810641967,2.));
#63912=CARTESIAN_POINT('Ctrl Pts',(-38.2253661047038,40.1307533458135,2.));
#63913=CARTESIAN_POINT('Ctrl Pts',(-38.2799014945792,40.1571104299641,2.));
#63914=CARTESIAN_POINT('Ctrl Pts',(-38.3210824949725,40.1770133057894,2.));
#63915=CARTESIAN_POINT('Ctrl Pts',(-38.3631974573963,40.1950818318592,2.));
#63916=CARTESIAN_POINT('Ctrl Pts',(-38.4061067602759,40.2112658265376,2.));
#63917=CARTESIAN_POINT('Ctrl Pts',(-38.4283821944242,40.2196673964425,2.));
#63918=CARTESIAN_POINT('Ctrl Pts',(-38.450871698748,40.2275608160985,2.));
#63919=CARTESIAN_POINT('Ctrl Pts',(-38.4735555240439,40.2349372243507,2.));
#63920=CARTESIAN_POINT('Ctrl Pts',(-38.4855017473361,40.2388219403951,2.));
#63921=CARTESIAN_POINT('Ctrl Pts',(-38.4975038315009,40.2425636902965,2.));
#63922=CARTESIAN_POINT('Ctrl Pts',(-38.5095371704194,40.2461549840613,2.));
#63923=CARTESIAN_POINT('Ctrl Pts',(-38.5662684087183,40.2630861570093,2.));
#63924=CARTESIAN_POINT('Ctrl Pts',(-38.6237986216546,40.276712917215,2.));
#63925=CARTESIAN_POINT('Ctrl Pts',(-38.6818163301137,40.2869751451508,2.));
#63926=CARTESIAN_POINT('Ctrl Pts',(-38.7386491569881,40.2970277900951,2.));
#63927=CARTESIAN_POINT('Ctrl Pts',(-38.795950805549,40.3038518408609,2.));
#63928=CARTESIAN_POINT('Ctrl Pts',(-38.8534268715751,40.3073420065163,2.));
#63929=CARTESIAN_POINT('Ctrl Pts',(-38.8950337651222,40.3098685355732,2.));
#63930=CARTESIAN_POINT('Ctrl Pts',(-38.9367320688478,40.3106470090916,2.));
#63931=CARTESIAN_POINT('Ctrl Pts',(-38.9784050690481,40.3096213125545,2.));
#63932=CARTESIAN_POINT('Ctrl Pts',(-39.0001855019627,40.3090852312907,2.));
#63933=CARTESIAN_POINT('Ctrl Pts',(-39.021958929381,40.3080560888435,2.));
#63934=CARTESIAN_POINT('Ctrl Pts',(-39.0437079205564,40.3065243689262,2.));
#63935=CARTESIAN_POINT('Ctrl Pts',(-39.0538226985227,40.3058120137303,2.));
#63936=CARTESIAN_POINT('Ctrl Pts',(-39.0639271474701,40.304991238704,2.));
#63937=CARTESIAN_POINT('Ctrl Pts',(-39.0740116259078,40.3040622330021,2.));
#63938=CARTESIAN_POINT('Ctrl Pts',(-39.1295483097472,40.2989460640037,2.));
#63939=CARTESIAN_POINT('Ctrl Pts',(-39.1845546342211,40.2905462413972,2.));
#63940=CARTESIAN_POINT('Ctrl Pts',(-39.2387593259822,40.2787734967599,2.));
#63941=CARTESIAN_POINT('Ctrl Pts',(-39.2750276515155,40.2708963606476,2.));
#63942=CARTESIAN_POINT('Ctrl Pts',(-39.310936935959,40.2615081906221,2.));
#63943=CARTESIAN_POINT('Ctrl Pts',(-39.3464011448468,40.2505700228958,2.));
#63944=CARTESIAN_POINT('Ctrl Pts',(-39.3988910752724,40.2343806398264,2.));
#63945=CARTESIAN_POINT('Ctrl Pts',(-39.4504076476632,40.2147967478769,2.));
#63946=CARTESIAN_POINT('Ctrl Pts',(-39.5007091188364,40.1920209197932,2.));
#63947=CARTESIAN_POINT('Ctrl Pts',(-39.5162447293996,40.1849866047501,2.));
#63948=CARTESIAN_POINT('Ctrl Pts',(-39.5316641987849,40.1776475888762,2.));
#63949=CARTESIAN_POINT('Ctrl Pts',(-39.5469597255045,40.1700092883095,2.));
#63950=CARTESIAN_POINT('Ctrl Pts',(-39.5603821271851,40.1633063914271,2.));
#63951=CARTESIAN_POINT('Ctrl Pts',(-39.5737147687466,40.1563697365981,2.));
#63952=CARTESIAN_POINT('Ctrl Pts',(-39.5869207826588,40.1492204403469,2.));
#63953=CARTESIAN_POINT('Ctrl Pts',(-39.635889783268,40.1227102537904,2.));
#63954=CARTESIAN_POINT('Ctrl Pts',(-39.6831882131042,40.0932490202857,2.));
#63955=CARTESIAN_POINT('Ctrl Pts',(-39.7285927500411,40.0610855615979,2.));
#63956=CARTESIAN_POINT('Ctrl Pts',(-39.7739426813613,40.0289607841877,2.));
#63957=CARTESIAN_POINT('Ctrl Pts',(-39.8174040329096,39.9941393127112,2.));
#63958=CARTESIAN_POINT('Ctrl Pts',(-39.8587164117659,39.9568341503958,2.));
#63959=CARTESIAN_POINT('Ctrl Pts',(-39.8851222214993,39.9329896503829,2.));
#63960=CARTESIAN_POINT('Ctrl Pts',(-39.9106492841629,39.9081297964286,2.));
#63961=CARTESIAN_POINT('Ctrl Pts',(-39.9352193294817,39.8823054325709,2.));
#63962=CARTESIAN_POINT('Ctrl Pts',(-39.9478799226003,39.8689985070399,2.));
#63963=CARTESIAN_POINT('Ctrl Pts',(-39.9602862681352,39.855435438132,2.));
#63964=CARTESIAN_POINT('Ctrl Pts',(-39.9724266997145,39.8416229521415,2.));
#63965=CARTESIAN_POINT('Ctrl Pts',(-39.9797490690399,39.8332921013752,2.));
#63966=CARTESIAN_POINT('Ctrl Pts',(-39.9869741812552,39.824870935248,2.));
#63967=CARTESIAN_POINT('Ctrl Pts',(-39.9940910778001,39.8163713684992,2.));
#63968=CARTESIAN_POINT('Ctrl Pts',(-40.0285072441039,39.7752688316156,2.));
#63969=CARTESIAN_POINT('Ctrl Pts',(-40.0604511582545,39.7322729488062,2.));
#63970=CARTESIAN_POINT('Ctrl Pts',(-40.0896714279657,39.6875760500042,2.));
#63971=CARTESIAN_POINT('Ctrl Pts',(-40.1080207191978,39.6595079855614,2.));
#63972=CARTESIAN_POINT('Ctrl Pts',(-40.1252950915649,39.6307687140437,2.));
#63973=CARTESIAN_POINT('Ctrl Pts',(-40.141422040912,39.6014032998966,2.));
#63974=CARTESIAN_POINT('Ctrl Pts',(-40.1473185206672,39.5906664539939,2.));
#63975=CARTESIAN_POINT('Ctrl Pts',(-40.1530626680629,39.5798436443556,2.));
#63976=CARTESIAN_POINT('Ctrl Pts',(-40.1586468583156,39.5689444882778,2.));
#63977=CARTESIAN_POINT('Ctrl Pts',(-40.1820879991975,39.5231923484773,2.));
#63978=CARTESIAN_POINT('Ctrl Pts',(-40.2026786416958,39.4761684519491,2.));
#63979=CARTESIAN_POINT('Ctrl Pts',(-40.2201722454389,39.4280435374464,2.));
#63980=CARTESIAN_POINT('Ctrl Pts',(-40.2299448374156,39.4011591309937,2.));
#63981=CARTESIAN_POINT('Ctrl Pts',(-40.2387500543247,39.3739309307784,2.));
#63982=CARTESIAN_POINT('Ctrl Pts',(-40.2465377789656,39.3463880711444,2.));
#63983=CARTESIAN_POINT('Ctrl Pts',(-40.2520072382767,39.3270442246388,2.));
#63984=CARTESIAN_POINT('Ctrl Pts',(-40.2569746809645,39.3075451531312,2.));
#63985=CARTESIAN_POINT('Ctrl Pts',(-40.2614422049139,39.2879094456029,2.));
#63986=CARTESIAN_POINT('Origin',(-39.0658530619283,38.8697713466882,4.5));
#63987=CARTESIAN_POINT('Origin',(14.1292828945603,53.2669068454841,6.));
#63988=CARTESIAN_POINT('Ctrl Pts',(13.8936870225526,54.5092654229862,6.));
#63989=CARTESIAN_POINT('Ctrl Pts',(13.9423636521365,54.524108905134,6.));
#63990=CARTESIAN_POINT('Ctrl Pts',(13.9918505584143,54.5357341393502,6.));
#63991=CARTESIAN_POINT('Ctrl Pts',(14.041869470803,54.5442851897488,6.));
#63992=CARTESIAN_POINT('Ctrl Pts',(14.0755804158076,54.5500482896634,6.));
#63993=CARTESIAN_POINT('Ctrl Pts',(14.1095337101478,54.5544140915427,6.));
#63994=CARTESIAN_POINT('Ctrl Pts',(14.1436500643726,54.5574153942341,6.));
#63995=CARTESIAN_POINT('Ctrl Pts',(14.159412263785,54.5588020351163,6.));
#63996=CARTESIAN_POINT('Ctrl Pts',(14.1752093214863,54.5598972886015,6.));
#63997=CARTESIAN_POINT('Ctrl Pts',(14.191033635951,54.5607037375757,6.));
#63998=CARTESIAN_POINT('Ctrl Pts',(14.2042983435199,54.5613797422037,6.));
#63999=CARTESIAN_POINT('Ctrl Pts',(14.2175747323894,54.5618523554142,6.));
#64000=CARTESIAN_POINT('Ctrl Pts',(14.230851131071,54.5621236288019,6.));
#64001=CARTESIAN_POINT('Ctrl Pts',(14.2845943079395,54.5632217499119,6.));
#64002=CARTESIAN_POINT('Ctrl Pts',(14.3383718685865,54.5610264739163,6.));
#64003=CARTESIAN_POINT('Ctrl Pts',(14.3918835284631,54.5556664140625,6.));
#64004=CARTESIAN_POINT('Ctrl Pts',(14.4123675638192,54.5536146059928,6.));
#64005=CARTESIAN_POINT('Ctrl Pts',(14.4328128170711,54.5510985259764,6.));
#64006=CARTESIAN_POINT('Ctrl Pts',(14.4532029278659,54.5481234359019,6.));
#64007=CARTESIAN_POINT('Ctrl Pts',(14.4678705661123,54.5459833030991,6.));
#64008=CARTESIAN_POINT('Ctrl Pts',(14.4825096747067,54.5436056261043,6.));
#64009=CARTESIAN_POINT('Ctrl Pts',(14.4971141904897,54.5409920215303,6.));
#64010=CARTESIAN_POINT('Ctrl Pts',(14.5083899393717,54.5389741286202,6.));
#64011=CARTESIAN_POINT('Ctrl Pts',(14.5196453769788,54.5368154091208,6.));
#64012=CARTESIAN_POINT('Ctrl Pts',(14.5308625723425,54.5345199552782,6.));
#64013=CARTESIAN_POINT('Ctrl Pts',(14.5863736833702,54.5231603249085,6.));
#64014=CARTESIAN_POINT('Ctrl Pts',(14.6410375585735,54.5084412328018,6.));
#64015=CARTESIAN_POINT('Ctrl Pts',(14.6945239552559,54.4905089639947,6.));
#64016=CARTESIAN_POINT('Ctrl Pts',(14.7472373376177,54.4728358620309,6.));
#64017=CARTESIAN_POINT('Ctrl Pts',(14.7988082441058,54.4520415392015,6.));
#64018=CARTESIAN_POINT('Ctrl Pts',(14.8489245844431,54.4282130800221,6.));
#64019=CARTESIAN_POINT('Ctrl Pts',(14.8750932855581,54.4157708341977,6.));
#64020=CARTESIAN_POINT('Ctrl Pts',(14.9008653564499,54.402500473298,6.));
#64021=CARTESIAN_POINT('Ctrl Pts',(14.9261951331621,54.3884088627284,6.));
#64022=CARTESIAN_POINT('Ctrl Pts',(14.9397870441658,54.3808473307443,6.));
#64023=CARTESIAN_POINT('Ctrl Pts',(14.9532515800927,54.3730492659916,6.));
#64024=CARTESIAN_POINT('Ctrl Pts',(14.9665814890931,54.3650152874695,6.));
#64025=CARTESIAN_POINT('Ctrl Pts',(14.976060531546,54.3593022384552,6.));
#64026=CARTESIAN_POINT('Ctrl Pts',(14.9854714930861,54.3534698864814,6.));
#64027=CARTESIAN_POINT('Ctrl Pts',(14.9948117120544,54.3475183602377,6.));
#64028=CARTESIAN_POINT('Ctrl Pts',(15.003022232497,54.3422866704823,6.));
#64029=CARTESIAN_POINT('Ctrl Pts',(15.0111697860467,54.3369681734725,6.));
#64030=CARTESIAN_POINT('Ctrl Pts',(15.0192523730691,54.3315638161437,6.));
#64031=CARTESIAN_POINT('Ctrl Pts',(15.0592738168297,54.3048037970687,6.));
#64032=CARTESIAN_POINT('Ctrl Pts',(15.0977061905865,54.2759385109608,6.));
#64033=CARTESIAN_POINT('Ctrl Pts',(15.1343580440251,54.2450336527682,6.));
#64034=CARTESIAN_POINT('Ctrl Pts',(15.1760762697649,54.2098568273262,6.));
#64035=CARTESIAN_POINT('Ctrl Pts',(15.2154892262316,54.1720387363143,6.));
#64036=CARTESIAN_POINT('Ctrl Pts',(15.2525505184408,54.1318952661649,6.));
#64037=CARTESIAN_POINT('Ctrl Pts',(15.2887783562941,54.0926545640536,6.));
#64038=CARTESIAN_POINT('Ctrl Pts',(15.3227594146192,54.0511910496008,6.));
#64039=CARTESIAN_POINT('Ctrl Pts',(15.3544244053206,54.0077622836781,6.));
#64040=CARTESIAN_POINT('Ctrl Pts',(15.3621778074482,53.9971284360551,6.));
#64041=CARTESIAN_POINT('Ctrl Pts',(15.3697922131791,53.9863766152115,6.));
#64042=CARTESIAN_POINT('Ctrl Pts',(15.3772663285767,53.9755103369004,6.));
#64043=CARTESIAN_POINT('Ctrl Pts',(15.3829111783903,53.9673035450815,6.));
#64044=CARTESIAN_POINT('Ctrl Pts',(15.3884748239509,53.959033039286,6.));
#64045=CARTESIAN_POINT('Ctrl Pts',(15.3939506112589,53.9507101506015,6.));
#64046=CARTESIAN_POINT('Ctrl Pts',(15.4256178027551,53.9025778008681,6.));
#64047=CARTESIAN_POINT('Ctrl Pts',(15.4544095036352,53.8526099943005,6.));
#64048=CARTESIAN_POINT('Ctrl Pts',(15.4802788953979,53.8011564089304,6.));
#64049=CARTESIAN_POINT('Ctrl Pts',(15.5067035063861,53.748598506146,6.));
#64050=CARTESIAN_POINT('Ctrl Pts',(15.5300796467746,53.6944895429324,6.));
#64051=CARTESIAN_POINT('Ctrl Pts',(15.5503219670269,53.6391607086969,6.));
#64052=CARTESIAN_POINT('Ctrl Pts',(15.5707432288469,53.5833427690514,6.));
#64053=CARTESIAN_POINT('Ctrl Pts',(15.5879756421407,53.5262822853792,6.));
#64054=CARTESIAN_POINT('Ctrl Pts',(15.6018865037402,53.468291582188,6.));
#64055=CARTESIAN_POINT('Ctrl Pts',(15.6050386064391,53.4551512996301,6.));
#64056=CARTESIAN_POINT('Ctrl Pts',(15.6080206160607,53.4419594370947,6.));
#64057=CARTESIAN_POINT('Ctrl Pts',(15.6108253926933,53.4287461304931,6.));
#64058=CARTESIAN_POINT('Ctrl Pts',(15.6234580838842,53.3692335047938,6.));
#64059=CARTESIAN_POINT('Ctrl Pts',(15.6325248597468,53.3091883988419,6.));
#64060=CARTESIAN_POINT('Ctrl Pts',(15.6379479683223,53.2489633020841,6.));
#64061=CARTESIAN_POINT('Ctrl Pts',(15.643323424427,53.1892673989841,6.));
#64062=CARTESIAN_POINT('Ctrl Pts',(15.6451194085375,53.1293935642736,6.));
#64063=CARTESIAN_POINT('Ctrl Pts',(15.6432152689552,53.0696627699222,6.));
#64064=CARTESIAN_POINT('Ctrl Pts',(15.6418200559671,53.0258964510863,6.));
#64065=CARTESIAN_POINT('Ctrl Pts',(15.6384374018724,52.9822063985706,6.));
#64066=CARTESIAN_POINT('Ctrl Pts',(15.6330021738796,52.9387162761377,6.));
#64067=CARTESIAN_POINT('Ctrl Pts',(15.6299816095937,52.9145471500616,6.));
#64068=CARTESIAN_POINT('Ctrl Pts',(15.626326826898,52.8904397607359,6.));
#64069=CARTESIAN_POINT('Ctrl Pts',(15.6220514315181,52.8664094746825,6.));
#64070=CARTESIAN_POINT('Ctrl Pts',(15.2209662466057,52.1764590205668,6.));
#64071=CARTESIAN_POINT('Ctrl Pts',(15.1741443796226,52.1372711016556,6.));
#64072=CARTESIAN_POINT('Ctrl Pts',(15.1249225029807,52.1011828129762,6.));
#64073=CARTESIAN_POINT('Ctrl Pts',(15.0736468678487,52.0682420900143,6.));
#64074=CARTESIAN_POINT('Ctrl Pts',(15.0261004125926,52.0376970834751,6.));
#64075=CARTESIAN_POINT('Ctrl Pts',(14.9767869967282,52.0098588542107,6.));
#64076=CARTESIAN_POINT('Ctrl Pts',(14.9259704605611,51.9848043154176,6.));
#64077=CARTESIAN_POINT('Ctrl Pts',(14.9137051793975,51.9787570523434,6.));
#64078=CARTESIAN_POINT('Ctrl Pts',(14.901351848406,51.9728720566584,6.));
#64079=CARTESIAN_POINT('Ctrl Pts',(14.8889282288742,51.9671568053379,6.));
#64080=CARTESIAN_POINT('Ctrl Pts',(14.8342503523039,51.942003281804,6.));
#64081=CARTESIAN_POINT('Ctrl Pts',(14.7781470460569,51.9201009098466,6.));
#64082=CARTESIAN_POINT('Ctrl Pts',(14.7209451682992,51.901525951817,6.));
#64083=CARTESIAN_POINT('Ctrl Pts',(14.6856380617977,51.8900608033443,6.));
#64084=CARTESIAN_POINT('Ctrl Pts',(14.649912165413,51.8798643401536,6.));
#64085=CARTESIAN_POINT('Ctrl Pts',(14.6138441166823,51.8709644322168,6.));
#64086=CARTESIAN_POINT('Ctrl Pts',(14.6015017903692,51.8679189231921,6.));
#64087=CARTESIAN_POINT('Ctrl Pts',(14.5891194067602,51.8650253042931,6.));
#64088=CARTESIAN_POINT('Ctrl Pts',(14.5767000729095,51.8622849006199,6.));
#64089=CARTESIAN_POINT('Ctrl Pts',(14.5650829794111,51.859721516297,6.));
#64090=CARTESIAN_POINT('Ctrl Pts',(14.5534409516981,51.8572938729425,6.));
#64091=CARTESIAN_POINT('Ctrl Pts',(14.5417825460264,51.8550036366239,6.));
#64092=CARTESIAN_POINT('Ctrl Pts',(14.4840742560038,51.8436671275493,6.));
#64093=CARTESIAN_POINT('Ctrl Pts',(14.4259183529976,51.8356828275334,6.));
#64094=CARTESIAN_POINT('Ctrl Pts',(14.367620963293,51.8311224894092,6.));
#64095=CARTESIAN_POINT('Ctrl Pts',(14.3108124223156,51.8266786171104,6.));
#64096=CARTESIAN_POINT('Ctrl Pts',(14.2538685533622,51.8254861890659,6.));
#64097=CARTESIAN_POINT('Ctrl Pts',(14.1970797852662,51.8276601888178,6.));
#64098=CARTESIAN_POINT('Ctrl Pts',(14.1662905485933,51.8288388689535,6.));
#64099=CARTESIAN_POINT('Ctrl Pts',(14.1355471146555,51.8310079452875,6.));
#64100=CARTESIAN_POINT('Ctrl Pts',(14.1048981746267,51.8341917567403,6.));
#64101=CARTESIAN_POINT('Ctrl Pts',(14.0793989213186,51.8368406188101,6.));
#64102=CARTESIAN_POINT('Ctrl Pts',(14.0539650963251,51.8401919425187,6.));
#64103=CARTESIAN_POINT('Ctrl Pts',(14.0286260527374,51.8442620100932,6.));
#64104=CARTESIAN_POINT('Ctrl Pts',(14.0177944477837,51.8460018296703,6.));
#64105=CARTESIAN_POINT('Ctrl Pts',(14.0069789238117,51.8478733580886,6.));
#64106=CARTESIAN_POINT('Ctrl Pts',(13.9961993347096,51.8498743913219,6.));
#64107=CARTESIAN_POINT('Ctrl Pts',(13.9463007653032,51.8591371465837,6.));
#64108=CARTESIAN_POINT('Ctrl Pts',(13.8970847123029,51.8711850123457,6.));
#64109=CARTESIAN_POINT('Ctrl Pts',(13.8487579820866,51.8860904144816,6.));
#64110=CARTESIAN_POINT('Ctrl Pts',(13.7947539043108,51.9027468796019,6.));
#64111=CARTESIAN_POINT('Ctrl Pts',(13.7418592133624,51.9229715823681,6.));
#64112=CARTESIAN_POINT('Ctrl Pts',(13.6903202642341,51.946518424925,6.));
#64113=CARTESIAN_POINT('Ctrl Pts',(13.646584361829,51.9665002527549,6.));
#64114=CARTESIAN_POINT('Ctrl Pts',(13.6038249088318,51.9888755884478,6.));
#64115=CARTESIAN_POINT('Ctrl Pts',(13.5622133001607,52.0135148505961,6.));
#64116=CARTESIAN_POINT('Ctrl Pts',(13.5507734482952,52.020288669683,6.));
#64117=CARTESIAN_POINT('Ctrl Pts',(13.5394204822265,52.0272336869092,6.));
#64118=CARTESIAN_POINT('Ctrl Pts',(13.5281582767437,52.0343473928043,6.));
#64119=CARTESIAN_POINT('Ctrl Pts',(13.5193898407158,52.0398859238812,6.));
#64120=CARTESIAN_POINT('Ctrl Pts',(13.5106749799805,52.0455277717941,6.));
#64121=CARTESIAN_POINT('Ctrl Pts',(13.5020295298397,52.0512622212478,6.));
#64122=CARTESIAN_POINT('Ctrl Pts',(13.4557689091919,52.0819464755643,6.));
#64123=CARTESIAN_POINT('Ctrl Pts',(13.4114050030068,52.1153327759281,6.));
#64124=CARTESIAN_POINT('Ctrl Pts',(13.3691631576739,52.1511816197357,6.));
#64125=CARTESIAN_POINT('Ctrl Pts',(13.3271578441964,52.1868297290946,6.));
#64126=CARTESIAN_POINT('Ctrl Pts',(13.2872501899337,52.2249138500805,6.));
#64127=CARTESIAN_POINT('Ctrl Pts',(13.2497024979355,52.2652291267845,6.));
#64128=CARTESIAN_POINT('Ctrl Pts',(13.2148651398199,52.3026342949139,6.));
#64129=CARTESIAN_POINT('Ctrl Pts',(13.1820592965135,52.341961003002,6.));
#64130=CARTESIAN_POINT('Ctrl Pts',(13.1515339536892,52.3830588009893,6.));
#64131=CARTESIAN_POINT('Ctrl Pts',(13.1436930287378,52.393615430985,6.));
#64132=CARTESIAN_POINT('Ctrl Pts',(13.136000309683,52.4042927640824,6.));
#64133=CARTESIAN_POINT('Ctrl Pts',(13.1284766278933,52.4150644154215,6.));
#64134=CARTESIAN_POINT('Ctrl Pts',(13.0980644553258,52.4586055072062,6.));
#64135=CARTESIAN_POINT('Ctrl Pts',(13.0703588458694,52.5037520469927,6.));
#64136=CARTESIAN_POINT('Ctrl Pts',(13.0455900654387,52.5503113513023,6.));
#64137=CARTESIAN_POINT('Ctrl Pts',(13.0216615115385,52.5952912333701,6.));
#64138=CARTESIAN_POINT('Ctrl Pts',(13.0004736387414,52.641590479389,6.));
#64139=CARTESIAN_POINT('Ctrl Pts',(12.98228031951,52.6890470685081,6.));
#64140=CARTESIAN_POINT('Ctrl Pts',(12.9695523308681,52.7222475482892,6.));
#64141=CARTESIAN_POINT('Ctrl Pts',(12.9582909257621,52.7560147190195,6.));
#64142=CARTESIAN_POINT('Ctrl Pts',(12.9485983183411,52.7902936156639,6.));
#64143=CARTESIAN_POINT('Ctrl Pts',(12.943130825006,52.8096299645733,6.));
#64144=CARTESIAN_POINT('Ctrl Pts',(12.9381627931205,52.8291291517902,6.));
#64145=CARTESIAN_POINT('Ctrl Pts',(12.9336933707122,52.8487726938778,6.));
#64146=CARTESIAN_POINT('Origin',(14.1292828945603,53.2669068454841,0.895788276411274));
#64147=CARTESIAN_POINT('Ctrl Pts',(14.9010809748678,54.6051974101417,2.14578827641127));
#64148=CARTESIAN_POINT('Ctrl Pts',(14.8597272487244,54.6294211798578,2.14826884812012));
#64149=CARTESIAN_POINT('Ctrl Pts',(14.3688277705329,54.885598628679,2.17691792328789));
#64150=CARTESIAN_POINT('Ctrl Pts',(13.1694755608909,54.8098887390118,2.23173550191458));
#64151=CARTESIAN_POINT('Ctrl Pts',(12.3130077055018,53.3174154968919,2.31024101229137));
#64152=CARTESIAN_POINT('Ctrl Pts',(13.0852322400692,51.7797767714816,2.38874652266814));
#64153=CARTESIAN_POINT('Ctrl Pts',(14.7938791388702,51.5757659053288,2.46725203304493));
#64154=CARTESIAN_POINT('Ctrl Pts',(15.9064540032169,52.8884432158558,2.5457575434217));
#64155=CARTESIAN_POINT('Ctrl Pts',(15.5416657446855,54.1408201433548,2.60526962454382));
#64156=CARTESIAN_POINT('Ctrl Pts',(15.0227829664514,54.5334351262247,2.63861320220701));
#64157=CARTESIAN_POINT('Ctrl Pts',(14.9016274172746,54.6020379108679,2.64578827641127));
#64158=CARTESIAN_POINT('Ctrl Pts',(14.9013089558621,54.600969116598,2.10421172358873));
#64159=CARTESIAN_POINT('Ctrl Pts',(14.6040162957702,54.7699114721225,2.12181148931034));
#64160=CARTESIAN_POINT('Ctrl Pts',(13.7242010739631,54.9558633776928,2.16557975849087));
#64161=CARTESIAN_POINT('Ctrl Pts',(12.4888977717378,54.0475500892828,2.23551653113034));
#64162=CARTESIAN_POINT('Ctrl Pts',(12.5727324025626,52.3295818538895,2.31402204150712));
#64163=CARTESIAN_POINT('Ctrl Pts',(14.0528383317196,51.4513683986094,2.3925275518839));
#64164=CARTESIAN_POINT('Ctrl Pts',(15.6013423678816,52.2018016959779,2.47103306226067));
#64165=CARTESIAN_POINT('Ctrl Pts',(15.8066350265236,53.7346571674393,2.54159445282895));
#64166=CARTESIAN_POINT('Ctrl Pts',(15.2043102739953,54.4236472184416,2.5859873399383));
#64167=CARTESIAN_POINT('Ctrl Pts',(14.8992309062956,54.6029598038327,2.60421172358873));
#64168=CARTESIAN_POINT('Ctrl Pts',(12.9355708698302,52.8497595669186,2.));
#64169=CARTESIAN_POINT('Ctrl Pts',(13.0727468794464,52.4572155888145,2.02616850345893));
#64170=CARTESIAN_POINT('Ctrl Pts',(13.762195269905,51.8244143348174,2.07850551037678));
#64171=CARTESIAN_POINT('Ctrl Pts',(15.132331970736,52.1652352880051,2.15701102075356));
#64172=CARTESIAN_POINT('Ctrl Pts',(15.600345878683,53.4958301810381,2.23551653113034));
#64173=CARTESIAN_POINT('Ctrl Pts',(14.7503158422929,54.6202478137908,2.31402204150712));
#64174=CARTESIAN_POINT('Ctrl Pts',(13.3427136311611,54.5313920070952,2.3925275518839));
#64175=CARTESIAN_POINT('Ctrl Pts',(12.6408318404031,53.3082990617544,2.47103306226068));
#64176=CARTESIAN_POINT('Ctrl Pts',(13.2736756018811,52.0481926662384,2.54953857263746));
#64177=CARTESIAN_POINT('Ctrl Pts',(14.6739244700172,51.8810042409304,2.62804408301423));
#64178=CARTESIAN_POINT('Ctrl Pts',(15.5856878633849,52.9567530803091,2.70654959339101));
#64179=CARTESIAN_POINT('Ctrl Pts',(15.1913315822309,54.3106417984377,2.78505510376779));
#64180=CARTESIAN_POINT('Ctrl Pts',(13.8444953540085,54.7284908735361,2.86356061414457));
#64181=CARTESIAN_POINT('Ctrl Pts',(12.7530680664412,53.8355533167568,2.94206612452135));
#64182=CARTESIAN_POINT('Ctrl Pts',(12.8958606092945,52.4326417450687,3.02057163489813));
#64183=CARTESIAN_POINT('Ctrl Pts',(14.1448167496288,51.7779181217064,3.09907714527491));
#64184=CARTESIAN_POINT('Ctrl Pts',(15.3798411765859,52.4585553969251,3.17758265565169));
#64185=CARTESIAN_POINT('Ctrl Pts',(15.4933354964796,53.86414126306,3.25608816602848));
#64186=CARTESIAN_POINT('Ctrl Pts',(14.3835148696119,54.7341132075812,3.33459367640524));
#64187=CARTESIAN_POINT('Ctrl Pts',(13.0456930357207,54.2882595546367,3.41309918678203));
#64188=CARTESIAN_POINT('Ctrl Pts',(12.6796603121051,52.9264325363301,3.4916046971588));
#64189=CARTESIAN_POINT('Ctrl Pts',(13.6136836011906,51.8699509600852,3.57011020753559));
#64190=CARTESIAN_POINT('Ctrl Pts',(15.0101085852912,52.066292638923,3.64861571791237));
#64191=CARTESIAN_POINT('Ctrl Pts',(15.6165881539763,53.3393736780174,3.72712122828915));
#64192=CARTESIAN_POINT('Ctrl Pts',(14.8892170051293,54.5474647404685,3.80562673866593));
#64193=CARTESIAN_POINT('Ctrl Pts',(13.4803188806438,54.6071210383936,3.88413224904271));
#64194=CARTESIAN_POINT('Ctrl Pts',(12.6534271115016,53.4648413867365,3.96263775941949));
#64195=CARTESIAN_POINT('Ctrl Pts',(13.1501178953861,52.1450493326719,4.04114326979627));
#64196=CARTESIAN_POINT('Ctrl Pts',(14.5249471286252,51.8313657668162,4.11964878017305));
#64197=CARTESIAN_POINT('Ctrl Pts',(15.5449352706107,52.805109568325,4.19815429054982));
#64198=CARTESIAN_POINT('Ctrl Pts',(15.2953327061785,54.1930041465599,4.2766598009266));
#64199=CARTESIAN_POINT('Ctrl Pts',(13.9999889501244,54.7503526485877,4.35516531130338));
#64200=CARTESIAN_POINT('Ctrl Pts',(12.8205990758801,53.9773116872669,4.43367082168016));
#64201=CARTESIAN_POINT('Ctrl Pts',(12.8148679650961,52.5671627753774,4.51217633205694));
#64202=CARTESIAN_POINT('Ctrl Pts',(13.9879354060904,51.7845609801148,4.59068184243372));
#64203=CARTESIAN_POINT('Ctrl Pts',(15.2877666458998,52.3313621994942,4.6691873528105));
#64204=CARTESIAN_POINT('Ctrl Pts',(15.5486420944497,53.7171820950402,4.74769286318728));
#64205=CARTESIAN_POINT('Ctrl Pts',(14.5366025126985,54.699184449441,4.82619837356406));
#64206=CARTESIAN_POINT('Ctrl Pts',(13.1592689266914,54.3966861834431,4.90470388394084));
#64207=CARTESIAN_POINT('Ctrl Pts',(12.651867102821,53.0809749777223,4.98320939431762));
#64208=CARTESIAN_POINT('Ctrl Pts',(13.4694465335298,51.9320118320646,5.06171490469439));
#64209=CARTESIAN_POINT('Ctrl Pts',(14.8787836035794,51.980214388546,5.14022041507118));
#64210=CARTESIAN_POINT('Ctrl Pts',(15.6159492071913,53.1823530914927,5.21872592544796));
#64211=CARTESIAN_POINT('Ctrl Pts',(15.0198399508834,54.4603220891203,5.29723143582474));
#64212=CARTESIAN_POINT('Ctrl Pts',(13.6250522726906,54.6680069657356,5.37573694620152));
#64213=CARTESIAN_POINT('Ctrl Pts',(12.6824820007894,53.6191538682575,5.4542424565783));
#64214=CARTESIAN_POINT('Ctrl Pts',(13.0374143051106,52.2543934093273,5.53274796695507));
#64215=CARTESIAN_POINT('Ctrl Pts',(14.3716061738679,51.7976868080881,5.61125347733186));
#64216=CARTESIAN_POINT('Ctrl Pts',(15.4883847851255,52.6585961458811,5.68975898770863));
#64217=CARTESIAN_POINT('Ctrl Pts',(15.3864730097086,54.0650841092748,5.76826449808542));
#64218=CARTESIAN_POINT('Ctrl Pts',(14.156713139869,54.755685297877,5.84677000846219));
#64219=CARTESIAN_POINT('Ctrl Pts',(12.9030960095781,54.1112396708051,5.92527551883898));
#64220=CARTESIAN_POINT('Ctrl Pts',(12.7476560431649,52.7093273325191,6.00378102921575));
#64221=CARTESIAN_POINT('Ctrl Pts',(13.8343697837273,51.8079468650312,6.08228653959253));
#64222=CARTESIAN_POINT('Ctrl Pts',(14.7300614275787,52.0790796540862,6.13462354651038));
#64223=CARTESIAN_POINT('Ctrl Pts',(15.0239255378924,52.3732767258419,6.16079204996931));
#64224=CARTESIAN_POINT('Ctrl Pts',(12.8479344393867,52.8191346777449,1.94640265001023));
#64225=CARTESIAN_POINT('Ctrl Pts',(12.9951812328907,52.3977720630513,1.97257115346916));
#64226=CARTESIAN_POINT('Ctrl Pts',(13.7352455128293,51.7185136720468,2.02490816038701));
#64227=CARTESIAN_POINT('Ctrl Pts',(15.2059708708849,52.0843560132567,2.10341367076379));
#64228=CARTESIAN_POINT('Ctrl Pts',(15.7083440442499,53.5126365996361,2.18191918114057));
#64229=CARTESIAN_POINT('Ctrl Pts',(14.7959090084834,54.7196034114378,2.26042469151735));
#64230=CARTESIAN_POINT('Ctrl Pts',(13.2849676077377,54.6242242510673,2.33893020189412));
#64231=CARTESIAN_POINT('Ctrl Pts',(12.5315571287693,53.311337873467,2.41743571227091));
#64232=CARTESIAN_POINT('Ctrl Pts',(13.2108611479438,51.9587207013194,2.49594122264769));
#64233=CARTESIAN_POINT('Ctrl Pts',(14.7139093596349,51.7792581290633,2.57444673302446));
#64234=CARTESIAN_POINT('Ctrl Pts',(15.6926099099956,52.9339831254913,2.65295224340124));
#64235=CARTESIAN_POINT('Ctrl Pts',(15.2693019419295,54.3872676543484,2.73145775377802));
#64236=CARTESIAN_POINT('Ctrl Pts',(13.8235876618921,54.8357931410496,2.80996326415481));
#64237=CARTESIAN_POINT('Ctrl Pts',(12.6520331831853,53.8773005270505,2.88846877453158));
#64238=CARTESIAN_POINT('Ctrl Pts',(12.8053088480064,52.3713941292876,2.96697428490836));
#64239=CARTESIAN_POINT('Ctrl Pts',(14.1459571684074,51.6686039370295,3.04547979528514));
#64240=CARTESIAN_POINT('Ctrl Pts',(15.4716509779683,52.3992102332441,3.12398530566192));
#64241=CARTESIAN_POINT('Ctrl Pts',(15.5934774892658,53.90798725892,3.2024908160387));
#64242=CARTESIAN_POINT('Ctrl Pts',(14.4021793232963,54.8418282390413,3.28099632641548));
#64243=CARTESIAN_POINT('Ctrl Pts',(12.9661412298193,54.3632422169536,3.35950183679226));
#64244=CARTESIAN_POINT('Ctrl Pts',(12.5732361947429,52.9014365971975,3.43800734716904));
#64245=CARTESIAN_POINT('Ctrl Pts',(13.5758308522243,51.7673933710292,3.51651285754582));
#64246=CARTESIAN_POINT('Ctrl Pts',(15.0747744492344,51.978149484441,3.5950183679226));
#64247=CARTESIAN_POINT('Ctrl Pts',(15.7257787470296,53.3446938343006,3.67352387829938));
#64248=CARTESIAN_POINT('Ctrl Pts',(14.945007607421,54.6414769649982,3.75202938867616));
#64249=CARTESIAN_POINT('Ctrl Pts',(13.4326751537753,54.7055129331413,3.83053489905294));
#64250=CARTESIAN_POINT('Ctrl Pts',(12.5450770823512,53.4793727613876,3.90904040942971));
#64251=CARTESIAN_POINT('Ctrl Pts',(13.0782324459937,52.0626881049618,3.9875459198065));
#64252=CARTESIAN_POINT('Ctrl Pts',(14.5539948389685,51.7259754437876,4.06605143018328));
#64253=CARTESIAN_POINT('Ctrl Pts',(15.6488654635012,52.77120669718,4.14455694056005));
#64254=CARTESIAN_POINT('Ctrl Pts',(15.3809383138062,54.2609936281335,4.22306245093684));
#64255=CARTESIAN_POINT('Ctrl Pts',(13.9904968284622,54.8592598994548,4.30156796131361));
#64256=CARTESIAN_POINT('Ctrl Pts',(12.724521985198,54.029466095712,4.3800734716904));
#64257=CARTESIAN_POINT('Ctrl Pts',(12.7183701246174,52.51579102804,4.45857898206717));
#64258=CARTESIAN_POINT('Ctrl Pts',(13.9775583728655,51.6757344812336,4.53708449244395));
#64259=CARTESIAN_POINT('Ctrl Pts',(15.3728167908182,52.2626791406019,4.61559000282073));
#64260=CARTESIAN_POINT('Ctrl Pts',(15.6528444240053,53.7502390759288,4.69409551319751));
#64261=CARTESIAN_POINT('Ctrl Pts',(14.5665059036703,54.8043351843039,4.77260102357429));
#64262=CARTESIAN_POINT('Ctrl Pts',(13.0880553007387,54.4796289923587,4.85110653395107));
#64263=CARTESIAN_POINT('Ctrl Pts',(12.5434025455521,53.0673247799706,4.92961204432785));
#64264=CARTESIAN_POINT('Ctrl Pts',(13.4210046127318,51.834010445156,5.00811755470463));
#64265=CARTESIAN_POINT('Ctrl Pts',(14.9338082371531,51.8857517948312,5.08662306508141));
#64266=CARTESIAN_POINT('Ctrl Pts',(15.725092891933,53.1761455732414,5.16512857545819));
#64267=CARTESIAN_POINT('Ctrl Pts',(15.0852202435382,54.5479367313644,5.24363408583497));
#64268=CARTESIAN_POINT('Ctrl Pts',(13.5880341553344,54.770868804009,5.32213959621175));
#64269=CARTESIAN_POINT('Ctrl Pts',(12.5762650378488,53.6450141017733,5.40064510658853));
#64270=CARTESIAN_POINT('Ctrl Pts',(12.9572547157705,52.1800596826977,5.4791506169653));
#64271=CARTESIAN_POINT('Ctrl Pts',(14.3893963500342,51.6898239425509,5.55765612734209));
#64272=CARTESIAN_POINT('Ctrl Pts',(15.5881633211799,52.6139369841995,5.63616163771886));
#64273=CARTESIAN_POINT('Ctrl Pts',(15.478769687465,54.1236823346512,5.71466714809565));
#64274=CARTESIAN_POINT('Ctrl Pts',(14.1587269327564,54.8649840454693,5.79317265847242));
#64275=CARTESIAN_POINT('Ctrl Pts',(12.8130754355785,54.1732264091344,5.8716781688492));
#64276=CARTESIAN_POINT('Ctrl Pts',(12.6462238359385,52.6683926035456,5.95018367922598));
#64277=CARTESIAN_POINT('Ctrl Pts',(13.8127187223415,51.7008372421088,6.02868918960276));
#64278=CARTESIAN_POINT('Ctrl Pts',(14.7741676148585,51.9918752589882,6.08102619652061));
#64279=CARTESIAN_POINT('Ctrl Pts',(15.0896057741302,52.3076708240835,6.10719469997954));
#64280=CARTESIAN_POINT('Ctrl Pts',(12.7602980089432,52.7885097885711,1.89280530002046));
#64281=CARTESIAN_POINT('Ctrl Pts',(12.9176155863349,52.3383285372882,1.91897380347939));
#64282=CARTESIAN_POINT('Ctrl Pts',(13.7082957557536,51.6126130092761,1.97131081039724));
#64283=CARTESIAN_POINT('Ctrl Pts',(15.2796097710338,52.0034767385083,2.04981632077402));
#64284=CARTESIAN_POINT('Ctrl Pts',(15.8163422098168,53.5294430182342,2.1283218311508));
#64285=CARTESIAN_POINT('Ctrl Pts',(14.8415021746739,54.8189590090846,2.20682734152758));
#64286=CARTESIAN_POINT('Ctrl Pts',(13.2272215843143,54.7170564950396,2.28533285190435));
#64287=CARTESIAN_POINT('Ctrl Pts',(12.4222824171356,53.3143766851794,2.36383836228114));
#64288=CARTESIAN_POINT('Ctrl Pts',(13.1480466940064,51.8692487364006,2.44234387265791));
#64289=CARTESIAN_POINT('Ctrl Pts',(14.7538942492525,51.677512017196,2.52084938303469));
#64290=CARTESIAN_POINT('Ctrl Pts',(15.7995319566062,52.9112131706735,2.59935489341147));
#64291=CARTESIAN_POINT('Ctrl Pts',(15.347272301628,54.4638935102592,2.67786040378825));
#64292=CARTESIAN_POINT('Ctrl Pts',(13.8026799697756,54.9430954085631,2.75636591416504));
#64293=CARTESIAN_POINT('Ctrl Pts',(12.5509982999295,53.9190477373443,2.83487142454181));
#64294=CARTESIAN_POINT('Ctrl Pts',(12.7147570867183,52.3101465135065,2.91337693491859));
#64295=CARTESIAN_POINT('Ctrl Pts',(14.147097587186,51.5592897523524,2.99188244529537));
#64296=CARTESIAN_POINT('Ctrl Pts',(15.5634607793508,52.3398650695633,3.07038795567215));
#64297=CARTESIAN_POINT('Ctrl Pts',(15.693619482052,53.9518332547799,3.14889346604893));
#64298=CARTESIAN_POINT('Ctrl Pts',(14.4208437769808,54.9495432705015,3.22739897642571));
#64299=CARTESIAN_POINT('Ctrl Pts',(12.8865894239179,54.4382248792704,3.30590448680249));
#64300=CARTESIAN_POINT('Ctrl Pts',(12.4668120773806,52.876440658065,3.38440999717926));
#64301=CARTESIAN_POINT('Ctrl Pts',(13.5379781032581,51.6648357819733,3.46291550755605));
#64302=CARTESIAN_POINT('Ctrl Pts',(15.1394403131777,51.8900063299591,3.54142101793282));
#64303=CARTESIAN_POINT('Ctrl Pts',(15.8349693400828,53.3500139905838,3.61992652830961));
#64304=CARTESIAN_POINT('Ctrl Pts',(15.0007982097127,54.7354891895278,3.69843203868638));
#64305=CARTESIAN_POINT('Ctrl Pts',(13.3850314269068,54.8039048278889,3.77693754906317));
#64306=CARTESIAN_POINT('Ctrl Pts',(12.4367270532009,53.4939041360386,3.85544305943994));
#64307=CARTESIAN_POINT('Ctrl Pts',(13.0063469966013,51.9803268772517,3.93394856981673));
#64308=CARTESIAN_POINT('Ctrl Pts',(14.5830425493117,51.620585120759,4.0124540801935));
#64309=CARTESIAN_POINT('Ctrl Pts',(15.7527956563917,52.7373038260349,4.09095959057029));
#64310=CARTESIAN_POINT('Ctrl Pts',(15.4665439214339,54.3289831097072,4.16946510094706));
#64311=CARTESIAN_POINT('Ctrl Pts',(13.9810047068001,54.9681671503218,4.24797061132385));
#64312=CARTESIAN_POINT('Ctrl Pts',(12.628444894516,54.0816205041572,4.32647612170062));
#64313=CARTESIAN_POINT('Ctrl Pts',(12.6218722841387,52.4644192807024,4.40498163207741));
#64314=CARTESIAN_POINT('Ctrl Pts',(13.9671813396405,51.5669079823527,4.48348714245418));
#64315=CARTESIAN_POINT('Ctrl Pts',(15.4578669357366,52.1939960817095,4.56199265283096));
#64316=CARTESIAN_POINT('Ctrl Pts',(15.7570467535609,53.7832960568176,4.64049816320774));
#64317=CARTESIAN_POINT('Ctrl Pts',(14.5964092946421,54.9094859191667,4.71900367358452));
#64318=CARTESIAN_POINT('Ctrl Pts',(13.016841674786,54.5625718012743,4.7975091839613));
#64319=CARTESIAN_POINT('Ctrl Pts',(12.4349379882832,53.0536745822187,4.87601469433807));
#64320=CARTESIAN_POINT('Ctrl Pts',(13.3725626919339,51.7360090582476,4.95452020471486));
#64321=CARTESIAN_POINT('Ctrl Pts',(14.9888328707268,51.7912892011163,5.03302571509164));
#64322=CARTESIAN_POINT('Ctrl Pts',(15.8342365766747,53.16993805499,5.11153122546842));
#64323=CARTESIAN_POINT('Ctrl Pts',(15.150600536193,54.6355513736084,5.1900367358452));
#64324=CARTESIAN_POINT('Ctrl Pts',(13.5510160379782,54.8737306422823,5.26854224622198));
#64325=CARTESIAN_POINT('Ctrl Pts',(12.4700480749082,53.6708743352892,5.34704775659876));
#64326=CARTESIAN_POINT('Ctrl Pts',(12.8770951264304,52.105725956068,5.42555326697553));
#64327=CARTESIAN_POINT('Ctrl Pts',(14.4071865262006,51.581961077014,5.50405877735232));
#64328=CARTESIAN_POINT('Ctrl Pts',(15.6879418572343,52.5692778225177,5.58256428772909));
#64329=CARTESIAN_POINT('Ctrl Pts',(15.5710663652214,54.1822805600277,5.66106979810588));
#64330=CARTESIAN_POINT('Ctrl Pts',(14.1607407256438,54.9742827930615,5.73957530848265));
#64331=CARTESIAN_POINT('Ctrl Pts',(12.7230548615789,54.2352131474636,5.81808081885943));
#64332=CARTESIAN_POINT('Ctrl Pts',(12.544791628712,52.6274578745722,5.89658632923621));
#64333=CARTESIAN_POINT('Ctrl Pts',(13.7910676609557,51.5937276191864,5.97509183961299));
#64334=CARTESIAN_POINT('Ctrl Pts',(14.8182738021382,51.9046708638902,6.02742884653084));
#64335=CARTESIAN_POINT('Ctrl Pts',(15.1552860103679,52.2420649223251,6.05359734998977));
#64336=CARTESIAN_POINT('Ctrl Pts',(12.6726615784997,52.7578848993974,1.83920795003069));
#64337=CARTESIAN_POINT('Ctrl Pts',(12.8400499397792,52.278885011525,1.86537645348962));
#64338=CARTESIAN_POINT('Ctrl Pts',(13.681345998678,51.5067123465054,1.91771346040747));
#64339=CARTESIAN_POINT('Ctrl Pts',(15.3532486711827,51.92259746376,1.99621897078425));
#64340=CARTESIAN_POINT('Ctrl Pts',(15.9243403753838,53.5462494368323,2.07472448116102));
#64341=CARTESIAN_POINT('Ctrl Pts',(14.8870953408643,54.9183146067315,2.15322999153781));
#64342=CARTESIAN_POINT('Ctrl Pts',(13.1694755608909,54.8098887390118,2.23173550191458));
#64343=CARTESIAN_POINT('Ctrl Pts',(12.3130077055018,53.3174154968919,2.31024101229137));
#64344=CARTESIAN_POINT('Ctrl Pts',(13.0852322400692,51.7797767714816,2.38874652266814));
#64345=CARTESIAN_POINT('Ctrl Pts',(14.7938791388702,51.5757659053288,2.46725203304493));
#64346=CARTESIAN_POINT('Ctrl Pts',(15.9064540032169,52.8884432158558,2.5457575434217));
#64347=CARTESIAN_POINT('Ctrl Pts',(15.4252426613265,54.54051936617,2.62426305379848));
#64348=CARTESIAN_POINT('Ctrl Pts',(13.7817722776592,55.0503976760766,2.70276856417526));
#64349=CARTESIAN_POINT('Ctrl Pts',(12.4499634166736,53.9607949476381,2.78127407455204));
#64350=CARTESIAN_POINT('Ctrl Pts',(12.6242053254301,52.2488988977253,2.85977958492882));
#64351=CARTESIAN_POINT('Ctrl Pts',(14.1482380059646,51.4499755676755,2.9382850953056));
#64352=CARTESIAN_POINT('Ctrl Pts',(15.6552705807332,52.2805199058823,3.01679060568238));
#64353=CARTESIAN_POINT('Ctrl Pts',(15.7937614748382,53.9956792506399,3.09529611605916));
#64354=CARTESIAN_POINT('Ctrl Pts',(14.4395082306652,55.0572583019616,3.17380162643594));
#64355=CARTESIAN_POINT('Ctrl Pts',(12.8070376180166,54.5132075415872,3.25230713681272));
#64356=CARTESIAN_POINT('Ctrl Pts',(12.3603879600183,52.8514447189324,3.3308126471895));
#64357=CARTESIAN_POINT('Ctrl Pts',(13.5001253542918,51.5622781929174,3.40931815756628));
#64358=CARTESIAN_POINT('Ctrl Pts',(15.2041061771209,51.8018631754771,3.48782366794306));
#64359=CARTESIAN_POINT('Ctrl Pts',(15.944159933136,53.3553341468671,3.56632917831984));
#64360=CARTESIAN_POINT('Ctrl Pts',(15.0565888120043,54.8295014140575,3.64483468869661));
#64361=CARTESIAN_POINT('Ctrl Pts',(13.3373877000383,54.9022967226367,3.7233401990734));
#64362=CARTESIAN_POINT('Ctrl Pts',(12.3283770240505,53.5084355106896,3.80184570945017));
#64363=CARTESIAN_POINT('Ctrl Pts',(12.9344615472089,51.8979656495417,3.88035121982696));
#64364=CARTESIAN_POINT('Ctrl Pts',(14.6120902596549,51.5151947977303,3.95885673020373));
#64365=CARTESIAN_POINT('Ctrl Pts',(15.8567258492822,52.7034009548899,4.03736224058051));
#64366=CARTESIAN_POINT('Ctrl Pts',(15.5521495290616,54.3969725912808,4.11586775095729));
#64367=CARTESIAN_POINT('Ctrl Pts',(13.9715125851379,55.077074401189,4.19437326133407));
#64368=CARTESIAN_POINT('Ctrl Pts',(12.5323678038339,54.1337749126023,4.27287877171085));
#64369=CARTESIAN_POINT('Ctrl Pts',(12.5253744436601,52.413047533365,4.35138428208763));
#64370=CARTESIAN_POINT('Ctrl Pts',(13.9568043064156,51.4580814834716,4.42988979246441));
#64371=CARTESIAN_POINT('Ctrl Pts',(15.5429170806551,52.1253130228171,4.50839530284119));
#64372=CARTESIAN_POINT('Ctrl Pts',(15.8612490831165,53.8163530377063,4.58690081321797));
#64373=CARTESIAN_POINT('Ctrl Pts',(14.6263126856138,55.0146366540294,4.66540632359475));
#64374=CARTESIAN_POINT('Ctrl Pts',(12.9456280488333,54.6455146101901,4.74391183397153));
#64375=CARTESIAN_POINT('Ctrl Pts',(12.3264734310144,53.0400243844668,4.8224173443483));
#64376=CARTESIAN_POINT('Ctrl Pts',(13.3241207711359,51.6380076713391,4.90092285472509));
#64377=CARTESIAN_POINT('Ctrl Pts',(15.0438575043004,51.6968266074015,4.97942836510187));
#64378=CARTESIAN_POINT('Ctrl Pts',(15.9433802614164,53.1637305367386,5.05793387547864));
#64379=CARTESIAN_POINT('Ctrl Pts',(15.2159808288478,54.7231660158524,5.13643938585543));
#64380=CARTESIAN_POINT('Ctrl Pts',(13.513997920622,54.9765924805557,5.21494489623221));
#64381=CARTESIAN_POINT('Ctrl Pts',(12.3638311119676,53.696734568805,5.29345040660898));
#64382=CARTESIAN_POINT('Ctrl Pts',(12.7969355370903,52.0313922294383,5.37195591698577));
#64383=CARTESIAN_POINT('Ctrl Pts',(14.424976702367,51.4740982114769,5.45046142736254));
#64384=CARTESIAN_POINT('Ctrl Pts',(15.7877203932888,52.5246186608361,5.52896693773932));
#64385=CARTESIAN_POINT('Ctrl Pts',(15.6633630429778,54.2408787854042,5.60747244811611));
#64386=CARTESIAN_POINT('Ctrl Pts',(14.1627545185313,55.0835815406539,5.68597795849288));
#64387=CARTESIAN_POINT('Ctrl Pts',(12.6330342875793,54.2971998857928,5.76448346886966));
#64388=CARTESIAN_POINT('Ctrl Pts',(12.4433594214855,52.5865231455987,5.84298897924644));
#64389=CARTESIAN_POINT('Ctrl Pts',(13.7694165995699,51.486617996264,5.92149448962322));
#64390=CARTESIAN_POINT('Ctrl Pts',(14.8623799894179,51.8174664687921,5.97383149654107));
#64391=CARTESIAN_POINT('Ctrl Pts',(15.2209662466057,52.1764590205668,6.));
#64392=CARTESIAN_POINT('Ctrl Pts',(12.9355708698302,52.8497595669186,2.));
#64393=CARTESIAN_POINT('Ctrl Pts',(12.9469576730111,52.8006000143775,2.));
#64394=CARTESIAN_POINT('Ctrl Pts',(12.961472067899,52.7523805759131,2.));
#64395=CARTESIAN_POINT('Ctrl Pts',(12.978838111258,52.7052630574514,2.));
#64396=CARTESIAN_POINT('Ctrl Pts',(12.9969823676722,52.6560340926898,2.));
#64397=CARTESIAN_POINT('Ctrl Pts',(13.0182396625101,52.6080072539831,2.));
#64398=CARTESIAN_POINT('Ctrl Pts',(13.0423523228538,52.5613664966406,2.));
#64399=CARTESIAN_POINT('Ctrl Pts',(13.0616899932819,52.5239619306927,2.));
#64400=CARTESIAN_POINT('Ctrl Pts',(13.0828653436295,52.4874486478152,2.));
#64401=CARTESIAN_POINT('Ctrl Pts',(13.1057691188089,52.4519266272332,2.));
#64402=CARTESIAN_POINT('Ctrl Pts',(13.1154541423168,52.4369058893117,2.));
#64403=CARTESIAN_POINT('Ctrl Pts',(13.1254484616954,52.4220624809456,2.));
#64404=CARTESIAN_POINT('Ctrl Pts',(13.1357448170144,52.4074044118627,2.));
#64405=CARTESIAN_POINT('Ctrl Pts',(13.1415823490888,52.3990940004822,2.));
#64406=CARTESIAN_POINT('Ctrl Pts',(13.1475174809101,52.3908426597185,2.));
#64407=CARTESIAN_POINT('Ctrl Pts',(13.1535391079478,52.3826647593444,2.));
#64408=CARTESIAN_POINT('Ctrl Pts',(13.1858180051981,52.3388271712232,2.));
#64409=CARTESIAN_POINT('Ctrl Pts',(13.2206401756997,52.2970090605356,2.));
#64410=CARTESIAN_POINT('Ctrl Pts',(13.2577323841621,52.2574000923877,2.));
#64411=CARTESIAN_POINT('Ctrl Pts',(13.2955035907129,52.2170660551546,2.));
#64412=CARTESIAN_POINT('Ctrl Pts',(13.3356292075102,52.1790218018834,2.));
#64413=CARTESIAN_POINT('Ctrl Pts',(13.3778710217058,52.1434855491538,2.));
#64414=CARTESIAN_POINT('Ctrl Pts',(13.4080812323462,52.1180709759216,2.));
#64415=CARTESIAN_POINT('Ctrl Pts',(13.4393749054926,52.0939395106326,2.));
#64416=CARTESIAN_POINT('Ctrl Pts',(13.4716779317629,52.0711807776388,2.));
#64417=CARTESIAN_POINT('Ctrl Pts',(13.4854146711569,52.0615027127585,2.));
#64418=CARTESIAN_POINT('Ctrl Pts',(13.4993340562547,52.0520730061524,2.));
#64419=CARTESIAN_POINT('Ctrl Pts',(13.5134308827525,52.042899142872,2.));
#64420=CARTESIAN_POINT('Ctrl Pts',(13.521831360858,52.0374323211272,2.));
#64421=CARTESIAN_POINT('Ctrl Pts',(13.5302901168969,52.0320595108474,2.));
#64422=CARTESIAN_POINT('Ctrl Pts',(13.5387993574829,52.0267858960721,2.));
#64423=CARTESIAN_POINT('Ctrl Pts',(13.5870981540731,51.9968526435391,2.));
#64424=CARTESIAN_POINT('Ctrl Pts',(13.6370817516734,51.9700725296277,2.));
#64425=CARTESIAN_POINT('Ctrl Pts',(13.6884925441937,51.946663606087,2.));
#64426=CARTESIAN_POINT('Ctrl Pts',(13.7200525423943,51.9322933630192,2.));
#64427=CARTESIAN_POINT('Ctrl Pts',(13.7521512848191,51.9191940299568,2.));
#64428=CARTESIAN_POINT('Ctrl Pts',(13.7847364470978,51.9074225450413,2.));
#64429=CARTESIAN_POINT('Ctrl Pts',(13.8364187923908,51.8887521470605,2.));
#64430=CARTESIAN_POINT('Ctrl Pts',(13.889323789898,51.8734194145927,2.));
#64431=CARTESIAN_POINT('Ctrl Pts',(13.943161175005,51.8613307211758,2.));
#64432=CARTESIAN_POINT('Ctrl Pts',(13.9592695283984,51.8577137374528,2.));
#64433=CARTESIAN_POINT('Ctrl Pts',(13.9754615001933,51.8543874911094,2.));
#64434=CARTESIAN_POINT('Ctrl Pts',(13.9917296362982,51.8513502983977,2.));
#64435=CARTESIAN_POINT('Ctrl Pts',(14.0067700369102,51.848542318748,2.));
#64436=CARTESIAN_POINT('Ctrl Pts',(14.0218822544722,51.8459805725644,2.));
#64437=CARTESIAN_POINT('Ctrl Pts',(14.0370239759719,51.8436690391775,2.));
#64438=CARTESIAN_POINT('Ctrl Pts',(14.0931183782243,51.8351056744616,2.));
#64439=CARTESIAN_POINT('Ctrl Pts',(14.1496871524976,51.8299561325418,2.));
#64440=CARTESIAN_POINT('Ctrl Pts',(14.2064063479419,51.8280805152347,2.));
#64441=CARTESIAN_POINT('Ctrl Pts',(14.2644669778257,51.8261605387362,2.));
#64442=CARTESIAN_POINT('Ctrl Pts',(14.3226861857367,51.8276710218956,2.));
#64443=CARTESIAN_POINT('Ctrl Pts',(14.3807392826023,51.8325126403789,2.));
#64444=CARTESIAN_POINT('Ctrl Pts',(14.4159849881094,51.8354521262711,2.));
#64445=CARTESIAN_POINT('Ctrl Pts',(14.4511698447437,51.8396204788396,2.));
#64446=CARTESIAN_POINT('Ctrl Pts',(14.4862227576295,51.8450046114997,2.));
#64447=CARTESIAN_POINT('Ctrl Pts',(14.5055224539705,51.8479690477433,2.));
#64448=CARTESIAN_POINT('Ctrl Pts',(14.5247821602859,51.851302164794,2.));
#64449=CARTESIAN_POINT('Ctrl Pts',(14.5439899738579,51.8550026668836,2.));
#64450=CARTESIAN_POINT('Ctrl Pts',(14.5555560513146,51.8572309420403,2.));
#64451=CARTESIAN_POINT('Ctrl Pts',(14.567105278279,51.8595928680997,2.));
#64452=CARTESIAN_POINT('Ctrl Pts',(14.5786287781909,51.8620869089327,2.));
#64453=CARTESIAN_POINT('Ctrl Pts',(14.6376831017328,51.8748680861278,2.));
#64454=CARTESIAN_POINT('Ctrl Pts',(14.6958774997188,51.8910736753892,2.));
#64455=CARTESIAN_POINT('Ctrl Pts',(14.7528646870533,51.9106036961834,2.));
#64456=CARTESIAN_POINT('Ctrl Pts',(14.7899177176958,51.9233021024882,2.));
#64457=CARTESIAN_POINT('Ctrl Pts',(14.8264606634288,51.937407019632,2.));
#64458=CARTESIAN_POINT('Ctrl Pts',(14.8623979324725,51.9529027870001,2.));
#64459=CARTESIAN_POINT('Ctrl Pts',(14.8772478015379,51.9593058922613,2.));
#64460=CARTESIAN_POINT('Ctrl Pts',(14.8919942354036,51.9659465911201,2.));
#64461=CARTESIAN_POINT('Ctrl Pts',(14.9066303802712,51.9728242372186,2.));
#64462=CARTESIAN_POINT('Ctrl Pts',(14.9173472275455,51.977860172809,2.));
#64463=CARTESIAN_POINT('Ctrl Pts',(14.9280038817855,51.9830227414594,2.));
#64464=CARTESIAN_POINT('Ctrl Pts',(14.9385887529819,51.9883069953249,2.));
#64465=CARTESIAN_POINT('Ctrl Pts',(14.9930076776348,52.015474393739,2.));
#64466=CARTESIAN_POINT('Ctrl Pts',(15.0455947546072,52.0458841567652,2.));
#64467=CARTESIAN_POINT('Ctrl Pts',(15.0960008498488,52.0794651524452,2.));
#64468=CARTESIAN_POINT('Ctrl Pts',(15.1196129597981,52.0951957532466,2.));
#64469=CARTESIAN_POINT('Ctrl Pts',(15.1427463702482,52.1116229529516,2.));
#64470=CARTESIAN_POINT('Ctrl Pts',(15.1653640074689,52.1287432229353,2.));
#64471=CARTESIAN_POINT('Ctrl Pts',(15.1847945994588,52.1434510802399,2.));
#64472=CARTESIAN_POINT('Ctrl Pts',(15.2038445286663,52.1586704870383,2.));
#64473=CARTESIAN_POINT('Ctrl Pts',(15.2225082026616,52.1743802571171,2.));
#64474=CARTESIAN_POINT('Ctrl Pts',(14.7622249872189,54.3610567043162,2.80658032638059));
#64475=CARTESIAN_POINT('Ctrl Pts',(14.8615128627433,54.3048362110035,2.79940525217632));
#64476=CARTESIAN_POINT('Ctrl Pts',(14.9530160801183,54.235599890915,2.79223017797206));
#64477=CARTESIAN_POINT('Ctrl Pts',(15.0325849243862,54.154635191266,2.7850551037678));
#64478=CARTESIAN_POINT('Ctrl Pts',(15.3227836759489,53.8593455590615,2.75888660030887));
#64479=CARTESIAN_POINT('Ctrl Pts',(15.4542357696669,53.4080493196853,2.73271809684994));
#64480=CARTESIAN_POINT('Ctrl Pts',(15.3680012509646,53.0031097267674,2.70654959339102));
#64481=CARTESIAN_POINT('Ctrl Pts',(15.2817667322623,52.5981701338495,2.68038108993209));
#64482=CARTESIAN_POINT('Ctrl Pts',(14.9778456011397,52.23958718739,2.65421258647316));
#64483=CARTESIAN_POINT('Ctrl Pts',(14.5925102242224,52.0881604517115,2.62804408301424));
#64484=CARTESIAN_POINT('Ctrl Pts',(14.2071748473051,51.9367337160331,2.60187557955531));
#64485=CARTESIAN_POINT('Ctrl Pts',(13.7404252245931,51.9924631911358,2.57570707609639));
#64486=CARTESIAN_POINT('Ctrl Pts',(13.4015764529908,52.2303456612731,2.54953857263746));
#64487=CARTESIAN_POINT('Ctrl Pts',(13.0627276813884,52.4682281314104,2.52337006917853));
#64488=CARTESIAN_POINT('Ctrl Pts',(12.8517797608958,52.8882635965824,2.49720156571961));
#64489=CARTESIAN_POINT('Ctrl Pts',(12.8632860991091,53.3021301533919,2.47103306226068));
#64490=CARTESIAN_POINT('Ctrl Pts',(12.8747924373225,53.7159967102013,2.44486455880175));
#64491=CARTESIAN_POINT('Ctrl Pts',(13.1087530342418,54.1236943586483,2.41869605534283));
#64492=CARTESIAN_POINT('Ctrl Pts',(13.4603337012234,54.3423524839877,2.3925275518839));
#64493=CARTESIAN_POINT('Ctrl Pts',(13.811914368205,54.5610106093271,2.36635904842497));
#64494=CARTESIAN_POINT('Ctrl Pts',(14.281115105249,54.5906292115589,2.34019054496605));
#64495=CARTESIAN_POINT('Ctrl Pts',(14.6573871465026,54.4180355738828,2.31402204150712));
#64496=CARTESIAN_POINT('Ctrl Pts',(14.6930548254675,54.4016750320804,2.31154146979828));
#64497=CARTESIAN_POINT('Ctrl Pts',(14.7278874868095,54.3834974973412,2.30906089808943));
#64498=CARTESIAN_POINT('Ctrl Pts',(14.7617771735939,54.3636459375188,2.30658032638059));
#64499=CARTESIAN_POINT('Ctrl Pts',(15.6194800884629,52.866705242183,2.));
#64500=CARTESIAN_POINT('Ctrl Pts',(15.7510836294753,53.3567463262429,2.02616850345893));
#64501=CARTESIAN_POINT('Ctrl Pts',(15.4911223508182,54.468705692608,2.07850551037678));
#64502=CARTESIAN_POINT('Ctrl Pts',(13.8755519245003,55.0671510173416,2.15701102075356));
#64503=CARTESIAN_POINT('Ctrl Pts',(12.4888977717378,54.0475500892828,2.23551653113034));
#64504=CARTESIAN_POINT('Ctrl Pts',(12.5727324025626,52.3295818538895,2.31402204150712));
#64505=CARTESIAN_POINT('Ctrl Pts',(14.0528383317196,51.4513683986094,2.3925275518839));
#64506=CARTESIAN_POINT('Ctrl Pts',(15.6013423678816,52.2018016959779,2.47103306226067));
#64507=CARTESIAN_POINT('Ctrl Pts',(15.8297478005623,53.907232954514,2.54953857263746));
#64508=CARTESIAN_POINT('Ctrl Pts',(14.5330963425821,55.0385110233129,2.62804408301424));
#64509=CARTESIAN_POINT('Ctrl Pts',(12.8743150895914,54.5809192738243,2.70654959339101));
#64510=CARTESIAN_POINT('Ctrl Pts',(12.3410089780029,52.9449163922479,2.78505510376779));
#64511=CARTESIAN_POINT('Ctrl Pts',(13.4114743235374,51.5976690199096,2.86356061414457));
#64512=CARTESIAN_POINT('Ctrl Pts',(15.125685020798,51.7474403844543,2.94206612452135));
#64513=CARTESIAN_POINT('Ctrl Pts',(15.9462998191018,53.2599021194416,3.02057163489813));
#64514=CARTESIAN_POINT('Ctrl Pts',(15.1373700363305,54.7786474915821,3.09907714527491));
#64515=CARTESIAN_POINT('Ctrl Pts',(13.4243640409751,54.9416270991707,3.17758265565169));
#64516=CARTESIAN_POINT('Ctrl Pts',(12.3435458814549,53.6026781745395,3.25608816602847));
#64517=CARTESIAN_POINT('Ctrl Pts',(12.8642192037884,51.9626013374103,3.33459367640525));
#64518=CARTESIAN_POINT('Ctrl Pts',(14.5194316817765,51.4922567887357,3.41309918678203));
#64519=CARTESIAN_POINT('Ctrl Pts',(15.824749470772,52.6134605506407,3.49160469715881));
#64520=CARTESIAN_POINT('Ctrl Pts',(15.6095325175198,54.3206905095792,3.57011020753559));
#64521=CARTESIAN_POINT('Ctrl Pts',(14.0667925161087,55.0828622138133,3.64861571791237));
#64522=CARTESIAN_POINT('Ctrl Pts',(12.5800953694062,54.216441978079,3.72712122828915));
#64523=CARTESIAN_POINT('Ctrl Pts',(12.482746426243,52.4984560584277,3.80562673866593));
#64524=CARTESIAN_POINT('Ctrl Pts',(13.8620505314459,51.4696350750293,3.88413224904271));
#64525=CARTESIAN_POINT('Ctrl Pts',(15.4810149732843,52.0526501422855,3.96263775941949));
#64526=CARTESIAN_POINT('Ctrl Pts',(15.8877139511439,53.7246394886753,4.04114326979626));
#64527=CARTESIAN_POINT('Ctrl Pts',(14.7174101533174,54.9861233184473,4.11964878017305));
#64528=CARTESIAN_POINT('Ctrl Pts',(13.0196598476916,54.705772943414,4.19815429054983));
#64529=CARTESIAN_POINT('Ctrl Pts',(12.317045870665,53.1350132444558,4.2766598009266));
#64530=CARTESIAN_POINT('Ctrl Pts',(13.239689139382,51.6825388628568,4.35516531130338));
#64531=CARTESIAN_POINT('Ctrl Pts',(14.9601412381249,51.6509633535716,4.43367082168016));
#64532=CARTESIAN_POINT('Ctrl Pts',(15.9354598188275,53.0686043860759,4.51217633205695));
#64533=CARTESIAN_POINT('Ctrl Pts',(15.2909560004752,54.6640877757789,4.59068184243372));
#64534=CARTESIAN_POINT('Ctrl Pts',(13.6046361114517,55.0065460966708,4.6691873528105));
#64535=CARTESIAN_POINT('Ctrl Pts',(12.3888319545388,53.7888545684046,4.74769286318728));
#64536=CARTESIAN_POINT('Ctrl Pts',(12.7339055288242,52.1030679359729,4.82619837356406));
#64537=CARTESIAN_POINT('Ctrl Pts',(14.3303867955418,51.461039661442,4.90470388394084));
#64538=CARTESIAN_POINT('Ctrl Pts',(15.7465131069793,52.4385560995514,4.98320939431762));
#64539=CARTESIAN_POINT('Ctrl Pts',(15.7122693095411,54.1589569990369,5.0617149046944));
#64540=CARTESIAN_POINT('Ctrl Pts',(14.2583648731494,55.079346475668,5.14022041507118));
#64541=CARTESIAN_POINT('Ctrl Pts',(12.6886982319545,54.374296277089,5.21872592544795));
#64542=CARTESIAN_POINT('Ctrl Pts',(12.4109789893207,52.6761143673659,5.29723143582474));
#64543=CARTESIAN_POINT('Ctrl Pts',(13.6742819091468,51.5077662723951,5.37573694620152));
#64544=CARTESIAN_POINT('Ctrl Pts',(15.3456277491901,51.9170631330653,5.4542424565783));
#64545=CARTESIAN_POINT('Ctrl Pts',(15.9261522494264,53.5369201511685,5.53274796695508));
#64546=CARTESIAN_POINT('Ctrl Pts',(14.895150144613,54.9146464419454,5.61125347733186));
#64547=CARTESIAN_POINT('Ctrl Pts',(13.1774033105245,54.8145932898247,5.68975898770864));
#64548=CARTESIAN_POINT('Ctrl Pts',(12.3131175991141,53.326633245717,5.76826449808541));
#64549=CARTESIAN_POINT('Ctrl Pts',(13.0780276880699,51.7849182946399,5.8467700084622));
#64550=CARTESIAN_POINT('Ctrl Pts',(14.7848942477639,51.5726692650909,5.92527551883897));
#64551=CARTESIAN_POINT('Ctrl Pts',(15.9054717137609,52.8790772926886,6.00378102921575));
#64552=CARTESIAN_POINT('Ctrl Pts',(15.4296884573085,54.5349259880616,6.08228653959253));
#64553=CARTESIAN_POINT('Ctrl Pts',(14.340318424872,54.8774262527002,6.13462354651039));
#64554=CARTESIAN_POINT('Ctrl Pts',(13.8417981729249,54.7828888819299,6.16079204996931));
#64555=CARTESIAN_POINT('Ctrl Pts',(15.5298235927831,52.8907830444123,1.94640265001023));
#64556=CARTESIAN_POINT('Ctrl Pts',(15.6535093143589,53.3513412073422,1.97257115346916));
#64557=CARTESIAN_POINT('Ctrl Pts',(15.4091883934694,54.3964004476471,2.02490816038701));
#64558=CARTESIAN_POINT('Ctrl Pts',(13.8908174408455,54.9588407987497,2.10341367076379));
#64559=CARTESIAN_POINT('Ctrl Pts',(12.5875902013567,54.0005833268291,2.18191918114057));
#64560=CARTESIAN_POINT('Ctrl Pts',(12.6663809901671,52.3859752455852,2.26042469151735));
#64561=CARTESIAN_POINT('Ctrl Pts',(14.0574375563363,51.5605987847521,2.33893020189413));
#64562=CARTESIAN_POINT('Ctrl Pts',(15.5127771133299,52.2658828763921,2.4174357122709));
#64563=CARTESIAN_POINT('Ctrl Pts',(15.7274407199138,53.8687082577405,2.49594122264769));
#64564=CARTESIAN_POINT('Ctrl Pts',(14.5088012366685,54.9319239065435,2.57444673302447));
#64565=CARTESIAN_POINT('Ctrl Pts',(12.9498192014263,54.5018627905034,2.65295224340124));
#64566=CARTESIAN_POINT('Ctrl Pts',(12.4485990159725,52.9642886845845,2.73145775377802));
#64567=CARTESIAN_POINT('Ctrl Pts',(13.4546606892816,51.6980973487976,2.8099632641548));
#64568=CARTESIAN_POINT('Ctrl Pts',(15.0657373016022,51.8388578416581,2.88846877453159));
#64569=CARTESIAN_POINT('Ctrl Pts',(15.8369804815592,53.2603235530564,2.96697428490836));
#64570=CARTESIAN_POINT('Ctrl Pts',(15.0767192977297,54.6876948517164,3.04547979528514));
#64571=CARTESIAN_POINT('Ctrl Pts',(13.4667749074092,54.8408689244782,3.12398530566192));
#64572=CARTESIAN_POINT('Ctrl Pts',(12.4509832887027,53.5824767670773,3.2024908160387));
#64573=CARTESIAN_POINT('Ctrl Pts',(12.9403307263376,52.0410738118106,3.28099632641548));
#64574=CARTESIAN_POINT('Ctrl Pts',(14.4959586990071,51.5990271583197,3.35950183679226));
#64575=CARTESIAN_POINT('Ctrl Pts',(15.7227431105484,52.6527746126658,3.43800734716904));
#64576=CARTESIAN_POINT('Ctrl Pts',(15.5204745093119,54.2572904770774,3.51651285754582));
#64577=CARTESIAN_POINT('Ctrl Pts',(14.0705521986317,54.9736067439323,3.5950183679226));
#64578=CARTESIAN_POINT('Ctrl Pts',(12.6733009701311,54.1593139732339,3.67352387829938));
#64579=CARTESIAN_POINT('Ctrl Pts',(12.5818089465338,52.5446892716908,3.75202938867616));
#64580=CARTESIAN_POINT('Ctrl Pts',(13.8781283480644,51.5777664615214,3.83053489905293));
#64581=CARTESIAN_POINT('Ctrl Pts',(15.3996891180402,52.1257049039707,3.90904040942972));
#64582=CARTESIAN_POINT('Ctrl Pts',(15.781919384443,53.6971003784726,3.98754591980649));
#64583=CARTESIAN_POINT('Ctrl Pts',(14.682025957689,54.8826880651051,4.06605143018328));
#64584=CARTESIAN_POINT('Ctrl Pts',(13.0864194109997,54.6192047411515,4.14455694056005));
#64585=CARTESIAN_POINT('Ctrl Pts',(12.4260776293936,53.142948515116,4.22306245093684));
#64586=CARTESIAN_POINT('Ctrl Pts',(13.2932108202671,51.7778610670395,4.30156796131361));
#64587=CARTESIAN_POINT('Ctrl Pts',(14.9101533252533,51.7481852724521,4.38007347169039));
#64588=CARTESIAN_POINT('Ctrl Pts',(15.8267926610378,53.0805350914,4.45857898206717));
#64589=CARTESIAN_POINT('Ctrl Pts',(15.2210648879244,54.5800275275423,4.53708449244395));
#64590=CARTESIAN_POINT('Ctrl Pts',(13.6362010561689,54.9018821235761,4.61559000282073));
#64591=CARTESIAN_POINT('Ctrl Pts',(12.4935447622286,53.7574520104367,4.69409551319751));
#64592=CARTESIAN_POINT('Ctrl Pts',(12.8178572670738,52.1730893523261,4.77260102357429));
#64593=CARTESIAN_POINT('Ctrl Pts',(14.3182875437761,51.5696881839643,4.85110653395107));
#64594=CARTESIAN_POINT('Ctrl Pts',(15.6492137736117,52.488393144862,4.92961204432785));
#64595=CARTESIAN_POINT('Ctrl Pts',(15.6170302262462,54.1052875309521,5.00811755470463));
#64596=CARTESIAN_POINT('Ctrl Pts',(14.2505987614542,54.9703025272977,5.08662306508142));
#64597=CARTESIAN_POINT('Ctrl Pts',(12.7753698302556,54.3076710974169,5.16512857545818));
#64598=CARTESIAN_POINT('Ctrl Pts',(12.5143593387719,52.7116589137379,5.24363408583497));
#64599=CARTESIAN_POINT('Ctrl Pts',(13.701656671393,51.6136035265765,5.32213959621175));
#64600=CARTESIAN_POINT('Ctrl Pts',(15.2724473555814,51.9982753762946,5.40064510658853));
#64601=CARTESIAN_POINT('Ctrl Pts',(15.8180450739392,53.5206750214142,5.4791506169653));
#64602=CARTESIAN_POINT('Ctrl Pts',(14.8490723677412,54.8155115364335,5.55765612734209));
#64603=CARTESIAN_POINT('Ctrl Pts',(13.2346723673735,54.7214780003996,5.63616163771886));
#64604=CARTESIAN_POINT('Ctrl Pts',(12.4223856990886,53.3230398556835,5.71466714809565));
#64605=CARTESIAN_POINT('Ctrl Pts',(13.1412755979873,51.8740809240221,5.79317265847242));
#64606=CARTESIAN_POINT('Ctrl Pts',(14.7454499267729,51.674601683786,5.8716781688492));
#64607=CARTESIAN_POINT('Ctrl Pts',(15.7986087657921,52.9024107406156,5.95018367922598));
#64608=CARTESIAN_POINT('Ctrl Pts',(15.3514506199299,54.4586366531711,6.02868918960276));
#64609=CARTESIAN_POINT('Ctrl Pts',(14.3276216447485,54.7805306694404,6.08102619652062));
#64610=CARTESIAN_POINT('Ctrl Pts',(13.8590944561341,54.691681062282,6.10719469997954));
#64611=CARTESIAN_POINT('Ctrl Pts',(15.4401670971033,52.9148608466415,1.89280530002046));
#64612=CARTESIAN_POINT('Ctrl Pts',(15.5559349992425,53.3459360884415,1.91897380347939));
#64613=CARTESIAN_POINT('Ctrl Pts',(15.3272544361205,54.3240952026862,1.97131081039724));
#64614=CARTESIAN_POINT('Ctrl Pts',(13.9060829571906,54.8505305801576,2.04981632077402));
#64615=CARTESIAN_POINT('Ctrl Pts',(12.6862826309757,53.9536165643755,2.1283218311508));
#64616=CARTESIAN_POINT('Ctrl Pts',(12.7600295777716,52.4423686372807,2.20682734152758));
#64617=CARTESIAN_POINT('Ctrl Pts',(14.0620367809532,51.6698291708949,2.28533285190436));
#64618=CARTESIAN_POINT('Ctrl Pts',(15.4242118587781,52.3299640568063,2.36383836228113));
#64619=CARTESIAN_POINT('Ctrl Pts',(15.6251336392654,53.8301835609669,2.44234387265791));
#64620=CARTESIAN_POINT('Ctrl Pts',(14.4845061307549,54.8253367897741,2.5208493830347));
#64621=CARTESIAN_POINT('Ctrl Pts',(13.0253233132612,54.4228063071824,2.59935489341147));
#64622=CARTESIAN_POINT('Ctrl Pts',(12.5561890539421,52.9836609769212,2.67786040378825));
#64623=CARTESIAN_POINT('Ctrl Pts',(13.4978470550258,51.7985256776855,2.75636591416503));
#64624=CARTESIAN_POINT('Ctrl Pts',(15.0057895824064,51.9302752988621,2.83487142454181));
#64625=CARTESIAN_POINT('Ctrl Pts',(15.7276611440166,53.2607449866712,2.91337693491859));
#64626=CARTESIAN_POINT('Ctrl Pts',(15.016068559129,54.5967422118507,2.99188244529537));
#64627=CARTESIAN_POINT('Ctrl Pts',(13.5091857738433,54.7401107497857,3.07038795567215));
#64628=CARTESIAN_POINT('Ctrl Pts',(12.5584206959504,53.5622753596153,3.14889346604893));
#64629=CARTESIAN_POINT('Ctrl Pts',(13.0164422488867,52.1195462862108,3.22739897642571));
#64630=CARTESIAN_POINT('Ctrl Pts',(14.4724857162377,51.7057975279038,3.30590448680249));
#64631=CARTESIAN_POINT('Ctrl Pts',(15.6207367503249,52.6920886746908,3.38440999717927));
#64632=CARTESIAN_POINT('Ctrl Pts',(15.4314165011041,54.1938904445757,3.46291550755605));
#64633=CARTESIAN_POINT('Ctrl Pts',(14.0743118811546,54.8643512740511,3.54142101793283));
#64634=CARTESIAN_POINT('Ctrl Pts',(12.7665065708559,54.1021859683889,3.61992652830961));
#64635=CARTESIAN_POINT('Ctrl Pts',(12.6808714668247,52.590922484954,3.69843203868639));
#64636=CARTESIAN_POINT('Ctrl Pts',(13.894206164683,51.6858978480135,3.77693754906317));
#64637=CARTESIAN_POINT('Ctrl Pts',(15.3183632627962,52.1987596656559,3.85544305943995));
#64638=CARTESIAN_POINT('Ctrl Pts',(15.6761248177421,53.6695612682698,3.93394856981672));
#64639=CARTESIAN_POINT('Ctrl Pts',(14.6466417620606,54.7792528117632,4.01245408019351));
#64640=CARTESIAN_POINT('Ctrl Pts',(13.1531789743077,54.5326365388889,4.09095959057028));
#64641=CARTESIAN_POINT('Ctrl Pts',(12.5351093881223,53.1508837857763,4.16946510094706));
#64642=CARTESIAN_POINT('Ctrl Pts',(13.3467325011522,51.8731832712222,4.24797061132384));
#64643=CARTESIAN_POINT('Ctrl Pts',(14.8601654123817,51.8454071913326,4.32647612170062));
#64644=CARTESIAN_POINT('Ctrl Pts',(15.7181255032481,53.0924657967241,4.40498163207741));
#64645=CARTESIAN_POINT('Ctrl Pts',(15.1511737753737,54.4959672793057,4.48348714245418));
#64646=CARTESIAN_POINT('Ctrl Pts',(13.6677660008861,54.7972181504814,4.56199265283096));
#64647=CARTESIAN_POINT('Ctrl Pts',(12.5982575699184,53.7260494524688,4.64049816320774));
#64648=CARTESIAN_POINT('Ctrl Pts',(12.9018090053235,52.2431107686793,4.71900367358452));
#64649=CARTESIAN_POINT('Ctrl Pts',(14.3061882920104,51.6783367064865,4.7975091839613));
#64650=CARTESIAN_POINT('Ctrl Pts',(15.5519144402441,52.5382301901725,4.87601469433808));
#64651=CARTESIAN_POINT('Ctrl Pts',(15.5217911429513,54.0516180628673,4.95452020471485));
#64652=CARTESIAN_POINT('Ctrl Pts',(14.242832649759,54.8612585789273,5.03302571509164));
#64653=CARTESIAN_POINT('Ctrl Pts',(12.8620414285566,54.2410459177449,5.11153122546842));
#64654=CARTESIAN_POINT('Ctrl Pts',(12.617739688223,52.7472034601098,5.19003673584519));
#64655=CARTESIAN_POINT('Ctrl Pts',(13.7290314336392,51.7194407807578,5.26854224622198));
#64656=CARTESIAN_POINT('Ctrl Pts',(15.1992669619728,52.079487619524,5.34704775659876));
#64657=CARTESIAN_POINT('Ctrl Pts',(15.709937898452,53.5044298916597,5.42555326697553));
#64658=CARTESIAN_POINT('Ctrl Pts',(14.8029945908694,54.7163766309217,5.50405877735232));
#64659=CARTESIAN_POINT('Ctrl Pts',(13.2919414242225,54.6283627109744,5.5825642877291));
#64660=CARTESIAN_POINT('Ctrl Pts',(12.531653799063,53.3194464656501,5.66106979810587));
#64661=CARTESIAN_POINT('Ctrl Pts',(13.2045235079047,51.9632435534043,5.73957530848265));
#64662=CARTESIAN_POINT('Ctrl Pts',(14.706005605782,51.7765341024811,5.81808081885944));
#64663=CARTESIAN_POINT('Ctrl Pts',(15.6917458178233,52.9257441885424,5.89658632923621));
#64664=CARTESIAN_POINT('Ctrl Pts',(15.2732127825514,54.3823473182807,5.975091839613));
#64665=CARTESIAN_POINT('Ctrl Pts',(14.314924864625,54.6836350861806,6.02742884653084));
#64666=CARTESIAN_POINT('Ctrl Pts',(13.8763907393433,54.6004732426341,6.05359734998977));
#64667=CARTESIAN_POINT('Ctrl Pts',(15.3505106014235,52.9389386488708,1.83920795003069));
#64668=CARTESIAN_POINT('Ctrl Pts',(15.4583606841261,53.3405309695408,1.86537645348962));
#64669=CARTESIAN_POINT('Ctrl Pts',(15.2453204787717,54.2517899577253,1.91771346040747));
#64670=CARTESIAN_POINT('Ctrl Pts',(13.9213484735358,54.7422203615657,1.99621897078425));
#64671=CARTESIAN_POINT('Ctrl Pts',(12.7849750605946,53.9066498019219,2.07472448116103));
#64672=CARTESIAN_POINT('Ctrl Pts',(12.8536781653762,52.4987620289764,2.15322999153781));
#64673=CARTESIAN_POINT('Ctrl Pts',(14.0666360055699,51.7790595570376,2.23173550191458));
#64674=CARTESIAN_POINT('Ctrl Pts',(15.3356466042264,52.3940452372206,2.31024101229137));
#64675=CARTESIAN_POINT('Ctrl Pts',(15.522826558617,53.7916588641933,2.38874652266814));
#64676=CARTESIAN_POINT('Ctrl Pts',(14.4602110248413,54.7187496730049,2.46725203304493));
#64677=CARTESIAN_POINT('Ctrl Pts',(13.1008274250962,54.3437498238614,2.5457575434217));
#64678=CARTESIAN_POINT('Ctrl Pts',(12.6637790919117,53.0030332692579,2.62426305379848));
#64679=CARTESIAN_POINT('Ctrl Pts',(13.54103342077,51.8989540065735,2.70276856417526));
#64680=CARTESIAN_POINT('Ctrl Pts',(14.9458418632107,52.021692756066,2.78127407455204));
#64681=CARTESIAN_POINT('Ctrl Pts',(15.618341806474,53.2611664202859,2.85977958492882));
#64682=CARTESIAN_POINT('Ctrl Pts',(14.9554178205282,54.505789571985,2.9382850953056));
#64683=CARTESIAN_POINT('Ctrl Pts',(13.5515966402774,54.6393525750931,3.01679060568238));
#64684=CARTESIAN_POINT('Ctrl Pts',(12.6658581031982,53.5420739521532,3.09529611605916));
#64685=CARTESIAN_POINT('Ctrl Pts',(13.0925537714358,52.1980187606109,3.17380162643594));
#64686=CARTESIAN_POINT('Ctrl Pts',(14.4490127334682,51.8125678974878,3.25230713681272));
#64687=CARTESIAN_POINT('Ctrl Pts',(15.5187303901013,52.7314027367158,3.3308126471895));
#64688=CARTESIAN_POINT('Ctrl Pts',(15.3423584928962,54.130490412074,3.40931815756628));
#64689=CARTESIAN_POINT('Ctrl Pts',(14.0780715636776,54.75509580417,3.48782366794306));
#64690=CARTESIAN_POINT('Ctrl Pts',(12.8597121715808,54.0450579635439,3.56632917831984));
#64691=CARTESIAN_POINT('Ctrl Pts',(12.7799339871155,52.6371556982171,3.64483468869662));
#64692=CARTESIAN_POINT('Ctrl Pts',(13.9102839813016,51.7940292345055,3.7233401990734));
#64693=CARTESIAN_POINT('Ctrl Pts',(15.2370374075522,52.2718144273411,3.80184570945018));
#64694=CARTESIAN_POINT('Ctrl Pts',(15.5703302510412,53.642022158067,3.88035121982695));
#64695=CARTESIAN_POINT('Ctrl Pts',(14.6112575664322,54.6758175584211,3.95885673020374));
#64696=CARTESIAN_POINT('Ctrl Pts',(13.2199385376158,54.4460683366263,4.03736224058051));
#64697=CARTESIAN_POINT('Ctrl Pts',(12.6441411468509,53.1588190564366,4.11586775095729));
#64698=CARTESIAN_POINT('Ctrl Pts',(13.4002541820373,51.9685054754049,4.19437326133407));
#64699=CARTESIAN_POINT('Ctrl Pts',(14.81017749951,51.942629110213,4.27287877171085));
#64700=CARTESIAN_POINT('Ctrl Pts',(15.6094583454585,53.1043965020482,4.35138428208763));
#64701=CARTESIAN_POINT('Ctrl Pts',(15.081282662823,54.4119070310692,4.42988979246441));
#64702=CARTESIAN_POINT('Ctrl Pts',(13.6993309456032,54.6925541773866,4.50839530284119));
#64703=CARTESIAN_POINT('Ctrl Pts',(12.7029703776082,53.6946468945009,4.58690081321797));
#64704=CARTESIAN_POINT('Ctrl Pts',(12.9857607435731,52.3131321850324,4.66540632359475));
#64705=CARTESIAN_POINT('Ctrl Pts',(14.2940890402447,51.7869852290089,4.74391183397153));
#64706=CARTESIAN_POINT('Ctrl Pts',(15.4546151068764,52.5880672354829,4.82241734434831));
#64707=CARTESIAN_POINT('Ctrl Pts',(15.4265520596564,53.9979485947826,4.90092285472509));
#64708=CARTESIAN_POINT('Ctrl Pts',(14.2350665380638,54.752214630557,4.97942836510187));
#64709=CARTESIAN_POINT('Ctrl Pts',(12.9487130268577,54.1744207380728,5.05793387547865));
#64710=CARTESIAN_POINT('Ctrl Pts',(12.7211200376741,52.7827480064819,5.13643938585542));
#64711=CARTESIAN_POINT('Ctrl Pts',(13.7564061958854,51.8252780349391,5.21494489623221));
#64712=CARTESIAN_POINT('Ctrl Pts',(15.1260865683642,52.1606998627533,5.29345040660899));
#64713=CARTESIAN_POINT('Ctrl Pts',(15.6018307229648,53.4881847619054,5.37195591698577));
#64714=CARTESIAN_POINT('Ctrl Pts',(14.7569168139975,54.6172417254098,5.45046142736255));
#64715=CARTESIAN_POINT('Ctrl Pts',(13.3492104810715,54.5352474215493,5.52896693773932));
#64716=CARTESIAN_POINT('Ctrl Pts',(12.6409218990375,53.3158530756166,5.60747244811611));
#64717=CARTESIAN_POINT('Ctrl Pts',(13.2677714178221,52.0524061827865,5.68597795849288));
#64718=CARTESIAN_POINT('Ctrl Pts',(14.666561284791,51.8784665211761,5.76448346886967));
#64719=CARTESIAN_POINT('Ctrl Pts',(15.5848828698546,52.9490776364694,5.84298897924644));
#64720=CARTESIAN_POINT('Ctrl Pts',(15.1949749451728,54.3060579833902,5.92149448962322));
#64721=CARTESIAN_POINT('Ctrl Pts',(14.3022280845014,54.5867395029208,5.97383149654107));
#64722=CARTESIAN_POINT('Ctrl Pts',(13.8936870225526,54.5092654229862,6.));
#64723=CARTESIAN_POINT('Ctrl Pts',(14.7602610286104,54.3618122024717,2.44341967361941));
#64724=CARTESIAN_POINT('Ctrl Pts',(14.651278048058,54.4258677305587,2.45136379342792));
#64725=CARTESIAN_POINT('Ctrl Pts',(14.5332929975391,54.473801003601,2.45930791323642));
#64726=CARTESIAN_POINT('Ctrl Pts',(14.4107496805131,54.5017345633457,2.46725203304492));
#64727=CARTESIAN_POINT('Ctrl Pts',(14.0070831582596,54.5937497232904,2.49342053650385));
#64728=CARTESIAN_POINT('Ctrl Pts',(13.5539552916779,54.4687497735759,2.51958903996277));
#64729=CARTESIAN_POINT('Ctrl Pts',(13.2545499695229,54.182797039618,2.5457575434217));
#64730=CARTESIAN_POINT('Ctrl Pts',(12.955144647368,53.8968443056602,2.57192604688063));
#64731=CARTESIAN_POINT('Ctrl Pts',(12.8094618696398,53.449938787459,2.59809455033955));
#64732=CARTESIAN_POINT('Ctrl Pts',(12.8828295355855,53.0424728179111,2.62426305379848));
#64733=CARTESIAN_POINT('Ctrl Pts',(12.9561972015311,52.6350068483631,2.65043155725741));
#64734=CARTESIAN_POINT('Ctrl Pts',(13.2486153111506,52.2669804274683,2.67660006071633));
#64735=CARTESIAN_POINT('Ctrl Pts',(13.6289591063671,52.1034236752696,2.70276856417526));
#64736=CARTESIAN_POINT('Ctrl Pts',(14.0093029015836,51.939866923071,2.72893706763419));
#64737=CARTESIAN_POINT('Ctrl Pts',(14.4775723823971,51.9807798395685,2.75510557109311));
#64738=CARTESIAN_POINT('Ctrl Pts',(14.8237904466811,52.2078152418539,2.78127407455204));
#64739=CARTESIAN_POINT('Ctrl Pts',(15.1700085109651,52.4348506441393,2.80744257801097));
#64740=CARTESIAN_POINT('Ctrl Pts',(15.3941751587195,52.8480085322126,2.83361108146989));
#64741=CARTESIAN_POINT('Ctrl Pts',(15.3957711516058,53.2620246681991,2.85977958492882));
#64742=CARTESIAN_POINT('Ctrl Pts',(15.397367144492,53.6760408041856,2.88594808838775));
#64743=CARTESIAN_POINT('Ctrl Pts',(15.1763924825101,54.0909151880853,2.91211659184667));
#64744=CARTESIAN_POINT('Ctrl Pts',(14.8319349548107,54.3206128805532,2.9382850953056));
#64745=CARTESIAN_POINT('Ctrl Pts',(14.8094060374994,54.3356360398807,2.9399966214102));
#64746=CARTESIAN_POINT('Ctrl Pts',(14.7863488988009,54.3498670707759,2.94170814751481));
#64747=CARTESIAN_POINT('Ctrl Pts',(14.7628222445741,54.3633003878638,2.94341967361941));
#64748=CARTESIAN_POINT('Ctrl Pts',(15.6194800884629,52.866705242183,2.));
#64749=CARTESIAN_POINT('Ctrl Pts',(15.6300231873965,52.926941249885,2.));
#64750=CARTESIAN_POINT('Ctrl Pts',(15.6366567833015,52.987630087735,2.));
#64751=CARTESIAN_POINT('Ctrl Pts',(15.6395415323775,53.0484503647743,2.));
#64752=CARTESIAN_POINT('Ctrl Pts',(15.6424094897195,53.1089166152119,2.));
#64753=CARTESIAN_POINT('Ctrl Pts',(15.6415715704011,53.1695138895016,2.));
#64754=CARTESIAN_POINT('Ctrl Pts',(15.6371309452724,53.2299210873137,2.));
#64755=CARTESIAN_POINT('Ctrl Pts',(15.6337777267599,53.275535956418,2.));
#64756=CARTESIAN_POINT('Ctrl Pts',(15.628369049543,53.3210424392735,2.));
#64757=CARTESIAN_POINT('Ctrl Pts',(15.6209312260544,53.3662945441232,2.));
#64758=CARTESIAN_POINT('Ctrl Pts',(15.6170700144012,53.3897863565923,2.));
#64759=CARTESIAN_POINT('Ctrl Pts',(15.6126617095029,53.4132094747523,2.));
#64760=CARTESIAN_POINT('Ctrl Pts',(15.6077085063715,53.4365423663732,2.));
#64761=CARTESIAN_POINT('Ctrl Pts',(15.6050999838077,53.4488302481048,2.));
#64762=CARTESIAN_POINT('Ctrl Pts',(15.6023397247443,53.4610950218001,2.));
#64763=CARTESIAN_POINT('Ctrl Pts',(15.5994335441749,53.4733116341268,2.));
#64764=CARTESIAN_POINT('Ctrl Pts',(15.5857322512059,53.5309072929574,2.));
#64765=CARTESIAN_POINT('Ctrl Pts',(15.5687698297175,53.5875426491662,2.));
#64766=CARTESIAN_POINT('Ctrl Pts',(15.5486498653391,53.6429179274572,2.));
#64767=CARTESIAN_POINT('Ctrl Pts',(15.5289409667744,53.6971618476902,2.));
#64768=CARTESIAN_POINT('Ctrl Pts',(15.5062016386482,53.7501975064157,2.));
#64769=CARTESIAN_POINT('Ctrl Pts',(15.4804878124203,53.8017173360065,2.));
#64770=CARTESIAN_POINT('Ctrl Pts',(15.4618733917387,53.8390129050498,2.));
#64771=CARTESIAN_POINT('Ctrl Pts',(15.4416993411855,53.8755136264573,2.));
#64772=CARTESIAN_POINT('Ctrl Pts',(15.4199753876479,53.9110903776723,2.));
#64773=CARTESIAN_POINT('Ctrl Pts',(15.4086212485451,53.9296847546774,2.));
#64774=CARTESIAN_POINT('Ctrl Pts',(15.3968435749493,53.9480265377065,2.));
#64775=CARTESIAN_POINT('Ctrl Pts',(15.3846428359354,53.9660958743824,2.));
#64776=CARTESIAN_POINT('Ctrl Pts',(15.3789686731488,53.9744993290933,2.));
#64777=CARTESIAN_POINT('Ctrl Pts',(15.373205772738,53.9828396302133,2.));
#64778=CARTESIAN_POINT('Ctrl Pts',(15.3673591187829,53.9911085225651,2.));
#64779=CARTESIAN_POINT('Ctrl Pts',(15.3351612285484,54.0366458316568,2.));
#64780=CARTESIAN_POINT('Ctrl Pts',(15.3003846167745,54.0800821194656,2.));
#64781=CARTESIAN_POINT('Ctrl Pts',(15.2630875305729,54.1211378587784,2.));
#64782=CARTESIAN_POINT('Ctrl Pts',(15.238131587418,54.1486087633668,2.));
#64783=CARTESIAN_POINT('Ctrl Pts',(15.2120464130742,54.1750132365563,2.));
#64784=CARTESIAN_POINT('Ctrl Pts',(15.1848412564379,54.2002572946035,2.));
#64785=CARTESIAN_POINT('Ctrl Pts',(15.1445758545731,54.237620142962,2.));
#64786=CARTESIAN_POINT('Ctrl Pts',(15.1018570560095,54.2724429083027,2.));
#64787=CARTESIAN_POINT('Ctrl Pts',(15.0569812349608,54.3046174971127,2.));
#64788=CARTESIAN_POINT('Ctrl Pts',(15.0431218621612,54.3145542427938,2.));
#64789=CARTESIAN_POINT('Ctrl Pts',(15.0290566706299,54.324238085577,2.));
#64790=CARTESIAN_POINT('Ctrl Pts',(15.0147942526811,54.3336649770073,2.));
#64791=CARTESIAN_POINT('Ctrl Pts',(15.0022772711783,54.341938204316,2.));
#64792=CARTESIAN_POINT('Ctrl Pts',(14.9896026925807,54.3500168035479,2.));
#64793=CARTESIAN_POINT('Ctrl Pts',(14.9768072444527,54.3578794016111,2.));
#64794=CARTESIAN_POINT('Ctrl Pts',(14.9293632591135,54.3870329711855,2.));
#64795=CARTESIAN_POINT('Ctrl Pts',(14.8801986446945,54.413264340731,2.));
#64796=CARTESIAN_POINT('Ctrl Pts',(14.8296406251874,54.4365044915685,2.));
#64797=CARTESIAN_POINT('Ctrl Pts',(14.7791435079019,54.4597166473058,2.));
#64798=CARTESIAN_POINT('Ctrl Pts',(14.7272551246491,54.4799449628023,2.));
#64799=CARTESIAN_POINT('Ctrl Pts',(14.6742902116473,54.4970704070682,2.));
#64800=CARTESIAN_POINT('Ctrl Pts',(14.6404359644482,54.5080166918955,2.));
#64801=CARTESIAN_POINT('Ctrl Pts',(14.6061417257392,54.5176942656993,2.));
#64802=CARTESIAN_POINT('Ctrl Pts',(14.571490685664,54.5260607579884,2.));
#64803=CARTESIAN_POINT('Ctrl Pts',(14.5536361910167,54.530371725032,2.));
#64804=CARTESIAN_POINT('Ctrl Pts',(14.5356869955305,54.5343344557618,2.));
#64805=CARTESIAN_POINT('Ctrl Pts',(14.5176547593681,54.5379422095229,2.));
#64806=CARTESIAN_POINT('Ctrl Pts',(14.5067786943717,54.5401182105492,2.));
#64807=CARTESIAN_POINT('Ctrl Pts',(14.4958730433768,54.5421648311648,2.));
#64808=CARTESIAN_POINT('Ctrl Pts',(14.4849536044948,54.5440785381581,2.));
#64809=CARTESIAN_POINT('Ctrl Pts',(14.432148545745,54.5533329889869,2.));
#64810=CARTESIAN_POINT('Ctrl Pts',(14.3789399495959,54.5594997842103,2.));
#64811=CARTESIAN_POINT('Ctrl Pts',(14.3256201373498,54.5624573557269,2.));
#64812=CARTESIAN_POINT('Ctrl Pts',(14.2921372783298,54.5643146006412,2.));
#64813=CARTESIAN_POINT('Ctrl Pts',(14.2586106300373,54.5649053533655,2.));
#64814=CARTESIAN_POINT('Ctrl Pts',(14.225115486905,54.5641893509564,2.));
#64815=CARTESIAN_POINT('Ctrl Pts',(14.212869318331,54.5639275731169,2.));
#64816=CARTESIAN_POINT('Ctrl Pts',(14.2006248769065,54.5634909095329,2.));
#64817=CARTESIAN_POINT('Ctrl Pts',(14.1883942978659,54.562877565257,2.));
#64818=CARTESIAN_POINT('Ctrl Pts',(14.1370506808453,54.5603027637289,2.));
#64819=CARTESIAN_POINT('Ctrl Pts',(14.0860310640551,54.5546235246645,2.));
#64820=CARTESIAN_POINT('Ctrl Pts',(14.0356066352152,54.5457116917125,2.));
#64821=CARTESIAN_POINT('Ctrl Pts',(14.0074349171617,54.5407327231642,2.));
#64822=CARTESIAN_POINT('Ctrl Pts',(13.9794492439462,54.5347439009404,2.));
#64823=CARTESIAN_POINT('Ctrl Pts',(13.9516999296066,54.5277163783411,2.));
#64824=CARTESIAN_POINT('Ctrl Pts',(13.932212693117,54.5227812295604,2.));
#64825=CARTESIAN_POINT('Ctrl Pts',(13.9128420740716,54.517333696643,2.));
#64826=CARTESIAN_POINT('Ctrl Pts',(13.8936031194075,54.5113848919291,2.));
#64827=CARTESIAN_POINT('Origin',(14.1292828945603,53.2669068454841,4.5));
#64828=CARTESIAN_POINT('Origin',(39.0658530619283,-38.8697713466883,7.));
#64829=CARTESIAN_POINT('',(39.0658530619283,-38.8697713466882,7.));
#64830=CARTESIAN_POINT('Origin',(39.0658530619283,-38.8697713466883,7.));
#64831=CARTESIAN_POINT('',(39.0658530619283,-38.8697713466882,7.));
#64832=CARTESIAN_POINT('Origin',(-14.1292828945604,-53.2669068454841,7.));
#64833=CARTESIAN_POINT('',(-14.1292828945603,-53.2669068454841,7.));
#64834=CARTESIAN_POINT('Origin',(-14.1292828945604,-53.2669068454841,7.));
#64835=CARTESIAN_POINT('',(-14.1292828945603,-53.2669068454841,7.));
#64836=CARTESIAN_POINT('Origin',(-53.1951359564886,-14.3971354987959,7.));
#64837=CARTESIAN_POINT('',(-53.1951359564886,-14.3971354987959,7.));
#64838=CARTESIAN_POINT('Origin',(-53.1951359564886,-14.3971354987959,7.));
#64839=CARTESIAN_POINT('',(-53.1951359564886,-14.3971354987959,7.));
#64840=CARTESIAN_POINT('Origin',(-39.0658530619283,38.8697713466882,7.));
#64841=CARTESIAN_POINT('',(-39.0658530619283,38.8697713466882,7.));
#64842=CARTESIAN_POINT('Origin',(-39.0658530619283,38.8697713466882,7.));
#64843=CARTESIAN_POINT('',(-39.0658530619283,38.8697713466882,7.));
#64844=CARTESIAN_POINT('Origin',(14.1292828945603,53.2669068454841,7.));
#64845=CARTESIAN_POINT('',(14.1292828945603,53.2669068454841,7.));
#64846=CARTESIAN_POINT('Origin',(14.1292828945603,53.2669068454841,7.));
#64847=CARTESIAN_POINT('',(14.1292828945603,53.2669068454841,7.));
#64848=CARTESIAN_POINT('Origin',(39.0658530619283,-38.8697713466883,14.));
#64849=CARTESIAN_POINT('Ctrl Pts',(39.3014489339361,-37.6274127691862,14.));
#64850=CARTESIAN_POINT('Ctrl Pts',(39.2527755161121,-37.6125702664346,14.));
#64851=CARTESIAN_POINT('Ctrl Pts',(39.2032917181168,-37.6009462766898,14.));
#64852=CARTESIAN_POINT('Ctrl Pts',(39.1532758042432,-37.5923965983573,14.));
#64853=CARTESIAN_POINT('Ctrl Pts',(39.11957228402,-37.5866353469022,14.));
#64854=CARTESIAN_POINT('Ctrl Pts',(39.0856264423049,-37.5822710037892,14.));
#64855=CARTESIAN_POINT('Ctrl Pts',(39.0515175292276,-37.5792707431897,14.));
#64856=CARTESIAN_POINT('Ctrl Pts',(39.0357879604487,-37.5778871515945,14.));
#64857=CARTESIAN_POINT('Ctrl Pts',(39.020023659971,-37.5767937802474,14.));
#64858=CARTESIAN_POINT('Ctrl Pts',(39.0042321835127,-37.5759880571028,14.));
#64859=CARTESIAN_POINT('Ctrl Pts',(38.9909279654484,-37.5753092404992,14.));
#64860=CARTESIAN_POINT('Ctrl Pts',(38.9776118489143,-37.5748350538309,14.));
#64861=CARTESIAN_POINT('Ctrl Pts',(38.964295763777,-37.5745634329246,14.));
#64862=CARTESIAN_POINT('Ctrl Pts',(38.9105541147734,-37.5734672131832,14.));
#64863=CARTESIAN_POINT('Ctrl Pts',(38.8567779423384,-37.5756644894702,14.));
#64864=CARTESIAN_POINT('Ctrl Pts',(38.8032675464005,-37.581026481916,14.));
#64865=CARTESIAN_POINT('Ctrl Pts',(38.7827897374601,-37.5830784543397,14.));
#64866=CARTESIAN_POINT('Ctrl Pts',(38.7623506706579,-37.5855944285777,14.));
#64867=CARTESIAN_POINT('Ctrl Pts',(38.741966693386,-37.5885691376506,14.));
#64868=CARTESIAN_POINT('Ctrl Pts',(38.7273323755428,-37.5907047776921,14.));
#64869=CARTESIAN_POINT('Ctrl Pts',(38.7127264476943,-37.5930768844319,14.));
#64870=CARTESIAN_POINT('Ctrl Pts',(38.6981549324168,-37.5956838482276,14.));
#64871=CARTESIAN_POINT('Ctrl Pts',(38.6868487314646,-37.5977066204644,14.));
#64872=CARTESIAN_POINT('Ctrl Pts',(38.6755628687237,-37.5998709906565,14.));
#64873=CARTESIAN_POINT('Ctrl Pts',(38.6643154441843,-37.6021728300854,14.));
#64874=CARTESIAN_POINT('Ctrl Pts',(38.6087986246104,-37.6135346137375,14.));
#64875=CARTESIAN_POINT('Ctrl Pts',(38.5541290481433,-37.6282564371478,14.));
#64876=CARTESIAN_POINT('Ctrl Pts',(38.5006370918184,-37.646191772746,14.));
#64877=CARTESIAN_POINT('Ctrl Pts',(38.4479217174824,-37.6638667279142,14.));
#64878=CARTESIAN_POINT('Ctrl Pts',(38.396348804881,-37.6846628180258,14.));
#64879=CARTESIAN_POINT('Ctrl Pts',(38.3462305040151,-37.7084927625726,14.));
#64880=CARTESIAN_POINT('Ctrl Pts',(38.3200575603805,-37.7209373144561,14.));
#64881=CARTESIAN_POINT('Ctrl Pts',(38.2942813568713,-37.7342101082399,14.));
#64882=CARTESIAN_POINT('Ctrl Pts',(38.2689475825533,-37.7483042482809,14.));
#64883=CARTESIAN_POINT('Ctrl Pts',(38.2553600451045,-37.7558635109953,14.));
#64884=CARTESIAN_POINT('Ctrl Pts',(38.2418997994627,-37.7636591075236,14.));
#64885=CARTESIAN_POINT('Ctrl Pts',(38.2285740909778,-37.7716904151908,14.));
#64886=CARTESIAN_POINT('Ctrl Pts',(38.2191033712726,-37.7773983491343,14.));
#64887=CARTESIAN_POINT('Ctrl Pts',(38.2097006104897,-37.7832253493693,14.));
#64888=CARTESIAN_POINT('Ctrl Pts',(38.2003684633688,-37.7891712859343,14.));
#64889=CARTESIAN_POINT('Ctrl Pts',(38.1921418096808,-37.7944128622123,14.));
#64890=CARTESIAN_POINT('Ctrl Pts',(38.1839782827807,-37.799741616598,14.));
#64891=CARTESIAN_POINT('Ctrl Pts',(38.1758800165188,-37.805156517765,14.));
#64892=CARTESIAN_POINT('Ctrl Pts',(38.1358534009022,-37.8319202917141,14.));
#64893=CARTESIAN_POINT('Ctrl Pts',(38.0974162938763,-37.8607893617484,14.));
#64894=CARTESIAN_POINT('Ctrl Pts',(38.0607602397062,-37.8916978987796,14.));
#64895=CARTESIAN_POINT('Ctrl Pts',(38.0190399864289,-37.9268765895189,14.));
#64896=CARTESIAN_POINT('Ctrl Pts',(37.9796253872743,-37.9646960620489,14.));
#64897=CARTESIAN_POINT('Ctrl Pts',(37.9425628056484,-38.0048405338641,14.));
#64898=CARTESIAN_POINT('Ctrl Pts',(37.9063354033645,-38.0440803780985,14.));
#64899=CARTESIAN_POINT('Ctrl Pts',(37.8723549080301,-38.0855424637378,14.));
#64900=CARTESIAN_POINT('Ctrl Pts',(37.840690574833,-38.128969359293,14.));
#64901=CARTESIAN_POINT('Ctrl Pts',(37.8329319648795,-38.1396101121555,14.));
#64902=CARTESIAN_POINT('Ctrl Pts',(37.8253125495561,-38.150368975123,14.));
#64903=CARTESIAN_POINT('Ctrl Pts',(37.8178336250567,-38.1612424270076,14.));
#64904=CARTESIAN_POINT('Ctrl Pts',(37.8121884193454,-38.1694498735041,14.));
#64905=CARTESIAN_POINT('Ctrl Pts',(37.8066244559601,-38.1777210085551,14.));
#64906=CARTESIAN_POINT('Ctrl Pts',(37.8011483696327,-38.1860445283744,14.));
#64907=CARTESIAN_POINT('Ctrl Pts',(37.7694817125934,-38.234177087235,14.));
#64908=CARTESIAN_POINT('Ctrl Pts',(37.740690869399,-38.2841447569426,14.));
#64909=CARTESIAN_POINT('Ctrl Pts',(37.714822629006,-38.3355979876329,14.));
#64910=CARTESIAN_POINT('Ctrl Pts',(37.688399760224,-38.3881544020733,14.));
#64911=CARTESIAN_POINT('Ctrl Pts',(37.6650255379469,-38.4422615831566,14.));
#64912=CARTESIAN_POINT('Ctrl Pts',(37.6447852836523,-38.497588492234,14.));
#64913=CARTESIAN_POINT('Ctrl Pts',(37.6243676757527,-38.5534001989154,14.));
#64914=CARTESIAN_POINT('Ctrl Pts',(37.6071385772686,-38.6104541129556,14.));
#64915=CARTESIAN_POINT('Ctrl Pts',(37.5932306356489,-38.6684381301182,14.));
#64916=CARTESIAN_POINT('Ctrl Pts',(37.5900811837451,-38.6815686046512,14.));
#64917=CARTESIAN_POINT('Ctrl Pts',(37.5871015926663,-38.6947505762787,14.));
#64918=CARTESIAN_POINT('Ctrl Pts',(37.5842989888732,-38.7079539606268,14.));
#64919=CARTESIAN_POINT('Ctrl Pts',(37.5716672473774,-38.7674635275383,14.));
#64920=CARTESIAN_POINT('Ctrl Pts',(37.5626014399524,-38.8275056873519,14.));
#64921=CARTESIAN_POINT('Ctrl Pts',(37.5571792782293,-38.8877281078776,14.));
#64922=CARTESIAN_POINT('Ctrl Pts',(37.5518047857275,-38.9474210798112,14.));
#64923=CARTESIAN_POINT('Ctrl Pts',(37.5500097107535,-39.0072922465006,14.));
#64924=CARTESIAN_POINT('Ctrl Pts',(37.55191466572,-39.0670207918836,14.));
#64925=CARTESIAN_POINT('Ctrl Pts',(37.5533104035149,-39.1107831850594,14.));
#64926=CARTESIAN_POINT('Ctrl Pts',(37.5566933253821,-39.1544695447415,14.));
#64927=CARTESIAN_POINT('Ctrl Pts',(37.5621285378972,-39.1979562890069,14.));
#64928=CARTESIAN_POINT('Ctrl Pts',(37.565149248657,-39.2221247784535,14.));
#64929=CARTESIAN_POINT('Ctrl Pts',(37.5688041553789,-39.2462316220403,14.));
#64930=CARTESIAN_POINT('Ctrl Pts',(37.5730796542559,-39.2702614469549,14.));
#64931=CARTESIAN_POINT('Ctrl Pts',(37.9741697098829,-39.9602191716056,14.));
#64932=CARTESIAN_POINT('Ctrl Pts',(38.020991576866,-39.9994070905167,14.));
#64933=CARTESIAN_POINT('Ctrl Pts',(38.0702141503049,-40.0354948198824,14.));
#64934=CARTESIAN_POINT('Ctrl Pts',(38.1214910131339,-40.0684345608226,14.));
#64935=CARTESIAN_POINT('Ctrl Pts',(38.1690376391703,-40.0989780351658,14.));
#64936=CARTESIAN_POINT('Ctrl Pts',(38.2183516107569,-40.1268144785211,14.));
#64937=CARTESIAN_POINT('Ctrl Pts',(38.269168974583,-40.1518670892131,14.));
#64938=CARTESIAN_POINT('Ctrl Pts',(38.2814354208216,-40.1579143628033,14.));
#64939=CARTESIAN_POINT('Ctrl Pts',(38.2937899478069,-40.1637993357403,14.));
#64940=CARTESIAN_POINT('Ctrl Pts',(38.3062147884412,-40.1695145314963,14.));
#64941=CARTESIAN_POINT('Ctrl Pts',(38.3608949816838,-40.1946664040676,14.));
#64942=CARTESIAN_POINT('Ctrl Pts',(38.4170009394504,-40.2165668551763,14.));
#64943=CARTESIAN_POINT('Ctrl Pts',(38.4742056409767,-40.2351397541773,14.));
#64944=CARTESIAN_POINT('Ctrl Pts',(38.5095144293503,-40.2466036119165,14.));
#64945=CARTESIAN_POINT('Ctrl Pts',(38.5452420718463,-40.2567987360604,14.));
#64946=CARTESIAN_POINT('Ctrl Pts',(38.5813118928663,-40.2656972878978,14.));
#64947=CARTESIAN_POINT('Ctrl Pts',(38.5936535320381,-40.2687420137329,14.));
#64948=CARTESIAN_POINT('Ctrl Pts',(38.606035223169,-40.2716348792846,14.));
#64949=CARTESIAN_POINT('Ctrl Pts',(38.6184538586389,-40.2743745611435,14.));
#64950=CARTESIAN_POINT('Ctrl Pts',(38.6300726309494,-40.2769377847601,14.));
#64951=CARTESIAN_POINT('Ctrl Pts',(38.6417163481208,-40.2793652420776,14.));
#64952=CARTESIAN_POINT('Ctrl Pts',(38.6533764439016,-40.2816552664683,14.));
#64953=CARTESIAN_POINT('Ctrl Pts',(38.7110876105802,-40.2929896484314,14.));
#64954=CARTESIAN_POINT('Ctrl Pts',(38.7692463793663,-40.3009718362976,14.));
#64955=CARTESIAN_POINT('Ctrl Pts',(38.8275464696014,-40.3055302032883,14.));
#64956=CARTESIAN_POINT('Ctrl Pts',(38.884358538419,-40.3099722248722,14.));
#64957=CARTESIAN_POINT('Ctrl Pts',(38.9413057829595,-40.3111628333597,14.));
#64958=CARTESIAN_POINT('Ctrl Pts',(38.9980976135487,-40.3089871593233,14.));
#64959=CARTESIAN_POINT('Ctrl Pts',(39.0288884010392,-40.3078075756365,14.));
#64960=CARTESIAN_POINT('Ctrl Pts',(39.0596332939681,-40.3056376455304,14.));
#64961=CARTESIAN_POINT('Ctrl Pts',(39.0902835748068,-40.3024530490142,14.));
#64962=CARTESIAN_POINT('Ctrl Pts',(39.1157839679843,-40.2998035312594,14.));
#64963=CARTESIAN_POINT('Ctrl Pts',(39.1412188509075,-40.2964515980885,14.));
#64964=CARTESIAN_POINT('Ctrl Pts',(39.1665588545923,-40.2923809784595,14.));
#64965=CARTESIAN_POINT('Ctrl Pts',(39.177388964653,-40.2906412289651,14.));
#64966=CARTESIAN_POINT('Ctrl Pts',(39.1882029800145,-40.2887698277109,14.));
#64967=CARTESIAN_POINT('Ctrl Pts',(39.1989810533142,-40.2867689791834,14.));
#64968=CARTESIAN_POINT('Ctrl Pts',(39.2488808956908,-40.2775055400359,14.));
#64969=CARTESIAN_POINT('Ctrl Pts',(39.2980978217139,-40.2654572977741,14.));
#64970=CARTESIAN_POINT('Ctrl Pts',(39.3464249159924,-40.2505519130058,14.));
#64971=CARTESIAN_POINT('Ctrl Pts',(39.4004290144141,-40.2338955864035,14.));
#64972=CARTESIAN_POINT('Ctrl Pts',(39.453323106219,-40.213671565055,14.));
#64973=CARTESIAN_POINT('Ctrl Pts',(39.5048609693631,-40.1901258318535,14.));
#64974=CARTESIAN_POINT('Ctrl Pts',(39.5485960623522,-40.1701448941847,14.));
#64975=CARTESIAN_POINT('Ctrl Pts',(39.5913543500861,-40.1477707447876,14.));
#64976=CARTESIAN_POINT('Ctrl Pts',(39.6329645160386,-40.1231328973124,14.));
#64977=CARTESIAN_POINT('Ctrl Pts',(39.6444045721053,-40.1163591113871,14.));
#64978=CARTESIAN_POINT('Ctrl Pts',(39.6557577122762,-40.109414126601,14.));
#64979=CARTESIAN_POINT('Ctrl Pts',(39.6670200627834,-40.1023004514028,14.));
#64980=CARTESIAN_POINT('Ctrl Pts',(39.6757877124576,-40.0967625122316,14.));
#64981=CARTESIAN_POINT('Ctrl Pts',(39.6845017797731,-40.0911212766431,14.));
#64982=CARTESIAN_POINT('Ctrl Pts',(39.6931464328262,-40.0853874573566,14.));
#64983=CARTESIAN_POINT('Ctrl Pts',(39.7394049739124,-40.0547051253513,14.));
#64984=CARTESIAN_POINT('Ctrl Pts',(39.7837665094937,-40.0213210070133,14.));
#64985=CARTESIAN_POINT('Ctrl Pts',(39.8260058213226,-39.9854744939929,14.));
#64986=CARTESIAN_POINT('Ctrl Pts',(39.8680089351017,-39.9498284311244,14.));
#64987=CARTESIAN_POINT('Ctrl Pts',(39.9079141963546,-39.9117464670036,14.));
#64988=CARTESIAN_POINT('Ctrl Pts',(39.9454594213871,-39.871433353871,14.));
#64989=CARTESIAN_POINT('Ctrl Pts',(39.9802942732058,-39.8340304265716,14.));
#64990=CARTESIAN_POINT('Ctrl Pts',(40.0130975716486,-39.7947059892306,14.));
#64991=CARTESIAN_POINT('Ctrl Pts',(40.0436204335297,-39.7536104031421,14.));
#64992=CARTESIAN_POINT('Ctrl Pts',(40.0514607527674,-39.7430542988211,14.));
#64993=CARTESIAN_POINT('Ctrl Pts',(40.059152868768,-39.7323774869518,14.));
#64994=CARTESIAN_POINT('Ctrl Pts',(40.0666759532076,-39.7216063497953,14.));
#64995=CARTESIAN_POINT('Ctrl Pts',(40.0970859623337,-39.6780669768348,14.));
#64996=CARTESIAN_POINT('Ctrl Pts',(40.1247894553757,-39.6329220142745,14.));
#64997=CARTESIAN_POINT('Ctrl Pts',(40.1495562730571,-39.5863640526291,14.));
#64998=CARTESIAN_POINT('Ctrl Pts',(40.1734835191653,-39.54138436162,14.));
#64999=CARTESIAN_POINT('Ctrl Pts',(40.1946700927784,-39.4950850230299,14.));
#65000=CARTESIAN_POINT('Ctrl Pts',(40.2128622006869,-39.4476279812285,14.));
#65001=CARTESIAN_POINT('Ctrl Pts',(40.2255879517124,-39.4144308112573,14.));
#65002=CARTESIAN_POINT('Ctrl Pts',(40.2368474822756,-39.3806668978155,14.));
#65003=CARTESIAN_POINT('Ctrl Pts',(40.2465386396389,-39.3463911596944,14.));
#65004=CARTESIAN_POINT('Ctrl Pts',(40.2520057165832,-39.327055172195,14.));
#65005=CARTESIAN_POINT('Ctrl Pts',(40.2569733939395,-39.3075562909784,14.));
#65006=CARTESIAN_POINT('Ctrl Pts',(40.261442519219,-39.2879130030575,14.));
#65007=CARTESIAN_POINT('Origin',(39.0658530619283,-38.8697713466883,19.1042117235887));
#65008=CARTESIAN_POINT('Ctrl Pts',(38.2940537528419,-37.5314721085808,17.8542117235887));
#65009=CARTESIAN_POINT('Ctrl Pts',(38.3354082297679,-37.5072482534306,17.8517311518799));
#65010=CARTESIAN_POINT('Ctrl Pts',(38.8263155408625,-37.2510699656701,17.8230820767121));
#65011=CARTESIAN_POINT('Ctrl Pts',(40.0256568276714,-37.3267811177079,17.7682644980854));
#65012=CARTESIAN_POINT('Ctrl Pts',(40.8821443104935,-38.8192615374441,17.6897589877086));
#65013=CARTESIAN_POINT('Ctrl Pts',(40.1099071502118,-40.3569109628883,17.6112534773319));
#65014=CARTESIAN_POINT('Ctrl Pts',(38.4012543668155,-40.5609220251472,17.5327479669551));
#65015=CARTESIAN_POINT('Ctrl Pts',(37.2886704652103,-39.2482374965453,17.4542424565783));
#65016=CARTESIAN_POINT('Ctrl Pts',(37.6534618751482,-37.995852754822,17.3947303754562));
#65017=CARTESIAN_POINT('Ctrl Pts',(38.1723477780672,-37.603235418619,17.361386797793));
#65018=CARTESIAN_POINT('Ctrl Pts',(38.2935040424574,-37.5346322273253,17.3542117235887));
#65019=CARTESIAN_POINT('Ctrl Pts',(38.2938718037176,-37.5356881270256,17.8957882764113));
#65020=CARTESIAN_POINT('Ctrl Pts',(38.5911486295276,-37.3667504425096,17.8781885106897));
#65021=CARTESIAN_POINT('Ctrl Pts',(39.4708982524073,-37.1808200198998,17.8344202415091));
#65022=CARTESIAN_POINT('Ctrl Pts',(40.7062722211716,-38.0891100356719,17.7644834688697));
#65023=CARTESIAN_POINT('Ctrl Pts',(40.6223994863181,-39.8071108514352,17.6859779584929));
#65024=CARTESIAN_POINT('Ctrl Pts',(39.1423049297703,-40.6853144575312,17.6074724481161));
#65025=CARTESIAN_POINT('Ctrl Pts',(37.593781529679,-39.9348860603428,17.5289669377393));
#65026=CARTESIAN_POINT('Ctrl Pts',(37.3884926508269,-38.402016881723,17.458405547171));
#65027=CARTESIAN_POINT('Ctrl Pts',(37.9908199438394,-37.7130239262802,17.4140126600617));
#65028=CARTESIAN_POINT('Ctrl Pts',(38.2959007276492,-37.5337106753506,17.3957882764113));
#65029=CARTESIAN_POINT('Ctrl Pts',(40.2595650866584,-39.2869186252539,18.));
#65030=CARTESIAN_POINT('Ctrl Pts',(40.1223890770422,-39.679462603358,17.9738314965411));
#65031=CARTESIAN_POINT('Ctrl Pts',(39.4328412785483,-40.3122408191566,17.9214944896232));
#65032=CARTESIAN_POINT('Ctrl Pts',(38.0628399617007,-39.9714590750956,17.8429889792464));
#65033=CARTESIAN_POINT('Ctrl Pts',(37.5947572398929,-38.6408443652932,17.7644834688697));
#65034=CARTESIAN_POINT('Ctrl Pts',(38.4448300096771,-37.5164220658531,17.6859779584929));
#65035=CARTESIAN_POINT('Ctrl Pts',(39.8524194013853,-37.6052793541117,17.6074724481161));
#65036=CARTESIAN_POINT('Ctrl Pts',(40.5543172769709,-38.8283781815623,17.5289669377393));
#65037=CARTESIAN_POINT('Ctrl Pts',(39.9214631686259,-40.0884933458361,17.4504614273625));
#65038=CARTESIAN_POINT('Ctrl Pts',(38.5212094780202,-40.2556819318544,17.3719559169858));
#65039=CARTESIAN_POINT('Ctrl Pts',(37.6094386785518,-39.1799271772095,17.293450406609));
#65040=CARTESIAN_POINT('Ctrl Pts',(38.0037983665503,-37.8260300114723,17.2149448962322));
#65041=CARTESIAN_POINT('Ctrl Pts',(39.350642117465,-37.4081786211339,17.1364393858554));
#65042=CARTESIAN_POINT('Ctrl Pts',(40.4420762478648,-38.3011214248007,17.0579338754787));
#65043=CARTESIAN_POINT('Ctrl Pts',(40.2992826919135,-39.7040414735315,16.9794283651019));
#65044=CARTESIAN_POINT('Ctrl Pts',(39.0503191421164,-40.358768990196,16.9009228547251));
#65045=CARTESIAN_POINT('Ctrl Pts',(37.8152872634063,-39.6781276508141,16.8224173443483));
#65046=CARTESIAN_POINT('Ctrl Pts',(37.7017922854028,-38.2725333429822,16.7439118339715));
#65047=CARTESIAN_POINT('Ctrl Pts',(38.8116195577816,-37.4025561853298,16.6654063235948));
#65048=CARTESIAN_POINT('Ctrl Pts',(40.1494494228946,-37.8484125098358,16.586900813218));
#65049=CARTESIAN_POINT('Ctrl Pts',(40.5154843389836,-39.2102476987511,16.5083953028412));
#65050=CARTESIAN_POINT('Ctrl Pts',(39.5814554487361,-40.2667356115709,16.4298897924644));
#65051=CARTESIAN_POINT('Ctrl Pts',(38.1850220871887,-40.0703927553964,16.3513842820876));
#65052=CARTESIAN_POINT('Ctrl Pts',(37.5785388809249,-38.7973040793768,16.2728787717108));
#65053=CARTESIAN_POINT('Ctrl Pts',(38.3059143927449,-37.5892057701993,16.1943732613341));
#65054=CARTESIAN_POINT('Ctrl Pts',(39.7148209687577,-37.5295491143576,16.1158677509573));
#65055=CARTESIAN_POINT('Ctrl Pts',(40.5417176980217,-38.6718356181182,16.0373622405805));
#65056=CARTESIAN_POINT('Ctrl Pts',(40.0450239347318,-39.9916355890619,15.9588567302037));
#65057=CARTESIAN_POINT('Ctrl Pts',(38.6701864544171,-40.3053210365855,15.880351219827));
#65058=CARTESIAN_POINT('Ctrl Pts',(37.6501921939814,-39.3315713939809,15.8018457094502));
#65059=CARTESIAN_POINT('Ctrl Pts',(37.8997962556048,-37.9436684903302,15.7233401990734));
#65060=CARTESIAN_POINT('Ctrl Pts',(39.195147782035,-37.3863166449999,15.6448346886966));
#65061=CARTESIAN_POINT('Ctrl Pts',(40.3745447306992,-38.1593622434704,15.5663291783198));
#65062=CARTESIAN_POINT('Ctrl Pts',(40.3802758763629,-39.5695196142836,15.4878236679431));
#65063=CARTESIAN_POINT('Ctrl Pts',(39.2072013976485,-40.3521261040356,15.4093181575663));
#65064=CARTESIAN_POINT('Ctrl Pts',(37.9073623625386,-39.8053216046427,15.3308126471895));
#65065=CARTESIAN_POINT('Ctrl Pts',(37.6464853455349,-38.4194933961106,15.2523071368127));
#65066=CARTESIAN_POINT('Ctrl Pts',(38.6585310049342,-37.4374851510426,15.173801626436));
#65067=CARTESIAN_POINT('Ctrl Pts',(40.0358728399512,-37.7399852318106,15.0952961160591));
#65068=CARTESIAN_POINT('Ctrl Pts',(40.5432777323755,-39.0557043292571,15.0167906056824));
#65069=CARTESIAN_POINT('Ctrl Pts',(39.7256933501734,-40.2046743690254,14.9382850953056));
#65070=CARTESIAN_POINT('Ctrl Pts',(38.3163479152336,-40.1564715183471,14.8597795849288));
#65071=CARTESIAN_POINT('Ctrl Pts',(37.5791777219181,-38.954325616703,14.781274074552));
#65072=CARTESIAN_POINT('Ctrl Pts',(38.1752908680604,-37.676348923403,14.7027685641753));
#65073=CARTESIAN_POINT('Ctrl Pts',(39.5700863286924,-37.4686628699809,14.6242630537985));
#65074=CARTESIAN_POINT('Ctrl Pts',(40.5126633343826,-38.5175221013622,14.5457575434217));
#65075=CARTESIAN_POINT('Ctrl Pts',(40.1577269226072,-39.8822911025123,14.4672520330449));
#65076=CARTESIAN_POINT('Ctrl Pts',(38.8235306389232,-40.3389996506625,14.3887465226681));
#65077=CARTESIAN_POINT('Ctrl Pts',(37.7067389013686,-39.4780868997918,14.3102410122914));
#65078=CARTESIAN_POINT('Ctrl Pts',(37.8086626184681,-38.0715866597083,14.2317355019146));
#65079=CARTESIAN_POINT('Ctrl Pts',(39.0384102949243,-37.3809896965113,14.1532299915378));
#65080=CARTESIAN_POINT('Ctrl Pts',(40.2920679536969,-38.0254209930877,14.074724481161));
#65081=CARTESIAN_POINT('Ctrl Pts',(40.4474545117342,-39.4273810345935,13.9962189707842));
#65082=CARTESIAN_POINT('Ctrl Pts',(39.3608457503204,-40.3286674512605,13.9177134604075));
#65083=CARTESIAN_POINT('Ctrl Pts',(38.4650745289098,-40.0575985380862,13.8653764534896));
#65084=CARTESIAN_POINT('Ctrl Pts',(38.1712104185962,-39.7634014663305,13.8392079500307));
#65085=CARTESIAN_POINT('Ctrl Pts',(40.3472015171019,-39.3175435144276,18.0535973499898));
#65086=CARTESIAN_POINT('Ctrl Pts',(40.1999547235979,-39.7389061291211,18.0274288465308));
#65087=CARTESIAN_POINT('Ctrl Pts',(39.4597837375779,-40.4181397905768,17.975091839613));
#65088=CARTESIAN_POINT('Ctrl Pts',(37.9892037027278,-40.0523395370335,17.8965863292362));
#65089=CARTESIAN_POINT('Ctrl Pts',(37.4867566635289,-38.6240376790355,17.8180808188594));
#65090=CARTESIAN_POINT('Ctrl Pts',(38.3992375699639,-37.4170658579415,17.7395753084827));
#65091=CARTESIAN_POINT('Ctrl Pts',(39.9101652101474,-37.5124466086438,17.6610697981059));
#65092=CARTESIAN_POINT('Ctrl Pts',(40.6635929548117,-38.8253393001895,17.5825642877291));
#65093=CARTESIAN_POINT('Ctrl Pts',(39.9842778291545,-40.1779658848535,17.5040587773523));
#65094=CARTESIAN_POINT('Ctrl Pts',(38.481224440952,-40.3574286296186,17.4255532669755));
#65095=CARTESIAN_POINT('Ctrl Pts',(37.5025159407713,-39.2026972836548,17.3470477565988));
#65096=CARTESIAN_POINT('Ctrl Pts',(37.9258275657957,-37.7494036870074,17.268542246222));
#65097=CARTESIAN_POINT('Ctrl Pts',(39.3715499208041,-37.3008757150928,17.1900367358452));
#65098=CARTESIAN_POINT('Ctrl Pts',(40.5431117447103,-38.2593739611798,17.1115312254684));
#65099=CARTESIAN_POINT('Ctrl Pts',(40.3898349924146,-39.7652894583281,17.0330257150916));
#65100=CARTESIAN_POINT('Ctrl Pts',(39.0491787185847,-40.4680838297154,16.9545202047148));
#65101=CARTESIAN_POINT('Ctrl Pts',(37.7234769101999,-39.7374731709667,16.8760146943381));
#65102=CARTESIAN_POINT('Ctrl Pts',(37.6016496924775,-38.2286870838463,16.7975091839613));
#65103=CARTESIAN_POINT('Ctrl Pts',(38.7929549918386,-37.2948405078714,16.7190036735845));
#65104=CARTESIAN_POINT('Ctrl Pts',(40.22900170615,-37.7734293976536,16.6404981632077));
#65105=CARTESIAN_POINT('Ctrl Pts',(40.6219090946604,-39.2352437878639,16.561992652831));
#65106=CARTESIAN_POINT('Ctrl Pts',(39.6193084248072,-40.3692938158071,16.4834871424542));
#65107=CARTESIAN_POINT('Ctrl Pts',(38.1203558353197,-40.1585364386243,16.4049816320774));
#65108=CARTESIAN_POINT('Ctrl Pts',(37.469347632893,-38.7919838911743,16.3264761217006));
#65109=CARTESIAN_POINT('Ctrl Pts',(38.2501234557823,-37.4951929817316,16.2479706113238));
#65110=CARTESIAN_POINT('Ctrl Pts',(39.7624649814247,-37.4311566293954,16.1694651009471));
#65111=CARTESIAN_POINT('Ctrl Pts',(40.650068377118,-38.6573041563001,16.0909595905703));
#65112=CARTESIAN_POINT('Ctrl Pts',(40.116909815337,-40.0739973108231,16.0124540801935));
#65113=CARTESIAN_POINT('Ctrl Pts',(38.6411385698271,-40.4107119918079,15.9339485698167));
#65114=CARTESIAN_POINT('Ctrl Pts',(37.5462613776579,-39.3654744684955,15.8554430594399));
#65115=CARTESIAN_POINT('Ctrl Pts',(37.8141901344604,-37.8756786009153,15.7769375490632));
#65116=CARTESIAN_POINT('Ctrl Pts',(39.2046399606431,-37.2774087408428,15.6984320386864));
#65117=CARTESIAN_POINT('Ctrl Pts',(40.4706223976961,-38.1072075221718,15.6199265283096));
#65118=CARTESIAN_POINT('Ctrl Pts',(40.4767742957171,-39.6208916697799,15.5414210179328));
#65119=CARTESIAN_POINT('Ctrl Pts',(39.2175784930743,-40.4609532557217,15.462915507556));
#65120=CARTESIAN_POINT('Ctrl Pts',(37.8223117075287,-39.8740050755378,15.3844099971793));
#65121=CARTESIAN_POINT('Ctrl Pts',(37.5422823907398,-38.3864362169263,15.3059044868025));
#65122=CARTESIAN_POINT('Ctrl Pts',(38.6286274349137,-37.3323337854206,15.2273989764257));
#65123=CARTESIAN_POINT('Ctrl Pts',(40.1070868924566,-37.6570419253671,15.1488934660489));
#65124=CARTESIAN_POINT('Ctrl Pts',(40.6517429414752,-39.0693546088525,15.0703879556722));
#65125=CARTESIAN_POINT('Ctrl Pts',(39.774135559288,-40.302676343909,14.9918824452954));
#65126=CARTESIAN_POINT('Ctrl Pts',(38.2613229558678,-40.2509346784385,14.9133769349186));
#65127=CARTESIAN_POINT('Ctrl Pts',(37.4700333744308,-38.9605331728383,14.8348714245418));
#65128=CARTESIAN_POINT('Ctrl Pts',(38.1099101982325,-37.5887337540646,14.756365914165));
#65129=CARTESIAN_POINT('Ctrl Pts',(39.6071046402236,-37.3658004182179,14.6778604037883));
#65130=CARTESIAN_POINT('Ctrl Pts',(40.6188809858598,-38.4916617046775,14.5993548934115));
#65131=CARTESIAN_POINT('Ctrl Pts',(40.2378868989348,-39.9566252931007,14.5208493830347));
#65132=CARTESIAN_POINT('Ctrl Pts',(38.8057405256223,-40.4468631230908,14.4423438726579));
#65133=CARTESIAN_POINT('Ctrl Pts',(37.6069594645119,-39.5227464177935,14.3638383622811));
#65134=CARTESIAN_POINT('Ctrl Pts',(37.7163659166087,-38.0129878893579,14.2853328519043));
#65135=CARTESIAN_POINT('Ctrl Pts',(39.0363955827559,-37.2716907141535,14.2068273415276));
#65136=CARTESIAN_POINT('Ctrl Pts',(40.3820905838163,-37.9634329679189,14.1283218311508));
#65137=CARTESIAN_POINT('Ctrl Pts',(40.5488848541016,-39.4683179788618,14.049816320774));
#65138=CARTESIAN_POINT('Ctrl Pts',(39.3825026538969,-40.4357723847318,13.9713108103972));
#65139=CARTESIAN_POINT('Ctrl Pts',(38.4209683416301,-40.1448029331842,13.9189738034794));
#65140=CARTESIAN_POINT('Ctrl Pts',(38.1055301823584,-39.8290073680889,13.8928053000205));
#65141=CARTESIAN_POINT('Ctrl Pts',(40.4348379475454,-39.3481684036013,18.1071946999795));
#65142=CARTESIAN_POINT('Ctrl Pts',(40.2775203701536,-39.7983496548843,18.0810261965206));
#65143=CARTESIAN_POINT('Ctrl Pts',(39.4867261966074,-40.5240387619969,18.0286891896027));
#65144=CARTESIAN_POINT('Ctrl Pts',(37.915567443755,-40.1332199989714,17.950183679226));
#65145=CARTESIAN_POINT('Ctrl Pts',(37.378756087165,-38.6072309927778,17.8716781688492));
#65146=CARTESIAN_POINT('Ctrl Pts',(38.3536451302507,-37.3177096500299,17.7931726584724));
#65147=CARTESIAN_POINT('Ctrl Pts',(39.9679110189094,-37.4196138631759,17.7146671480956));
#65148=CARTESIAN_POINT('Ctrl Pts',(40.7728686326526,-38.8223004188168,17.6361616377189));
#65149=CARTESIAN_POINT('Ctrl Pts',(40.0470924896831,-40.2674384238709,17.5576561273421));
#65150=CARTESIAN_POINT('Ctrl Pts',(38.4412394038838,-40.459175327383,17.4791506169653));
#65151=CARTESIAN_POINT('Ctrl Pts',(37.3955932029908,-39.2254673901001,17.4006451065885));
#65152=CARTESIAN_POINT('Ctrl Pts',(37.8478567650411,-37.6727773625425,17.3221395962118));
#65153=CARTESIAN_POINT('Ctrl Pts',(39.3924577241432,-37.1935728090517,17.243634085835));
#65154=CARTESIAN_POINT('Ctrl Pts',(40.6441472415558,-38.2176264975589,17.1651285754582));
#65155=CARTESIAN_POINT('Ctrl Pts',(40.4803872929157,-39.8265374431247,17.0866230650814));
#65156=CARTESIAN_POINT('Ctrl Pts',(39.048038295053,-40.5773986692348,17.0081175547046));
#65157=CARTESIAN_POINT('Ctrl Pts',(37.6316665569935,-39.7968186911193,16.9296120443279));
#65158=CARTESIAN_POINT('Ctrl Pts',(37.5015070995521,-38.1848408247104,16.8511065339511));
#65159=CARTESIAN_POINT('Ctrl Pts',(38.7742904258956,-37.187124830413,16.7726010235743));
#65160=CARTESIAN_POINT('Ctrl Pts',(40.3085539894053,-37.6984462854713,16.6940955131975));
#65161=CARTESIAN_POINT('Ctrl Pts',(40.7283338503372,-39.2602398769767,16.6155900028207));
#65162=CARTESIAN_POINT('Ctrl Pts',(39.6571614008785,-40.4718520200432,16.5370844924439));
#65163=CARTESIAN_POINT('Ctrl Pts',(38.0556895834507,-40.2466801218523,16.4585789820672));
#65164=CARTESIAN_POINT('Ctrl Pts',(37.360156384861,-38.7866637029718,16.3800734716904));
#65165=CARTESIAN_POINT('Ctrl Pts',(38.1943325188197,-37.4011801932639,16.3015679613136));
#65166=CARTESIAN_POINT('Ctrl Pts',(39.8101089940916,-37.3327641444332,16.2230624509368));
#65167=CARTESIAN_POINT('Ctrl Pts',(40.7584190562143,-38.6427726944821,16.1445569405601));
#65168=CARTESIAN_POINT('Ctrl Pts',(40.1887956959422,-40.1563590325843,16.0660514301833));
#65169=CARTESIAN_POINT('Ctrl Pts',(38.6120906852372,-40.5161029470303,15.9875459198065));
#65170=CARTESIAN_POINT('Ctrl Pts',(37.4423305613344,-39.3993775430101,15.9090404094297));
#65171=CARTESIAN_POINT('Ctrl Pts',(37.728584013316,-37.8076887115003,15.830534899053));
#65172=CARTESIAN_POINT('Ctrl Pts',(39.2141321392512,-37.1685008366856,15.7520293886761));
#65173=CARTESIAN_POINT('Ctrl Pts',(40.566700064693,-38.0550528008733,15.6735238782994));
#65174=CARTESIAN_POINT('Ctrl Pts',(40.5732727150713,-39.6722637252762,15.5950183679226));
#65175=CARTESIAN_POINT('Ctrl Pts',(39.2279555885002,-40.5697804074078,15.5165128575458));
#65176=CARTESIAN_POINT('Ctrl Pts',(37.7372610525188,-39.9426885464328,15.4380073471691));
#65177=CARTESIAN_POINT('Ctrl Pts',(37.4380794359446,-38.3533790377419,15.3595018367922));
#65178=CARTESIAN_POINT('Ctrl Pts',(38.5987238648931,-37.2271824197985,15.2809963264155));
#65179=CARTESIAN_POINT('Ctrl Pts',(40.1783009449621,-37.5740986189236,15.2024908160387));
#65180=CARTESIAN_POINT('Ctrl Pts',(40.7602081505748,-39.083004888448,15.1239853056619));
#65181=CARTESIAN_POINT('Ctrl Pts',(39.8225777684026,-40.4006783187926,15.0454797952851));
#65182=CARTESIAN_POINT('Ctrl Pts',(38.2062979965018,-40.34539783853,14.9669742849084));
#65183=CARTESIAN_POINT('Ctrl Pts',(37.3608890269436,-38.9667407289735,14.8884687745316));
#65184=CARTESIAN_POINT('Ctrl Pts',(38.0445295284046,-37.5011185847263,14.8099632641548));
#65185=CARTESIAN_POINT('Ctrl Pts',(39.6441229517549,-37.2629379664549,14.731457753778));
#65186=CARTESIAN_POINT('Ctrl Pts',(40.7250986373369,-38.4658013079928,14.6529522434012));
#65187=CARTESIAN_POINT('Ctrl Pts',(40.3180468752625,-40.030959483689,14.5744467330245));
#65188=CARTESIAN_POINT('Ctrl Pts',(38.7879504123214,-40.554726595519,14.4959412226477));
#65189=CARTESIAN_POINT('Ctrl Pts',(37.5071800276552,-39.5674059357952,14.4174357122709));
#65190=CARTESIAN_POINT('Ctrl Pts',(37.6240692147493,-37.9543891190076,14.3389302018941));
#65191=CARTESIAN_POINT('Ctrl Pts',(39.0343808705876,-37.1623917317957,14.2604246915173));
#65192=CARTESIAN_POINT('Ctrl Pts',(40.4721132139355,-37.9014449427502,14.1819191811406));
#65193=CARTESIAN_POINT('Ctrl Pts',(40.6503151964691,-39.50925492313,14.1034136707638));
#65194=CARTESIAN_POINT('Ctrl Pts',(39.4041595574733,-40.5428773182031,14.024908160387));
#65195=CARTESIAN_POINT('Ctrl Pts',(38.3768621543504,-40.2320073282822,13.9725711534692));
#65196=CARTESIAN_POINT('Ctrl Pts',(38.0398499461206,-39.8946132698472,13.9464026500102));
#65197=CARTESIAN_POINT('Ctrl Pts',(40.5224743779889,-39.378793292775,18.1607920499693));
#65198=CARTESIAN_POINT('Ctrl Pts',(40.3550860167094,-39.8577931806474,18.1346235465104));
#65199=CARTESIAN_POINT('Ctrl Pts',(39.513668655637,-40.6299377334171,18.0822865395925));
#65200=CARTESIAN_POINT('Ctrl Pts',(37.8419311847822,-40.2141004609093,18.0037810292158));
#65201=CARTESIAN_POINT('Ctrl Pts',(37.2707555108009,-38.59042430652,17.925275518839));
#65202=CARTESIAN_POINT('Ctrl Pts',(38.3080526905375,-37.2183534421184,17.8467700084622));
#65203=CARTESIAN_POINT('Ctrl Pts',(40.0256568276714,-37.3267811177079,17.7682644980854));
#65204=CARTESIAN_POINT('Ctrl Pts',(40.8821443104935,-38.8192615374441,17.6897589877086));
#65205=CARTESIAN_POINT('Ctrl Pts',(40.1099071502118,-40.3569109628883,17.6112534773319));
#65206=CARTESIAN_POINT('Ctrl Pts',(38.4012543668155,-40.5609220251472,17.5327479669551));
#65207=CARTESIAN_POINT('Ctrl Pts',(37.2886704652103,-39.2482374965453,17.4542424565783));
#65208=CARTESIAN_POINT('Ctrl Pts',(37.7698859642864,-37.5961510380776,17.3757369462015));
#65209=CARTESIAN_POINT('Ctrl Pts',(39.4133655274823,-37.0862699030106,17.2972314358247));
#65210=CARTESIAN_POINT('Ctrl Pts',(40.7451827384013,-38.1758790339381,17.218725925448));
#65211=CARTESIAN_POINT('Ctrl Pts',(40.5709395934168,-39.8877854279213,17.1402204150712));
#65212=CARTESIAN_POINT('Ctrl Pts',(39.0468978715213,-40.6867135087542,17.0617149046944));
#65213=CARTESIAN_POINT('Ctrl Pts',(37.5398562037872,-39.856164211272,16.9832093943176));
#65214=CARTESIAN_POINT('Ctrl Pts',(37.4013645066268,-38.1409945655745,16.9047038839408));
#65215=CARTESIAN_POINT('Ctrl Pts',(38.7556258599525,-37.0794091529547,16.8261983735641));
#65216=CARTESIAN_POINT('Ctrl Pts',(40.3881062726606,-37.623463173289,16.7476928631873));
#65217=CARTESIAN_POINT('Ctrl Pts',(40.834758606014,-39.2852359660895,16.6691873528105));
#65218=CARTESIAN_POINT('Ctrl Pts',(39.6950143769496,-40.5744102242793,16.5906818424337));
#65219=CARTESIAN_POINT('Ctrl Pts',(37.9910233315818,-40.3348238050803,16.5121763320569));
#65220=CARTESIAN_POINT('Ctrl Pts',(37.2509651368289,-38.7813435147692,16.4336708216802));
#65221=CARTESIAN_POINT('Ctrl Pts',(38.1385415818571,-37.3071674047963,16.3551653113034));
#65222=CARTESIAN_POINT('Ctrl Pts',(39.8577530067585,-37.234371659471,16.2766598009266));
#65223=CARTESIAN_POINT('Ctrl Pts',(40.8667697353107,-38.6282412326641,16.1981542905498));
#65224=CARTESIAN_POINT('Ctrl Pts',(40.2606815765474,-40.2387207543454,16.119648780173));
#65225=CARTESIAN_POINT('Ctrl Pts',(38.5830428006472,-40.6214939022528,16.0411432697963));
#65226=CARTESIAN_POINT('Ctrl Pts',(37.3383997450109,-39.4332806175246,15.9626377594195));
#65227=CARTESIAN_POINT('Ctrl Pts',(37.6429778921717,-37.7396988220853,15.8841322490427));
#65228=CARTESIAN_POINT('Ctrl Pts',(39.2236243178593,-37.0595929325284,15.8056267386659));
#65229=CARTESIAN_POINT('Ctrl Pts',(40.6627777316899,-38.0028980795747,15.7271212282892));
#65230=CARTESIAN_POINT('Ctrl Pts',(40.6697711344255,-39.7236357807726,15.6486157179124));
#65231=CARTESIAN_POINT('Ctrl Pts',(39.2383326839261,-40.6786075590939,15.5701102075356));
#65232=CARTESIAN_POINT('Ctrl Pts',(37.6522103975089,-40.0113720173278,15.4916046971588));
#65233=CARTESIAN_POINT('Ctrl Pts',(37.3338764811494,-38.3203218585575,15.413099186782));
#65234=CARTESIAN_POINT('Ctrl Pts',(38.5688202948726,-37.1220310541764,15.3345936764053));
#65235=CARTESIAN_POINT('Ctrl Pts',(40.2495149974675,-37.4911553124802,15.2560881660285));
#65236=CARTESIAN_POINT('Ctrl Pts',(40.8686733596745,-39.0966551680434,15.1775826556517));
#65237=CARTESIAN_POINT('Ctrl Pts',(39.8710199775172,-40.4986802936762,15.0990771452749));
#65238=CARTESIAN_POINT('Ctrl Pts',(38.151273037136,-40.4398609986215,15.0205716348981));
#65239=CARTESIAN_POINT('Ctrl Pts',(37.2517446794564,-38.9729482851088,14.9420661245214));
#65240=CARTESIAN_POINT('Ctrl Pts',(37.9791488585767,-37.4135034153879,14.8635606141446));
#65241=CARTESIAN_POINT('Ctrl Pts',(39.6811412632861,-37.160075514692,14.7850551037678));
#65242=CARTESIAN_POINT('Ctrl Pts',(40.831316288814,-38.4399409113081,14.706549593391));
#65243=CARTESIAN_POINT('Ctrl Pts',(40.3982068515902,-40.1052936742774,14.6280440830142));
#65244=CARTESIAN_POINT('Ctrl Pts',(38.7701602990205,-40.6625900679474,14.5495385726375));
#65245=CARTESIAN_POINT('Ctrl Pts',(37.4074005907985,-39.6120654537969,14.4710330622607));
#65246=CARTESIAN_POINT('Ctrl Pts',(37.5317725128899,-37.8957903486573,14.3925275518839));
#65247=CARTESIAN_POINT('Ctrl Pts',(39.0323661584192,-37.0530927494379,14.3140220415071));
#65248=CARTESIAN_POINT('Ctrl Pts',(40.5621358440548,-37.8394569175814,14.2355165311303));
#65249=CARTESIAN_POINT('Ctrl Pts',(40.7517455388365,-39.5501918673983,14.1570110207536));
#65250=CARTESIAN_POINT('Ctrl Pts',(39.4258164610498,-40.6499822516745,14.0785055103768));
#65251=CARTESIAN_POINT('Ctrl Pts',(38.3327559670706,-40.3192117233802,14.0261685034589));
#65252=CARTESIAN_POINT('Ctrl Pts',(37.9741697098829,-39.9602191716056,14.));
#65253=CARTESIAN_POINT('Ctrl Pts',(38.4329072841441,-37.7756148875603,17.1934196736194));
#65254=CARTESIAN_POINT('Ctrl Pts',(38.3336188224971,-37.831835714126,17.2005947478237));
#65255=CARTESIAN_POINT('Ctrl Pts',(38.2421150540945,-37.9010724492168,17.2077698220279));
#65256=CARTESIAN_POINT('Ctrl Pts',(38.1625457103697,-37.9820376407054,17.2149448962322));
#65257=CARTESIAN_POINT('Ctrl Pts',(37.8723451372175,-38.2773290667181,17.2411133996911));
#65258=CARTESIAN_POINT('Ctrl Pts',(37.7408919078847,-38.7286281219638,17.26728190315));
#65259=CARTESIAN_POINT('Ctrl Pts',(37.8271270931296,-39.1335701086941,17.293450406609));
#65260=CARTESIAN_POINT('Ctrl Pts',(37.9133622783746,-39.5385120954245,17.3196189100679));
#65261=CARTESIAN_POINT('Ctrl Pts',(38.2172858781974,-39.8970970136394,17.3457874135268));
#65262=CARTESIAN_POINT('Ctrl Pts',(38.6026232932098,-40.0485247084105,17.3719559169858));
#65263=CARTESIAN_POINT('Ctrl Pts',(38.9879607082221,-40.1999524031816,17.3981244204447));
#65264=CARTESIAN_POINT('Ctrl Pts',(39.454711938424,-40.1442228745088,17.4242929239036));
#65265=CARTESIAN_POINT('Ctrl Pts',(39.7935632382491,-39.9063389161268,17.4504614273625));
#65266=CARTESIAN_POINT('Ctrl Pts',(40.1324145380743,-39.6684549577448,17.4766299308215));
#65267=CARTESIAN_POINT('Ctrl Pts',(40.3433659075226,-39.2484165696536,17.5027984342804));
#65268=CARTESIAN_POINT('Ctrl Pts',(40.3318586129825,-38.8345475710328,17.5289669377393));
#65269=CARTESIAN_POINT('Ctrl Pts',(40.3203513184423,-38.4206785724121,17.5551354411983));
#65270=CARTESIAN_POINT('Ctrl Pts',(40.0863853599138,-38.0129789632619,17.5813039446572));
#65271=CARTESIAN_POINT('Ctrl Pts',(39.7348041486982,-37.7943196106437,17.6074724481161));
#65272=CARTESIAN_POINT('Ctrl Pts',(39.3832229374826,-37.5756602580255,17.633640951575));
#65273=CARTESIAN_POINT('Ctrl Pts',(38.9140264735798,-37.5460411619393,17.659809455034));
#65274=CARTESIAN_POINT('Ctrl Pts',(38.5377494466644,-37.7186353304695,17.6859779584929));
#65275=CARTESIAN_POINT('Ctrl Pts',(38.5020812950974,-37.7349959225928,17.6884585302017));
#65276=CARTESIAN_POINT('Ctrl Pts',(38.4672480779576,-37.7531735168604,17.6909391019106));
#65277=CARTESIAN_POINT('Ctrl Pts',(38.4333577759012,-37.7730251466968,17.6934196736194));
#65278=CARTESIAN_POINT('Ctrl Pts',(37.5756558680257,-39.2699729499894,18.));
#65279=CARTESIAN_POINT('Ctrl Pts',(37.4440523270134,-38.7799318659295,17.9738314965411));
#65280=CARTESIAN_POINT('Ctrl Pts',(37.7041245449082,-37.6679293649188,17.9214944896232));
#65281=CARTESIAN_POINT('Ctrl Pts',(39.3195387437205,-37.0695352316426,17.8429889792464));
#65282=CARTESIAN_POINT('Ctrl Pts',(40.7062722211716,-38.0891100356719,17.7644834688697));
#65283=CARTESIAN_POINT('Ctrl Pts',(40.6223994863181,-39.8071108514352,17.6859779584929));
#65284=CARTESIAN_POINT('Ctrl Pts',(39.1423049297703,-40.6853144575312,17.6074724481161));
#65285=CARTESIAN_POINT('Ctrl Pts',(37.593781529679,-39.9348860603428,17.5289669377393));
#65286=CARTESIAN_POINT('Ctrl Pts',(37.365380302334,-38.2294395514345,17.4504614273625));
#65287=CARTESIAN_POINT('Ctrl Pts',(38.6620363043874,-37.0981581562678,17.3719559169858));
#65288=CARTESIAN_POINT('Ctrl Pts',(40.3208285827551,-37.5557507395872,17.293450406609));
#65289=CARTESIAN_POINT('Ctrl Pts',(40.8541369642562,-39.1917640019411,17.2149448962322));
#65290=CARTESIAN_POINT('Ctrl Pts',(39.7836658898431,-40.5390185509755,17.1364393858554));
#65291=CARTESIAN_POINT('Ctrl Pts',(38.0694451486085,-40.389246627264,17.0579338754786));
#65292=CARTESIAN_POINT('Ctrl Pts',(37.2488257543949,-38.87677605618,16.9794283651019));
#65293=CARTESIAN_POINT('Ctrl Pts',(38.0577601193366,-37.3580220610822,16.9009228547251));
#65294=CARTESIAN_POINT('Ctrl Pts',(39.7707759682514,-37.1950414723212,16.8224173443483));
#65295=CARTESIAN_POINT('Ctrl Pts',(40.8516003110939,-38.5339981005298,16.7439118339715));
#65296=CARTESIAN_POINT('Ctrl Pts',(40.3309240105073,-40.1740843304588,16.6654063235947));
#65297=CARTESIAN_POINT('Ctrl Pts',(38.6757020358417,-40.644431583443,16.586900813218));
#65298=CARTESIAN_POINT('Ctrl Pts',(37.3703767628973,-39.5232213878114,16.5083953028412));
#65299=CARTESIAN_POINT('Ctrl Pts',(37.5855949493635,-37.8159816397815,16.4298897924644));
#65300=CARTESIAN_POINT('Ctrl Pts',(39.1283437989466,-37.0538055634981,16.3513842820876));
#65301=CARTESIAN_POINT('Ctrl Pts',(40.6150494715948,-37.9202307686755,16.2728787717108));
#65302=CARTESIAN_POINT('Ctrl Pts',(40.7123989731982,-39.6382265407265,16.1943732613341));
#65303=CARTESIAN_POINT('Ctrl Pts',(39.333086957597,-40.6670534245635,16.1158677509573));
#65304=CARTESIAN_POINT('Ctrl Pts',(37.7141132310224,-40.0840350136355,16.0373622405805));
#65305=CARTESIAN_POINT('Ctrl Pts',(37.3074119207117,-38.4120360784117,15.9588567302037));
#65306=CARTESIAN_POINT('Ctrl Pts',(38.4777224302706,-37.150545013987,15.880351219827));
#65307=CARTESIAN_POINT('Ctrl Pts',(40.1754824724718,-37.430896996864,15.8018457094502));
#65308=CARTESIAN_POINT('Ctrl Pts',(40.8781004790678,-39.0016657040982,15.7233401990734));
#65309=CARTESIAN_POINT('Ctrl Pts',(39.9554519188484,-40.454148415738,15.6448346886966));
#65310=CARTESIAN_POINT('Ctrl Pts',(38.2349899535507,-40.4857241059463,15.5663291783198));
#65311=CARTESIAN_POINT('Ctrl Pts',(37.2596657788943,-39.0680749435716,15.4878236679431));
#65312=CARTESIAN_POINT('Ctrl Pts',(37.904173294426,-37.4725824031402,15.4093181575663));
#65313=CARTESIAN_POINT('Ctrl Pts',(39.5905028527061,-37.1301221194426,15.3308126471895));
#65314=CARTESIAN_POINT('Ctrl Pts',(40.8063139857151,-38.3478206288557,15.2523071368127));
#65315=CARTESIAN_POINT('Ctrl Pts',(40.4612384258705,-40.0336169338117,15.1738016264359));
#65316=CARTESIAN_POINT('Ctrl Pts',(38.8647480157521,-40.6756488816116,15.0952961160592));
#65317=CARTESIAN_POINT('Ctrl Pts',(37.4486135593306,-39.6981268544226,15.0167906056824));
#65318=CARTESIAN_POINT('Ctrl Pts',(37.482857597304,-37.9777160555697,14.9382850953056));
#65319=CARTESIAN_POINT('Ctrl Pts',(38.9367702893063,-37.0573213639055,14.8597795849288));
#65320=CARTESIAN_POINT('Ctrl Pts',(40.5064460859517,-37.7623754838001,14.7812740745521));
#65321=CARTESIAN_POINT('Ctrl Pts',(40.7841666383236,-39.4605673674226,14.7027685641753));
#65322=CARTESIAN_POINT('Ctrl Pts',(39.5208569909583,-40.6289217126118,14.6242630537985));
#65323=CARTESIAN_POINT('Ctrl Pts',(37.8495006293029,-40.2196233657656,14.5457575434217));
#65324=CARTESIAN_POINT('Ctrl Pts',(37.2689744719433,-38.5997554156836,14.4672520330449));
#65325=CARTESIAN_POINT('Ctrl Pts',(38.2999795535027,-37.2220243444981,14.3887465226682));
#65326=CARTESIAN_POINT('Ctrl Pts',(40.0177412802272,-37.3220721610692,14.3102410122913));
#65327=CARTESIAN_POINT('Ctrl Pts',(40.8820235552811,-38.8100518816853,14.2317355019146));
#65328=CARTESIAN_POINT('Ctrl Pts',(40.1171224362185,-40.3517547545304,14.1532299915378));
#65329=CARTESIAN_POINT('Ctrl Pts',(38.4102262410485,-40.5640442208952,14.074724481161));
#65330=CARTESIAN_POINT('Ctrl Pts',(37.2896688855125,-39.2575551350437,13.9962189707842));
#65331=CARTESIAN_POINT('Ctrl Pts',(37.7654127933167,-37.6018660619834,13.9177134604075));
#65332=CARTESIAN_POINT('Ctrl Pts',(38.8548175316166,-37.2592519394722,13.8653764534896));
#65333=CARTESIAN_POINT('Ctrl Pts',(39.3533377835638,-37.3537893102425,13.8392079500307));
#65334=CARTESIAN_POINT('Ctrl Pts',(37.6653123637055,-39.2458951477601,18.0535973499898));
#65335=CARTESIAN_POINT('Ctrl Pts',(37.5416266421298,-38.7853369848302,18.0274288465308));
#65336=CARTESIAN_POINT('Ctrl Pts',(37.7860518276885,-37.7402372050404,17.975091839613));
#65337=CARTESIAN_POINT('Ctrl Pts',(39.304275952107,-37.1778449655031,17.8965863292362));
#65338=CARTESIAN_POINT('Ctrl Pts',(40.6075777437792,-38.1360778851249,17.8180808188594));
#65339=CARTESIAN_POINT('Ctrl Pts',(40.528751143438,-39.7507165865677,17.7395753084826));
#65340=CARTESIAN_POINT('Ctrl Pts',(39.137705265654,-40.5760837907846,17.6610697981059));
#65341=CARTESIAN_POINT('Ctrl Pts',(37.6823475097464,-39.8708043045094,17.5825642877291));
#65342=CARTESIAN_POINT('Ctrl Pts',(37.4676878554874,-38.267964590315,17.5040587773523));
#65343=CARTESIAN_POINT('Ctrl Pts',(38.6863316094155,-37.2047458152724,17.4255532669755));
#65344=CARTESIAN_POINT('Ctrl Pts',(40.2453240067019,-37.6348077149766,17.3470477565988));
#65345=CARTESIAN_POINT('Ctrl Pts',(40.7465463255008,-39.172391577122,17.268542246222));
#65346=CARTESIAN_POINT('Ctrl Pts',(39.7404792679866,-40.4385896578249,17.1900367358452));
#65347=CARTESIAN_POINT('Ctrl Pts',(38.1293932159793,-40.2978286394393,17.1115312254684));
#65348=CARTESIAN_POINT('Ctrl Pts',(37.3581457166218,-38.876354623561,17.0330257150916));
#65349=CARTESIAN_POINT('Ctrl Pts',(38.118411206939,-37.4489752207369,16.9545202047148));
#65350=CARTESIAN_POINT('Ctrl Pts',(39.7283648579877,-37.2958002258341,16.8760146943381));
#65351=CARTESIAN_POINT('Ctrl Pts',(40.7441622880019,-38.5541996233328,16.7975091839613));
#65352=CARTESIAN_POINT('Ctrl Pts',(40.2548120512981,-40.0956114062894,16.7190036735845));
#65353=CARTESIAN_POINT('Ctrl Pts',(38.6991751533109,-40.5376606013873,16.6404981632077));
#65354=CARTESIAN_POINT('Ctrl Pts',(37.4723837080864,-39.4839071003945,16.561992652831));
#65355=CARTESIAN_POINT('Ctrl Pts',(37.6746534683415,-37.8793820358441,16.4834871424542));
#65356=CARTESIAN_POINT('Ctrl Pts',(39.1245840948508,-37.1630616599808,16.4049816320774));
#65357=CARTESIAN_POINT('Ctrl Pts',(40.5218433363406,-37.9773591011396,16.3264761217006));
#65358=CARTESIAN_POINT('Ctrl Pts',(40.6133358847798,-39.5919930623209,16.2479706113238));
#65359=CARTESIAN_POINT('Ctrl Pts',(39.3170090487735,-40.5589214179339,16.1694651009471));
#65360=CARTESIAN_POINT('Ctrl Pts',(37.7954395526701,-40.010979832982,16.0909595905703));
#65361=CARTESIAN_POINT('Ctrl Pts',(37.4132070941463,-38.4395753465506,16.0124540801935));
#65362=CARTESIAN_POINT('Ctrl Pts',(38.5131068288268,-37.2539808605321,15.9339485698167));
#65363=CARTESIAN_POINT('Ctrl Pts',(40.1087225262984,-37.517465695595,15.8554430594399));
#65364=CARTESIAN_POINT('Ctrl Pts',(40.7690680950382,-38.9937303879309,15.7769375490632));
#65365=CARTESIAN_POINT('Ctrl Pts',(39.9019299310211,-40.3588256648782,15.6984320386864));
#65366=CARTESIAN_POINT('Ctrl Pts',(38.2849781530934,-40.3885016295036,15.6199265283096));
#65367=CARTESIAN_POINT('Ctrl Pts',(37.3683335599107,-39.0561441698123,15.5414210179328));
#65368=CARTESIAN_POINT('Ctrl Pts',(37.9740648077657,-37.5566431334877,15.462915507556));
#65369=CARTESIAN_POINT('Ctrl Pts',(39.558937727035,-37.2347866927388,15.3844099971793));
#65370=CARTESIAN_POINT('Ctrl Pts',(40.7016005773602,-38.37922336701,15.3059044868025));
#65371=CARTESIAN_POINT('Ctrl Pts',(40.3772862064154,-39.9635951157055,15.2273989764257));
#65372=CARTESIAN_POINT('Ctrl Pts',(38.8768473364175,-40.566999736337,15.1488934660489));
#65373=CARTESIAN_POINT('Ctrl Pts',(37.5459134516342,-39.6482895226222,15.0703879556721));
#65374=CARTESIAN_POINT('Ctrl Pts',(37.5780972250634,-38.0313858327519,14.9918824452954));
#65375=CARTESIAN_POINT('Ctrl Pts',(38.9445364487738,-37.1663659351315,14.9133769349186));
#65376=CARTESIAN_POINT('Ctrl Pts',(40.4197739845928,-37.829001050405,14.8348714245418));
#65377=CARTESIAN_POINT('Ctrl Pts',(40.6807857070153,-39.425022607912,14.756365914165));
#65378=CARTESIAN_POINT('Ctrl Pts',(39.4934820516118,-40.5230838692526,14.6778604037882));
#65379=CARTESIAN_POINT('Ctrl Pts',(37.9226814788354,-40.1384106227729,14.5993548934115));
#65380=CARTESIAN_POINT('Ctrl Pts',(37.3770822030539,-38.6160007033882,14.5208493830347));
#65381=CARTESIAN_POINT('Ctrl Pts',(38.3460577069044,-37.3211596955696,14.4423438726579));
#65382=CARTESIAN_POINT('Ctrl Pts',(39.9604717039048,-37.4151882170629,14.3638383622811));
#65383=CARTESIAN_POINT('Ctrl Pts',(40.7727551425788,-38.8136448544663,14.2853328519044));
#65384=CARTESIAN_POINT('Ctrl Pts',(40.053873673907,-40.2625924345728,14.2068273415276));
#65385=CARTESIAN_POINT('Ctrl Pts',(38.4496714926396,-40.4621096787767,14.1283218311508));
#65386=CARTESIAN_POINT('Ctrl Pts',(37.3965315541519,-39.2342244404969,14.049816320774));
#65387=CARTESIAN_POINT('Ctrl Pts',(37.8436527187451,-37.6781485467081,13.9713108103972));
#65388=CARTESIAN_POINT('Ctrl Pts',(38.8675143117402,-37.356147522732,13.9189738034794));
#65389=CARTESIAN_POINT('Ctrl Pts',(39.3360415003545,-37.4449971298904,13.8928053000205));
#65390=CARTESIAN_POINT('Ctrl Pts',(37.7549688593853,-39.2218173455308,18.1071946999795));
#65391=CARTESIAN_POINT('Ctrl Pts',(37.6392009572462,-38.7907421037308,18.0810261965206));
#65392=CARTESIAN_POINT('Ctrl Pts',(37.8679791104688,-37.812545045162,18.0286891896028));
#65393=CARTESIAN_POINT('Ctrl Pts',(39.2890131604934,-37.2861546993636,17.950183679226));
#65394=CARTESIAN_POINT('Ctrl Pts',(40.5088832663869,-38.1830457345779,17.8716781688492));
#65395=CARTESIAN_POINT('Ctrl Pts',(40.4351028005577,-39.6943223217001,17.7931726584724));
#65396=CARTESIAN_POINT('Ctrl Pts',(39.1331056015378,-40.466853124038,17.7146671480956));
#65397=CARTESIAN_POINT('Ctrl Pts',(37.7709134898136,-39.8067225486761,17.6361616377189));
#65398=CARTESIAN_POINT('Ctrl Pts',(37.5699954086408,-38.3064896291956,17.5576561273421));
#65399=CARTESIAN_POINT('Ctrl Pts',(38.7106269144436,-37.3113334742769,17.4791506169653));
#65400=CARTESIAN_POINT('Ctrl Pts',(40.1698194306487,-37.713864690366,17.4006451065885));
#65401=CARTESIAN_POINT('Ctrl Pts',(40.6389556867455,-39.1530191523028,17.3221395962118));
#65402=CARTESIAN_POINT('Ctrl Pts',(39.6972926461299,-40.3381607646743,17.243634085835));
#65403=CARTESIAN_POINT('Ctrl Pts',(38.1893412833502,-40.2064106516147,17.1651285754582));
#65404=CARTESIAN_POINT('Ctrl Pts',(37.4674656788486,-38.875933190942,17.0866230650814));
#65405=CARTESIAN_POINT('Ctrl Pts',(38.1790622945415,-37.5399283803915,17.0081175547046));
#65406=CARTESIAN_POINT('Ctrl Pts',(39.6859537477239,-37.396558979347,16.9296120443278));
#65407=CARTESIAN_POINT('Ctrl Pts',(40.63672426491,-38.5744011461358,16.8511065339511));
#65408=CARTESIAN_POINT('Ctrl Pts',(40.1787000920889,-40.01713848212,16.7726010235743));
#65409=CARTESIAN_POINT('Ctrl Pts',(38.7226482707802,-40.4308896193315,16.6940955131975));
#65410=CARTESIAN_POINT('Ctrl Pts',(37.5743906532754,-39.4445928129776,16.6155900028207));
#65411=CARTESIAN_POINT('Ctrl Pts',(37.7637119873195,-37.9427824319066,16.537084492444));
#65412=CARTESIAN_POINT('Ctrl Pts',(39.1208243907549,-37.2723177564635,16.4585789820672));
#65413=CARTESIAN_POINT('Ctrl Pts',(40.4286372010862,-38.0344874336038,16.3800734716904));
#65414=CARTESIAN_POINT('Ctrl Pts',(40.5142727963614,-39.5457595839153,16.3015679613136));
#65415=CARTESIAN_POINT('Ctrl Pts',(39.3009311399501,-40.4507894113044,16.2230624509368));
#65416=CARTESIAN_POINT('Ctrl Pts',(37.8767658743178,-39.9379246523286,16.14455694056));
#65417=CARTESIAN_POINT('Ctrl Pts',(37.5190022675809,-38.4671146146895,16.0660514301833));
#65418=CARTESIAN_POINT('Ctrl Pts',(38.548491227383,-37.3574167070772,15.9875459198065));
#65419=CARTESIAN_POINT('Ctrl Pts',(40.0419625801251,-37.6040343943261,15.9090404094297));
#65420=CARTESIAN_POINT('Ctrl Pts',(40.6600357110085,-38.9857950717635,15.8305348990529));
#65421=CARTESIAN_POINT('Ctrl Pts',(39.8484079431939,-40.2635029140183,15.7520293886762));
#65422=CARTESIAN_POINT('Ctrl Pts',(38.3349663526361,-40.2912791530608,15.6735238782994));
#65423=CARTESIAN_POINT('Ctrl Pts',(37.4770013409271,-39.044213396053,15.5950183679226));
#65424=CARTESIAN_POINT('Ctrl Pts',(38.0439563211054,-37.640703863835,15.5165128575458));
#65425=CARTESIAN_POINT('Ctrl Pts',(39.5273726013638,-37.3394512660349,15.438007347169));
#65426=CARTESIAN_POINT('Ctrl Pts',(40.5968871690054,-38.4106261051643,15.3595018367923));
#65427=CARTESIAN_POINT('Ctrl Pts',(40.2933339869602,-39.8935732975993,15.2809963264155));
#65428=CARTESIAN_POINT('Ctrl Pts',(38.8889466570829,-40.4583505910623,15.2024908160387));
#65429=CARTESIAN_POINT('Ctrl Pts',(37.6432133439378,-39.5984521908219,15.1239853056619));
#65430=CARTESIAN_POINT('Ctrl Pts',(37.6733368528227,-38.0850556099341,15.0454797952851));
#65431=CARTESIAN_POINT('Ctrl Pts',(38.9523026082414,-37.2754105063575,14.9669742849084));
#65432=CARTESIAN_POINT('Ctrl Pts',(40.3331018832338,-37.89562661701,14.8884687745316));
#65433=CARTESIAN_POINT('Ctrl Pts',(40.577404775707,-39.3894778484014,14.8099632641548));
#65434=CARTESIAN_POINT('Ctrl Pts',(39.4661071122653,-40.4172460258934,14.731457753778));
#65435=CARTESIAN_POINT('Ctrl Pts',(37.9958623283679,-40.0571978797803,14.6529522434012));
#65436=CARTESIAN_POINT('Ctrl Pts',(37.4851899341644,-38.6322459910928,14.5744467330245));
#65437=CARTESIAN_POINT('Ctrl Pts',(38.3921358603061,-37.4202950466411,14.4959412226477));
#65438=CARTESIAN_POINT('Ctrl Pts',(39.9032021275825,-37.5083042730566,14.4174357122709));
#65439=CARTESIAN_POINT('Ctrl Pts',(40.6634867298766,-38.8172378272473,14.3389302018941));
#65440=CARTESIAN_POINT('Ctrl Pts',(39.9906249115955,-40.1734301146151,14.2604246915173));
#65441=CARTESIAN_POINT('Ctrl Pts',(38.4891167442306,-40.3601751366582,14.1819191811406));
#65442=CARTESIAN_POINT('Ctrl Pts',(37.5033942227913,-39.2108937459501,14.1034136707638));
#65443=CARTESIAN_POINT('Ctrl Pts',(37.9218926441736,-37.7544310314327,14.024908160387));
#65444=CARTESIAN_POINT('Ctrl Pts',(38.8802110918637,-37.4530431059918,13.9725711534692));
#65445=CARTESIAN_POINT('Ctrl Pts',(39.3187452171453,-37.5362049495383,13.9464026500102));
#65446=CARTESIAN_POINT('Ctrl Pts',(37.8446253550651,-39.1977395433015,18.1607920499693));
#65447=CARTESIAN_POINT('Ctrl Pts',(37.7367752723626,-38.7961472226316,18.1346235465104));
#65448=CARTESIAN_POINT('Ctrl Pts',(37.9499063932491,-37.8848528852836,18.0822865395925));
#65449=CARTESIAN_POINT('Ctrl Pts',(39.2737503688799,-37.3944644332241,18.0037810292158));
#65450=CARTESIAN_POINT('Ctrl Pts',(40.4101887889945,-38.230013584031,17.925275518839));
#65451=CARTESIAN_POINT('Ctrl Pts',(40.3414544576775,-39.6379280568325,17.8467700084622));
#65452=CARTESIAN_POINT('Ctrl Pts',(39.1285059374216,-40.3576224572915,17.7682644980854));
#65453=CARTESIAN_POINT('Ctrl Pts',(37.8594794698809,-39.7426407928426,17.6897589877086));
#65454=CARTESIAN_POINT('Ctrl Pts',(37.6723029617942,-38.3450146680762,17.6112534773319));
#65455=CARTESIAN_POINT('Ctrl Pts',(38.7349222194717,-37.4179211332815,17.5327479669551));
#65456=CARTESIAN_POINT('Ctrl Pts',(40.0943148545955,-37.7929216657554,17.4542424565783));
#65457=CARTESIAN_POINT('Ctrl Pts',(40.5313650479902,-39.1336467274836,17.3757369462015));
#65458=CARTESIAN_POINT('Ctrl Pts',(39.6541060242733,-40.2377318715238,17.2972314358247));
#65459=CARTESIAN_POINT('Ctrl Pts',(38.249289350721,-40.11499266379,17.218725925448));
#65460=CARTESIAN_POINT('Ctrl Pts',(37.5767856410754,-38.8755117583229,17.1402204150712));
#65461=CARTESIAN_POINT('Ctrl Pts',(38.2397133821439,-37.6308815400462,17.0617149046944));
#65462=CARTESIAN_POINT('Ctrl Pts',(39.6435426374601,-37.4973177328599,16.9832093943176));
#65463=CARTESIAN_POINT('Ctrl Pts',(40.529286241818,-38.5946026689388,16.9047038839408));
#65464=CARTESIAN_POINT('Ctrl Pts',(40.1025881328798,-39.9386655579506,16.8261983735641));
#65465=CARTESIAN_POINT('Ctrl Pts',(38.7461213882494,-40.3241186372758,16.7476928631873));
#65466=CARTESIAN_POINT('Ctrl Pts',(37.6763975984644,-39.4052785255607,16.6691873528105));
#65467=CARTESIAN_POINT('Ctrl Pts',(37.8527705062976,-38.0061828279691,16.5906818424337));
#65468=CARTESIAN_POINT('Ctrl Pts',(39.1170646866591,-37.3815738529462,16.5121763320569));
#65469=CARTESIAN_POINT('Ctrl Pts',(40.335431065832,-38.0916157660679,16.4336708216802));
#65470=CARTESIAN_POINT('Ctrl Pts',(40.4152097079431,-39.4995261055097,16.3551653113034));
#65471=CARTESIAN_POINT('Ctrl Pts',(39.2848532311266,-40.3426574046748,16.2766598009266));
#65472=CARTESIAN_POINT('Ctrl Pts',(37.9580921959656,-39.8648694716751,16.1981542905498));
#65473=CARTESIAN_POINT('Ctrl Pts',(37.6247974410155,-38.4946538828284,16.119648780173));
#65474=CARTESIAN_POINT('Ctrl Pts',(38.5838756259392,-37.4608525536223,16.0411432697963));
#65475=CARTESIAN_POINT('Ctrl Pts',(39.9752026339518,-37.6906030930571,15.9626377594195));
#65476=CARTESIAN_POINT('Ctrl Pts',(40.5510033269788,-38.9778597555962,15.8841322490427));
#65477=CARTESIAN_POINT('Ctrl Pts',(39.7948859553666,-40.1681801631584,15.8056267386659));
#65478=CARTESIAN_POINT('Ctrl Pts',(38.3849545521788,-40.1940566766182,15.7271212282891));
#65479=CARTESIAN_POINT('Ctrl Pts',(37.5856691219435,-39.0322826222936,15.6486157179124));
#65480=CARTESIAN_POINT('Ctrl Pts',(38.1138478344451,-37.7247645941825,15.5701102075356));
#65481=CARTESIAN_POINT('Ctrl Pts',(39.4958074756927,-37.4441158393311,15.4916046971588));
#65482=CARTESIAN_POINT('Ctrl Pts',(40.4921737606505,-38.4420288433187,15.413099186782));
#65483=CARTESIAN_POINT('Ctrl Pts',(40.2093817675051,-39.823551479493,15.3345936764052));
#65484=CARTESIAN_POINT('Ctrl Pts',(38.9010459777483,-40.3497014457878,15.2560881660285));
#65485=CARTESIAN_POINT('Ctrl Pts',(37.7405132362414,-39.5486148590214,15.1775826556517));
#65486=CARTESIAN_POINT('Ctrl Pts',(37.768576480582,-38.1387253871164,15.0990771452749));
#65487=CARTESIAN_POINT('Ctrl Pts',(38.9600687677089,-37.3844550775834,15.0205716348981));
#65488=CARTESIAN_POINT('Ctrl Pts',(40.2464297818749,-37.962252183615,14.9420661245214));
#65489=CARTESIAN_POINT('Ctrl Pts',(40.4740238443987,-39.3539330888908,14.8635606141446));
#65490=CARTESIAN_POINT('Ctrl Pts',(39.4387321729189,-40.3114081825343,14.7850551037678));
#65491=CARTESIAN_POINT('Ctrl Pts',(38.0690431779005,-39.9759851367875,14.706549593391));
#65492=CARTESIAN_POINT('Ctrl Pts',(37.593297665275,-38.6484912787976,14.6280440830142));
#65493=CARTESIAN_POINT('Ctrl Pts',(38.4382140137078,-37.5194303977126,14.5495385726375));
#65494=CARTESIAN_POINT('Ctrl Pts',(39.8459325512601,-37.6014203290504,14.4710330622607));
#65495=CARTESIAN_POINT('Ctrl Pts',(40.5542183171743,-38.8208308000283,14.3925275518839));
#65496=CARTESIAN_POINT('Ctrl Pts',(39.9273761492841,-40.0842677946575,14.3140220415071));
#65497=CARTESIAN_POINT('Ctrl Pts',(38.5285619958217,-40.2582405945397,14.2355165311304));
#65498=CARTESIAN_POINT('Ctrl Pts',(37.6102568914307,-39.1875630514034,14.1570110207535));
#65499=CARTESIAN_POINT('Ctrl Pts',(38.0001325696021,-37.8307135161573,14.0785055103768));
#65500=CARTESIAN_POINT('Ctrl Pts',(38.8929078719872,-37.5499386892516,14.0261685034589));
#65501=CARTESIAN_POINT('Ctrl Pts',(39.3014489339361,-37.6274127691862,14.));
#65502=CARTESIAN_POINT('Ctrl Pts',(38.4348713855213,-37.7748596688487,17.5565803263806));
#65503=CARTESIAN_POINT('Ctrl Pts',(38.5438548719482,-37.7108039030124,17.5486362065721));
#65504=CARTESIAN_POINT('Ctrl Pts',(38.6618404864523,-37.6628704742542,17.5406920867636));
#65505=CARTESIAN_POINT('Ctrl Pts',(38.7843844490461,-37.6349368111596,17.5327479669551));
#65506=CARTESIAN_POINT('Ctrl Pts',(39.1880530978463,-37.5429213107728,17.5065794634961));
#65507=CARTESIAN_POINT('Ctrl Pts',(39.6411839762209,-37.6679214882641,17.4804109600372));
#65508=CARTESIAN_POINT('Ctrl Pts',(39.9405911143073,-37.9538757539645,17.4542424565783));
#65509=CARTESIAN_POINT('Ctrl Pts',(40.2399982523938,-38.2398300196648,17.4280739531194));
#65510=CARTESIAN_POINT('Ctrl Pts',(40.385681650192,-38.6867383735742,17.4019054496604));
#65511=CARTESIAN_POINT('Ctrl Pts',(40.3123135118049,-39.0942067412023,17.3757369462015));
#65512=CARTESIAN_POINT('Ctrl Pts',(40.2389453734179,-39.5016751088304,17.3495684427426));
#65513=CARTESIAN_POINT('Ctrl Pts',(39.9465256988456,-39.8697034901771,17.3233999392837));
#65514=CARTESIAN_POINT('Ctrl Pts',(39.5661797493007,-40.0332611462281,17.2972314358247));
#65515=CARTESIAN_POINT('Ctrl Pts',(39.1858337997559,-40.1968188022792,17.2710629323658));
#65516=CARTESIAN_POINT('Ctrl Pts',(38.7175615752384,-40.1559057330346,17.2448944289069));
#65517=CARTESIAN_POINT('Ctrl Pts',(38.3713415113721,-39.9288690475011,17.218725925448));
#65518=CARTESIAN_POINT('Ctrl Pts',(38.0251214475058,-39.7018323619677,17.192557421989));
#65519=CARTESIAN_POINT('Ctrl Pts',(37.8009535442906,-39.2886720601453,17.1663889185301));
#65520=CARTESIAN_POINT('Ctrl Pts',(37.7993575495278,-38.8746535395213,17.1402204150712));
#65521=CARTESIAN_POINT('Ctrl Pts',(37.7977615547649,-38.4606350188973,17.1140519116123));
#65522=CARTESIAN_POINT('Ctrl Pts',(38.0187374684544,-38.0457582794717,17.0878834081533));
#65523=CARTESIAN_POINT('Ctrl Pts',(38.3631969678519,-37.8160592752279,17.0617149046944));
#65524=CARTESIAN_POINT('Ctrl Pts',(38.3857260141201,-37.8010360301049,17.0600033785898));
#65525=CARTESIAN_POINT('Ctrl Pts',(38.4087832848556,-37.7868049178791,17.0582918524852));
#65526=CARTESIAN_POINT('Ctrl Pts',(38.4323100738575,-37.7733715239653,17.0565803263806));
#65527=CARTESIAN_POINT('Origin',(39.0658530619283,-38.8697713466883,15.5));
#65528=CARTESIAN_POINT('Origin',(-14.1292828945604,-53.2669068454841,14.));
#65529=CARTESIAN_POINT('Ctrl Pts',(-12.9355708698302,-52.8497595669186,
14.));
#65530=CARTESIAN_POINT('Ctrl Pts',(-12.9470539462122,-52.8001843799443,
14.));
#65531=CARTESIAN_POINT('Ctrl Pts',(-12.9617293958119,-52.7515166200284,
14.));
#65532=CARTESIAN_POINT('Ctrl Pts',(-12.9793332579477,-52.703925204681,14.));
#65533=CARTESIAN_POINT('Ctrl Pts',(-12.9911966085512,-52.6718530581471,
14.));
#65534=CARTESIAN_POINT('Ctrl Pts',(-13.0043910411209,-52.6402695886307,
14.));
#65535=CARTESIAN_POINT('Ctrl Pts',(-13.0188485042637,-52.6092270378974,
14.));
#65536=CARTESIAN_POINT('Ctrl Pts',(-13.0255213915096,-52.5948992516997,
14.));
#65537=CARTESIAN_POINT('Ctrl Pts',(-13.0324634794559,-52.580686716332,14.));
#65538=CARTESIAN_POINT('Ctrl Pts',(-13.0396687478568,-52.5665947050473,
14.));
#65539=CARTESIAN_POINT('Ctrl Pts',(-13.0457249481659,-52.5547500327394,
14.));
#65540=CARTESIAN_POINT('Ctrl Pts',(-13.0519637639886,-52.5429971707098,
14.));
#65541=CARTESIAN_POINT('Ctrl Pts',(-13.058377507715,-52.5313453176613,14.));
#65542=CARTESIAN_POINT('Ctrl Pts',(-13.0842985632228,-52.4842545166369,
14.));
#65543=CARTESIAN_POINT('Ctrl Pts',(-13.1130890591351,-52.4387805987043,
14.));
#65544=CARTESIAN_POINT('Ctrl Pts',(-13.1444873892514,-52.3951192737037,
14.));
#65545=CARTESIAN_POINT('Ctrl Pts',(-13.1565047144364,-52.3784084378536,
14.));
#65546=CARTESIAN_POINT('Ctrl Pts',(-13.1689046041074,-52.3619632326173,
14.));
#65547=CARTESIAN_POINT('Ctrl Pts',(-13.1816743223107,-52.3457951881003,
14.));
#65548=CARTESIAN_POINT('Ctrl Pts',(-13.1908504260224,-52.3341771045262,
14.));
#65549=CARTESIAN_POINT('Ctrl Pts',(-13.2002175167485,-52.3227021433122,
14.));
#65550=CARTESIAN_POINT('Ctrl Pts',(-13.2097711771542,-52.3113747298545,
14.));
#65551=CARTESIAN_POINT('Ctrl Pts',(-13.2171669954176,-52.3026057881325,
14.));
#65552=CARTESIAN_POINT('Ctrl Pts',(-13.2246749676875,-52.2939250678948,
14.));
#65553=CARTESIAN_POINT('Ctrl Pts',(-13.232282522036,-52.2853461206881,14.));
#65554=CARTESIAN_POINT('Ctrl Pts',(-13.2698783495994,-52.2429497597705,
14.));
#65555=CARTESIAN_POINT('Ctrl Pts',(-13.3099602111104,-52.2029670203149,
14.));
#65556=CARTESIAN_POINT('Ctrl Pts',(-13.3522361487837,-52.1656107563157,
14.));
#65557=CARTESIAN_POINT('Ctrl Pts',(-13.3938995696844,-52.1287957301818,
14.));
#65558=CARTESIAN_POINT('Ctrl Pts',(-13.4376947734015,-52.094530697541,14.));
#65559=CARTESIAN_POINT('Ctrl Pts',(-13.4833901901288,-52.0630423693105,
14.));
#65560=CARTESIAN_POINT('Ctrl Pts',(-13.5072520755132,-52.0465993443205,
14.));
#65561=CARTESIAN_POINT('Ctrl Pts',(-13.5316328454894,-52.0309139558741,
14.));
#65562=CARTESIAN_POINT('Ctrl Pts',(-13.5565037015348,-52.0160223211125,
14.));
#65563=CARTESIAN_POINT('Ctrl Pts',(-13.5698458264541,-52.0080336113198,
14.));
#65564=CARTESIAN_POINT('Ctrl Pts',(-13.5833290354763,-52.0002733832278,
14.));
#65565=CARTESIAN_POINT('Ctrl Pts',(-13.5969491667113,-51.9927476035094,
14.));
#65566=CARTESIAN_POINT('Ctrl Pts',(-13.6066315694002,-51.9873976088197,
14.));
#65567=CARTESIAN_POINT('Ctrl Pts',(-13.6163831716242,-51.9821661014994,
14.));
#65568=CARTESIAN_POINT('Ctrl Pts',(-13.6262025324358,-51.9770553186038,
14.));
#65569=CARTESIAN_POINT('Ctrl Pts',(-13.6348477565866,-51.9725556505942,
14.));
#65570=CARTESIAN_POINT('Ctrl Pts',(-13.6435368082189,-51.9681540962248,
14.));
#65571=CARTESIAN_POINT('Ctrl Pts',(-13.6522677898872,-51.9638519547314,
14.));
#65572=CARTESIAN_POINT('Ctrl Pts',(-13.6954565667737,-51.9425709308842,
14.));
#65573=CARTESIAN_POINT('Ctrl Pts',(-13.7396739228985,-51.9237189359356,
14.));
#65574=CARTESIAN_POINT('Ctrl Pts',(-13.7847671512145,-51.9074289316259,
14.));
#65575=CARTESIAN_POINT('Ctrl Pts',(-13.8360916879565,-51.8888878567031,
14.));
#65576=CARTESIAN_POINT('Ctrl Pts',(-13.8885506645623,-51.8736638854944,
14.));
#65577=CARTESIAN_POINT('Ctrl Pts',(-13.941847374976,-51.8616392672994,14.));
#65578=CARTESIAN_POINT('Ctrl Pts',(-13.9939442075944,-51.849885361354,14.));
#65579=CARTESIAN_POINT('Ctrl Pts',(-14.0468423626068,-51.8411885354972,
14.));
#65580=CARTESIAN_POINT('Ctrl Pts',(-14.1002842110383,-51.8354800340536,
14.));
#65581=CARTESIAN_POINT('Ctrl Pts',(-14.1133747158346,-51.8340817447407,
14.));
#65582=CARTESIAN_POINT('Ctrl Pts',(-14.12649790077,-51.8328629457924,14.));
#65583=CARTESIAN_POINT('Ctrl Pts',(-14.1396500710028,-51.8318229995033,
14.));
#65584=CARTESIAN_POINT('Ctrl Pts',(-14.1495801723766,-51.8310378232252,
14.));
#65585=CARTESIAN_POINT('Ctrl Pts',(-14.1595248274499,-51.8303548395322,
14.));
#65586=CARTESIAN_POINT('Ctrl Pts',(-14.1694709141462,-51.8297741437814,
14.));
#65587=CARTESIAN_POINT('Ctrl Pts',(-14.2269882874541,-51.8264160296513,
14.));
#65588=CARTESIAN_POINT('Ctrl Pts',(-14.2846572205454,-51.82646594941,14.));
#65589=CARTESIAN_POINT('Ctrl Pts',(-14.3421515419977,-51.829789630806,14.));
#65590=CARTESIAN_POINT('Ctrl Pts',(-14.4008791521421,-51.83318460722,14.));
#65591=CARTESIAN_POINT('Ctrl Pts',(-14.4594256017928,-51.839995169772,14.));
#65592=CARTESIAN_POINT('Ctrl Pts',(-14.5174614757873,-51.8501296661509,
14.));
#65593=CARTESIAN_POINT('Ctrl Pts',(-14.5760079663998,-51.8603533287973,
14.));
#65594=CARTESIAN_POINT('Ctrl Pts',(-14.6340360433043,-51.8739596390729,
14.));
#65595=CARTESIAN_POINT('Ctrl Pts',(-14.6912089918265,-51.8909073923744,
14.));
#65596=CARTESIAN_POINT('Ctrl Pts',(-14.7041595778874,-51.8947463292028,
14.));
#65597=CARTESIAN_POINT('Ctrl Pts',(-14.7170698109426,-51.8987582304422,
14.));
#65598=CARTESIAN_POINT('Ctrl Pts',(-14.7299100502027,-51.9029342190779,
14.));
#65599=CARTESIAN_POINT('Ctrl Pts',(-14.7877641556196,-51.9217499188366,
14.));
#65600=CARTESIAN_POINT('Ctrl Pts',(-14.844296494245,-51.9439200711751,14.));
#65601=CARTESIAN_POINT('Ctrl Pts',(-14.89916300966,-51.9693357901013,14.));
#65602=CARTESIAN_POINT('Ctrl Pts',(-14.9535472830576,-51.9945281209106,
14.));
#65603=CARTESIAN_POINT('Ctrl Pts',(-15.0062960530717,-52.0229093771236,
14.));
#65604=CARTESIAN_POINT('Ctrl Pts',(-15.0570711074075,-52.0544235838658,
14.));
#65605=CARTESIAN_POINT('Ctrl Pts',(-15.0942742803416,-52.0775142235243,
14.));
#65606=CARTESIAN_POINT('Ctrl Pts',(-15.1304178629323,-52.1022878477978,
14.));
#65607=CARTESIAN_POINT('Ctrl Pts',(-15.1653622380934,-52.1287390412771,
14.));
#65608=CARTESIAN_POINT('Ctrl Pts',(-15.1847827002204,-52.1434393871498,
14.));
#65609=CARTESIAN_POINT('Ctrl Pts',(-15.2038326363704,-52.1586581279523,
14.));
#65610=CARTESIAN_POINT('Ctrl Pts',(-15.2225055381225,-52.1743757967134,
14.));
#65611=CARTESIAN_POINT('Ctrl Pts',(-15.619480088463,-52.8667052421829,14.));
#65612=CARTESIAN_POINT('Ctrl Pts',(-15.6300068882699,-52.9268481278985,
14.));
#65613=CARTESIAN_POINT('Ctrl Pts',(-15.636648860063,-52.9875198480058,14.));
#65614=CARTESIAN_POINT('Ctrl Pts',(-15.6395377285819,-53.0483965304075,
14.));
#65615=CARTESIAN_POINT('Ctrl Pts',(-15.6422164647752,-53.104845126599,14.));
#65616=CARTESIAN_POINT('Ctrl Pts',(-15.6416673528963,-53.1614706817463,
14.));
#65617=CARTESIAN_POINT('Ctrl Pts',(-15.6379557899095,-53.2180062233411,
14.));
#65618=CARTESIAN_POINT('Ctrl Pts',(-15.6370599130155,-53.2316524649873,
14.));
#65619=CARTESIAN_POINT('Ctrl Pts',(-15.635979458861,-53.2452938319618,14.));
#65620=CARTESIAN_POINT('Ctrl Pts',(-15.6347168346783,-53.2589112013707,
14.));
#65621=CARTESIAN_POINT('Ctrl Pts',(-15.6291600434172,-53.3188410525236,
14.));
#65622=CARTESIAN_POINT('Ctrl Pts',(-15.6200747337923,-53.3783798722155,
14.));
#65623=CARTESIAN_POINT('Ctrl Pts',(-15.6075583989801,-53.4372064199324,
14.));
#65624=CARTESIAN_POINT('Ctrl Pts',(-15.5998328638199,-53.4735162957514,
14.));
#65625=CARTESIAN_POINT('Ctrl Pts',(-15.5907991790431,-53.5095545289945,
14.));
#65626=CARTESIAN_POINT('Ctrl Pts',(-15.5804715530903,-53.5452408049524,
14.));
#65627=CARTESIAN_POINT('Ctrl Pts',(-15.5769376859793,-53.5574517968589,
14.));
#65628=CARTESIAN_POINT('Ctrl Pts',(-15.5732522649477,-53.5696215399255,
14.));
#65629=CARTESIAN_POINT('Ctrl Pts',(-15.5694156969316,-53.5817466809952,
14.));
#65630=CARTESIAN_POINT('Ctrl Pts',(-15.5658265665456,-53.5930898168563,
14.));
#65631=CARTESIAN_POINT('Ctrl Pts',(-15.5621073992277,-53.6043866740437,
14.));
#65632=CARTESIAN_POINT('Ctrl Pts',(-15.5582610327256,-53.6156290047355,
14.));
#65633=CARTESIAN_POINT('Ctrl Pts',(-15.5392227656906,-53.6712748964329,
14.));
#65634=CARTESIAN_POINT('Ctrl Pts',(-15.5170576051387,-53.7256323263301,
14.));
#65635=CARTESIAN_POINT('Ctrl Pts',(-15.4918565786129,-53.7784002654543,
14.));
#65636=CARTESIAN_POINT('Ctrl Pts',(-15.4672989399537,-53.8298210272427,
14.));
#65637=CARTESIAN_POINT('Ctrl Pts',(-15.4398578622449,-53.8797331989486,
14.));
#65638=CARTESIAN_POINT('Ctrl Pts',(-15.4095790814541,-53.9278277241228,
14.));
#65639=CARTESIAN_POINT('Ctrl Pts',(-15.3931628297317,-53.9539031410025,
14.));
#65640=CARTESIAN_POINT('Ctrl Pts',(-15.375911821029,-53.9794436627758,14.));
#65641=CARTESIAN_POINT('Ctrl Pts',(-15.3578293393444,-54.0043949447235,
14.));
#65642=CARTESIAN_POINT('Ctrl Pts',(-15.3427850973266,-54.0251538831713,
14.));
#65643=CARTESIAN_POINT('Ctrl Pts',(-15.3271652651206,-54.0455049012987,
14.));
#65644=CARTESIAN_POINT('Ctrl Pts',(-15.3109704283096,-54.0654144328928,
14.));
#65645=CARTESIAN_POINT('Ctrl Pts',(-15.3040483576438,-54.0739242552656,
14.));
#65646=CARTESIAN_POINT('Ctrl Pts',(-15.2970202959566,-54.0823543061125,
14.));
#65647=CARTESIAN_POINT('Ctrl Pts',(-15.2898980773051,-54.0906884968018,
14.));
#65648=CARTESIAN_POINT('Ctrl Pts',(-15.2569263347024,-54.1292709671884,
14.));
#65649=CARTESIAN_POINT('Ctrl Pts',(-15.2218841350179,-54.1658696979238,
14.));
#65650=CARTESIAN_POINT('Ctrl Pts',(-15.1848122311441,-54.2002693479339,
14.));
#65651=CARTESIAN_POINT('Ctrl Pts',(-15.1433853438147,-54.2387100611489,
14.));
#65652=CARTESIAN_POINT('Ctrl Pts',(-15.0994234021571,-54.2744057498397,
14.));
#65653=CARTESIAN_POINT('Ctrl Pts',(-15.0532626173756,-54.3072661456667,
14.));
#65654=CARTESIAN_POINT('Ctrl Pts',(-15.014090564972,-54.335151484996,14.));
#65655=CARTESIAN_POINT('Ctrl Pts',(-14.9733341416966,-54.3609943509891,
14.));
#65656=CARTESIAN_POINT('Ctrl Pts',(-14.9311912107729,-54.3847111211312,
14.));
#65657=CARTESIAN_POINT('Ctrl Pts',(-14.9196049423273,-54.391231523474,14.));
#65658=CARTESIAN_POINT('Ctrl Pts',(-14.9079138627992,-54.3975910665321,
14.));
#65659=CARTESIAN_POINT('Ctrl Pts',(-14.8961220820674,-54.4037876495833,
14.));
#65660=CARTESIAN_POINT('Ctrl Pts',(-14.8869418707018,-54.4086118524283,
14.));
#65661=CARTESIAN_POINT('Ctrl Pts',(-14.8776989839247,-54.4133380017209,
14.));
#65662=CARTESIAN_POINT('Ctrl Pts',(-14.8684106168714,-54.4179577422776,
14.));
#65663=CARTESIAN_POINT('Ctrl Pts',(-14.8187084869932,-54.4426780126799,
14.));
#65664=CARTESIAN_POINT('Ctrl Pts',(-14.7676148803933,-54.464404589055,14.));
#65665=CARTESIAN_POINT('Ctrl Pts',(-14.7154497956283,-54.4830620982051,
14.));
#65666=CARTESIAN_POINT('Ctrl Pts',(-14.6635765838803,-54.501615215241,14.));
#65667=CARTESIAN_POINT('Ctrl Pts',(-14.6106426601789,-54.5171336375863,
14.));
#65668=CARTESIAN_POINT('Ctrl Pts',(-14.5569565025172,-54.5294926610513,
14.));
#65669=CARTESIAN_POINT('Ctrl Pts',(-14.5071457936645,-54.5409595222745,
14.));
#65670=CARTESIAN_POINT('Ctrl Pts',(-14.456686763942,-54.5497062605737,14.));
#65671=CARTESIAN_POINT('Ctrl Pts',(-14.4058341277,-54.5555924980414,14.));
#65672=CARTESIAN_POINT('Ctrl Pts',(-14.3927717853308,-54.557104475684,14.));
#65673=CARTESIAN_POINT('Ctrl Pts',(-14.3796790109819,-54.5584277519287,
14.));
#65674=CARTESIAN_POINT('Ctrl Pts',(-14.3665890681527,-54.5595574794671,
14.));
#65675=CARTESIAN_POINT('Ctrl Pts',(-14.313676726872,-54.5641240791723,14.));
#65676=CARTESIAN_POINT('Ctrl Pts',(-14.2607272248055,-54.565543985866,14.));
#65677=CARTESIAN_POINT('Ctrl Pts',(-14.2080224885386,-54.5637141509322,
14.));
#65678=CARTESIAN_POINT('Ctrl Pts',(-14.1571049407467,-54.5619463646896,
14.));
#65679=CARTESIAN_POINT('Ctrl Pts',(-14.1064149890402,-54.557145321735,14.));
#65680=CARTESIAN_POINT('Ctrl Pts',(-14.0562198243703,-54.5491721895645,
14.));
#65681=CARTESIAN_POINT('Ctrl Pts',(-14.0211056129848,-54.543594555737,14.));
#65682=CARTESIAN_POINT('Ctrl Pts',(-13.986233796236,-54.5364636409164,14.));
#65683=CARTESIAN_POINT('Ctrl Pts',(-13.9517030424607,-54.5277184245241,
14.));
#65684=CARTESIAN_POINT('Ctrl Pts',(-13.93222381495,-54.5227851392317,14.));
#65685=CARTESIAN_POINT('Ctrl Pts',(-13.9128532514771,-54.5173379031513,
14.));
#65686=CARTESIAN_POINT('Ctrl Pts',(-13.8936069362009,-54.5113866946539,
14.));
#65687=CARTESIAN_POINT('Origin',(-14.1292828945604,-53.2669068454841,19.1042117235887));
#65688=CARTESIAN_POINT('Ctrl Pts',(-13.3561844802682,-51.9293619476186,
17.8542117235887));
#65689=CARTESIAN_POINT('Ctrl Pts',(-13.3145289674606,-51.9530637836679,
17.8517311518799));
#65690=CARTESIAN_POINT('Ctrl Pts',(-12.8472204745978,-52.2501100679509,
17.8230820767121));
#65691=CARTESIAN_POINT('Ctrl Pts',(-12.3131148719809,-53.3266292410367,
17.7682644980854));
#65692=CARTESIAN_POINT('Ctrl Pts',(-13.177398497422,-54.8146003900027,17.6897589877086));
#65693=CARTESIAN_POINT('Ctrl Pts',(-14.8951536251653,-54.9146504373755,
17.6112534773319));
#65694=CARTESIAN_POINT('Ctrl Pts',(-15.9261572824593,-53.5369216264006,
17.5327479669551));
#65695=CARTESIAN_POINT('Ctrl Pts',(-15.3456319213627,-51.9170585592589,
17.4542424565783));
#65696=CARTESIAN_POINT('Ctrl Pts',(-14.0786429713653,-51.6067853756627,
17.3947303754562));
#65697=CARTESIAN_POINT('Ctrl Pts',(-13.4791850640252,-51.8598443884631,
17.361386797793));
#65698=CARTESIAN_POINT('Ctrl Pts',(-13.3591951473146,-51.9304670067727,
17.3542117235887));
#65699=CARTESIAN_POINT('Ctrl Pts',(-13.3599426557471,-51.9312965605688,
17.8957882764113));
#65700=CARTESIAN_POINT('Ctrl Pts',(-13.0649944461637,-52.1042822226529,
17.8781885106897));
#65701=CARTESIAN_POINT('Ctrl Pts',(-12.4640754788204,-52.7732237750949,
17.8344202415091));
#65702=CARTESIAN_POINT('Ctrl Pts',(-12.6330157688953,-54.2972115132025,
17.7644834688697));
#65703=CARTESIAN_POINT('Ctrl Pts',(-14.1627629159668,-55.0835833760402,
17.6859779584929));
#65704=CARTESIAN_POINT('Ctrl Pts',(-15.6633630152513,-54.2408836460551,
17.6074724481161));
#65705=CARTESIAN_POINT('Ctrl Pts',(-15.7877283921755,-52.5246154983424,
17.5289669377393));
#65706=CARTESIAN_POINT('Ctrl Pts',(-14.5628755318023,-51.5803972945988,
17.458405547171));
#65707=CARTESIAN_POINT('Ctrl Pts',(-13.6650283227152,-51.7575311866648,
17.4140126600617));
#65708=CARTESIAN_POINT('Ctrl Pts',(-13.3571987246687,-51.9320818411208,
17.3957882764113));
#65709=CARTESIAN_POINT('Ctrl Pts',(-13.8936870225526,-54.5092654229862,
18.));
#65710=CARTESIAN_POINT('Ctrl Pts',(-14.3022280845015,-54.5867395029208,
17.9738314965411));
#65711=CARTESIAN_POINT('Ctrl Pts',(-15.1949907864185,-54.306005850961,17.9214944896232));
#65712=CARTESIAN_POINT('Ctrl Pts',(-15.5848805170292,-52.9490991612648,
17.8429889792464));
#65713=CARTESIAN_POINT('Ctrl Pts',(-14.6665684258224,-51.8784501685123,
17.7644834688696));
#65714=CARTESIAN_POINT('Ctrl Pts',(-13.2677649070697,-52.0524087826961,
17.6859779584929));
#65715=CARTESIAN_POINT('Ctrl Pts',(-12.6409196641315,-53.3158497937513,
17.6074724481161));
#65716=CARTESIAN_POINT('Ctrl Pts',(-13.3492065366981,-54.5352532401981,
17.5289669377393));
#65717=CARTESIAN_POINT('Ctrl Pts',(-14.7569196663361,-54.6172449996945,
17.4504614273625));
#65718=CARTESIAN_POINT('Ctrl Pts',(-15.6018348475728,-53.488185970869,17.3719559169858));
#65719=CARTESIAN_POINT('Ctrl Pts',(-15.1260899874907,-52.160696114485,17.293450406609));
#65720=CARTESIAN_POINT('Ctrl Pts',(-13.7564048649609,-51.8252736441527,
17.2149448962322));
#65721=CARTESIAN_POINT('Ctrl Pts',(-12.7211156974588,-52.7827464099985,
17.1364393858554));
#65722=CARTESIAN_POINT('Ctrl Pts',(-12.9487092675231,-54.174423630146,17.0579338754786));
#65723=CARTESIAN_POINT('Ctrl Pts',(-14.2350668963379,-54.7522192803303,
16.9794283651019));
#65724=CARTESIAN_POINT('Ctrl Pts',(-15.4265561246117,-53.9979509037444,
16.900922854725));
#65725=CARTESIAN_POINT('Ctrl Pts',(-15.4546192812222,-52.5880650956991,
16.8224173443483));
#65726=CARTESIAN_POINT('Ctrl Pts',(-14.2940895544972,-51.7869805788023,
16.7439118339715));
#65727=CARTESIAN_POINT('Ctrl Pts',(-12.9857571502944,-52.3131291848103,
16.6654063235948));
#65728=CARTESIAN_POINT('Ctrl Pts',(-12.7029658920433,-53.6946482401116,
16.586900813218));
#65729=CARTESIAN_POINT('Ctrl Pts',(-13.6993295943645,-54.69255865938,16.5083953028412));
#65730=CARTESIAN_POINT('Ctrl Pts',(-15.0812856557068,-54.4119106312665,
16.4298897924644));
#65731=CARTESIAN_POINT('Ctrl Pts',(-15.6094629994388,-53.1043959909962,
16.3513842820876));
#65732=CARTESIAN_POINT('Ctrl Pts',(-14.8101796402302,-51.9426249466013,
16.2728787717108));
#65733=CARTESIAN_POINT('Ctrl Pts',(-13.4002518899393,-51.9685013930707,
16.1943732613341));
#65734=CARTESIAN_POINT('Ctrl Pts',(-12.6441364773908,-53.1588187166123,
16.1158677509573));
#65735=CARTESIAN_POINT('Ctrl Pts',(-13.2199356785565,-54.4460720440219,
16.0373622405805));
#65736=CARTESIAN_POINT('Ctrl Pts',(-14.6112590818024,-54.6758219881874,
15.9588567302038));
#65737=CARTESIAN_POINT('Ctrl Pts',(-15.5703347818477,-53.6420233374598,
15.8803512198269));
#65738=CARTESIAN_POINT('Ctrl Pts',(-15.2370408904378,-52.2718112986816,
15.8018457094502));
#65739=CARTESIAN_POINT('Ctrl Pts',(-13.9102832927596,-51.7940246036041,
15.7233401990734));
#65740=CARTESIAN_POINT('Ctrl Pts',(-12.7799297446004,-52.6371537182599,
15.6448346886966));
#65741=CARTESIAN_POINT('Ctrl Pts',(-12.8597081799673,-54.0450604100449,
15.5663291783198));
#65742=CARTESIAN_POINT('Ctrl Pts',(-14.0780714025733,-54.7551004833527,
15.4878236679431));
#65743=CARTESIAN_POINT('Ctrl Pts',(-15.3423623071066,-54.1304931269541,
15.4093181575663));
#65744=CARTESIAN_POINT('Ctrl Pts',(-15.5187347583226,-52.7314010536376,
15.3308126471895));
#65745=CARTESIAN_POINT('Ctrl Pts',(-14.4490137393998,-51.8125633237516,
15.2523071368127));
#65746=CARTESIAN_POINT('Ctrl Pts',(-13.0925505105556,-52.1980154020928,
15.1738016264359));
#65747=CARTESIAN_POINT('Ctrl Pts',(-12.6658535045584,-53.5420748131919,
15.0952961160591));
#65748=CARTESIAN_POINT('Ctrl Pts',(-13.551594819097,-54.6393568979555,15.0167906056824));
#65749=CARTESIAN_POINT('Ctrl Pts',(-14.9554204274106,-54.5057934526205,
14.9382850953056));
#65750=CARTESIAN_POINT('Ctrl Pts',(-15.6183464700209,-53.2611664293564,
14.8597795849288));
#65751=CARTESIAN_POINT('Ctrl Pts',(-14.9458444656461,-52.0216887907143,
14.7812740745521));
#65752=CARTESIAN_POINT('Ctrl Pts',(-13.5410315037528,-51.8989497980972,
14.7027685641753));
#65753=CARTESIAN_POINT('Ctrl Pts',(-12.6637746137877,-53.0030322708737,
14.6242630537985));
#65754=CARTESIAN_POINT('Ctrl Pts',(-13.1008239433931,-54.3437535140763,
14.5457575434217));
#65755=CARTESIAN_POINT('Ctrl Pts',(-14.4602125392812,-54.7187536954986,
14.4672520330449));
#65756=CARTESIAN_POINT('Ctrl Pts',(-15.5228300373051,-53.7916614633287,
14.3887465226681));
#65757=CARTESIAN_POINT('Ctrl Pts',(-15.3356521111637,-52.3940408681935,
14.3102410122914));
#65758=CARTESIAN_POINT('Ctrl Pts',(-14.0666325655589,-51.7790575741688,
14.2317355019146));
#65759=CARTESIAN_POINT('Ctrl Pts',(-12.8536802704289,-52.4987553418111,
14.1532299915378));
#65760=CARTESIAN_POINT('Ctrl Pts',(-12.7849592886011,-53.9066581474695,
14.074724481161));
#65761=CARTESIAN_POINT('Ctrl Pts',(-13.9213697617029,-54.7422164034654,
13.9962189707842));
#65762=CARTESIAN_POINT('Ctrl Pts',(-15.2452696789899,-54.2518096584208,
13.9177134604075));
#65763=CARTESIAN_POINT('Ctrl Pts',(-15.4583606841261,-53.3405309695408,
13.8653764534896));
#65764=CARTESIAN_POINT('Ctrl Pts',(-15.3505106014235,-52.9389386488708,
13.8392079500307));
#65765=CARTESIAN_POINT('Ctrl Pts',(-13.8763907393434,-54.6004732426341,
18.0535973499898));
#65766=CARTESIAN_POINT('Ctrl Pts',(-14.3149248646251,-54.6836350861806,
18.0274288465308));
#65767=CARTESIAN_POINT('Ctrl Pts',(-15.2732297867829,-54.3822913585465,
17.975091839613));
#65768=CARTESIAN_POINT('Ctrl Pts',(-15.6917432922651,-52.9257672935819,
17.8965863292362));
#65769=CARTESIAN_POINT('Ctrl Pts',(-14.7060132710725,-51.7765165492856,
17.8180808188594));
#65770=CARTESIAN_POINT('Ctrl Pts',(-13.2045165191651,-51.9632463441864,
17.7395753084827));
#65771=CARTESIAN_POINT('Ctrl Pts',(-12.5316514000813,-53.3194429428464,
17.6610697981059));
#65772=CARTESIAN_POINT('Ctrl Pts',(-13.2919371902728,-54.6283689567997,
17.5825642877291));
#65773=CARTESIAN_POINT('Ctrl Pts',(-14.8029976526125,-54.7163801455882,
17.5040587773523));
#65774=CARTESIAN_POINT('Ctrl Pts',(-15.7099423258683,-53.5044311893795,
17.4255532669755));
#65775=CARTESIAN_POINT('Ctrl Pts',(-15.1992706321147,-52.0794835960763,
17.3470477565988));
#65776=CARTESIAN_POINT('Ctrl Pts',(-13.7290300050048,-51.7194360676216,
17.268542246222));
#65777=CARTESIAN_POINT('Ctrl Pts',(-12.6177350293705,-52.7472017464206,
17.1900367358452));
#65778=CARTESIAN_POINT('Ctrl Pts',(-12.8620373932302,-54.2410490221397,
17.1115312254684));
#65779=CARTESIAN_POINT('Ctrl Pts',(-14.2428330343358,-54.8612635700639,
17.0330257150916));
#65780=CARTESIAN_POINT('Ctrl Pts',(-15.5217955063355,-54.0516205413417,
16.9545202047148));
#65781=CARTESIAN_POINT('Ctrl Pts',(-15.5519189210496,-52.5382278932962,
16.8760146943381));
#65782=CARTESIAN_POINT('Ctrl Pts',(-14.3061888440168,-51.6783317148849,
16.7975091839613));
#65783=CARTESIAN_POINT('Ctrl Pts',(-12.901805148244,-52.2431075481956,16.7190036735845));
#65784=CARTESIAN_POINT('Ctrl Pts',(-12.5982527550455,-53.7260508968676,
16.6404981632077));
#65785=CARTESIAN_POINT('Ctrl Pts',(-13.6677645504461,-54.7972229615204,
16.561992652831));
#65786=CARTESIAN_POINT('Ctrl Pts',(-15.1511769879803,-54.4959711438118,
16.4834871424542));
#65787=CARTESIAN_POINT('Ctrl Pts',(-15.7181304989006,-53.0924652481532,
16.4049816320774));
#65788=CARTESIAN_POINT('Ctrl Pts',(-14.8601677102629,-51.8454027220491,
16.3264761217006));
#65789=CARTESIAN_POINT('Ctrl Pts',(-13.3467300407797,-51.8731788891832,
16.2479706113238));
#65790=CARTESIAN_POINT('Ctrl Pts',(-12.5351043758535,-53.1508834210038,
16.1694651009471));
#65791=CARTESIAN_POINT('Ctrl Pts',(-13.1531759053504,-54.5326405184631,
16.0909595905703));
#65792=CARTESIAN_POINT('Ctrl Pts',(-14.6466433886818,-54.7792575667409,
16.0124540801935));
#65793=CARTESIAN_POINT('Ctrl Pts',(-15.676129681178,-53.6695625342478,15.9339485698167));
#65794=CARTESIAN_POINT('Ctrl Pts',(-15.3183670013781,-52.1987563073057,
15.8554430594399));
#65795=CARTESIAN_POINT('Ctrl Pts',(-13.8942054255916,-51.6858928771342,
15.7769375490632));
#65796=CARTESIAN_POINT('Ctrl Pts',(-12.680866912845,-52.5909203596381,15.6984320386864));
#65797=CARTESIAN_POINT('Ctrl Pts',(-12.7665022861979,-54.1021885944999,
15.6199265283096));
#65798=CARTESIAN_POINT('Ctrl Pts',(-14.0743117082228,-54.8643562967563,
15.5414210179328));
#65799=CARTESIAN_POINT('Ctrl Pts',(-15.431420595335,-54.1938933587688,15.4629155075561));
#65800=CARTESIAN_POINT('Ctrl Pts',(-15.6207414392394,-52.6920868680494,
15.3844099971793));
#65801=CARTESIAN_POINT('Ctrl Pts',(-14.4724867960198,-51.7057926183865,
15.3059044868025));
#65802=CARTESIAN_POINT('Ctrl Pts',(-13.0164387486087,-52.1195426811267,
15.2273989764257));
#65803=CARTESIAN_POINT('Ctrl Pts',(-12.5584157597012,-53.5622762838672,
15.1488934660489));
#65804=CARTESIAN_POINT('Ctrl Pts',(-13.5091838189608,-54.7401153900112,
15.0703879556722));
#65805=CARTESIAN_POINT('Ctrl Pts',(-15.0160713573958,-54.5967463773831,
14.9918824452954));
#65806=CARTESIAN_POINT('Ctrl Pts',(-15.727666149938,-53.2607449964075,14.9133769349186));
#65807=CARTESIAN_POINT('Ctrl Pts',(-15.0057923758998,-51.9302710423938,
14.8348714245418));
#65808=CARTESIAN_POINT('Ctrl Pts',(-13.4978449972707,-51.7985211602437,
14.756365914165));
#65809=CARTESIAN_POINT('Ctrl Pts',(-12.5561842470564,-52.9836599052406,
14.6778604037882));
#65810=CARTESIAN_POINT('Ctrl Pts',(-13.0253195759487,-54.4228102683146,
14.5993548934115));
#65811=CARTESIAN_POINT('Ctrl Pts',(-14.4845077563775,-54.8253411075794,
14.5208493830347));
#65812=CARTESIAN_POINT('Ctrl Pts',(-15.6251373733416,-53.830186350918,14.4423438726579));
#65813=CARTESIAN_POINT('Ctrl Pts',(-15.4242177700075,-52.3299593670269,
14.3638383622811));
#65814=CARTESIAN_POINT('Ctrl Pts',(-14.0620330883935,-51.6698270424536,
14.2853328519044));
#65815=CARTESIAN_POINT('Ctrl Pts',(-12.7600318373669,-52.4423614591769,
14.2068273415276));
#65816=CARTESIAN_POINT('Ctrl Pts',(-12.6862657010804,-53.9536255226119,
14.1283218311508));
#65817=CARTESIAN_POINT('Ctrl Pts',(-13.9061058082296,-54.8505263314733,
14.049816320774));
#65818=CARTESIAN_POINT('Ctrl Pts',(-15.3271999068701,-54.3241163497093,
13.9713108103972));
#65819=CARTESIAN_POINT('Ctrl Pts',(-15.5559349992425,-53.3459360884415,
13.9189738034794));
#65820=CARTESIAN_POINT('Ctrl Pts',(-15.4401670971033,-52.9148608466415,
13.8928053000205));
#65821=CARTESIAN_POINT('Ctrl Pts',(-13.8590944561342,-54.691681062282,18.1071946999795));
#65822=CARTESIAN_POINT('Ctrl Pts',(-14.3276216447486,-54.7805306694404,
18.0810261965206));
#65823=CARTESIAN_POINT('Ctrl Pts',(-15.3514687871474,-54.4585768661319,
18.0286891896028));
#65824=CARTESIAN_POINT('Ctrl Pts',(-15.798606067501,-52.902435425899,17.950183679226));
#65825=CARTESIAN_POINT('Ctrl Pts',(-14.7454581163227,-51.6745829300588,
17.8716781688492));
#65826=CARTESIAN_POINT('Ctrl Pts',(-13.1412681312604,-51.8740839056767,
17.7931726584724));
#65827=CARTESIAN_POINT('Ctrl Pts',(-12.4223831360311,-53.3230360919416,
17.7146671480956));
#65828=CARTESIAN_POINT('Ctrl Pts',(-13.2346678438474,-54.7214846734011,
17.6361616377189));
#65829=CARTESIAN_POINT('Ctrl Pts',(-14.849075638889,-54.8155152914819,17.5576561273421));
#65830=CARTESIAN_POINT('Ctrl Pts',(-15.8180498041638,-53.52067640789,17.4791506169653));
#65831=CARTESIAN_POINT('Ctrl Pts',(-15.2724512767387,-51.9982710776676,
17.4006451065885));
#65832=CARTESIAN_POINT('Ctrl Pts',(-13.7016551450487,-51.6135984910905,
17.3221395962117));
#65833=CARTESIAN_POINT('Ctrl Pts',(-12.5143543612823,-52.7116570828427,
17.243634085835));
#65834=CARTESIAN_POINT('Ctrl Pts',(-12.7753655189374,-54.3076744141334,
17.1651285754582));
#65835=CARTESIAN_POINT('Ctrl Pts',(-14.2505991723337,-54.9703078597976,
17.0866230650814));
#65836=CARTESIAN_POINT('Ctrl Pts',(-15.6170348880593,-54.1052901789391,
17.0081175547046));
#65837=CARTESIAN_POINT('Ctrl Pts',(-15.6492185608771,-52.4883906908934,
16.9296120443279));
#65838=CARTESIAN_POINT('Ctrl Pts',(-14.3182881335364,-51.5696828509675,
16.851106533951));
#65839=CARTESIAN_POINT('Ctrl Pts',(-12.8178531461936,-52.173085911581,16.7726010235743));
#65840=CARTESIAN_POINT('Ctrl Pts',(-12.4935396180478,-53.7574535536235,
16.6940955131975));
#65841=CARTESIAN_POINT('Ctrl Pts',(-13.6361995065277,-54.9018872636609,
16.6155900028207));
#65842=CARTESIAN_POINT('Ctrl Pts',(-15.2210683202537,-54.580031656357,16.5370844924439));
#65843=CARTESIAN_POINT('Ctrl Pts',(-15.8267979983625,-53.0805345053102,
16.4585789820672));
#65844=CARTESIAN_POINT('Ctrl Pts',(-14.9101557802956,-51.7481804974968,
16.3800734716904));
#65845=CARTESIAN_POINT('Ctrl Pts',(-13.2932081916201,-51.7778563852958,
16.3015679613136));
#65846=CARTESIAN_POINT('Ctrl Pts',(-12.4260722743163,-53.1429481253953,
16.2230624509368));
#65847=CARTESIAN_POINT('Ctrl Pts',(-13.0864161321444,-54.6192089929043,
16.14455694056));
#65848=CARTESIAN_POINT('Ctrl Pts',(-14.6820276955612,-54.8826931452944,
16.0660514301833));
#65849=CARTESIAN_POINT('Ctrl Pts',(-15.7819245805084,-53.6971017310358,
15.9875459198065));
#65850=CARTESIAN_POINT('Ctrl Pts',(-15.3996931123184,-52.1257013159298,
15.9090404094297));
#65851=CARTESIAN_POINT('Ctrl Pts',(-13.8781275584237,-51.5777611506643,
15.8305348990529));
#65852=CARTESIAN_POINT('Ctrl Pts',(-12.5818040810897,-52.5446870010162,
15.7520293886761));
#65853=CARTESIAN_POINT('Ctrl Pts',(-12.6732963924285,-54.1593167789549,
15.6735238782994));
#65854=CARTESIAN_POINT('Ctrl Pts',(-14.0705520138724,-54.9736121101599,
15.5950183679226));
#65855=CARTESIAN_POINT('Ctrl Pts',(-15.5204788835633,-54.2572935905836,
15.5165128575458));
#65856=CARTESIAN_POINT('Ctrl Pts',(-15.7227481201562,-52.6527726824611,
15.438007347169));
#65857=CARTESIAN_POINT('Ctrl Pts',(-14.4959598526397,-51.5990219130214,
15.3595018367922));
#65858=CARTESIAN_POINT('Ctrl Pts',(-12.9403269866619,-52.0410699601608,
15.2809963264155));
#65859=CARTESIAN_POINT('Ctrl Pts',(-12.4509780148441,-53.5824777545425,
15.2024908160387));
#65860=CARTESIAN_POINT('Ctrl Pts',(-13.4667728188247,-54.8408738820669,
15.1239853056619));
#65861=CARTESIAN_POINT('Ctrl Pts',(-15.076722287381,-54.6876993021459,15.0454797952851));
#65862=CARTESIAN_POINT('Ctrl Pts',(-15.8369858298552,-53.2603235634587,
14.9669742849083));
#65863=CARTESIAN_POINT('Ctrl Pts',(-15.0657402861535,-51.8388532940734,
14.8884687745316));
#65864=CARTESIAN_POINT('Ctrl Pts',(-13.4546584907886,-51.6980925223903,
14.8099632641548));
#65865=CARTESIAN_POINT('Ctrl Pts',(-12.4485938803251,-52.9642875396075,
14.731457753778));
#65866=CARTESIAN_POINT('Ctrl Pts',(-12.9498152085044,-54.5018670225529,
14.6529522434012));
#65867=CARTESIAN_POINT('Ctrl Pts',(-14.5088029734737,-54.9319285196604,
14.5744467330245));
#65868=CARTESIAN_POINT('Ctrl Pts',(-15.7274447093781,-53.8687112385072,
14.4959412226477));
#65869=CARTESIAN_POINT('Ctrl Pts',(-15.5127834288513,-52.2658778658603,
14.4174357122709));
#65870=CARTESIAN_POINT('Ctrl Pts',(-14.0574336112281,-51.5605965107385,
14.3389302018941));
#65871=CARTESIAN_POINT('Ctrl Pts',(-12.666383404305,-52.3859675765427,14.2604246915173));
#65872=CARTESIAN_POINT('Ctrl Pts',(-12.5875721135598,-54.0005928977544,
14.1819191811406));
#65873=CARTESIAN_POINT('Ctrl Pts',(-13.8908418547563,-54.9588362594811,
14.1034136707638));
#65874=CARTESIAN_POINT('Ctrl Pts',(-15.4091301347503,-54.3964230409977,
14.024908160387));
#65875=CARTESIAN_POINT('Ctrl Pts',(-15.6535093143589,-53.3513412073421,
13.9725711534692));
#65876=CARTESIAN_POINT('Ctrl Pts',(-15.5298235927831,-52.8907830444122,
13.9464026500102));
#65877=CARTESIAN_POINT('Ctrl Pts',(-13.841798172925,-54.7828888819299,18.1607920499693));
#65878=CARTESIAN_POINT('Ctrl Pts',(-14.3403184248721,-54.8774262527002,
18.1346235465104));
#65879=CARTESIAN_POINT('Ctrl Pts',(-15.4297077875118,-54.5348623737173,
18.0822865395925));
#65880=CARTESIAN_POINT('Ctrl Pts',(-15.905468842737,-52.8791035582161,18.0037810292158));
#65881=CARTESIAN_POINT('Ctrl Pts',(-14.7849029615728,-51.572649310832,17.925275518839));
#65882=CARTESIAN_POINT('Ctrl Pts',(-13.0780197433558,-51.7849214671671,
17.8467700084622));
#65883=CARTESIAN_POINT('Ctrl Pts',(-12.3131148719809,-53.3266292410367,
17.7682644980854));
#65884=CARTESIAN_POINT('Ctrl Pts',(-13.177398497422,-54.8146003900027,17.6897589877086));
#65885=CARTESIAN_POINT('Ctrl Pts',(-14.8951536251653,-54.9146504373755,
17.6112534773319));
#65886=CARTESIAN_POINT('Ctrl Pts',(-15.9261572824593,-53.5369216264006,
17.5327479669551));
#65887=CARTESIAN_POINT('Ctrl Pts',(-15.3456319213627,-51.9170585592589,
17.4542424565783));
#65888=CARTESIAN_POINT('Ctrl Pts',(-13.6742802850926,-51.5077609145594,
17.3757369462015));
#65889=CARTESIAN_POINT('Ctrl Pts',(-12.410973693194,-52.6761124192647,17.2972314358248));
#65890=CARTESIAN_POINT('Ctrl Pts',(-12.6886936446445,-54.3742998061273,
17.2187259254479));
#65891=CARTESIAN_POINT('Ctrl Pts',(-14.2583653103316,-55.0793521495312,
17.1402204150712));
#65892=CARTESIAN_POINT('Ctrl Pts',(-15.7122742697832,-54.1589598165365,
17.0617149046944));
#65893=CARTESIAN_POINT('Ctrl Pts',(-15.7465182007045,-52.4385534884905,
16.9832093943176));
#65894=CARTESIAN_POINT('Ctrl Pts',(-14.3303874230559,-51.4610339870501,
16.9047038839408));
#65895=CARTESIAN_POINT('Ctrl Pts',(-12.7339011441433,-52.1030642749663,
16.8261983735641));
#65896=CARTESIAN_POINT('Ctrl Pts',(-12.38882648105,-53.7888562103795,16.7476928631873));
#65897=CARTESIAN_POINT('Ctrl Pts',(-13.6046344626093,-55.0065515658013,
16.6691873528105));
#65898=CARTESIAN_POINT('Ctrl Pts',(-15.2909596525272,-54.6640921689023,
16.5906818424337));
#65899=CARTESIAN_POINT('Ctrl Pts',(-15.9354654978244,-53.0686037624671,
16.5121763320569));
#65900=CARTESIAN_POINT('Ctrl Pts',(-14.9601438503283,-51.6509582729447,
16.4336708216802));
#65901=CARTESIAN_POINT('Ctrl Pts',(-13.2396863424605,-51.6825338814083,
16.3551653113034));
#65902=CARTESIAN_POINT('Ctrl Pts',(-12.317040172779,-53.1350128297868,16.2766598009266));
#65903=CARTESIAN_POINT('Ctrl Pts',(-13.0196563589383,-54.7057774673455,
16.1981542905498));
#65904=CARTESIAN_POINT('Ctrl Pts',(-14.7174120024405,-54.986128723848,16.1196487801731));
#65905=CARTESIAN_POINT('Ctrl Pts',(-15.8877194798387,-53.7246409278238,
16.0411432697963));
#65906=CARTESIAN_POINT('Ctrl Pts',(-15.4810192232586,-52.0526463245539,
15.9626377594195));
#65907=CARTESIAN_POINT('Ctrl Pts',(-13.8620496912558,-51.4696294241944,
15.8841322490427));
#65908=CARTESIAN_POINT('Ctrl Pts',(-12.4827412493343,-52.4984536423944,
15.8056267386659));
#65909=CARTESIAN_POINT('Ctrl Pts',(-12.5800904986592,-54.21644496341,15.7271212282892));
#65910=CARTESIAN_POINT('Ctrl Pts',(-14.0667923195219,-55.0828679235634,
15.6486157179124));
#65911=CARTESIAN_POINT('Ctrl Pts',(-15.6095371717916,-54.3206938223985,
15.5701102075356));
#65912=CARTESIAN_POINT('Ctrl Pts',(-15.8247548010729,-52.6134584968727,
15.4916046971588));
#65913=CARTESIAN_POINT('Ctrl Pts',(-14.5194329092597,-51.4922512076563,
15.413099186782));
#65914=CARTESIAN_POINT('Ctrl Pts',(-12.864215224715,-51.9625972391948,15.3345936764052));
#65915=CARTESIAN_POINT('Ctrl Pts',(-12.343540269987,-53.6026792252177,15.2560881660285));
#65916=CARTESIAN_POINT('Ctrl Pts',(-13.4243618186885,-54.9416323741227,
15.1775826556517));
#65917=CARTESIAN_POINT('Ctrl Pts',(-15.1373732173662,-54.7786522269085,
15.0990771452749));
#65918=CARTESIAN_POINT('Ctrl Pts',(-15.9463055097723,-53.2599021305098,
15.0205716348981));
#65919=CARTESIAN_POINT('Ctrl Pts',(-15.1256881964072,-51.7474355457531,
14.9420661245214));
#65920=CARTESIAN_POINT('Ctrl Pts',(-13.4114719843065,-51.5976638845367,
14.8635606141446));
#65921=CARTESIAN_POINT('Ctrl Pts',(-12.3410035135938,-52.9449151739745,
14.7850551037678));
#65922=CARTESIAN_POINT('Ctrl Pts',(-12.8743108410601,-54.5809237767912,
14.706549593391));
#65923=CARTESIAN_POINT('Ctrl Pts',(-14.53309819057,-55.0385159317414,14.6280440830142));
#65924=CARTESIAN_POINT('Ctrl Pts',(-15.8297520454146,-53.9072361260964,
14.5495385726375));
#65925=CARTESIAN_POINT('Ctrl Pts',(-15.6013490876951,-52.2017963646938,
14.4710330622607));
#65926=CARTESIAN_POINT('Ctrl Pts',(-14.0528341340627,-51.4513659790234,
14.3925275518839));
#65927=CARTESIAN_POINT('Ctrl Pts',(-12.572734971243,-52.3295736939085,14.3140220415071));
#65928=CARTESIAN_POINT('Ctrl Pts',(-12.4888785260391,-54.0475602728968,
14.2355165311304));
#65929=CARTESIAN_POINT('Ctrl Pts',(-13.8755779012831,-55.0671461874891,
14.1570110207535));
#65930=CARTESIAN_POINT('Ctrl Pts',(-15.4910603626305,-54.4687297322861,
14.0785055103768));
#65931=CARTESIAN_POINT('Ctrl Pts',(-15.7510836294753,-53.3567463262428,
14.0261685034589));
#65932=CARTESIAN_POINT('Ctrl Pts',(-15.619480088463,-52.8667052421829,14.));
#65933=CARTESIAN_POINT('Ctrl Pts',(-13.498190246218,-52.1716844371558,17.1934196736194));
#65934=CARTESIAN_POINT('Ctrl Pts',(-13.5965228772488,-52.1138086750997,
17.2005947478237));
#65935=CARTESIAN_POINT('Ctrl Pts',(-13.7022352452507,-52.0691825768203,
17.2077698220279));
#65936=CARTESIAN_POINT('Ctrl Pts',(-13.8121375241322,-52.0407561835157,
17.2149448962322));
#65937=CARTESIAN_POINT('Ctrl Pts',(-14.2129665724708,-51.9370811342635,
17.2411133996911));
#65938=CARTESIAN_POINT('Ctrl Pts',(-14.6695282799808,-52.0488886243742,
17.26728190315));
#65939=CARTESIAN_POINT('Ctrl Pts',(-14.9770999437494,-52.3260406788269,
17.293450406609));
#65940=CARTESIAN_POINT('Ctrl Pts',(-15.2846716075181,-52.6031927332796,
17.3196189100679));
#65941=CARTESIAN_POINT('Ctrl Pts',(-15.4432532275454,-53.0456893520743,
17.3457874135268));
#65942=CARTESIAN_POINT('Ctrl Pts',(-15.3817248406863,-53.4551141662759,
17.3719559169858));
#65943=CARTESIAN_POINT('Ctrl Pts',(-15.3201964538272,-53.8645389804775,
17.3981244204447));
#65944=CARTESIAN_POINT('Ctrl Pts',(-15.0385580600817,-54.240891990086,17.4242929239036));
#65945=CARTESIAN_POINT('Ctrl Pts',(-14.6631200082692,-54.4154032016409,
17.4504614273625));
#65946=CARTESIAN_POINT('Ctrl Pts',(-14.2876819564568,-54.5899144131957,
17.4766299308215));
#65947=CARTESIAN_POINT('Ctrl Pts',(-13.8184442465775,-54.5625838266969,
17.5027984342804));
#65948=CARTESIAN_POINT('Ctrl Pts',(-13.4657775795434,-54.3456846257064,
17.5289669377393));
#65949=CARTESIAN_POINT('Ctrl Pts',(-13.1131109125093,-54.1287854247158,
17.5551354411982));
#65950=CARTESIAN_POINT('Ctrl Pts',(-12.8770152883204,-53.7223176092336,
17.5813039446572));
#65951=CARTESIAN_POINT('Ctrl Pts',(-12.8634416833823,-53.3085101996499,
17.6074724481161));
#65952=CARTESIAN_POINT('Ctrl Pts',(-12.8498680784442,-52.8947027900662,
17.633640951575));
#65953=CARTESIAN_POINT('Ctrl Pts',(-13.058816492757,-52.4735557863811,17.659809455034));
#65954=CARTESIAN_POINT('Ctrl Pts',(-13.3964246197054,-52.2339891821747,
17.6859779584929));
#65955=CARTESIAN_POINT('Ctrl Pts',(-13.4284272586679,-52.2112801211956,
17.6884585302017));
#65956=CARTESIAN_POINT('Ctrl Pts',(-13.46158597893,-52.1902026642355,17.6909391019106));
#65957=CARTESIAN_POINT('Ctrl Pts',(-13.495722982135,-52.1707788329429,17.6934196736194));
#65958=CARTESIAN_POINT('Ctrl Pts',(-15.2209662466057,-52.1764590205667,
18.));
#65959=CARTESIAN_POINT('Ctrl Pts',(-14.8623799894179,-51.8174664687921,
17.9738314965411));
#65960=CARTESIAN_POINT('Ctrl Pts',(-13.7693646387388,-51.4866597864568,
17.9214944896232));
#65961=CARTESIAN_POINT('Ctrl Pts',(-12.4433767107148,-52.5865029592796,
17.8429889792464));
#65962=CARTESIAN_POINT('Ctrl Pts',(-12.6330157688953,-54.2972115132025,
17.7644834688697));
#65963=CARTESIAN_POINT('Ctrl Pts',(-14.1627629159668,-55.0835833760402,
17.6859779584929));
#65964=CARTESIAN_POINT('Ctrl Pts',(-15.6633630152513,-54.2408836460551,
17.6074724481161));
#65965=CARTESIAN_POINT('Ctrl Pts',(-15.7877283921755,-52.5246154983424,
17.5289669377393));
#65966=CARTESIAN_POINT('Ctrl Pts',(-14.4249760687641,-51.4740929477669,
17.4504614273625));
#65967=CARTESIAN_POINT('Ctrl Pts',(-12.7969322124135,-52.0313881696841,
17.3719559169858));
#65968=CARTESIAN_POINT('Ctrl Pts',(-12.3638250796578,-53.6967359986948,
17.293450406609));
#65969=CARTESIAN_POINT('Ctrl Pts',(-13.5139962436503,-54.9765978264216,
17.2149448962322));
#65970=CARTESIAN_POINT('Ctrl Pts',(-15.2159841085892,-54.7231706136822,
17.1364393858554));
#65971=CARTESIAN_POINT('Ctrl Pts',(-15.9433860453713,-53.1637302055401,
17.0579338754786));
#65972=CARTESIAN_POINT('Ctrl Pts',(-15.043860342301,-51.6968216692226,16.9794283651019));
#65973=CARTESIAN_POINT('Ctrl Pts',(-13.3241182586501,-51.6380025442003,
16.9009228547251));
#65974=CARTESIAN_POINT('Ctrl Pts',(-12.3264677464456,-53.0400236709193,
16.8224173443483));
#65975=CARTESIAN_POINT('Ctrl Pts',(-12.9456243299004,-54.6455189484075,
16.7439118339715));
#65976=CARTESIAN_POINT('Ctrl Pts',(-14.626314246609,-55.0146421540478,16.6654063235948));
#65977=CARTESIAN_POINT('Ctrl Pts',(-15.8612545351151,-53.8163547667627,
16.586900813218));
#65978=CARTESIAN_POINT('Ctrl Pts',(-15.5429215283994,-52.1253094303059,
16.5083953028412));
#65979=CARTESIAN_POINT('Ctrl Pts',(-13.9568037640838,-51.4580757912425,
16.4298897924644));
#65980=CARTESIAN_POINT('Ctrl Pts',(-12.5253693960519,-52.413044846331,16.3513842820876));
#65981=CARTESIAN_POINT('Ctrl Pts',(-12.5323627785853,-54.1337776405725,
16.2728787717109));
#65982=CARTESIAN_POINT('Ctrl Pts',(-13.9715120885842,-55.0770800976454,
16.1943732613341));
#65983=CARTESIAN_POINT('Ctrl Pts',(-15.5521540067467,-54.3969761475115,
16.1158677509573));
#65984=CARTESIAN_POINT('Ctrl Pts',(-15.8567312853938,-52.7033991815804,
16.0373622405805));
#65985=CARTESIAN_POINT('Ctrl Pts',(-14.612091779025,-51.5151892852255,15.9588567302037));
#65986=CARTESIAN_POINT('Ctrl Pts',(-12.934457787186,-51.8979613415929,15.880351219827));
#65987=CARTESIAN_POINT('Ctrl Pts',(-12.3283713567552,-53.5084362707541,
15.8018457094502));
#65988=CARTESIAN_POINT('Ctrl Pts',(-13.3373852079754,-54.9023018690979,
15.7233401990734));
#65989=CARTESIAN_POINT('Ctrl Pts',(-15.0565917302206,-54.8295063313936,
15.6448346886966));
#65990=CARTESIAN_POINT('Ctrl Pts',(-15.9441656443073,-53.3553344251958,
15.5663291783198));
#65991=CARTESIAN_POINT('Ctrl Pts',(-15.2041095597138,-51.8018585649929,
15.4878236679431));
#65992=CARTESIAN_POINT('Ctrl Pts',(-13.5001233739826,-51.5622728287798,
15.4093181575663));
#65993=CARTESIAN_POINT('Ctrl Pts',(-12.3603823942099,-52.8514434111319,
15.3308126471895));
#65994=CARTESIAN_POINT('Ctrl Pts',(-12.8070334555363,-54.5132114643009,
15.2523071368127));
#65995=CARTESIAN_POINT('Ctrl Pts',(-14.4395092097517,-55.0572639347494,
15.1738016264359));
#65996=CARTESIAN_POINT('Ctrl Pts',(-15.7937667074069,-53.9956815464662,
15.0952961160592));
#65997=CARTESIAN_POINT('Ctrl Pts',(-15.6552753932384,-52.280516797303,15.0167906056824));
#65998=CARTESIAN_POINT('Ctrl Pts',(-14.14823804594,-51.4499698581624,14.9382850953056));
#65999=CARTESIAN_POINT('Ctrl Pts',(-12.6242006263839,-52.248895679213,14.8597795849288));
#66000=CARTESIAN_POINT('Ctrl Pts',(-12.4499580614657,-53.9607971579716,
14.781274074552));
#66001=CARTESIAN_POINT('Ctrl Pts',(-13.7817713167744,-55.0504032414555,
14.7027685641753));
#66002=CARTESIAN_POINT('Ctrl Pts',(-15.4252464910755,-54.5405234556122,
14.6242630537985));
#66003=CARTESIAN_POINT('Ctrl Pts',(-15.9064600587524,-52.8884418877605,
14.5457575434217));
#66004=CARTESIAN_POINT('Ctrl Pts',(-14.7938803736306,-51.575760805285,14.4672520330449));
#66005=CARTESIAN_POINT('Ctrl Pts',(-13.0852305278661,-51.7797717538672,
14.3887465226681));
#66006=CARTESIAN_POINT('Ctrl Pts',(-12.312999126503,-53.317416116839,14.3102410122914));
#66007=CARTESIAN_POINT('Ctrl Pts',(-13.1694776941513,-54.8098931066082,
14.2317355019146));
#66008=CARTESIAN_POINT('Ctrl Pts',(-14.8870885705588,-54.9183199028175,
14.1532299915378));
#66009=CARTESIAN_POINT('Ctrl Pts',(-15.9243621047065,-53.5462518811827,
14.074724481161));
#66010=CARTESIAN_POINT('Ctrl Pts',(-15.3532243372684,-51.9225867742538,
13.9962189707843));
#66011=CARTESIAN_POINT('Ctrl Pts',(-13.681410943509,-51.5067274632874,13.9177134604075));
#66012=CARTESIAN_POINT('Ctrl Pts',(-12.8400499397792,-52.2788850115251,
13.8653764534896));
#66013=CARTESIAN_POINT('Ctrl Pts',(-12.6726615784997,-52.7578848993975,
13.8392079500307));
#66014=CARTESIAN_POINT('Ctrl Pts',(-15.1552860103679,-52.2420649223251,
18.0535973499898));
#66015=CARTESIAN_POINT('Ctrl Pts',(-14.8182738021382,-51.9046708638902,
18.0274288465308));
#66016=CARTESIAN_POINT('Ctrl Pts',(-13.7910188263055,-51.5937668951064,
17.975091839613));
#66017=CARTESIAN_POINT('Ctrl Pts',(-12.5448078777489,-52.6274389027464,
17.8965863292362));
#66018=CARTESIAN_POINT('Ctrl Pts',(-12.7230374570564,-54.2352240753197,
17.8180808188594));
#66019=CARTESIAN_POINT('Ctrl Pts',(-14.1607486178545,-54.9742845180233,
17.7395753084827));
#66020=CARTESIAN_POINT('Ctrl Pts',(-15.5710663391631,-54.1822851282416,
17.6610697981059));
#66021=CARTESIAN_POINT('Ctrl Pts',(-15.6879493748746,-52.5692748502928,
17.5825642877291));
#66022=CARTESIAN_POINT('Ctrl Pts',(-14.407185930718,-51.5819561299908,17.5040587773523));
#66023=CARTESIAN_POINT('Ctrl Pts',(-12.8770920017801,-52.1057221405655,
17.4255532669755));
#66024=CARTESIAN_POINT('Ctrl Pts',(-12.4700424055274,-53.6708756791509,
17.3470477565988));
#66025=CARTESIAN_POINT('Ctrl Pts',(-13.5510144619001,-54.8737356665186,
17.268542246222));
#66026=CARTESIAN_POINT('Ctrl Pts',(-15.1506036186114,-54.6355556948135,
17.1900367358452));
#66027=CARTESIAN_POINT('Ctrl Pts',(-15.8342420126427,-53.1699377437178,
17.1115312254684));
#66028=CARTESIAN_POINT('Ctrl Pts',(-14.9888355379813,-51.791284560039,17.0330257150916));
#66029=CARTESIAN_POINT('Ctrl Pts',(-13.3725603306097,-51.7360042395789,
16.9545202047149));
#66030=CARTESIAN_POINT('Ctrl Pts',(-12.4349326457219,-53.0536739116012,
16.8760146943381));
#66031=CARTESIAN_POINT('Ctrl Pts',(-13.0168381795997,-54.5625758784866,
16.7975091839613));
#66032=CARTESIAN_POINT('Ctrl Pts',(-14.5964107617212,-54.9094910882809,
16.7190036735845));
#66033=CARTESIAN_POINT('Ctrl Pts',(-15.7570518775445,-53.7832976818467,
16.6404981632077));
#66034=CARTESIAN_POINT('Ctrl Pts',(-15.457871115886,-52.1939927053388,16.561992652831));
#66035=CARTESIAN_POINT('Ctrl Pts',(-13.9671808299377,-51.5669026325919,
16.4834871424542));
#66036=CARTESIAN_POINT('Ctrl Pts',(-12.6218675402158,-52.4644167553317,
16.4049816320774));
#66037=CARTESIAN_POINT('Ctrl Pts',(-12.6284401716074,-54.0816230680013,
16.3264761217006));
#66038=CARTESIAN_POINT('Ctrl Pts',(-13.9810042401211,-54.9681725040556,
16.2479706113238));
#66039=CARTESIAN_POINT('Ctrl Pts',(-15.4665481297228,-54.3289864519802,
16.1694651009471));
#66040=CARTESIAN_POINT('Ctrl Pts',(-15.7528007654441,-52.7373021594152,
16.0909595905703));
#66041=CARTESIAN_POINT('Ctrl Pts',(-14.5830439772701,-51.6205799399095,
16.0124540801935));
#66042=CARTESIAN_POINT('Ctrl Pts',(-13.0063434627971,-51.9803228284872,
15.9339485698167));
#66043=CARTESIAN_POINT('Ctrl Pts',(-12.4367217268737,-53.4939048503744,
15.8554430594399));
#66044=CARTESIAN_POINT('Ctrl Pts',(-13.3850290847768,-54.8039096647176,
15.7769375490632));
#66045=CARTESIAN_POINT('Ctrl Pts',(-15.0008009523569,-54.7354938110165,
15.6984320386864));
#66046=CARTESIAN_POINT('Ctrl Pts',(-15.8349747076461,-53.3500142521672,
15.6199265283096));
#66047=CARTESIAN_POINT('Ctrl Pts',(-15.1394434922597,-51.8900019968609,
15.5414210179328));
#66048=CARTESIAN_POINT('Ctrl Pts',(-13.5379762420925,-51.6648307405647,
15.462915507556));
#66049=CARTESIAN_POINT('Ctrl Pts',(-12.4668068464345,-52.8764394289472,
15.3844099971793));
#66050=CARTESIAN_POINT('Ctrl Pts',(-12.8865855118699,-54.4382285659772,
15.3059044868025));
#66051=CARTESIAN_POINT('Ctrl Pts',(-14.4208446971614,-54.9495485643972,
15.2273989764257));
#66052=CARTESIAN_POINT('Ctrl Pts',(-15.6936243998074,-53.9518354124797,
15.1488934660489));
#66053=CARTESIAN_POINT('Ctrl Pts',(-15.5634653023156,-52.3398621480091,
15.0703879556722));
#66054=CARTESIAN_POINT('Ctrl Pts',(-14.1470976247563,-51.5592843863476,
14.9918824452954));
#66055=CARTESIAN_POINT('Ctrl Pts',(-12.7147526703863,-52.3101434886333,
14.9133769349186));
#66056=CARTESIAN_POINT('Ctrl Pts',(-12.5509932669133,-53.919049814695,14.8348714245418));
#66057=CARTESIAN_POINT('Ctrl Pts',(-13.8026790667016,-54.9431006391055,
14.756365914165));
#66058=CARTESIAN_POINT('Ctrl Pts',(-15.3472759009633,-54.4638973536635,
14.6778604037883));
#66059=CARTESIAN_POINT('Ctrl Pts',(-15.7995376478154,-52.9112119224821,
14.5993548934115));
#66060=CARTESIAN_POINT('Ctrl Pts',(-14.7538954097245,-51.6775072239921,
14.5208493830347));
#66061=CARTESIAN_POINT('Ctrl Pts',(-13.1480450848167,-51.8692440206668,
14.4423438726579));
#66062=CARTESIAN_POINT('Ctrl Pts',(-12.4222743542852,-53.3143772678279,
14.3638383622811));
#66063=CARTESIAN_POINT('Ctrl Pts',(-13.2272235892288,-54.7170605998631,
14.2853328519044));
#66064=CARTESIAN_POINT('Ctrl Pts',(-14.8414958116982,-54.8189639865359,
14.2068273415276));
#66065=CARTESIAN_POINT('Ctrl Pts',(-15.8163626318126,-53.5294453155223,
14.1283218311508));
#66066=CARTESIAN_POINT('Ctrl Pts',(-15.2795869011495,-52.0034666921275,
14.049816320774));
#66067=CARTESIAN_POINT('Ctrl Pts',(-13.708356793232,-51.6126272165693,13.9713108103972));
#66068=CARTESIAN_POINT('Ctrl Pts',(-12.9176155863349,-52.3383285372882,
13.9189738034794));
#66069=CARTESIAN_POINT('Ctrl Pts',(-12.7602980089432,-52.7885097885712,
13.8928053000205));
#66070=CARTESIAN_POINT('Ctrl Pts',(-15.0896057741301,-52.3076708240835,
18.1071946999795));
#66071=CARTESIAN_POINT('Ctrl Pts',(-14.7741676148584,-51.9918752589882,
18.0810261965206));
#66072=CARTESIAN_POINT('Ctrl Pts',(-13.8126730138722,-51.700874003756,18.0286891896028));
#66073=CARTESIAN_POINT('Ctrl Pts',(-12.646239044783,-52.6683748462133,17.950183679226));
#66074=CARTESIAN_POINT('Ctrl Pts',(-12.8130591452175,-54.1732366374368,
17.8716781688492));
#66075=CARTESIAN_POINT('Ctrl Pts',(-14.1587343197422,-54.8649856600065,
17.7931726584724));
#66076=CARTESIAN_POINT('Ctrl Pts',(-15.4787696630749,-54.123686610428,17.7146671480956));
#66077=CARTESIAN_POINT('Ctrl Pts',(-15.5881703575737,-52.6139342022434,
17.6361616377189));
#66078=CARTESIAN_POINT('Ctrl Pts',(-14.3893957926718,-51.6898193122147,
17.5576561273421));
#66079=CARTESIAN_POINT('Ctrl Pts',(-12.9572517911467,-52.1800561114469,
17.4791506169653));
#66080=CARTESIAN_POINT('Ctrl Pts',(-12.576259731397,-53.6450153596069,17.4006451065885));
#66081=CARTESIAN_POINT('Ctrl Pts',(-13.58803268015,-54.7708735066155,17.3221395962118));
#66082=CARTESIAN_POINT('Ctrl Pts',(-15.0852231286336,-54.547940775945,17.243634085835));
#66083=CARTESIAN_POINT('Ctrl Pts',(-15.725097979914,-53.1761452818954,17.1651285754582));
#66084=CARTESIAN_POINT('Ctrl Pts',(-14.9338107336617,-51.8857474508553,
17.0866230650814));
#66085=CARTESIAN_POINT('Ctrl Pts',(-13.4210024025693,-51.8340059349575,
17.0081175547046));
#66086=CARTESIAN_POINT('Ctrl Pts',(-12.5433975449982,-53.067324152283,16.9296120443279));
#66087=CARTESIAN_POINT('Ctrl Pts',(-13.0880520292989,-54.4796328085655,
16.8511065339511));
#66088=CARTESIAN_POINT('Ctrl Pts',(-14.5665072768334,-54.8043400225141,
16.7726010235743));
#66089=CARTESIAN_POINT('Ctrl Pts',(-15.6528492199738,-53.7502405969307,
16.6940955131975));
#66090=CARTESIAN_POINT('Ctrl Pts',(-15.3728207033727,-52.2626759803716,
16.6155900028207));
#66091=CARTESIAN_POINT('Ctrl Pts',(-13.9775578957916,-51.6757294739412,
16.5370844924439));
#66092=CARTESIAN_POINT('Ctrl Pts',(-12.7183656843796,-52.5157886643324,
16.4585789820672));
#66093=CARTESIAN_POINT('Ctrl Pts',(-12.7245175646294,-54.0294684954301,
16.3800734716904));
#66094=CARTESIAN_POINT('Ctrl Pts',(-13.990496391658,-54.8592649104658,16.3015679613136));
#66095=CARTESIAN_POINT('Ctrl Pts',(-15.3809422526988,-54.2609967564488,
16.2230624509368));
#66096=CARTESIAN_POINT('Ctrl Pts',(-15.6488702454944,-52.77120513725,16.1445569405601));
#66097=CARTESIAN_POINT('Ctrl Pts',(-14.5539961755152,-51.7259705945934,
16.0660514301833));
#66098=CARTESIAN_POINT('Ctrl Pts',(-13.0782291384082,-52.0626843153815,
15.9875459198065));
#66099=CARTESIAN_POINT('Ctrl Pts',(-12.5450720969922,-53.4793734299947,
15.9090404094297));
#66100=CARTESIAN_POINT('Ctrl Pts',(-13.4326729615783,-54.7055174603373,
15.8305348990529));
#66101=CARTESIAN_POINT('Ctrl Pts',(-14.9450101744931,-54.6414812906393,
15.7520293886762));
#66102=CARTESIAN_POINT('Ctrl Pts',(-15.725783770985,-53.3446940791386,15.6735238782994));
#66103=CARTESIAN_POINT('Ctrl Pts',(-15.0747774248056,-51.9781454287288,
15.5950183679226));
#66104=CARTESIAN_POINT('Ctrl Pts',(-13.5758291102025,-51.7673886523496,
15.5165128575458));
#66105=CARTESIAN_POINT('Ctrl Pts',(-12.5732312986591,-52.9014354467625,
15.438007347169));
#66106=CARTESIAN_POINT('Ctrl Pts',(-12.9661375682035,-54.3632456676534,
15.3595018367923));
#66107=CARTESIAN_POINT('Ctrl Pts',(-14.402180184571,-54.841833194045,15.2809963264155));
#66108=CARTESIAN_POINT('Ctrl Pts',(-15.593482092208,-53.9079892784932,15.2024908160387));
#66109=CARTESIAN_POINT('Ctrl Pts',(-15.4716552113927,-52.3992074987152,
15.1239853056619));
#66110=CARTESIAN_POINT('Ctrl Pts',(-14.1459572035726,-51.6685989145327,
15.0454797952851));
#66111=CARTESIAN_POINT('Ctrl Pts',(-12.8053047143887,-52.3713912980536,
14.9669742849084));
#66112=CARTESIAN_POINT('Ctrl Pts',(-12.6520284723609,-53.8773024714182,
14.8884687745316));
#66113=CARTESIAN_POINT('Ctrl Pts',(-13.8235868166289,-54.8357980367556,
14.8099632641548));
#66114=CARTESIAN_POINT('Ctrl Pts',(-15.2693053108511,-54.3872712517148,
14.731457753778));
#66115=CARTESIAN_POINT('Ctrl Pts',(-15.6926152368783,-52.9339819572036,
14.6529522434012));
#66116=CARTESIAN_POINT('Ctrl Pts',(-14.7139104458185,-51.7792536426992,
14.5744467330245));
#66117=CARTESIAN_POINT('Ctrl Pts',(-13.2108596417673,-51.9587162874664,
14.4959412226477));
#66118=CARTESIAN_POINT('Ctrl Pts',(-12.5315495820674,-53.3113384188168,
14.4174357122709));
#66119=CARTESIAN_POINT('Ctrl Pts',(-13.2849694843063,-54.624228093118,14.3389302018941));
#66120=CARTESIAN_POINT('Ctrl Pts',(-14.7959030528376,-54.7196080702543,
14.2604246915173));
#66121=CARTESIAN_POINT('Ctrl Pts',(-15.7083631589187,-53.5126387498619,
14.1819191811406));
#66122=CARTESIAN_POINT('Ctrl Pts',(-15.2059494650307,-52.0843466100013,
14.1034136707638));
#66123=CARTESIAN_POINT('Ctrl Pts',(-13.735302642955,-51.7185269698511,14.024908160387));
#66124=CARTESIAN_POINT('Ctrl Pts',(-12.9951812328907,-52.3977720630514,
13.9725711534692));
#66125=CARTESIAN_POINT('Ctrl Pts',(-12.8479344393867,-52.8191346777449,
13.9464026500102));
#66126=CARTESIAN_POINT('Ctrl Pts',(-15.0239255378924,-52.3732767258419,
18.1607920499693));
#66127=CARTESIAN_POINT('Ctrl Pts',(-14.7300614275787,-52.0790796540862,
18.1346235465104));
#66128=CARTESIAN_POINT('Ctrl Pts',(-13.834327201439,-51.8079811124057,18.0822865395925));
#66129=CARTESIAN_POINT('Ctrl Pts',(-12.7476702118172,-52.7093107896801,
18.0037810292157));
#66130=CARTESIAN_POINT('Ctrl Pts',(-12.9030808333786,-54.111249199554,17.925275518839));
#66131=CARTESIAN_POINT('Ctrl Pts',(-14.15672002163,-54.7556868019897,17.8467700084622));
#66132=CARTESIAN_POINT('Ctrl Pts',(-15.3864729869866,-54.0650880926144,
17.7682644980854));
#66133=CARTESIAN_POINT('Ctrl Pts',(-15.4883913402728,-52.6585935541939,
17.6897589877086));
#66134=CARTESIAN_POINT('Ctrl Pts',(-14.3716056546256,-51.7976824944385,
17.6112534773319));
#66135=CARTESIAN_POINT('Ctrl Pts',(-13.0374115805133,-52.2543900823285,
17.5327479669551));
#66136=CARTESIAN_POINT('Ctrl Pts',(-12.6824770572666,-53.6191550400628,
17.4542424565783));
#66137=CARTESIAN_POINT('Ctrl Pts',(-13.6250508983998,-54.6680113467125,
17.3757369462015));
#66138=CARTESIAN_POINT('Ctrl Pts',(-15.0198426386559,-54.4603258570761,
17.2972314358247));
#66139=CARTESIAN_POINT('Ctrl Pts',(-15.6159539471854,-53.1823528200732,
17.218725925448));
#66140=CARTESIAN_POINT('Ctrl Pts',(-14.878785929342,-51.9802103416716,17.1402204150712));
#66141=CARTESIAN_POINT('Ctrl Pts',(-13.4694444745289,-51.9320076303361,
17.0617149046944));
#66142=CARTESIAN_POINT('Ctrl Pts',(-12.6518624442745,-53.0809743929648,
16.9832093943176));
#66143=CARTESIAN_POINT('Ctrl Pts',(-13.1592658789981,-54.3966897386446,
16.9047038839409));
#66144=CARTESIAN_POINT('Ctrl Pts',(-14.5366037919456,-54.6991889567472,
16.8261983735641));
#66145=CARTESIAN_POINT('Ctrl Pts',(-15.5486465624032,-53.7171835120147,
16.7476928631873));
#66146=CARTESIAN_POINT('Ctrl Pts',(-15.2877702908594,-52.3313592554045,
16.6691873528105));
#66147=CARTESIAN_POINT('Ctrl Pts',(-13.9879349616455,-51.7845563152906,
16.5906818424337));
#66148=CARTESIAN_POINT('Ctrl Pts',(-12.8148638285435,-52.567160573333,16.5121763320569));
#66149=CARTESIAN_POINT('Ctrl Pts',(-12.8205949576515,-53.9773139228589,
16.4336708216802));
#66150=CARTESIAN_POINT('Ctrl Pts',(-13.9999885431949,-54.7503573168762,
16.3551653113034));
#66151=CARTESIAN_POINT('Ctrl Pts',(-15.2953363756749,-54.1930070609174,
16.2766598009266));
#66152=CARTESIAN_POINT('Ctrl Pts',(-15.5449397255447,-52.8051081150848,
16.1981542905498));
#66153=CARTESIAN_POINT('Ctrl Pts',(-14.5249483737603,-51.8313612492774,
16.119648780173));
#66154=CARTESIAN_POINT('Ctrl Pts',(-13.1501148140193,-52.1450458022758,
16.0411432697963));
#66155=CARTESIAN_POINT('Ctrl Pts',(-12.6534224671108,-53.464842009615,15.9626377594195));
#66156=CARTESIAN_POINT('Ctrl Pts',(-13.4803168383798,-54.607125255957,15.8841322490427));
#66157=CARTESIAN_POINT('Ctrl Pts',(-14.8892193966293,-54.5474687702622,
15.8056267386659));
#66158=CARTESIAN_POINT('Ctrl Pts',(-15.6165928343238,-53.3393739061099,
15.7271212282891));
#66159=CARTESIAN_POINT('Ctrl Pts',(-15.0101113573514,-52.0662888605968,
15.6486157179124));
#66160=CARTESIAN_POINT('Ctrl Pts',(-13.6136819783124,-51.8699465641345,
15.5701102075356));
#66161=CARTESIAN_POINT('Ctrl Pts',(-12.6796557508836,-52.9264314645779,
15.4916046971588));
#66162=CARTESIAN_POINT('Ctrl Pts',(-13.0456896245371,-54.2882627693297,
15.413099186782));
#66163=CARTESIAN_POINT('Ctrl Pts',(-14.3835156719806,-54.7341178236928,
15.3345936764052));
#66164=CARTESIAN_POINT('Ctrl Pts',(-15.4933397846086,-53.8641431445067,
15.2560881660285));
#66165=CARTESIAN_POINT('Ctrl Pts',(-15.3798451204699,-52.4585528494213,
15.1775826556517));
#66166=CARTESIAN_POINT('Ctrl Pts',(-14.1448167823889,-51.7779134427179,
15.0990771452749));
#66167=CARTESIAN_POINT('Ctrl Pts',(-12.8958567583911,-52.4326391074739,
15.0205716348981));
#66168=CARTESIAN_POINT('Ctrl Pts',(-12.7530636778084,-53.8355551281416,
14.9420661245214));
#66169=CARTESIAN_POINT('Ctrl Pts',(-13.8444945665562,-54.7284954344056,
14.8635606141446));
#66170=CARTESIAN_POINT('Ctrl Pts',(-15.1913347207389,-54.3106451497661,
14.7850551037678));
#66171=CARTESIAN_POINT('Ctrl Pts',(-15.5856928259413,-52.9567519919251,
14.706549593391));
#66172=CARTESIAN_POINT('Ctrl Pts',(-14.6739254819125,-51.8810000614065,
14.6280440830142));
#66173=CARTESIAN_POINT('Ctrl Pts',(-13.2736741987179,-52.048188554266,14.5495385726375));
#66174=CARTESIAN_POINT('Ctrl Pts',(-12.6408248098497,-53.3082995698058,
14.4710330622607));
#66175=CARTESIAN_POINT('Ctrl Pts',(-13.3427153793839,-54.5313955863729,
14.3925275518839));
#66176=CARTESIAN_POINT('Ctrl Pts',(-14.7503102939771,-54.6202521539727,
14.3140220415071));
#66177=CARTESIAN_POINT('Ctrl Pts',(-15.6003636860249,-53.4958321842015,
14.2355165311303));
#66178=CARTESIAN_POINT('Ctrl Pts',(-15.1323120289118,-52.1652265278751,
14.1570110207536));
#66179=CARTESIAN_POINT('Ctrl Pts',(-13.762248492678,-51.824426723133,14.0785055103768));
#66180=CARTESIAN_POINT('Ctrl Pts',(-13.0727468794464,-52.4572155888145,
14.0261685034589));
#66181=CARTESIAN_POINT('Ctrl Pts',(-12.9355708698302,-52.8497595669186,
14.));
#66182=CARTESIAN_POINT('Ctrl Pts',(-13.4965541629804,-52.1730078059394,
17.5565803263806));
#66183=CARTESIAN_POINT('Ctrl Pts',(-13.3865887223467,-52.2353622375859,
17.5486362065721));
#66184=CARTESIAN_POINT('Ctrl Pts',(-13.2860845507673,-52.3135738660447,
17.5406920867636));
#66185=CARTESIAN_POINT('Ctrl Pts',(-13.2006215056576,-52.4057329773026,
17.5327479669551));
#66186=CARTESIAN_POINT('Ctrl Pts',(-12.9191000727644,-52.7093117349066,
17.5065794634962));
#66187=CARTESIAN_POINT('Ctrl Pts',(-12.8007885650155,-53.1642333874847,
17.4804109600372));
#66188=CARTESIAN_POINT('Ctrl Pts',(-12.8987284513299,-53.5665035982154,
17.4542424565783));
#66189=CARTESIAN_POINT('Ctrl Pts',(-12.9966683376443,-53.968773808946,17.4280739531194));
#66190=CARTESIAN_POINT('Ctrl Pts',(-13.3108596180221,-54.3183925778293,
17.4019054496604));
#66191=CARTESIAN_POINT('Ctrl Pts',(-13.7004205482536,-54.4585877139982,
17.3757369462015));
#66192=CARTESIAN_POINT('Ctrl Pts',(-14.0899814784852,-54.5987828501671,
17.3495684427426));
#66193=CARTESIAN_POINT('Ctrl Pts',(-14.5549120585705,-54.5295543536216,
17.3233999392837));
#66194=CARTESIAN_POINT('Ctrl Pts',(-14.8867292333681,-54.2819445991817,
17.2972314358247));
#66195=CARTESIAN_POINT('Ctrl Pts',(-15.2185464081657,-54.0343348447418,
17.2710629323658));
#66196=CARTESIAN_POINT('Ctrl Pts',(-15.4172501776756,-53.6083438324075,
17.2448944289069));
#66197=CARTESIAN_POINT('Ctrl Pts',(-15.3937407261232,-53.1949912465067,
17.218725925448));
#66198=CARTESIAN_POINT('Ctrl Pts',(-15.3702312745709,-52.781638660606,17.192557421989));
#66199=CARTESIAN_POINT('Ctrl Pts',(-15.1245086019565,-52.3809245011388,
17.1663889185301));
#66200=CARTESIAN_POINT('Ctrl Pts',(-14.7667570231804,-52.1725336361826,
17.1402204150712));
#66201=CARTESIAN_POINT('Ctrl Pts',(-14.4090054444043,-51.9641427712264,
17.1140519116123));
#66202=CARTESIAN_POINT('Ctrl Pts',(-13.9392249594666,-51.9480752007813,
17.0878834081533));
#66203=CARTESIAN_POINT('Ctrl Pts',(-13.5680710452887,-52.1315358759968,
17.0617149046944));
#66204=CARTESIAN_POINT('Ctrl Pts',(-13.5437960761855,-52.1435349471433,
17.0600033785898));
#66205=CARTESIAN_POINT('Ctrl Pts',(-13.5199430009518,-52.1563875382182,
17.0582918524852));
#66206=CARTESIAN_POINT('Ctrl Pts',(-13.4965460097018,-52.1700456009991,
17.0565803263806));
#66207=CARTESIAN_POINT('Origin',(-14.1292828945604,-53.2669068454841,15.5));
#66208=CARTESIAN_POINT('Origin',(-53.1951359564886,-14.3971354987959,14.));
#66209=CARTESIAN_POINT('Ctrl Pts',(-52.2370198037663,-15.2223467977324,
14.));
#66210=CARTESIAN_POINT('Ctrl Pts',(-52.1998280045551,-15.187614600057,14.));
#66211=CARTESIAN_POINT('Ctrl Pts',(-52.1650182492936,-15.1505714365352,
14.));
#66212=CARTESIAN_POINT('Ctrl Pts',(-52.1326048428076,-15.1115303634521,
14.));
#66213=CARTESIAN_POINT('Ctrl Pts',(-52.1107612978768,-15.0852204032691,
14.));
#66214=CARTESIAN_POINT('Ctrl Pts',(-52.0900064961692,-15.0580020338226,
14.));
#66215=CARTESIAN_POINT('Ctrl Pts',(-52.0703516540902,-15.0299603099463,
14.));
#66216=CARTESIAN_POINT('Ctrl Pts',(-52.0612801328574,-15.017017896442,14.));
#66217=CARTESIAN_POINT('Ctrl Pts',(-52.0524430090281,-15.0038999832866,
14.));
#66218=CARTESIAN_POINT('Ctrl Pts',(-52.0438418390641,-14.9906144201694,
14.));
#66219=CARTESIAN_POINT('Ctrl Pts',(-52.036611845359,-14.9794468071462,14.));
#66220=CARTESIAN_POINT('Ctrl Pts',(-52.0295526827715,-14.9681669384272,
14.));
#66221=CARTESIAN_POINT('Ctrl Pts',(-52.022668475442,-14.956786074209,14.));
#66222=CARTESIAN_POINT('Ctrl Pts',(-51.9948472065506,-14.9107923862691,
14.));
#66223=CARTESIAN_POINT('Ctrl Pts',(-51.9698609199132,-14.8631221292342,
14.));
#66224=CARTESIAN_POINT('Ctrl Pts',(-51.947748300236,-14.8140997169745,14.));
#66225=CARTESIAN_POINT('Ctrl Pts',(-51.9392849994114,-14.7953370634237,
14.));
#66226=CARTESIAN_POINT('Ctrl Pts',(-51.9312430201854,-14.776375916002,14.));
#66227=CARTESIAN_POINT('Ctrl Pts',(-51.9236259797948,-14.757233069302,14.));
#66228=CARTESIAN_POINT('Ctrl Pts',(-51.918152652305,-14.7434777176558,14.));
#66229=CARTESIAN_POINT('Ctrl Pts',(-51.9128987520874,-14.7296285333462,
14.));
#66230=CARTESIAN_POINT('Ctrl Pts',(-51.9078659027834,-14.7156915540625,
14.));
#66231=CARTESIAN_POINT('Ctrl Pts',(-51.9039695335319,-14.7049017182738,
14.));
#66232=CARTESIAN_POINT('Ctrl Pts',(-51.9002056527562,-14.6940588600005,
14.));
#66233=CARTESIAN_POINT('Ctrl Pts',(-51.8965797112069,-14.6831806448979,
14.));
#66234=CARTESIAN_POINT('Ctrl Pts',(-51.8786612859968,-14.629423439747,14.));
#66235=CARTESIAN_POINT('Ctrl Pts',(-51.8640761421938,-14.5747200728836,
14.));
#66236=CARTESIAN_POINT('Ctrl Pts',(-51.8528626358983,-14.5194298174396,
14.));
#66237=CARTESIAN_POINT('Ctrl Pts',(-51.8418116070222,-14.4649406867982,
14.));
#66238=CARTESIAN_POINT('Ctrl Pts',(-51.8340348275742,-14.409880375256,14.));
#66239=CARTESIAN_POINT('Ctrl Pts',(-51.8296128481337,-14.354562785674,14.));
#66240=CARTESIAN_POINT('Ctrl Pts',(-51.8273037118427,-14.3256762077624,
14.));
#66241=CARTESIAN_POINT('Ctrl Pts',(-51.8259101526051,-14.2967190813249,
14.));
#66242=CARTESIAN_POINT('Ctrl Pts',(-51.8254490493326,-14.2677344056925,
14.));
#66243=CARTESIAN_POINT('Ctrl Pts',(-51.8252016892536,-14.2521854992281,
14.));
#66244=CARTESIAN_POINT('Ctrl Pts',(-51.8252227392431,-14.2366286515745,
14.));
#66245=CARTESIAN_POINT('Ctrl Pts',(-51.8255152855579,-14.2210704503188,
14.));
#66246=CARTESIAN_POINT('Ctrl Pts',(-51.8257232519346,-14.2100103802406,
14.));
#66247=CARTESIAN_POINT('Ctrl Pts',(-51.8260684275002,-14.1989496254671,
14.));
#66248=CARTESIAN_POINT('Ctrl Pts',(-51.8265520290651,-14.1878905523495,
14.));
#66249=CARTESIAN_POINT('Ctrl Pts',(-51.8269778211602,-14.1781534748575,
14.));
#66250=CARTESIAN_POINT('Ctrl Pts',(-51.8275105014082,-14.1684274978297,
14.));
#66251=CARTESIAN_POINT('Ctrl Pts',(-51.8281502461755,-14.1587149162952,
14.));
#66252=CARTESIAN_POINT('Ctrl Pts',(-51.8313147365973,-14.1106717390646,
14.));
#66253=CARTESIAN_POINT('Ctrl Pts',(-51.8370971206981,-14.0629523055729,
14.));
#66254=CARTESIAN_POINT('Ctrl Pts',(-51.8455361922423,-14.0157553469174,
14.));
#66255=CARTESIAN_POINT('Ctrl Pts',(-51.8551414270627,-13.9620364196248,
14.));
#66256=CARTESIAN_POINT('Ctrl Pts',(-51.8681865747697,-13.9089935983908,
14.));
#66257=CARTESIAN_POINT('Ctrl Pts',(-51.8844213082613,-13.8568249617529,
14.));
#66258=CARTESIAN_POINT('Ctrl Pts',(-51.9002905362141,-13.8058308393532,
14.));
#66259=CARTESIAN_POINT('Ctrl Pts',(-51.9192079284338,-13.7556712969149,
14.));
#66260=CARTESIAN_POINT('Ctrl Pts',(-51.9409851275907,-13.7065350685516,
14.));
#66261=CARTESIAN_POINT('Ctrl Pts',(-51.9463194725313,-13.6944991042717,
14.));
#66262=CARTESIAN_POINT('Ctrl Pts',(-51.9518256037611,-13.6825245847688,
14.));
#66263=CARTESIAN_POINT('Ctrl Pts',(-51.9575011215412,-13.6706143910813,
14.));
#66264=CARTESIAN_POINT('Ctrl Pts',(-51.9617861950524,-13.6616220739992,
14.));
#66265=CARTESIAN_POINT('Ctrl Pts',(-51.9661670467492,-13.6526682499682,
14.));
#66266=CARTESIAN_POINT('Ctrl Pts',(-51.9706371983683,-13.6437643302994,
14.));
#66267=CARTESIAN_POINT('Ctrl Pts',(-51.9964876791123,-13.5922737716888,
14.));
#66268=CARTESIAN_POINT('Ctrl Pts',(-52.0253653817646,-13.5423559816578,
14.));
#66269=CARTESIAN_POINT('Ctrl Pts',(-52.056990938761,-13.4942262955812,14.));
#66270=CARTESIAN_POINT('Ctrl Pts',(-52.0892948739252,-13.4450642125649,
14.));
#66271=CARTESIAN_POINT('Ctrl Pts',(-52.1244662109051,-13.3977668163443,
14.));
#66272=CARTESIAN_POINT('Ctrl Pts',(-52.1622608704981,-13.3525735612878,
14.));
#66273=CARTESIAN_POINT('Ctrl Pts',(-52.2003880180872,-13.3069827311511,
14.));
#66274=CARTESIAN_POINT('Ctrl Pts',(-52.2411854112278,-13.2635321825438,
14.));
#66275=CARTESIAN_POINT('Ctrl Pts',(-52.2844490105985,-13.2224929144395,
14.));
#66276=CARTESIAN_POINT('Ctrl Pts',(-52.2942488213998,-13.2131969458032,
14.));
#66277=CARTESIAN_POINT('Ctrl Pts',(-52.3041782446756,-13.204022403894,14.));
#66278=CARTESIAN_POINT('Ctrl Pts',(-52.3142147728346,-13.1949905193645,
14.));
#66279=CARTESIAN_POINT('Ctrl Pts',(-52.3594366695135,-13.154295276693,14.));
#66280=CARTESIAN_POINT('Ctrl Pts',(-52.4069027254174,-13.1164219433845,
14.));
#66281=CARTESIAN_POINT('Ctrl Pts',(-52.4563466159028,-13.081614036475,14.));
#66282=CARTESIAN_POINT('Ctrl Pts',(-52.5053559226553,-13.0471120713103,
14.));
#66283=CARTESIAN_POINT('Ctrl Pts',(-52.5563091708902,-13.0156209538648,
14.));
#66284=CARTESIAN_POINT('Ctrl Pts',(-52.6089887803891,-12.9874055955952,
14.));
#66285=CARTESIAN_POINT('Ctrl Pts',(-52.6475874040962,-12.9667320559282,
14.));
#66286=CARTESIAN_POINT('Ctrl Pts',(-52.6871137410699,-12.9478176360512,
14.));
#66287=CARTESIAN_POINT('Ctrl Pts',(-52.7274932936822,-12.9307805393251,
14.));
#66288=CARTESIAN_POINT('Ctrl Pts',(-52.7499343911042,-12.9213121048654,
14.));
#66289=CARTESIAN_POINT('Ctrl Pts',(-52.7726391696466,-12.9124237518852,
14.));
#66290=CARTESIAN_POINT('Ctrl Pts',(-52.7955875161457,-12.9041113834231,
14.));
#66291=CARTESIAN_POINT('Ctrl Pts',(-53.5936497983459,-12.9064860705774,
14.));
#66292=CARTESIAN_POINT('Ctrl Pts',(-53.6509984651359,-12.9274410373818,
14.));
#66293=CARTESIAN_POINT('Ctrl Pts',(-53.7068627003681,-12.9520247913344,
14.));
#66294=CARTESIAN_POINT('Ctrl Pts',(-53.7610278853563,-12.9799613169679,
14.));
#66295=CARTESIAN_POINT('Ctrl Pts',(-53.8112531574186,-13.0058657720292,
14.));
#66296=CARTESIAN_POINT('Ctrl Pts',(-53.8600177560829,-13.0346541103165,
14.));
#66297=CARTESIAN_POINT('Ctrl Pts',(-53.9071231753197,-13.0661362083695,
14.));
#66298=CARTESIAN_POINT('Ctrl Pts',(-53.9184932356252,-13.073735192928,14.));
#66299=CARTESIAN_POINT('Ctrl Pts',(-53.929766785557,-13.0814915892485,14.));
#66300=CARTESIAN_POINT('Ctrl Pts',(-53.9409284677904,-13.089393751099,14.));
#66301=CARTESIAN_POINT('Ctrl Pts',(-53.9900508425651,-13.1241710317841,
14.));
#66302=CARTESIAN_POINT('Ctrl Pts',(-54.0370703142149,-13.1618085881906,
14.));
#66303=CARTESIAN_POINT('Ctrl Pts',(-54.0817574272605,-13.2020613661078,
14.));
#66304=CARTESIAN_POINT('Ctrl Pts',(-54.10933993136,-13.2269068380179,14.));
#66305=CARTESIAN_POINT('Ctrl Pts',(-54.1360331111675,-13.2527493803639,
14.));
#66306=CARTESIAN_POINT('Ctrl Pts',(-54.1617745164173,-13.2795365303592,
14.));
#66307=CARTESIAN_POINT('Ctrl Pts',(-54.1705826003128,-13.2887024427169,
14.));
#66308=CARTESIAN_POINT('Ctrl Pts',(-54.1792791849711,-13.2979789799756,
14.));
#66309=CARTESIAN_POINT('Ctrl Pts',(-54.1878615699546,-13.3073641131248,
14.));
#66310=CARTESIAN_POINT('Ctrl Pts',(-54.195890456635,-13.3161439768432,14.));
#66311=CARTESIAN_POINT('Ctrl Pts',(-54.2038142461512,-13.3250133167635,
14.));
#66312=CARTESIAN_POINT('Ctrl Pts',(-54.2116272144904,-13.3339655513165,
14.));
#66313=CARTESIAN_POINT('Ctrl Pts',(-54.250298832142,-13.3782761611554,14.));
#66314=CARTESIAN_POINT('Ctrl Pts',(-54.286291162471,-13.4246505091249,14.));
#66315=CARTESIAN_POINT('Ctrl Pts',(-54.3193890208801,-13.4728592463024,
14.));
#66316=CARTESIAN_POINT('Ctrl Pts',(-54.3516418894012,-13.5198372121435,
14.));
#66317=CARTESIAN_POINT('Ctrl Pts',(-54.3811465604949,-13.5685580127126,
14.));
#66318=CARTESIAN_POINT('Ctrl Pts',(-54.4076582516214,-13.6188275090082,
14.));
#66319=CARTESIAN_POINT('Ctrl Pts',(-54.422032099109,-13.6460821292277,14.));
#66320=CARTESIAN_POINT('Ctrl Pts',(-54.4355253353237,-13.6737922214405,
14.));
#66321=CARTESIAN_POINT('Ctrl Pts',(-54.4480925383944,-13.7019277688883,
14.));
#66322=CARTESIAN_POINT('Ctrl Pts',(-54.4585481854562,-13.7253359490815,
14.));
#66323=CARTESIAN_POINT('Ctrl Pts',(-54.4683627680535,-13.7490386437541,
14.));
#66324=CARTESIAN_POINT('Ctrl Pts',(-54.4775075098049,-13.7730185624462,
14.));
#66325=CARTESIAN_POINT('Ctrl Pts',(-54.4814161888852,-13.7832681472993,
14.));
#66326=CARTESIAN_POINT('Ctrl Pts',(-54.4852027887794,-13.7935696368397,
14.));
#66327=CARTESIAN_POINT('Ctrl Pts',(-54.4888592933946,-13.8039047382203,
14.));
#66328=CARTESIAN_POINT('Ctrl Pts',(-54.5057868221325,-13.8517503569301,
14.));
#66329=CARTESIAN_POINT('Ctrl Pts',(-54.5199611541528,-13.9003971684769,
14.));
#66330=CARTESIAN_POINT('Ctrl Pts',(-54.5312161752957,-13.9497022076935,
14.));
#66331=CARTESIAN_POINT('Ctrl Pts',(-54.5437933673149,-14.0047993006149,
14.));
#66332=CARTESIAN_POINT('Ctrl Pts',(-54.5527257730479,-14.060719293395,14.));
#66333=CARTESIAN_POINT('Ctrl Pts',(-54.5581033230398,-14.1171258864099,
14.));
#66334=CARTESIAN_POINT('Ctrl Pts',(-54.5626667133147,-14.1649925354209,
14.));
#66335=CARTESIAN_POINT('Ctrl Pts',(-54.5646690852638,-14.2132100479209,
14.));
#66336=CARTESIAN_POINT('Ctrl Pts',(-54.564136951052,-14.2615652592475,14.));
#66337=CARTESIAN_POINT('Ctrl Pts',(-54.5639906524104,-14.2748594650661,
14.));
#66338=CARTESIAN_POINT('Ctrl Pts',(-54.5636526398204,-14.2881640100053,
14.));
#66339=CARTESIAN_POINT('Ctrl Pts',(-54.5631231489384,-14.3014742844609,
14.));
#66340=CARTESIAN_POINT('Ctrl Pts',(-54.5627109268488,-14.3118366709255,
14.));
#66341=CARTESIAN_POINT('Ctrl Pts',(-54.5621824503484,-14.322204308924,14.));
#66342=CARTESIAN_POINT('Ctrl Pts',(-54.5615390811975,-14.3325581294891,
14.));
#66343=CARTESIAN_POINT('Ctrl Pts',(-54.5580964056233,-14.3879615399713,
14.));
#66344=CARTESIAN_POINT('Ctrl Pts',(-54.551365377527,-14.4430731532169,14.));
#66345=CARTESIAN_POINT('Ctrl Pts',(-54.5414407207137,-14.4975781576669,
14.));
#66346=CARTESIAN_POINT('Ctrl Pts',(-54.5315715932723,-14.5517782015807,
14.));
#66347=CARTESIAN_POINT('Ctrl Pts',(-54.5185439871495,-14.6053794990709,
14.));
#66348=CARTESIAN_POINT('Ctrl Pts',(-54.5024041439982,-14.6580525500535,
14.));
#66349=CARTESIAN_POINT('Ctrl Pts',(-54.4874293906239,-14.7069232819772,
14.));
#66350=CARTESIAN_POINT('Ctrl Pts',(-54.4697747813372,-14.7549954142157,
14.));
#66351=CARTESIAN_POINT('Ctrl Pts',(-54.4494461021838,-14.8019781702512,
14.));
#66352=CARTESIAN_POINT('Ctrl Pts',(-54.4442243438061,-14.8140464703156,
14.));
#66353=CARTESIAN_POINT('Ctrl Pts',(-54.4388239492052,-14.8260467746001,
14.));
#66354=CARTESIAN_POINT('Ctrl Pts',(-54.43325735223,-14.8379478524605,14.));
#66355=CARTESIAN_POINT('Ctrl Pts',(-54.4107559776503,-14.8860545524844,
14.));
#66356=CARTESIAN_POINT('Ctrl Pts',(-54.3855109054517,-14.9326200894641,
14.));
#66357=CARTESIAN_POINT('Ctrl Pts',(-54.3575738558942,-14.9773487851076,
14.));
#66358=CARTESIAN_POINT('Ctrl Pts',(-54.3305841285965,-15.0205607676511,
14.));
#66359=CARTESIAN_POINT('Ctrl Pts',(-54.3010813191933,-15.0620590195604,
14.));
#66360=CARTESIAN_POINT('Ctrl Pts',(-54.2690787903782,-15.1015427316642,
14.));
#66361=CARTESIAN_POINT('Ctrl Pts',(-54.246691332214,-15.129163672434,14.));
#66362=CARTESIAN_POINT('Ctrl Pts',(-54.2230798921333,-15.1557980567137,
14.));
#66363=CARTESIAN_POINT('Ctrl Pts',(-54.1982409588253,-15.1813299258066,
14.));
#66364=CARTESIAN_POINT('Ctrl Pts',(-54.1842289958931,-15.1957327827604,
14.));
#66365=CARTESIAN_POINT('Ctrl Pts',(-54.1698262703445,-15.2097845594384,
14.));
#66366=CARTESIAN_POINT('Ctrl Pts',(-54.1550492157917,-15.2234767486837,
14.));
#66367=CARTESIAN_POINT('Origin',(-53.1951359564886,-14.3971354987959,19.1042117235887));
#66368=CARTESIAN_POINT('Ctrl Pts',(-51.650238794436,-14.3978859537331,17.8542117235887));
#66369=CARTESIAN_POINT('Ctrl Pts',(-51.6499374336204,-14.4458116120497,
17.8517311518799));
#66370=CARTESIAN_POINT('Ctrl Pts',(-51.673532852059,-14.9990358635577,17.8230820767121));
#66371=CARTESIAN_POINT('Ctrl Pts',(-52.3387729531489,-15.9998443555804,
17.7682644980854));
#66372=CARTESIAN_POINT('Ctrl Pts',(-54.0595357659418,-15.9953385078432,
17.6897589877087));
#66373=CARTESIAN_POINT('Ctrl Pts',(-55.0050592474358,-14.557743765663,17.6112534773318));
#66374=CARTESIAN_POINT('Ctrl Pts',(-54.3274128937127,-12.9760039404155,
17.5327479669551));
#66375=CARTESIAN_POINT('Ctrl Pts',(-52.6343075214603,-12.6688220685915,
17.4542424565783));
#66376=CARTESIAN_POINT('Ctrl Pts',(-51.7321085269852,-13.6109301706732,
17.3947303754562));
#66377=CARTESIAN_POINT('Ctrl Pts',(-51.6515351015305,-14.2566054984256,
17.361386797793));
#66378=CARTESIAN_POINT('Ctrl Pts',(-51.652701124777,-14.3958311332085,17.3542117235887));
#66379=CARTESIAN_POINT('Ctrl Pts',(-51.6537934596095,-14.3955992295121,
17.8957882764113));
#66380=CARTESIAN_POINT('Ctrl Pts',(-51.6561292792194,-14.73752448157,17.8781885106897));
#66381=CARTESIAN_POINT('Ctrl Pts',(-51.9349899776299,-15.5924054167524,
17.8344202415091));
#66382=CARTESIAN_POINT('Ctrl Pts',(-53.3392724282712,-16.2080937050947,
17.7644834688697));
#66383=CARTESIAN_POINT('Ctrl Pts',(-54.7851641391705,-15.2764790675083,
17.6859779584929));
#66384=CARTESIAN_POINT('Ctrl Pts',(-54.8056647755616,-13.5555715973232,
17.6074724481161));
#66385=CARTESIAN_POINT('Ctrl Pts',(-53.3815155728066,-12.5897336831025,
17.5289669377393));
#66386=CARTESIAN_POINT('Ctrl Pts',(-51.9513720532365,-13.1783784136204,
17.458405547171));
#66387=CARTESIAN_POINT('Ctrl Pts',(-51.6558508817824,-14.0445039022943,
17.4140126600617));
#66388=CARTESIAN_POINT('Ctrl Pts',(-51.6531013855762,-14.3983675031589,
17.3957882764113));
#66389=CARTESIAN_POINT('Ctrl Pts',(-54.153252109211,-15.2223467977324,18.));
#66390=CARTESIAN_POINT('Ctrl Pts',(-54.4246171615437,-14.9072768995629,
17.9738314965411));
#66391=CARTESIAN_POINT('Ctrl Pts',(-54.6278752336732,-13.9937540324533,
17.9214944896232));
#66392=CARTESIAN_POINT('Ctrl Pts',(-53.6477056068469,-12.9776474013965,
17.8429889792464));
#66393=CARTESIAN_POINT('Ctrl Pts',(-52.2613397426835,-13.2376039347744,
17.7644834688697));
#66394=CARTESIAN_POINT('Ctrl Pts',(-51.7125907601688,-14.5359830763925,
17.6859779584929));
#66395=CARTESIAN_POINT('Ctrl Pts',(-52.4933400927667,-15.7105673519417,
17.6074724481161));
#66396=CARTESIAN_POINT('Ctrl Pts',(-53.903518042719,-15.7068747761389,17.5289669377394));
#66397=CARTESIAN_POINT('Ctrl Pts',(-54.6783815828028,-14.5287551705091,
17.4504614273625));
#66398=CARTESIAN_POINT('Ctrl Pts',(-54.1230453454191,-13.2325075949904,
17.3719559169858));
#66399=CARTESIAN_POINT('Ctrl Pts',(-52.7355328741211,-12.9807697615999,
17.293450406609));
#66400=CARTESIAN_POINT('Ctrl Pts',(-51.7602058672859,-13.9992407208286,
17.2149448962322));
#66401=CARTESIAN_POINT('Ctrl Pts',(-52.0717570426275,-15.3745639123133,
17.1364393858554));
#66402=CARTESIAN_POINT('Ctrl Pts',(-53.390781746669,-15.8733007472588,17.0579338754786));
#66403=CARTESIAN_POINT('Ctrl Pts',(-54.5343463517261,-15.0481801280675,
16.9794283651019));
#66404=CARTESIAN_POINT('Ctrl Pts',(-54.4768753865949,-13.6391859025932,
16.9009228547251));
#66405=CARTESIAN_POINT('Ctrl Pts',(-53.2699099545465,-12.9099395406961,
16.8224173443483));
#66406=CARTESIAN_POINT('Ctrl Pts',(-51.9958854602389,-13.5144455498356,
16.7439118339715));
#66407=CARTESIAN_POINT('Ctrl Pts',(-51.7973773032626,-14.9105690485955,
16.6654063235948));
#66408=CARTESIAN_POINT('Ctrl Pts',(-52.8524123453517,-15.8462330551256,
16.586900813218));
#66409=CARTESIAN_POINT('Ctrl Pts',(-54.2148100652166,-15.4823119617458,
16.5083953028412));
#66410=CARTESIAN_POINT('Ctrl Pts',(-54.6627398052285,-14.1451787985144,
16.4298897924644));
#66411=CARTESIAN_POINT('Ctrl Pts',(-53.7944875223078,-13.0340064035767,
16.3513842820877));
#66412=CARTESIAN_POINT('Ctrl Pts',(-52.3887225069356,-13.145320583037,16.2728787717108));
#66413=CARTESIAN_POINT('Ctrl Pts',(-51.706168244238,-14.3792921414933,16.1943732613341));
#66414=CARTESIAN_POINT('Ctrl Pts',(-52.3589556241958,-15.6292660458124,
16.1158677509573));
#66415=CARTESIAN_POINT('Ctrl Pts',(-53.7616494051484,-15.7742359839284,
16.0373622405805));
#66416=CARTESIAN_POINT('Ctrl Pts',(-54.6562804572666,-14.6841894679763,
15.9588567302037));
#66417=CARTESIAN_POINT('Ctrl Pts',(-54.2405223843948,-13.33670612834,15.880351219827));
#66418=CARTESIAN_POINT('Ctrl Pts',(-52.8872369102522,-12.9402410582164,
15.8018457094502));
#66419=CARTESIAN_POINT('Ctrl Pts',(-51.8100826208389,-13.8503535583387,
15.7233401990734));
#66420=CARTESIAN_POINT('Ctrl Pts',(-51.9750770902176,-15.2508331012045,
15.6448346886966));
#66421=CARTESIAN_POINT('Ctrl Pts',(-53.2342493568711,-15.885696339624,15.5663291783198));
#66422=CARTESIAN_POINT('Ctrl Pts',(-54.4583437946506,-15.1855828256918,
15.4878236679431));
#66423=CARTESIAN_POINT('Ctrl Pts',(-54.549563415235,-13.7783710083418,15.4093181575663));
#66424=CARTESIAN_POINT('Ctrl Pts',(-53.4261002848556,-12.9260818890411,
15.3308126471895));
#66425=CARTESIAN_POINT('Ctrl Pts',(-52.0955028666328,-13.393068633948,15.2523071368127));
#66426=CARTESIAN_POINT('Ctrl Pts',(-51.751082520038,-14.7605263839362,15.1738016264359));
#66427=CARTESIAN_POINT('Ctrl Pts',(-52.7017236774067,-15.8020866088358,
15.0952961160592));
#66428=CARTESIAN_POINT('Ctrl Pts',(-54.0948685923953,-15.5836531566747,
15.0167906056824));
#66429=CARTESIAN_POINT('Ctrl Pts',(-54.6811121004696,-14.3011227048956,
14.9382850953056));
#66430=CARTESIAN_POINT('Ctrl Pts',(-53.9346964498466,-13.1046983170808,
14.8597795849288));
#66431=CARTESIAN_POINT('Ctrl Pts',(-52.5250262261246,-13.0673633133234,
14.781274074552));
#66432=CARTESIAN_POINT('Ctrl Pts',(-51.7163246046947,-14.2225976133251,
14.7027685641753));
#66433=CARTESIAN_POINT('Ctrl Pts',(-52.2338596624079,-15.5343656873115,
14.6242630537985));
#66434=CARTESIAN_POINT('Ctrl Pts',(-53.6134830839557,-15.8262305186475,
14.5457575434217));
#66435=CARTESIAN_POINT('Ctrl Pts',(-54.6179371276052,-14.8364654611899,
14.4672520330449));
#66436=CARTESIAN_POINT('Ctrl Pts',(-54.3463604457024,-13.4526655408848,
14.3887465226682));
#66437=CARTESIAN_POINT('Ctrl Pts',(-53.0423964320333,-12.9159559714002,
14.3102410122914));
#66438=CARTESIAN_POINT('Ctrl Pts',(-51.8752954493436,-13.7074676781063,
14.2317355019146));
#66439=CARTESIAN_POINT('Ctrl Pts',(-51.8920958234221,-15.1177639193799,
14.1532299915378));
#66440=CARTESIAN_POINT('Ctrl Pts',(-53.0770150197731,-15.881229923416,14.074724481161));
#66441=CARTESIAN_POINT('Ctrl Pts',(-54.3688351006163,-15.3148479080822,
13.9962189707843));
#66442=CARTESIAN_POINT('Ctrl Pts',(-54.6060800258316,-13.9231151648839,
13.9177134604075));
#66443=CARTESIAN_POINT('Ctrl Pts',(-53.9234352130359,-13.2829324314546,
13.8653764534896));
#66444=CARTESIAN_POINT('Ctrl Pts',(-53.5217210200197,-13.1755371825403,
13.8392079500307));
#66445=CARTESIAN_POINT('Ctrl Pts',(-54.2235922564453,-15.2829297282066,
18.0535973499898));
#66446=CARTESIAN_POINT('Ctrl Pts',(-54.514879588223,-14.9447289570595,18.0274288465308));
#66447=CARTESIAN_POINT('Ctrl Pts',(-54.7330598623,-13.9641397611006,17.975091839613));
#66448=CARTESIAN_POINT('Ctrl Pts',(-53.68093103129,-12.8734356088235,17.8965863292362));
#66449=CARTESIAN_POINT('Ctrl Pts',(-52.192785045031,-13.1524768646333,17.8180808188594));
#66450=CARTESIAN_POINT('Ctrl Pts',(-51.6037496273957,-14.5461765785306,
17.7395753084826));
#66451=CARTESIAN_POINT('Ctrl Pts',(-52.441817712894,-15.8069930198213,17.6610697981059));
#66452=CARTESIAN_POINT('Ctrl Pts',(-53.95552395046,-15.8030293533737,17.5825642877291));
#66453=CARTESIAN_POINT('Ctrl Pts',(-54.7872741376805,-14.5384180355604,
17.5040587773523));
#66454=CARTESIAN_POINT('Ctrl Pts',(-54.1911678615169,-13.1470063767988,
17.4255532669755));
#66455=CARTESIAN_POINT('Ctrl Pts',(-52.7017910899008,-12.8767871972638,
17.3470477565988));
#66456=CARTESIAN_POINT('Ctrl Pts',(-51.6548604000807,-13.9700292549886,
17.268542246222));
#66457=CARTESIAN_POINT('Ctrl Pts',(-51.9892841211801,-15.4463218701793,
17.1900367358452));
#66458=CARTESIAN_POINT('Ctrl Pts',(-53.405145092541,-15.9816734958279,17.1115312254684));
#66459=CARTESIAN_POINT('Ctrl Pts',(-54.6326645526155,-15.0959766034206,
17.0330257150916));
#66460=CARTESIAN_POINT('Ctrl Pts',(-54.5709743535871,-13.5835409935271,
16.9545202047149));
#66461=CARTESIAN_POINT('Ctrl Pts',(-53.2753994915068,-12.8007569720048,
16.8760146943381));
#66462=CARTESIAN_POINT('Ctrl Pts',(-51.9078424226205,-13.4496428212774,
16.7975091839613));
#66463=CARTESIAN_POINT('Ctrl Pts',(-51.6947607789649,-14.9482627993849,
16.7190036735845));
#66464=CARTESIAN_POINT('Ctrl Pts',(-52.8272512735969,-15.9526186276675,
16.6404981632078));
#66465=CARTESIAN_POINT('Ctrl Pts',(-54.2896694929959,-15.5619802482706,
16.5619926528309));
#66466=CARTESIAN_POINT('Ctrl Pts',(-54.7704840181913,-14.1266813842457,
16.4834871424542));
#66467=CARTESIAN_POINT('Ctrl Pts',(-53.8384889487163,-12.9339322100829,
16.4049816320774));
#66468=CARTESIAN_POINT('Ctrl Pts',(-52.3295196215526,-13.0534185258236,
16.3264761217006));
#66469=CARTESIAN_POINT('Ctrl Pts',(-51.5968556021234,-14.377982170488,16.2479706113238));
#66470=CARTESIAN_POINT('Ctrl Pts',(-52.2975674015667,-15.7197229740698,
16.1694651009471));
#66471=CARTESIAN_POINT('Ctrl Pts',(-53.803240019476,-15.8753358877401,16.0909595905703));
#66472=CARTESIAN_POINT('Ctrl Pts',(-54.7635504568624,-14.7052635500685,
16.0124540801935));
#66473=CARTESIAN_POINT('Ctrl Pts',(-54.3172694834252,-13.2588546508992,
15.9339485698167));
#66474=CARTESIAN_POINT('Ctrl Pts',(-52.8646324857427,-12.8332830770114,
15.8554430594399));
#66475=CARTESIAN_POINT('Ctrl Pts',(-51.7083988580924,-13.8102115337131,
15.7769375490632));
#66476=CARTESIAN_POINT('Ctrl Pts',(-51.8855064050308,-15.3135073551311,
15.6984320386864));
#66477=CARTESIAN_POINT('Ctrl Pts',(-53.2371208691966,-15.994979111252,15.6199265283096));
#66478=CARTESIAN_POINT('Ctrl Pts',(-54.5510822638553,-15.2434667272446,
15.5414210179328));
#66479=CARTESIAN_POINT('Ctrl Pts',(-54.6489987776341,-13.7329443810606,
15.4629155075561));
#66480=CARTESIAN_POINT('Ctrl Pts',(-53.4430565430473,-12.8180844116938,
15.3844099971793));
#66481=CARTESIAN_POINT('Ctrl Pts',(-52.0147732460912,-13.3193550127907,
15.3059044868025));
#66482=CARTESIAN_POINT('Ctrl Pts',(-51.6450672618196,-14.787204744688,15.2273989764257));
#66483=CARTESIAN_POINT('Ctrl Pts',(-52.6654997892495,-15.9052311677249,
15.1488934660489));
#66484=CARTESIAN_POINT('Ctrl Pts',(-54.160922510703,-15.6707614123012,15.0703879556721));
#66485=CARTESIAN_POINT('Ctrl Pts',(-54.7902051164439,-14.2940739206327,
14.9918824452954));
#66486=CARTESIAN_POINT('Ctrl Pts',(-53.9889913219701,-13.0098139740974,
14.9133769349186));
#66487=CARTESIAN_POINT('Ctrl Pts',(-52.4758300853821,-12.9697380190954,
14.8348714245418));
#66488=CARTESIAN_POINT('Ctrl Pts',(-51.6077575923118,-14.2097839053763,
14.756365914165));
#66489=CARTESIAN_POINT('Ctrl Pts',(-52.1632875132312,-15.6178555008087,
14.6778604037883));
#66490=CARTESIAN_POINT('Ctrl Pts',(-53.644196060099,-15.9311476039325,14.5993548934115));
#66491=CARTESIAN_POINT('Ctrl Pts',(-54.7223921496577,-14.8687188932518,
14.5208493830347));
#66492=CARTESIAN_POINT('Ctrl Pts',(-54.4308776515139,-13.3833272297531,
14.4423438726579));
#66493=CARTESIAN_POINT('Ctrl Pts',(-53.0311830518934,-12.8072150992822,
14.3638383622811));
#66494=CARTESIAN_POINT('Ctrl Pts',(-51.778399289797,-13.6568356791444,14.2853328519043));
#66495=CARTESIAN_POINT('Ctrl Pts',(-51.7964330642132,-15.1706688923949,
14.2068273415276));
#66496=CARTESIAN_POINT('Ctrl Pts',(-53.0683431650544,-15.9901847928655,
14.1283218311508));
#66497=CARTESIAN_POINT('Ctrl Pts',(-54.4550022843884,-15.3822218123885,
14.049816320774));
#66498=CARTESIAN_POINT('Ctrl Pts',(-54.70966455814,-13.888314937391,13.9713108103972));
#66499=CARTESIAN_POINT('Ctrl Pts',(-53.9769033408726,-13.2011331552573,
13.9189738034794));
#66500=CARTESIAN_POINT('Ctrl Pts',(-53.5456972794617,-13.0858534785527,
13.8928053000205));
#66501=CARTESIAN_POINT('Ctrl Pts',(-54.2939324036796,-15.3435126586807,
18.1071946999795));
#66502=CARTESIAN_POINT('Ctrl Pts',(-54.6051420149022,-14.9821810145562,
18.0810261965206));
#66503=CARTESIAN_POINT('Ctrl Pts',(-54.8382444909268,-13.934525489748,18.0286891896028));
#66504=CARTESIAN_POINT('Ctrl Pts',(-53.7141564557331,-12.7692238162505,
17.950183679226));
#66505=CARTESIAN_POINT('Ctrl Pts',(-52.1242303473785,-13.0673497944923,
17.8716781688492));
#66506=CARTESIAN_POINT('Ctrl Pts',(-51.4949084946225,-14.5563700806686,
17.7931726584724));
#66507=CARTESIAN_POINT('Ctrl Pts',(-52.3902953330214,-15.9034186877009,
17.7146671480956));
#66508=CARTESIAN_POINT('Ctrl Pts',(-54.0075298582009,-15.8991839306084,
17.6361616377189));
#66509=CARTESIAN_POINT('Ctrl Pts',(-54.8961666925581,-14.5480809006117,
17.5576561273421));
#66510=CARTESIAN_POINT('Ctrl Pts',(-54.2592903776148,-13.0615051586072,
17.4791506169653));
#66511=CARTESIAN_POINT('Ctrl Pts',(-52.6680493056806,-12.7728046329277,
17.4006451065885));
#66512=CARTESIAN_POINT('Ctrl Pts',(-51.5495149328755,-13.9408177891487,
17.3221395962117));
#66513=CARTESIAN_POINT('Ctrl Pts',(-51.9068111997328,-15.5180798280453,
17.243634085835));
#66514=CARTESIAN_POINT('Ctrl Pts',(-53.419508438413,-16.090046244397,17.1651285754582));
#66515=CARTESIAN_POINT('Ctrl Pts',(-54.7309827535048,-15.1437730787738,
17.0866230650814));
#66516=CARTESIAN_POINT('Ctrl Pts',(-54.6650733205792,-13.5278960844609,
17.0081175547046));
#66517=CARTESIAN_POINT('Ctrl Pts',(-53.2808890284672,-12.6915744033134,
16.9296120443278));
#66518=CARTESIAN_POINT('Ctrl Pts',(-51.819799385002,-13.3848400927192,16.8511065339511));
#66519=CARTESIAN_POINT('Ctrl Pts',(-51.5921442546672,-14.9859565501742,
16.7726010235743));
#66520=CARTESIAN_POINT('Ctrl Pts',(-52.8020902018422,-16.0590042002094,
16.6940955131975));
#66521=CARTESIAN_POINT('Ctrl Pts',(-54.3645289207752,-15.6416485347953,
16.6155900028207));
#66522=CARTESIAN_POINT('Ctrl Pts',(-54.878228231154,-14.108183969977,16.5370844924439));
#66523=CARTESIAN_POINT('Ctrl Pts',(-53.8824903751248,-12.8338580165892,
16.4585789820672));
#66524=CARTESIAN_POINT('Ctrl Pts',(-52.2703167361696,-12.9615164686102,
16.3800734716904));
#66525=CARTESIAN_POINT('Ctrl Pts',(-51.4875429600088,-14.3766721994827,
16.3015679613136));
#66526=CARTESIAN_POINT('Ctrl Pts',(-52.2361791789376,-15.8101799023271,
16.2230624509368));
#66527=CARTESIAN_POINT('Ctrl Pts',(-53.8448306338036,-15.9764357915517,
16.1445569405601));
#66528=CARTESIAN_POINT('Ctrl Pts',(-54.8708204564582,-14.7263376321606,
16.0660514301833));
#66529=CARTESIAN_POINT('Ctrl Pts',(-54.3940165824557,-13.1810031734583,
15.9875459198065));
#66530=CARTESIAN_POINT('Ctrl Pts',(-52.8420280612331,-12.7263250958063,
15.9090404094297));
#66531=CARTESIAN_POINT('Ctrl Pts',(-51.6067150953462,-13.7700695090875,
15.8305348990529));
#66532=CARTESIAN_POINT('Ctrl Pts',(-51.7959357198438,-15.3761816090578,
15.7520293886762));
#66533=CARTESIAN_POINT('Ctrl Pts',(-53.2399923815221,-16.1042618828799,
15.6735238782994));
#66534=CARTESIAN_POINT('Ctrl Pts',(-54.6438207330599,-15.3013506287974,
15.5950183679226));
#66535=CARTESIAN_POINT('Ctrl Pts',(-54.7484341400332,-13.6875177537793,
15.5165128575458));
#66536=CARTESIAN_POINT('Ctrl Pts',(-53.460012801239,-12.7100869343466,15.438007347169));
#66537=CARTESIAN_POINT('Ctrl Pts',(-51.9340436255495,-13.2456413916334,
15.3595018367923));
#66538=CARTESIAN_POINT('Ctrl Pts',(-51.5390520036012,-14.8138831054396,
15.2809963264155));
#66539=CARTESIAN_POINT('Ctrl Pts',(-52.6292759010924,-16.0083757266141,
15.2024908160387));
#66540=CARTESIAN_POINT('Ctrl Pts',(-54.2269764290105,-15.7578696679277,
15.1239853056619));
#66541=CARTESIAN_POINT('Ctrl Pts',(-54.8992981324183,-14.2870251363698,
15.0454797952851));
#66542=CARTESIAN_POINT('Ctrl Pts',(-54.0432861940934,-12.914929631114,14.9669742849084));
#66543=CARTESIAN_POINT('Ctrl Pts',(-52.4266339446397,-12.8721127248673,
14.8884687745316));
#66544=CARTESIAN_POINT('Ctrl Pts',(-51.4991905799289,-14.1969701974275,
14.8099632641548));
#66545=CARTESIAN_POINT('Ctrl Pts',(-52.0927153640546,-15.7013453143059,
14.731457753778));
#66546=CARTESIAN_POINT('Ctrl Pts',(-53.6749090362423,-16.0360646892175,
14.6529522434013));
#66547=CARTESIAN_POINT('Ctrl Pts',(-54.8268471717101,-14.9009723253137,
14.5744467330245));
#66548=CARTESIAN_POINT('Ctrl Pts',(-54.5153948573255,-13.3139889186213,
14.4959412226477));
#66549=CARTESIAN_POINT('Ctrl Pts',(-53.0199696717534,-12.6984742271642,
14.4174357122709));
#66550=CARTESIAN_POINT('Ctrl Pts',(-51.6815031302505,-13.6062036801825,
14.3389302018941));
#66551=CARTESIAN_POINT('Ctrl Pts',(-51.7007703050042,-15.22357386541,14.2604246915173));
#66552=CARTESIAN_POINT('Ctrl Pts',(-53.0596713103357,-16.099139662315,14.1819191811406));
#66553=CARTESIAN_POINT('Ctrl Pts',(-54.5411694681605,-15.4495957166949,
14.1034136707638));
#66554=CARTESIAN_POINT('Ctrl Pts',(-54.8132490904484,-13.853514709898,14.024908160387));
#66555=CARTESIAN_POINT('Ctrl Pts',(-54.0303714687093,-13.11933387906,13.9725711534692));
#66556=CARTESIAN_POINT('Ctrl Pts',(-53.5696735389038,-12.996169774565,13.9464026500102));
#66557=CARTESIAN_POINT('Ctrl Pts',(-54.3642725509138,-15.4040955891549,
18.1607920499693));
#66558=CARTESIAN_POINT('Ctrl Pts',(-54.6954044415815,-15.0196330720529,
18.1346235465104));
#66559=CARTESIAN_POINT('Ctrl Pts',(-54.9434291195537,-13.9049112183953,
18.0822865395925));
#66560=CARTESIAN_POINT('Ctrl Pts',(-53.7473818801761,-12.6650120236775,
18.0037810292157));
#66561=CARTESIAN_POINT('Ctrl Pts',(-52.055675649726,-12.9822227243512,17.925275518839));
#66562=CARTESIAN_POINT('Ctrl Pts',(-51.3860673618493,-14.5665635828067,
17.8467700084622));
#66563=CARTESIAN_POINT('Ctrl Pts',(-52.3387729531489,-15.9998443555804,
17.7682644980854));
#66564=CARTESIAN_POINT('Ctrl Pts',(-54.0595357659418,-15.9953385078432,
17.6897589877087));
#66565=CARTESIAN_POINT('Ctrl Pts',(-55.0050592474358,-14.557743765663,17.6112534773318));
#66566=CARTESIAN_POINT('Ctrl Pts',(-54.3274128937127,-12.9760039404155,
17.5327479669551));
#66567=CARTESIAN_POINT('Ctrl Pts',(-52.6343075214603,-12.6688220685915,
17.4542424565783));
#66568=CARTESIAN_POINT('Ctrl Pts',(-51.4441694656704,-13.9116063233087,
17.3757369462015));
#66569=CARTESIAN_POINT('Ctrl Pts',(-51.8243382782854,-15.5898377859113,
17.2972314358247));
#66570=CARTESIAN_POINT('Ctrl Pts',(-53.4338717842849,-16.1984189929661,
17.218725925448));
#66571=CARTESIAN_POINT('Ctrl Pts',(-54.829300954394,-15.1915695541269,17.1402204150712));
#66572=CARTESIAN_POINT('Ctrl Pts',(-54.7591722875713,-13.4722511753948,
17.0617149046944));
#66573=CARTESIAN_POINT('Ctrl Pts',(-53.2863785654275,-12.582391834622,16.9832093943176));
#66574=CARTESIAN_POINT('Ctrl Pts',(-51.7317563473836,-13.320037364161,16.9047038839409));
#66575=CARTESIAN_POINT('Ctrl Pts',(-51.4895277303695,-15.0236503009635,
16.8261983735641));
#66576=CARTESIAN_POINT('Ctrl Pts',(-52.7769291300874,-16.1653897727513,
16.7476928631873));
#66577=CARTESIAN_POINT('Ctrl Pts',(-54.4393883485545,-15.72131682132,16.6691873528105));
#66578=CARTESIAN_POINT('Ctrl Pts',(-54.9859724441167,-14.0896865557083,
16.5906818424337));
#66579=CARTESIAN_POINT('Ctrl Pts',(-53.9264918015333,-12.7337838230954,
16.5121763320569));
#66580=CARTESIAN_POINT('Ctrl Pts',(-52.2111138507866,-12.8696144113969,
16.4336708216802));
#66581=CARTESIAN_POINT('Ctrl Pts',(-51.3782303178942,-14.3753622284773,
16.3551653113034));
#66582=CARTESIAN_POINT('Ctrl Pts',(-52.1747909563085,-15.9006368305844,
16.2766598009266));
#66583=CARTESIAN_POINT('Ctrl Pts',(-53.8864212481312,-16.0775356953633,
16.1981542905498));
#66584=CARTESIAN_POINT('Ctrl Pts',(-54.978090456054,-14.7474117142528,16.119648780173));
#66585=CARTESIAN_POINT('Ctrl Pts',(-54.4707636814861,-13.1031516960174,
16.0411432697963));
#66586=CARTESIAN_POINT('Ctrl Pts',(-52.8194236367236,-12.6193671146013,
15.9626377594195));
#66587=CARTESIAN_POINT('Ctrl Pts',(-51.5050313325997,-13.7299274844619,
15.8841322490427));
#66588=CARTESIAN_POINT('Ctrl Pts',(-51.706365034657,-15.4388558629844,15.8056267386659));
#66589=CARTESIAN_POINT('Ctrl Pts',(-53.2428638938474,-16.2135446545079,
15.7271212282891));
#66590=CARTESIAN_POINT('Ctrl Pts',(-54.7365592022647,-15.3592345303502,
15.6486157179124));
#66591=CARTESIAN_POINT('Ctrl Pts',(-54.8478695024322,-13.6420911264981,
15.5701102075356));
#66592=CARTESIAN_POINT('Ctrl Pts',(-53.4769690594307,-12.6020894569994,
15.4916046971588));
#66593=CARTESIAN_POINT('Ctrl Pts',(-51.8533140050079,-13.1719277704761,
15.413099186782));
#66594=CARTESIAN_POINT('Ctrl Pts',(-51.4330367453828,-14.8405614661914,
15.3345936764053));
#66595=CARTESIAN_POINT('Ctrl Pts',(-52.5930520129352,-16.1115202855033,
15.2560881660285));
#66596=CARTESIAN_POINT('Ctrl Pts',(-54.2930303473181,-15.8449779235543,
15.1775826556517));
#66597=CARTESIAN_POINT('Ctrl Pts',(-55.0083911483927,-14.2799763521069,
15.0990771452749));
#66598=CARTESIAN_POINT('Ctrl Pts',(-54.0975810662168,-12.8200452881305,
15.0205716348981));
#66599=CARTESIAN_POINT('Ctrl Pts',(-52.3774378038974,-12.7744874306393,
14.9420661245214));
#66600=CARTESIAN_POINT('Ctrl Pts',(-51.3906235675459,-14.1841564894788,
14.8635606141446));
#66601=CARTESIAN_POINT('Ctrl Pts',(-52.0221432148781,-15.784835127803,14.7850551037678));
#66602=CARTESIAN_POINT('Ctrl Pts',(-53.7056220123855,-16.1409817745025,
14.706549593391));
#66603=CARTESIAN_POINT('Ctrl Pts',(-54.9313021937626,-14.9332257573755,
14.6280440830142));
#66604=CARTESIAN_POINT('Ctrl Pts',(-54.599912063137,-13.2446506074896,14.5495385726375));
#66605=CARTESIAN_POINT('Ctrl Pts',(-53.0087562916135,-12.5897333550461,
14.4710330622607));
#66606=CARTESIAN_POINT('Ctrl Pts',(-51.584606970704,-13.5555716812206,14.3925275518839));
#66607=CARTESIAN_POINT('Ctrl Pts',(-51.6051075457953,-15.276478838425,14.3140220415071));
#66608=CARTESIAN_POINT('Ctrl Pts',(-53.0509994556171,-16.2080945317645,
14.2355165311303));
#66609=CARTESIAN_POINT('Ctrl Pts',(-54.6273366519326,-15.5169696210013,
14.1570110207536));
#66610=CARTESIAN_POINT('Ctrl Pts',(-54.9168336227569,-13.8187144824051,
14.0785055103768));
#66611=CARTESIAN_POINT('Ctrl Pts',(-54.083839596546,-13.0375346028626,14.0261685034589));
#66612=CARTESIAN_POINT('Ctrl Pts',(-53.5936497983459,-12.9064860705774,
14.));
#66613=CARTESIAN_POINT('Ctrl Pts',(-51.9310991161132,-14.3960665614756,
17.1934196736194));
#66614=CARTESIAN_POINT('Ctrl Pts',(-51.9301435513723,-14.2819701161204,
17.2005947478237));
#66615=CARTESIAN_POINT('Ctrl Pts',(-51.944352401566,-14.1681074628443,17.2077698220279));
#66616=CARTESIAN_POINT('Ctrl Pts',(-51.9746855643153,-14.0587160928713,
17.2149448962322));
#66617=CARTESIAN_POINT('Ctrl Pts',(-52.0853148695643,-13.6597504010857,
17.2411133996911));
#66618=CARTESIAN_POINT('Ctrl Pts',(-52.4104238718427,-13.3202600813428,
17.26728190315));
#66619=CARTESIAN_POINT('Ctrl Pts',(-52.8042304515315,-13.1924712270364,
17.293450406609));
#66620=CARTESIAN_POINT('Ctrl Pts',(-53.1980370312204,-13.0646823727301,
17.3196189100679));
#66621=CARTESIAN_POINT('Ctrl Pts',(-53.6605411883197,-13.1485949838602,
17.3457874135268));
#66622=CARTESIAN_POINT('Ctrl Pts',(-53.9843493064334,-13.4065925520117,
17.3719559169858));
#66623=CARTESIAN_POINT('Ctrl Pts',(-54.308157424547,-13.6645901201633,17.3981244204447));
#66624=CARTESIAN_POINT('Ctrl Pts',(-54.4932695036749,-14.0966726453362,
17.4242929239036));
#66625=CARTESIAN_POINT('Ctrl Pts',(-54.4566816198916,-14.5090671755276,
17.4504614273625));
#66626=CARTESIAN_POINT('Ctrl Pts',(-54.4200937361082,-14.921461705719,17.4766299308214));
#66627=CARTESIAN_POINT('Ctrl Pts',(-54.1618058894136,-15.314168240929,17.5027984342804));
#66628=CARTESIAN_POINT('Ctrl Pts',(-53.7976323077409,-15.5111369378344,
17.5289669377393));
#66629=CARTESIAN_POINT('Ctrl Pts',(-53.4334587260682,-15.7081056347398,
17.5551354411983));
#66630=CARTESIAN_POINT('Ctrl Pts',(-52.9633994094174,-15.7093364933408,
17.5813039446572));
#66631=CARTESIAN_POINT('Ctrl Pts',(-52.5982448623257,-15.5141878767164,
17.6074724481161));
#66632=CARTESIAN_POINT('Ctrl Pts',(-52.233090315234,-15.319039260092,17.633640951575));
#66633=CARTESIAN_POINT('Ctrl Pts',(-51.9728405377014,-14.9275111682423,
17.659809455034));
#66634=CARTESIAN_POINT('Ctrl Pts',(-51.9341738126876,-14.5153505987144,
17.6859779584929));
#66635=CARTESIAN_POINT('Ctrl Pts',(-51.9305085062518,-14.4762809648747,
17.6884585302017));
#66636=CARTESIAN_POINT('Ctrl Pts',(-51.9288342506125,-14.4370259363911,
17.6909391019106));
#66637=CARTESIAN_POINT('Ctrl Pts',(-51.929081218047,-14.3977505022101,17.6934196736194));
#66638=CARTESIAN_POINT('Ctrl Pts',(-52.7966221146314,-12.9064860705774,
18.));
#66639=CARTESIAN_POINT('Ctrl Pts',(-52.3064323164313,-13.0375346028627,
17.9738314965411));
#66640=CARTESIAN_POINT('Ctrl Pts',(-51.4734379005318,-13.818711947887,17.9214944896232));
#66641=CARTESIAN_POINT('Ctrl Pts',(-51.7629355980163,-15.5169705450585,
17.8429889792465));
#66642=CARTESIAN_POINT('Ctrl Pts',(-53.3392724282712,-16.2080937050947,
17.7644834688697));
#66643=CARTESIAN_POINT('Ctrl Pts',(-54.7851641391705,-15.2764790675083,
17.6859779584929));
#66644=CARTESIAN_POINT('Ctrl Pts',(-54.8056647755616,-13.5555715973232,
17.6074724481161));
#66645=CARTESIAN_POINT('Ctrl Pts',(-53.3815155728066,-12.5897336831025,
17.5289669377393));
#66646=CARTESIAN_POINT('Ctrl Pts',(-51.7903600412662,-13.244650694059,17.4504614273625));
#66647=CARTESIAN_POINT('Ctrl Pts',(-51.4589699241079,-14.9332257213623,
17.3719559169858));
#66648=CARTESIAN_POINT('Ctrl Pts',(-52.6846499703254,-16.1409815416267,
17.293450406609));
#66649=CARTESIAN_POINT('Ctrl Pts',(-54.3681285487899,-15.7848349642756,
17.2149448962322));
#66650=CARTESIAN_POINT('Ctrl Pts',(-54.9996481235109,-14.1841565112764,
17.1364393858554));
#66651=CARTESIAN_POINT('Ctrl Pts',(-54.0128340063977,-12.7744876345319,
17.0579338754786));
#66652=CARTESIAN_POINT('Ctrl Pts',(-52.292690959438,-12.8200454826231,16.9794283651019));
#66653=CARTESIAN_POINT('Ctrl Pts',(-51.3818809893341,-14.2799763673288,
16.9009228547251));
#66654=CARTESIAN_POINT('Ctrl Pts',(-52.0972417021453,-15.8449777434614,
16.8224173443483));
#66655=CARTESIAN_POINT('Ctrl Pts',(-53.7972198251955,-16.11152007286,16.7439118339715));
#66656=CARTESIAN_POINT('Ctrl Pts',(-54.9572349488979,-14.8405614110472,
16.6654063235947));
#66657=CARTESIAN_POINT('Ctrl Pts',(-54.5369577413632,-13.1719279226262,
16.586900813218));
#66658=CARTESIAN_POINT('Ctrl Pts',(-52.9133028885493,-12.602089679815,16.5083953028412));
#66659=CARTESIAN_POINT('Ctrl Pts',(-51.5424026157113,-13.6420912202446,
16.4298897924644));
#66660=CARTESIAN_POINT('Ctrl Pts',(-51.6537129020729,-15.359234410906,16.3513842820876));
#66661=CARTESIAN_POINT('Ctrl Pts',(-53.1474080250528,-16.2135444290179,
16.2728787717108));
#66662=CARTESIAN_POINT('Ctrl Pts',(-54.6839066935018,-15.4388557336608,
16.1943732613341));
#66663=CARTESIAN_POINT('Ctrl Pts',(-54.8852403705632,-13.7299275672916,
16.1158677509573));
#66664=CARTESIAN_POINT('Ctrl Pts',(-53.570848229612,-12.6193673352972,16.0373622405805));
#66665=CARTESIAN_POINT('Ctrl Pts',(-51.9195083898505,-13.1031518566562,
15.9588567302037));
#66666=CARTESIAN_POINT('Ctrl Pts',(-51.4121816782638,-14.7474116707683,
15.8803512198269));
#66667=CARTESIAN_POINT('Ctrl Pts',(-52.503850750664,-16.077535486755,15.8018457094502));
#66668=CARTESIAN_POINT('Ctrl Pts',(-54.2154808300007,-15.9006366439348,
15.7233401990734));
#66669=CARTESIAN_POINT('Ctrl Pts',(-55.0120413695279,-14.3753622311824,
15.6448346886966));
#66670=CARTESIAN_POINT('Ctrl Pts',(-54.1791579400319,-12.8696146010229,
15.5663291783198));
#66671=CARTESIAN_POINT('Ctrl Pts',(-52.4637802022359,-12.7337840295961,
15.4878236679431));
#66672=CARTESIAN_POINT('Ctrl Pts',(-51.4042996911802,-14.0896865938602,
15.4093181575663));
#66673=CARTESIAN_POINT('Ctrl Pts',(-51.9508837188856,-15.7213166569629,
15.3308126471895));
#66674=CARTESIAN_POINT('Ctrl Pts',(-53.6133427309768,-16.1653895531783,
15.2523071368127));
#66675=CARTESIAN_POINT('Ctrl Pts',(-54.9007439708605,-15.0236502232965,
15.1738016264359));
#66676=CARTESIAN_POINT('Ctrl Pts',(-54.6585153839456,-13.3200374976642,
15.0952961160592));
#66677=CARTESIAN_POINT('Ctrl Pts',(-53.1038933588347,-12.5823920603089,
15.0167906056824));
#66678=CARTESIAN_POINT('Ctrl Pts',(-51.6310998196598,-13.4722512894541,
14.9382850953056));
#66679=CARTESIAN_POINT('Ctrl Pts',(-51.5609711612584,-15.1915694569347,
14.8597795849288));
#66680=CARTESIAN_POINT('Ctrl Pts',(-52.9564001587445,-16.1984187666639,
14.7812740745521));
#66681=CARTESIAN_POINT('Ctrl Pts',(-54.5659334636339,-15.5898376428623,
14.7027685641752));
#66682=CARTESIAN_POINT('Ctrl Pts',(-54.9461022318155,-13.911606374279,14.6242630537985));
#66683=CARTESIAN_POINT('Ctrl Pts',(-53.7559643179139,-12.6688223002735,
14.5457575434217));
#66684=CARTESIAN_POINT('Ctrl Pts',(-52.0628591682458,-12.9760040856147,
14.4672520330449));
#66685=CARTESIAN_POINT('Ctrl Pts',(-51.3852128724656,-14.5577438020024,
14.3887465226681));
#66686=CARTESIAN_POINT('Ctrl Pts',(-52.3307362917628,-15.9953382094595,
14.3102410122914));
#66687=CARTESIAN_POINT('Ctrl Pts',(-54.0514987748276,-15.9998443309588,
14.2317355019146));
#66688=CARTESIAN_POINT('Ctrl Pts',(-55.0042044918326,-14.5665632650764,
14.1532299915378));
#66689=CARTESIAN_POINT('Ctrl Pts',(-54.3345957734336,-12.9822233909153,
14.074724481161));
#66690=CARTESIAN_POINT('Ctrl Pts',(-52.642890831849,-12.6650114501325,13.9962189707843));
#66691=CARTESIAN_POINT('Ctrl Pts',(-51.4468410434119,-13.9049130927216,
13.9177134604075));
#66692=CARTESIAN_POINT('Ctrl Pts',(-51.6948674713958,-15.0196330720529,
13.8653764534896));
#66693=CARTESIAN_POINT('Ctrl Pts',(-52.0259993620635,-15.404095589155,13.8392079500307));
#66694=CARTESIAN_POINT('Ctrl Pts',(-52.8205983740734,-12.996169774565,18.0535973499898));
#66695=CARTESIAN_POINT('Ctrl Pts',(-52.359900444268,-13.11933387906,18.0274288465308));
#66696=CARTESIAN_POINT('Ctrl Pts',(-51.5770224562855,-13.8535123278671,
17.975091839613));
#66697=CARTESIAN_POINT('Ctrl Pts',(-51.8491027615148,-15.449596585157,17.8965863292362));
#66698=CARTESIAN_POINT('Ctrl Pts',(-53.3306005753026,-16.0991388853812,
17.8180808188594));
#66699=CARTESIAN_POINT('Ctrl Pts',(-54.6895013936797,-15.2235740807106,
17.7395753084826));
#66700=CARTESIAN_POINT('Ctrl Pts',(-54.7087686260451,-13.6062036013328,
17.6610697981059));
#66701=CARTESIAN_POINT('Ctrl Pts',(-53.370302195588,-12.6984745354833,17.5825642877291));
#66702=CARTESIAN_POINT('Ctrl Pts',(-51.8748772355608,-13.3139889999824,
17.5040587773523));
#66703=CARTESIAN_POINT('Ctrl Pts',(-51.5634249338331,-14.9009722914672,
17.4255532669756));
#66704=CARTESIAN_POINT('Ctrl Pts',(-52.7153629422732,-16.0360644703525,
17.3470477565987));
#66705=CARTESIAN_POINT('Ctrl Pts',(-54.2975564085964,-15.7013451606169,
17.268542246222));
#66706=CARTESIAN_POINT('Ctrl Pts',(-54.8910811244797,-14.1969702179137,
17.1900367358452));
#66707=CARTESIAN_POINT('Ctrl Pts',(-53.9636378718331,-12.8721129164929,
17.1115312254684));
#66708=CARTESIAN_POINT('Ctrl Pts',(-52.3469858247822,-12.9149298139051,
17.0330257150916));
#66709=CARTESIAN_POINT('Ctrl Pts',(-51.4909739917866,-14.2870251506759,
16.9545202047148));
#66710=CARTESIAN_POINT('Ctrl Pts',(-52.1632956122412,-15.75786949867,16.8760146943381));
#66711=CARTESIAN_POINT('Ctrl Pts',(-53.7609959415414,-16.0083755267644,
16.7975091839613));
#66712=CARTESIAN_POINT('Ctrl Pts',(-54.8512197038372,-14.8138830536132,
16.7190036735845));
#66713=CARTESIAN_POINT('Ctrl Pts',(-54.4562281308453,-13.2456415346295,
16.6404981632077));
#66714=CARTESIAN_POINT('Ctrl Pts',(-52.9302591446351,-12.7100871437567,
16.561992652831));
#66715=CARTESIAN_POINT('Ctrl Pts',(-51.6418379657667,-13.6875178418857,
16.4834871424542));
#66716=CARTESIAN_POINT('Ctrl Pts',(-51.7464513597646,-15.3013505165395,
16.4049816320774));
#66717=CARTESIAN_POINT('Ctrl Pts',(-53.1502795370219,-16.1042616709564,
16.3264761217006));
#66718=CARTESIAN_POINT('Ctrl Pts',(-54.5943360194343,-15.3761814875148,
16.2479706113238));
#66719=CARTESIAN_POINT('Ctrl Pts',(-54.7835566204401,-13.7700695869338,
16.1694651009471));
#66720=CARTESIAN_POINT('Ctrl Pts',(-53.5482438079087,-12.7263253032243,
16.0909595905703));
#66721=CARTESIAN_POINT('Ctrl Pts',(-51.9962554793534,-13.1810033244324,
16.0124540801935));
#66722=CARTESIAN_POINT('Ctrl Pts',(-51.5194516645429,-14.7263375912924,
15.9339485698167));
#66723=CARTESIAN_POINT('Ctrl Pts',(-52.5454413598283,-15.9764355954941,
15.8554430594399));
#66724=CARTESIAN_POINT('Ctrl Pts',(-54.1540926149925,-15.8101797269071,
15.7769375490632));
#66725=CARTESIAN_POINT('Ctrl Pts',(-54.9027287409836,-14.376672202025,15.6984320386864));
#66726=CARTESIAN_POINT('Ctrl Pts',(-54.1199550619985,-12.9615166468276,
15.6199265283096));
#66727=CARTESIAN_POINT('Ctrl Pts',(-52.507781623182,-12.8338582106659,15.5414210179328));
#66728=CARTESIAN_POINT('Ctrl Pts',(-51.5120438907672,-14.1081840058335,
15.462915507556));
#66729=CARTESIAN_POINT('Ctrl Pts',(-52.0257431373717,-15.6416483803266,
15.3844099971793));
#66730=CARTESIAN_POINT('Ctrl Pts',(-53.5881816623453,-16.0590039938468,
15.3059044868025));
#66731=CARTESIAN_POINT('Ctrl Pts',(-54.7981274593024,-14.98595647718,15.2273989764257));
#66732=CARTESIAN_POINT('Ctrl Pts',(-54.5704723572559,-13.3848402181903,
15.1488934660489));
#66733=CARTESIAN_POINT('Ctrl Pts',(-53.1093828951161,-12.691574615422,15.0703879556721));
#66734=CARTESIAN_POINT('Ctrl Pts',(-51.7251987749648,-13.5278961916579,
14.9918824452954));
#66735=CARTESIAN_POINT('Ctrl Pts',(-51.659289349954,-15.143772987429,14.9133769349186));
#66736=CARTESIAN_POINT('Ctrl Pts',(-52.9707635028084,-16.0900460317101,
14.8348714245418));
#66737=CARTESIAN_POINT('Ctrl Pts',(-54.4834605524782,-15.5180796936027,
14.756365914165));
#66738=CARTESIAN_POINT('Ctrl Pts',(-54.8407567775752,-13.9408178370524,
14.6778604037883));
#66739=CARTESIAN_POINT('Ctrl Pts',(-53.7222225381219,-12.7728048506706,
14.5993548934115));
#66740=CARTESIAN_POINT('Ctrl Pts',(-52.1309816753803,-13.0615052950706,
14.5208493830347));
#66741=CARTESIAN_POINT('Ctrl Pts',(-51.4941054148939,-14.5480809347647,
14.4423438726579));
#66742=CARTESIAN_POINT('Ctrl Pts',(-52.3827421907963,-15.8991836501767,
14.3638383622811));
#66743=CARTESIAN_POINT('Ctrl Pts',(-53.9999764060854,-15.9034186645606,
14.2853328519044));
#66744=CARTESIAN_POINT('Ctrl Pts',(-54.8953633626269,-14.5563697820543,
14.2068273415276));
#66745=CARTESIAN_POINT('Ctrl Pts',(-54.2660411052506,-13.0673504209531,
14.1283218311508));
#66746=CARTESIAN_POINT('Ctrl Pts',(-52.676116208218,-12.7692232772124,14.049816320774));
#66747=CARTESIAN_POINT('Ctrl Pts',(-51.5520257773267,-13.934527251307,13.9713108103972));
#66748=CARTESIAN_POINT('Ctrl Pts',(-51.7851298980751,-14.9821810145562,
13.9189738034794));
#66749=CARTESIAN_POINT('Ctrl Pts',(-52.0963395092977,-15.3435126586808,
13.8928053000205));
#66750=CARTESIAN_POINT('Ctrl Pts',(-52.8445746335155,-13.0858534785527,
18.1071946999795));
#66751=CARTESIAN_POINT('Ctrl Pts',(-52.4133685721046,-13.2011331552573,
18.0810261965206));
#66752=CARTESIAN_POINT('Ctrl Pts',(-51.6806070120392,-13.8883127078473,
18.0286891896027));
#66753=CARTESIAN_POINT('Ctrl Pts',(-51.9352699250133,-15.3822226252554,
17.950183679226));
#66754=CARTESIAN_POINT('Ctrl Pts',(-53.3219287223341,-15.9901840656676,
17.8716781688492));
#66755=CARTESIAN_POINT('Ctrl Pts',(-54.5938386481889,-15.1706690939129,
17.7931726584724));
#66756=CARTESIAN_POINT('Ctrl Pts',(-54.6118724765287,-13.6568356053423,
17.7146671480956));
#66757=CARTESIAN_POINT('Ctrl Pts',(-53.3590888183695,-12.8072153878641,
17.6361616377188));
#66758=CARTESIAN_POINT('Ctrl Pts',(-51.9593944298553,-13.3833273059057,
17.5576561273421));
#66759=CARTESIAN_POINT('Ctrl Pts',(-51.6678799435583,-14.868718861572,17.4791506169653));
#66760=CARTESIAN_POINT('Ctrl Pts',(-52.7460759142211,-15.9311473990782,
17.4006451065885));
#66761=CARTESIAN_POINT('Ctrl Pts',(-54.2269842684028,-15.6178553569582,
17.3221395962117));
#66762=CARTESIAN_POINT('Ctrl Pts',(-54.7825141254484,-14.2097839245511,
17.243634085835));
#66763=CARTESIAN_POINT('Ctrl Pts',(-53.9144417372685,-12.9697381984539,
17.1651285754582));
#66764=CARTESIAN_POINT('Ctrl Pts',(-52.4012806901265,-13.009814145187,17.0866230650814));
#66765=CARTESIAN_POINT('Ctrl Pts',(-51.6000669942391,-14.2940739340229,
17.0081175547046));
#66766=CARTESIAN_POINT('Ctrl Pts',(-52.2293495223373,-15.6707612538786,
16.9296120443279));
#66767=CARTESIAN_POINT('Ctrl Pts',(-53.7247720578873,-15.9052309806687,
16.8511065339511));
#66768=CARTESIAN_POINT('Ctrl Pts',(-54.7452044587765,-14.7872046961792,
16.7726010235743));
#66769=CARTESIAN_POINT('Ctrl Pts',(-54.3754985203273,-13.3193551466328,
16.6940955131975));
#66770=CARTESIAN_POINT('Ctrl Pts',(-52.9472154007209,-12.8180846076984,
16.6155900028207));
#66771=CARTESIAN_POINT('Ctrl Pts',(-51.7412733158222,-13.7329444635267,
16.5370844924439));
#66772=CARTESIAN_POINT('Ctrl Pts',(-51.8391898174562,-15.2434666221729,
16.4585789820672));
#66773=CARTESIAN_POINT('Ctrl Pts',(-53.153151048991,-15.9949789128949,16.3800734716904));
#66774=CARTESIAN_POINT('Ctrl Pts',(-54.5047653453669,-15.3135072413688,
16.3015679613136));
#66775=CARTESIAN_POINT('Ctrl Pts',(-54.6818728703171,-13.8102116065761,
16.2230624509368));
#66776=CARTESIAN_POINT('Ctrl Pts',(-53.5256393862053,-12.8332832711514,
16.1445569405601));
#66777=CARTESIAN_POINT('Ctrl Pts',(-52.0730025688563,-13.2588547922085,
16.0660514301833));
#66778=CARTESIAN_POINT('Ctrl Pts',(-51.6267216508218,-14.7052635118164,
15.9875459198065));
#66779=CARTESIAN_POINT('Ctrl Pts',(-52.5870319689928,-15.8753357042332,
15.9090404094297));
#66780=CARTESIAN_POINT('Ctrl Pts',(-54.0927043999843,-15.7197228098794,
15.8305348990529));
#66781=CARTESIAN_POINT('Ctrl Pts',(-54.7934161124393,-14.3779821728676,
15.7520293886762));
#66782=CARTESIAN_POINT('Ctrl Pts',(-54.060752183965,-13.0534186926322,15.6735238782994));
#66783=CARTESIAN_POINT('Ctrl Pts',(-52.551783044128,-12.9339323917357,15.5950183679226));
#66784=CARTESIAN_POINT('Ctrl Pts',(-51.6197880903543,-14.1266814178069,
15.5165128575458));
#66785=CARTESIAN_POINT('Ctrl Pts',(-52.1006025558578,-15.5619801036903,
15.438007347169));
#66786=CARTESIAN_POINT('Ctrl Pts',(-53.5630205937139,-15.9526184345153,
15.3595018367923));
#66787=CARTESIAN_POINT('Ctrl Pts',(-54.6955109477442,-14.9482627310635,
15.2809963264155));
#66788=CARTESIAN_POINT('Ctrl Pts',(-54.4824293305661,-13.4496429387163,
15.2024908160387));
#66789=CARTESIAN_POINT('Ctrl Pts',(-53.1148724313975,-12.8007571705351,
15.1239853056619));
#66790=CARTESIAN_POINT('Ctrl Pts',(-51.8192977302698,-13.5835410938618,
15.0454797952851));
#66791=CARTESIAN_POINT('Ctrl Pts',(-51.7576075386495,-15.0959765179234,
14.9669742849084));
#66792=CARTESIAN_POINT('Ctrl Pts',(-52.9851268468723,-15.9816732967562,
14.8884687745316));
#66793=CARTESIAN_POINT('Ctrl Pts',(-54.4009876413224,-15.4463217443432,
14.8099632641548));
#66794=CARTESIAN_POINT('Ctrl Pts',(-54.7354113233349,-13.9700292998257,
14.731457753778));
#66795=CARTESIAN_POINT('Ctrl Pts',(-53.6884807583299,-12.8767874010678,
14.6529522434012));
#66796=CARTESIAN_POINT('Ctrl Pts',(-52.1991041825148,-13.1470065045264,
14.5744467330245));
#66797=CARTESIAN_POINT('Ctrl Pts',(-51.6029979573221,-14.5384180675271,
14.4959412226477));
#66798=CARTESIAN_POINT('Ctrl Pts',(-52.4347480898299,-15.803029090894,14.4174357122709));
#66799=CARTESIAN_POINT('Ctrl Pts',(-53.9484540373432,-15.8069929981624,
14.3389302018941));
#66800=CARTESIAN_POINT('Ctrl Pts',(-54.7865222334212,-14.5461762990323,
14.2604246915174));
#66801=CARTESIAN_POINT('Ctrl Pts',(-54.1974864370675,-13.1524774509909,
14.1819191811406));
#66802=CARTESIAN_POINT('Ctrl Pts',(-52.709341584587,-12.8734351042922,14.1034136707638));
#66803=CARTESIAN_POINT('Ctrl Pts',(-51.6572105112416,-13.9641414098923,
14.024908160387));
#66804=CARTESIAN_POINT('Ctrl Pts',(-51.8753923247544,-14.9447289570596,
13.9725711534692));
#66805=CARTESIAN_POINT('Ctrl Pts',(-52.166679656532,-15.2829297282066,13.9464026500102));
#66806=CARTESIAN_POINT('Ctrl Pts',(-52.8685508929575,-13.1755371825403,
18.1607920499693));
#66807=CARTESIAN_POINT('Ctrl Pts',(-52.4668366999413,-13.2829324314546,
18.1346235465104));
#66808=CARTESIAN_POINT('Ctrl Pts',(-51.7841915677929,-13.9231130878274,
18.0822865395925));
#66809=CARTESIAN_POINT('Ctrl Pts',(-52.0214370885118,-15.3148486653539,
18.0037810292158));
#66810=CARTESIAN_POINT('Ctrl Pts',(-53.3132568693655,-15.881229245954,17.925275518839));
#66811=CARTESIAN_POINT('Ctrl Pts',(-54.4981759026981,-15.1177641071153,
17.8467700084622));
#66812=CARTESIAN_POINT('Ctrl Pts',(-54.5149763270121,-13.7074676093518,
17.7682644980854));
#66813=CARTESIAN_POINT('Ctrl Pts',(-53.347875441151,-12.9159562402448,17.6897589877086));
#66814=CARTESIAN_POINT('Ctrl Pts',(-52.0439116241499,-13.4526656118291,
17.6112534773319));
#66815=CARTESIAN_POINT('Ctrl Pts',(-51.7723349532836,-14.8364654316768,
17.5327479669551));
#66816=CARTESIAN_POINT('Ctrl Pts',(-52.7767888861688,-15.826230327804,17.4542424565783));
#66817=CARTESIAN_POINT('Ctrl Pts',(-54.1564121282093,-15.5343655532995,
17.3757369462015));
#66818=CARTESIAN_POINT('Ctrl Pts',(-54.6739471264171,-14.2225976311884,
17.2972314358247));
#66819=CARTESIAN_POINT('Ctrl Pts',(-53.8652456027039,-13.0673634804149,
17.218725925448));
#66820=CARTESIAN_POINT('Ctrl Pts',(-52.4555755554708,-13.104698476469,17.1402204150712));
#66821=CARTESIAN_POINT('Ctrl Pts',(-51.7091599966916,-14.30112271737,17.0617149046944));
#66822=CARTESIAN_POINT('Ctrl Pts',(-52.2954034324334,-15.5836530090872,
16.9832093943176));
#66823=CARTESIAN_POINT('Ctrl Pts',(-53.6885481742331,-15.802086434573,16.9047038839408));
#66824=CARTESIAN_POINT('Ctrl Pts',(-54.6391892137158,-14.7605263387452,
16.8261983735641));
#66825=CARTESIAN_POINT('Ctrl Pts',(-54.2947689098094,-13.3930687586361,
16.7476928631873));
#66826=CARTESIAN_POINT('Ctrl Pts',(-52.9641716568067,-12.9260820716401,
16.6691873528105));
#66827=CARTESIAN_POINT('Ctrl Pts',(-51.8407086658775,-13.7783710851678,
16.5906818424337));
#66828=CARTESIAN_POINT('Ctrl Pts',(-51.931928275148,-15.1855827278064,16.5121763320569));
#66829=CARTESIAN_POINT('Ctrl Pts',(-53.15602256096,-15.8856961548333,16.4336708216802));
#66830=CARTESIAN_POINT('Ctrl Pts',(-54.4151946712995,-15.2508329952228,
16.3551653113034));
#66831=CARTESIAN_POINT('Ctrl Pts',(-54.5801891201939,-13.8503536262183,
16.2766598009266));
#66832=CARTESIAN_POINT('Ctrl Pts',(-53.5030349645019,-12.9402412390784,
16.1981542905498));
#66833=CARTESIAN_POINT('Ctrl Pts',(-52.1497496583592,-13.3367062599847,
16.119648780173));
#66834=CARTESIAN_POINT('Ctrl Pts',(-51.7339916371008,-14.6841894323404,
16.0411432697963));
#66835=CARTESIAN_POINT('Ctrl Pts',(-52.6286225781573,-15.7742358129723,
15.9626377594195));
#66836=CARTESIAN_POINT('Ctrl Pts',(-54.031316184976,-15.6292658928517,15.8841322490427));
#66837=CARTESIAN_POINT('Ctrl Pts',(-54.6841034838951,-14.3792921437102,
15.8056267386659));
#66838=CARTESIAN_POINT('Ctrl Pts',(-54.0015493059316,-13.1453207384369,
15.7271212282891));
#66839=CARTESIAN_POINT('Ctrl Pts',(-52.5957844650741,-13.0340065728055,
15.6486157179124));
#66840=CARTESIAN_POINT('Ctrl Pts',(-51.7275322899413,-14.1451788297802,
15.5701102075356));
#66841=CARTESIAN_POINT('Ctrl Pts',(-52.1754619743441,-15.482311827054,15.4916046971588));
#66842=CARTESIAN_POINT('Ctrl Pts',(-53.5378595250825,-15.8462328751838,
15.413099186782));
#66843=CARTESIAN_POINT('Ctrl Pts',(-54.5928944361861,-14.9105689849469,
15.3345936764052));
#66844=CARTESIAN_POINT('Ctrl Pts',(-54.3943863038764,-13.5144456592424,
15.2560881660285));
#66845=CARTESIAN_POINT('Ctrl Pts',(-53.120361967679,-12.9099397256483,15.1775826556517));
#66846=CARTESIAN_POINT('Ctrl Pts',(-51.9133966855747,-13.6391859960657,
15.0990771452749));
#66847=CARTESIAN_POINT('Ctrl Pts',(-51.8559257273451,-15.0481800484177,
15.0205716348981));
#66848=CARTESIAN_POINT('Ctrl Pts',(-52.9994901909362,-15.8733005618024,
14.9420661245214));
#66849=CARTESIAN_POINT('Ctrl Pts',(-54.3185147301667,-15.3745637950836,
14.8635606141446));
#66850=CARTESIAN_POINT('Ctrl Pts',(-54.6300658690945,-13.9992407625991,
14.7850551037678));
#66851=CARTESIAN_POINT('Ctrl Pts',(-53.654738978538,-12.980769951465,14.706549593391));
#66852=CARTESIAN_POINT('Ctrl Pts',(-52.2672266896493,-13.2325077139822,
14.6280440830142));
#66853=CARTESIAN_POINT('Ctrl Pts',(-51.7118904997504,-14.5287552002895,
14.5495385726375));
#66854=CARTESIAN_POINT('Ctrl Pts',(-52.4867539888634,-15.7068745316112,
14.4710330622607));
#66855=CARTESIAN_POINT('Ctrl Pts',(-53.8969316686011,-15.7105673317642,
14.3925275518839));
#66856=CARTESIAN_POINT('Ctrl Pts',(-54.6776811042154,-14.5359828160102,
14.3140220415071));
#66857=CARTESIAN_POINT('Ctrl Pts',(-54.1289317688846,-13.2376044810286,
14.2355165311303));
#66858=CARTESIAN_POINT('Ctrl Pts',(-52.742566960956,-12.9776469313721,14.1570110207535));
#66859=CARTESIAN_POINT('Ctrl Pts',(-51.7623952451564,-13.9937555684777,
14.0785055103768));
#66860=CARTESIAN_POINT('Ctrl Pts',(-51.9656547514336,-14.9072768995629,
14.0261685034589));
#66861=CARTESIAN_POINT('Ctrl Pts',(-52.2370198037663,-15.2223467977324,
14.));
#66862=CARTESIAN_POINT('Ctrl Pts',(-51.9314271328212,-14.3981451355535,
17.5565803263806));
#66863=CARTESIAN_POINT('Ctrl Pts',(-51.9304449349957,-14.5245552242527,
17.5486362065721));
#66864=CARTESIAN_POINT('Ctrl Pts',(-51.9479261083582,-14.6507002121319,
17.5406920867636));
#66865=CARTESIAN_POINT('Ctrl Pts',(-51.9850067205755,-14.7707929443901,
17.5327479669551));
#66866=CARTESIAN_POINT('Ctrl Pts',(-52.107152930912,-15.1663870637192,17.5065794634962));
#66867=CARTESIAN_POINT('Ctrl Pts',(-52.4419709085404,-15.4963086957616,
17.4804109600372));
#66868=CARTESIAN_POINT('Ctrl Pts',(-52.8393171043614,-15.6126253826987,
17.4542424565783));
#66869=CARTESIAN_POINT('Ctrl Pts',(-53.2366633001823,-15.7289420696358,
17.4280739531194));
#66870=CARTESIAN_POINT('Ctrl Pts',(-53.6965377141958,-15.6316538114677,
17.4019054496604));
#66871=CARTESIAN_POINT('Ctrl Pts',(-54.0127307542372,-15.3643816953651,
17.3757369462015));
#66872=CARTESIAN_POINT('Ctrl Pts',(-54.3289237942786,-15.0971095792625,
17.3495684427426));
#66873=CARTESIAN_POINT('Ctrl Pts',(-54.5014354603478,-14.6598536052254,
17.3233999392837));
#66874=CARTESIAN_POINT('Ctrl Pts',(-54.4529077060969,-14.248686593078,17.2972314358247));
#66875=CARTESIAN_POINT('Ctrl Pts',(-54.404379951846,-13.8375195809306,17.2710629323658));
#66876=CARTESIAN_POINT('Ctrl Pts',(-54.134812777275,-13.4524415306728,17.2448944289069));
#66877=CARTESIAN_POINT('Ctrl Pts',(-53.7650841821172,-13.2661250048862,
17.218725925448));
#66878=CARTESIAN_POINT('Ctrl Pts',(-53.3953555869595,-13.0798084790996,
17.192557421989));
#66879=CARTESIAN_POINT('Ctrl Pts',(-52.9254655712151,-13.0922534777843,
17.1663889185301));
#66880=CARTESIAN_POINT('Ctrl Pts',(-52.5661179702131,-13.2978800172768,
17.1402204150712));
#66881=CARTESIAN_POINT('Ctrl Pts',(-52.206770369211,-13.5035065567693,17.1140519116123));
#66882=CARTESIAN_POINT('Ctrl Pts',(-51.9579651829513,-13.9023146370697,
17.0878834081533));
#66883=CARTESIAN_POINT('Ctrl Pts',(-51.9312698291117,-14.3154737258394,
17.0617149046944));
#66884=CARTESIAN_POINT('Ctrl Pts',(-51.9295238448586,-14.3424960034753,
17.0600033785898));
#66885=CARTESIAN_POINT('Ctrl Pts',(-51.9287279775559,-14.3695796702728,
17.0582918524852));
#66886=CARTESIAN_POINT('Ctrl Pts',(-51.9288577112775,-14.3966710926088,
17.0565803263806));
#66887=CARTESIAN_POINT('Origin',(-53.1951359564886,-14.3971354987959,15.5));
#66888=CARTESIAN_POINT('Origin',(-39.0658530619283,38.8697713466882,14.));
#66889=CARTESIAN_POINT('Ctrl Pts',(-39.3014489339361,37.6274127691862,14.));
#66890=CARTESIAN_POINT('Ctrl Pts',(-39.2527755161194,37.6125702664367,14.));
#66891=CARTESIAN_POINT('Ctrl Pts',(-39.2032917181315,37.6009462766933,14.));
#66892=CARTESIAN_POINT('Ctrl Pts',(-39.1532758042656,37.5923965983611,14.));
#66893=CARTESIAN_POINT('Ctrl Pts',(-39.1195722840575,37.586635346908,14.));
#66894=CARTESIAN_POINT('Ctrl Pts',(-39.0856264423578,37.5822710037957,14.));
#66895=CARTESIAN_POINT('Ctrl Pts',(-39.051517529296,37.5792707431957,14.));
#66896=CARTESIAN_POINT('Ctrl Pts',(-39.0357879605352,37.5778871516012,14.));
#66897=CARTESIAN_POINT('Ctrl Pts',(-39.0200236600756,37.5767937802542,14.));
#66898=CARTESIAN_POINT('Ctrl Pts',(-39.0042321836355,37.575988057109,14.));
#66899=CARTESIAN_POINT('Ctrl Pts',(-38.9909279655358,37.5753092405024,14.));
#66900=CARTESIAN_POINT('Ctrl Pts',(-38.9776118489662,37.5748350538321,14.));
#66901=CARTESIAN_POINT('Ctrl Pts',(-38.9642957637935,37.5745634329249,14.));
#66902=CARTESIAN_POINT('Ctrl Pts',(-38.9105541147896,37.5734672131828,14.));
#66903=CARTESIAN_POINT('Ctrl Pts',(-38.8567779423543,37.5756644894692,14.));
#66904=CARTESIAN_POINT('Ctrl Pts',(-38.8032675464162,37.5810264819144,14.));
#66905=CARTESIAN_POINT('Ctrl Pts',(-38.7827897374805,37.5830784543374,14.));
#66906=CARTESIAN_POINT('Ctrl Pts',(-38.762350670683,37.5855944285744,14.));
#66907=CARTESIAN_POINT('Ctrl Pts',(-38.7419666934157,37.5885691376463,14.));
#66908=CARTESIAN_POINT('Ctrl Pts',(-38.7273323755994,37.5907047776834,14.));
#66909=CARTESIAN_POINT('Ctrl Pts',(-38.7127264477777,37.5930768844181,14.));
#66910=CARTESIAN_POINT('Ctrl Pts',(-38.6981549325269,37.5956838482079,14.));
#66911=CARTESIAN_POINT('Ctrl Pts',(-38.6868487316631,37.5977066204279,14.));
#66912=CARTESIAN_POINT('Ctrl Pts',(-38.6755628690101,37.5998709906011,14.));
#66913=CARTESIAN_POINT('Ctrl Pts',(-38.664315444558,37.6021728300089,14.));
#66914=CARTESIAN_POINT('Ctrl Pts',(-38.6087986249492,37.6135346136523,14.));
#66915=CARTESIAN_POINT('Ctrl Pts',(-38.5541290484473,37.628256437058,14.));
#66916=CARTESIAN_POINT('Ctrl Pts',(-38.5006370920885,37.6461917726554,14.));
#66917=CARTESIAN_POINT('Ctrl Pts',(-38.4479217177469,37.6638667278135,14.));
#66918=CARTESIAN_POINT('Ctrl Pts',(-38.3963488051394,37.6846628179155,14.));
#66919=CARTESIAN_POINT('Ctrl Pts',(-38.3462305042669,37.7084927624528,14.));
#66920=CARTESIAN_POINT('Ctrl Pts',(-38.3200575606107,37.7209373143401,14.));
#66921=CARTESIAN_POINT('Ctrl Pts',(-38.2942813570802,37.7342101081289,14.));
#66922=CARTESIAN_POINT('Ctrl Pts',(-38.2689475827414,37.7483042481762,14.));
#66923=CARTESIAN_POINT('Ctrl Pts',(-38.2553600453312,37.7558635108663,14.));
#66924=CARTESIAN_POINT('Ctrl Pts',(-38.2418997997272,37.7636591073689,14.));
#66925=CARTESIAN_POINT('Ctrl Pts',(-38.2285740912793,37.7716904150091,14.));
#66926=CARTESIAN_POINT('Ctrl Pts',(-38.219103371651,37.7773983489029,14.));
#66927=CARTESIAN_POINT('Ctrl Pts',(-38.2097006109437,37.7832253490862,14.));
#66928=CARTESIAN_POINT('Ctrl Pts',(-38.2003684638973,37.7891712855976,14.));
#66929=CARTESIAN_POINT('Ctrl Pts',(-38.1921418100671,37.7944128619607,14.));
#66930=CARTESIAN_POINT('Ctrl Pts',(-38.1839782830262,37.799741616435,14.));
#66931=CARTESIAN_POINT('Ctrl Pts',(-38.1758800166261,37.8051565176932,14.));
#66932=CARTESIAN_POINT('Ctrl Pts',(-38.135853400971,37.8319202916625,14.));
#66933=CARTESIAN_POINT('Ctrl Pts',(-38.097416293909,37.8607893617207,14.));
#66934=CARTESIAN_POINT('Ctrl Pts',(-38.0607602397062,37.8916978987796,14.));
#66935=CARTESIAN_POINT('Ctrl Pts',(-38.0190399864272,37.9268765895204,14.));
#66936=CARTESIAN_POINT('Ctrl Pts',(-37.979625387271,37.964696062052,14.));
#66937=CARTESIAN_POINT('Ctrl Pts',(-37.9425628056437,38.0048405338692,14.));
#66938=CARTESIAN_POINT('Ctrl Pts',(-37.9063354033603,38.0440803781036,14.));
#66939=CARTESIAN_POINT('Ctrl Pts',(-37.8723549080262,38.0855424637427,14.));
#66940=CARTESIAN_POINT('Ctrl Pts',(-37.8406905748295,38.1289693592978,14.));
#66941=CARTESIAN_POINT('Ctrl Pts',(-37.8329319648674,38.1396101121722,14.));
#66942=CARTESIAN_POINT('Ctrl Pts',(-37.8253125495357,38.1503689751519,14.));
#66943=CARTESIAN_POINT('Ctrl Pts',(-37.8178336250283,38.1612424270489,14.));
#66944=CARTESIAN_POINT('Ctrl Pts',(-37.8121884193235,38.1694498735365,14.));
#66945=CARTESIAN_POINT('Ctrl Pts',(-37.8066244559446,38.1777210085785,14.));
#66946=CARTESIAN_POINT('Ctrl Pts',(-37.8011483696233,38.1860445283887,14.));
#66947=CARTESIAN_POINT('Ctrl Pts',(-37.7694817125821,38.2341770872534,14.));
#66948=CARTESIAN_POINT('Ctrl Pts',(-37.7406908693863,38.2841447569653,14.));
#66949=CARTESIAN_POINT('Ctrl Pts',(-37.7148226289923,38.3355979876602,14.));
#66950=CARTESIAN_POINT('Ctrl Pts',(-37.6883997602119,38.3881544021,14.));
#66951=CARTESIAN_POINT('Ctrl Pts',(-37.6650255379363,38.4422615831827,14.));
#66952=CARTESIAN_POINT('Ctrl Pts',(-37.6447852836431,38.4975884922593,14.));
#66953=CARTESIAN_POINT('Ctrl Pts',(-37.6243676757452,38.553400198939,14.));
#66954=CARTESIAN_POINT('Ctrl Pts',(-37.6071385772626,38.6104541129774,14.));
#66955=CARTESIAN_POINT('Ctrl Pts',(-37.5932306356442,38.6684381301379,14.));
#66956=CARTESIAN_POINT('Ctrl Pts',(-37.5900811837444,38.681568604655,14.));
#66957=CARTESIAN_POINT('Ctrl Pts',(-37.5871015926692,38.6947505762665,14.));
#66958=CARTESIAN_POINT('Ctrl Pts',(-37.5842989888792,38.7079539605985,14.));
#66959=CARTESIAN_POINT('Ctrl Pts',(-37.5716672473803,38.7674635275195,14.));
#66960=CARTESIAN_POINT('Ctrl Pts',(-37.5626014399533,38.8275056873427,14.));
#66961=CARTESIAN_POINT('Ctrl Pts',(-37.5571792782293,38.887728107878,14.));
#66962=CARTESIAN_POINT('Ctrl Pts',(-37.5518047857275,38.9474210798117,14.));
#66963=CARTESIAN_POINT('Ctrl Pts',(-37.5500097107535,39.0072922465011,14.));
#66964=CARTESIAN_POINT('Ctrl Pts',(-37.5519146657201,39.0670207918841,14.));
#66965=CARTESIAN_POINT('Ctrl Pts',(-37.553310403515,39.1107831850598,14.));
#66966=CARTESIAN_POINT('Ctrl Pts',(-37.5566933253822,39.1544695447416,14.));
#66967=CARTESIAN_POINT('Ctrl Pts',(-37.5621285378972,39.1979562890069,14.));
#66968=CARTESIAN_POINT('Ctrl Pts',(-37.565149248657,39.2221247784534,14.));
#66969=CARTESIAN_POINT('Ctrl Pts',(-37.568804155379,39.2462316220403,14.));
#66970=CARTESIAN_POINT('Ctrl Pts',(-37.573079654256,39.2702614469549,14.));
#66971=CARTESIAN_POINT('Ctrl Pts',(-37.9741697098829,39.9602191716055,14.));
#66972=CARTESIAN_POINT('Ctrl Pts',(-38.020991576866,39.9994070905167,14.));
#66973=CARTESIAN_POINT('Ctrl Pts',(-38.0702141503049,40.0354948198823,14.));
#66974=CARTESIAN_POINT('Ctrl Pts',(-38.1214910131339,40.0684345608225,14.));
#66975=CARTESIAN_POINT('Ctrl Pts',(-38.1690376391659,40.0989780351629,14.));
#66976=CARTESIAN_POINT('Ctrl Pts',(-38.2183516107479,40.126814478516,14.));
#66977=CARTESIAN_POINT('Ctrl Pts',(-38.2691689745691,40.1518670892062,14.));
#66978=CARTESIAN_POINT('Ctrl Pts',(-38.2814354207102,40.1579143627485,14.));
#66979=CARTESIAN_POINT('Ctrl Pts',(-38.2937899475964,40.1637993356401,14.));
#66980=CARTESIAN_POINT('Ctrl Pts',(-38.3062147881308,40.1695145313534,14.));
#66981=CARTESIAN_POINT('Ctrl Pts',(-38.360894981368,40.1946664039371,14.));
#66982=CARTESIAN_POINT('Ctrl Pts',(-38.4170009391299,40.2165668550583,14.));
#66983=CARTESIAN_POINT('Ctrl Pts',(-38.4742056406521,40.2351397540719,14.));
#66984=CARTESIAN_POINT('Ctrl Pts',(-38.5095144290366,40.2466036118232,14.));
#66985=CARTESIAN_POINT('Ctrl Pts',(-38.5452420715441,40.2567987359784,14.));
#66986=CARTESIAN_POINT('Ctrl Pts',(-38.581311892576,40.2656972878261,14.));
#66987=CARTESIAN_POINT('Ctrl Pts',(-38.5936535300867,40.268742013254,14.));
#66988=CARTESIAN_POINT('Ctrl Pts',(-38.6060352195458,40.2716348784393,14.));
#66989=CARTESIAN_POINT('Ctrl Pts',(-38.6184538533342,40.2743745599732,14.));
#66990=CARTESIAN_POINT('Ctrl Pts',(-38.6300726272152,40.2769377839793,14.));
#66991=CARTESIAN_POINT('Ctrl Pts',(-38.6417163459698,40.2793652416505,14.));
#66992=CARTESIAN_POINT('Ctrl Pts',(-38.653376443336,40.2816552663571,14.));
#66993=CARTESIAN_POINT('Ctrl Pts',(-38.7110876100587,40.2929896483515,14.));
#66994=CARTESIAN_POINT('Ctrl Pts',(-38.7692463788907,40.3009718362435,14.));
#66995=CARTESIAN_POINT('Ctrl Pts',(-38.8275464691728,40.3055302032547,14.));
#66996=CARTESIAN_POINT('Ctrl Pts',(-38.8843585379937,40.3099722248553,14.));
#66997=CARTESIAN_POINT('Ctrl Pts',(-38.9413057825382,40.3111628333593,14.));
#66998=CARTESIAN_POINT('Ctrl Pts',(-38.9980976131321,40.3089871593392,14.));
#66999=CARTESIAN_POINT('Ctrl Pts',(-39.0288884006191,40.3078075756615,14.));
#67000=CARTESIAN_POINT('Ctrl Pts',(-39.0596332935447,40.3056376455648,14.));
#67001=CARTESIAN_POINT('Ctrl Pts',(-39.0902835743803,40.3024530490585,14.));
#67002=CARTESIAN_POINT('Ctrl Pts',(-39.1157839675052,40.2998035313171,14.));
#67003=CARTESIAN_POINT('Ctrl Pts',(-39.1412188503762,40.2964515981625,14.));
#67004=CARTESIAN_POINT('Ctrl Pts',(-39.1665588540094,40.2923809785531,14.));
#67005=CARTESIAN_POINT('Ctrl Pts',(-39.1773889643725,40.290641229015,14.));
#67006=CARTESIAN_POINT('Ctrl Pts',(-39.1882029800359,40.2887698277096,14.));
#67007=CARTESIAN_POINT('Ctrl Pts',(-39.1989810536353,40.2867689791238,14.));
#67008=CARTESIAN_POINT('Ctrl Pts',(-39.2488808959019,40.2775055399842,14.));
#67009=CARTESIAN_POINT('Ctrl Pts',(-39.2980978218176,40.2654572977421,14.));
#67010=CARTESIAN_POINT('Ctrl Pts',(-39.3464249159924,40.2505519130058,14.));
#67011=CARTESIAN_POINT('Ctrl Pts',(-39.4004290144133,40.2338955864037,14.));
#67012=CARTESIAN_POINT('Ctrl Pts',(-39.4533231062175,40.2136715650556,14.));
#67013=CARTESIAN_POINT('Ctrl Pts',(-39.5048609693609,40.1901258318545,14.));
#67014=CARTESIAN_POINT('Ctrl Pts',(-39.5485960623501,40.1701448941857,14.));
#67015=CARTESIAN_POINT('Ctrl Pts',(-39.5913543500841,40.1477707447887,14.));
#67016=CARTESIAN_POINT('Ctrl Pts',(-39.6329645160367,40.1231328973135,14.));
#67017=CARTESIAN_POINT('Ctrl Pts',(-39.6444045721025,40.1163591113887,14.));
#67018=CARTESIAN_POINT('Ctrl Pts',(-39.6557577122726,40.1094141266032,14.));
#67019=CARTESIAN_POINT('Ctrl Pts',(-39.6670200627789,40.1023004514057,14.));
#67020=CARTESIAN_POINT('Ctrl Pts',(-39.6757877124543,40.0967625122337,14.));
#67021=CARTESIAN_POINT('Ctrl Pts',(-39.6845017797711,40.0911212766444,14.));
#67022=CARTESIAN_POINT('Ctrl Pts',(-39.6931464328254,40.0853874573571,14.));
#67023=CARTESIAN_POINT('Ctrl Pts',(-39.7394049739142,40.0547051253501,14.));
#67024=CARTESIAN_POINT('Ctrl Pts',(-39.7837665094979,40.0213210070101,14.));
#67025=CARTESIAN_POINT('Ctrl Pts',(-39.826005821329,39.9854744939875,14.));
#67026=CARTESIAN_POINT('Ctrl Pts',(-39.8680089351073,39.9498284311192,14.));
#67027=CARTESIAN_POINT('Ctrl Pts',(-39.9079141963595,39.9117464669987,14.));
#67028=CARTESIAN_POINT('Ctrl Pts',(-39.9454594213913,39.8714333538664,14.));
#67029=CARTESIAN_POINT('Ctrl Pts',(-39.9802942732095,39.8340304265673,14.));
#67030=CARTESIAN_POINT('Ctrl Pts',(-40.0130975716519,39.7947059892265,14.));
#67031=CARTESIAN_POINT('Ctrl Pts',(-40.0436204335325,39.7536104031384,14.));
#67032=CARTESIAN_POINT('Ctrl Pts',(-40.0514607527816,39.743054298802,14.));
#67033=CARTESIAN_POINT('Ctrl Pts',(-40.0591528687932,39.7323774869168,14.));
#67034=CARTESIAN_POINT('Ctrl Pts',(-40.0666759532432,39.7216063497443,14.));
#67035=CARTESIAN_POINT('Ctrl Pts',(-40.0970859623649,39.6780669767858,14.));
#67036=CARTESIAN_POINT('Ctrl Pts',(-40.1247894554028,39.6329220142279,14.));
#67037=CARTESIAN_POINT('Ctrl Pts',(-40.1495562730805,39.586364052585,14.));
#67038=CARTESIAN_POINT('Ctrl Pts',(-40.1734835191867,39.5413843615755,14.));
#67039=CARTESIAN_POINT('Ctrl Pts',(-40.1946700927978,39.4950850229851,14.));
#67040=CARTESIAN_POINT('Ctrl Pts',(-40.2128622007042,39.4476279811834,14.));
#67041=CARTESIAN_POINT('Ctrl Pts',(-40.2255879517226,39.4144308112267,14.));
#67042=CARTESIAN_POINT('Ctrl Pts',(-40.23684748228,39.3806668978,14.));
#67043=CARTESIAN_POINT('Ctrl Pts',(-40.2465386396389,39.3463911596944,14.));
#67044=CARTESIAN_POINT('Ctrl Pts',(-40.2520057165832,39.327055172195,14.));
#67045=CARTESIAN_POINT('Ctrl Pts',(-40.2569733939395,39.3075562909784,14.));
#67046=CARTESIAN_POINT('Ctrl Pts',(-40.261442519219,39.2879130030575,14.));
#67047=CARTESIAN_POINT('Origin',(-39.0658530619283,38.8697713466882,19.1042117235887));
#67048=CARTESIAN_POINT('Ctrl Pts',(-38.2940537528419,37.5314721085808,17.8542117235887));
#67049=CARTESIAN_POINT('Ctrl Pts',(-38.3354082297679,37.5072482534305,17.8517311518799));
#67050=CARTESIAN_POINT('Ctrl Pts',(-38.8263155408625,37.2510699656701,17.8230820767121));
#67051=CARTESIAN_POINT('Ctrl Pts',(-40.0256568276714,37.3267811177079,17.7682644980854));
#67052=CARTESIAN_POINT('Ctrl Pts',(-40.8821443104935,38.819261537444,17.6897589877086));
#67053=CARTESIAN_POINT('Ctrl Pts',(-40.1099071502118,40.3569109628884,17.6112534773319));
#67054=CARTESIAN_POINT('Ctrl Pts',(-38.4012543668155,40.5609220251471,17.5327479669551));
#67055=CARTESIAN_POINT('Ctrl Pts',(-37.2886704652103,39.2482374965454,17.4542424565783));
#67056=CARTESIAN_POINT('Ctrl Pts',(-37.6534618751483,37.995852754822,17.3947303754562));
#67057=CARTESIAN_POINT('Ctrl Pts',(-38.1723477780673,37.603235418619,17.361386797793));
#67058=CARTESIAN_POINT('Ctrl Pts',(-38.2935040424574,37.5346322273253,17.3542117235887));
#67059=CARTESIAN_POINT('Ctrl Pts',(-38.2938718037177,37.5356881270255,17.8957882764113));
#67060=CARTESIAN_POINT('Ctrl Pts',(-38.5911486295276,37.3667504425096,17.8781885106897));
#67061=CARTESIAN_POINT('Ctrl Pts',(-39.4708982524073,37.1808200198997,17.8344202415091));
#67062=CARTESIAN_POINT('Ctrl Pts',(-40.7062722211717,38.0891100356719,17.7644834688697));
#67063=CARTESIAN_POINT('Ctrl Pts',(-40.6223994863181,39.8071108514352,17.6859779584929));
#67064=CARTESIAN_POINT('Ctrl Pts',(-39.1423049297703,40.6853144575311,17.6074724481161));
#67065=CARTESIAN_POINT('Ctrl Pts',(-37.5937815296791,39.9348860603428,17.5289669377393));
#67066=CARTESIAN_POINT('Ctrl Pts',(-37.388492650827,38.4020168817229,17.4584055471711));
#67067=CARTESIAN_POINT('Ctrl Pts',(-37.9908199438395,37.7130239262801,17.4140126600617));
#67068=CARTESIAN_POINT('Ctrl Pts',(-38.2959007276492,37.5337106753505,17.3957882764113));
#67069=CARTESIAN_POINT('Ctrl Pts',(-40.2595650866584,39.2869186252538,18.));
#67070=CARTESIAN_POINT('Ctrl Pts',(-40.1223890770422,39.6794626033579,17.9738314965411));
#67071=CARTESIAN_POINT('Ctrl Pts',(-39.4328412785483,40.3122408191566,17.9214944896232));
#67072=CARTESIAN_POINT('Ctrl Pts',(-38.0628399617007,39.9714590750955,17.8429889792464));
#67073=CARTESIAN_POINT('Ctrl Pts',(-37.594757239893,38.6408443652931,17.7644834688697));
#67074=CARTESIAN_POINT('Ctrl Pts',(-38.4448300096771,37.516422065853,17.6859779584929));
#67075=CARTESIAN_POINT('Ctrl Pts',(-39.8524194013854,37.6052793541117,17.6074724481161));
#67076=CARTESIAN_POINT('Ctrl Pts',(-40.5543172769709,38.8283781815623,17.5289669377393));
#67077=CARTESIAN_POINT('Ctrl Pts',(-39.9214631686259,40.088493345836,17.4504614273626));
#67078=CARTESIAN_POINT('Ctrl Pts',(-38.5212094780202,40.2556819318544,17.3719559169858));
#67079=CARTESIAN_POINT('Ctrl Pts',(-37.6094386785518,39.1799271772095,17.293450406609));
#67080=CARTESIAN_POINT('Ctrl Pts',(-38.0037983665504,37.8260300114723,17.2149448962322));
#67081=CARTESIAN_POINT('Ctrl Pts',(-39.350642117465,37.4081786211339,17.1364393858554));
#67082=CARTESIAN_POINT('Ctrl Pts',(-40.4420762478649,38.3011214248006,17.0579338754786));
#67083=CARTESIAN_POINT('Ctrl Pts',(-40.2992826919135,39.7040414735315,16.9794283651019));
#67084=CARTESIAN_POINT('Ctrl Pts',(-39.0503191421165,40.358768990196,16.9009228547251));
#67085=CARTESIAN_POINT('Ctrl Pts',(-37.8152872634063,39.678127650814,16.8224173443483));
#67086=CARTESIAN_POINT('Ctrl Pts',(-37.7017922854029,38.2725333429822,16.7439118339715));
#67087=CARTESIAN_POINT('Ctrl Pts',(-38.8116195577816,37.4025561853298,16.6654063235948));
#67088=CARTESIAN_POINT('Ctrl Pts',(-40.1494494228947,37.8484125098358,16.586900813218));
#67089=CARTESIAN_POINT('Ctrl Pts',(-40.5154843389836,39.2102476987511,16.5083953028412));
#67090=CARTESIAN_POINT('Ctrl Pts',(-39.5814554487361,40.2667356115709,16.4298897924644));
#67091=CARTESIAN_POINT('Ctrl Pts',(-38.1850220871887,40.0703927553964,16.3513842820876));
#67092=CARTESIAN_POINT('Ctrl Pts',(-37.578538880925,38.7973040793768,16.2728787717109));
#67093=CARTESIAN_POINT('Ctrl Pts',(-38.305914392745,37.5892057701993,16.1943732613341));
#67094=CARTESIAN_POINT('Ctrl Pts',(-39.7148209687578,37.5295491143576,16.1158677509573));
#67095=CARTESIAN_POINT('Ctrl Pts',(-40.5417176980217,38.6718356181182,16.0373622405805));
#67096=CARTESIAN_POINT('Ctrl Pts',(-40.0450239347318,39.9916355890619,15.9588567302037));
#67097=CARTESIAN_POINT('Ctrl Pts',(-38.670186454417,40.3053210365854,15.880351219827));
#67098=CARTESIAN_POINT('Ctrl Pts',(-37.6501921939814,39.3315713939809,15.8018457094502));
#67099=CARTESIAN_POINT('Ctrl Pts',(-37.8997962556048,37.9436684903302,15.7233401990734));
#67100=CARTESIAN_POINT('Ctrl Pts',(-39.1951477820351,37.3863166449999,15.6448346886966));
#67101=CARTESIAN_POINT('Ctrl Pts',(-40.3745447306992,38.1593622434704,15.5663291783198));
#67102=CARTESIAN_POINT('Ctrl Pts',(-40.380275876363,39.5695196142836,15.4878236679431));
#67103=CARTESIAN_POINT('Ctrl Pts',(-39.2072013976484,40.3521261040355,15.4093181575663));
#67104=CARTESIAN_POINT('Ctrl Pts',(-37.9073623625386,39.8053216046427,15.3308126471895));
#67105=CARTESIAN_POINT('Ctrl Pts',(-37.646485345535,38.4194933961106,15.2523071368127));
#67106=CARTESIAN_POINT('Ctrl Pts',(-38.6585310049343,37.4374851510426,15.1738016264359));
#67107=CARTESIAN_POINT('Ctrl Pts',(-40.0358728399513,37.7399852318106,15.0952961160592));
#67108=CARTESIAN_POINT('Ctrl Pts',(-40.5432777323755,39.0557043292571,15.0167906056824));
#67109=CARTESIAN_POINT('Ctrl Pts',(-39.7256933501734,40.2046743690254,14.9382850953056));
#67110=CARTESIAN_POINT('Ctrl Pts',(-38.3163479152336,40.156471518347,14.8597795849288));
#67111=CARTESIAN_POINT('Ctrl Pts',(-37.5791777219181,38.954325616703,14.781274074552));
#67112=CARTESIAN_POINT('Ctrl Pts',(-38.1752908680605,37.6763489234029,14.7027685641753));
#67113=CARTESIAN_POINT('Ctrl Pts',(-39.5700863286924,37.468662869981,14.6242630537985));
#67114=CARTESIAN_POINT('Ctrl Pts',(-40.5126633343826,38.5175221013622,14.5457575434217));
#67115=CARTESIAN_POINT('Ctrl Pts',(-40.1577269226072,39.8822911025123,14.4672520330449));
#67116=CARTESIAN_POINT('Ctrl Pts',(-38.8235306389231,40.3389996506624,14.3887465226681));
#67117=CARTESIAN_POINT('Ctrl Pts',(-37.7067389013687,39.4780868997918,14.3102410122914));
#67118=CARTESIAN_POINT('Ctrl Pts',(-37.8086626184681,38.0715866597082,14.2317355019146));
#67119=CARTESIAN_POINT('Ctrl Pts',(-39.0384102949244,37.3809896965113,14.1532299915378));
#67120=CARTESIAN_POINT('Ctrl Pts',(-40.292067953697,38.0254209930878,14.074724481161));
#67121=CARTESIAN_POINT('Ctrl Pts',(-40.4474545117342,39.4273810345935,13.9962189707842));
#67122=CARTESIAN_POINT('Ctrl Pts',(-39.3608457503204,40.3286674512605,13.9177134604075));
#67123=CARTESIAN_POINT('Ctrl Pts',(-38.4650745289098,40.0575985380861,13.8653764534896));
#67124=CARTESIAN_POINT('Ctrl Pts',(-38.1712104185962,39.7634014663304,13.8392079500307));
#67125=CARTESIAN_POINT('Ctrl Pts',(-40.3472015171019,39.3175435144276,18.0535973499898));
#67126=CARTESIAN_POINT('Ctrl Pts',(-40.1999547235979,39.7389061291211,18.0274288465308));
#67127=CARTESIAN_POINT('Ctrl Pts',(-39.4597837375779,40.4181397905767,17.975091839613));
#67128=CARTESIAN_POINT('Ctrl Pts',(-37.9892037027278,40.0523395370335,17.8965863292362));
#67129=CARTESIAN_POINT('Ctrl Pts',(-37.486756663529,38.6240376790354,17.8180808188594));
#67130=CARTESIAN_POINT('Ctrl Pts',(-38.399237569964,37.4170658579415,17.7395753084826));
#67131=CARTESIAN_POINT('Ctrl Pts',(-39.9101652101474,37.5124466086439,17.6610697981059));
#67132=CARTESIAN_POINT('Ctrl Pts',(-40.6635929548118,38.8253393001895,17.5825642877291));
#67133=CARTESIAN_POINT('Ctrl Pts',(-39.9842778291546,40.1779658848535,17.5040587773523));
#67134=CARTESIAN_POINT('Ctrl Pts',(-38.481224440952,40.3574286296185,17.4255532669755));
#67135=CARTESIAN_POINT('Ctrl Pts',(-37.5025159407713,39.2026972836548,17.3470477565987));
#67136=CARTESIAN_POINT('Ctrl Pts',(-37.9258275657958,37.7494036870074,17.268542246222));
#67137=CARTESIAN_POINT('Ctrl Pts',(-39.3715499208041,37.3008757150928,17.1900367358452));
#67138=CARTESIAN_POINT('Ctrl Pts',(-40.5431117447104,38.2593739611798,17.1115312254684));
#67139=CARTESIAN_POINT('Ctrl Pts',(-40.3898349924146,39.7652894583281,17.0330257150916));
#67140=CARTESIAN_POINT('Ctrl Pts',(-39.0491787185848,40.4680838297154,16.9545202047148));
#67141=CARTESIAN_POINT('Ctrl Pts',(-37.7234769101999,39.7374731709667,16.8760146943381));
#67142=CARTESIAN_POINT('Ctrl Pts',(-37.6016496924775,38.2286870838463,16.7975091839613));
#67143=CARTESIAN_POINT('Ctrl Pts',(-38.7929549918386,37.2948405078714,16.7190036735845));
#67144=CARTESIAN_POINT('Ctrl Pts',(-40.22900170615,37.7734293976535,16.6404981632077));
#67145=CARTESIAN_POINT('Ctrl Pts',(-40.6219090946604,39.2352437878639,16.561992652831));
#67146=CARTESIAN_POINT('Ctrl Pts',(-39.6193084248073,40.369293815807,16.4834871424542));
#67147=CARTESIAN_POINT('Ctrl Pts',(-38.1203558353197,40.1585364386243,16.4049816320774));
#67148=CARTESIAN_POINT('Ctrl Pts',(-37.469347632893,38.7919838911743,16.3264761217006));
#67149=CARTESIAN_POINT('Ctrl Pts',(-38.2501234557824,37.4951929817316,16.2479706113238));
#67150=CARTESIAN_POINT('Ctrl Pts',(-39.7624649814247,37.4311566293954,16.1694651009471));
#67151=CARTESIAN_POINT('Ctrl Pts',(-40.6500683771181,38.6573041563001,16.0909595905703));
#67152=CARTESIAN_POINT('Ctrl Pts',(-40.116909815337,40.0739973108231,16.0124540801935));
#67153=CARTESIAN_POINT('Ctrl Pts',(-38.6411385698271,40.4107119918078,15.9339485698167));
#67154=CARTESIAN_POINT('Ctrl Pts',(-37.5462613776579,39.3654744684955,15.85544305944));
#67155=CARTESIAN_POINT('Ctrl Pts',(-37.8141901344604,37.8756786009152,15.7769375490632));
#67156=CARTESIAN_POINT('Ctrl Pts',(-39.2046399606432,37.2774087408428,15.6984320386864));
#67157=CARTESIAN_POINT('Ctrl Pts',(-40.4706223976961,38.1072075221719,15.6199265283096));
#67158=CARTESIAN_POINT('Ctrl Pts',(-40.4767742957171,39.6208916697799,15.5414210179328));
#67159=CARTESIAN_POINT('Ctrl Pts',(-39.2175784930743,40.4609532557217,15.462915507556));
#67160=CARTESIAN_POINT('Ctrl Pts',(-37.8223117075287,39.8740050755377,15.3844099971793));
#67161=CARTESIAN_POINT('Ctrl Pts',(-37.5422823907398,38.3864362169262,15.3059044868025));
#67162=CARTESIAN_POINT('Ctrl Pts',(-38.6286274349138,37.3323337854205,15.2273989764257));
#67163=CARTESIAN_POINT('Ctrl Pts',(-40.1070868924567,37.6570419253671,15.1488934660489));
#67164=CARTESIAN_POINT('Ctrl Pts',(-40.6517429414752,39.0693546088525,15.0703879556721));
#67165=CARTESIAN_POINT('Ctrl Pts',(-39.774135559288,40.302676343909,14.9918824452954));
#67166=CARTESIAN_POINT('Ctrl Pts',(-38.2613229558677,40.2509346784385,14.9133769349186));
#67167=CARTESIAN_POINT('Ctrl Pts',(-37.4700333744309,38.9605331728382,14.8348714245418));
#67168=CARTESIAN_POINT('Ctrl Pts',(-38.1099101982326,37.5887337540646,14.756365914165));
#67169=CARTESIAN_POINT('Ctrl Pts',(-39.6071046402237,37.3658004182179,14.6778604037883));
#67170=CARTESIAN_POINT('Ctrl Pts',(-40.6188809858598,38.4916617046775,14.5993548934115));
#67171=CARTESIAN_POINT('Ctrl Pts',(-40.2378868989348,39.9566252931006,14.5208493830347));
#67172=CARTESIAN_POINT('Ctrl Pts',(-38.8057405256223,40.4468631230907,14.4423438726579));
#67173=CARTESIAN_POINT('Ctrl Pts',(-37.6069594645119,39.5227464177934,14.3638383622811));
#67174=CARTESIAN_POINT('Ctrl Pts',(-37.7163659166087,38.0129878893579,14.2853328519043));
#67175=CARTESIAN_POINT('Ctrl Pts',(-39.036395582756,37.2716907141535,14.2068273415276));
#67176=CARTESIAN_POINT('Ctrl Pts',(-40.3820905838163,37.963432967919,14.1283218311508));
#67177=CARTESIAN_POINT('Ctrl Pts',(-40.5488848541016,39.4683179788618,14.049816320774));
#67178=CARTESIAN_POINT('Ctrl Pts',(-39.3825026538969,40.4357723847318,13.9713108103972));
#67179=CARTESIAN_POINT('Ctrl Pts',(-38.4209683416301,40.1448029331841,13.9189738034794));
#67180=CARTESIAN_POINT('Ctrl Pts',(-38.1055301823584,39.8290073680888,13.8928053000205));
#67181=CARTESIAN_POINT('Ctrl Pts',(-40.4348379475454,39.3481684036013,18.1071946999795));
#67182=CARTESIAN_POINT('Ctrl Pts',(-40.2775203701537,39.7983496548842,18.0810261965206));
#67183=CARTESIAN_POINT('Ctrl Pts',(-39.4867261966074,40.5240387619969,18.0286891896027));
#67184=CARTESIAN_POINT('Ctrl Pts',(-37.9155674437551,40.1332199989714,17.950183679226));
#67185=CARTESIAN_POINT('Ctrl Pts',(-37.3787560871649,38.6072309927777,17.8716781688492));
#67186=CARTESIAN_POINT('Ctrl Pts',(-38.3536451302508,37.3177096500299,17.7931726584724));
#67187=CARTESIAN_POINT('Ctrl Pts',(-39.9679110189094,37.4196138631759,17.7146671480956));
#67188=CARTESIAN_POINT('Ctrl Pts',(-40.7728686326527,38.8223004188168,17.6361616377188));
#67189=CARTESIAN_POINT('Ctrl Pts',(-40.0470924896831,40.2674384238709,17.5576561273421));
#67190=CARTESIAN_POINT('Ctrl Pts',(-38.4412394038838,40.4591753273829,17.4791506169653));
#67191=CARTESIAN_POINT('Ctrl Pts',(-37.3955932029908,39.2254673901001,17.4006451065885));
#67192=CARTESIAN_POINT('Ctrl Pts',(-37.8478567650412,37.6727773625425,17.3221395962117));
#67193=CARTESIAN_POINT('Ctrl Pts',(-39.3924577241432,37.1935728090517,17.243634085835));
#67194=CARTESIAN_POINT('Ctrl Pts',(-40.6441472415558,38.2176264975589,17.1651285754582));
#67195=CARTESIAN_POINT('Ctrl Pts',(-40.4803872929157,39.8265374431247,17.0866230650814));
#67196=CARTESIAN_POINT('Ctrl Pts',(-39.0480382950531,40.5773986692348,17.0081175547046));
#67197=CARTESIAN_POINT('Ctrl Pts',(-37.6316665569936,39.7968186911193,16.9296120443279));
#67198=CARTESIAN_POINT('Ctrl Pts',(-37.5015070995522,38.1848408247104,16.8511065339511));
#67199=CARTESIAN_POINT('Ctrl Pts',(-38.7742904258956,37.187124830413,16.7726010235743));
#67200=CARTESIAN_POINT('Ctrl Pts',(-40.3085539894054,37.6984462854713,16.6940955131975));
#67201=CARTESIAN_POINT('Ctrl Pts',(-40.7283338503372,39.2602398769767,16.6155900028207));
#67202=CARTESIAN_POINT('Ctrl Pts',(-39.6571614008785,40.4718520200432,16.5370844924439));
#67203=CARTESIAN_POINT('Ctrl Pts',(-38.0556895834507,40.2466801218523,16.4585789820672));
#67204=CARTESIAN_POINT('Ctrl Pts',(-37.360156384861,38.7866637029717,16.3800734716904));
#67205=CARTESIAN_POINT('Ctrl Pts',(-38.1943325188198,37.4011801932639,16.3015679613136));
#67206=CARTESIAN_POINT('Ctrl Pts',(-39.8101089940917,37.3327641444332,16.2230624509368));
#67207=CARTESIAN_POINT('Ctrl Pts',(-40.7584190562144,38.6427726944821,16.1445569405601));
#67208=CARTESIAN_POINT('Ctrl Pts',(-40.1887956959422,40.1563590325842,16.0660514301833));
#67209=CARTESIAN_POINT('Ctrl Pts',(-38.6120906852372,40.5161029470303,15.9875459198065));
#67210=CARTESIAN_POINT('Ctrl Pts',(-37.4423305613345,39.39937754301,15.9090404094297));
#67211=CARTESIAN_POINT('Ctrl Pts',(-37.7285840133161,37.8076887115003,15.8305348990529));
#67212=CARTESIAN_POINT('Ctrl Pts',(-39.2141321392513,37.1685008366855,15.7520293886762));
#67213=CARTESIAN_POINT('Ctrl Pts',(-40.566700064693,38.0550528008733,15.6735238782994));
#67214=CARTESIAN_POINT('Ctrl Pts',(-40.5732727150713,39.6722637252762,15.5950183679226));
#67215=CARTESIAN_POINT('Ctrl Pts',(-39.2279555885002,40.5697804074078,15.5165128575458));
#67216=CARTESIAN_POINT('Ctrl Pts',(-37.7372610525188,39.9426885464327,15.438007347169));
#67217=CARTESIAN_POINT('Ctrl Pts',(-37.4380794359446,38.3533790377419,15.3595018367923));
#67218=CARTESIAN_POINT('Ctrl Pts',(-38.5987238648932,37.2271824197985,15.2809963264155));
#67219=CARTESIAN_POINT('Ctrl Pts',(-40.1783009449622,37.5740986189236,15.2024908160387));
#67220=CARTESIAN_POINT('Ctrl Pts',(-40.7602081505748,39.083004888448,15.1239853056619));
#67221=CARTESIAN_POINT('Ctrl Pts',(-39.8225777684026,40.4006783187926,15.0454797952851));
#67222=CARTESIAN_POINT('Ctrl Pts',(-38.2062979965018,40.3453978385299,14.9669742849084));
#67223=CARTESIAN_POINT('Ctrl Pts',(-37.3608890269436,38.9667407289735,14.8884687745316));
#67224=CARTESIAN_POINT('Ctrl Pts',(-38.0445295284047,37.5011185847262,14.8099632641548));
#67225=CARTESIAN_POINT('Ctrl Pts',(-39.6441229517549,37.262937966455,14.731457753778));
#67226=CARTESIAN_POINT('Ctrl Pts',(-40.725098637337,38.4658013079928,14.6529522434012));
#67227=CARTESIAN_POINT('Ctrl Pts',(-40.3180468752625,40.030959483689,14.5744467330245));
#67228=CARTESIAN_POINT('Ctrl Pts',(-38.7879504123214,40.5547265955191,14.4959412226477));
#67229=CARTESIAN_POINT('Ctrl Pts',(-37.5071800276552,39.5674059357951,14.4174357122709));
#67230=CARTESIAN_POINT('Ctrl Pts',(-37.6240692147494,37.9543891190076,14.3389302018941));
#67231=CARTESIAN_POINT('Ctrl Pts',(-39.0343808705876,37.1623917317957,14.2604246915173));
#67232=CARTESIAN_POINT('Ctrl Pts',(-40.4721132139356,37.9014449427502,14.1819191811406));
#67233=CARTESIAN_POINT('Ctrl Pts',(-40.6503151964691,39.50925492313,14.1034136707638));
#67234=CARTESIAN_POINT('Ctrl Pts',(-39.4041595574733,40.5428773182031,14.024908160387));
#67235=CARTESIAN_POINT('Ctrl Pts',(-38.3768621543504,40.2320073282821,13.9725711534692));
#67236=CARTESIAN_POINT('Ctrl Pts',(-38.0398499461206,39.8946132698472,13.9464026500102));
#67237=CARTESIAN_POINT('Ctrl Pts',(-40.5224743779889,39.378793292775,18.1607920499693));
#67238=CARTESIAN_POINT('Ctrl Pts',(-40.3550860167094,39.8577931806474,18.1346235465104));
#67239=CARTESIAN_POINT('Ctrl Pts',(-39.513668655637,40.6299377334171,18.0822865395925));
#67240=CARTESIAN_POINT('Ctrl Pts',(-37.8419311847822,40.2141004609093,18.0037810292157));
#67241=CARTESIAN_POINT('Ctrl Pts',(-37.270755510801,38.59042430652,17.925275518839));
#67242=CARTESIAN_POINT('Ctrl Pts',(-38.3080526905376,37.2183534421183,17.8467700084622));
#67243=CARTESIAN_POINT('Ctrl Pts',(-40.0256568276714,37.3267811177079,17.7682644980854));
#67244=CARTESIAN_POINT('Ctrl Pts',(-40.8821443104935,38.819261537444,17.6897589877086));
#67245=CARTESIAN_POINT('Ctrl Pts',(-40.1099071502118,40.3569109628884,17.6112534773319));
#67246=CARTESIAN_POINT('Ctrl Pts',(-38.4012543668155,40.5609220251471,17.5327479669551));
#67247=CARTESIAN_POINT('Ctrl Pts',(-37.2886704652103,39.2482374965454,17.4542424565783));
#67248=CARTESIAN_POINT('Ctrl Pts',(-37.7698859642865,37.5961510380776,17.3757369462015));
#67249=CARTESIAN_POINT('Ctrl Pts',(-39.4133655274823,37.0862699030106,17.2972314358247));
#67250=CARTESIAN_POINT('Ctrl Pts',(-40.7451827384013,38.1758790339381,17.218725925448));
#67251=CARTESIAN_POINT('Ctrl Pts',(-40.5709395934168,39.8877854279213,17.1402204150712));
#67252=CARTESIAN_POINT('Ctrl Pts',(-39.0468978715213,40.6867135087542,17.0617149046944));
#67253=CARTESIAN_POINT('Ctrl Pts',(-37.5398562037872,39.8561642112719,16.9832093943176));
#67254=CARTESIAN_POINT('Ctrl Pts',(-37.4013645066268,38.1409945655744,16.9047038839409));
#67255=CARTESIAN_POINT('Ctrl Pts',(-38.7556258599526,37.0794091529546,16.826198373564));
#67256=CARTESIAN_POINT('Ctrl Pts',(-40.3881062726607,37.6234631732891,16.7476928631873));
#67257=CARTESIAN_POINT('Ctrl Pts',(-40.834758606014,39.2852359660895,16.6691873528105));
#67258=CARTESIAN_POINT('Ctrl Pts',(-39.6950143769496,40.5744102242793,16.5906818424337));
#67259=CARTESIAN_POINT('Ctrl Pts',(-37.9910233315818,40.3348238050802,16.5121763320569));
#67260=CARTESIAN_POINT('Ctrl Pts',(-37.250965136829,38.7813435147693,16.4336708216802));
#67261=CARTESIAN_POINT('Ctrl Pts',(-38.1385415818572,37.3071674047962,16.3551653113034));
#67262=CARTESIAN_POINT('Ctrl Pts',(-39.8577530067586,37.234371659471,16.2766598009266));
#67263=CARTESIAN_POINT('Ctrl Pts',(-40.8667697353107,38.628241232664,16.1981542905498));
#67264=CARTESIAN_POINT('Ctrl Pts',(-40.2606815765474,40.2387207543455,16.119648780173));
#67265=CARTESIAN_POINT('Ctrl Pts',(-38.5830428006473,40.6214939022527,16.0411432697963));
#67266=CARTESIAN_POINT('Ctrl Pts',(-37.3383997450109,39.4332806175246,15.9626377594195));
#67267=CARTESIAN_POINT('Ctrl Pts',(-37.6429778921718,37.7396988220852,15.8841322490427));
#67268=CARTESIAN_POINT('Ctrl Pts',(-39.2236243178593,37.0595929325284,15.8056267386659));
#67269=CARTESIAN_POINT('Ctrl Pts',(-40.6627777316899,38.0028980795747,15.7271212282892));
#67270=CARTESIAN_POINT('Ctrl Pts',(-40.6697711344255,39.7236357807725,15.6486157179124));
#67271=CARTESIAN_POINT('Ctrl Pts',(-39.2383326839261,40.6786075590939,15.5701102075356));
#67272=CARTESIAN_POINT('Ctrl Pts',(-37.6522103975089,40.0113720173278,15.4916046971588));
#67273=CARTESIAN_POINT('Ctrl Pts',(-37.3338764811494,38.3203218585575,15.413099186782));
#67274=CARTESIAN_POINT('Ctrl Pts',(-38.5688202948727,37.1220310541764,15.3345936764052));
#67275=CARTESIAN_POINT('Ctrl Pts',(-40.2495149974676,37.4911553124801,15.2560881660285));
#67276=CARTESIAN_POINT('Ctrl Pts',(-40.8686733596744,39.0966551680435,15.1775826556517));
#67277=CARTESIAN_POINT('Ctrl Pts',(-39.8710199775172,40.4986802936762,15.0990771452749));
#67278=CARTESIAN_POINT('Ctrl Pts',(-38.151273037136,40.4398609986214,15.0205716348981));
#67279=CARTESIAN_POINT('Ctrl Pts',(-37.2517446794564,38.9729482851087,14.9420661245214));
#67280=CARTESIAN_POINT('Ctrl Pts',(-37.9791488585767,37.413503415388,14.8635606141446));
#67281=CARTESIAN_POINT('Ctrl Pts',(-39.6811412632862,37.1600755146919,14.7850551037678));
#67282=CARTESIAN_POINT('Ctrl Pts',(-40.8313162888141,38.4399409113082,14.706549593391));
#67283=CARTESIAN_POINT('Ctrl Pts',(-40.3982068515902,40.1052936742774,14.6280440830142));
#67284=CARTESIAN_POINT('Ctrl Pts',(-38.7701602990205,40.6625900679474,14.5495385726375));
#67285=CARTESIAN_POINT('Ctrl Pts',(-37.4074005907986,39.6120654537968,14.4710330622607));
#67286=CARTESIAN_POINT('Ctrl Pts',(-37.5317725128899,37.8957903486572,14.3925275518839));
#67287=CARTESIAN_POINT('Ctrl Pts',(-39.0323661584193,37.0530927494379,14.3140220415071));
#67288=CARTESIAN_POINT('Ctrl Pts',(-40.5621358440549,37.8394569175814,14.2355165311304));
#67289=CARTESIAN_POINT('Ctrl Pts',(-40.7517455388365,39.5501918673983,14.1570110207535));
#67290=CARTESIAN_POINT('Ctrl Pts',(-39.4258164610498,40.6499822516744,14.0785055103768));
#67291=CARTESIAN_POINT('Ctrl Pts',(-38.3327559670706,40.3192117233802,14.0261685034589));
#67292=CARTESIAN_POINT('Ctrl Pts',(-37.9741697098829,39.9602191716055,14.));
#67293=CARTESIAN_POINT('Ctrl Pts',(-38.4329072841441,37.7756148875603,17.1934196736194));
#67294=CARTESIAN_POINT('Ctrl Pts',(-38.3336188224971,37.831835714126,17.2005947478237));
#67295=CARTESIAN_POINT('Ctrl Pts',(-38.2421150540945,37.9010724492168,17.2077698220279));
#67296=CARTESIAN_POINT('Ctrl Pts',(-38.1625457103698,37.9820376407054,17.2149448962322));
#67297=CARTESIAN_POINT('Ctrl Pts',(-37.8723451372176,38.277329066718,17.2411133996911));
#67298=CARTESIAN_POINT('Ctrl Pts',(-37.7408919078847,38.7286281219637,17.2672819031501));
#67299=CARTESIAN_POINT('Ctrl Pts',(-37.8271270931297,39.1335701086941,17.293450406609));
#67300=CARTESIAN_POINT('Ctrl Pts',(-37.9133622783746,39.5385120954244,17.3196189100679));
#67301=CARTESIAN_POINT('Ctrl Pts',(-38.2172858781974,39.8970970136394,17.3457874135268));
#67302=CARTESIAN_POINT('Ctrl Pts',(-38.6026232932098,40.0485247084105,17.3719559169858));
#67303=CARTESIAN_POINT('Ctrl Pts',(-38.9879607082221,40.1999524031816,17.3981244204447));
#67304=CARTESIAN_POINT('Ctrl Pts',(-39.454711938424,40.1442228745088,17.4242929239036));
#67305=CARTESIAN_POINT('Ctrl Pts',(-39.7935632382492,39.9063389161268,17.4504614273625));
#67306=CARTESIAN_POINT('Ctrl Pts',(-40.1324145380743,39.6684549577448,17.4766299308215));
#67307=CARTESIAN_POINT('Ctrl Pts',(-40.3433659075226,39.2484165696535,17.5027984342804));
#67308=CARTESIAN_POINT('Ctrl Pts',(-40.3318586129825,38.8345475710328,17.5289669377393));
#67309=CARTESIAN_POINT('Ctrl Pts',(-40.3203513184424,38.4206785724121,17.5551354411982));
#67310=CARTESIAN_POINT('Ctrl Pts',(-40.0863853599139,38.0129789632619,17.5813039446572));
#67311=CARTESIAN_POINT('Ctrl Pts',(-39.7348041486982,37.7943196106437,17.6074724481161));
#67312=CARTESIAN_POINT('Ctrl Pts',(-39.3832229374826,37.5756602580255,17.633640951575));
#67313=CARTESIAN_POINT('Ctrl Pts',(-38.9140264735798,37.5460411619393,17.659809455034));
#67314=CARTESIAN_POINT('Ctrl Pts',(-38.5377494466644,37.7186353304695,17.6859779584929));
#67315=CARTESIAN_POINT('Ctrl Pts',(-38.5020812950974,37.7349959225928,17.6884585302017));
#67316=CARTESIAN_POINT('Ctrl Pts',(-38.4672480779576,37.7531735168604,17.6909391019106));
#67317=CARTESIAN_POINT('Ctrl Pts',(-38.4333577759012,37.7730251466967,17.6934196736194));
#67318=CARTESIAN_POINT('Ctrl Pts',(-37.5756558680257,39.2699729499893,18.));
#67319=CARTESIAN_POINT('Ctrl Pts',(-37.4440523270134,38.7799318659294,17.9738314965411));
#67320=CARTESIAN_POINT('Ctrl Pts',(-37.7041245449082,37.6679293649188,17.9214944896232));
#67321=CARTESIAN_POINT('Ctrl Pts',(-39.3195387437205,37.0695352316425,17.8429889792464));
#67322=CARTESIAN_POINT('Ctrl Pts',(-40.7062722211717,38.0891100356719,17.7644834688697));
#67323=CARTESIAN_POINT('Ctrl Pts',(-40.6223994863181,39.8071108514352,17.6859779584929));
#67324=CARTESIAN_POINT('Ctrl Pts',(-39.1423049297703,40.6853144575311,17.6074724481161));
#67325=CARTESIAN_POINT('Ctrl Pts',(-37.5937815296791,39.9348860603428,17.5289669377393));
#67326=CARTESIAN_POINT('Ctrl Pts',(-37.3653803023341,38.2294395514344,17.4504614273626));
#67327=CARTESIAN_POINT('Ctrl Pts',(-38.6620363043874,37.0981581562677,17.3719559169858));
#67328=CARTESIAN_POINT('Ctrl Pts',(-40.3208285827552,37.5557507395872,17.293450406609));
#67329=CARTESIAN_POINT('Ctrl Pts',(-40.8541369642561,39.1917640019411,17.2149448962322));
#67330=CARTESIAN_POINT('Ctrl Pts',(-39.7836658898432,40.5390185509755,17.1364393858554));
#67331=CARTESIAN_POINT('Ctrl Pts',(-38.0694451486085,40.389246627264,17.0579338754786));
#67332=CARTESIAN_POINT('Ctrl Pts',(-37.248825754395,38.87677605618,16.9794283651019));
#67333=CARTESIAN_POINT('Ctrl Pts',(-38.0577601193366,37.3580220610822,16.9009228547251));
#67334=CARTESIAN_POINT('Ctrl Pts',(-39.7707759682515,37.1950414723212,16.8224173443483));
#67335=CARTESIAN_POINT('Ctrl Pts',(-40.8516003110939,38.5339981005298,16.7439118339715));
#67336=CARTESIAN_POINT('Ctrl Pts',(-40.3309240105073,40.1740843304588,16.6654063235948));
#67337=CARTESIAN_POINT('Ctrl Pts',(-38.6757020358417,40.644431583443,16.586900813218));
#67338=CARTESIAN_POINT('Ctrl Pts',(-37.3703767628973,39.5232213878114,16.5083953028412));
#67339=CARTESIAN_POINT('Ctrl Pts',(-37.5855949493635,37.8159816397814,16.4298897924644));
#67340=CARTESIAN_POINT('Ctrl Pts',(-39.1283437989466,37.053805563498,16.3513842820876));
#67341=CARTESIAN_POINT('Ctrl Pts',(-40.6150494715949,37.9202307686755,16.2728787717109));
#67342=CARTESIAN_POINT('Ctrl Pts',(-40.7123989731982,39.6382265407265,16.1943732613341));
#67343=CARTESIAN_POINT('Ctrl Pts',(-39.333086957597,40.6670534245635,16.1158677509573));
#67344=CARTESIAN_POINT('Ctrl Pts',(-37.7141132310224,40.0840350136354,16.0373622405805));
#67345=CARTESIAN_POINT('Ctrl Pts',(-37.3074119207117,38.4120360784117,15.9588567302037));
#67346=CARTESIAN_POINT('Ctrl Pts',(-38.4777224302706,37.150545013987,15.8803512198269));
#67347=CARTESIAN_POINT('Ctrl Pts',(-40.1754824724718,37.4308969968639,15.8018457094502));
#67348=CARTESIAN_POINT('Ctrl Pts',(-40.8781004790679,39.0016657040982,15.7233401990734));
#67349=CARTESIAN_POINT('Ctrl Pts',(-39.9554519188483,40.454148415738,15.6448346886966));
#67350=CARTESIAN_POINT('Ctrl Pts',(-38.2349899535507,40.4857241059463,15.5663291783198));
#67351=CARTESIAN_POINT('Ctrl Pts',(-37.2596657788943,39.0680749435715,15.4878236679431));
#67352=CARTESIAN_POINT('Ctrl Pts',(-37.9041732944261,37.4725824031402,15.4093181575663));
#67353=CARTESIAN_POINT('Ctrl Pts',(-39.5905028527061,37.1301221194426,15.3308126471895));
#67354=CARTESIAN_POINT('Ctrl Pts',(-40.8063139857151,38.3478206288557,15.2523071368127));
#67355=CARTESIAN_POINT('Ctrl Pts',(-40.4612384258706,40.0336169338117,15.1738016264359));
#67356=CARTESIAN_POINT('Ctrl Pts',(-38.8647480157521,40.6756488816116,15.0952961160592));
#67357=CARTESIAN_POINT('Ctrl Pts',(-37.4486135593306,39.6981268544225,15.0167906056824));
#67358=CARTESIAN_POINT('Ctrl Pts',(-37.4828575973041,37.9777160555697,14.9382850953056));
#67359=CARTESIAN_POINT('Ctrl Pts',(-38.9367702893064,37.0573213639055,14.8597795849288));
#67360=CARTESIAN_POINT('Ctrl Pts',(-40.5064460859517,37.7623754838001,14.781274074552));
#67361=CARTESIAN_POINT('Ctrl Pts',(-40.7841666383236,39.4605673674226,14.7027685641753));
#67362=CARTESIAN_POINT('Ctrl Pts',(-39.5208569909583,40.6289217126118,14.6242630537985));
#67363=CARTESIAN_POINT('Ctrl Pts',(-37.8495006293028,40.2196233657655,14.5457575434217));
#67364=CARTESIAN_POINT('Ctrl Pts',(-37.2689744719433,38.5997554156835,14.4672520330449));
#67365=CARTESIAN_POINT('Ctrl Pts',(-38.2999795535027,37.2220243444981,14.3887465226681));
#67366=CARTESIAN_POINT('Ctrl Pts',(-40.0177412802272,37.3220721610693,14.3102410122914));
#67367=CARTESIAN_POINT('Ctrl Pts',(-40.8820235552812,38.8100518816852,14.2317355019146));
#67368=CARTESIAN_POINT('Ctrl Pts',(-40.1171224362185,40.3517547545305,14.1532299915378));
#67369=CARTESIAN_POINT('Ctrl Pts',(-38.4102262410485,40.5640442208951,14.074724481161));
#67370=CARTESIAN_POINT('Ctrl Pts',(-37.2896688855126,39.2575551350437,13.9962189707843));
#67371=CARTESIAN_POINT('Ctrl Pts',(-37.7654127933167,37.6018660619833,13.9177134604075));
#67372=CARTESIAN_POINT('Ctrl Pts',(-38.8548175316167,37.2592519394721,13.8653764534896));
#67373=CARTESIAN_POINT('Ctrl Pts',(-39.3533377835638,37.3537893102425,13.8392079500307));
#67374=CARTESIAN_POINT('Ctrl Pts',(-37.6653123637055,39.2458951477601,18.0535973499898));
#67375=CARTESIAN_POINT('Ctrl Pts',(-37.5416266421298,38.7853369848301,18.0274288465308));
#67376=CARTESIAN_POINT('Ctrl Pts',(-37.7860518276885,37.7402372050404,17.975091839613));
#67377=CARTESIAN_POINT('Ctrl Pts',(-39.304275952107,37.1778449655031,17.8965863292362));
#67378=CARTESIAN_POINT('Ctrl Pts',(-40.6075777437793,38.1360778851249,17.8180808188594));
#67379=CARTESIAN_POINT('Ctrl Pts',(-40.528751143438,39.7507165865677,17.7395753084826));
#67380=CARTESIAN_POINT('Ctrl Pts',(-39.1377052656541,40.5760837907846,17.6610697981059));
#67381=CARTESIAN_POINT('Ctrl Pts',(-37.6823475097464,39.8708043045094,17.5825642877291));
#67382=CARTESIAN_POINT('Ctrl Pts',(-37.4676878554875,38.267964590315,17.5040587773523));
#67383=CARTESIAN_POINT('Ctrl Pts',(-38.6863316094155,37.2047458152723,17.4255532669755));
#67384=CARTESIAN_POINT('Ctrl Pts',(-40.2453240067019,37.6348077149766,17.3470477565987));
#67385=CARTESIAN_POINT('Ctrl Pts',(-40.7465463255009,39.1723915771219,17.268542246222));
#67386=CARTESIAN_POINT('Ctrl Pts',(-39.7404792679866,40.4385896578249,17.1900367358452));
#67387=CARTESIAN_POINT('Ctrl Pts',(-38.1293932159794,40.2978286394393,17.1115312254684));
#67388=CARTESIAN_POINT('Ctrl Pts',(-37.3581457166218,38.876354623561,17.0330257150916));
#67389=CARTESIAN_POINT('Ctrl Pts',(-38.1184112069391,37.4489752207368,16.9545202047149));
#67390=CARTESIAN_POINT('Ctrl Pts',(-39.7283648579877,37.2958002258341,16.8760146943381));
#67391=CARTESIAN_POINT('Ctrl Pts',(-40.7441622880019,38.5541996233327,16.7975091839613));
#67392=CARTESIAN_POINT('Ctrl Pts',(-40.2548120512981,40.0956114062894,16.7190036735845));
#67393=CARTESIAN_POINT('Ctrl Pts',(-38.6991751533109,40.5376606013872,16.6404981632077));
#67394=CARTESIAN_POINT('Ctrl Pts',(-37.4723837080864,39.4839071003945,16.561992652831));
#67395=CARTESIAN_POINT('Ctrl Pts',(-37.6746534683415,37.8793820358439,16.4834871424542));
#67396=CARTESIAN_POINT('Ctrl Pts',(-39.1245840948508,37.1630616599808,16.4049816320774));
#67397=CARTESIAN_POINT('Ctrl Pts',(-40.5218433363406,37.9773591011396,16.3264761217006));
#67398=CARTESIAN_POINT('Ctrl Pts',(-40.6133358847799,39.5919930623209,16.2479706113239));
#67399=CARTESIAN_POINT('Ctrl Pts',(-39.3170090487735,40.5589214179339,16.1694651009471));
#67400=CARTESIAN_POINT('Ctrl Pts',(-37.7954395526702,40.010979832982,16.0909595905703));
#67401=CARTESIAN_POINT('Ctrl Pts',(-37.4132070941463,38.4395753465506,16.0124540801935));
#67402=CARTESIAN_POINT('Ctrl Pts',(-38.5131068288268,37.2539808605321,15.9339485698167));
#67403=CARTESIAN_POINT('Ctrl Pts',(-40.1087225262985,37.517465695595,15.85544305944));
#67404=CARTESIAN_POINT('Ctrl Pts',(-40.7690680950382,38.9937303879309,15.7769375490632));
#67405=CARTESIAN_POINT('Ctrl Pts',(-39.9019299310211,40.3588256648781,15.6984320386864));
#67406=CARTESIAN_POINT('Ctrl Pts',(-38.2849781530935,40.3885016295036,15.6199265283096));
#67407=CARTESIAN_POINT('Ctrl Pts',(-37.3683335599107,39.0561441698122,15.5414210179328));
#67408=CARTESIAN_POINT('Ctrl Pts',(-37.9740648077658,37.5566431334877,15.4629155075561));
#67409=CARTESIAN_POINT('Ctrl Pts',(-39.558937727035,37.2347866927387,15.3844099971793));
#67410=CARTESIAN_POINT('Ctrl Pts',(-40.7016005773603,38.37922336701,15.3059044868025));
#67411=CARTESIAN_POINT('Ctrl Pts',(-40.3772862064154,39.9635951157055,15.2273989764257));
#67412=CARTESIAN_POINT('Ctrl Pts',(-38.8768473364175,40.5669997363369,15.1488934660489));
#67413=CARTESIAN_POINT('Ctrl Pts',(-37.5459134516342,39.6482895226222,15.0703879556721));
#67414=CARTESIAN_POINT('Ctrl Pts',(-37.5780972250634,38.0313858327519,14.9918824452954));
#67415=CARTESIAN_POINT('Ctrl Pts',(-38.9445364487739,37.1663659351315,14.9133769349186));
#67416=CARTESIAN_POINT('Ctrl Pts',(-40.4197739845928,37.829001050405,14.8348714245418));
#67417=CARTESIAN_POINT('Ctrl Pts',(-40.6807857070153,39.425022607912,14.756365914165));
#67418=CARTESIAN_POINT('Ctrl Pts',(-39.4934820516118,40.5230838692526,14.6778604037883));
#67419=CARTESIAN_POINT('Ctrl Pts',(-37.9226814788354,40.1384106227729,14.5993548934115));
#67420=CARTESIAN_POINT('Ctrl Pts',(-37.3770822030539,38.6160007033882,14.5208493830347));
#67421=CARTESIAN_POINT('Ctrl Pts',(-38.3460577069044,37.3211596955696,14.4423438726579));
#67422=CARTESIAN_POINT('Ctrl Pts',(-39.9604717039049,37.415188217063,14.3638383622811));
#67423=CARTESIAN_POINT('Ctrl Pts',(-40.7727551425788,38.8136448544662,14.2853328519044));
#67424=CARTESIAN_POINT('Ctrl Pts',(-40.0538736739071,40.2625924345728,14.2068273415276));
#67425=CARTESIAN_POINT('Ctrl Pts',(-38.4496714926395,40.4621096787766,14.1283218311508));
#67426=CARTESIAN_POINT('Ctrl Pts',(-37.396531554152,39.2342244404969,14.049816320774));
#67427=CARTESIAN_POINT('Ctrl Pts',(-37.8436527187452,37.678148546708,13.9713108103972));
#67428=CARTESIAN_POINT('Ctrl Pts',(-38.8675143117402,37.356147522732,13.9189738034794));
#67429=CARTESIAN_POINT('Ctrl Pts',(-39.3360415003546,37.4449971298904,13.8928053000205));
#67430=CARTESIAN_POINT('Ctrl Pts',(-37.7549688593853,39.2218173455308,18.1071946999795));
#67431=CARTESIAN_POINT('Ctrl Pts',(-37.6392009572462,38.7907421037308,18.0810261965206));
#67432=CARTESIAN_POINT('Ctrl Pts',(-37.8679791104688,37.812545045162,18.0286891896028));
#67433=CARTESIAN_POINT('Ctrl Pts',(-39.2890131604935,37.2861546993635,17.950183679226));
#67434=CARTESIAN_POINT('Ctrl Pts',(-40.5088832663869,38.1830457345779,17.8716781688492));
#67435=CARTESIAN_POINT('Ctrl Pts',(-40.4351028005577,39.6943223217001,17.7931726584724));
#67436=CARTESIAN_POINT('Ctrl Pts',(-39.1331056015378,40.4668531240381,17.7146671480957));
#67437=CARTESIAN_POINT('Ctrl Pts',(-37.7709134898136,39.806722548676,17.6361616377188));
#67438=CARTESIAN_POINT('Ctrl Pts',(-37.5699954086408,38.3064896291956,17.5576561273421));
#67439=CARTESIAN_POINT('Ctrl Pts',(-38.7106269144436,37.3113334742769,17.4791506169653));
#67440=CARTESIAN_POINT('Ctrl Pts',(-40.1698194306487,37.713864690366,17.4006451065885));
#67441=CARTESIAN_POINT('Ctrl Pts',(-40.6389556867456,39.1530191523028,17.3221395962117));
#67442=CARTESIAN_POINT('Ctrl Pts',(-39.6972926461299,40.3381607646743,17.243634085835));
#67443=CARTESIAN_POINT('Ctrl Pts',(-38.1893412833502,40.2064106516146,17.1651285754582));
#67444=CARTESIAN_POINT('Ctrl Pts',(-37.4674656788486,38.8759331909419,17.0866230650814));
#67445=CARTESIAN_POINT('Ctrl Pts',(-38.1790622945415,37.5399283803915,17.0081175547046));
#67446=CARTESIAN_POINT('Ctrl Pts',(-39.6859537477239,37.396558979347,16.9296120443278));
#67447=CARTESIAN_POINT('Ctrl Pts',(-40.63672426491,38.5744011461357,16.8511065339511));
#67448=CARTESIAN_POINT('Ctrl Pts',(-40.1787000920889,40.01713848212,16.7726010235743));
#67449=CARTESIAN_POINT('Ctrl Pts',(-38.7226482707802,40.4308896193314,16.6940955131975));
#67450=CARTESIAN_POINT('Ctrl Pts',(-37.5743906532754,39.4445928129776,16.6155900028207));
#67451=CARTESIAN_POINT('Ctrl Pts',(-37.7637119873195,37.9427824319065,16.537084492444));
#67452=CARTESIAN_POINT('Ctrl Pts',(-39.120824390755,37.2723177564635,16.4585789820672));
#67453=CARTESIAN_POINT('Ctrl Pts',(-40.4286372010863,38.0344874336038,16.3800734716904));
#67454=CARTESIAN_POINT('Ctrl Pts',(-40.5142727963614,39.5457595839153,16.3015679613136));
#67455=CARTESIAN_POINT('Ctrl Pts',(-39.3009311399501,40.4507894113043,16.2230624509368));
#67456=CARTESIAN_POINT('Ctrl Pts',(-37.8767658743179,39.9379246523285,16.14455694056));
#67457=CARTESIAN_POINT('Ctrl Pts',(-37.5190022675809,38.4671146146895,16.0660514301833));
#67458=CARTESIAN_POINT('Ctrl Pts',(-38.5484912273831,37.3574167070772,15.9875459198065));
#67459=CARTESIAN_POINT('Ctrl Pts',(-40.0419625801251,37.604034394326,15.9090404094297));
#67460=CARTESIAN_POINT('Ctrl Pts',(-40.6600357110086,38.9857950717635,15.8305348990529));
#67461=CARTESIAN_POINT('Ctrl Pts',(-39.8484079431939,40.2635029140183,15.7520293886762));
#67462=CARTESIAN_POINT('Ctrl Pts',(-38.3349663526362,40.2912791530608,15.6735238782994));
#67463=CARTESIAN_POINT('Ctrl Pts',(-37.4770013409272,39.0442133960529,15.5950183679226));
#67464=CARTESIAN_POINT('Ctrl Pts',(-38.0439563211054,37.640703863835,15.5165128575458));
#67465=CARTESIAN_POINT('Ctrl Pts',(-39.5273726013639,37.3394512660349,15.438007347169));
#67466=CARTESIAN_POINT('Ctrl Pts',(-40.5968871690055,38.4106261051643,15.3595018367923));
#67467=CARTESIAN_POINT('Ctrl Pts',(-40.2933339869602,39.8935732975992,15.2809963264155));
#67468=CARTESIAN_POINT('Ctrl Pts',(-38.8889466570829,40.4583505910623,15.2024908160387));
#67469=CARTESIAN_POINT('Ctrl Pts',(-37.6432133439378,39.5984521908218,15.1239853056619));
#67470=CARTESIAN_POINT('Ctrl Pts',(-37.6733368528227,38.0850556099341,15.0454797952851));
#67471=CARTESIAN_POINT('Ctrl Pts',(-38.9523026082414,37.2754105063574,14.9669742849084));
#67472=CARTESIAN_POINT('Ctrl Pts',(-40.3331018832339,37.89562661701,14.8884687745316));
#67473=CARTESIAN_POINT('Ctrl Pts',(-40.577404775707,39.3894778484014,14.8099632641548));
#67474=CARTESIAN_POINT('Ctrl Pts',(-39.4661071122653,40.4172460258934,14.731457753778));
#67475=CARTESIAN_POINT('Ctrl Pts',(-37.995862328368,40.0571978797802,14.6529522434012));
#67476=CARTESIAN_POINT('Ctrl Pts',(-37.4851899341645,38.6322459910928,14.5744467330245));
#67477=CARTESIAN_POINT('Ctrl Pts',(-38.3921358603061,37.4202950466411,14.4959412226477));
#67478=CARTESIAN_POINT('Ctrl Pts',(-39.9032021275825,37.5083042730567,14.4174357122709));
#67479=CARTESIAN_POINT('Ctrl Pts',(-40.6634867298766,38.8172378272473,14.3389302018941));
#67480=CARTESIAN_POINT('Ctrl Pts',(-39.9906249115956,40.1734301146151,14.2604246915173));
#67481=CARTESIAN_POINT('Ctrl Pts',(-38.4891167442306,40.3601751366581,14.1819191811406));
#67482=CARTESIAN_POINT('Ctrl Pts',(-37.5033942227913,39.2108937459501,14.1034136707638));
#67483=CARTESIAN_POINT('Ctrl Pts',(-37.9218926441736,37.7544310314326,14.024908160387));
#67484=CARTESIAN_POINT('Ctrl Pts',(-38.8802110918637,37.4530431059918,13.9725711534692));
#67485=CARTESIAN_POINT('Ctrl Pts',(-39.3187452171454,37.5362049495383,13.9464026500102));
#67486=CARTESIAN_POINT('Ctrl Pts',(-37.8446253550651,39.1977395433015,18.1607920499693));
#67487=CARTESIAN_POINT('Ctrl Pts',(-37.7367752723626,38.7961472226315,18.1346235465104));
#67488=CARTESIAN_POINT('Ctrl Pts',(-37.9499063932492,37.8848528852835,18.0822865395925));
#67489=CARTESIAN_POINT('Ctrl Pts',(-39.2737503688799,37.3944644332241,18.0037810292158));
#67490=CARTESIAN_POINT('Ctrl Pts',(-40.4101887889945,38.2300135840309,17.925275518839));
#67491=CARTESIAN_POINT('Ctrl Pts',(-40.3414544576775,39.6379280568325,17.8467700084622));
#67492=CARTESIAN_POINT('Ctrl Pts',(-39.1285059374216,40.3576224572915,17.7682644980854));
#67493=CARTESIAN_POINT('Ctrl Pts',(-37.8594794698809,39.7426407928426,17.6897589877086));
#67494=CARTESIAN_POINT('Ctrl Pts',(-37.6723029617942,38.3450146680762,17.6112534773319));
#67495=CARTESIAN_POINT('Ctrl Pts',(-38.7349222194718,37.4179211332814,17.5327479669551));
#67496=CARTESIAN_POINT('Ctrl Pts',(-40.0943148545955,37.7929216657555,17.4542424565783));
#67497=CARTESIAN_POINT('Ctrl Pts',(-40.5313650479903,39.1336467274836,17.3757369462015));
#67498=CARTESIAN_POINT('Ctrl Pts',(-39.6541060242733,40.2377318715238,17.2972314358247));
#67499=CARTESIAN_POINT('Ctrl Pts',(-38.2492893507211,40.11499266379,17.218725925448));
#67500=CARTESIAN_POINT('Ctrl Pts',(-37.5767856410754,38.8755117583229,17.1402204150712));
#67501=CARTESIAN_POINT('Ctrl Pts',(-38.239713382144,37.6308815400461,17.0617149046944));
#67502=CARTESIAN_POINT('Ctrl Pts',(-39.6435426374601,37.4973177328599,16.9832093943176));
#67503=CARTESIAN_POINT('Ctrl Pts',(-40.5292862418181,38.5946026689388,16.9047038839408));
#67504=CARTESIAN_POINT('Ctrl Pts',(-40.1025881328798,39.9386655579506,16.8261983735641));
#67505=CARTESIAN_POINT('Ctrl Pts',(-38.7461213882494,40.3241186372757,16.7476928631873));
#67506=CARTESIAN_POINT('Ctrl Pts',(-37.6763975984645,39.4052785255607,16.6691873528105));
#67507=CARTESIAN_POINT('Ctrl Pts',(-37.8527705062975,38.0061828279691,16.5906818424337));
#67508=CARTESIAN_POINT('Ctrl Pts',(-39.1170646866591,37.3815738529462,16.5121763320569));
#67509=CARTESIAN_POINT('Ctrl Pts',(-40.335431065832,38.0916157660679,16.4336708216802));
#67510=CARTESIAN_POINT('Ctrl Pts',(-40.4152097079431,39.4995261055097,16.3551653113034));
#67511=CARTESIAN_POINT('Ctrl Pts',(-39.2848532311266,40.3426574046748,16.2766598009266));
#67512=CARTESIAN_POINT('Ctrl Pts',(-37.9580921959656,39.8648694716751,16.1981542905498));
#67513=CARTESIAN_POINT('Ctrl Pts',(-37.6247974410155,38.4946538828284,16.1196487801731));
#67514=CARTESIAN_POINT('Ctrl Pts',(-38.5838756259393,37.4608525536223,16.0411432697963));
#67515=CARTESIAN_POINT('Ctrl Pts',(-39.9752026339518,37.6906030930571,15.9626377594195));
#67516=CARTESIAN_POINT('Ctrl Pts',(-40.5510033269789,38.9778597555962,15.8841322490427));
#67517=CARTESIAN_POINT('Ctrl Pts',(-39.7948859553666,40.1681801631584,15.8056267386659));
#67518=CARTESIAN_POINT('Ctrl Pts',(-38.3849545521789,40.1940566766181,15.7271212282891));
#67519=CARTESIAN_POINT('Ctrl Pts',(-37.5856691219436,39.0322826222935,15.6486157179124));
#67520=CARTESIAN_POINT('Ctrl Pts',(-38.1138478344451,37.7247645941825,15.5701102075356));
#67521=CARTESIAN_POINT('Ctrl Pts',(-39.4958074756928,37.444115839331,15.4916046971588));
#67522=CARTESIAN_POINT('Ctrl Pts',(-40.4921737606506,38.4420288433187,15.413099186782));
#67523=CARTESIAN_POINT('Ctrl Pts',(-40.209381767505,39.823551479493,15.3345936764052));
#67524=CARTESIAN_POINT('Ctrl Pts',(-38.9010459777483,40.3497014457877,15.2560881660285));
#67525=CARTESIAN_POINT('Ctrl Pts',(-37.7405132362414,39.5486148590214,15.1775826556517));
#67526=CARTESIAN_POINT('Ctrl Pts',(-37.768576480582,38.1387253871163,15.0990771452749));
#67527=CARTESIAN_POINT('Ctrl Pts',(-38.960068767709,37.3844550775834,15.0205716348981));
#67528=CARTESIAN_POINT('Ctrl Pts',(-40.2464297818749,37.9622521836149,14.9420661245214));
#67529=CARTESIAN_POINT('Ctrl Pts',(-40.4740238443987,39.3539330888908,14.8635606141446));
#67530=CARTESIAN_POINT('Ctrl Pts',(-39.4387321729189,40.3114081825342,14.7850551037678));
#67531=CARTESIAN_POINT('Ctrl Pts',(-38.0690431779005,39.9759851367876,14.706549593391));
#67532=CARTESIAN_POINT('Ctrl Pts',(-37.5932976652751,38.6484912787975,14.6280440830142));
#67533=CARTESIAN_POINT('Ctrl Pts',(-38.4382140137078,37.5194303977126,14.5495385726375));
#67534=CARTESIAN_POINT('Ctrl Pts',(-39.8459325512601,37.6014203290504,14.4710330622607));
#67535=CARTESIAN_POINT('Ctrl Pts',(-40.5542183171743,38.8208308000283,14.3925275518839));
#67536=CARTESIAN_POINT('Ctrl Pts',(-39.9273761492841,40.0842677946574,14.3140220415071));
#67537=CARTESIAN_POINT('Ctrl Pts',(-38.5285619958217,40.2582405945396,14.2355165311303));
#67538=CARTESIAN_POINT('Ctrl Pts',(-37.6102568914307,39.1875630514033,14.1570110207536));
#67539=CARTESIAN_POINT('Ctrl Pts',(-38.0001325696021,37.8307135161573,14.0785055103768));
#67540=CARTESIAN_POINT('Ctrl Pts',(-38.8929078719873,37.5499386892516,14.0261685034589));
#67541=CARTESIAN_POINT('Ctrl Pts',(-39.3014489339362,37.6274127691862,14.));
#67542=CARTESIAN_POINT('Ctrl Pts',(-38.4348713855213,37.7748596688486,17.5565803263806));
#67543=CARTESIAN_POINT('Ctrl Pts',(-38.5438548719482,37.7108039030124,17.5486362065721));
#67544=CARTESIAN_POINT('Ctrl Pts',(-38.6618404864523,37.6628704742542,17.5406920867636));
#67545=CARTESIAN_POINT('Ctrl Pts',(-38.7843844490461,37.6349368111595,17.5327479669551));
#67546=CARTESIAN_POINT('Ctrl Pts',(-39.1880530978463,37.5429213107728,17.5065794634961));
#67547=CARTESIAN_POINT('Ctrl Pts',(-39.6411839762209,37.6679214882641,17.4804109600372));
#67548=CARTESIAN_POINT('Ctrl Pts',(-39.9405911143073,37.9538757539645,17.4542424565783));
#67549=CARTESIAN_POINT('Ctrl Pts',(-40.2399982523938,38.2398300196648,17.4280739531194));
#67550=CARTESIAN_POINT('Ctrl Pts',(-40.385681650192,38.6867383735742,17.4019054496604));
#67551=CARTESIAN_POINT('Ctrl Pts',(-40.312313511805,39.0942067412023,17.3757369462015));
#67552=CARTESIAN_POINT('Ctrl Pts',(-40.2389453734179,39.5016751088303,17.3495684427426));
#67553=CARTESIAN_POINT('Ctrl Pts',(-39.9465256988456,39.869703490177,17.3233999392837));
#67554=CARTESIAN_POINT('Ctrl Pts',(-39.5661797493007,40.0332611462281,17.2972314358247));
#67555=CARTESIAN_POINT('Ctrl Pts',(-39.1858337997559,40.1968188022792,17.2710629323658));
#67556=CARTESIAN_POINT('Ctrl Pts',(-38.7175615752385,40.1559057330346,17.2448944289069));
#67557=CARTESIAN_POINT('Ctrl Pts',(-38.3713415113722,39.9288690475011,17.218725925448));
#67558=CARTESIAN_POINT('Ctrl Pts',(-38.0251214475059,39.7018323619676,17.192557421989));
#67559=CARTESIAN_POINT('Ctrl Pts',(-37.8009535442906,39.2886720601453,17.1663889185301));
#67560=CARTESIAN_POINT('Ctrl Pts',(-37.7993575495278,38.8746535395213,17.1402204150712));
#67561=CARTESIAN_POINT('Ctrl Pts',(-37.797761554765,38.4606350188973,17.1140519116123));
#67562=CARTESIAN_POINT('Ctrl Pts',(-38.0187374684545,38.0457582794717,17.0878834081533));
#67563=CARTESIAN_POINT('Ctrl Pts',(-38.3631969678519,37.8160592752279,17.0617149046944));
#67564=CARTESIAN_POINT('Ctrl Pts',(-38.3857260141202,37.8010360301049,17.0600033785898));
#67565=CARTESIAN_POINT('Ctrl Pts',(-38.4087832848556,37.7868049178791,17.0582918524852));
#67566=CARTESIAN_POINT('Ctrl Pts',(-38.4323100738575,37.7733715239653,17.0565803263806));
#67567=CARTESIAN_POINT('Origin',(-39.0658530619283,38.8697713466882,15.5));
#67568=CARTESIAN_POINT('Origin',(14.1292828945603,53.2669068454841,14.));
#67569=CARTESIAN_POINT('Ctrl Pts',(12.9355708698302,52.8497595669186,14.));
#67570=CARTESIAN_POINT('Ctrl Pts',(12.9470539462111,52.800184379949,14.));
#67571=CARTESIAN_POINT('Ctrl Pts',(12.9617293958091,52.7515166200376,14.));
#67572=CARTESIAN_POINT('Ctrl Pts',(12.9793332579427,52.7039252046945,14.));
#67573=CARTESIAN_POINT('Ctrl Pts',(12.991196608558,52.6718530581276,14.));
#67574=CARTESIAN_POINT('Ctrl Pts',(13.0043910411423,52.640269588579,14.));
#67575=CARTESIAN_POINT('Ctrl Pts',(13.0188485043022,52.6092270378147,14.));
#67576=CARTESIAN_POINT('Ctrl Pts',(13.0255213915297,52.5948992516592,14.));
#67577=CARTESIAN_POINT('Ctrl Pts',(13.0324634794561,52.5806867163328,14.));
#67578=CARTESIAN_POINT('Ctrl Pts',(13.0396687478355,52.5665947050889,14.));
#67579=CARTESIAN_POINT('Ctrl Pts',(13.0457249481514,52.5547500327666,14.));
#67580=CARTESIAN_POINT('Ctrl Pts',(13.0519637639815,52.5429971707228,14.));
#67581=CARTESIAN_POINT('Ctrl Pts',(13.0583775077155,52.5313453176603,14.));
#67582=CARTESIAN_POINT('Ctrl Pts',(13.0842985632238,52.4842545166353,14.));
#67583=CARTESIAN_POINT('Ctrl Pts',(13.1130890591366,52.4387805987021,14.));
#67584=CARTESIAN_POINT('Ctrl Pts',(13.1444873892533,52.395119273701,14.));
#67585=CARTESIAN_POINT('Ctrl Pts',(13.1565047144307,52.3784084378615,14.));
#67586=CARTESIAN_POINT('Ctrl Pts',(13.1689046040936,52.3619632326356,14.));
#67587=CARTESIAN_POINT('Ctrl Pts',(13.1816743222884,52.3457951881286,14.));
#67588=CARTESIAN_POINT('Ctrl Pts',(13.1908504259838,52.3341771045746,14.));
#67589=CARTESIAN_POINT('Ctrl Pts',(13.2002175166929,52.32270214338,14.));
#67590=CARTESIAN_POINT('Ctrl Pts',(13.2097711770809,52.3113747299413,14.));
#67591=CARTESIAN_POINT('Ctrl Pts',(13.2171669953397,52.3026057882235,14.));
#67592=CARTESIAN_POINT('Ctrl Pts',(13.2246749676048,52.2939250679898,14.));
#67593=CARTESIAN_POINT('Ctrl Pts',(13.2322825219484,52.2853461207869,14.));
#67594=CARTESIAN_POINT('Ctrl Pts',(13.2698783495153,52.2429497598573,14.));
#67595=CARTESIAN_POINT('Ctrl Pts',(13.3099602110309,52.2029670203905,14.));
#67596=CARTESIAN_POINT('Ctrl Pts',(13.3522361487098,52.165610756381,14.));
#67597=CARTESIAN_POINT('Ctrl Pts',(13.393899569609,52.1287957302432,14.));
#67598=CARTESIAN_POINT('Ctrl Pts',(13.4376947733247,52.0945306975985,14.));
#67599=CARTESIAN_POINT('Ctrl Pts',(13.4833901900509,52.0630423693642,14.));
#67600=CARTESIAN_POINT('Ctrl Pts',(13.5072520754399,52.0465993443685,14.));
#67601=CARTESIAN_POINT('Ctrl Pts',(13.5316328454212,52.0309139559169,14.));
#67602=CARTESIAN_POINT('Ctrl Pts',(13.5565037014717,52.0160223211503,14.));
#67603=CARTESIAN_POINT('Ctrl Pts',(13.5698458263775,52.0080336113647,14.));
#67604=CARTESIAN_POINT('Ctrl Pts',(13.583329035386,52.0002733832793,14.));
#67605=CARTESIAN_POINT('Ctrl Pts',(13.5969491666071,51.9927476035671,14.));
#67606=CARTESIAN_POINT('Ctrl Pts',(13.606631569296,51.9873976088762,14.));
#67607=CARTESIAN_POINT('Ctrl Pts',(13.61638317152,51.9821661015547,14.));
#67608=CARTESIAN_POINT('Ctrl Pts',(13.6262025323318,51.977055318658,14.));
#67609=CARTESIAN_POINT('Ctrl Pts',(13.6348477565097,51.9725556506333,14.));
#67610=CARTESIAN_POINT('Ctrl Pts',(13.6435368081695,51.9681540962494,14.));
#67611=CARTESIAN_POINT('Ctrl Pts',(13.6522677898656,51.9638519547421,14.));
#67612=CARTESIAN_POINT('Ctrl Pts',(13.6954565667589,51.9425709308905,14.));
#67613=CARTESIAN_POINT('Ctrl Pts',(13.739673922891,51.9237189359383,14.));
#67614=CARTESIAN_POINT('Ctrl Pts',(13.7847671512145,51.9074289316259,14.));
#67615=CARTESIAN_POINT('Ctrl Pts',(13.8360916879594,51.888887856702,14.));
#67616=CARTESIAN_POINT('Ctrl Pts',(13.8885506645683,51.8736638854927,14.));
#67617=CARTESIAN_POINT('Ctrl Pts',(13.9418473749851,51.8616392672974,14.));
#67618=CARTESIAN_POINT('Ctrl Pts',(13.9939442076033,51.8498853613524,14.));
#67619=CARTESIAN_POINT('Ctrl Pts',(14.0468423626153,51.841188535496,14.));
#67620=CARTESIAN_POINT('Ctrl Pts',(14.1002842110465,51.8354800340528,14.));
#67621=CARTESIAN_POINT('Ctrl Pts',(14.1133747158556,51.8340817447386,14.));
#67622=CARTESIAN_POINT('Ctrl Pts',(14.1264979008037,51.8328629457893,14.));
#67623=CARTESIAN_POINT('Ctrl Pts',(14.1396500710493,51.8318229994997,14.));
#67624=CARTESIAN_POINT('Ctrl Pts',(14.1495801724506,51.8310378232197,14.));
#67625=CARTESIAN_POINT('Ctrl Pts',(14.1595248275512,51.8303548395254,14.));
#67626=CARTESIAN_POINT('Ctrl Pts',(14.169470914275,51.8297741437739,14.));
#67627=CARTESIAN_POINT('Ctrl Pts',(14.2269882875851,51.8264160296488,14.));
#67628=CARTESIAN_POINT('Ctrl Pts',(14.2846572206784,51.8264659494126,14.));
#67629=CARTESIAN_POINT('Ctrl Pts',(14.3421515421323,51.8297896308138,14.));
#67630=CARTESIAN_POINT('Ctrl Pts',(14.4008791522774,51.8331846072331,14.));
#67631=CARTESIAN_POINT('Ctrl Pts',(14.4594256019286,51.8399951697904,14.));
#67632=CARTESIAN_POINT('Ctrl Pts',(14.5174614759233,51.8501296661746,14.));
#67633=CARTESIAN_POINT('Ctrl Pts',(14.5760079665237,51.8603533288243,14.));
#67634=CARTESIAN_POINT('Ctrl Pts',(14.6340360434159,51.8739596391018,14.));
#67635=CARTESIAN_POINT('Ctrl Pts',(14.6912089919261,51.8909073924039,14.));
#67636=CARTESIAN_POINT('Ctrl Pts',(14.7041595779211,51.8947463292138,14.));
#67637=CARTESIAN_POINT('Ctrl Pts',(14.7170698109109,51.8987582304328,14.));
#67638=CARTESIAN_POINT('Ctrl Pts',(14.7299100501063,51.9029342190465,14.));
#67639=CARTESIAN_POINT('Ctrl Pts',(14.7877641555218,51.9217499188006,14.));
#67640=CARTESIAN_POINT('Ctrl Pts',(14.8442964941461,51.9439200711341,14.));
#67641=CARTESIAN_POINT('Ctrl Pts',(14.8991630095604,51.9693357900552,14.));
#67642=CARTESIAN_POINT('Ctrl Pts',(14.9535472829614,51.9945281208612,14.));
#67643=CARTESIAN_POINT('Ctrl Pts',(15.0062960529788,52.0229093770711,14.));
#67644=CARTESIAN_POINT('Ctrl Pts',(15.0570711073182,52.0544235838104,14.));
#67645=CARTESIAN_POINT('Ctrl Pts',(15.0942742802838,52.0775142234847,14.));
#67646=CARTESIAN_POINT('Ctrl Pts',(15.1304178629043,52.1022878477767,14.));
#67647=CARTESIAN_POINT('Ctrl Pts',(15.1653622380935,52.1287390412771,14.));
#67648=CARTESIAN_POINT('Ctrl Pts',(15.1847827002204,52.1434393871499,14.));
#67649=CARTESIAN_POINT('Ctrl Pts',(15.2038326363704,52.1586581279523,14.));
#67650=CARTESIAN_POINT('Ctrl Pts',(15.2225055381224,52.1743757967134,14.));
#67651=CARTESIAN_POINT('Ctrl Pts',(15.6194800884629,52.8667052421829,14.));
#67652=CARTESIAN_POINT('Ctrl Pts',(15.6300068882699,52.9268481278985,14.));
#67653=CARTESIAN_POINT('Ctrl Pts',(15.6366488600629,52.9875198480058,14.));
#67654=CARTESIAN_POINT('Ctrl Pts',(15.6395377285819,53.0483965304076,14.));
#67655=CARTESIAN_POINT('Ctrl Pts',(15.6422164647753,53.1048451266012,14.));
#67656=CARTESIAN_POINT('Ctrl Pts',(15.6416673528962,53.1614706817507,14.));
#67657=CARTESIAN_POINT('Ctrl Pts',(15.637955789909,53.2180062233477,14.));
#67658=CARTESIAN_POINT('Ctrl Pts',(15.6370599130148,53.2316524649969,14.));
#67659=CARTESIAN_POINT('Ctrl Pts',(15.63597945886,53.2452938319744,14.));
#67660=CARTESIAN_POINT('Ctrl Pts',(15.6347168346769,53.2589112013863,14.));
#67661=CARTESIAN_POINT('Ctrl Pts',(15.6291600434151,53.3188410525391,14.));
#67662=CARTESIAN_POINT('Ctrl Pts',(15.6200747337896,53.378379872231,14.));
#67663=CARTESIAN_POINT('Ctrl Pts',(15.6075583989768,53.4372064199478,14.));
#67664=CARTESIAN_POINT('Ctrl Pts',(15.5998328638163,53.473516295766,14.));
#67665=CARTESIAN_POINT('Ctrl Pts',(15.5907991790393,53.5095545290085,14.));
#67666=CARTESIAN_POINT('Ctrl Pts',(15.5804715530865,53.5452408049656,14.));
#67667=CARTESIAN_POINT('Ctrl Pts',(15.5769376859297,53.5574517970299,14.));
#67668=CARTESIAN_POINT('Ctrl Pts',(15.5732522648484,53.5696215402532,14.));
#67669=CARTESIAN_POINT('Ctrl Pts',(15.5694156967786,53.5817466814784,14.));
#67670=CARTESIAN_POINT('Ctrl Pts',(15.5658265664347,53.5930898171937,14.));
#67671=CARTESIAN_POINT('Ctrl Pts',(15.5621073991623,53.604386674236,14.));
#67672=CARTESIAN_POINT('Ctrl Pts',(15.5582610327089,53.6156290047843,14.));
#67673=CARTESIAN_POINT('Ctrl Pts',(15.5392227656735,53.6712748964768,14.));
#67674=CARTESIAN_POINT('Ctrl Pts',(15.5170576051216,53.7256323263693,14.));
#67675=CARTESIAN_POINT('Ctrl Pts',(15.4918565785963,53.778400265489,14.));
#67676=CARTESIAN_POINT('Ctrl Pts',(15.4672989399364,53.8298210272756,14.));
#67677=CARTESIAN_POINT('Ctrl Pts',(15.4398578622269,53.8797331989797,14.));
#67678=CARTESIAN_POINT('Ctrl Pts',(15.4095790814356,53.9278277241522,14.));
#67679=CARTESIAN_POINT('Ctrl Pts',(15.393162829712,53.9539031410322,14.));
#67680=CARTESIAN_POINT('Ctrl Pts',(15.3759118210083,53.9794436628058,14.));
#67681=CARTESIAN_POINT('Ctrl Pts',(15.3578293393225,54.0043949447537,14.));
#67682=CARTESIAN_POINT('Ctrl Pts',(15.3427850973017,54.0251538832043,14.));
#67683=CARTESIAN_POINT('Ctrl Pts',(15.3271652650927,54.0455049013344,14.));
#67684=CARTESIAN_POINT('Ctrl Pts',(15.3109704282784,54.0654144329311,14.));
#67685=CARTESIAN_POINT('Ctrl Pts',(15.3040483577008,54.0739242551948,14.));
#67686=CARTESIAN_POINT('Ctrl Pts',(15.2970202961045,54.0823543059347,14.));
#67687=CARTESIAN_POINT('Ctrl Pts',(15.2898980775462,54.0906884965195,14.));
#67688=CARTESIAN_POINT('Ctrl Pts',(15.2569263348732,54.1292709670099,14.));
#67689=CARTESIAN_POINT('Ctrl Pts',(15.2218841351082,54.1658696978399,14.));
#67690=CARTESIAN_POINT('Ctrl Pts',(15.1848122311441,54.2002693479339,14.));
#67691=CARTESIAN_POINT('Ctrl Pts',(15.1433853438138,54.2387100611496,14.));
#67692=CARTESIAN_POINT('Ctrl Pts',(15.0994234021552,54.2744057498411,14.));
#67693=CARTESIAN_POINT('Ctrl Pts',(15.0532626173727,54.3072661456687,14.));
#67694=CARTESIAN_POINT('Ctrl Pts',(15.0140905649692,54.3351514849978,14.));
#67695=CARTESIAN_POINT('Ctrl Pts',(14.9733341416939,54.3609943509907,14.));
#67696=CARTESIAN_POINT('Ctrl Pts',(14.9311912107702,54.3847111211327,14.));
#67697=CARTESIAN_POINT('Ctrl Pts',(14.9196049423228,54.3912315234765,14.));
#67698=CARTESIAN_POINT('Ctrl Pts',(14.9079138627929,54.3975910665355,14.));
#67699=CARTESIAN_POINT('Ctrl Pts',(14.8961220820593,54.4037876495875,14.));
#67700=CARTESIAN_POINT('Ctrl Pts',(14.8869418706782,54.4086118524406,14.));
#67701=CARTESIAN_POINT('Ctrl Pts',(14.8776989838853,54.4133380017409,14.));
#67702=CARTESIAN_POINT('Ctrl Pts',(14.8684106168162,54.417957742305,14.));
#67703=CARTESIAN_POINT('Ctrl Pts',(14.8187084869401,54.4426780127036,14.));
#67704=CARTESIAN_POINT('Ctrl Pts',(14.7676148803425,54.4644045890752,14.));
#67705=CARTESIAN_POINT('Ctrl Pts',(14.7154497955799,54.4830620982223,14.));
#67706=CARTESIAN_POINT('Ctrl Pts',(14.6635765838278,54.5016152152576,14.));
#67707=CARTESIAN_POINT('Ctrl Pts',(14.6106426601222,54.5171336376019,14.));
#67708=CARTESIAN_POINT('Ctrl Pts',(14.5569565024563,54.5294926610653,14.));
#67709=CARTESIAN_POINT('Ctrl Pts',(14.5071457936081,54.5409595222851,14.));
#67710=CARTESIAN_POINT('Ctrl Pts',(14.4566867638904,54.5497062605815,14.));
#67711=CARTESIAN_POINT('Ctrl Pts',(14.4058341276533,54.5555924980468,14.));
#67712=CARTESIAN_POINT('Ctrl Pts',(14.3927717853116,54.5571044756858,14.));
#67713=CARTESIAN_POINT('Ctrl Pts',(14.3796790109904,54.5584277519276,14.));
#67714=CARTESIAN_POINT('Ctrl Pts',(14.3665890681889,54.559557479464,14.));
#67715=CARTESIAN_POINT('Ctrl Pts',(14.313676726905,54.5641240791709,14.));
#67716=CARTESIAN_POINT('Ctrl Pts',(14.2607272248354,54.5655439858659,14.));
#67717=CARTESIAN_POINT('Ctrl Pts',(14.2080224885655,54.5637141509331,14.));
#67718=CARTESIAN_POINT('Ctrl Pts',(14.1571049407721,54.5619463646915,14.));
#67719=CARTESIAN_POINT('Ctrl Pts',(14.1064149890642,54.5571453217378,14.));
#67720=CARTESIAN_POINT('Ctrl Pts',(14.0562198243928,54.5491721895681,14.));
#67721=CARTESIAN_POINT('Ctrl Pts',(14.0211056129997,54.54359455574,14.));
#67722=CARTESIAN_POINT('Ctrl Pts',(13.9862337962434,54.5364636409183,14.));
#67723=CARTESIAN_POINT('Ctrl Pts',(13.9517030424607,54.5277184245241,14.));
#67724=CARTESIAN_POINT('Ctrl Pts',(13.93222381495,54.5227851392317,14.));
#67725=CARTESIAN_POINT('Ctrl Pts',(13.9128532514771,54.5173379031513,14.));
#67726=CARTESIAN_POINT('Ctrl Pts',(13.8936069362009,54.5113866946539,14.));
#67727=CARTESIAN_POINT('Origin',(14.1292828945603,53.2669068454841,19.1042117235887));
#67728=CARTESIAN_POINT('Ctrl Pts',(13.3561844802682,51.9293619476186,17.8542117235887));
#67729=CARTESIAN_POINT('Ctrl Pts',(13.3145289674605,51.9530637836679,17.8517311518799));
#67730=CARTESIAN_POINT('Ctrl Pts',(12.8472204745978,52.2501100679509,17.8230820767121));
#67731=CARTESIAN_POINT('Ctrl Pts',(12.3131148719809,53.3266292410367,17.7682644980854));
#67732=CARTESIAN_POINT('Ctrl Pts',(13.177398497422,54.8146003900027,17.6897589877087));
#67733=CARTESIAN_POINT('Ctrl Pts',(14.8951536251653,54.9146504373755,17.6112534773318));
#67734=CARTESIAN_POINT('Ctrl Pts',(15.9261572824593,53.5369216264007,17.5327479669551));
#67735=CARTESIAN_POINT('Ctrl Pts',(15.3456319213627,51.9170585592589,17.4542424565783));
#67736=CARTESIAN_POINT('Ctrl Pts',(14.0786429713653,51.6067853756627,17.3947303754562));
#67737=CARTESIAN_POINT('Ctrl Pts',(13.4791850640252,51.8598443884631,17.361386797793));
#67738=CARTESIAN_POINT('Ctrl Pts',(13.3591951473145,51.9304670067728,17.3542117235887));
#67739=CARTESIAN_POINT('Ctrl Pts',(13.3599426557471,51.9312965605688,17.8957882764113));
#67740=CARTESIAN_POINT('Ctrl Pts',(13.0649944461637,52.1042822226529,17.8781885106897));
#67741=CARTESIAN_POINT('Ctrl Pts',(12.4640754788204,52.7732237750949,17.8344202415091));
#67742=CARTESIAN_POINT('Ctrl Pts',(12.6330157688953,54.2972115132025,17.7644834688697));
#67743=CARTESIAN_POINT('Ctrl Pts',(14.1627629159667,55.0835833760401,17.6859779584929));
#67744=CARTESIAN_POINT('Ctrl Pts',(15.6633630152513,54.2408836460551,17.6074724481161));
#67745=CARTESIAN_POINT('Ctrl Pts',(15.7877283921754,52.5246154983423,17.5289669377393));
#67746=CARTESIAN_POINT('Ctrl Pts',(14.5628755318023,51.5803972945989,17.4584055471711));
#67747=CARTESIAN_POINT('Ctrl Pts',(13.6650283227152,51.7575311866648,17.4140126600617));
#67748=CARTESIAN_POINT('Ctrl Pts',(13.3571987246687,51.9320818411208,17.3957882764113));
#67749=CARTESIAN_POINT('Ctrl Pts',(13.8936870225526,54.5092654229862,18.));
#67750=CARTESIAN_POINT('Ctrl Pts',(14.3022280845015,54.5867395029208,17.9738314965411));
#67751=CARTESIAN_POINT('Ctrl Pts',(15.1949907864185,54.306005850961,17.9214944896232));
#67752=CARTESIAN_POINT('Ctrl Pts',(15.5848805170291,52.9490991612648,17.8429889792464));
#67753=CARTESIAN_POINT('Ctrl Pts',(14.6665684258223,51.8784501685123,17.7644834688696));
#67754=CARTESIAN_POINT('Ctrl Pts',(13.2677649070697,52.052408782696,17.6859779584929));
#67755=CARTESIAN_POINT('Ctrl Pts',(12.6409196641315,53.3158497937513,17.6074724481161));
#67756=CARTESIAN_POINT('Ctrl Pts',(13.3492065366981,54.5352532401981,17.5289669377393));
#67757=CARTESIAN_POINT('Ctrl Pts',(14.7569196663361,54.6172449996945,17.4504614273625));
#67758=CARTESIAN_POINT('Ctrl Pts',(15.6018348475728,53.488185970869,17.3719559169858));
#67759=CARTESIAN_POINT('Ctrl Pts',(15.1260899874907,52.1606961144849,17.293450406609));
#67760=CARTESIAN_POINT('Ctrl Pts',(13.7564048649609,51.8252736441527,17.2149448962322));
#67761=CARTESIAN_POINT('Ctrl Pts',(12.7211156974588,52.7827464099985,17.1364393858554));
#67762=CARTESIAN_POINT('Ctrl Pts',(12.948709267523,54.1744236301459,17.0579338754786));
#67763=CARTESIAN_POINT('Ctrl Pts',(14.2350668963378,54.7522192803303,16.9794283651019));
#67764=CARTESIAN_POINT('Ctrl Pts',(15.4265561246117,53.9979509037444,16.900922854725));
#67765=CARTESIAN_POINT('Ctrl Pts',(15.4546192812222,52.5880650956991,16.8224173443483));
#67766=CARTESIAN_POINT('Ctrl Pts',(14.2940895544972,51.7869805788024,16.7439118339715));
#67767=CARTESIAN_POINT('Ctrl Pts',(12.9857571502944,52.3131291848103,16.6654063235948));
#67768=CARTESIAN_POINT('Ctrl Pts',(12.7029658920433,53.6946482401115,16.586900813218));
#67769=CARTESIAN_POINT('Ctrl Pts',(13.6993295943645,54.69255865938,16.5083953028412));
#67770=CARTESIAN_POINT('Ctrl Pts',(15.0812856557068,54.4119106312665,16.4298897924644));
#67771=CARTESIAN_POINT('Ctrl Pts',(15.6094629994387,53.1043959909962,16.3513842820876));
#67772=CARTESIAN_POINT('Ctrl Pts',(14.8101796402302,51.9426249466013,16.2728787717108));
#67773=CARTESIAN_POINT('Ctrl Pts',(13.4002518899393,51.9685013930707,16.1943732613341));
#67774=CARTESIAN_POINT('Ctrl Pts',(12.6441364773908,53.1588187166123,16.1158677509573));
#67775=CARTESIAN_POINT('Ctrl Pts',(13.2199356785564,54.4460720440219,16.0373622405805));
#67776=CARTESIAN_POINT('Ctrl Pts',(14.6112590818024,54.6758219881873,15.9588567302037));
#67777=CARTESIAN_POINT('Ctrl Pts',(15.5703347818477,53.6420233374599,15.8803512198269));
#67778=CARTESIAN_POINT('Ctrl Pts',(15.2370408904378,52.2718112986816,15.8018457094502));
#67779=CARTESIAN_POINT('Ctrl Pts',(13.9102832927596,51.7940246036041,15.7233401990734));
#67780=CARTESIAN_POINT('Ctrl Pts',(12.7799297446004,52.6371537182599,15.6448346886966));
#67781=CARTESIAN_POINT('Ctrl Pts',(12.8597081799673,54.0450604100449,15.5663291783198));
#67782=CARTESIAN_POINT('Ctrl Pts',(14.0780714025732,54.7551004833527,15.4878236679431));
#67783=CARTESIAN_POINT('Ctrl Pts',(15.3423623071066,54.1304931269541,15.4093181575663));
#67784=CARTESIAN_POINT('Ctrl Pts',(15.5187347583226,52.7314010536377,15.3308126471895));
#67785=CARTESIAN_POINT('Ctrl Pts',(14.4490137393998,51.8125633237516,15.2523071368127));
#67786=CARTESIAN_POINT('Ctrl Pts',(13.0925505105556,52.1980154020928,15.1738016264359));
#67787=CARTESIAN_POINT('Ctrl Pts',(12.6658535045584,53.5420748131919,15.0952961160591));
#67788=CARTESIAN_POINT('Ctrl Pts',(13.551594819097,54.6393568979554,15.0167906056824));
#67789=CARTESIAN_POINT('Ctrl Pts',(14.9554204274106,54.5057934526205,14.9382850953056));
#67790=CARTESIAN_POINT('Ctrl Pts',(15.6183464700208,53.2611664293564,14.8597795849288));
#67791=CARTESIAN_POINT('Ctrl Pts',(14.9458444656461,52.0216887907143,14.781274074552));
#67792=CARTESIAN_POINT('Ctrl Pts',(13.5410315037528,51.8989497980972,14.7027685641753));
#67793=CARTESIAN_POINT('Ctrl Pts',(12.6637746137877,53.0030322708737,14.6242630537985));
#67794=CARTESIAN_POINT('Ctrl Pts',(13.1008239433931,54.3437535140763,14.5457575434217));
#67795=CARTESIAN_POINT('Ctrl Pts',(14.4602125392811,54.7187536954986,14.4672520330449));
#67796=CARTESIAN_POINT('Ctrl Pts',(15.5228300373051,53.7916614633287,14.3887465226681));
#67797=CARTESIAN_POINT('Ctrl Pts',(15.3356521111637,52.3940408681935,14.3102410122914));
#67798=CARTESIAN_POINT('Ctrl Pts',(14.0666325655588,51.7790575741688,14.2317355019146));
#67799=CARTESIAN_POINT('Ctrl Pts',(12.8536802704289,52.4987553418112,14.1532299915378));
#67800=CARTESIAN_POINT('Ctrl Pts',(12.7849592886011,53.9066581474694,14.074724481161));
#67801=CARTESIAN_POINT('Ctrl Pts',(13.9213697617028,54.7422164034654,13.9962189707843));
#67802=CARTESIAN_POINT('Ctrl Pts',(15.2452696789898,54.2518096584207,13.9177134604075));
#67803=CARTESIAN_POINT('Ctrl Pts',(15.4583606841261,53.3405309695408,13.8653764534896));
#67804=CARTESIAN_POINT('Ctrl Pts',(15.3505106014235,52.9389386488708,13.8392079500307));
#67805=CARTESIAN_POINT('Ctrl Pts',(13.8763907393434,54.6004732426341,18.0535973499898));
#67806=CARTESIAN_POINT('Ctrl Pts',(14.314924864625,54.6836350861806,18.0274288465308));
#67807=CARTESIAN_POINT('Ctrl Pts',(15.2732297867829,54.3822913585465,17.975091839613));
#67808=CARTESIAN_POINT('Ctrl Pts',(15.6917432922651,52.9257672935819,17.8965863292362));
#67809=CARTESIAN_POINT('Ctrl Pts',(14.7060132710725,51.7765165492856,17.8180808188594));
#67810=CARTESIAN_POINT('Ctrl Pts',(13.2045165191651,51.9632463441864,17.7395753084827));
#67811=CARTESIAN_POINT('Ctrl Pts',(12.5316514000813,53.3194429428464,17.6610697981059));
#67812=CARTESIAN_POINT('Ctrl Pts',(13.2919371902727,54.6283689567997,17.5825642877291));
#67813=CARTESIAN_POINT('Ctrl Pts',(14.8029976526125,54.7163801455881,17.5040587773523));
#67814=CARTESIAN_POINT('Ctrl Pts',(15.7099423258683,53.5044311893796,17.4255532669755));
#67815=CARTESIAN_POINT('Ctrl Pts',(15.1992706321147,52.0794835960762,17.3470477565988));
#67816=CARTESIAN_POINT('Ctrl Pts',(13.7290300050048,51.7194360676216,17.268542246222));
#67817=CARTESIAN_POINT('Ctrl Pts',(12.6177350293705,52.7472017464205,17.1900367358452));
#67818=CARTESIAN_POINT('Ctrl Pts',(12.8620373932302,54.2410490221397,17.1115312254684));
#67819=CARTESIAN_POINT('Ctrl Pts',(14.2428330343357,54.8612635700639,17.0330257150916));
#67820=CARTESIAN_POINT('Ctrl Pts',(15.5217955063355,54.0516205413418,16.9545202047148));
#67821=CARTESIAN_POINT('Ctrl Pts',(15.5519189210496,52.5382278932962,16.8760146943381));
#67822=CARTESIAN_POINT('Ctrl Pts',(14.3061888440168,51.678331714885,16.7975091839613));
#67823=CARTESIAN_POINT('Ctrl Pts',(12.901805148244,52.2431075481956,16.7190036735845));
#67824=CARTESIAN_POINT('Ctrl Pts',(12.5982527550455,53.7260508968675,16.6404981632077));
#67825=CARTESIAN_POINT('Ctrl Pts',(13.6677645504461,54.7972229615204,16.561992652831));
#67826=CARTESIAN_POINT('Ctrl Pts',(15.1511769879803,54.4959711438117,16.4834871424542));
#67827=CARTESIAN_POINT('Ctrl Pts',(15.7181304989006,53.0924652481532,16.4049816320774));
#67828=CARTESIAN_POINT('Ctrl Pts',(14.8601677102629,51.8454027220491,16.3264761217006));
#67829=CARTESIAN_POINT('Ctrl Pts',(13.3467300407797,51.8731788891832,16.2479706113238));
#67830=CARTESIAN_POINT('Ctrl Pts',(12.5351043758535,53.1508834210038,16.1694651009471));
#67831=CARTESIAN_POINT('Ctrl Pts',(13.1531759053504,54.5326405184631,16.0909595905703));
#67832=CARTESIAN_POINT('Ctrl Pts',(14.6466433886817,54.7792575667409,16.0124540801935));
#67833=CARTESIAN_POINT('Ctrl Pts',(15.676129681178,53.6695625342478,15.9339485698167));
#67834=CARTESIAN_POINT('Ctrl Pts',(15.318367001378,52.1987563073058,15.8554430594399));
#67835=CARTESIAN_POINT('Ctrl Pts',(13.8942054255916,51.6858928771342,15.7769375490632));
#67836=CARTESIAN_POINT('Ctrl Pts',(12.680866912845,52.5909203596381,15.6984320386864));
#67837=CARTESIAN_POINT('Ctrl Pts',(12.7665022861979,54.1021885944998,15.6199265283096));
#67838=CARTESIAN_POINT('Ctrl Pts',(14.0743117082228,54.8643562967563,15.5414210179328));
#67839=CARTESIAN_POINT('Ctrl Pts',(15.4314205953349,54.1938933587689,15.4629155075561));
#67840=CARTESIAN_POINT('Ctrl Pts',(15.6207414392393,52.6920868680493,15.3844099971793));
#67841=CARTESIAN_POINT('Ctrl Pts',(14.4724867960198,51.7057926183866,15.3059044868025));
#67842=CARTESIAN_POINT('Ctrl Pts',(13.0164387486087,52.1195426811267,15.2273989764257));
#67843=CARTESIAN_POINT('Ctrl Pts',(12.5584157597012,53.5622762838672,15.1488934660489));
#67844=CARTESIAN_POINT('Ctrl Pts',(13.5091838189608,54.7401153900111,15.0703879556721));
#67845=CARTESIAN_POINT('Ctrl Pts',(15.0160713573958,54.5967463773832,14.9918824452954));
#67846=CARTESIAN_POINT('Ctrl Pts',(15.727666149938,53.2607449964075,14.9133769349186));
#67847=CARTESIAN_POINT('Ctrl Pts',(15.0057923758998,51.930271042394,14.8348714245418));
#67848=CARTESIAN_POINT('Ctrl Pts',(13.4978449972707,51.7985211602437,14.756365914165));
#67849=CARTESIAN_POINT('Ctrl Pts',(12.5561842470564,52.9836599052407,14.6778604037882));
#67850=CARTESIAN_POINT('Ctrl Pts',(13.0253195759487,54.4228102683146,14.5993548934115));
#67851=CARTESIAN_POINT('Ctrl Pts',(14.4845077563774,54.8253411075795,14.5208493830347));
#67852=CARTESIAN_POINT('Ctrl Pts',(15.6251373733416,53.830186350918,14.4423438726579));
#67853=CARTESIAN_POINT('Ctrl Pts',(15.4242177700075,52.3299593670269,14.3638383622811));
#67854=CARTESIAN_POINT('Ctrl Pts',(14.0620330883935,51.6698270424536,14.2853328519044));
#67855=CARTESIAN_POINT('Ctrl Pts',(12.7600318373669,52.442361459177,14.2068273415276));
#67856=CARTESIAN_POINT('Ctrl Pts',(12.6862657010804,53.9536255226118,14.1283218311508));
#67857=CARTESIAN_POINT('Ctrl Pts',(13.9061058082296,54.8505263314733,14.049816320774));
#67858=CARTESIAN_POINT('Ctrl Pts',(15.32719990687,54.3241163497092,13.9713108103972));
#67859=CARTESIAN_POINT('Ctrl Pts',(15.5559349992425,53.3459360884415,13.9189738034794));
#67860=CARTESIAN_POINT('Ctrl Pts',(15.4401670971033,52.9148608466415,13.8928053000205));
#67861=CARTESIAN_POINT('Ctrl Pts',(13.8590944561342,54.691681062282,18.1071946999795));
#67862=CARTESIAN_POINT('Ctrl Pts',(14.3276216447486,54.7805306694404,18.0810261965206));
#67863=CARTESIAN_POINT('Ctrl Pts',(15.3514687871473,54.4585768661318,18.0286891896028));
#67864=CARTESIAN_POINT('Ctrl Pts',(15.798606067501,52.9024354258991,17.950183679226));
#67865=CARTESIAN_POINT('Ctrl Pts',(14.7454581163227,51.6745829300588,17.8716781688492));
#67866=CARTESIAN_POINT('Ctrl Pts',(13.1412681312604,51.8740839056768,17.7931726584724));
#67867=CARTESIAN_POINT('Ctrl Pts',(12.4223831360311,53.3230360919415,17.7146671480956));
#67868=CARTESIAN_POINT('Ctrl Pts',(13.2346678438474,54.7214846734012,17.6361616377189));
#67869=CARTESIAN_POINT('Ctrl Pts',(14.8490756388889,54.8155152914818,17.5576561273421));
#67870=CARTESIAN_POINT('Ctrl Pts',(15.8180498041638,53.5206764078901,17.4791506169653));
#67871=CARTESIAN_POINT('Ctrl Pts',(15.2724512767386,51.9982710776676,17.4006451065885));
#67872=CARTESIAN_POINT('Ctrl Pts',(13.7016551450487,51.6135984910905,17.3221395962117));
#67873=CARTESIAN_POINT('Ctrl Pts',(12.5143543612823,52.7116570828427,17.243634085835));
#67874=CARTESIAN_POINT('Ctrl Pts',(12.7753655189374,54.3076744141334,17.1651285754582));
#67875=CARTESIAN_POINT('Ctrl Pts',(14.2505991723336,54.9703078597976,17.0866230650814));
#67876=CARTESIAN_POINT('Ctrl Pts',(15.6170348880593,54.1052901789391,17.0081175547046));
#67877=CARTESIAN_POINT('Ctrl Pts',(15.649218560877,52.4883906908934,16.9296120443279));
#67878=CARTESIAN_POINT('Ctrl Pts',(14.3182881335363,51.5696828509675,16.8511065339511));
#67879=CARTESIAN_POINT('Ctrl Pts',(12.8178531461937,52.173085911581,16.7726010235743));
#67880=CARTESIAN_POINT('Ctrl Pts',(12.4935396180477,53.7574535536235,16.6940955131975));
#67881=CARTESIAN_POINT('Ctrl Pts',(13.6361995065277,54.9018872636609,16.6155900028207));
#67882=CARTESIAN_POINT('Ctrl Pts',(15.2210683202537,54.580031656357,16.5370844924439));
#67883=CARTESIAN_POINT('Ctrl Pts',(15.8267979983625,53.0805345053102,16.4585789820672));
#67884=CARTESIAN_POINT('Ctrl Pts',(14.9101557802956,51.7481804974969,16.3800734716904));
#67885=CARTESIAN_POINT('Ctrl Pts',(13.2932081916201,51.7778563852958,16.3015679613136));
#67886=CARTESIAN_POINT('Ctrl Pts',(12.4260722743162,53.1429481253953,16.2230624509368));
#67887=CARTESIAN_POINT('Ctrl Pts',(13.0864161321444,54.6192089929043,16.14455694056));
#67888=CARTESIAN_POINT('Ctrl Pts',(14.6820276955611,54.8826931452944,16.0660514301833));
#67889=CARTESIAN_POINT('Ctrl Pts',(15.7819245805083,53.6971017310358,15.9875459198065));
#67890=CARTESIAN_POINT('Ctrl Pts',(15.3996931123183,52.1257013159298,15.9090404094297));
#67891=CARTESIAN_POINT('Ctrl Pts',(13.8781275584237,51.5777611506643,15.8305348990529));
#67892=CARTESIAN_POINT('Ctrl Pts',(12.5818040810897,52.5446870010162,15.7520293886761));
#67893=CARTESIAN_POINT('Ctrl Pts',(12.6732963924285,54.1593167789549,15.6735238782994));
#67894=CARTESIAN_POINT('Ctrl Pts',(14.0705520138724,54.9736121101599,15.5950183679226));
#67895=CARTESIAN_POINT('Ctrl Pts',(15.5204788835632,54.2572935905837,15.5165128575458));
#67896=CARTESIAN_POINT('Ctrl Pts',(15.7227481201561,52.6527726824611,15.438007347169));
#67897=CARTESIAN_POINT('Ctrl Pts',(14.4959598526397,51.5990219130214,15.3595018367923));
#67898=CARTESIAN_POINT('Ctrl Pts',(12.9403269866619,52.0410699601607,15.2809963264155));
#67899=CARTESIAN_POINT('Ctrl Pts',(12.4509780148441,53.5824777545425,15.2024908160387));
#67900=CARTESIAN_POINT('Ctrl Pts',(13.4667728188246,54.8408738820669,15.1239853056619));
#67901=CARTESIAN_POINT('Ctrl Pts',(15.0767222873809,54.6876993021459,15.0454797952852));
#67902=CARTESIAN_POINT('Ctrl Pts',(15.8369858298551,53.2603235634587,14.9669742849083));
#67903=CARTESIAN_POINT('Ctrl Pts',(15.0657402861535,51.8388532940734,14.8884687745316));
#67904=CARTESIAN_POINT('Ctrl Pts',(13.4546584907886,51.6980925223903,14.8099632641548));
#67905=CARTESIAN_POINT('Ctrl Pts',(12.4485938803251,52.9642875396075,14.731457753778));
#67906=CARTESIAN_POINT('Ctrl Pts',(12.9498152085044,54.5018670225528,14.6529522434012));
#67907=CARTESIAN_POINT('Ctrl Pts',(14.5088029734737,54.9319285196604,14.5744467330245));
#67908=CARTESIAN_POINT('Ctrl Pts',(15.7274447093781,53.8687112385071,14.4959412226477));
#67909=CARTESIAN_POINT('Ctrl Pts',(15.5127834288513,52.2658778658604,14.4174357122709));
#67910=CARTESIAN_POINT('Ctrl Pts',(14.0574336112281,51.5605965107385,14.3389302018941));
#67911=CARTESIAN_POINT('Ctrl Pts',(12.666383404305,52.3859675765427,14.2604246915173));
#67912=CARTESIAN_POINT('Ctrl Pts',(12.5875721135598,54.0005928977544,14.1819191811406));
#67913=CARTESIAN_POINT('Ctrl Pts',(13.8908418547563,54.9588362594811,14.1034136707638));
#67914=CARTESIAN_POINT('Ctrl Pts',(15.4091301347503,54.3964230409977,14.024908160387));
#67915=CARTESIAN_POINT('Ctrl Pts',(15.6535093143589,53.3513412073422,13.9725711534692));
#67916=CARTESIAN_POINT('Ctrl Pts',(15.5298235927831,52.8907830444122,13.9464026500102));
#67917=CARTESIAN_POINT('Ctrl Pts',(13.841798172925,54.7828888819299,18.1607920499693));
#67918=CARTESIAN_POINT('Ctrl Pts',(14.3403184248721,54.8774262527002,18.1346235465104));
#67919=CARTESIAN_POINT('Ctrl Pts',(15.4297077875118,54.5348623737173,18.0822865395925));
#67920=CARTESIAN_POINT('Ctrl Pts',(15.905468842737,52.8791035582161,18.0037810292158));
#67921=CARTESIAN_POINT('Ctrl Pts',(14.7849029615728,51.5726493108321,17.925275518839));
#67922=CARTESIAN_POINT('Ctrl Pts',(13.0780197433558,51.7849214671671,17.8467700084622));
#67923=CARTESIAN_POINT('Ctrl Pts',(12.3131148719809,53.3266292410367,17.7682644980854));
#67924=CARTESIAN_POINT('Ctrl Pts',(13.177398497422,54.8146003900027,17.6897589877087));
#67925=CARTESIAN_POINT('Ctrl Pts',(14.8951536251653,54.9146504373755,17.6112534773318));
#67926=CARTESIAN_POINT('Ctrl Pts',(15.9261572824593,53.5369216264007,17.5327479669551));
#67927=CARTESIAN_POINT('Ctrl Pts',(15.3456319213627,51.9170585592589,17.4542424565783));
#67928=CARTESIAN_POINT('Ctrl Pts',(13.6742802850926,51.5077609145594,17.3757369462015));
#67929=CARTESIAN_POINT('Ctrl Pts',(12.410973693194,52.6761124192647,17.2972314358247));
#67930=CARTESIAN_POINT('Ctrl Pts',(12.6886936446445,54.3742998061272,17.2187259254479));
#67931=CARTESIAN_POINT('Ctrl Pts',(14.2583653103316,55.0793521495312,17.1402204150712));
#67932=CARTESIAN_POINT('Ctrl Pts',(15.7122742697831,54.1589598165365,17.0617149046944));
#67933=CARTESIAN_POINT('Ctrl Pts',(15.7465182007044,52.4385534884905,16.9832093943176));
#67934=CARTESIAN_POINT('Ctrl Pts',(14.3303874230559,51.4610339870501,16.9047038839408));
#67935=CARTESIAN_POINT('Ctrl Pts',(12.7339011441433,52.1030642749663,16.8261983735641));
#67936=CARTESIAN_POINT('Ctrl Pts',(12.38882648105,53.7888562103795,16.7476928631873));
#67937=CARTESIAN_POINT('Ctrl Pts',(13.6046344626092,55.0065515658014,16.6691873528105));
#67938=CARTESIAN_POINT('Ctrl Pts',(15.2909596525271,54.6640921689023,16.5906818424337));
#67939=CARTESIAN_POINT('Ctrl Pts',(15.9354654978243,53.0686037624672,16.512176332057));
#67940=CARTESIAN_POINT('Ctrl Pts',(14.9601438503283,51.6509582729447,16.4336708216802));
#67941=CARTESIAN_POINT('Ctrl Pts',(13.2396863424605,51.6825338814083,16.3551653113034));
#67942=CARTESIAN_POINT('Ctrl Pts',(12.317040172779,53.1350128297868,16.2766598009266));
#67943=CARTESIAN_POINT('Ctrl Pts',(13.0196563589383,54.7057774673455,16.1981542905498));
#67944=CARTESIAN_POINT('Ctrl Pts',(14.7174120024405,54.9861287238479,16.1196487801731));
#67945=CARTESIAN_POINT('Ctrl Pts',(15.8877194798386,53.7246409278238,16.0411432697963));
#67946=CARTESIAN_POINT('Ctrl Pts',(15.4810192232586,52.0526463245539,15.9626377594195));
#67947=CARTESIAN_POINT('Ctrl Pts',(13.8620496912558,51.4696294241944,15.8841322490427));
#67948=CARTESIAN_POINT('Ctrl Pts',(12.4827412493343,52.4984536423944,15.8056267386659));
#67949=CARTESIAN_POINT('Ctrl Pts',(12.5800904986591,54.2164449634099,15.7271212282891));
#67950=CARTESIAN_POINT('Ctrl Pts',(14.0667923195219,55.0828679235634,15.6486157179124));
#67951=CARTESIAN_POINT('Ctrl Pts',(15.6095371717915,54.3206938223985,15.5701102075356));
#67952=CARTESIAN_POINT('Ctrl Pts',(15.8247548010729,52.6134584968728,15.4916046971588));
#67953=CARTESIAN_POINT('Ctrl Pts',(14.5194329092597,51.4922512076563,15.413099186782));
#67954=CARTESIAN_POINT('Ctrl Pts',(12.864215224715,51.9625972391947,15.3345936764052));
#67955=CARTESIAN_POINT('Ctrl Pts',(12.343540269987,53.6026792252177,15.2560881660285));
#67956=CARTESIAN_POINT('Ctrl Pts',(13.4243618186884,54.9416323741225,15.1775826556517));
#67957=CARTESIAN_POINT('Ctrl Pts',(15.1373732173661,54.7786522269087,15.0990771452749));
#67958=CARTESIAN_POINT('Ctrl Pts',(15.9463055097723,53.2599021305098,15.0205716348981));
#67959=CARTESIAN_POINT('Ctrl Pts',(15.1256881964072,51.7474355457531,14.9420661245214));
#67960=CARTESIAN_POINT('Ctrl Pts',(13.4114719843064,51.5976638845367,14.8635606141446));
#67961=CARTESIAN_POINT('Ctrl Pts',(12.3410035135938,52.9449151739745,14.7850551037678));
#67962=CARTESIAN_POINT('Ctrl Pts',(12.8743108410601,54.5809237767911,14.706549593391));
#67963=CARTESIAN_POINT('Ctrl Pts',(14.53309819057,55.0385159317414,14.6280440830142));
#67964=CARTESIAN_POINT('Ctrl Pts',(15.8297520454146,53.9072361260964,14.5495385726375));
#67965=CARTESIAN_POINT('Ctrl Pts',(15.6013490876951,52.2017963646938,14.4710330622607));
#67966=CARTESIAN_POINT('Ctrl Pts',(14.0528341340627,51.4513659790234,14.3925275518839));
#67967=CARTESIAN_POINT('Ctrl Pts',(12.572734971243,52.3295736939085,14.3140220415071));
#67968=CARTESIAN_POINT('Ctrl Pts',(12.4888785260391,54.0475602728967,14.2355165311303));
#67969=CARTESIAN_POINT('Ctrl Pts',(13.875577901283,55.0671461874891,14.1570110207536));
#67970=CARTESIAN_POINT('Ctrl Pts',(15.4910603626305,54.4687297322861,14.0785055103768));
#67971=CARTESIAN_POINT('Ctrl Pts',(15.7510836294753,53.3567463262428,14.0261685034589));
#67972=CARTESIAN_POINT('Ctrl Pts',(15.6194800884629,52.8667052421829,14.));
#67973=CARTESIAN_POINT('Ctrl Pts',(13.498190246218,52.1716844371558,17.1934196736194));
#67974=CARTESIAN_POINT('Ctrl Pts',(13.5965228772488,52.1138086750997,17.2005947478237));
#67975=CARTESIAN_POINT('Ctrl Pts',(13.7022352452507,52.0691825768203,17.2077698220279));
#67976=CARTESIAN_POINT('Ctrl Pts',(13.8121375241322,52.0407561835157,17.2149448962322));
#67977=CARTESIAN_POINT('Ctrl Pts',(14.2129665724708,51.9370811342635,17.2411133996911));
#67978=CARTESIAN_POINT('Ctrl Pts',(14.6695282799807,52.0488886243742,17.2672819031501));
#67979=CARTESIAN_POINT('Ctrl Pts',(14.9770999437494,52.3260406788269,17.293450406609));
#67980=CARTESIAN_POINT('Ctrl Pts',(15.284671607518,52.6031927332796,17.3196189100679));
#67981=CARTESIAN_POINT('Ctrl Pts',(15.4432532275454,53.0456893520743,17.3457874135268));
#67982=CARTESIAN_POINT('Ctrl Pts',(15.3817248406863,53.4551141662759,17.3719559169858));
#67983=CARTESIAN_POINT('Ctrl Pts',(15.3201964538272,53.8645389804775,17.3981244204447));
#67984=CARTESIAN_POINT('Ctrl Pts',(15.0385580600817,54.240891990086,17.4242929239036));
#67985=CARTESIAN_POINT('Ctrl Pts',(14.6631200082692,54.4154032016409,17.4504614273625));
#67986=CARTESIAN_POINT('Ctrl Pts',(14.2876819564568,54.5899144131957,17.4766299308215));
#67987=CARTESIAN_POINT('Ctrl Pts',(13.8184442465774,54.5625838266969,17.5027984342804));
#67988=CARTESIAN_POINT('Ctrl Pts',(13.4657775795433,54.3456846257064,17.5289669377393));
#67989=CARTESIAN_POINT('Ctrl Pts',(13.1131109125092,54.1287854247159,17.5551354411982));
#67990=CARTESIAN_POINT('Ctrl Pts',(12.8770152883204,53.7223176092336,17.5813039446572));
#67991=CARTESIAN_POINT('Ctrl Pts',(12.8634416833823,53.3085101996499,17.6074724481161));
#67992=CARTESIAN_POINT('Ctrl Pts',(12.8498680784442,52.8947027900662,17.633640951575));
#67993=CARTESIAN_POINT('Ctrl Pts',(13.0588164927569,52.4735557863811,17.659809455034));
#67994=CARTESIAN_POINT('Ctrl Pts',(13.3964246197054,52.2339891821746,17.6859779584929));
#67995=CARTESIAN_POINT('Ctrl Pts',(13.4284272586679,52.2112801211956,17.6884585302017));
#67996=CARTESIAN_POINT('Ctrl Pts',(13.46158597893,52.1902026642355,17.6909391019106));
#67997=CARTESIAN_POINT('Ctrl Pts',(13.4957229821349,52.1707788329429,17.6934196736194));
#67998=CARTESIAN_POINT('Ctrl Pts',(15.2209662466057,52.1764590205668,18.));
#67999=CARTESIAN_POINT('Ctrl Pts',(14.8623799894179,51.8174664687922,17.9738314965411));
#68000=CARTESIAN_POINT('Ctrl Pts',(13.7693646387388,51.4866597864568,17.9214944896232));
#68001=CARTESIAN_POINT('Ctrl Pts',(12.4433767107148,52.5865029592797,17.8429889792465));
#68002=CARTESIAN_POINT('Ctrl Pts',(12.6330157688953,54.2972115132025,17.7644834688697));
#68003=CARTESIAN_POINT('Ctrl Pts',(14.1627629159667,55.0835833760401,17.6859779584929));
#68004=CARTESIAN_POINT('Ctrl Pts',(15.6633630152513,54.2408836460551,17.6074724481161));
#68005=CARTESIAN_POINT('Ctrl Pts',(15.7877283921754,52.5246154983423,17.5289669377393));
#68006=CARTESIAN_POINT('Ctrl Pts',(14.4249760687642,51.474092947767,17.4504614273626));
#68007=CARTESIAN_POINT('Ctrl Pts',(12.7969322124135,52.031388169684,17.3719559169858));
#68008=CARTESIAN_POINT('Ctrl Pts',(12.3638250796578,53.6967359986949,17.293450406609));
#68009=CARTESIAN_POINT('Ctrl Pts',(13.5139962436502,54.9765978264215,17.2149448962322));
#68010=CARTESIAN_POINT('Ctrl Pts',(15.2159841085891,54.7231706136823,17.1364393858554));
#68011=CARTESIAN_POINT('Ctrl Pts',(15.9433860453712,53.1637302055401,17.0579338754786));
#68012=CARTESIAN_POINT('Ctrl Pts',(15.043860342301,51.6968216692226,16.9794283651019));
#68013=CARTESIAN_POINT('Ctrl Pts',(13.3241182586501,51.6380025442004,16.9009228547251));
#68014=CARTESIAN_POINT('Ctrl Pts',(12.3264677464456,53.0400236709192,16.8224173443483));
#68015=CARTESIAN_POINT('Ctrl Pts',(12.9456243299004,54.6455189484075,16.7439118339715));
#68016=CARTESIAN_POINT('Ctrl Pts',(14.6263142466089,55.0146421540478,16.6654063235947));
#68017=CARTESIAN_POINT('Ctrl Pts',(15.8612545351151,53.8163547667627,16.586900813218));
#68018=CARTESIAN_POINT('Ctrl Pts',(15.5429215283993,52.1253094303059,16.5083953028412));
#68019=CARTESIAN_POINT('Ctrl Pts',(13.9568037640838,51.4580757912425,16.4298897924644));
#68020=CARTESIAN_POINT('Ctrl Pts',(12.5253693960519,52.413044846331,16.3513842820876));
#68021=CARTESIAN_POINT('Ctrl Pts',(12.5323627785853,54.1337776405724,16.2728787717109));
#68022=CARTESIAN_POINT('Ctrl Pts',(13.9715120885841,55.0770800976453,16.1943732613341));
#68023=CARTESIAN_POINT('Ctrl Pts',(15.5521540067467,54.3969761475115,16.1158677509573));
#68024=CARTESIAN_POINT('Ctrl Pts',(15.8567312853937,52.7033991815805,16.0373622405805));
#68025=CARTESIAN_POINT('Ctrl Pts',(14.612091779025,51.5151892852256,15.9588567302038));
#68026=CARTESIAN_POINT('Ctrl Pts',(12.934457787186,51.8979613415929,15.8803512198269));
#68027=CARTESIAN_POINT('Ctrl Pts',(12.3283713567551,53.5084362707541,15.8018457094502));
#68028=CARTESIAN_POINT('Ctrl Pts',(13.3373852079753,54.9023018690978,15.7233401990734));
#68029=CARTESIAN_POINT('Ctrl Pts',(15.0565917302206,54.8295063313936,15.6448346886966));
#68030=CARTESIAN_POINT('Ctrl Pts',(15.9441656443073,53.3553344251959,15.5663291783198));
#68031=CARTESIAN_POINT('Ctrl Pts',(15.2041095597138,51.8018585649929,15.4878236679431));
#68032=CARTESIAN_POINT('Ctrl Pts',(13.5001233739826,51.5622728287798,15.4093181575663));
#68033=CARTESIAN_POINT('Ctrl Pts',(12.3603823942099,52.8514434111319,15.3308126471895));
#68034=CARTESIAN_POINT('Ctrl Pts',(12.8070334555363,54.5132114643008,15.2523071368127));
#68035=CARTESIAN_POINT('Ctrl Pts',(14.4395092097517,55.0572639347494,15.1738016264359));
#68036=CARTESIAN_POINT('Ctrl Pts',(15.7937667074068,53.9956815464663,15.0952961160592));
#68037=CARTESIAN_POINT('Ctrl Pts',(15.6552753932384,52.2805167973031,15.0167906056824));
#68038=CARTESIAN_POINT('Ctrl Pts',(14.14823804594,51.4499698581624,14.9382850953056));
#68039=CARTESIAN_POINT('Ctrl Pts',(12.6242006263839,52.248895679213,14.8597795849288));
#68040=CARTESIAN_POINT('Ctrl Pts',(12.4499580614657,53.9607971579715,14.781274074552));
#68041=CARTESIAN_POINT('Ctrl Pts',(13.7817713167743,55.0504032414556,14.7027685641753));
#68042=CARTESIAN_POINT('Ctrl Pts',(15.4252464910755,54.5405234556122,14.6242630537985));
#68043=CARTESIAN_POINT('Ctrl Pts',(15.9064600587523,52.8884418877606,14.5457575434217));
#68044=CARTESIAN_POINT('Ctrl Pts',(14.7938803736306,51.575760805285,14.4672520330449));
#68045=CARTESIAN_POINT('Ctrl Pts',(13.0852305278661,51.7797717538672,14.3887465226681));
#68046=CARTESIAN_POINT('Ctrl Pts',(12.312999126503,53.317416116839,14.3102410122914));
#68047=CARTESIAN_POINT('Ctrl Pts',(13.1694776941512,54.809893106608,14.2317355019146));
#68048=CARTESIAN_POINT('Ctrl Pts',(14.8870885705587,54.9183199028175,14.1532299915378));
#68049=CARTESIAN_POINT('Ctrl Pts',(15.9243621047064,53.5462518811827,14.074724481161));
#68050=CARTESIAN_POINT('Ctrl Pts',(15.3532243372684,51.9225867742538,13.9962189707842));
#68051=CARTESIAN_POINT('Ctrl Pts',(13.6814109435091,51.5067274632874,13.9177134604075));
#68052=CARTESIAN_POINT('Ctrl Pts',(12.8400499397792,52.278885011525,13.8653764534896));
#68053=CARTESIAN_POINT('Ctrl Pts',(12.6726615784997,52.7578848993974,13.8392079500307));
#68054=CARTESIAN_POINT('Ctrl Pts',(15.1552860103679,52.2420649223251,18.0535973499898));
#68055=CARTESIAN_POINT('Ctrl Pts',(14.8182738021381,51.9046708638902,18.0274288465308));
#68056=CARTESIAN_POINT('Ctrl Pts',(13.7910188263055,51.5937668951064,17.975091839613));
#68057=CARTESIAN_POINT('Ctrl Pts',(12.5448078777489,52.6274389027465,17.8965863292362));
#68058=CARTESIAN_POINT('Ctrl Pts',(12.7230374570564,54.2352240753196,17.8180808188594));
#68059=CARTESIAN_POINT('Ctrl Pts',(14.1607486178545,54.9742845180234,17.7395753084826));
#68060=CARTESIAN_POINT('Ctrl Pts',(15.5710663391631,54.1822851282415,17.6610697981059));
#68061=CARTESIAN_POINT('Ctrl Pts',(15.6879493748746,52.5692748502929,17.5825642877291));
#68062=CARTESIAN_POINT('Ctrl Pts',(14.407185930718,51.5819561299908,17.5040587773523));
#68063=CARTESIAN_POINT('Ctrl Pts',(12.8770920017801,52.1057221405655,17.4255532669755));
#68064=CARTESIAN_POINT('Ctrl Pts',(12.4700424055274,53.6708756791509,17.3470477565988));
#68065=CARTESIAN_POINT('Ctrl Pts',(13.5510144619001,54.8737356665185,17.268542246222));
#68066=CARTESIAN_POINT('Ctrl Pts',(15.1506036186114,54.6355556948135,17.1900367358452));
#68067=CARTESIAN_POINT('Ctrl Pts',(15.8342420126426,53.1699377437178,17.1115312254684));
#68068=CARTESIAN_POINT('Ctrl Pts',(14.9888355379813,51.791284560039,17.0330257150916));
#68069=CARTESIAN_POINT('Ctrl Pts',(13.3725603306097,51.736004239579,16.9545202047149));
#68070=CARTESIAN_POINT('Ctrl Pts',(12.4349326457219,53.0536739116011,16.876014694338));
#68071=CARTESIAN_POINT('Ctrl Pts',(13.0168381795996,54.5625758784866,16.7975091839613));
#68072=CARTESIAN_POINT('Ctrl Pts',(14.5964107617212,54.9094910882809,16.7190036735845));
#68073=CARTESIAN_POINT('Ctrl Pts',(15.7570518775444,53.7832976818467,16.6404981632077));
#68074=CARTESIAN_POINT('Ctrl Pts',(15.457871115886,52.1939927053388,16.561992652831));
#68075=CARTESIAN_POINT('Ctrl Pts',(13.9671808299377,51.5669026325918,16.4834871424542));
#68076=CARTESIAN_POINT('Ctrl Pts',(12.6218675402158,52.4644167553317,16.4049816320774));
#68077=CARTESIAN_POINT('Ctrl Pts',(12.6284401716074,54.0816230680013,16.3264761217006));
#68078=CARTESIAN_POINT('Ctrl Pts',(13.981004240121,54.9681725040555,16.2479706113238));
#68079=CARTESIAN_POINT('Ctrl Pts',(15.4665481297227,54.3289864519802,16.1694651009471));
#68080=CARTESIAN_POINT('Ctrl Pts',(15.752800765444,52.7373021594152,16.0909595905703));
#68081=CARTESIAN_POINT('Ctrl Pts',(14.5830439772701,51.6205799399096,16.0124540801935));
#68082=CARTESIAN_POINT('Ctrl Pts',(13.0063434627971,51.9803228284871,15.9339485698167));
#68083=CARTESIAN_POINT('Ctrl Pts',(12.4367217268737,53.4939048503744,15.85544305944));
#68084=CARTESIAN_POINT('Ctrl Pts',(13.3850290847768,54.8039096647175,15.7769375490631));
#68085=CARTESIAN_POINT('Ctrl Pts',(15.0008009523568,54.7354938110165,15.6984320386864));
#68086=CARTESIAN_POINT('Ctrl Pts',(15.8349747076461,53.3500142521672,15.6199265283096));
#68087=CARTESIAN_POINT('Ctrl Pts',(15.1394434922597,51.8900019968609,15.5414210179329));
#68088=CARTESIAN_POINT('Ctrl Pts',(13.5379762420926,51.6648307405647,15.462915507556));
#68089=CARTESIAN_POINT('Ctrl Pts',(12.4668068464345,52.8764394289472,15.3844099971793));
#68090=CARTESIAN_POINT('Ctrl Pts',(12.8865855118699,54.4382285659771,15.3059044868025));
#68091=CARTESIAN_POINT('Ctrl Pts',(14.4208446971613,54.9495485643971,15.2273989764257));
#68092=CARTESIAN_POINT('Ctrl Pts',(15.6936243998074,53.9518354124798,15.1488934660489));
#68093=CARTESIAN_POINT('Ctrl Pts',(15.5634653023155,52.3398621480091,15.0703879556721));
#68094=CARTESIAN_POINT('Ctrl Pts',(14.1470976247563,51.5592843863476,14.9918824452954));
#68095=CARTESIAN_POINT('Ctrl Pts',(12.7147526703863,52.3101434886333,14.9133769349186));
#68096=CARTESIAN_POINT('Ctrl Pts',(12.5509932669133,53.9190498146948,14.8348714245418));
#68097=CARTESIAN_POINT('Ctrl Pts',(13.8026790667016,54.9431006391056,14.756365914165));
#68098=CARTESIAN_POINT('Ctrl Pts',(15.3472759009633,54.4638973536635,14.6778604037883));
#68099=CARTESIAN_POINT('Ctrl Pts',(15.7995376478153,52.9112119224821,14.5993548934115));
#68100=CARTESIAN_POINT('Ctrl Pts',(14.7538954097245,51.6775072239921,14.5208493830347));
#68101=CARTESIAN_POINT('Ctrl Pts',(13.1480450848167,51.8692440206669,14.4423438726579));
#68102=CARTESIAN_POINT('Ctrl Pts',(12.4222743542852,53.3143772678278,14.3638383622811));
#68103=CARTESIAN_POINT('Ctrl Pts',(13.2272235892287,54.7170605998631,14.2853328519043));
#68104=CARTESIAN_POINT('Ctrl Pts',(14.8414958116982,54.8189639865359,14.2068273415276));
#68105=CARTESIAN_POINT('Ctrl Pts',(15.8163626318126,53.5294453155223,14.1283218311508));
#68106=CARTESIAN_POINT('Ctrl Pts',(15.2795869011495,52.0034666921275,14.049816320774));
#68107=CARTESIAN_POINT('Ctrl Pts',(13.7083567932321,51.6126272165693,13.9713108103972));
#68108=CARTESIAN_POINT('Ctrl Pts',(12.9176155863349,52.3383285372882,13.9189738034794));
#68109=CARTESIAN_POINT('Ctrl Pts',(12.7602980089432,52.7885097885712,13.8928053000205));
#68110=CARTESIAN_POINT('Ctrl Pts',(15.0896057741301,52.3076708240835,18.1071946999795));
#68111=CARTESIAN_POINT('Ctrl Pts',(14.7741676148584,51.9918752589882,18.0810261965206));
#68112=CARTESIAN_POINT('Ctrl Pts',(13.8126730138722,51.700874003756,18.0286891896027));
#68113=CARTESIAN_POINT('Ctrl Pts',(12.646239044783,52.6683748462133,17.950183679226));
#68114=CARTESIAN_POINT('Ctrl Pts',(12.8130591452175,54.1732366374368,17.8716781688492));
#68115=CARTESIAN_POINT('Ctrl Pts',(14.1587343197422,54.8649856600065,17.7931726584724));
#68116=CARTESIAN_POINT('Ctrl Pts',(15.4787696630748,54.123686610428,17.7146671480956));
#68117=CARTESIAN_POINT('Ctrl Pts',(15.5881703575737,52.6139342022434,17.6361616377189));
#68118=CARTESIAN_POINT('Ctrl Pts',(14.3893957926718,51.6898193122148,17.5576561273421));
#68119=CARTESIAN_POINT('Ctrl Pts',(12.9572517911467,52.1800561114469,17.4791506169653));
#68120=CARTESIAN_POINT('Ctrl Pts',(12.576259731397,53.6450153596069,17.4006451065885));
#68121=CARTESIAN_POINT('Ctrl Pts',(13.5880326801499,54.7708735066155,17.3221395962118));
#68122=CARTESIAN_POINT('Ctrl Pts',(15.0852231286336,54.5479407759449,17.243634085835));
#68123=CARTESIAN_POINT('Ctrl Pts',(15.725097979914,53.1761452818955,17.1651285754582));
#68124=CARTESIAN_POINT('Ctrl Pts',(14.9338107336616,51.8857474508553,17.0866230650814));
#68125=CARTESIAN_POINT('Ctrl Pts',(13.4210024025693,51.8340059349576,17.0081175547046));
#68126=CARTESIAN_POINT('Ctrl Pts',(12.5433975449982,53.0673241522829,16.9296120443278));
#68127=CARTESIAN_POINT('Ctrl Pts',(13.0880520292989,54.4796328085656,16.8511065339511));
#68128=CARTESIAN_POINT('Ctrl Pts',(14.5665072768334,54.804340022514,16.7726010235743));
#68129=CARTESIAN_POINT('Ctrl Pts',(15.6528492199738,53.7502405969307,16.6940955131975));
#68130=CARTESIAN_POINT('Ctrl Pts',(15.3728207033727,52.2626759803717,16.6155900028207));
#68131=CARTESIAN_POINT('Ctrl Pts',(13.9775578957916,51.6757294739412,16.5370844924439));
#68132=CARTESIAN_POINT('Ctrl Pts',(12.7183656843797,52.5157886643324,16.4585789820672));
#68133=CARTESIAN_POINT('Ctrl Pts',(12.7245175646294,54.0294684954301,16.3800734716904));
#68134=CARTESIAN_POINT('Ctrl Pts',(13.990496391658,54.8592649104658,16.3015679613136));
#68135=CARTESIAN_POINT('Ctrl Pts',(15.3809422526988,54.2609967564488,16.2230624509369));
#68136=CARTESIAN_POINT('Ctrl Pts',(15.6488702454943,52.77120513725,16.14455694056));
#68137=CARTESIAN_POINT('Ctrl Pts',(14.5539961755152,51.7259705945935,16.0660514301833));
#68138=CARTESIAN_POINT('Ctrl Pts',(13.0782291384082,52.0626843153815,15.9875459198065));
#68139=CARTESIAN_POINT('Ctrl Pts',(12.5450720969922,53.4793734299947,15.9090404094297));
#68140=CARTESIAN_POINT('Ctrl Pts',(13.4326729615782,54.7055174603372,15.8305348990529));
#68141=CARTESIAN_POINT('Ctrl Pts',(14.9450101744931,54.6414812906394,15.7520293886762));
#68142=CARTESIAN_POINT('Ctrl Pts',(15.7257837709849,53.3446940791385,15.6735238782994));
#68143=CARTESIAN_POINT('Ctrl Pts',(15.0747774248056,51.9781454287288,15.5950183679226));
#68144=CARTESIAN_POINT('Ctrl Pts',(13.5758291102025,51.7673886523496,15.5165128575458));
#68145=CARTESIAN_POINT('Ctrl Pts',(12.5732312986591,52.9014354467625,15.438007347169));
#68146=CARTESIAN_POINT('Ctrl Pts',(12.9661375682035,54.3632456676534,15.3595018367923));
#68147=CARTESIAN_POINT('Ctrl Pts',(14.402180184571,54.841833194045,15.2809963264155));
#68148=CARTESIAN_POINT('Ctrl Pts',(15.593482092208,53.9079892784933,15.2024908160387));
#68149=CARTESIAN_POINT('Ctrl Pts',(15.4716552113927,52.3992074987152,15.1239853056619));
#68150=CARTESIAN_POINT('Ctrl Pts',(14.1459572035726,51.6685989145327,15.0454797952851));
#68151=CARTESIAN_POINT('Ctrl Pts',(12.8053047143887,52.3713912980536,14.9669742849084));
#68152=CARTESIAN_POINT('Ctrl Pts',(12.6520284723608,53.8773024714181,14.8884687745316));
#68153=CARTESIAN_POINT('Ctrl Pts',(13.8235868166289,54.8357980367556,14.8099632641548));
#68154=CARTESIAN_POINT('Ctrl Pts',(15.269305310851,54.3872712517148,14.731457753778));
#68155=CARTESIAN_POINT('Ctrl Pts',(15.6926152368783,52.9339819572036,14.6529522434012));
#68156=CARTESIAN_POINT('Ctrl Pts',(14.7139104458185,51.7792536426993,14.5744467330245));
#68157=CARTESIAN_POINT('Ctrl Pts',(13.2108596417673,51.9587162874664,14.4959412226477));
#68158=CARTESIAN_POINT('Ctrl Pts',(12.5315495820674,53.3113384188168,14.4174357122709));
#68159=CARTESIAN_POINT('Ctrl Pts',(13.2849694843063,54.6242280931179,14.3389302018941));
#68160=CARTESIAN_POINT('Ctrl Pts',(14.7959030528376,54.7196080702544,14.2604246915174));
#68161=CARTESIAN_POINT('Ctrl Pts',(15.7083631589187,53.5126387498619,14.1819191811406));
#68162=CARTESIAN_POINT('Ctrl Pts',(15.2059494650307,52.0843466100013,14.1034136707638));
#68163=CARTESIAN_POINT('Ctrl Pts',(13.7353026429551,51.7185269698512,14.024908160387));
#68164=CARTESIAN_POINT('Ctrl Pts',(12.9951812328907,52.3977720630513,13.9725711534692));
#68165=CARTESIAN_POINT('Ctrl Pts',(12.8479344393867,52.8191346777449,13.9464026500102));
#68166=CARTESIAN_POINT('Ctrl Pts',(15.0239255378924,52.3732767258419,18.1607920499693));
#68167=CARTESIAN_POINT('Ctrl Pts',(14.7300614275787,52.0790796540862,18.1346235465104));
#68168=CARTESIAN_POINT('Ctrl Pts',(13.8343272014389,51.8079811124056,18.0822865395925));
#68169=CARTESIAN_POINT('Ctrl Pts',(12.7476702118172,52.7093107896802,18.0037810292157));
#68170=CARTESIAN_POINT('Ctrl Pts',(12.9030808333786,54.111249199554,17.925275518839));
#68171=CARTESIAN_POINT('Ctrl Pts',(14.1567200216299,54.7556868019897,17.8467700084622));
#68172=CARTESIAN_POINT('Ctrl Pts',(15.3864729869866,54.0650880926144,17.7682644980854));
#68173=CARTESIAN_POINT('Ctrl Pts',(15.4883913402728,52.6585935541939,17.6897589877086));
#68174=CARTESIAN_POINT('Ctrl Pts',(14.3716056546256,51.7976824944386,17.6112534773319));
#68175=CARTESIAN_POINT('Ctrl Pts',(13.0374115805133,52.2543900823284,17.5327479669551));
#68176=CARTESIAN_POINT('Ctrl Pts',(12.6824770572666,53.6191550400629,17.4542424565783));
#68177=CARTESIAN_POINT('Ctrl Pts',(13.6250508983997,54.6680113467124,17.3757369462015));
#68178=CARTESIAN_POINT('Ctrl Pts',(15.0198426386559,54.4603258570762,17.2972314358247));
#68179=CARTESIAN_POINT('Ctrl Pts',(15.6159539471853,53.1823528200731,17.218725925448));
#68180=CARTESIAN_POINT('Ctrl Pts',(14.878785929342,51.9802103416717,17.1402204150712));
#68181=CARTESIAN_POINT('Ctrl Pts',(13.4694444745289,51.9320076303362,17.0617149046944));
#68182=CARTESIAN_POINT('Ctrl Pts',(12.6518624442745,53.0809743929648,16.9832093943176));
#68183=CARTESIAN_POINT('Ctrl Pts',(13.1592658789981,54.3966897386446,16.9047038839409));
#68184=CARTESIAN_POINT('Ctrl Pts',(14.5366037919456,54.6991889567471,16.8261983735641));
#68185=CARTESIAN_POINT('Ctrl Pts',(15.5486465624031,53.7171835120148,16.7476928631873));
#68186=CARTESIAN_POINT('Ctrl Pts',(15.2877702908594,52.3313592554045,16.6691873528105));
#68187=CARTESIAN_POINT('Ctrl Pts',(13.9879349616455,51.7845563152907,16.5906818424337));
#68188=CARTESIAN_POINT('Ctrl Pts',(12.8148638285435,52.567160573333,16.5121763320569));
#68189=CARTESIAN_POINT('Ctrl Pts',(12.8205949576515,53.9773139228589,16.4336708216802));
#68190=CARTESIAN_POINT('Ctrl Pts',(13.9999885431949,54.7503573168761,16.3551653113034));
#68191=CARTESIAN_POINT('Ctrl Pts',(15.2953363756748,54.1930070609175,16.2766598009266));
#68192=CARTESIAN_POINT('Ctrl Pts',(15.5449397255447,52.8051081150848,16.1981542905498));
#68193=CARTESIAN_POINT('Ctrl Pts',(14.5249483737603,51.8313612492774,16.119648780173));
#68194=CARTESIAN_POINT('Ctrl Pts',(13.1501148140193,52.1450458022758,16.0411432697963));
#68195=CARTESIAN_POINT('Ctrl Pts',(12.6534224671108,53.4648420096149,15.9626377594195));
#68196=CARTESIAN_POINT('Ctrl Pts',(13.4803168383797,54.6071252559569,15.8841322490427));
#68197=CARTESIAN_POINT('Ctrl Pts',(14.8892193966293,54.5474687702622,15.8056267386659));
#68198=CARTESIAN_POINT('Ctrl Pts',(15.6165928343238,53.3393739061099,15.7271212282891));
#68199=CARTESIAN_POINT('Ctrl Pts',(15.0101113573514,52.0662888605968,15.6486157179124));
#68200=CARTESIAN_POINT('Ctrl Pts',(13.6136819783124,51.8699465641344,15.5701102075356));
#68201=CARTESIAN_POINT('Ctrl Pts',(12.6796557508836,52.9264314645779,15.4916046971588));
#68202=CARTESIAN_POINT('Ctrl Pts',(13.0456896245371,54.2882627693297,15.413099186782));
#68203=CARTESIAN_POINT('Ctrl Pts',(14.3835156719806,54.7341178236928,15.3345936764053));
#68204=CARTESIAN_POINT('Ctrl Pts',(15.4933397846085,53.8641431445068,15.2560881660285));
#68205=CARTESIAN_POINT('Ctrl Pts',(15.3798451204699,52.4585528494213,15.1775826556517));
#68206=CARTESIAN_POINT('Ctrl Pts',(14.1448167823889,51.7779134427179,15.0990771452749));
#68207=CARTESIAN_POINT('Ctrl Pts',(12.8958567583911,52.4326391074739,15.0205716348981));
#68208=CARTESIAN_POINT('Ctrl Pts',(12.7530636778084,53.8355551281415,14.9420661245213));
#68209=CARTESIAN_POINT('Ctrl Pts',(13.8444945665562,54.7284954344056,14.8635606141446));
#68210=CARTESIAN_POINT('Ctrl Pts',(15.1913347207388,54.3106451497661,14.7850551037678));
#68211=CARTESIAN_POINT('Ctrl Pts',(15.5856928259413,52.9567519919252,14.706549593391));
#68212=CARTESIAN_POINT('Ctrl Pts',(14.6739254819125,51.8810000614065,14.6280440830142));
#68213=CARTESIAN_POINT('Ctrl Pts',(13.2736741987179,52.048188554266,14.5495385726375));
#68214=CARTESIAN_POINT('Ctrl Pts',(12.6408248098497,53.3082995698058,14.4710330622607));
#68215=CARTESIAN_POINT('Ctrl Pts',(13.3427153793838,54.5313955863728,14.3925275518839));
#68216=CARTESIAN_POINT('Ctrl Pts',(14.750310293977,54.6202521539728,14.3140220415071));
#68217=CARTESIAN_POINT('Ctrl Pts',(15.6003636860248,53.4958321842015,14.2355165311303));
#68218=CARTESIAN_POINT('Ctrl Pts',(15.1323120289118,52.1652265278751,14.1570110207536));
#68219=CARTESIAN_POINT('Ctrl Pts',(13.7622484926781,51.824426723133,14.0785055103768));
#68220=CARTESIAN_POINT('Ctrl Pts',(13.0727468794464,52.4572155888145,14.0261685034589));
#68221=CARTESIAN_POINT('Ctrl Pts',(12.9355708698302,52.8497595669186,14.));
#68222=CARTESIAN_POINT('Ctrl Pts',(13.4965541629804,52.1730078059394,17.5565803263806));
#68223=CARTESIAN_POINT('Ctrl Pts',(13.3865887223467,52.2353622375858,17.5486362065721));
#68224=CARTESIAN_POINT('Ctrl Pts',(13.2860845507673,52.3135738660446,17.5406920867636));
#68225=CARTESIAN_POINT('Ctrl Pts',(13.2006215056575,52.4057329773025,17.5327479669551));
#68226=CARTESIAN_POINT('Ctrl Pts',(12.9191000727644,52.7093117349065,17.5065794634961));
#68227=CARTESIAN_POINT('Ctrl Pts',(12.8007885650155,53.1642333874847,17.4804109600372));
#68228=CARTESIAN_POINT('Ctrl Pts',(12.8987284513299,53.5665035982154,17.4542424565783));
#68229=CARTESIAN_POINT('Ctrl Pts',(12.9966683376443,53.9687738089461,17.4280739531194));
#68230=CARTESIAN_POINT('Ctrl Pts',(13.310859618022,54.3183925778293,17.4019054496604));
#68231=CARTESIAN_POINT('Ctrl Pts',(13.7004205482536,54.4585877139982,17.3757369462015));
#68232=CARTESIAN_POINT('Ctrl Pts',(14.0899814784851,54.598782850167,17.3495684427426));
#68233=CARTESIAN_POINT('Ctrl Pts',(14.5549120585705,54.5295543536216,17.3233999392837));
#68234=CARTESIAN_POINT('Ctrl Pts',(14.8867292333681,54.2819445991817,17.2972314358247));
#68235=CARTESIAN_POINT('Ctrl Pts',(15.2185464081657,54.0343348447418,17.2710629323658));
#68236=CARTESIAN_POINT('Ctrl Pts',(15.4172501776755,53.6083438324075,17.2448944289069));
#68237=CARTESIAN_POINT('Ctrl Pts',(15.3937407261232,53.1949912465067,17.2187259254479));
#68238=CARTESIAN_POINT('Ctrl Pts',(15.3702312745709,52.7816386606059,17.192557421989));
#68239=CARTESIAN_POINT('Ctrl Pts',(15.1245086019564,52.3809245011388,17.1663889185301));
#68240=CARTESIAN_POINT('Ctrl Pts',(14.7667570231804,52.1725336361826,17.1402204150712));
#68241=CARTESIAN_POINT('Ctrl Pts',(14.4090054444043,51.9641427712265,17.1140519116122));
#68242=CARTESIAN_POINT('Ctrl Pts',(13.9392249594666,51.9480752007813,17.0878834081533));
#68243=CARTESIAN_POINT('Ctrl Pts',(13.5680710452887,52.1315358759968,17.0617149046944));
#68244=CARTESIAN_POINT('Ctrl Pts',(13.5437960761855,52.1435349471433,17.0600033785898));
#68245=CARTESIAN_POINT('Ctrl Pts',(13.5199430009518,52.1563875382183,17.0582918524852));
#68246=CARTESIAN_POINT('Ctrl Pts',(13.4965460097018,52.1700456009992,17.0565803263806));
#68247=CARTESIAN_POINT('Origin',(14.1292828945603,53.2669068454841,15.5));
#68248=CARTESIAN_POINT('Origin',(39.0658530619283,-38.8697713466883,13.));
#68249=CARTESIAN_POINT('',(39.0658530619283,-38.8697713466882,13.));
#68250=CARTESIAN_POINT('Origin',(39.0658530619283,-38.8697713466883,13.));
#68251=CARTESIAN_POINT('',(39.0658530619283,-38.8697713466882,13.));
#68252=CARTESIAN_POINT('Origin',(-14.1292828945604,-53.2669068454841,13.));
#68253=CARTESIAN_POINT('',(-14.1292828945603,-53.2669068454841,13.));
#68254=CARTESIAN_POINT('Origin',(-14.1292828945604,-53.2669068454841,13.));
#68255=CARTESIAN_POINT('',(-14.1292828945603,-53.2669068454841,13.));
#68256=CARTESIAN_POINT('Origin',(-53.1951359564886,-14.3971354987959,13.));
#68257=CARTESIAN_POINT('',(-53.1951359564886,-14.3971354987959,13.));
#68258=CARTESIAN_POINT('Origin',(-53.1951359564886,-14.3971354987959,13.));
#68259=CARTESIAN_POINT('',(-53.1951359564886,-14.3971354987959,13.));
#68260=CARTESIAN_POINT('Origin',(-39.0658530619283,38.8697713466882,13.));
#68261=CARTESIAN_POINT('',(-39.0658530619283,38.8697713466882,13.));
#68262=CARTESIAN_POINT('Origin',(-39.0658530619283,38.8697713466882,13.));
#68263=CARTESIAN_POINT('',(-39.0658530619283,38.8697713466882,13.));
#68264=CARTESIAN_POINT('Origin',(14.1292828945603,53.2669068454841,13.));
#68265=CARTESIAN_POINT('',(14.1292828945603,53.2669068454841,13.));
#68266=CARTESIAN_POINT('Origin',(14.1292828945603,53.2669068454841,13.));
#68267=CARTESIAN_POINT('',(14.1292828945603,53.2669068454841,13.));
#68268=CARTESIAN_POINT('Origin',(53.1951359564886,14.3971354987959,6.));
#68269=CARTESIAN_POINT('Ctrl Pts',(54.153252109211,15.2223467977324,6.));
#68270=CARTESIAN_POINT('Ctrl Pts',(54.1904452248552,15.1876133706834,6.));
#68271=CARTESIAN_POINT('Ctrl Pts',(54.2252563920727,15.1505690966098,6.));
#68272=CARTESIAN_POINT('Ctrl Pts',(54.2576712403435,15.1115269977852,6.));
#68273=CARTESIAN_POINT('Ctrl Pts',(54.2795176350337,15.08521408423,6.));
#68274=CARTESIAN_POINT('Ctrl Pts',(54.3002751129807,15.0579926438161,6.));
#68275=CARTESIAN_POINT('Ctrl Pts',(54.3199324346534,15.0299477423818,6.));
#68276=CARTESIAN_POINT('Ctrl Pts',(54.3290141536083,15.0169909460702,6.));
#68277=CARTESIAN_POINT('Ctrl Pts',(54.3378609651789,15.0038582769416,6.));
#68278=CARTESIAN_POINT('Ctrl Pts',(54.346471305624,14.9905576089646,6.));
#68279=CARTESIAN_POINT('Ctrl Pts',(54.3536893844502,14.9794076119916,6.));
#68280=CARTESIAN_POINT('Ctrl Pts',(54.3607371493116,14.9681457925481,6.));
#68281=CARTESIAN_POINT('Ctrl Pts',(54.3676105396587,14.9567832872257,6.));
#68282=CARTESIAN_POINT('Ctrl Pts',(54.395433097869,14.9107893963246,6.));
#68283=CARTESIAN_POINT('Ctrl Pts',(54.4204206822113,14.8631190274542,6.));
#68284=CARTESIAN_POINT('Ctrl Pts',(54.4425345345286,14.8140965425426,6.));
#68285=CARTESIAN_POINT('Ctrl Pts',(54.4509995916132,14.7953310137123,6.));
#68286=CARTESIAN_POINT('Ctrl Pts',(54.4590431896973,14.7763669365288,6.));
#68287=CARTESIAN_POINT('Ctrl Pts',(54.4666617056761,14.7572211103019,6.));
#68288=CARTESIAN_POINT('Ctrl Pts',(54.472141946642,14.7434489082736,6.));
#68289=CARTESIAN_POINT('Ctrl Pts',(54.4774022167645,14.7295826470911,6.));
#68290=CARTESIAN_POINT('Ctrl Pts',(54.4824408846806,14.7156283853978,6.));
#68291=CARTESIAN_POINT('Ctrl Pts',(54.4863313548671,14.7048539823218,6.));
#68292=CARTESIAN_POINT('Ctrl Pts',(54.4900897012419,14.6940267513306,6.));
#68293=CARTESIAN_POINT('Ctrl Pts',(54.4937105016155,14.6831642693743,6.));
#68294=CARTESIAN_POINT('Ctrl Pts',(54.5116283443036,14.6294103412881,6.));
#68295=CARTESIAN_POINT('Ctrl Pts',(54.5262131829647,14.5747104062488,6.));
#68296=CARTESIAN_POINT('Ctrl Pts',(54.5374265846686,14.5194236084943,6.));
#68297=CARTESIAN_POINT('Ctrl Pts',(54.5484779141318,14.464935895213,6.));
#68298=CARTESIAN_POINT('Ctrl Pts',(54.556254950168,14.4098769850011,6.));
#68299=CARTESIAN_POINT('Ctrl Pts',(54.5606770668685,14.3545607001755,6.));
#68300=CARTESIAN_POINT('Ctrl Pts',(54.5629861190308,14.3256767525692,6.));
#68301=CARTESIAN_POINT('Ctrl Pts',(54.5643796851138,14.2967222396706,6.));
#68302=CARTESIAN_POINT('Ctrl Pts',(54.564840878929,14.2677401408177,6.));
#68303=CARTESIAN_POINT('Ctrl Pts',(54.5650883530361,14.2521885033157,6.));
#68304=CARTESIAN_POINT('Ctrl Pts',(54.5650672991613,14.2366289098418,6.));
#68305=CARTESIAN_POINT('Ctrl Pts',(54.5647746275356,14.2210679501262,6.));
#68306=CARTESIAN_POINT('Ctrl Pts',(54.5645665072066,14.2100024700117,6.));
#68307=CARTESIAN_POINT('Ctrl Pts',(54.5642210307105,14.1989362983826,6.));
#68308=CARTESIAN_POINT('Ctrl Pts',(54.5637369787284,14.1878718045722,6.));
#68309=CARTESIAN_POINT('Ctrl Pts',(54.5633114560967,14.1781451787148,6.));
#68310=CARTESIAN_POINT('Ctrl Pts',(54.5627792671695,14.1684296794964,6.));
#68311=CARTESIAN_POINT('Ctrl Pts',(54.5621402322824,14.1587275143162,6.));
#68312=CARTESIAN_POINT('Ctrl Pts',(54.5589760897275,14.1106878308172,6.));
#68313=CARTESIAN_POINT('Ctrl Pts',(54.553194193765,14.0629716936048,6.));
#68314=CARTESIAN_POINT('Ctrl Pts',(54.5447557136211,14.0157777529758,6.));
#68315=CARTESIAN_POINT('Ctrl Pts',(54.5351507946179,13.9620602624492,6.));
#68316=CARTESIAN_POINT('Ctrl Pts',(54.522105840848,13.9090185683937,6.));
#68317=CARTESIAN_POINT('Ctrl Pts',(54.505871219518,13.8568507922163,6.));
#68318=CARTESIAN_POINT('Ctrl Pts',(54.4900017008387,13.8058562243927,6.));
#68319=CARTESIAN_POINT('Ctrl Pts',(54.4710837860578,13.7556960236983,6.));
#68320=CARTESIAN_POINT('Ctrl Pts',(54.449305884129,13.7065589745936,6.));
#68321=CARTESIAN_POINT('Ctrl Pts',(54.443973358842,13.6945273033271,6.));
#68322=CARTESIAN_POINT('Ctrl Pts',(54.4384691646966,13.6825570212106,6.));
#68323=CARTESIAN_POINT('Ctrl Pts',(54.432795699503,13.670651006764,6.));
#68324=CARTESIAN_POINT('Ctrl Pts',(54.428510829431,13.6616590198145,6.));
#68325=CARTESIAN_POINT('Ctrl Pts',(54.4241301793592,13.6527055014145,6.));
#68326=CARTESIAN_POINT('Ctrl Pts',(54.4196602351137,13.6438018792426,6.));
#68327=CARTESIAN_POINT('Ctrl Pts',(54.3938099878154,13.5923111173108,6.));
#68328=CARTESIAN_POINT('Ctrl Pts',(54.3649324447401,13.5423928807606,6.));
#68329=CARTESIAN_POINT('Ctrl Pts',(54.3333070254305,13.4942625534384,6.));
#68330=CARTESIAN_POINT('Ctrl Pts',(54.3010028577955,13.4450992475886,6.));
#68331=CARTESIAN_POINT('Ctrl Pts',(54.2658311992691,13.3978004683614,6.));
#68332=CARTESIAN_POINT('Ctrl Pts',(54.2280361919916,13.3526057240142,6.));
#68333=CARTESIAN_POINT('Ctrl Pts',(54.1899071161005,13.3070115050625,6.));
#68334=CARTESIAN_POINT('Ctrl Pts',(54.1491075472284,13.2635576362327,6.));
#68335=CARTESIAN_POINT('Ctrl Pts',(54.1058416126115,13.2225152020132,6.));
#68336=CARTESIAN_POINT('Ctrl Pts',(54.0960379392214,13.2132153539044,6.));
#68337=CARTESIAN_POINT('Ctrl Pts',(54.0861045521762,13.2040370186399,6.));
#68338=CARTESIAN_POINT('Ctrl Pts',(54.0760639794891,13.1950014470312,6.));
#68339=CARTESIAN_POINT('Ctrl Pts',(54.0308409079937,13.1543049336347,6.));
#68340=CARTESIAN_POINT('Ctrl Pts',(53.9833737359527,13.116430352764,6.));
#68341=CARTESIAN_POINT('Ctrl Pts',(53.9339288506769,13.0816212828191,6.));
#68342=CARTESIAN_POINT('Ctrl Pts',(53.8849184369623,13.0471180797172,6.));
#68343=CARTESIAN_POINT('Ctrl Pts',(53.8339641912571,13.0156258220742,6.));
#68344=CARTESIAN_POINT('Ctrl Pts',(53.781283756076,12.9874094818381,6.));
#68345=CARTESIAN_POINT('Ctrl Pts',(53.7426834464002,12.9667346436884,6.));
#68346=CARTESIAN_POINT('Ctrl Pts',(53.7031554637372,12.9478191087148,6.));
#68347=CARTESIAN_POINT('Ctrl Pts',(53.6627743368928,12.9307811146157,6.));
#68348=CARTESIAN_POINT('Ctrl Pts',(53.6403329837275,12.921312442672,6.));
#68349=CARTESIAN_POINT('Ctrl Pts',(53.6176279860555,12.912423887492,6.));
#68350=CARTESIAN_POINT('Ctrl Pts',(53.5946794545979,12.9041113494969,6.));
#68351=CARTESIAN_POINT('Ctrl Pts',(52.7966221146314,12.9064860705774,6.));
#68352=CARTESIAN_POINT('Ctrl Pts',(52.7392734478414,12.9274410373818,6.));
#68353=CARTESIAN_POINT('Ctrl Pts',(52.6834091366923,12.9520243011176,6.));
#68354=CARTESIAN_POINT('Ctrl Pts',(52.6292438196105,12.9799599642101,6.));
#68355=CARTESIAN_POINT('Ctrl Pts',(52.5790178579261,13.0058639119705,6.));
#68356=CARTESIAN_POINT('Ctrl Pts',(52.5302525542226,13.0346514876389,6.));
#68357=CARTESIAN_POINT('Ctrl Pts',(52.4831464368633,13.0661326532235,6.));
#68358=CARTESIAN_POINT('Ctrl Pts',(52.4717767044421,13.0737310809664,6.));
#68359=CARTESIAN_POINT('Ctrl Pts',(52.4605034749784,13.0814868964051,6.));
#68360=CARTESIAN_POINT('Ctrl Pts',(52.4493421044021,13.0893884562265,6.));
#68361=CARTESIAN_POINT('Ctrl Pts',(52.4002195795496,13.1241641646442,6.));
#68362=CARTESIAN_POINT('Ctrl Pts',(52.3531999206732,13.1617999131515,6.));
#68363=CARTESIAN_POINT('Ctrl Pts',(52.3085126015214,13.2020507625132,6.));
#68364=CARTESIAN_POINT('Ctrl Pts',(52.280929942436,13.2268950690618,6.));
#68365=CARTESIAN_POINT('Ctrl Pts',(52.2542366022306,13.2527364020391,6.));
#68366=CARTESIAN_POINT('Ctrl Pts',(52.2284950356621,13.2795223256871,6.));
#68367=CARTESIAN_POINT('Ctrl Pts',(52.2196863977047,13.2886883375202,6.));
#68368=CARTESIAN_POINT('Ctrl Pts',(52.2109892715066,13.2979649848007,6.));
#68369=CARTESIAN_POINT('Ctrl Pts',(52.2024063581496,13.3073502392712,6.));
#68370=CARTESIAN_POINT('Ctrl Pts',(52.1943778466578,13.3161292657201,6.));
#68371=CARTESIAN_POINT('Ctrl Pts',(52.1864544233969,13.3249977565961,6.));
#68372=CARTESIAN_POINT('Ctrl Pts',(52.178641809422,13.3339491348872,6.));
#68373=CARTESIAN_POINT('Ctrl Pts',(52.1399699654117,13.3782577755114,6.));
#68374=CARTESIAN_POINT('Ctrl Pts',(52.1039774129999,13.4246301645838,6.));
#68375=CARTESIAN_POINT('Ctrl Pts',(52.0708793546467,13.4728370625887,6.));
#68376=CARTESIAN_POINT('Ctrl Pts',(52.0386265755808,13.5198128221398,6.));
#68377=CARTESIAN_POINT('Ctrl Pts',(52.0091219665516,13.5685314991462,6.));
#68378=CARTESIAN_POINT('Ctrl Pts',(51.9826103203801,13.6187990638417,6.));
#68379=CARTESIAN_POINT('Ctrl Pts',(51.9682364690781,13.6460526902509,6.));
#68380=CARTESIAN_POINT('Ctrl Pts',(51.9547432274533,13.6737618469323,6.));
#68381=CARTESIAN_POINT('Ctrl Pts',(51.9421760191701,13.7018965350937,6.));
#68382=CARTESIAN_POINT('Ctrl Pts',(51.931720374266,13.72530398584,6.));
#68383=CARTESIAN_POINT('Ctrl Pts',(51.921905793166,13.7490060034822,6.));
#68384=CARTESIAN_POINT('Ctrl Pts',(51.9127610532135,13.7729853083355,6.));
#68385=CARTESIAN_POINT('Ctrl Pts',(51.9088519886793,13.7832356435714,6.));
#68386=CARTESIAN_POINT('Ctrl Pts',(51.9050650272194,13.7935379061066,6.));
#68387=CARTESIAN_POINT('Ctrl Pts',(51.9014081869821,13.8038738000364,6.));
#68388=CARTESIAN_POINT('Ctrl Pts',(51.884480682992,13.8517186262746,6.));
#68389=CARTESIAN_POINT('Ctrl Pts',(51.8703064127051,13.9003649240817,6.));
#68390=CARTESIAN_POINT('Ctrl Pts',(51.8590515016651,13.9496698048621,6.));
#68391=CARTESIAN_POINT('Ctrl Pts',(51.8464743828165,14.0047669391876,6.));
#68392=CARTESIAN_POINT('Ctrl Pts',(51.8375421395455,14.0606874236405,6.));
#68393=CARTESIAN_POINT('Ctrl Pts',(51.8321648228282,14.1170948620919,6.));
#68394=CARTESIAN_POINT('Ctrl Pts',(51.8276016369013,14.1649621614995,6.));
#68395=CARTESIAN_POINT('Ctrl Pts',(51.8255995131662,14.2131805783558,6.));
#68396=CARTESIAN_POINT('Ctrl Pts',(51.8261319285704,14.2615368910685,6.));
#68397=CARTESIAN_POINT('Ctrl Pts',(51.8262783001781,14.2748310053615,6.));
#68398=CARTESIAN_POINT('Ctrl Pts',(51.8266163768542,14.2881354730531,6.));
#68399=CARTESIAN_POINT('Ctrl Pts',(51.8271459227334,14.3014456837622,6.));
#68400=CARTESIAN_POINT('Ctrl Pts',(51.8275582116147,14.3118086232134,6.));
#68401=CARTESIAN_POINT('Ctrl Pts',(51.8280867629365,14.3221768232861,6.));
#68402=CARTESIAN_POINT('Ctrl Pts',(51.8287302146398,14.3325312126212,6.));
#68403=CARTESIAN_POINT('Ctrl Pts',(51.8321732391026,14.3879361724563,6.));
#68404=CARTESIAN_POINT('Ctrl Pts',(51.8389046601923,14.4430495470118,6.));
#68405=CARTESIAN_POINT('Ctrl Pts',(51.8488297362235,14.4975564316795,6.));
#68406=CARTESIAN_POINT('Ctrl Pts',(51.8586992382099,14.551758112836,6.));
#68407=CARTESIAN_POINT('Ctrl Pts',(51.8717272178009,14.6053611705282,6.));
#68408=CARTESIAN_POINT('Ctrl Pts',(51.8878674165316,14.6580360179265,6.));
#68409=CARTESIAN_POINT('Ctrl Pts',(51.9028425534762,14.7069085917089,6.));
#68410=CARTESIAN_POINT('Ctrl Pts',(51.9204975501424,14.754982591428,6.));
#68411=CARTESIAN_POINT('Ctrl Pts',(51.9408266061613,14.8019671660544,6.));
#68412=CARTESIAN_POINT('Ctrl Pts',(51.9460484511811,14.8140359097675,6.));
#68413=CARTESIAN_POINT('Ctrl Pts',(51.9514489311321,14.826036655033,6.));
#68414=CARTESIAN_POINT('Ctrl Pts',(51.9570156117501,14.837938168984,6.));
#68415=CARTESIAN_POINT('Ctrl Pts',(51.9795172113669,14.8860463900468,6.));
#68416=CARTESIAN_POINT('Ctrl Pts',(52.0047624527444,14.9326133843823,6.));
#68417=CARTESIAN_POINT('Ctrl Pts',(52.0326996004424,14.9773433961128,6.));
#68418=CARTESIAN_POINT('Ctrl Pts',(52.0596890512563,15.0205560556354,6.));
#68419=CARTESIAN_POINT('Ctrl Pts',(52.0891914488154,15.0620548998909,6.));
#68420=CARTESIAN_POINT('Ctrl Pts',(52.1211934155598,15.1015390599859,6.));
#68421=CARTESIAN_POINT('Ctrl Pts',(52.1435818547643,15.1291620096904,6.));
#68422=CARTESIAN_POINT('Ctrl Pts',(52.1671943525027,15.1557982112413,6.));
#68423=CARTESIAN_POINT('Ctrl Pts',(52.1920344148669,15.1813316631752,6.));
#68424=CARTESIAN_POINT('Ctrl Pts',(52.2060464360847,15.1957348182485,6.));
#68425=CARTESIAN_POINT('Ctrl Pts',(52.2204492103834,15.2097868473553,6.));
#68426=CARTESIAN_POINT('Ctrl Pts',(52.2352263046383,15.223479246524,6.));
#68427=CARTESIAN_POINT('Origin',(53.1951359564886,14.3971354987959,0.895788276411274));
#68428=CARTESIAN_POINT('Ctrl Pts',(54.7400287307462,14.397884086359,2.14578827641127));
#68429=CARTESIAN_POINT('Ctrl Pts',(54.7403302631026,14.4458093584932,2.14826884812012));
#68430=CARTESIAN_POINT('Ctrl Pts',(54.7167366550282,14.9990296040617,2.17691792328789));
#68431=CARTESIAN_POINT('Ctrl Pts',(54.0514939360652,15.9998439808924,2.23173550191458));
#68432=CARTESIAN_POINT('Ctrl Pts',(52.3307400382945,15.9953304824803,2.31024101229137));
#68433=CARTESIAN_POINT('Ctrl Pts',(51.3852180733224,14.5577448223715,2.38874652266814));
#68434=CARTESIAN_POINT('Ctrl Pts',(52.0628629644955,12.9760077060224,2.46725203304493));
#68435=CARTESIAN_POINT('Ctrl Pts',(53.7559624418889,12.6688282037076,2.5457575434217));
#68436=CARTESIAN_POINT('Ctrl Pts',(54.658158616602,13.6109326580654,2.60526962454382));
#68437=CARTESIAN_POINT('Ctrl Pts',(54.7387317829834,14.2566058695901,2.63861320220701));
#68438=CARTESIAN_POINT('Ctrl Pts',(54.7375657625992,14.3958310564158,2.64578827641127));
#68439=CARTESIAN_POINT('Ctrl Pts',(54.7364807484814,14.3955730757723,2.10421172358873));
#68440=CARTESIAN_POINT('Ctrl Pts',(54.7341428408094,14.7375070363914,2.12181148931034));
#68441=CARTESIAN_POINT('Ctrl Pts',(54.4552744897983,15.5924244351668,2.16557975849087));
#68442=CARTESIAN_POINT('Ctrl Pts',(53.0510002557363,16.2080728204287,2.23551653113034));
#68443=CARTESIAN_POINT('Ctrl Pts',(51.605113325188,15.2764851170283,2.31402204150712));
#68444=CARTESIAN_POINT('Ctrl Pts',(51.5846111642588,13.5555692706413,2.3925275518839));
#68445=CARTESIAN_POINT('Ctrl Pts',(53.0087575469087,12.5897418281553,2.47103306226068));
#68446=CARTESIAN_POINT('Ctrl Pts',(54.4388957804212,13.178381042198,2.54159445282895));
#68447=CARTESIAN_POINT('Ctrl Pts',(54.7344163061994,14.0445046478413,2.5859873399383));
#68448=CARTESIAN_POINT('Ctrl Pts',(54.73716587472,14.3983674417199,2.60421172358873));
#68449=CARTESIAN_POINT('Ctrl Pts',(52.2370198037663,15.2223467977324,2.));
#68450=CARTESIAN_POINT('Ctrl Pts',(51.9656547514336,14.9072768995629,2.02616850345893));
#68451=CARTESIAN_POINT('Ctrl Pts',(51.7623579720558,13.9937953994845,2.07850551037678));
#68452=CARTESIAN_POINT('Ctrl Pts',(52.7425844632288,12.9776340948198,2.15701102075356));
#68453=CARTESIAN_POINT('Ctrl Pts',(54.1289211584486,13.2376188657684,2.23551653113034));
#68454=CARTESIAN_POINT('Ctrl Pts',(54.6776801082256,14.5359758627139,2.31402204150712));
#68455=CARTESIAN_POINT('Ctrl Pts',(53.8969277031994,15.7105670448821,2.3925275518839));
#68456=CARTESIAN_POINT('Ctrl Pts',(52.4867570591739,15.7068681992943,2.47103306226068));
#68457=CARTESIAN_POINT('Ctrl Pts',(51.7118947618914,14.5287560364896,2.54953857263746));
#68458=CARTESIAN_POINT('Ctrl Pts',(52.2672298007042,13.2325106809332,2.62804408301423));
#68459=CARTESIAN_POINT('Ctrl Pts',(53.6547374411216,12.9807747893732,2.70654959339102));
#68460=CARTESIAN_POINT('Ctrl Pts',(54.6300613996379,13.9992418052107,2.7850551037678));
#68461=CARTESIAN_POINT('Ctrl Pts',(54.3185111760821,15.374560833818,2.86356061414457));
#68462=CARTESIAN_POINT('Ctrl Pts',(52.9994908161496,15.8732958581993,2.94206612452135));
#68463=CARTESIAN_POINT('Ctrl Pts',(51.855929934815,15.0481780331667,3.02057163489813));
#68464=CARTESIAN_POINT('Ctrl Pts',(51.9134007191539,13.6391883627491,3.09907714527491));
#68465=CARTESIAN_POINT('Ctrl Pts',(53.1203622018241,12.909944412367,3.17758265565169));
#68466=CARTESIAN_POINT('Ctrl Pts',(54.394382532434,13.5144484306959,3.25608816602847));
#68467=CARTESIAN_POINT('Ctrl Pts',(54.592890039674,14.9105673726083,3.33459367640525));
#68468=CARTESIAN_POINT('Ctrl Pts',(53.5378584472409,15.8462283160988,3.41309918678203));
#68469=CARTESIAN_POINT('Ctrl Pts',(52.1754651814132,15.4823084146089,3.49160469715881));
#68470=CARTESIAN_POINT('Ctrl Pts',(51.7275369059285,14.1451796218823,3.57011020753559));
#68471=CARTESIAN_POINT('Ctrl Pts',(52.5957863501673,13.0340108603602,3.64861571791237));
#68472=CARTESIAN_POINT('Ctrl Pts',(54.0015467695737,13.1453246755956,3.72712122828915));
#68473=CARTESIAN_POINT('Ctrl Pts',(54.6840988007338,14.3792921998829,3.80562673866593));
#68474=CARTESIAN_POINT('Ctrl Pts',(54.0313135549908,15.6292620174801,3.8841322490427));
#68475=CARTESIAN_POINT('Ctrl Pts',(52.6286243599757,15.7742314816778,3.96263775941949));
#68476=CARTESIAN_POINT('Ctrl Pts',(51.7339962327512,14.6841885294771,4.04114326979627));
#68477=CARTESIAN_POINT('Ctrl Pts',(52.149752946345,13.3367095952976,4.11964878017304));
#68478=CARTESIAN_POINT('Ctrl Pts',(53.5030339960934,12.9402458213459,4.19815429054983));
#68479=CARTESIAN_POINT('Ctrl Pts',(54.5801847638566,13.8503553460012,4.2766598009266));
#68480=CARTESIAN_POINT('Ctrl Pts',(54.41519083395,15.2508303100965,4.35516531130338));
#68481=CARTESIAN_POINT('Ctrl Pts',(53.1560226839298,15.885691473038,4.43367082168017));
#68482=CARTESIAN_POINT('Ctrl Pts',(51.9319322483355,15.1855802477898,4.51217633205694));
#68483=CARTESIAN_POINT('Ctrl Pts',(51.8407129256901,13.7783730316416,4.59068184243372));
#68484=CARTESIAN_POINT('Ctrl Pts',(52.9641723835949,12.9260866978538,4.6691873528105));
#68485=CARTESIAN_POINT('Ctrl Pts',(54.2947654505407,13.3930719178224,4.74769286318728));
#68486=CARTESIAN_POINT('Ctrl Pts',(54.6391846730619,14.7605251935738,4.82619837356406));
#68487=CARTESIAN_POINT('Ctrl Pts',(53.6885466200217,15.8020820199204,4.90470388394084));
#68488=CARTESIAN_POINT('Ctrl Pts',(52.2954062665962,15.5836492690769,4.98320939431762));
#68489=CARTESIAN_POINT('Ctrl Pts',(51.7091646625422,14.3011230348445,5.0617149046944));
#68490=CARTESIAN_POINT('Ctrl Pts',(52.455577895988,13.1047025120629,5.14022041507118));
#68491=CARTESIAN_POINT('Ctrl Pts',(53.8652434689878,13.0673677185785,5.21872592544796));
#68492=CARTESIAN_POINT('Ctrl Pts',(54.6739425216854,14.2225980750992,5.29723143582474));
#68493=CARTESIAN_POINT('Ctrl Pts',(54.1564090232194,15.5343621736369,5.37573694620152));
#68494=CARTESIAN_POINT('Ctrl Pts',(52.7767903419412,15.826225464705,5.4542424565783));
#68495=CARTESIAN_POINT('Ctrl Pts',(51.7723391952092,14.8364647334447,5.53274796695507));
#68496=CARTESIAN_POINT('Ctrl Pts',(52.0439156164789,13.4526673224972,5.61125347733186));
#68497=CARTESIAN_POINT('Ctrl Pts',(53.3478744097592,12.9159632016583,5.68975898770863));
#68498=CARTESIAN_POINT('Ctrl Pts',(54.5149728893469,13.7074656120611,5.76826449808541));
#68499=CARTESIAN_POINT('Ctrl Pts',(54.498171162037,15.1177692904017,5.84677000846219));
#68500=CARTESIAN_POINT('Ctrl Pts',(53.3132562085964,15.88121138355,5.92527551883897));
#68501=CARTESIAN_POINT('Ctrl Pts',(52.0214443153046,15.3148691319142,6.00378102921575));
#68502=CARTESIAN_POINT('Ctrl Pts',(51.7841832172828,13.9230591799233,6.08228653959253));
#68503=CARTESIAN_POINT('Ctrl Pts',(52.4668366999413,13.2829324314547,6.13462354651038));
#68504=CARTESIAN_POINT('Ctrl Pts',(52.8685508929576,13.1755371825404,6.16079204996931));
#68505=CARTESIAN_POINT('Ctrl Pts',(52.166679656532,15.2829297282066,1.94640265001023));
#68506=CARTESIAN_POINT('Ctrl Pts',(51.8753923247544,14.9447289570595,1.97257115346916));
#68507=CARTESIAN_POINT('Ctrl Pts',(51.6571705017343,13.9641841650946,2.02490816038701));
#68508=CARTESIAN_POINT('Ctrl Pts',(52.70936037179,12.8734213253438,2.10341367076379));
#68509=CARTESIAN_POINT('Ctrl Pts',(54.1974750476659,13.1524928917871,2.18191918114057));
#68510=CARTESIAN_POINT('Ctrl Pts',(54.7865211643106,14.5461688352594,2.26042469151735));
#68511=CARTESIAN_POINT('Ctrl Pts',(53.9484497808213,15.8069926902189,2.33893020189413));
#68512=CARTESIAN_POINT('Ctrl Pts',(52.4347513855474,15.8030222936896,2.4174357122709));
#68513=CARTESIAN_POINT('Ctrl Pts',(51.6030025323684,14.5384189651169,2.49594122264769));
#68514=CARTESIAN_POINT('Ctrl Pts',(52.199107521968,13.1470096892963,2.57444673302446));
#68515=CARTESIAN_POINT('Ctrl Pts',(53.688479108044,12.8767925941513,2.65295224340125));
#68516=CARTESIAN_POINT('Ctrl Pts',(54.7354065257528,13.9700304189807,2.73145775377802));
#68517=CARTESIAN_POINT('Ctrl Pts',(54.4009838263145,15.4463185656761,2.8099632641548));
#68518=CARTESIAN_POINT('Ctrl Pts',(52.9851275179858,15.9816682478379,2.88846877453158));
#68519=CARTESIAN_POINT('Ctrl Pts',(51.757612055011,15.0959743547226,2.96697428490836));
#68520=CARTESIAN_POINT('Ctrl Pts',(51.8193020599744,13.5835436342954,3.04547979528514));
#68521=CARTESIAN_POINT('Ctrl Pts',(53.1148726827324,12.8007622013296,3.12398530566192));
#68522=CARTESIAN_POINT('Ctrl Pts',(54.4824252822431,13.4496459136362,3.2024908160387));
#68523=CARTESIAN_POINT('Ctrl Pts',(54.695506228462,14.9482610003549,3.28099632641548));
#68524=CARTESIAN_POINT('Ctrl Pts',(53.5630194367425,15.9526135407249,3.35950183679226));
#68525=CARTESIAN_POINT('Ctrl Pts',(52.1006059983742,15.5619764407204,3.43800734716904));
#68526=CARTESIAN_POINT('Ctrl Pts',(51.6197930452243,14.1266822680612,3.51651285754582));
#68527=CARTESIAN_POINT('Ctrl Pts',(52.5517850676155,12.9339369940615,3.5950183679226));
#68528=CARTESIAN_POINT('Ctrl Pts',(54.0607494614003,13.0534229188377,3.67352387829937));
#68529=CARTESIAN_POINT('Ctrl Pts',(54.7934110854636,14.3779822331642,3.75202938867616));
#68530=CARTESIAN_POINT('Ctrl Pts',(54.0927015769186,15.7197186499972,3.83053489905293));
#68531=CARTESIAN_POINT('Ctrl Pts',(52.5870338816236,15.8753310549564,3.90904040942972));
#68532=CARTESIAN_POINT('Ctrl Pts',(51.6267265838621,14.7052625426694,3.98754591980649));
#68533=CARTESIAN_POINT('Ctrl Pts',(52.0730060982299,13.2588583723836,4.06605143018328));
#68534=CARTESIAN_POINT('Ctrl Pts',(53.525638346701,12.8332881898262,4.14455694056005));
#68535=CARTESIAN_POINT('Ctrl Pts',(54.681868194159,13.8102134526169,4.22306245093683));
#68536=CARTESIAN_POINT('Ctrl Pts',(54.5047612262982,15.3135043591139,4.30156796131361));
#68537=CARTESIAN_POINT('Ctrl Pts',(53.1531511809886,15.9949738873852,4.38007347169039));
#68538=CARTESIAN_POINT('Ctrl Pts',(51.8391940823356,15.2434639600858,4.45857898206717));
#68539=CARTESIAN_POINT('Ctrl Pts',(51.741277888369,13.7329465529009,4.53708449244395));
#68540=CARTESIAN_POINT('Ctrl Pts',(52.9472161808664,12.8180895735458,4.61559000282073));
#68541=CARTESIAN_POINT('Ctrl Pts',(54.3754948070961,13.3193585377509,4.69409551319751));
#68542=CARTESIAN_POINT('Ctrl Pts',(54.7451995847704,14.787203466935,4.77260102357429));
#68543=CARTESIAN_POINT('Ctrl Pts',(53.7247703895732,15.9052262419141,4.85110653395107));
#68544=CARTESIAN_POINT('Ctrl Pts',(52.2293525645705,15.6707572392952,4.92961204432785));
#68545=CARTESIAN_POINT('Ctrl Pts',(51.6000720026333,14.2940742748049,5.00811755470463));
#68546=CARTESIAN_POINT('Ctrl Pts',(52.4012832024729,13.0098184770543,5.08662306508141));
#68547=CARTESIAN_POINT('Ctrl Pts',(53.9144394469056,12.9697427477624,5.16512857545819));
#68548=CARTESIAN_POINT('Ctrl Pts',(54.78250918266,14.2097844010516,5.24363408583497));
#68549=CARTESIAN_POINT('Ctrl Pts',(54.2269809354599,15.6178517291775,5.32213959621174));
#68550=CARTESIAN_POINT('Ctrl Pts',(52.746077476869,15.9311421789545,5.40064510658853));
#68551=CARTESIAN_POINT('Ctrl Pts',(51.6678844969052,14.8687181120791,5.4791506169653));
#68552=CARTESIAN_POINT('Ctrl Pts',(51.9593987152815,13.3833291421626,5.5576561273421));
#68553=CARTESIAN_POINT('Ctrl Pts',(53.359087711258,12.80722286035,5.63616163771885));
#68554=CARTESIAN_POINT('Ctrl Pts',(54.611868786487,13.6568334614203,5.71466714809565));
#68555=CARTESIAN_POINT('Ctrl Pts',(54.5938335594919,15.1706746577306,5.79317265847242));
#68556=CARTESIAN_POINT('Ctrl Pts',(53.3219280130545,15.9901648918943,5.87167816884921));
#68557=CARTESIAN_POINT('Ctrl Pts',(51.9352776823615,15.3822445943694,5.95018367922598));
#68558=CARTESIAN_POINT('Ctrl Pts',(51.680598048476,13.8882548422916,6.02868918960276));
#68559=CARTESIAN_POINT('Ctrl Pts',(52.4133685721047,13.2011331552573,6.08102619652061));
#68560=CARTESIAN_POINT('Ctrl Pts',(52.8445746335155,13.0858534785527,6.10719469997954));
#68561=CARTESIAN_POINT('Ctrl Pts',(52.0963395092977,15.3435126586808,1.89280530002046));
#68562=CARTESIAN_POINT('Ctrl Pts',(51.7851298980751,14.9821810145562,1.91897380347939));
#68563=CARTESIAN_POINT('Ctrl Pts',(51.5519830314128,13.9345729307046,1.97131081039724));
#68564=CARTESIAN_POINT('Ctrl Pts',(52.6761362803514,12.7692085558677,2.04981632077402));
#68565=CARTESIAN_POINT('Ctrl Pts',(54.2660289368831,13.0673669178057,2.1283218311508));
#68566=CARTESIAN_POINT('Ctrl Pts',(54.8953622203958,14.5563618078048,2.20682734152758));
#68567=CARTESIAN_POINT('Ctrl Pts',(53.9999718584432,15.9034183355556,2.28533285190436));
#68568=CARTESIAN_POINT('Ctrl Pts',(52.382745711921,15.899176388085,2.36383836228113));
#68569=CARTESIAN_POINT('Ctrl Pts',(51.4941103028454,14.5480818937442,2.44234387265791));
#68570=CARTESIAN_POINT('Ctrl Pts',(52.1309852432318,13.0615086976594,2.52084938303469));
#68571=CARTESIAN_POINT('Ctrl Pts',(53.7222207749664,12.7728103989295,2.59935489341147));
#68572=CARTESIAN_POINT('Ctrl Pts',(54.8407516518678,13.9408190327507,2.67786040378825));
#68573=CARTESIAN_POINT('Ctrl Pts',(54.483456476547,15.5180762975341,2.75636591416503));
#68574=CARTESIAN_POINT('Ctrl Pts',(52.9707642198219,16.0900406374764,2.83487142454181));
#68575=CARTESIAN_POINT('Ctrl Pts',(51.6592941752072,15.1437706762785,2.91337693491859));
#68576=CARTESIAN_POINT('Ctrl Pts',(51.7252034007948,13.5278989058417,2.99188244529537));
#68577=CARTESIAN_POINT('Ctrl Pts',(53.1093831636409,12.6915799902922,3.07038795567215));
#68578=CARTESIAN_POINT('Ctrl Pts',(54.5704680320522,13.3848433965765,3.14889346604893));
#68579=CARTESIAN_POINT('Ctrl Pts',(54.7981224172499,14.9859546281015,3.22739897642571));
#68580=CARTESIAN_POINT('Ctrl Pts',(53.5881804262442,16.0589987653509,3.30590448680249));
#68581=CARTESIAN_POINT('Ctrl Pts',(52.0257468153352,15.6416444668319,3.38440999717927));
#68582=CARTESIAN_POINT('Ctrl Pts',(51.5120491845202,14.10818491424,3.46291550755605));
#68583=CARTESIAN_POINT('Ctrl Pts',(52.5077837850637,12.8338631277627,3.54142101793282));
#68584=CARTESIAN_POINT('Ctrl Pts',(54.1199521532269,12.9615211620797,3.61992652830961));
#68585=CARTESIAN_POINT('Ctrl Pts',(54.9027233701934,14.3766722664456,3.69843203868638));
#68586=CARTESIAN_POINT('Ctrl Pts',(54.1540895988462,15.8101752825143,3.77693754906317));
#68587=CARTESIAN_POINT('Ctrl Pts',(52.5454434032715,15.9764306282351,3.85544305943994));
#68588=CARTESIAN_POINT('Ctrl Pts',(51.5194569349729,14.7263365558616,3.93394856981673));
#68589=CARTESIAN_POINT('Ctrl Pts',(51.9962592501147,13.1810071494696,4.0124540801935));
#68590=CARTESIAN_POINT('Ctrl Pts',(53.5482426973085,12.7263305583065,4.09095959057029));
#68591=CARTESIAN_POINT('Ctrl Pts',(54.7835516244613,13.7700715592326,4.16946510094706));
#68592=CARTESIAN_POINT('Ctrl Pts',(54.5943316186464,15.3761784081312,4.24797061132384));
#68593=CARTESIAN_POINT('Ctrl Pts',(53.1502796780473,16.1042563017325,4.32647612170062));
#68594=CARTESIAN_POINT('Ctrl Pts',(51.7464559163357,15.3013476723818,4.4049816320774));
#68595=CARTESIAN_POINT('Ctrl Pts',(51.6418428510479,13.6875200741603,4.48348714245418));
#68596=CARTESIAN_POINT('Ctrl Pts',(52.9302599781379,12.7100924492379,4.56199265283096));
#68597=CARTESIAN_POINT('Ctrl Pts',(54.4562241636517,13.2456451576795,4.64049816320774));
#68598=CARTESIAN_POINT('Ctrl Pts',(54.8512144964787,14.8138817402962,4.71900367358452));
#68599=CARTESIAN_POINT('Ctrl Pts',(53.7609941591248,16.0083704639078,4.7975091839613));
#68600=CARTESIAN_POINT('Ctrl Pts',(52.1632988625446,15.7578652095136,4.87601469433808));
#68601=CARTESIAN_POINT('Ctrl Pts',(51.4909793427245,14.2870255147652,4.95452020471486));
#68602=CARTESIAN_POINT('Ctrl Pts',(52.3469885089579,12.9149344420457,5.03302571509164));
#68603=CARTESIAN_POINT('Ctrl Pts',(53.9636354248233,12.8721177769464,5.11153122546841));
#68604=CARTESIAN_POINT('Ctrl Pts',(54.8910758436347,14.1969707270041,5.1900367358452));
#68605=CARTESIAN_POINT('Ctrl Pts',(54.2975528477005,15.7013412847181,5.26854224622198));
#68606=CARTESIAN_POINT('Ctrl Pts',(52.7153646117967,16.0360588932041,5.34704775659875));
#68607=CARTESIAN_POINT('Ctrl Pts',(51.5634297986012,14.9009714907135,5.42555326697554));
#68608=CARTESIAN_POINT('Ctrl Pts',(51.874881814084,13.3139909618281,5.50405877735232));
#68609=CARTESIAN_POINT('Ctrl Pts',(53.3703010127568,12.6984825190418,5.58256428772909));
#68610=CARTESIAN_POINT('Ctrl Pts',(54.7087646836271,13.6062013107796,5.66106979810587));
#68611=CARTESIAN_POINT('Ctrl Pts',(54.6894959569468,15.2235800250595,5.73957530848266));
#68612=CARTESIAN_POINT('Ctrl Pts',(53.3305998175126,16.0991184002386,5.81808081885943));
#68613=CARTESIAN_POINT('Ctrl Pts',(51.8491110494184,15.4496200568245,5.89658632923621));
#68614=CARTESIAN_POINT('Ctrl Pts',(51.5770128796691,13.8534505046598,5.97509183961299));
#68615=CARTESIAN_POINT('Ctrl Pts',(52.359900444268,13.11933387906,6.02742884653084));
#68616=CARTESIAN_POINT('Ctrl Pts',(52.8205983740735,12.9961697745651,6.05359734998977));
#68617=CARTESIAN_POINT('Ctrl Pts',(52.0259993620635,15.4040955891549,1.83920795003069));
#68618=CARTESIAN_POINT('Ctrl Pts',(51.6948674713958,15.0196330720529,1.86537645348961));
#68619=CARTESIAN_POINT('Ctrl Pts',(51.4467955610913,13.9049616963147,1.91771346040747));
#68620=CARTESIAN_POINT('Ctrl Pts',(52.6429121889126,12.6649957863917,1.99621897078425));
#68621=CARTESIAN_POINT('Ctrl Pts',(54.3345828261004,12.9822409438244,2.07472448116103));
#68622=CARTESIAN_POINT('Ctrl Pts',(55.0042032764809,14.5665547803503,2.15322999153781));
#68623=CARTESIAN_POINT('Ctrl Pts',(54.0514939360652,15.9998439808924,2.23173550191458));
#68624=CARTESIAN_POINT('Ctrl Pts',(52.3307400382945,15.9953304824803,2.31024101229137));
#68625=CARTESIAN_POINT('Ctrl Pts',(51.3852180733224,14.5577448223715,2.38874652266814));
#68626=CARTESIAN_POINT('Ctrl Pts',(52.0628629644955,12.9760077060224,2.46725203304493));
#68627=CARTESIAN_POINT('Ctrl Pts',(53.7559624418889,12.6688282037076,2.5457575434217));
#68628=CARTESIAN_POINT('Ctrl Pts',(54.9460967779827,13.9116076465207,2.62426305379849));
#68629=CARTESIAN_POINT('Ctrl Pts',(54.5659291267794,15.5898340293922,2.70276856417526));
#68630=CARTESIAN_POINT('Ctrl Pts',(52.9564009216582,16.198413027115,2.78127407455204));
#68631=CARTESIAN_POINT('Ctrl Pts',(51.5609762954032,15.1915669978344,2.85977958492882));
#68632=CARTESIAN_POINT('Ctrl Pts',(51.6311047416152,13.472254177388,2.9382850953056));
#68633=CARTESIAN_POINT('Ctrl Pts',(53.1038936445493,12.5823977792548,3.01679060568238));
#68634=CARTESIAN_POINT('Ctrl Pts',(54.6585107818612,13.3200408795168,3.09529611605916));
#68635=CARTESIAN_POINT('Ctrl Pts',(54.9007386060379,15.0236482558482,3.17380162643594));
#68636=CARTESIAN_POINT('Ctrl Pts',(53.6133414157458,16.1653839899769,3.25230713681272));
#68637=CARTESIAN_POINT('Ctrl Pts',(51.9508876322963,15.7213124929433,3.3308126471895));
#68638=CARTESIAN_POINT('Ctrl Pts',(51.4043053238161,14.0896875604189,3.40931815756628));
#68639=CARTESIAN_POINT('Ctrl Pts',(52.4637825025118,12.7337892614639,3.48782366794306));
#68640=CARTESIAN_POINT('Ctrl Pts',(54.1791548450535,12.8696194053218,3.56632917831983));
#68641=CARTESIAN_POINT('Ctrl Pts',(55.0120356549231,14.3753622997269,3.64483468869662));
#68642=CARTESIAN_POINT('Ctrl Pts',(54.215477620774,15.9006319150314,3.72334019907339));
#68643=CARTESIAN_POINT('Ctrl Pts',(52.5038529249194,16.0775302015138,3.80184570945018));
#68644=CARTESIAN_POINT('Ctrl Pts',(51.4121872860838,14.7474105690538,3.88035121982695));
#68645=CARTESIAN_POINT('Ctrl Pts',(51.9195124019995,13.1031559265556,3.95885673020373));
#68646=CARTESIAN_POINT('Ctrl Pts',(53.5708470479161,12.6193729267869,4.03736224058052));
#68647=CARTESIAN_POINT('Ctrl Pts',(54.8852350547637,13.7299296658483,4.11586775095729));
#68648=CARTESIAN_POINT('Ctrl Pts',(54.6839020109947,15.4388524571485,4.19437326133407));
#68649=CARTESIAN_POINT('Ctrl Pts',(53.147408175106,16.2135387160798,4.27287877171085));
#68650=CARTESIAN_POINT('Ctrl Pts',(51.6537177503359,15.3592313846778,4.35138428208763));
#68651=CARTESIAN_POINT('Ctrl Pts',(51.5424078137269,13.6420935954197,4.42988979246441));
#68652=CARTESIAN_POINT('Ctrl Pts',(52.9133037754092,12.6020953249299,4.50839530284119));
#68653=CARTESIAN_POINT('Ctrl Pts',(54.5369535202073,13.171931777608,4.58690081321797));
#68654=CARTESIAN_POINT('Ctrl Pts',(54.9572294081871,14.8405600136574,4.66540632359475));
#68655=CARTESIAN_POINT('Ctrl Pts',(53.7972179286764,16.1115146859015,4.74391183397153));
#68656=CARTESIAN_POINT('Ctrl Pts',(52.0972451605188,15.8449731797319,4.82241734434831));
#68657=CARTESIAN_POINT('Ctrl Pts',(51.3818866828157,14.2799767547255,4.90092285472509));
#68658=CARTESIAN_POINT('Ctrl Pts',(52.2926938154427,12.820050407037,4.97942836510186));
#68659=CARTESIAN_POINT('Ctrl Pts',(54.0128314027411,12.7744928061304,5.05793387547865));
#68660=CARTESIAN_POINT('Ctrl Pts',(54.9996425046093,14.1841570529565,5.13643938585542));
#68661=CARTESIAN_POINT('Ctrl Pts',(54.368124759941,15.7848308402587,5.21494489623221));
#68662=CARTESIAN_POINT('Ctrl Pts',(52.6846517467245,16.1409756074537,5.29345040660899));
#68663=CARTESIAN_POINT('Ctrl Pts',(51.4589751002972,14.933224869348,5.37195591698576));
#68664=CARTESIAN_POINT('Ctrl Pts',(51.7903649128864,13.2446527814935,5.45046142736255));
#68665=CARTESIAN_POINT('Ctrl Pts',(53.3815143142557,12.5897421777335,5.52896693773932));
#68666=CARTESIAN_POINT('Ctrl Pts',(54.8056605807673,13.5555691601388,5.60747244811611));
#68667=CARTESIAN_POINT('Ctrl Pts',(54.7851583544017,15.2764853923884,5.68597795849288));
#68668=CARTESIAN_POINT('Ctrl Pts',(53.3392716219708,16.2080719085829,5.76448346886966));
#68669=CARTESIAN_POINT('Ctrl Pts',(51.7629444164752,15.5169955192796,5.84298897924645));
#68670=CARTESIAN_POINT('Ctrl Pts',(51.4734277108623,13.8186461670281,5.92149448962322));
#68671=CARTESIAN_POINT('Ctrl Pts',(52.3064323164313,13.0375346028627,5.97383149654107));
#68672=CARTESIAN_POINT('Ctrl Pts',(52.7966221146314,12.9064860705774,6.));
#68673=CARTESIAN_POINT('Ctrl Pts',(52.2370198037663,15.2223467977324,2.));
#68674=CARTESIAN_POINT('Ctrl Pts',(52.2001398221828,15.1879057962806,2.));
#68675=CARTESIAN_POINT('Ctrl Pts',(52.1656378013754,15.151226274978,2.));
#68676=CARTESIAN_POINT('Ctrl Pts',(52.1335158959969,15.112628111498,2.));
#68677=CARTESIAN_POINT('Ctrl Pts',(52.0999545216909,15.0723002605561,2.));
#68678=CARTESIAN_POINT('Ctrl Pts',(52.0689907405515,15.0298774985354,2.));
#68679=CARTESIAN_POINT('Ctrl Pts',(52.0406550241375,14.9856749556985,2.));
#68680=CARTESIAN_POINT('Ctrl Pts',(52.0179305604288,14.9502257344452,2.));
#68681=CARTESIAN_POINT('Ctrl Pts',(51.996896813921,14.9136306734541,2.));
#68682=CARTESIAN_POINT('Ctrl Pts',(51.9775857407062,14.8760343811028,2.));
#68683=CARTESIAN_POINT('Ctrl Pts',(51.9694199887415,14.8601366630052,2.));
#68684=CARTESIAN_POINT('Ctrl Pts',(51.9615624516275,14.8440597542843,2.));
#68685=CARTESIAN_POINT('Ctrl Pts',(51.9540164358694,14.8278139468967,2.));
#68686=CARTESIAN_POINT('Ctrl Pts',(51.949738091225,14.8186031043464,2.));
#68687=CARTESIAN_POINT('Ctrl Pts',(51.9455597069868,14.8093372706419,2.));
#68688=CARTESIAN_POINT('Ctrl Pts',(51.9414881758679,14.8000332484628,2.));
#68689=CARTESIAN_POINT('Ctrl Pts',(51.9196632025192,14.7501601097928,2.));
#68690=CARTESIAN_POINT('Ctrl Pts',(51.9008587821431,14.6990941700718,2.));
#68691=CARTESIAN_POINT('Ctrl Pts',(51.8851025499004,14.6471668919071,2.));
#68692=CARTESIAN_POINT('Ctrl Pts',(51.8690578813861,14.594289024142,2.));
#68693=CARTESIAN_POINT('Ctrl Pts',(51.8561734275543,14.5405170692708,2.));
#68694=CARTESIAN_POINT('Ctrl Pts',(51.8465190610403,14.486166435836,2.));
#68695=CARTESIAN_POINT('Ctrl Pts',(51.8396145127802,14.4472962965087,2.));
#68696=CARTESIAN_POINT('Ctrl Pts',(51.8343629002769,14.4081294056505,2.));
#68697=CARTESIAN_POINT('Ctrl Pts',(51.8308047851301,14.3687747569505,2.));
#68698=CARTESIAN_POINT('Ctrl Pts',(51.8292917204563,14.3520394557475,2.));
#68699=CARTESIAN_POINT('Ctrl Pts',(51.8280850589952,14.3352701585883,2.));
#68700=CARTESIAN_POINT('Ctrl Pts',(51.8271886807074,14.3184751149596,2.));
#68701=CARTESIAN_POINT('Ctrl Pts',(51.8266545203237,14.308466788039,2.));
#68702=CARTESIAN_POINT('Ctrl Pts',(51.8262309124747,14.2984549962446,2.));
#68703=CARTESIAN_POINT('Ctrl Pts',(51.8259184499979,14.288449081502,2.));
#68704=CARTESIAN_POINT('Ctrl Pts',(51.824144879443,14.2316544354973,2.));
#68705=CARTESIAN_POINT('Ctrl Pts',(51.8259444031715,14.1749772815937,2.));
#68706=CARTESIAN_POINT('Ctrl Pts',(51.8313770542921,14.1187497413728,2.));
#68707=CARTESIAN_POINT('Ctrl Pts',(51.8347120697962,14.084232575769,2.));
#68708=CARTESIAN_POINT('Ctrl Pts',(51.8394171165415,14.0498843036968,2.));
#68709=CARTESIAN_POINT('Ctrl Pts',(51.845515342272,14.0157787106909,2.));
#68710=CARTESIAN_POINT('Ctrl Pts',(51.8551874830705,13.961685255947,2.));
#68711=CARTESIAN_POINT('Ctrl Pts',(51.8683614486687,13.908201794507,2.));
#68712=CARTESIAN_POINT('Ctrl Pts',(51.8848110251023,13.8555328884195,2.));
#68713=CARTESIAN_POINT('Ctrl Pts',(51.8897327932487,13.8397741760092,2.));
#68714=CARTESIAN_POINT('Ctrl Pts',(51.89494815524,13.8240884170169,2.));
#68715=CARTESIAN_POINT('Ctrl Pts',(51.9004519259219,13.8084812249402,2.));
#68716=CARTESIAN_POINT('Ctrl Pts',(51.9055403383179,13.7940518756411,2.));
#68717=CARTESIAN_POINT('Ctrl Pts',(51.9108779029635,13.7796834481737,2.));
#68718=CARTESIAN_POINT('Ctrl Pts',(51.9164469096144,13.7654145762709,2.));
#68719=CARTESIAN_POINT('Ctrl Pts',(51.9370780110834,13.7125537049294,2.));
#68720=CARTESIAN_POINT('Ctrl Pts',(51.9609027535646,13.6609889336899,2.));
#68721=CARTESIAN_POINT('Ctrl Pts',(51.9876380075304,13.6109308617546,2.));
#68722=CARTESIAN_POINT('Ctrl Pts',(52.0150055546563,13.5596889081725,2.));
#68723=CARTESIAN_POINT('Ctrl Pts',(52.045423253279,13.5100248567638,2.));
#68724=CARTESIAN_POINT('Ctrl Pts',(52.0786427430285,13.4621702328152,2.));
#68725=CARTESIAN_POINT('Ctrl Pts',(52.0988112436273,13.4331163244306,2.));
#68726=CARTESIAN_POINT('Ctrl Pts',(52.120013548353,13.4047295468198,2.));
#68727=CARTESIAN_POINT('Ctrl Pts',(52.1422027768495,13.3770649262704,2.));
#68728=CARTESIAN_POINT('Ctrl Pts',(52.1544198936821,13.3618331257853,2.));
#68729=CARTESIAN_POINT('Ctrl Pts',(52.1669363024278,13.3468202983598,2.));
#68730=CARTESIAN_POINT('Ctrl Pts',(52.179744929617,13.3320361041125,2.));
#68731=CARTESIAN_POINT('Ctrl Pts',(52.1874577031776,13.3231337337943,2.));
#68732=CARTESIAN_POINT('Ctrl Pts',(52.1952777965343,13.3143127818621,2.));
#68733=CARTESIAN_POINT('Ctrl Pts',(52.2031994409785,13.305580167691,2.));
#68734=CARTESIAN_POINT('Ctrl Pts',(52.2437953927624,13.260828249534,2.));
#68735=CARTESIAN_POINT('Ctrl Pts',(52.2869270094075,13.2185332555424,2.));
#68736=CARTESIAN_POINT('Ctrl Pts',(52.3323340644797,13.1789459514192,2.));
#68737=CARTESIAN_POINT('Ctrl Pts',(52.361857692103,13.1532063207894,2.));
#68738=CARTESIAN_POINT('Ctrl Pts',(52.3923443514829,13.1286116909656,2.));
#68739=CARTESIAN_POINT('Ctrl Pts',(52.4237326847812,13.1052370160116,2.));
#68740=CARTESIAN_POINT('Ctrl Pts',(52.4367029257511,13.0955781671691,2.));
#68741=CARTESIAN_POINT('Ctrl Pts',(52.4498272129069,13.086127694501,2.));
#68742=CARTESIAN_POINT('Ctrl Pts',(52.463101559564,13.0768912104406,2.));
#68743=CARTESIAN_POINT('Ctrl Pts',(52.4728212298238,13.0701281220758,2.));
#68744=CARTESIAN_POINT('Ctrl Pts',(52.4826204710268,13.0634804790307,2.));
#68745=CARTESIAN_POINT('Ctrl Pts',(52.4924892033939,13.0569558444863,2.));
#68746=CARTESIAN_POINT('Ctrl Pts',(52.5432262965278,13.0234114156552,2.));
#68747=CARTESIAN_POINT('Ctrl Pts',(52.5958554391195,12.993074592538,2.));
#68748=CARTESIAN_POINT('Ctrl Pts',(52.6501404639279,12.966212166386,2.));
#68749=CARTESIAN_POINT('Ctrl Pts',(52.6755695106503,12.9536288454405,2.));
#68750=CARTESIAN_POINT('Ctrl Pts',(52.7013624782246,12.9418083828109,2.));
#68751=CARTESIAN_POINT('Ctrl Pts',(52.7274977743507,12.930781120438,2.));
#68752=CARTESIAN_POINT('Ctrl Pts',(52.7499504413758,12.9213076693218,2.));
#68753=CARTESIAN_POINT('Ctrl Pts',(52.7726557928972,12.9124196555961,2.));
#68754=CARTESIAN_POINT('Ctrl Pts',(52.7955926848293,12.9041113294173,2.));
#68755=CARTESIAN_POINT('Ctrl Pts',(54.4591686783466,14.3960664985434,2.80658032638058));
#68756=CARTESIAN_POINT('Ctrl Pts',(54.4601242407418,14.2819704202925,2.79940525217632));
#68757=CARTESIAN_POINT('Ctrl Pts',(54.4459154362348,14.1681081402059,2.79223017797205));
#68758=CARTESIAN_POINT('Ctrl Pts',(54.4155823692925,14.0587171406723,2.78505510376779));
#68759=CARTESIAN_POINT('Ctrl Pts',(54.3049534134658,13.6597527999315,2.75888660030886));
#68760=CARTESIAN_POINT('Ctrl Pts',(53.9798454272937,13.3202637946524,2.73271809684994));
#68761=CARTESIAN_POINT('Ctrl Pts',(53.5860401608047,13.1924752739395,2.70654959339101));
#68762=CARTESIAN_POINT('Ctrl Pts',(53.1922348943158,13.0646867532265,2.68038108993208));
#68763=CARTESIAN_POINT('Ctrl Pts',(52.72973234751,13.1485987170799,2.65421258647316));
#68764=CARTESIAN_POINT('Ctrl Pts',(52.405925234305,13.4065955915993,2.62804408301423));
#68765=CARTESIAN_POINT('Ctrl Pts',(52.0821181210999,13.6645924661187,2.6018755795553));
#68766=CARTESIAN_POINT('Ctrl Pts',(51.8970064414957,14.0966742513041,2.57570707609638));
#68767=CARTESIAN_POINT('Ctrl Pts',(51.9335943179073,14.509067171031,2.54953857263745));
#68768=CARTESIAN_POINT('Ctrl Pts',(51.9701821943189,14.9214600907578,2.52337006917852));
#68769=CARTESIAN_POINT('Ctrl Pts',(52.2284696267464,15.314164145026,2.4972015657196));
#68770=CARTESIAN_POINT('Ctrl Pts',(52.5926417836311,15.5111326464248,2.47103306226067));
#68771=CARTESIAN_POINT('Ctrl Pts',(52.9568139405157,15.7081011478236,2.44486455880174));
#68772=CARTESIAN_POINT('Ctrl Pts',(53.4268708218575,15.7093340963528,2.41869605534282));
#68773=CARTESIAN_POINT('Ctrl Pts',(53.7920246633662,15.5141853735895,2.39252755188389));
#68774=CARTESIAN_POINT('Ctrl Pts',(54.1571785048748,15.3190366508261,2.36635904842496));
#68775=CARTESIAN_POINT('Ctrl Pts',(54.4174293065502,14.92750625677,2.34019054496604));
#68776=CARTESIAN_POINT('Ctrl Pts',(54.456094882425,14.5153482269177,2.31402204150711));
#68777=CARTESIAN_POINT('Ctrl Pts',(54.4597600799313,14.4762788338196,2.31154146979827));
#68778=CARTESIAN_POINT('Ctrl Pts',(54.461434207113,14.4370240895848,2.30906089808942));
#68779=CARTESIAN_POINT('Ctrl Pts',(54.4611870990995,14.3977489718831,2.30658032638058));
#68780=CARTESIAN_POINT('Ctrl Pts',(53.5936497983459,12.9064860705774,2.));
#68781=CARTESIAN_POINT('Ctrl Pts',(54.083839596546,13.0375346028627,2.02616850345893));
#68782=CARTESIAN_POINT('Ctrl Pts',(54.9168437793101,13.8186488783651,2.07850551037678));
#68783=CARTESIAN_POINT('Ctrl Pts',(54.6273278627067,15.5169944524465,2.15701102075356));
#68784=CARTESIAN_POINT('Ctrl Pts',(53.0510002557363,16.2080728204287,2.23551653113034));
#68785=CARTESIAN_POINT('Ctrl Pts',(51.605113325188,15.2764851170283,2.31402204150712));
#68786=CARTESIAN_POINT('Ctrl Pts',(51.5846111642588,13.5555692706413,2.3925275518839));
#68787=CARTESIAN_POINT('Ctrl Pts',(53.0087575469087,12.5897418281553,2.47103306226068));
#68788=CARTESIAN_POINT('Ctrl Pts',(54.5999071972633,13.244652701567,2.54953857263746));
#68789=CARTESIAN_POINT('Ctrl Pts',(54.9312970207009,14.9332249012822,2.62804408301423));
#68790=CARTESIAN_POINT('Ctrl Pts',(53.7056202382209,16.1409758479641,2.70654959339102));
#68791=CARTESIAN_POINT('Ctrl Pts',(52.0221470001078,15.7848310056966,2.78505510376779));
#68792=CARTESIAN_POINT('Ctrl Pts',(51.3906291820654,14.1841570315506,2.86356061414457));
#68793=CARTESIAN_POINT('Ctrl Pts',(52.3774404052229,12.7744925974775,2.94206612452135));
#68794=CARTESIAN_POINT('Ctrl Pts',(54.0975782126823,12.8200502087089,3.02057163489813));
#68795=CARTESIAN_POINT('Ctrl Pts',(55.0083854595842,14.2799767390429,3.09907714527492));
#68796=CARTESIAN_POINT('Ctrl Pts',(54.293026891849,15.8449733636912,3.17758265565169));
#68797=CARTESIAN_POINT('Ctrl Pts',(52.5930539078611,16.1115149029784,3.25608816602847));
#68798=CARTESIAN_POINT('Ctrl Pts',(51.4330422815012,14.8405600699842,3.33459367640525));
#68799=CARTESIAN_POINT('Ctrl Pts',(51.8533182226522,13.1719316222439,3.41309918678203));
#68800=CARTESIAN_POINT('Ctrl Pts',(53.4769681733105,12.6020950974316,3.49160469715881));
#68801=CARTESIAN_POINT('Ctrl Pts',(54.8478643087328,13.642093499697,3.57011020753559));
#68802=CARTESIAN_POINT('Ctrl Pts',(54.7365543580298,15.3592315066375,3.64861571791237));
#68803=CARTESIAN_POINT('Ctrl Pts',(53.2428637439183,16.2135389463141,3.72712122828915));
#68804=CARTESIAN_POINT('Ctrl Pts',(51.7063697132749,15.4388525891942,3.80562673866593));
#68805=CARTESIAN_POINT('Ctrl Pts',(51.5050366439836,13.7299295812751,3.88413224904271));
#68806=CARTESIAN_POINT('Ctrl Pts',(52.8194248174382,12.6193727014466,3.96263775941949));
#68807=CARTESIAN_POINT('Ctrl Pts',(54.4707596726698,13.1031557625362,4.04114326979626));
#68808=CARTESIAN_POINT('Ctrl Pts',(54.978084852892,14.7474106134536,4.11964878017304));
#68809=CARTESIAN_POINT('Ctrl Pts',(53.8864190756817,16.077530414512,4.19815429054983));
#68810=CARTESIAN_POINT('Ctrl Pts',(52.1747941628695,15.9006321056092,4.2766598009266));
#68811=CARTESIAN_POINT('Ctrl Pts',(51.3782360277522,14.3753622969642,4.35516531130339));
#68812=CARTESIAN_POINT('Ctrl Pts',(52.2111169431944,12.8696192117062,4.43367082168016));
#68813=CARTESIAN_POINT('Ctrl Pts',(53.9264895031678,12.7337890506155,4.51217633205695));
#68814=CARTESIAN_POINT('Ctrl Pts',(54.9859668161601,14.0896875214679,4.59068184243372));
#68815=CARTESIAN_POINT('Ctrl Pts',(54.4393844383933,15.7213126607523,4.6691873528105));
#68816=CARTESIAN_POINT('Ctrl Pts',(52.7769304442279,16.1653842141838,4.74769286318728));
#68817=CARTESIAN_POINT('Ctrl Pts',(51.4895330907317,15.0236483351255,4.82619837356406));
#68818=CARTESIAN_POINT('Ctrl Pts',(51.7317609456535,13.3200407432483,4.90470388394085));
#68819=CARTESIAN_POINT('Ctrl Pts',(53.2863782799342,12.5823975487372,4.98320939431761));
#68820=CARTESIAN_POINT('Ctrl Pts',(54.7591673697362,13.4722540610765,5.06171490469441));
#68821=CARTESIAN_POINT('Ctrl Pts',(54.8292958244512,15.1915670968036,5.14022041507117));
#68822=CARTESIAN_POINT('Ctrl Pts',(53.4338710221273,16.1984132586634,5.21872592544796));
#68823=CARTESIAN_POINT('Ctrl Pts',(51.8243426112988,15.5898341745865,5.29723143582474));
#68824=CARTESIAN_POINT('Ctrl Pts',(51.4441749154368,13.9116075960113,5.37573694620152));
#68825=CARTESIAN_POINT('Ctrl Pts',(52.6343093950298,12.6688279644592,5.45424245657829));
#68826=CARTESIAN_POINT('Ctrl Pts',(54.3274091023452,12.976007562431,5.53274796695508));
#68827=CARTESIAN_POINT('Ctrl Pts',(55.0050540475836,14.5577447773064,5.61125347733185));
#68828=CARTESIAN_POINT('Ctrl Pts',(54.0595320288467,15.9953308004787,5.68975898770864));
#68829=CARTESIAN_POINT('Ctrl Pts',(52.3387777758966,15.9998439842325,5.76826449808541));
#68830=CARTESIAN_POINT('Ctrl Pts',(51.386068598834,14.5665551393412,5.8467700084622));
#68831=CARTESIAN_POINT('Ctrl Pts',(52.0556885439603,12.9822402103747,5.92527551883896));
#68832=CARTESIAN_POINT('Ctrl Pts',(53.7473606277103,12.6649964614199,6.00378102921576));
#68833=CARTESIAN_POINT('Ctrl Pts',(54.9434744748871,13.9049596945687,6.08228653959253));
#68834=CARTESIAN_POINT('Ctrl Pts',(54.6954044415815,15.0196330720529,6.13462354651039));
#68835=CARTESIAN_POINT('Ctrl Pts',(54.3642725509138,15.404095589155,6.16079204996931));
#68836=CARTESIAN_POINT('Ctrl Pts',(53.5696735389038,12.996169774565,1.94640265001023));
#68837=CARTESIAN_POINT('Ctrl Pts',(54.0303714687093,13.11933387906,1.97257115346916));
#68838=CARTESIAN_POINT('Ctrl Pts',(54.813258635941,13.8534530528714,2.02490816038701));
#68839=CARTESIAN_POINT('Ctrl Pts',(54.5411612077311,15.4496190541765,2.10341367076379));
#68840=CARTESIAN_POINT('Ctrl Pts',(53.0596720623164,16.099119257224,2.18191918114057));
#68841=CARTESIAN_POINT('Ctrl Pts',(51.7007757366845,15.2235797662663,2.26042469151735));
#68842=CARTESIAN_POINT('Ctrl Pts',(51.6815070715035,13.6062014146337,2.33893020189412));
#68843=CARTESIAN_POINT('Ctrl Pts',(53.0199708515249,12.6984821904957,2.41743571227091));
#68844=CARTESIAN_POINT('Ctrl Pts',(54.515390284203,13.3139908867102,2.49594122264768));
#68845=CARTESIAN_POINT('Ctrl Pts',(54.8268423098815,14.9009715207264,2.57444673302447));
#68846=CARTESIAN_POINT('Ctrl Pts',(53.6749073688187,16.0360591192445,2.65295224340125));
#68847=CARTESIAN_POINT('Ctrl Pts',(52.0927189215492,15.7013414402026,2.73145775377802));
#68848=CARTESIAN_POINT('Ctrl Pts',(51.4991958566553,14.1969707068861,2.8099632641548));
#68849=CARTESIAN_POINT('Ctrl Pts',(52.4266363894587,12.8721175808469,2.88846877453159));
#68850=CARTESIAN_POINT('Ctrl Pts',(54.0432835122395,12.9149342556498,2.96697428490836));
#68851=CARTESIAN_POINT('Ctrl Pts',(54.8992927858723,14.2870255000261,3.04547979528514));
#68852=CARTESIAN_POINT('Ctrl Pts',(54.2269731814369,15.7578653824051,3.12398530566192));
#68853=CARTESIAN_POINT('Ctrl Pts',(52.6292776820116,16.0083706679245,3.2024908160387));
#68854=CARTESIAN_POINT('Ctrl Pts',(51.5390572066436,14.8138817932341,3.28099632641548));
#68855=CARTESIAN_POINT('Ctrl Pts',(51.9340475894427,13.2456450116627,3.35950183679226));
#68856=CARTESIAN_POINT('Ctrl Pts',(53.4600119684315,12.7100922354268,3.43800734716904));
#68857=CARTESIAN_POINT('Ctrl Pts',(54.7484292588084,13.6875199841967,3.51651285754582));
#68858=CARTESIAN_POINT('Ctrl Pts',(54.6438161802745,15.3013477870039,3.5950183679226));
#68859=CARTESIAN_POINT('Ctrl Pts',(53.2399922406132,16.104256518115,3.67352387829938));
#68860=CARTESIAN_POINT('Ctrl Pts',(51.7959401169765,15.3761785322324,3.75202938867615));
#68861=CARTESIAN_POINT('Ctrl Pts',(51.606720087175,13.7700714797477,3.83053489905294));
#68862=CARTESIAN_POINT('Ctrl Pts',(52.8420291709109,12.7263303465236,3.90904040942971));
#68863=CARTESIAN_POINT('Ctrl Pts',(54.3940128148265,13.1810069953183,3.9875459198065));
#68864=CARTESIAN_POINT('Ctrl Pts',(54.8708151904059,14.7263365975901,4.06605143018327));
#68865=CARTESIAN_POINT('Ctrl Pts',(53.8448285920578,15.9764308284185,4.14455694056006));
#68866=CARTESIAN_POINT('Ctrl Pts',(52.2361821925785,15.8101754616261,4.22306245093683));
#68867=CARTESIAN_POINT('Ctrl Pts',(51.4875483263378,14.3766722638491,4.30156796131361));
#68868=CARTESIAN_POINT('Ctrl Pts',(52.2703196425253,12.9615209801128,4.38007347169039));
#68869=CARTESIAN_POINT('Ctrl Pts',(53.8824882150385,12.8338629295998,4.45857898206717));
#68870=CARTESIAN_POINT('Ctrl Pts',(54.8782229417988,14.1081848776325,4.53708449244395));
#68871=CARTESIAN_POINT('Ctrl Pts',(54.3645252458656,15.6416446245447,4.61559000282073));
#68872=CARTESIAN_POINT('Ctrl Pts',(52.8020914369185,16.0589989760686,4.69409551319751));
#68873=CARTESIAN_POINT('Ctrl Pts',(51.5921492925276,14.9859547026092,4.77260102357429));
#68874=CARTESIAN_POINT('Ctrl Pts',(51.8198037066208,13.3848432685065,4.85110653395107));
#68875=CARTESIAN_POINT('Ctrl Pts',(53.2808887601503,12.6915797736435,4.92961204432785));
#68876=CARTESIAN_POINT('Ctrl Pts',(54.6650686986216,13.527898796528,5.00811755470463));
#68877=CARTESIAN_POINT('Ctrl Pts',(54.7309779322007,15.1437707692933,5.08662306508141));
#68878=CARTESIAN_POINT('Ctrl Pts',(53.41950772211,16.0900408550939,5.16512857545819));
#68879=CARTESIAN_POINT('Ctrl Pts',(51.9068152720538,15.5180764339929,5.24363408583497));
#68880=CARTESIAN_POINT('Ctrl Pts',(51.5495200547613,13.9408189852801,5.32213959621175));
#68881=CARTESIAN_POINT('Ctrl Pts',(52.6680510665282,12.7728101740752,5.40064510658852));
#68882=CARTESIAN_POINT('Ctrl Pts',(54.2592868143519,13.061508562707,5.47915061696532));
#68883=CARTESIAN_POINT('Ctrl Pts',(54.8961618055507,14.5480818513904,5.55765612734208));
#68884=CARTESIAN_POINT('Ctrl Pts',(54.0075263459451,15.8991766869513,5.63616163771887));
#68885=CARTESIAN_POINT('Ctrl Pts',(52.3902998656124,15.9034183386948,5.71466714809564));
#68886=CARTESIAN_POINT('Ctrl Pts',(51.4949096571851,14.5563621451974,5.79317265847243));
#68887=CARTESIAN_POINT('Ctrl Pts',(52.1242424658418,13.0673662284834,5.8716781688492));
#68888=CARTESIAN_POINT('Ctrl Pts',(53.7141364819045,12.7692091902835,5.95018367922599));
#68889=CARTESIAN_POINT('Ctrl Pts',(54.8382871174936,13.9345710493921,6.02868918960276));
#68890=CARTESIAN_POINT('Ctrl Pts',(54.6051420149022,14.9821810145562,6.08102619652062));
#68891=CARTESIAN_POINT('Ctrl Pts',(54.2939324036795,15.3435126586808,6.10719469997954));
#68892=CARTESIAN_POINT('Ctrl Pts',(53.5456972794618,13.0858534785527,1.89280530002046));
#68893=CARTESIAN_POINT('Ctrl Pts',(53.9769033408726,13.2011331552573,1.91897380347939));
#68894=CARTESIAN_POINT('Ctrl Pts',(54.7096734925719,13.8882572273778,1.97131081039724));
#68895=CARTESIAN_POINT('Ctrl Pts',(54.4549945527556,15.3822436559065,2.04981632077402));
#68896=CARTESIAN_POINT('Ctrl Pts',(53.0683438688966,15.9901656940193,2.1283218311508));
#68897=CARTESIAN_POINT('Ctrl Pts',(51.7964381481809,15.1706744155041,2.20682734152758));
#68898=CARTESIAN_POINT('Ctrl Pts',(51.7784029787483,13.6568335586262,2.28533285190436));
#68899=CARTESIAN_POINT('Ctrl Pts',(53.0311841561409,12.807222552836,2.36383836228114));
#68900=CARTESIAN_POINT('Ctrl Pts',(54.4308733711429,13.3833290718535,2.44234387265792));
#68901=CARTESIAN_POINT('Ctrl Pts',(54.722387599062,14.8687181401707,2.5208493830347));
#68902=CARTESIAN_POINT('Ctrl Pts',(53.6441944994167,15.9311423905248,2.59935489341147));
#68903=CARTESIAN_POINT('Ctrl Pts',(52.1632908429905,15.6178518747085,2.67786040378825));
#68904=CARTESIAN_POINT('Ctrl Pts',(51.6077625312453,14.2097843822215,2.75636591416503));
#68905=CARTESIAN_POINT('Ctrl Pts',(52.4758323736945,12.9697425642164,2.83487142454181));
#68906=CARTESIAN_POINT('Ctrl Pts',(53.9889888117966,13.0098183025906,2.91337693491859));
#68907=CARTESIAN_POINT('Ctrl Pts',(54.7902001121604,14.2940742610093,2.99188244529538));
#68908=CARTESIAN_POINT('Ctrl Pts',(54.1609194710247,15.670757401119,3.07038795567215));
#68909=CARTESIAN_POINT('Ctrl Pts',(52.6655014561621,15.9052264328705,3.14889346604893));
#68910=CARTESIAN_POINT('Ctrl Pts',(51.645072131786,14.7872035164841,3.22739897642571));
#68911=CARTESIAN_POINT('Ctrl Pts',(52.0147769562332,13.3193584010816,3.30590448680249));
#68912=CARTESIAN_POINT('Ctrl Pts',(53.4430557635525,12.818089373422,3.38440999717927));
#68913=CARTESIAN_POINT('Ctrl Pts',(54.648994208884,13.7329464686964,3.46291550755605));
#68914=CARTESIAN_POINT('Ctrl Pts',(54.5510780025192,15.2434640673703,3.54142101793283));
#68915=CARTESIAN_POINT('Ctrl Pts',(53.2371207373081,15.9949740899159,3.61992652830961));
#68916=CARTESIAN_POINT('Ctrl Pts',(51.8855105206782,15.3135044752707,3.69843203868638));
#68917=CARTESIAN_POINT('Ctrl Pts',(51.7084035303663,13.8102133782203,3.77693754906317));
#68918=CARTESIAN_POINT('Ctrl Pts',(52.8646335243838,12.8332879916007,3.85544305943994));
#68919=CARTESIAN_POINT('Ctrl Pts',(54.3172659569832,13.2588582281004,3.93394856981673));
#68920=CARTESIAN_POINT('Ctrl Pts',(54.7635455279197,14.7052625817266,4.0124540801935));
#68921=CARTESIAN_POINT('Ctrl Pts',(53.8032381084338,15.875331242325,4.09095959057029));
#68922=CARTESIAN_POINT('Ctrl Pts',(52.2975702222875,15.7197188176431,4.16946510094706));
#68923=CARTESIAN_POINT('Ctrl Pts',(51.5968606249235,14.377982230734,4.24797061132384));
#68924=CARTESIAN_POINT('Ctrl Pts',(52.329522341856,13.0534227485195,4.32647612170062));
#68925=CARTESIAN_POINT('Ctrl Pts',(53.8384869269094,12.9339368085841,4.4049816320774));
#68926=CARTESIAN_POINT('Ctrl Pts',(54.7704790674375,14.1266822337971,4.48348714245418));
#68927=CARTESIAN_POINT('Ctrl Pts',(54.289666053338,15.5619765883372,4.56199265283096));
#68928=CARTESIAN_POINT('Ctrl Pts',(52.8272524296091,15.9526137379533,4.64049816320774));
#68929=CARTESIAN_POINT('Ctrl Pts',(51.6947654943235,14.9482610700929,4.71900367358452));
#68930=CARTESIAN_POINT('Ctrl Pts',(51.9078464675881,13.4496457937646,4.7975091839613));
#68931=CARTESIAN_POINT('Ctrl Pts',(53.2753992403664,12.8007619985498,4.87601469433808));
#68932=CARTESIAN_POINT('Ctrl Pts',(54.5709700275071,13.5835435319795,4.95452020471486));
#68933=CARTESIAN_POINT('Ctrl Pts',(54.6326600399502,15.095974441783,5.03302571509164));
#68934=CARTESIAN_POINT('Ctrl Pts',(53.4051444220927,15.9816684515245,5.11153122546842));
#68935=CARTESIAN_POINT('Ctrl Pts',(51.9892879328089,15.4463186933993,5.19003673584519));
#68936=CARTESIAN_POINT('Ctrl Pts',(51.6548651940858,13.970030374549,5.26854224622198));
#68937=CARTESIAN_POINT('Ctrl Pts',(52.7017927380267,12.8767923836913,5.34704775659875));
#68938=CARTESIAN_POINT('Ctrl Pts',(54.1911645263585,13.147009562983,5.42555326697554));
#68939=CARTESIAN_POINT('Ctrl Pts',(54.7872695635179,14.5384189254744,5.50405877735231));
#68940=CARTESIAN_POINT('Ctrl Pts',(53.9555206630434,15.8030225734238,5.5825642877291));
#68941=CARTESIAN_POINT('Ctrl Pts',(52.4418219553284,15.806992693157,5.66106979810588));
#68942=CARTESIAN_POINT('Ctrl Pts',(51.603750715536,14.5461691510535,5.73957530848265));
#68943=CARTESIAN_POINT('Ctrl Pts',(52.1927963877232,13.1524922465921,5.81808081885944));
#68944=CARTESIAN_POINT('Ctrl Pts',(53.6809123360987,12.873421919147,5.89658632923621));
#68945=CARTESIAN_POINT('Ctrl Pts',(54.7330997601003,13.9641824042154,5.975091839613));
#68946=CARTESIAN_POINT('Ctrl Pts',(54.5148795882229,14.9447289570596,6.02742884653085));
#68947=CARTESIAN_POINT('Ctrl Pts',(54.2235922564453,15.2829297282066,6.05359734998977));
#68948=CARTESIAN_POINT('Ctrl Pts',(53.5217210200197,13.1755371825404,1.83920795003069));
#68949=CARTESIAN_POINT('Ctrl Pts',(53.923435213036,13.2829324314546,1.86537645348962));
#68950=CARTESIAN_POINT('Ctrl Pts',(54.6060883492027,13.9230614018842,1.91771346040747));
#68951=CARTESIAN_POINT('Ctrl Pts',(54.36882789778,15.3148682576366,1.99621897078425));
#68952=CARTESIAN_POINT('Ctrl Pts',(53.0770156754767,15.8812121308145,2.07472448116103));
#68953=CARTESIAN_POINT('Ctrl Pts',(51.8921005596774,15.117769064742,2.15322999153781));
#68954=CARTESIAN_POINT('Ctrl Pts',(51.8752988859931,13.7074657026187,2.23173550191459));
#68955=CARTESIAN_POINT('Ctrl Pts',(53.042397460757,12.9159629151763,2.31024101229137));
#68956=CARTESIAN_POINT('Ctrl Pts',(54.3463564580827,13.4526672569968,2.38874652266814));
#68957=CARTESIAN_POINT('Ctrl Pts',(54.6179328882426,14.836464759615,2.46725203304492));
#68958=CARTESIAN_POINT('Ctrl Pts',(53.6134816300145,15.8262256618051,2.5457575434217));
#68959=CARTESIAN_POINT('Ctrl Pts',(52.2338627644319,15.5343623092145,2.62426305379848));
#68960=CARTESIAN_POINT('Ctrl Pts',(51.7163292058352,14.222598057557,2.70276856417526));
#68961=CARTESIAN_POINT('Ctrl Pts',(52.5250283579303,13.0673675475858,2.78127407455204));
#68962=CARTESIAN_POINT('Ctrl Pts',(53.9346941113537,13.1047023495315,2.85977958492882));
#68963=CARTESIAN_POINT('Ctrl Pts',(54.6811074384486,14.3011230219925,2.9382850953056));
#68964=CARTESIAN_POINT('Ctrl Pts',(54.0948657606125,15.5836494198329,3.01679060568238));
#68965=CARTESIAN_POINT('Ctrl Pts',(52.7017252303127,15.8020821978165,3.09529611605916));
#68966=CARTESIAN_POINT('Ctrl Pts',(51.7510870569283,14.7605252397341,3.17380162643594));
#68967=CARTESIAN_POINT('Ctrl Pts',(52.0955063230238,13.3930717905004,3.25230713681272));
#68968=CARTESIAN_POINT('Ctrl Pts',(53.4260995586735,12.9260865114173,3.33081264718949));
#68969=CARTESIAN_POINT('Ctrl Pts',(54.5495591589596,13.7783729531961,3.40931815756628));
#68970=CARTESIAN_POINT('Ctrl Pts',(54.4583398247639,15.1855803477368,3.48782366794305));
#68971=CARTESIAN_POINT('Ctrl Pts',(53.234249234003,15.8856916617167,3.56632917831984));
#68972=CARTESIAN_POINT('Ctrl Pts',(51.97508092438,15.250830418309,3.64483468869661));
#68973=CARTESIAN_POINT('Ctrl Pts',(51.8100869735575,13.8503552766928,3.7233401990734));
#68974=CARTESIAN_POINT('Ctrl Pts',(52.8872378778566,12.9402456366778,3.80184570945017));
#68975=CARTESIAN_POINT('Ctrl Pts',(54.2405190991399,13.3367094608825,3.88035121982696));
#68976=CARTESIAN_POINT('Ctrl Pts',(54.6562758654336,14.6841885658631,3.95885673020373));
#68977=CARTESIAN_POINT('Ctrl Pts',(53.7616476248098,15.7742316562315,4.03736224058052));
#68978=CARTESIAN_POINT('Ctrl Pts',(52.3589582519966,15.62926217366,4.11586775095729));
#68979=CARTESIAN_POINT('Ctrl Pts',(51.7061729235091,14.3792921976189,4.19437326133407));
#68980=CARTESIAN_POINT('Ctrl Pts',(52.3887250411869,13.1453245169262,4.27287877171086));
#68981=CARTESIAN_POINT('Ctrl Pts',(53.7944856387802,13.0340106875684,4.35138428208763));
#68982=CARTESIAN_POINT('Ctrl Pts',(54.6627351930762,14.1451795899617,4.42988979246442));
#68983=CARTESIAN_POINT('Ctrl Pts',(54.2148068608103,15.4823085521296,4.50839530284119));
#68984=CARTESIAN_POINT('Ctrl Pts',(52.8524134222997,15.8462284998381,4.58690081321797));
#68985=CARTESIAN_POINT('Ctrl Pts',(51.7973816961194,14.9105674375766,4.66540632359475));
#68986=CARTESIAN_POINT('Ctrl Pts',(51.9958892285554,13.5144483190228,4.74391183397153));
#68987=CARTESIAN_POINT('Ctrl Pts',(53.2699097205826,12.9099442234561,4.82241734434831));
#68988=CARTESIAN_POINT('Ctrl Pts',(54.4768713563924,13.6391882674309,4.90092285472509));
#68989=CARTESIAN_POINT('Ctrl Pts',(54.5343421476997,15.0481781142727,4.97942836510187));
#68990=CARTESIAN_POINT('Ctrl Pts',(53.3907811220753,15.873296047955,5.05793387547865));
#68991=CARTESIAN_POINT('Ctrl Pts',(52.0717605935641,15.3745609528057,5.13643938585542));
#68992=CARTESIAN_POINT('Ctrl Pts',(51.7602103334102,13.9992417638178,5.21494489623221));
#68993=CARTESIAN_POINT('Ctrl Pts',(52.7355344095251,12.9807745933074,5.29345040660898));
#68994=CARTESIAN_POINT('Ctrl Pts',(54.1230422383652,13.232510563259,5.37195591698578));
#68995=CARTESIAN_POINT('Ctrl Pts',(54.6783773214851,14.5287559995584,5.45046142736254));
#68996=CARTESIAN_POINT('Ctrl Pts',(53.9035149801418,15.7068684598963,5.52896693773933));
#68997=CARTESIAN_POINT('Ctrl Pts',(52.4933440450442,15.7105670476193,5.60747244811611));
#68998=CARTESIAN_POINT('Ctrl Pts',(51.7125917738871,14.5359761569097,5.68597795849288));
#68999=CARTESIAN_POINT('Ctrl Pts',(52.2613503096046,13.2376182647008,5.76448346886967));
#69000=CARTESIAN_POINT('Ctrl Pts',(53.6476881902928,12.9776346480105,5.84298897924644));
#69001=CARTESIAN_POINT('Ctrl Pts',(54.6279124027069,13.9937937590388,5.92149448962322));
#69002=CARTESIAN_POINT('Ctrl Pts',(54.4246171615437,14.9072768995629,5.97383149654108));
#69003=CARTESIAN_POINT('Ctrl Pts',(54.153252109211,15.2223467977324,6.));
#69004=CARTESIAN_POINT('Ctrl Pts',(54.4588409672492,14.3981450852038,2.44341967361942));
#69005=CARTESIAN_POINT('Ctrl Pts',(54.4598231909075,14.5245548856247,2.45136379342792));
#69006=CARTESIAN_POINT('Ctrl Pts',(54.4423420959139,14.6506995799382,2.45930791323643));
#69007=CARTESIAN_POINT('Ctrl Pts',(54.4052616068446,14.770791992877,2.46725203304493));
#69008=CARTESIAN_POINT('Ctrl Pts',(54.2831158021666,15.166385060345,2.49342053650386));
#69009=CARTESIAN_POINT('Ctrl Pts',(53.9482987160905,15.4963053610751,2.51958903996278));
#69010=CARTESIAN_POINT('Ctrl Pts',(53.5509536954554,15.6126216193417,2.54575754342171));
#69011=CARTESIAN_POINT('Ctrl Pts',(53.1536086748203,15.7289378776082,2.57192604688064));
#69012=CARTESIAN_POINT('Ctrl Pts',(52.6937357196261,15.6316500934114,2.59809455033956));
#69013=CARTESIAN_POINT('Ctrl Pts',(52.3775436489295,15.3643788260367,2.62426305379849));
#69014=CARTESIAN_POINT('Ctrl Pts',(52.061351578233,15.097107558662,2.65043155725741));
#69015=CARTESIAN_POINT('Ctrl Pts',(51.8888403920341,14.6598528081095,2.67660006071634));
#69016=CARTESIAN_POINT('Ctrl Pts',(51.9373679909505,14.2486870145047,2.70276856417527));
#69017=CARTESIAN_POINT('Ctrl Pts',(51.9858955898669,13.8375212208999,2.7289370676342));
#69018=CARTESIAN_POINT('Ctrl Pts',(52.2554619738986,13.4524443842429,2.75510557109312));
#69019=CARTESIAN_POINT('Ctrl Pts',(52.6251894581517,13.2661284329053,2.78127407455205));
#69020=CARTESIAN_POINT('Ctrl Pts',(52.9949169424048,13.0798124815677,2.80744257801097));
#69021=CARTESIAN_POINT('Ctrl Pts',(53.4648055268793,13.0922574155496,2.8336110814699));
#69022=CARTESIAN_POINT('Ctrl Pts',(53.824152040299,13.2978833279507,2.85977958492883));
#69023=CARTESIAN_POINT('Ctrl Pts',(54.1834985537187,13.5035092403518,2.88594808838775));
#69024=CARTESIAN_POINT('Ctrl Pts',(54.4323029960837,13.9023161311722,2.91211659184668));
#69025=CARTESIAN_POINT('Ctrl Pts',(54.4589982709602,14.3154739762224,2.93828509530561));
#69026=CARTESIAN_POINT('Ctrl Pts',(54.4607442500488,14.342496172514,2.93999662141021));
#69027=CARTESIAN_POINT('Ctrl Pts',(54.4615401150314,14.3695797577353,2.94170814751482));
#69028=CARTESIAN_POINT('Ctrl Pts',(54.4614103817624,14.3966710984295,2.94341967361942));
#69029=CARTESIAN_POINT('Ctrl Pts',(53.5936497983459,12.9064860705774,2.));
#69030=CARTESIAN_POINT('Ctrl Pts',(53.6510872607052,12.9274734829173,2.));
#69031=CARTESIAN_POINT('Ctrl Pts',(53.7069621322555,12.9520730502145,2.));
#69032=CARTESIAN_POINT('Ctrl Pts',(53.7610764088156,12.9799849419358,2.));
#69033=CARTESIAN_POINT('Ctrl Pts',(53.8148756915179,13.0077343612929,2.));
#69034=CARTESIAN_POINT('Ctrl Pts',(53.8669355047627,13.0387586838188,2.));
#69035=CARTESIAN_POINT('Ctrl Pts',(53.9170293533885,13.0728080082457,2.));
#69036=CARTESIAN_POINT('Ctrl Pts',(53.9548563761383,13.0985194399892,2.));
#69037=CARTESIAN_POINT('Ctrl Pts',(53.9915618038207,13.1259567612843,2.));
#69038=CARTESIAN_POINT('Ctrl Pts',(54.0270323602661,13.1550241879185,2.));
#69039=CARTESIAN_POINT('Ctrl Pts',(54.0454462553229,13.1701140144464,2.));
#69040=CARTESIAN_POINT('Ctrl Pts',(54.0635271127833,13.1856432908818,2.));
#69041=CARTESIAN_POINT('Ctrl Pts',(54.0812573827311,13.2015993500241,2.));
#69042=CARTESIAN_POINT('Ctrl Pts',(54.0905947396254,13.2100023477944,2.));
#69043=CARTESIAN_POINT('Ctrl Pts',(54.0998362160851,13.2185251993749,2.));
#69044=CARTESIAN_POINT('Ctrl Pts',(54.108963022778,13.2271503421169,2.));
#69045=CARTESIAN_POINT('Ctrl Pts',(54.1519916744371,13.2678138814072,2.));
#69046=CARTESIAN_POINT('Ctrl Pts',(54.1925581151732,13.3108214913442,2.));
#69047=CARTESIAN_POINT('Ctrl Pts',(54.2304545251895,13.3559335740381,2.));
#69048=CARTESIAN_POINT('Ctrl Pts',(54.2675766913303,13.4001239928139,2.));
#69049=CARTESIAN_POINT('Ctrl Pts',(54.3021372566419,13.4463347100738,2.));
#69050=CARTESIAN_POINT('Ctrl Pts',(54.3338978257104,13.4943635014692,2.));
#69051=CARTESIAN_POINT('Ctrl Pts',(54.3568895199349,13.5291318736403,2.));
#69052=CARTESIAN_POINT('Ctrl Pts',(54.3784130414483,13.5648534993931,2.));
#69053=CARTESIAN_POINT('Ctrl Pts',(54.3983614304516,13.6014553928064,2.));
#69054=CARTESIAN_POINT('Ctrl Pts',(54.4087875591326,13.6205855616955,2.));
#69055=CARTESIAN_POINT('Ctrl Pts',(54.418783168127,13.6399562244125,2.));
#69056=CARTESIAN_POINT('Ctrl Pts',(54.4283312993461,13.6595570484094,2.));
#69057=CARTESIAN_POINT('Ctrl Pts',(54.4327718218709,13.6686727484838,2.));
#69058=CARTESIAN_POINT('Ctrl Pts',(54.4371132830354,13.6778337206022,2.));
#69059=CARTESIAN_POINT('Ctrl Pts',(54.4413510256923,13.6870315208254,2.));
#69060=CARTESIAN_POINT('Ctrl Pts',(54.4646885493577,13.7376844032104,2.));
#69061=CARTESIAN_POINT('Ctrl Pts',(54.4849171742244,13.7895200079085,2.));
#69062=CARTESIAN_POINT('Ctrl Pts',(54.5018239464097,13.8423481255187,2.));
#69063=CARTESIAN_POINT('Ctrl Pts',(54.5131364715857,13.8776960561536,2.));
#69064=CARTESIAN_POINT('Ctrl Pts',(54.5229608260296,13.9134887100648,2.));
#69065=CARTESIAN_POINT('Ctrl Pts',(54.5312202420661,13.9496710849604,2.));
#69066=CARTESIAN_POINT('Ctrl Pts',(54.5434447189016,14.0032233702325,2.));
#69067=CARTESIAN_POINT('Ctrl Pts',(54.5522427226731,14.0576303083872,2.));
#69068=CARTESIAN_POINT('Ctrl Pts',(54.5576688283951,14.1125811869758,2.));
#69069=CARTESIAN_POINT('Ctrl Pts',(54.5593446193984,14.1295521404888,2.));
#69070=CARTESIAN_POINT('Ctrl Pts',(54.5606984801865,14.1465748861843,2.));
#69071=CARTESIAN_POINT('Ctrl Pts',(54.5617312008431,14.1636399586999,2.));
#69072=CARTESIAN_POINT('Ctrl Pts',(54.562637534785,14.1786165686302,2.));
#69073=CARTESIAN_POINT('Ctrl Pts',(54.5632965181378,14.1936323469634,2.));
#69074=CARTESIAN_POINT('Ctrl Pts',(54.5637080050311,14.2086448003361,2.));
#69075=CARTESIAN_POINT('Ctrl Pts',(54.5652337512309,14.2643092554044,2.));
#69076=CARTESIAN_POINT('Ctrl Pts',(54.5633684846636,14.3200027126169,2.));
#69077=CARTESIAN_POINT('Ctrl Pts',(54.5582160449964,14.3754072804563,2.));
#69078=CARTESIAN_POINT('Ctrl Pts',(54.553069811691,14.4307451108242,2.));
#69079=CARTESIAN_POINT('Ctrl Pts',(54.5446438644413,14.485795888494,2.));
#69080=CARTESIAN_POINT('Ctrl Pts',(54.5329924871137,14.5402275304281,2.));
#69081=CARTESIAN_POINT('Ctrl Pts',(54.5255451328294,14.5750192731003,2.));
#69082=CARTESIAN_POINT('Ctrl Pts',(54.5167790477696,14.6095577033489,2.));
#69083=CARTESIAN_POINT('Ctrl Pts',(54.5066991329774,14.6437495917835,2.));
#69084=CARTESIAN_POINT('Ctrl Pts',(54.501505292657,14.6613675193597,2.));
#69085=CARTESIAN_POINT('Ctrl Pts',(54.4959625199335,14.6788933418954,2.));
#69086=CARTESIAN_POINT('Ctrl Pts',(54.4900708072952,14.6963135911134,2.));
#69087=CARTESIAN_POINT('Ctrl Pts',(54.4865172473949,14.706820535847,2.));
#69088=CARTESIAN_POINT('Ctrl Pts',(54.482836847661,14.7172884125644,2.));
#69089=CARTESIAN_POINT('Ctrl Pts',(54.4790344472978,14.7277017731048,2.));
#69090=CARTESIAN_POINT('Ctrl Pts',(54.4606465121801,14.7780594892014,2.));
#69091=CARTESIAN_POINT('Ctrl Pts',(54.4393828187119,14.8272228510089,2.));
#69092=CARTESIAN_POINT('Ctrl Pts',(54.4152842461347,14.8748779185061,2.));
#69093=CARTESIAN_POINT('Ctrl Pts',(54.4001512378004,14.9048035305436,2.));
#69094=CARTESIAN_POINT('Ctrl Pts',(54.3838995195552,14.9341338196499,2.));
#69095=CARTESIAN_POINT('Ctrl Pts',(54.3665318697885,14.9627834478761,2.));
#69096=CARTESIAN_POINT('Ctrl Pts',(54.3601820699915,14.9732580605001,2.));
#69097=CARTESIAN_POINT('Ctrl Pts',(54.3536816777175,14.9836437344145,2.));
#69098=CARTESIAN_POINT('Ctrl Pts',(54.3470352062003,14.9939290625922,2.));
#69099=CARTESIAN_POINT('Ctrl Pts',(54.3191335463469,15.037106518111,2.));
#69100=CARTESIAN_POINT('Ctrl Pts',(54.2887053621599,15.0784511647158,2.));
#69101=CARTESIAN_POINT('Ctrl Pts',(54.2557752604927,15.1176640701999,2.));
#69102=CARTESIAN_POINT('Ctrl Pts',(54.2373775275913,15.1395719455134,2.));
#69103=CARTESIAN_POINT('Ctrl Pts',(54.218198261211,15.1608137789867,2.));
#69104=CARTESIAN_POINT('Ctrl Pts',(54.1982376363281,15.1813315747386,2.));
#69105=CARTESIAN_POINT('Ctrl Pts',(54.1842200551681,15.1957404356268,2.));
#69106=CARTESIAN_POINT('Ctrl Pts',(54.1698170448365,15.2097921118142,2.));
#69107=CARTESIAN_POINT('Ctrl Pts',(54.1550457523822,15.2234791283661,2.));
#69108=CARTESIAN_POINT('Origin',(53.1951359564886,14.3971354987959,4.5));
#69109=CARTESIAN_POINT('Origin',(53.1951359564886,14.3971354987959,7.));
#69110=CARTESIAN_POINT('',(53.1951359564886,14.3971354987959,7.));
#69111=CARTESIAN_POINT('Origin',(53.1951359564886,14.3971354987959,7.));
#69112=CARTESIAN_POINT('',(53.1951359564886,14.3971354987959,7.));
#69113=CARTESIAN_POINT('Origin',(53.1951359564886,14.3971354987959,14.));
#69114=CARTESIAN_POINT('Ctrl Pts',(52.2370198037663,15.2223467977324,14.));
#69115=CARTESIAN_POINT('Ctrl Pts',(52.1998280045505,15.1876146000526,14.));
#69116=CARTESIAN_POINT('Ctrl Pts',(52.1650182492849,15.1505714365259,14.));
#69117=CARTESIAN_POINT('Ctrl Pts',(52.1326048427955,15.1115303634374,14.));
#69118=CARTESIAN_POINT('Ctrl Pts',(52.1107612978531,15.0852204032398,14.));
#69119=CARTESIAN_POINT('Ctrl Pts',(52.0900064961352,15.0580020337776,14.));
#69120=CARTESIAN_POINT('Ctrl Pts',(52.0703516540471,15.0299603098848,14.));
#69121=CARTESIAN_POINT('Ctrl Pts',(52.0612801327296,15.0170178962581,14.));
#69122=CARTESIAN_POINT('Ctrl Pts',(52.0524430088201,15.0038999829769,14.));
#69123=CARTESIAN_POINT('Ctrl Pts',(52.0438418387803,14.990614419731,14.));
#69124=CARTESIAN_POINT('Ctrl Pts',(52.0366118451662,14.9794468068385,14.));
#69125=CARTESIAN_POINT('Ctrl Pts',(52.0295526826659,14.9681669382534,14.));
#69126=CARTESIAN_POINT('Ctrl Pts',(52.0226684754192,14.9567860741714,14.));
#69127=CARTESIAN_POINT('Ctrl Pts',(51.9948472065273,14.9107923862272,14.));
#69128=CARTESIAN_POINT('Ctrl Pts',(51.9698609198898,14.8631221291877,14.));
#69129=CARTESIAN_POINT('Ctrl Pts',(51.947748300213,14.8140997169234,14.));
#69130=CARTESIAN_POINT('Ctrl Pts',(51.9392849993811,14.7953370633544,14.));
#69131=CARTESIAN_POINT('Ctrl Pts',(51.9312430201486,14.7763759159143,14.));
#69132=CARTESIAN_POINT('Ctrl Pts',(51.9236259797524,14.7572330691954,14.));
#69133=CARTESIAN_POINT('Ctrl Pts',(51.9181526522308,14.743477717466,14.));
#69134=CARTESIAN_POINT('Ctrl Pts',(51.912898751984,14.729628533072,14.));
#69135=CARTESIAN_POINT('Ctrl Pts',(51.9078659026536,14.7156915537031,14.));
#69136=CARTESIAN_POINT('Ctrl Pts',(51.9039695334292,14.70490171798,14.));
#69137=CARTESIAN_POINT('Ctrl Pts',(51.900205652679,14.6940588597731,14.));
#69138=CARTESIAN_POINT('Ctrl Pts',(51.8965797111534,14.6831806447376,14.));
#69139=CARTESIAN_POINT('Ctrl Pts',(51.8786612859544,14.6294234395981,14.));
#69140=CARTESIAN_POINT('Ctrl Pts',(51.8640761421609,14.5747200727471,14.));
#69141=CARTESIAN_POINT('Ctrl Pts',(51.8528626358732,14.5194298173159,14.));
#69142=CARTESIAN_POINT('Ctrl Pts',(51.841811607002,14.4649406866733,14.));
#69143=CARTESIAN_POINT('Ctrl Pts',(51.834034827559,14.4098803751302,14.));
#69144=CARTESIAN_POINT('Ctrl Pts',(51.8296128481236,14.3545627855475,14.));
#69145=CARTESIAN_POINT('Ctrl Pts',(51.8273037118361,14.3256762076459,14.));
#69146=CARTESIAN_POINT('Ctrl Pts',(51.8259101526014,14.2967190812183,14.));
#69147=CARTESIAN_POINT('Ctrl Pts',(51.8254490493311,14.267734405596,14.));
#69148=CARTESIAN_POINT('Ctrl Pts',(51.8252016892528,14.2521854991105,14.));
#69149=CARTESIAN_POINT('Ctrl Pts',(51.8252227392438,14.2366286514356,14.));
#69150=CARTESIAN_POINT('Ctrl Pts',(51.8255152855609,14.2210704501588,14.));
#69151=CARTESIAN_POINT('Ctrl Pts',(51.8257232519385,14.210010380103,14.));
#69152=CARTESIAN_POINT('Ctrl Pts',(51.8260684275044,14.1989496253519,14.));
#69153=CARTESIAN_POINT('Ctrl Pts',(51.8265520290691,14.1878905522567,14.));
#69154=CARTESIAN_POINT('Ctrl Pts',(51.8269778211639,14.1781534747891,14.));
#69155=CARTESIAN_POINT('Ctrl Pts',(51.8275105014109,14.1684274977859,14.));
#69156=CARTESIAN_POINT('Ctrl Pts',(51.8281502461767,14.1587149162758,14.));
#69157=CARTESIAN_POINT('Ctrl Pts',(51.8313147365989,14.1106717390517,14.));
#69158=CARTESIAN_POINT('Ctrl Pts',(51.8370971206992,14.0629523055666,14.));
#69159=CARTESIAN_POINT('Ctrl Pts',(51.8455361922423,14.0157553469174,14.));
#69160=CARTESIAN_POINT('Ctrl Pts',(51.8551414270626,13.9620364196253,14.));
#69161=CARTESIAN_POINT('Ctrl Pts',(51.8681865747695,13.9089935983919,14.));
#69162=CARTESIAN_POINT('Ctrl Pts',(51.8844213082608,13.8568249617545,14.));
#69163=CARTESIAN_POINT('Ctrl Pts',(51.9002905362136,13.8058308393547,14.));
#69164=CARTESIAN_POINT('Ctrl Pts',(51.9192079284333,13.7556712969164,14.));
#69165=CARTESIAN_POINT('Ctrl Pts',(51.9409851275901,13.706535068553,14.));
#69166=CARTESIAN_POINT('Ctrl Pts',(51.9463194725345,13.6944991042644,14.));
#69167=CARTESIAN_POINT('Ctrl Pts',(51.9518256037684,13.682524584753,14.));
#69168=CARTESIAN_POINT('Ctrl Pts',(51.9575011215527,13.6706143910571,14.));
#69169=CARTESIAN_POINT('Ctrl Pts',(51.9617861950656,13.6616220739719,14.));
#69170=CARTESIAN_POINT('Ctrl Pts',(51.9661670467641,13.6526682499378,14.));
#69171=CARTESIAN_POINT('Ctrl Pts',(51.970637198385,13.6437643302661,14.));
#69172=CARTESIAN_POINT('Ctrl Pts',(51.9964876791319,13.5922737716532,14.));
#69173=CARTESIAN_POINT('Ctrl Pts',(52.0253653817872,13.5423559816202,14.));
#69174=CARTESIAN_POINT('Ctrl Pts',(52.0569909387869,13.4942262955418,14.));
#69175=CARTESIAN_POINT('Ctrl Pts',(52.0892948739529,13.445064212526,14.));
#69176=CARTESIAN_POINT('Ctrl Pts',(52.1244662109347,13.397766816306,14.));
#69177=CARTESIAN_POINT('Ctrl Pts',(52.1622608705295,13.3525735612502,14.));
#69178=CARTESIAN_POINT('Ctrl Pts',(52.2003880181175,13.3069827311179,14.));
#69179=CARTESIAN_POINT('Ctrl Pts',(52.2411854112565,13.2635321825146,14.));
#69180=CARTESIAN_POINT('Ctrl Pts',(52.2844490106252,13.2224929144142,14.));
#69181=CARTESIAN_POINT('Ctrl Pts',(52.2942488213751,13.2131969458271,14.));
#69182=CARTESIAN_POINT('Ctrl Pts',(52.3041782445982,13.2040224039658,14.));
#69183=CARTESIAN_POINT('Ctrl Pts',(52.3142147727034,13.1949905194826,14.));
#69184=CARTESIAN_POINT('Ctrl Pts',(52.3594366693831,13.154295276801,14.));
#69185=CARTESIAN_POINT('Ctrl Pts',(52.4069027252886,13.1164219434827,14.));
#69186=CARTESIAN_POINT('Ctrl Pts',(52.4563466157764,13.081614036564,14.));
#69187=CARTESIAN_POINT('Ctrl Pts',(52.5053559225274,13.0471120713928,14.));
#69188=CARTESIAN_POINT('Ctrl Pts',(52.5563091707611,13.0156209539409,14.));
#69189=CARTESIAN_POINT('Ctrl Pts',(52.608988780259,12.9874055956648,14.));
#69190=CARTESIAN_POINT('Ctrl Pts',(52.6475874040075,12.9667320559707,14.));
#69191=CARTESIAN_POINT('Ctrl Pts',(52.6871137410246,12.9478176360703,14.));
#69192=CARTESIAN_POINT('Ctrl Pts',(52.7274932936822,12.9307805393251,14.));
#69193=CARTESIAN_POINT('Ctrl Pts',(52.7499343911042,12.9213121048655,14.));
#69194=CARTESIAN_POINT('Ctrl Pts',(52.7726391696466,12.9124237518853,14.));
#69195=CARTESIAN_POINT('Ctrl Pts',(52.7955875161457,12.9041113834231,14.));
#69196=CARTESIAN_POINT('Ctrl Pts',(53.5936497983458,12.9064860705774,14.));
#69197=CARTESIAN_POINT('Ctrl Pts',(53.6509984651359,12.9274410373818,14.));
#69198=CARTESIAN_POINT('Ctrl Pts',(53.706862700368,12.9520247913344,14.));
#69199=CARTESIAN_POINT('Ctrl Pts',(53.7610278853563,12.9799613169679,14.));
#69200=CARTESIAN_POINT('Ctrl Pts',(53.811253157417,13.0058657720284,14.));
#69201=CARTESIAN_POINT('Ctrl Pts',(53.8600177560799,13.0346541103148,14.));
#69202=CARTESIAN_POINT('Ctrl Pts',(53.9071231753153,13.0661362083666,14.));
#69203=CARTESIAN_POINT('Ctrl Pts',(53.9184932356716,13.073735192959,14.));
#69204=CARTESIAN_POINT('Ctrl Pts',(53.9297667856534,13.0814915893148,14.));
#69205=CARTESIAN_POINT('Ctrl Pts',(53.9409284679357,13.0893937512018,14.));
#69206=CARTESIAN_POINT('Ctrl Pts',(53.9900508427055,13.1241710318921,14.));
#69207=CARTESIAN_POINT('Ctrl Pts',(54.0370703143504,13.1618085883035,14.));
#69208=CARTESIAN_POINT('Ctrl Pts',(54.0817574273909,13.2020613662253,14.));
#69209=CARTESIAN_POINT('Ctrl Pts',(54.1093399314821,13.2269068381337,14.));
#69210=CARTESIAN_POINT('Ctrl Pts',(54.1360331112816,13.2527493804774,14.));
#69211=CARTESIAN_POINT('Ctrl Pts',(54.1617745165237,13.2795365304701,14.));
#69212=CARTESIAN_POINT('Ctrl Pts',(54.1705826003212,13.2887024427274,14.));
#69213=CARTESIAN_POINT('Ctrl Pts',(54.1792791848838,13.2979789798834,14.));
#69214=CARTESIAN_POINT('Ctrl Pts',(54.1878615697741,13.3073641129274,14.));
#69215=CARTESIAN_POINT('Ctrl Pts',(54.1958904565107,13.3161439767043,14.));
#69216=CARTESIAN_POINT('Ctrl Pts',(54.2038142460818,13.3250133166843,14.));
#69217=CARTESIAN_POINT('Ctrl Pts',(54.2116272144744,13.3339655512983,14.));
#69218=CARTESIAN_POINT('Ctrl Pts',(54.2502988321281,13.3782761611381,14.));
#69219=CARTESIAN_POINT('Ctrl Pts',(54.286291162459,13.4246505091087,14.));
#69220=CARTESIAN_POINT('Ctrl Pts',(54.3193890208698,13.4728592462875,14.));
#69221=CARTESIAN_POINT('Ctrl Pts',(54.3516418893917,13.5198372121285,14.));
#69222=CARTESIAN_POINT('Ctrl Pts',(54.3811465604862,13.5685580126975,14.));
#69223=CARTESIAN_POINT('Ctrl Pts',(54.4076582516134,13.6188275089931,14.));
#69224=CARTESIAN_POINT('Ctrl Pts',(54.422032099101,13.6460821292118,14.));
#69225=CARTESIAN_POINT('Ctrl Pts',(54.4355253353158,13.6737922214238,14.));
#69226=CARTESIAN_POINT('Ctrl Pts',(54.4480925383866,13.7019277688707,14.));
#69227=CARTESIAN_POINT('Ctrl Pts',(54.4585481854474,13.7253359490609,14.));
#69228=CARTESIAN_POINT('Ctrl Pts',(54.4683627680438,13.7490386437303,14.));
#69229=CARTESIAN_POINT('Ctrl Pts',(54.4775075097945,13.7730185624192,14.));
#69230=CARTESIAN_POINT('Ctrl Pts',(54.4814161888883,13.7832681473069,14.));
#69231=CARTESIAN_POINT('Ctrl Pts',(54.4852027887952,13.7935696368824,14.));
#69232=CARTESIAN_POINT('Ctrl Pts',(54.4888592934221,13.8039047382981,14.));
#69233=CARTESIAN_POINT('Ctrl Pts',(54.5057868221478,13.8517503569829,14.));
#69234=CARTESIAN_POINT('Ctrl Pts',(54.5199611541589,13.9003971685037,14.));
#69235=CARTESIAN_POINT('Ctrl Pts',(54.5312161752957,13.9497022076934,14.));
#69236=CARTESIAN_POINT('Ctrl Pts',(54.5437933673147,14.0047993006142,14.));
#69237=CARTESIAN_POINT('Ctrl Pts',(54.5527257730476,14.0607192933935,14.));
#69238=CARTESIAN_POINT('Ctrl Pts',(54.5581033230396,14.1171258864077,14.));
#69239=CARTESIAN_POINT('Ctrl Pts',(54.5626667133145,14.1649925354187,14.));
#69240=CARTESIAN_POINT('Ctrl Pts',(54.5646690852637,14.2132100479189,14.));
#69241=CARTESIAN_POINT('Ctrl Pts',(54.564136951052,14.2615652592456,14.));
#69242=CARTESIAN_POINT('Ctrl Pts',(54.5639906524104,14.2748594650644,14.));
#69243=CARTESIAN_POINT('Ctrl Pts',(54.5636526398204,14.2881640100039,14.));
#69244=CARTESIAN_POINT('Ctrl Pts',(54.5631231489384,14.3014742844597,14.));
#69245=CARTESIAN_POINT('Ctrl Pts',(54.56271092685,14.3118366708953,14.));
#69246=CARTESIAN_POINT('Ctrl Pts',(54.5621824503514,14.3222043088647,14.));
#69247=CARTESIAN_POINT('Ctrl Pts',(54.5615390812029,14.3325581294009,14.));
#69248=CARTESIAN_POINT('Ctrl Pts',(54.5580964056323,14.3879615398826,14.));
#69249=CARTESIAN_POINT('Ctrl Pts',(54.5513653775396,14.4430731531279,14.));
#69250=CARTESIAN_POINT('Ctrl Pts',(54.5414407207299,14.4975781575777,14.));
#69251=CARTESIAN_POINT('Ctrl Pts',(54.5315715932928,14.5517782014875,14.));
#69252=CARTESIAN_POINT('Ctrl Pts',(54.5185439871748,14.6053794989741,14.));
#69253=CARTESIAN_POINT('Ctrl Pts',(54.5024041440289,14.6580525499533,14.));
#69254=CARTESIAN_POINT('Ctrl Pts',(54.4874293906556,14.7069232818865,14.));
#69255=CARTESIAN_POINT('Ctrl Pts',(54.4697747813692,14.7549954141343,14.));
#69256=CARTESIAN_POINT('Ctrl Pts',(54.4494461022151,14.801978170179,14.));
#69257=CARTESIAN_POINT('Ctrl Pts',(54.444224343838,14.8140464702437,14.));
#69258=CARTESIAN_POINT('Ctrl Pts',(54.4388239492377,14.8260467745287,14.));
#69259=CARTESIAN_POINT('Ctrl Pts',(54.4332573522632,14.8379478523894,14.));
#69260=CARTESIAN_POINT('Ctrl Pts',(54.4107559776874,14.8860545524122,14.));
#69261=CARTESIAN_POINT('Ctrl Pts',(54.385510905493,14.9326200893912,14.));
#69262=CARTESIAN_POINT('Ctrl Pts',(54.35757385594,14.9773487850342,14.));
#69263=CARTESIAN_POINT('Ctrl Pts',(54.3305841286444,15.0205607675808,14.));
#69264=CARTESIAN_POINT('Ctrl Pts',(54.3010813192433,15.0620590194932,14.));
#69265=CARTESIAN_POINT('Ctrl Pts',(54.26907879043,15.1015427316002,14.));
#69266=CARTESIAN_POINT('Ctrl Pts',(54.2466913322504,15.1291636723929,14.));
#69267=CARTESIAN_POINT('Ctrl Pts',(54.2230798921524,15.155798056694,14.));
#69268=CARTESIAN_POINT('Ctrl Pts',(54.1982409588252,15.1813299258066,14.));
#69269=CARTESIAN_POINT('Ctrl Pts',(54.184228995893,15.1957327827604,14.));
#69270=CARTESIAN_POINT('Ctrl Pts',(54.1698262703445,15.2097845594384,14.));
#69271=CARTESIAN_POINT('Ctrl Pts',(54.1550492157916,15.2234767486837,14.));
#69272=CARTESIAN_POINT('Origin',(53.1951359564886,14.3971354987959,19.1042117235887));
#69273=CARTESIAN_POINT('Ctrl Pts',(51.650238794436,14.3978859537331,17.8542117235887));
#69274=CARTESIAN_POINT('Ctrl Pts',(51.6499374336204,14.4458116120497,17.8517311518799));
#69275=CARTESIAN_POINT('Ctrl Pts',(51.673532852059,14.9990358635577,17.8230820767121));
#69276=CARTESIAN_POINT('Ctrl Pts',(52.3387729531489,15.9998443555804,17.7682644980854));
#69277=CARTESIAN_POINT('Ctrl Pts',(54.0595357659419,15.9953385078431,17.6897589877086));
#69278=CARTESIAN_POINT('Ctrl Pts',(55.0050592474358,14.557743765663,17.6112534773318));
#69279=CARTESIAN_POINT('Ctrl Pts',(54.3274128937127,12.9760039404156,17.5327479669551));
#69280=CARTESIAN_POINT('Ctrl Pts',(52.6343075214603,12.6688220685916,17.4542424565783));
#69281=CARTESIAN_POINT('Ctrl Pts',(51.7321085269852,13.6109301706732,17.3947303754562));
#69282=CARTESIAN_POINT('Ctrl Pts',(51.6515351015305,14.2566054984257,17.361386797793));
#69283=CARTESIAN_POINT('Ctrl Pts',(51.6527011247771,14.3958311332086,17.3542117235887));
#69284=CARTESIAN_POINT('Ctrl Pts',(51.6537934596096,14.3955992295121,17.8957882764113));
#69285=CARTESIAN_POINT('Ctrl Pts',(51.6561292792194,14.73752448157,17.8781885106897));
#69286=CARTESIAN_POINT('Ctrl Pts',(51.9349899776299,15.5924054167524,17.8344202415091));
#69287=CARTESIAN_POINT('Ctrl Pts',(53.3392724282712,16.2080937050947,17.7644834688697));
#69288=CARTESIAN_POINT('Ctrl Pts',(54.7851641391705,15.2764790675082,17.6859779584929));
#69289=CARTESIAN_POINT('Ctrl Pts',(54.8056647755616,13.5555715973232,17.6074724481161));
#69290=CARTESIAN_POINT('Ctrl Pts',(53.3815155728065,12.5897336831025,17.5289669377393));
#69291=CARTESIAN_POINT('Ctrl Pts',(51.9513720532365,13.1783784136204,17.458405547171));
#69292=CARTESIAN_POINT('Ctrl Pts',(51.6558508817824,14.0445039022943,17.4140126600617));
#69293=CARTESIAN_POINT('Ctrl Pts',(51.6531013855762,14.3983675031589,17.3957882764113));
#69294=CARTESIAN_POINT('Ctrl Pts',(54.1532521092111,15.2223467977324,18.));
#69295=CARTESIAN_POINT('Ctrl Pts',(54.4246171615437,14.9072768995628,17.9738314965411));
#69296=CARTESIAN_POINT('Ctrl Pts',(54.6278752336732,13.9937540324533,17.9214944896232));
#69297=CARTESIAN_POINT('Ctrl Pts',(53.6477056068469,12.9776474013965,17.8429889792464));
#69298=CARTESIAN_POINT('Ctrl Pts',(52.2613397426835,13.2376039347743,17.7644834688697));
#69299=CARTESIAN_POINT('Ctrl Pts',(51.7125907601688,14.5359830763926,17.6859779584929));
#69300=CARTESIAN_POINT('Ctrl Pts',(52.4933400927666,15.7105673519417,17.6074724481161));
#69301=CARTESIAN_POINT('Ctrl Pts',(53.9035180427191,15.7068747761389,17.5289669377393));
#69302=CARTESIAN_POINT('Ctrl Pts',(54.6783815828027,14.5287551705091,17.4504614273625));
#69303=CARTESIAN_POINT('Ctrl Pts',(54.1230453454192,13.2325075949904,17.3719559169858));
#69304=CARTESIAN_POINT('Ctrl Pts',(52.7355328741209,12.9807697615999,17.293450406609));
#69305=CARTESIAN_POINT('Ctrl Pts',(51.760205867286,13.9992407208286,17.2149448962322));
#69306=CARTESIAN_POINT('Ctrl Pts',(52.0717570426273,15.3745639123133,17.1364393858554));
#69307=CARTESIAN_POINT('Ctrl Pts',(53.3907817466691,15.8733007472588,17.0579338754786));
#69308=CARTESIAN_POINT('Ctrl Pts',(54.5343463517261,15.0481801280675,16.9794283651019));
#69309=CARTESIAN_POINT('Ctrl Pts',(54.4768753865949,13.6391859025932,16.9009228547251));
#69310=CARTESIAN_POINT('Ctrl Pts',(53.2699099545465,12.9099395406962,16.8224173443483));
#69311=CARTESIAN_POINT('Ctrl Pts',(51.9958854602388,13.5144455498356,16.7439118339715));
#69312=CARTESIAN_POINT('Ctrl Pts',(51.7973773032627,14.9105690485956,16.6654063235947));
#69313=CARTESIAN_POINT('Ctrl Pts',(52.8524123453517,15.8462330551256,16.586900813218));
#69314=CARTESIAN_POINT('Ctrl Pts',(54.2148100652166,15.4823119617458,16.5083953028412));
#69315=CARTESIAN_POINT('Ctrl Pts',(54.6627398052286,14.1451787985144,16.4298897924644));
#69316=CARTESIAN_POINT('Ctrl Pts',(53.7944875223078,13.0340064035767,16.3513842820876));
#69317=CARTESIAN_POINT('Ctrl Pts',(52.3887225069356,13.145320583037,16.2728787717108));
#69318=CARTESIAN_POINT('Ctrl Pts',(51.7061682442381,14.3792921414933,16.1943732613341));
#69319=CARTESIAN_POINT('Ctrl Pts',(52.3589556241958,15.6292660458125,16.1158677509573));
#69320=CARTESIAN_POINT('Ctrl Pts',(53.7616494051485,15.7742359839284,16.0373622405805));
#69321=CARTESIAN_POINT('Ctrl Pts',(54.6562804572665,14.6841894679762,15.9588567302037));
#69322=CARTESIAN_POINT('Ctrl Pts',(54.2405223843949,13.33670612834,15.880351219827));
#69323=CARTESIAN_POINT('Ctrl Pts',(52.8872369102521,12.9402410582164,15.8018457094502));
#69324=CARTESIAN_POINT('Ctrl Pts',(51.8100826208389,13.8503535583388,15.7233401990734));
#69325=CARTESIAN_POINT('Ctrl Pts',(51.9750770902176,15.2508331012045,15.6448346886966));
#69326=CARTESIAN_POINT('Ctrl Pts',(53.2342493568711,15.885696339624,15.5663291783198));
#69327=CARTESIAN_POINT('Ctrl Pts',(54.4583437946506,15.1855828256918,15.4878236679431));
#69328=CARTESIAN_POINT('Ctrl Pts',(54.549563415235,13.7783710083419,15.4093181575663));
#69329=CARTESIAN_POINT('Ctrl Pts',(53.4261002848556,12.9260818890411,15.3308126471895));
#69330=CARTESIAN_POINT('Ctrl Pts',(52.0955028666328,13.393068633948,15.2523071368127));
#69331=CARTESIAN_POINT('Ctrl Pts',(51.7510825200381,14.7605263839363,15.1738016264359));
#69332=CARTESIAN_POINT('Ctrl Pts',(52.7017236774067,15.8020866088358,15.0952961160592));
#69333=CARTESIAN_POINT('Ctrl Pts',(54.0948685923953,15.5836531566747,15.0167906056824));
#69334=CARTESIAN_POINT('Ctrl Pts',(54.6811121004696,14.3011227048956,14.9382850953056));
#69335=CARTESIAN_POINT('Ctrl Pts',(53.9346964498465,13.1046983170808,14.8597795849288));
#69336=CARTESIAN_POINT('Ctrl Pts',(52.5250262261246,13.0673633133234,14.7812740745521));
#69337=CARTESIAN_POINT('Ctrl Pts',(51.7163246046947,14.2225976133251,14.7027685641753));
#69338=CARTESIAN_POINT('Ctrl Pts',(52.2338596624079,15.5343656873115,14.6242630537985));
#69339=CARTESIAN_POINT('Ctrl Pts',(53.6134830839557,15.8262305186475,14.5457575434217));
#69340=CARTESIAN_POINT('Ctrl Pts',(54.6179371276052,14.8364654611899,14.4672520330449));
#69341=CARTESIAN_POINT('Ctrl Pts',(54.3463604457024,13.4526655408848,14.3887465226681));
#69342=CARTESIAN_POINT('Ctrl Pts',(53.0423964320332,12.9159559714002,14.3102410122914));
#69343=CARTESIAN_POINT('Ctrl Pts',(51.8752954493437,13.7074676781063,14.2317355019146));
#69344=CARTESIAN_POINT('Ctrl Pts',(51.892095823422,15.1177639193799,14.1532299915378));
#69345=CARTESIAN_POINT('Ctrl Pts',(53.0770150197732,15.881229923416,14.074724481161));
#69346=CARTESIAN_POINT('Ctrl Pts',(54.3688351006162,15.3148479080821,13.9962189707842));
#69347=CARTESIAN_POINT('Ctrl Pts',(54.6060800258316,13.9231151648839,13.9177134604075));
#69348=CARTESIAN_POINT('Ctrl Pts',(53.9234352130359,13.2829324314546,13.8653764534896));
#69349=CARTESIAN_POINT('Ctrl Pts',(53.5217210200197,13.1755371825403,13.8392079500307));
#69350=CARTESIAN_POINT('Ctrl Pts',(54.2235922564453,15.2829297282065,18.0535973499898));
#69351=CARTESIAN_POINT('Ctrl Pts',(54.514879588223,14.9447289570595,18.0274288465308));
#69352=CARTESIAN_POINT('Ctrl Pts',(54.7330598623,13.9641397611006,17.975091839613));
#69353=CARTESIAN_POINT('Ctrl Pts',(53.68093103129,12.8734356088235,17.8965863292362));
#69354=CARTESIAN_POINT('Ctrl Pts',(52.192785045031,13.1524768646333,17.8180808188594));
#69355=CARTESIAN_POINT('Ctrl Pts',(51.6037496273956,14.5461765785306,17.7395753084826));
#69356=CARTESIAN_POINT('Ctrl Pts',(52.441817712894,15.8069930198213,17.6610697981059));
#69357=CARTESIAN_POINT('Ctrl Pts',(53.95552395046,15.8030293533737,17.5825642877291));
#69358=CARTESIAN_POINT('Ctrl Pts',(54.7872741376804,14.5384180355604,17.5040587773523));
#69359=CARTESIAN_POINT('Ctrl Pts',(54.191167861517,13.1470063767988,17.4255532669756));
#69360=CARTESIAN_POINT('Ctrl Pts',(52.7017910899008,12.8767871972638,17.3470477565987));
#69361=CARTESIAN_POINT('Ctrl Pts',(51.6548604000808,13.9700292549887,17.268542246222));
#69362=CARTESIAN_POINT('Ctrl Pts',(51.9892841211801,15.4463218701793,17.1900367358452));
#69363=CARTESIAN_POINT('Ctrl Pts',(53.4051450925409,15.9816734958279,17.1115312254684));
#69364=CARTESIAN_POINT('Ctrl Pts',(54.6326645526155,15.0959766034206,17.0330257150917));
#69365=CARTESIAN_POINT('Ctrl Pts',(54.570974353587,13.5835409935271,16.9545202047148));
#69366=CARTESIAN_POINT('Ctrl Pts',(53.2753994915068,12.8007569720048,16.8760146943381));
#69367=CARTESIAN_POINT('Ctrl Pts',(51.9078424226204,13.4496428212774,16.7975091839613));
#69368=CARTESIAN_POINT('Ctrl Pts',(51.6947607789649,14.9482627993849,16.7190036735845));
#69369=CARTESIAN_POINT('Ctrl Pts',(52.827251273597,15.9526186276675,16.6404981632078));
#69370=CARTESIAN_POINT('Ctrl Pts',(54.2896694929959,15.5619802482706,16.561992652831));
#69371=CARTESIAN_POINT('Ctrl Pts',(54.7704840181913,14.1266813842457,16.4834871424542));
#69372=CARTESIAN_POINT('Ctrl Pts',(53.8384889487162,12.9339322100829,16.4049816320774));
#69373=CARTESIAN_POINT('Ctrl Pts',(52.3295196215527,13.0534185258236,16.3264761217006));
#69374=CARTESIAN_POINT('Ctrl Pts',(51.5968556021234,14.377982170488,16.2479706113238));
#69375=CARTESIAN_POINT('Ctrl Pts',(52.2975674015667,15.7197229740698,16.1694651009471));
#69376=CARTESIAN_POINT('Ctrl Pts',(53.803240019476,15.8753358877401,16.0909595905703));
#69377=CARTESIAN_POINT('Ctrl Pts',(54.7635504568624,14.7052635500684,16.0124540801935));
#69378=CARTESIAN_POINT('Ctrl Pts',(54.3172694834252,13.2588546508992,15.9339485698167));
#69379=CARTESIAN_POINT('Ctrl Pts',(52.8646324857426,12.8332830770114,15.8554430594399));
#69380=CARTESIAN_POINT('Ctrl Pts',(51.7083988580925,13.8102115337132,15.7769375490632));
#69381=CARTESIAN_POINT('Ctrl Pts',(51.8855064050308,15.3135073551311,15.6984320386864));
#69382=CARTESIAN_POINT('Ctrl Pts',(53.2371208691965,15.994979111252,15.6199265283096));
#69383=CARTESIAN_POINT('Ctrl Pts',(54.5510822638553,15.2434667272446,15.5414210179328));
#69384=CARTESIAN_POINT('Ctrl Pts',(54.6489987776341,13.7329443810606,15.4629155075561));
#69385=CARTESIAN_POINT('Ctrl Pts',(53.4430565430473,12.8180844116938,15.3844099971793));
#69386=CARTESIAN_POINT('Ctrl Pts',(52.0147732460911,13.3193550127907,15.3059044868025));
#69387=CARTESIAN_POINT('Ctrl Pts',(51.6450672618196,14.787204744688,15.2273989764257));
#69388=CARTESIAN_POINT('Ctrl Pts',(52.6654997892496,15.9052311677249,15.1488934660489));
#69389=CARTESIAN_POINT('Ctrl Pts',(54.1609225107029,15.6707614123012,15.0703879556721));
#69390=CARTESIAN_POINT('Ctrl Pts',(54.7902051164439,14.2940739206327,14.9918824452954));
#69391=CARTESIAN_POINT('Ctrl Pts',(53.9889913219699,13.0098139740974,14.9133769349186));
#69392=CARTESIAN_POINT('Ctrl Pts',(52.4758300853821,12.9697380190954,14.8348714245418));
#69393=CARTESIAN_POINT('Ctrl Pts',(51.6077575923118,14.2097839053763,14.756365914165));
#69394=CARTESIAN_POINT('Ctrl Pts',(52.1632875132313,15.6178555008087,14.6778604037883));
#69395=CARTESIAN_POINT('Ctrl Pts',(53.644196060099,15.9311476039325,14.5993548934115));
#69396=CARTESIAN_POINT('Ctrl Pts',(54.7223921496577,14.8687188932518,14.5208493830347));
#69397=CARTESIAN_POINT('Ctrl Pts',(54.4308776515139,13.3833272297531,14.4423438726579));
#69398=CARTESIAN_POINT('Ctrl Pts',(53.0311830518933,12.8072150992822,14.3638383622811));
#69399=CARTESIAN_POINT('Ctrl Pts',(51.7783992897971,13.6568356791444,14.2853328519044));
#69400=CARTESIAN_POINT('Ctrl Pts',(51.7964330642131,15.1706688923949,14.2068273415276));
#69401=CARTESIAN_POINT('Ctrl Pts',(53.0683431650545,15.9901847928655,14.1283218311508));
#69402=CARTESIAN_POINT('Ctrl Pts',(54.4550022843884,15.3822218123885,14.049816320774));
#69403=CARTESIAN_POINT('Ctrl Pts',(54.70966455814,13.888314937391,13.9713108103972));
#69404=CARTESIAN_POINT('Ctrl Pts',(53.9769033408726,13.2011331552573,13.9189738034794));
#69405=CARTESIAN_POINT('Ctrl Pts',(53.5456972794617,13.0858534785527,13.8928053000205));
#69406=CARTESIAN_POINT('Ctrl Pts',(54.2939324036796,15.3435126586807,18.1071946999795));
#69407=CARTESIAN_POINT('Ctrl Pts',(54.6051420149022,14.9821810145562,18.0810261965206));
#69408=CARTESIAN_POINT('Ctrl Pts',(54.8382444909268,13.934525489748,18.0286891896028));
#69409=CARTESIAN_POINT('Ctrl Pts',(53.714156455733,12.7692238162505,17.950183679226));
#69410=CARTESIAN_POINT('Ctrl Pts',(52.1242303473785,13.0673497944923,17.8716781688492));
#69411=CARTESIAN_POINT('Ctrl Pts',(51.4949084946224,14.5563700806686,17.7931726584724));
#69412=CARTESIAN_POINT('Ctrl Pts',(52.3902953330215,15.9034186877009,17.7146671480956));
#69413=CARTESIAN_POINT('Ctrl Pts',(54.0075298582009,15.8991839306084,17.6361616377189));
#69414=CARTESIAN_POINT('Ctrl Pts',(54.8961666925582,14.5480809006117,17.5576561273421));
#69415=CARTESIAN_POINT('Ctrl Pts',(54.2592903776148,13.0615051586072,17.4791506169653));
#69416=CARTESIAN_POINT('Ctrl Pts',(52.6680493056806,12.7728046329277,17.4006451065885));
#69417=CARTESIAN_POINT('Ctrl Pts',(51.5495149328755,13.9408177891487,17.3221395962118));
#69418=CARTESIAN_POINT('Ctrl Pts',(51.9068111997328,15.5180798280453,17.2436340858349));
#69419=CARTESIAN_POINT('Ctrl Pts',(53.4195084384129,16.090046244397,17.1651285754582));
#69420=CARTESIAN_POINT('Ctrl Pts',(54.7309827535048,15.1437730787738,17.0866230650814));
#69421=CARTESIAN_POINT('Ctrl Pts',(54.6650733205791,13.5278960844609,17.0081175547046));
#69422=CARTESIAN_POINT('Ctrl Pts',(53.2808890284672,12.6915744033134,16.9296120443278));
#69423=CARTESIAN_POINT('Ctrl Pts',(51.8197993850019,13.3848400927192,16.8511065339511));
#69424=CARTESIAN_POINT('Ctrl Pts',(51.5921442546672,14.9859565501742,16.7726010235743));
#69425=CARTESIAN_POINT('Ctrl Pts',(52.8020902018422,16.0590042002094,16.6940955131975));
#69426=CARTESIAN_POINT('Ctrl Pts',(54.3645289207752,15.6416485347953,16.6155900028207));
#69427=CARTESIAN_POINT('Ctrl Pts',(54.8782282311541,14.108183969977,16.5370844924439));
#69428=CARTESIAN_POINT('Ctrl Pts',(53.8824903751247,12.8338580165892,16.4585789820672));
#69429=CARTESIAN_POINT('Ctrl Pts',(52.2703167361696,12.9615164686103,16.3800734716904));
#69430=CARTESIAN_POINT('Ctrl Pts',(51.4875429600088,14.3766721994827,16.3015679613136));
#69431=CARTESIAN_POINT('Ctrl Pts',(52.2361791789377,15.8101799023271,16.2230624509368));
#69432=CARTESIAN_POINT('Ctrl Pts',(53.8448306338036,15.9764357915517,16.1445569405601));
#69433=CARTESIAN_POINT('Ctrl Pts',(54.8708204564582,14.7263376321606,16.0660514301832));
#69434=CARTESIAN_POINT('Ctrl Pts',(54.3940165824556,13.1810031734583,15.9875459198065));
#69435=CARTESIAN_POINT('Ctrl Pts',(52.8420280612332,12.7263250958063,15.9090404094297));
#69436=CARTESIAN_POINT('Ctrl Pts',(51.6067150953461,13.7700695090875,15.8305348990529));
#69437=CARTESIAN_POINT('Ctrl Pts',(51.7959357198439,15.3761816090578,15.7520293886761));
#69438=CARTESIAN_POINT('Ctrl Pts',(53.239992381522,16.1042618828799,15.6735238782994));
#69439=CARTESIAN_POINT('Ctrl Pts',(54.64382073306,15.3013506287974,15.5950183679226));
#69440=CARTESIAN_POINT('Ctrl Pts',(54.7484341400331,13.6875177537793,15.5165128575458));
#69441=CARTESIAN_POINT('Ctrl Pts',(53.460012801239,12.7100869343466,15.438007347169));
#69442=CARTESIAN_POINT('Ctrl Pts',(51.9340436255495,13.2456413916334,15.3595018367923));
#69443=CARTESIAN_POINT('Ctrl Pts',(51.5390520036012,14.8138831054397,15.2809963264155));
#69444=CARTESIAN_POINT('Ctrl Pts',(52.6292759010924,16.0083757266141,15.2024908160387));
#69445=CARTESIAN_POINT('Ctrl Pts',(54.2269764290105,15.7578696679277,15.1239853056619));
#69446=CARTESIAN_POINT('Ctrl Pts',(54.8992981324183,14.2870251363698,15.0454797952851));
#69447=CARTESIAN_POINT('Ctrl Pts',(54.0432861940933,12.9149296311139,14.9669742849084));
#69448=CARTESIAN_POINT('Ctrl Pts',(52.4266339446398,12.8721127248674,14.8884687745316));
#69449=CARTESIAN_POINT('Ctrl Pts',(51.4991905799288,14.1969701974276,14.8099632641548));
#69450=CARTESIAN_POINT('Ctrl Pts',(52.0927153640547,15.7013453143059,14.731457753778));
#69451=CARTESIAN_POINT('Ctrl Pts',(53.6749090362422,16.0360646892175,14.6529522434012));
#69452=CARTESIAN_POINT('Ctrl Pts',(54.8268471717102,14.9009723253136,14.5744467330245));
#69453=CARTESIAN_POINT('Ctrl Pts',(54.5153948573254,13.3139889186214,14.4959412226477));
#69454=CARTESIAN_POINT('Ctrl Pts',(53.0199696717534,12.6984742271641,14.4174357122709));
#69455=CARTESIAN_POINT('Ctrl Pts',(51.6815031302505,13.6062036801825,14.3389302018941));
#69456=CARTESIAN_POINT('Ctrl Pts',(51.7007703050042,15.22357386541,14.2604246915173));
#69457=CARTESIAN_POINT('Ctrl Pts',(53.0596713103358,16.099139662315,14.1819191811406));
#69458=CARTESIAN_POINT('Ctrl Pts',(54.5411694681605,15.4495957166949,14.1034136707638));
#69459=CARTESIAN_POINT('Ctrl Pts',(54.8132490904484,13.853514709898,14.024908160387));
#69460=CARTESIAN_POINT('Ctrl Pts',(54.0303714687093,13.11933387906,13.9725711534692));
#69461=CARTESIAN_POINT('Ctrl Pts',(53.5696735389038,12.996169774565,13.9464026500102));
#69462=CARTESIAN_POINT('Ctrl Pts',(54.3642725509139,15.4040955891549,18.1607920499693));
#69463=CARTESIAN_POINT('Ctrl Pts',(54.6954044415815,15.0196330720528,18.1346235465104));
#69464=CARTESIAN_POINT('Ctrl Pts',(54.9434291195537,13.9049112183953,18.0822865395925));
#69465=CARTESIAN_POINT('Ctrl Pts',(53.7473818801761,12.6650120236775,18.0037810292158));
#69466=CARTESIAN_POINT('Ctrl Pts',(52.055675649726,12.9822227243513,17.925275518839));
#69467=CARTESIAN_POINT('Ctrl Pts',(51.3860673618492,14.5665635828067,17.8467700084622));
#69468=CARTESIAN_POINT('Ctrl Pts',(52.3387729531489,15.9998443555804,17.7682644980854));
#69469=CARTESIAN_POINT('Ctrl Pts',(54.0595357659419,15.9953385078431,17.6897589877086));
#69470=CARTESIAN_POINT('Ctrl Pts',(55.0050592474358,14.557743765663,17.6112534773318));
#69471=CARTESIAN_POINT('Ctrl Pts',(54.3274128937127,12.9760039404156,17.5327479669551));
#69472=CARTESIAN_POINT('Ctrl Pts',(52.6343075214603,12.6688220685916,17.4542424565783));
#69473=CARTESIAN_POINT('Ctrl Pts',(51.4441694656704,13.9116063233088,17.3757369462015));
#69474=CARTESIAN_POINT('Ctrl Pts',(51.8243382782854,15.5898377859113,17.2972314358247));
#69475=CARTESIAN_POINT('Ctrl Pts',(53.4338717842849,16.1984189929661,17.2187259254479));
#69476=CARTESIAN_POINT('Ctrl Pts',(54.8293009543941,15.1915695541269,17.1402204150712));
#69477=CARTESIAN_POINT('Ctrl Pts',(54.7591722875712,13.4722511753948,17.0617149046944));
#69478=CARTESIAN_POINT('Ctrl Pts',(53.2863785654276,12.582391834622,16.9832093943176));
#69479=CARTESIAN_POINT('Ctrl Pts',(51.7317563473835,13.320037364161,16.9047038839408));
#69480=CARTESIAN_POINT('Ctrl Pts',(51.4895277303696,15.0236503009635,16.8261983735641));
#69481=CARTESIAN_POINT('Ctrl Pts',(52.7769291300874,16.1653897727513,16.7476928631873));
#69482=CARTESIAN_POINT('Ctrl Pts',(54.4393883485545,15.72131682132,16.6691873528105));
#69483=CARTESIAN_POINT('Ctrl Pts',(54.9859724441168,14.0896865557083,16.5906818424337));
#69484=CARTESIAN_POINT('Ctrl Pts',(53.9264918015332,12.7337838230954,16.5121763320569));
#69485=CARTESIAN_POINT('Ctrl Pts',(52.2111138507866,12.869614411397,16.4336708216802));
#69486=CARTESIAN_POINT('Ctrl Pts',(51.3782303178942,14.3753622284773,16.3551653113034));
#69487=CARTESIAN_POINT('Ctrl Pts',(52.1747909563085,15.9006368305844,16.2766598009266));
#69488=CARTESIAN_POINT('Ctrl Pts',(53.8864212481313,16.0775356953633,16.1981542905498));
#69489=CARTESIAN_POINT('Ctrl Pts',(54.9780904560539,14.7474117142528,16.119648780173));
#69490=CARTESIAN_POINT('Ctrl Pts',(54.4707636814861,13.1031516960174,16.0411432697963));
#69491=CARTESIAN_POINT('Ctrl Pts',(52.8194236367236,12.6193671146013,15.9626377594195));
#69492=CARTESIAN_POINT('Ctrl Pts',(51.5050313325997,13.7299274844619,15.8841322490427));
#69493=CARTESIAN_POINT('Ctrl Pts',(51.706365034657,15.4388558629845,15.8056267386659));
#69494=CARTESIAN_POINT('Ctrl Pts',(53.2428638938474,16.2135446545079,15.7271212282891));
#69495=CARTESIAN_POINT('Ctrl Pts',(54.7365592022647,15.3592345303502,15.6486157179124));
#69496=CARTESIAN_POINT('Ctrl Pts',(54.8478695024322,13.6420911264981,15.5701102075356));
#69497=CARTESIAN_POINT('Ctrl Pts',(53.4769690594307,12.6020894569994,15.4916046971588));
#69498=CARTESIAN_POINT('Ctrl Pts',(51.8533140050078,13.1719277704762,15.413099186782));
#69499=CARTESIAN_POINT('Ctrl Pts',(51.4330367453828,14.8405614661914,15.3345936764053));
#69500=CARTESIAN_POINT('Ctrl Pts',(52.5930520129352,16.1115202855033,15.2560881660285));
#69501=CARTESIAN_POINT('Ctrl Pts',(54.2930303473182,15.8449779235543,15.1775826556517));
#69502=CARTESIAN_POINT('Ctrl Pts',(55.0083911483926,14.2799763521069,15.0990771452749));
#69503=CARTESIAN_POINT('Ctrl Pts',(54.0975810662168,12.8200452881305,15.0205716348981));
#69504=CARTESIAN_POINT('Ctrl Pts',(52.3774378038973,12.7744874306393,14.9420661245214));
#69505=CARTESIAN_POINT('Ctrl Pts',(51.3906235675459,14.1841564894788,14.8635606141446));
#69506=CARTESIAN_POINT('Ctrl Pts',(52.0221432148781,15.7848351278031,14.7850551037678));
#69507=CARTESIAN_POINT('Ctrl Pts',(53.7056220123855,16.1409817745025,14.706549593391));
#69508=CARTESIAN_POINT('Ctrl Pts',(54.9313021937626,14.9332257573755,14.6280440830142));
#69509=CARTESIAN_POINT('Ctrl Pts',(54.5999120631369,13.2446506074896,14.5495385726375));
#69510=CARTESIAN_POINT('Ctrl Pts',(53.0087562916135,12.5897333550461,14.4710330622607));
#69511=CARTESIAN_POINT('Ctrl Pts',(51.584606970704,13.5555716812206,14.3925275518839));
#69512=CARTESIAN_POINT('Ctrl Pts',(51.6051075457953,15.2764788384251,14.3140220415071));
#69513=CARTESIAN_POINT('Ctrl Pts',(53.0509994556171,16.2080945317645,14.2355165311303));
#69514=CARTESIAN_POINT('Ctrl Pts',(54.6273366519326,15.5169696210012,14.1570110207535));
#69515=CARTESIAN_POINT('Ctrl Pts',(54.9168336227569,13.8187144824051,14.0785055103768));
#69516=CARTESIAN_POINT('Ctrl Pts',(54.0838395965459,13.0375346028627,14.0261685034589));
#69517=CARTESIAN_POINT('Ctrl Pts',(53.5936497983458,12.9064860705774,14.));
#69518=CARTESIAN_POINT('Ctrl Pts',(51.9310991161132,14.3960665614756,17.1934196736194));
#69519=CARTESIAN_POINT('Ctrl Pts',(51.9301435513723,14.2819701161205,17.2005947478237));
#69520=CARTESIAN_POINT('Ctrl Pts',(51.944352401566,14.1681074628443,17.2077698220279));
#69521=CARTESIAN_POINT('Ctrl Pts',(51.9746855643154,14.0587160928713,17.2149448962322));
#69522=CARTESIAN_POINT('Ctrl Pts',(52.0853148695643,13.6597504010857,17.2411133996911));
#69523=CARTESIAN_POINT('Ctrl Pts',(52.4104238718426,13.3202600813428,17.26728190315));
#69524=CARTESIAN_POINT('Ctrl Pts',(52.8042304515315,13.1924712270364,17.293450406609));
#69525=CARTESIAN_POINT('Ctrl Pts',(53.1980370312203,13.0646823727301,17.3196189100679));
#69526=CARTESIAN_POINT('Ctrl Pts',(53.6605411883198,13.1485949838602,17.3457874135268));
#69527=CARTESIAN_POINT('Ctrl Pts',(53.9843493064334,13.4065925520117,17.3719559169858));
#69528=CARTESIAN_POINT('Ctrl Pts',(54.308157424547,13.6645901201633,17.3981244204447));
#69529=CARTESIAN_POINT('Ctrl Pts',(54.4932695036749,14.0966726453362,17.4242929239036));
#69530=CARTESIAN_POINT('Ctrl Pts',(54.4566816198915,14.5090671755276,17.4504614273625));
#69531=CARTESIAN_POINT('Ctrl Pts',(54.4200937361082,14.921461705719,17.4766299308215));
#69532=CARTESIAN_POINT('Ctrl Pts',(54.1618058894136,15.314168240929,17.5027984342804));
#69533=CARTESIAN_POINT('Ctrl Pts',(53.7976323077409,15.5111369378344,17.5289669377393));
#69534=CARTESIAN_POINT('Ctrl Pts',(53.4334587260683,15.7081056347399,17.5551354411983));
#69535=CARTESIAN_POINT('Ctrl Pts',(52.9633994094174,15.7093364933408,17.5813039446572));
#69536=CARTESIAN_POINT('Ctrl Pts',(52.5982448623257,15.5141878767164,17.6074724481161));
#69537=CARTESIAN_POINT('Ctrl Pts',(52.233090315234,15.319039260092,17.633640951575));
#69538=CARTESIAN_POINT('Ctrl Pts',(51.9728405377014,14.9275111682423,17.6598094550339));
#69539=CARTESIAN_POINT('Ctrl Pts',(51.9341738126876,14.5153505987144,17.6859779584929));
#69540=CARTESIAN_POINT('Ctrl Pts',(51.9305085062518,14.4762809648747,17.6884585302017));
#69541=CARTESIAN_POINT('Ctrl Pts',(51.9288342506125,14.4370259363911,17.6909391019106));
#69542=CARTESIAN_POINT('Ctrl Pts',(51.929081218047,14.3977505022101,17.6934196736194));
#69543=CARTESIAN_POINT('Ctrl Pts',(52.7966221146313,12.9064860705774,18.));
#69544=CARTESIAN_POINT('Ctrl Pts',(52.3064323164312,13.0375346028627,17.9738314965411));
#69545=CARTESIAN_POINT('Ctrl Pts',(51.4734379005318,13.818711947887,17.9214944896232));
#69546=CARTESIAN_POINT('Ctrl Pts',(51.7629355980163,15.5169705450585,17.8429889792464));
#69547=CARTESIAN_POINT('Ctrl Pts',(53.3392724282712,16.2080937050947,17.7644834688697));
#69548=CARTESIAN_POINT('Ctrl Pts',(54.7851641391705,15.2764790675082,17.6859779584929));
#69549=CARTESIAN_POINT('Ctrl Pts',(54.8056647755616,13.5555715973232,17.6074724481161));
#69550=CARTESIAN_POINT('Ctrl Pts',(53.3815155728065,12.5897336831025,17.5289669377393));
#69551=CARTESIAN_POINT('Ctrl Pts',(51.7903600412662,13.244650694059,17.4504614273625));
#69552=CARTESIAN_POINT('Ctrl Pts',(51.458969924108,14.9332257213624,17.3719559169858));
#69553=CARTESIAN_POINT('Ctrl Pts',(52.6846499703254,16.1409815416267,17.293450406609));
#69554=CARTESIAN_POINT('Ctrl Pts',(54.36812854879,15.7848349642755,17.2149448962322));
#69555=CARTESIAN_POINT('Ctrl Pts',(54.9996481235109,14.1841565112764,17.1364393858554));
#69556=CARTESIAN_POINT('Ctrl Pts',(54.0128340063977,12.7744876345319,17.0579338754786));
#69557=CARTESIAN_POINT('Ctrl Pts',(52.292690959438,12.8200454826231,16.9794283651019));
#69558=CARTESIAN_POINT('Ctrl Pts',(51.3818809893341,14.2799763673289,16.9009228547251));
#69559=CARTESIAN_POINT('Ctrl Pts',(52.0972417021452,15.8449777434614,16.8224173443483));
#69560=CARTESIAN_POINT('Ctrl Pts',(53.7972198251956,16.11152007286,16.7439118339715));
#69561=CARTESIAN_POINT('Ctrl Pts',(54.9572349488979,14.8405614110472,16.6654063235948));
#69562=CARTESIAN_POINT('Ctrl Pts',(54.5369577413632,13.1719279226262,16.586900813218));
#69563=CARTESIAN_POINT('Ctrl Pts',(52.9133028885494,12.602089679815,16.5083953028412));
#69564=CARTESIAN_POINT('Ctrl Pts',(51.5424026157113,13.6420912202446,16.4298897924644));
#69565=CARTESIAN_POINT('Ctrl Pts',(51.6537129020729,15.359234410906,16.3513842820876));
#69566=CARTESIAN_POINT('Ctrl Pts',(53.1474080250528,16.2135444290179,16.2728787717109));
#69567=CARTESIAN_POINT('Ctrl Pts',(54.6839066935017,15.4388557336608,16.1943732613341));
#69568=CARTESIAN_POINT('Ctrl Pts',(54.8852403705633,13.7299275672916,16.1158677509573));
#69569=CARTESIAN_POINT('Ctrl Pts',(53.5708482296119,12.6193673352972,16.0373622405805));
#69570=CARTESIAN_POINT('Ctrl Pts',(51.9195083898506,13.1031518566562,15.9588567302037));
#69571=CARTESIAN_POINT('Ctrl Pts',(51.4121816782637,14.7474116707683,15.8803512198269));
#69572=CARTESIAN_POINT('Ctrl Pts',(52.503850750664,16.077535486755,15.8018457094502));
#69573=CARTESIAN_POINT('Ctrl Pts',(54.2154808300007,15.9006366439348,15.7233401990734));
#69574=CARTESIAN_POINT('Ctrl Pts',(55.0120413695279,14.3753622311824,15.6448346886966));
#69575=CARTESIAN_POINT('Ctrl Pts',(54.1791579400318,12.8696146010229,15.5663291783198));
#69576=CARTESIAN_POINT('Ctrl Pts',(52.4637802022359,12.7337840295962,15.4878236679431));
#69577=CARTESIAN_POINT('Ctrl Pts',(51.4042996911802,14.0896865938602,15.4093181575663));
#69578=CARTESIAN_POINT('Ctrl Pts',(51.9508837188856,15.721316656963,15.3308126471895));
#69579=CARTESIAN_POINT('Ctrl Pts',(53.6133427309768,16.1653895531783,15.2523071368127));
#69580=CARTESIAN_POINT('Ctrl Pts',(54.9007439708605,15.0236502232965,15.1738016264359));
#69581=CARTESIAN_POINT('Ctrl Pts',(54.6585153839456,13.3200374976642,15.0952961160592));
#69582=CARTESIAN_POINT('Ctrl Pts',(53.1038933588347,12.5823920603089,15.0167906056824));
#69583=CARTESIAN_POINT('Ctrl Pts',(51.6310998196597,13.4722512894541,14.9382850953056));
#69584=CARTESIAN_POINT('Ctrl Pts',(51.5609711612585,15.1915694569347,14.8597795849288));
#69585=CARTESIAN_POINT('Ctrl Pts',(52.9564001587445,16.1984187666638,14.781274074552));
#69586=CARTESIAN_POINT('Ctrl Pts',(54.5659334636339,15.5898376428623,14.7027685641752));
#69587=CARTESIAN_POINT('Ctrl Pts',(54.9461022318155,13.911606374279,14.6242630537985));
#69588=CARTESIAN_POINT('Ctrl Pts',(53.7559643179138,12.6688223002735,14.5457575434217));
#69589=CARTESIAN_POINT('Ctrl Pts',(52.0628591682458,12.9760040856148,14.4672520330449));
#69590=CARTESIAN_POINT('Ctrl Pts',(51.3852128724656,14.5577438020024,14.3887465226681));
#69591=CARTESIAN_POINT('Ctrl Pts',(52.3307362917628,15.9953382094595,14.3102410122914));
#69592=CARTESIAN_POINT('Ctrl Pts',(54.0514987748276,15.9998443309588,14.2317355019146));
#69593=CARTESIAN_POINT('Ctrl Pts',(55.0042044918326,14.5665632650764,14.1532299915378));
#69594=CARTESIAN_POINT('Ctrl Pts',(54.3345957734335,12.9822233909154,14.074724481161));
#69595=CARTESIAN_POINT('Ctrl Pts',(52.6428908318491,12.6650114501325,13.9962189707842));
#69596=CARTESIAN_POINT('Ctrl Pts',(51.4468410434118,13.9049130927216,13.9177134604075));
#69597=CARTESIAN_POINT('Ctrl Pts',(51.6948674713958,15.0196330720529,13.8653764534896));
#69598=CARTESIAN_POINT('Ctrl Pts',(52.0259993620635,15.404095589155,13.8392079500307));
#69599=CARTESIAN_POINT('Ctrl Pts',(52.8205983740734,12.9961697745651,18.0535973499898));
#69600=CARTESIAN_POINT('Ctrl Pts',(52.3599004442679,13.11933387906,18.0274288465308));
#69601=CARTESIAN_POINT('Ctrl Pts',(51.5770224562856,13.8535123278672,17.975091839613));
#69602=CARTESIAN_POINT('Ctrl Pts',(51.8491027615147,15.449596585157,17.8965863292362));
#69603=CARTESIAN_POINT('Ctrl Pts',(53.3306005753027,16.0991388853812,17.8180808188594));
#69604=CARTESIAN_POINT('Ctrl Pts',(54.6895013936796,15.2235740807106,17.7395753084826));
#69605=CARTESIAN_POINT('Ctrl Pts',(54.7087686260452,13.6062036013327,17.6610697981059));
#69606=CARTESIAN_POINT('Ctrl Pts',(53.370302195588,12.6984745354833,17.5825642877291));
#69607=CARTESIAN_POINT('Ctrl Pts',(51.8748772355608,13.3139889999824,17.5040587773523));
#69608=CARTESIAN_POINT('Ctrl Pts',(51.5634249338332,14.9009722914672,17.4255532669755));
#69609=CARTESIAN_POINT('Ctrl Pts',(52.7153629422732,16.0360644703525,17.3470477565987));
#69610=CARTESIAN_POINT('Ctrl Pts',(54.2975564085964,15.7013451606169,17.268542246222));
#69611=CARTESIAN_POINT('Ctrl Pts',(54.8910811244797,14.1969702179137,17.1900367358452));
#69612=CARTESIAN_POINT('Ctrl Pts',(53.9636378718331,12.8721129164929,17.1115312254684));
#69613=CARTESIAN_POINT('Ctrl Pts',(52.3469858247822,12.9149298139051,17.0330257150916));
#69614=CARTESIAN_POINT('Ctrl Pts',(51.4909739917867,14.2870251506759,16.9545202047149));
#69615=CARTESIAN_POINT('Ctrl Pts',(52.1632956122413,15.75786949867,16.8760146943381));
#69616=CARTESIAN_POINT('Ctrl Pts',(53.7609959415415,16.0083755267644,16.7975091839613));
#69617=CARTESIAN_POINT('Ctrl Pts',(54.8512197038372,14.8138830536132,16.7190036735845));
#69618=CARTESIAN_POINT('Ctrl Pts',(54.4562281308452,13.2456415346295,16.6404981632077));
#69619=CARTESIAN_POINT('Ctrl Pts',(52.9302591446352,12.7100871437567,16.561992652831));
#69620=CARTESIAN_POINT('Ctrl Pts',(51.6418379657667,13.6875178418857,16.4834871424542));
#69621=CARTESIAN_POINT('Ctrl Pts',(51.7464513597646,15.3013505165395,16.4049816320774));
#69622=CARTESIAN_POINT('Ctrl Pts',(53.1502795370219,16.1042616709564,16.3264761217006));
#69623=CARTESIAN_POINT('Ctrl Pts',(54.5943360194344,15.3761814875148,16.2479706113238));
#69624=CARTESIAN_POINT('Ctrl Pts',(54.7835566204401,13.7700695869339,16.1694651009471));
#69625=CARTESIAN_POINT('Ctrl Pts',(53.5482438079086,12.7263253032243,16.0909595905703));
#69626=CARTESIAN_POINT('Ctrl Pts',(51.9962554793534,13.1810033244324,16.0124540801935));
#69627=CARTESIAN_POINT('Ctrl Pts',(51.5194516645429,14.7263375912924,15.9339485698167));
#69628=CARTESIAN_POINT('Ctrl Pts',(52.5454413598284,15.9764355954941,15.85544305944));
#69629=CARTESIAN_POINT('Ctrl Pts',(54.1540926149925,15.8101797269071,15.7769375490631));
#69630=CARTESIAN_POINT('Ctrl Pts',(54.9027287409836,14.376672202025,15.6984320386864));
#69631=CARTESIAN_POINT('Ctrl Pts',(54.1199550619984,12.9615166468276,15.6199265283096));
#69632=CARTESIAN_POINT('Ctrl Pts',(52.507781623182,12.8338582106659,15.5414210179328));
#69633=CARTESIAN_POINT('Ctrl Pts',(51.5120438907673,14.1081840058336,15.462915507556));
#69634=CARTESIAN_POINT('Ctrl Pts',(52.0257431373717,15.6416483803266,15.3844099971793));
#69635=CARTESIAN_POINT('Ctrl Pts',(53.5881816623453,16.0590039938468,15.3059044868025));
#69636=CARTESIAN_POINT('Ctrl Pts',(54.7981274593024,14.98595647718,15.2273989764257));
#69637=CARTESIAN_POINT('Ctrl Pts',(54.5704723572558,13.3848402181903,15.1488934660489));
#69638=CARTESIAN_POINT('Ctrl Pts',(53.1093828951162,12.691574615422,15.0703879556721));
#69639=CARTESIAN_POINT('Ctrl Pts',(51.7251987749646,13.5278961916579,14.9918824452954));
#69640=CARTESIAN_POINT('Ctrl Pts',(51.6592893499541,15.143772987429,14.9133769349186));
#69641=CARTESIAN_POINT('Ctrl Pts',(52.9707635028083,16.0900460317101,14.8348714245418));
#69642=CARTESIAN_POINT('Ctrl Pts',(54.4834605524781,15.5180796936027,14.756365914165));
#69643=CARTESIAN_POINT('Ctrl Pts',(54.8407567775752,13.9408178370524,14.6778604037883));
#69644=CARTESIAN_POINT('Ctrl Pts',(53.7222225381219,12.7728048506706,14.5993548934115));
#69645=CARTESIAN_POINT('Ctrl Pts',(52.1309816753803,13.0615052950706,14.5208493830347));
#69646=CARTESIAN_POINT('Ctrl Pts',(51.4941054148939,14.5480809347647,14.4423438726579));
#69647=CARTESIAN_POINT('Ctrl Pts',(52.3827421907963,15.8991836501767,14.3638383622811));
#69648=CARTESIAN_POINT('Ctrl Pts',(53.9999764060855,15.9034186645606,14.2853328519044));
#69649=CARTESIAN_POINT('Ctrl Pts',(54.8953633626268,14.5563697820544,14.2068273415276));
#69650=CARTESIAN_POINT('Ctrl Pts',(54.2660411052506,13.0673504209531,14.1283218311508));
#69651=CARTESIAN_POINT('Ctrl Pts',(52.676116208218,12.7692232772124,14.049816320774));
#69652=CARTESIAN_POINT('Ctrl Pts',(51.5520257773267,13.934527251307,13.9713108103972));
#69653=CARTESIAN_POINT('Ctrl Pts',(51.7851298980751,14.9821810145562,13.9189738034794));
#69654=CARTESIAN_POINT('Ctrl Pts',(52.0963395092977,15.3435126586808,13.8928053000205));
#69655=CARTESIAN_POINT('Ctrl Pts',(52.8445746335154,13.0858534785527,18.1071946999795));
#69656=CARTESIAN_POINT('Ctrl Pts',(52.4133685721046,13.2011331552574,18.0810261965206));
#69657=CARTESIAN_POINT('Ctrl Pts',(51.6806070120392,13.8883127078473,18.0286891896028));
#69658=CARTESIAN_POINT('Ctrl Pts',(51.9352699250133,15.3822226252555,17.950183679226));
#69659=CARTESIAN_POINT('Ctrl Pts',(53.3219287223341,15.9901840656676,17.8716781688492));
#69660=CARTESIAN_POINT('Ctrl Pts',(54.5938386481888,15.1706690939129,17.7931726584724));
#69661=CARTESIAN_POINT('Ctrl Pts',(54.6118724765286,13.6568356053423,17.7146671480956));
#69662=CARTESIAN_POINT('Ctrl Pts',(53.3590888183695,12.8072153878641,17.6361616377189));
#69663=CARTESIAN_POINT('Ctrl Pts',(51.9593944298553,13.3833273059057,17.5576561273421));
#69664=CARTESIAN_POINT('Ctrl Pts',(51.6678799435584,14.868718861572,17.4791506169653));
#69665=CARTESIAN_POINT('Ctrl Pts',(52.746075914221,15.9311473990782,17.4006451065885));
#69666=CARTESIAN_POINT('Ctrl Pts',(54.2269842684029,15.6178553569582,17.3221395962117));
#69667=CARTESIAN_POINT('Ctrl Pts',(54.7825141254484,14.2097839245511,17.243634085835));
#69668=CARTESIAN_POINT('Ctrl Pts',(53.9144417372685,12.9697381984539,17.1651285754582));
#69669=CARTESIAN_POINT('Ctrl Pts',(52.4012806901265,13.009814145187,17.0866230650814));
#69670=CARTESIAN_POINT('Ctrl Pts',(51.6000669942391,14.294073934023,17.0081175547046));
#69671=CARTESIAN_POINT('Ctrl Pts',(52.2293495223373,15.6707612538786,16.9296120443278));
#69672=CARTESIAN_POINT('Ctrl Pts',(53.7247720578873,15.9052309806687,16.8511065339511));
#69673=CARTESIAN_POINT('Ctrl Pts',(54.7452044587765,14.7872046961792,16.7726010235743));
#69674=CARTESIAN_POINT('Ctrl Pts',(54.3754985203273,13.3193551466328,16.6940955131975));
#69675=CARTESIAN_POINT('Ctrl Pts',(52.9472154007209,12.8180846076984,16.6155900028207));
#69676=CARTESIAN_POINT('Ctrl Pts',(51.7412733158221,13.7329444635267,16.5370844924439));
#69677=CARTESIAN_POINT('Ctrl Pts',(51.8391898174563,15.243466622173,16.4585789820672));
#69678=CARTESIAN_POINT('Ctrl Pts',(53.153151048991,15.9949789128949,16.3800734716904));
#69679=CARTESIAN_POINT('Ctrl Pts',(54.5047653453669,15.3135072413688,16.3015679613136));
#69680=CARTESIAN_POINT('Ctrl Pts',(54.6818728703171,13.8102116065761,16.2230624509368));
#69681=CARTESIAN_POINT('Ctrl Pts',(53.5256393862053,12.8332832711514,16.14455694056));
#69682=CARTESIAN_POINT('Ctrl Pts',(52.0730025688563,13.2588547922086,16.0660514301833));
#69683=CARTESIAN_POINT('Ctrl Pts',(51.6267216508219,14.7052635118164,15.9875459198065));
#69684=CARTESIAN_POINT('Ctrl Pts',(52.5870319689928,15.8753357042332,15.9090404094297));
#69685=CARTESIAN_POINT('Ctrl Pts',(54.0927043999843,15.7197228098794,15.8305348990529));
#69686=CARTESIAN_POINT('Ctrl Pts',(54.7934161124393,14.3779821728676,15.7520293886762));
#69687=CARTESIAN_POINT('Ctrl Pts',(54.060752183965,13.0534186926323,15.6735238782993));
#69688=CARTESIAN_POINT('Ctrl Pts',(52.551783044128,12.9339323917357,15.5950183679226));
#69689=CARTESIAN_POINT('Ctrl Pts',(51.6197880903543,14.1266814178069,15.5165128575458));
#69690=CARTESIAN_POINT('Ctrl Pts',(52.1006025558579,15.5619801036903,15.438007347169));
#69691=CARTESIAN_POINT('Ctrl Pts',(53.5630205937139,15.9526184345153,15.3595018367923));
#69692=CARTESIAN_POINT('Ctrl Pts',(54.6955109477442,14.9482627310635,15.2809963264155));
#69693=CARTESIAN_POINT('Ctrl Pts',(54.4824293305661,13.4496429387163,15.2024908160387));
#69694=CARTESIAN_POINT('Ctrl Pts',(53.1148724313975,12.8007571705352,15.1239853056619));
#69695=CARTESIAN_POINT('Ctrl Pts',(51.8192977302697,13.5835410938618,15.0454797952851));
#69696=CARTESIAN_POINT('Ctrl Pts',(51.7576075386496,15.0959765179234,14.9669742849084));
#69697=CARTESIAN_POINT('Ctrl Pts',(52.9851268468722,15.9816732967562,14.8884687745316));
#69698=CARTESIAN_POINT('Ctrl Pts',(54.4009876413224,15.4463217443432,14.8099632641548));
#69699=CARTESIAN_POINT('Ctrl Pts',(54.7354113233349,13.9700292998257,14.731457753778));
#69700=CARTESIAN_POINT('Ctrl Pts',(53.6884807583299,12.8767874010678,14.6529522434012));
#69701=CARTESIAN_POINT('Ctrl Pts',(52.1991041825149,13.1470065045264,14.5744467330245));
#69702=CARTESIAN_POINT('Ctrl Pts',(51.602997957322,14.5384180675271,14.4959412226477));
#69703=CARTESIAN_POINT('Ctrl Pts',(52.4347480898299,15.803029090894,14.4174357122709));
#69704=CARTESIAN_POINT('Ctrl Pts',(53.9484540373433,15.8069929981624,14.3389302018941));
#69705=CARTESIAN_POINT('Ctrl Pts',(54.7865222334211,14.5461762990323,14.2604246915173));
#69706=CARTESIAN_POINT('Ctrl Pts',(54.1974864370675,13.1524774509909,14.1819191811406));
#69707=CARTESIAN_POINT('Ctrl Pts',(52.7093415845871,12.8734351042922,14.1034136707638));
#69708=CARTESIAN_POINT('Ctrl Pts',(51.6572105112416,13.9641414098923,14.024908160387));
#69709=CARTESIAN_POINT('Ctrl Pts',(51.8753923247544,14.9447289570596,13.9725711534692));
#69710=CARTESIAN_POINT('Ctrl Pts',(52.166679656532,15.2829297282066,13.9464026500102));
#69711=CARTESIAN_POINT('Ctrl Pts',(52.8685508929575,13.1755371825404,18.1607920499693));
#69712=CARTESIAN_POINT('Ctrl Pts',(52.4668366999413,13.2829324314547,18.1346235465104));
#69713=CARTESIAN_POINT('Ctrl Pts',(51.7841915677929,13.9231130878275,18.0822865395925));
#69714=CARTESIAN_POINT('Ctrl Pts',(52.0214370885118,15.3148486653539,18.0037810292157));
#69715=CARTESIAN_POINT('Ctrl Pts',(53.3132568693655,15.881229245954,17.925275518839));
#69716=CARTESIAN_POINT('Ctrl Pts',(54.498175902698,15.1177641071152,17.8467700084622));
#69717=CARTESIAN_POINT('Ctrl Pts',(54.5149763270121,13.7074676093518,17.7682644980854));
#69718=CARTESIAN_POINT('Ctrl Pts',(53.347875441151,12.9159562402449,17.6897589877086));
#69719=CARTESIAN_POINT('Ctrl Pts',(52.0439116241498,13.4526656118291,17.6112534773318));
#69720=CARTESIAN_POINT('Ctrl Pts',(51.7723349532836,14.8364654316769,17.5327479669551));
#69721=CARTESIAN_POINT('Ctrl Pts',(52.7767888861689,15.826230327804,17.4542424565783));
#69722=CARTESIAN_POINT('Ctrl Pts',(54.1564121282093,15.5343655532995,17.3757369462015));
#69723=CARTESIAN_POINT('Ctrl Pts',(54.6739471264171,14.2225976311884,17.2972314358247));
#69724=CARTESIAN_POINT('Ctrl Pts',(53.8652456027039,13.0673634804149,17.218725925448));
#69725=CARTESIAN_POINT('Ctrl Pts',(52.4555755554707,13.104698476469,17.1402204150712));
#69726=CARTESIAN_POINT('Ctrl Pts',(51.7091599966917,14.3011227173701,17.0617149046944));
#69727=CARTESIAN_POINT('Ctrl Pts',(52.2954034324334,15.5836530090872,16.9832093943176));
#69728=CARTESIAN_POINT('Ctrl Pts',(53.6885481742333,15.802086434573,16.9047038839408));
#69729=CARTESIAN_POINT('Ctrl Pts',(54.6391892137158,14.7605263387452,16.8261983735641));
#69730=CARTESIAN_POINT('Ctrl Pts',(54.2947689098094,13.3930687586361,16.7476928631873));
#69731=CARTESIAN_POINT('Ctrl Pts',(52.9641716568067,12.9260820716401,16.6691873528105));
#69732=CARTESIAN_POINT('Ctrl Pts',(51.8407086658775,13.7783710851678,16.5906818424337));
#69733=CARTESIAN_POINT('Ctrl Pts',(51.931928275148,15.1855827278064,16.5121763320569));
#69734=CARTESIAN_POINT('Ctrl Pts',(53.15602256096,15.8856961548334,16.4336708216802));
#69735=CARTESIAN_POINT('Ctrl Pts',(54.4151946712995,15.2508329952228,16.3551653113034));
#69736=CARTESIAN_POINT('Ctrl Pts',(54.5801891201939,13.8503536262184,16.2766598009266));
#69737=CARTESIAN_POINT('Ctrl Pts',(53.5030349645019,12.9402412390784,16.1981542905498));
#69738=CARTESIAN_POINT('Ctrl Pts',(52.1497496583591,13.3367062599848,16.119648780173));
#69739=CARTESIAN_POINT('Ctrl Pts',(51.7339916371008,14.6841894323404,16.0411432697963));
#69740=CARTESIAN_POINT('Ctrl Pts',(52.6286225781573,15.7742358129723,15.9626377594195));
#69741=CARTESIAN_POINT('Ctrl Pts',(54.031316184976,15.6292658928517,15.8841322490427));
#69742=CARTESIAN_POINT('Ctrl Pts',(54.6841034838951,14.3792921437102,15.8056267386659));
#69743=CARTESIAN_POINT('Ctrl Pts',(54.0015493059315,13.1453207384369,15.7271212282891));
#69744=CARTESIAN_POINT('Ctrl Pts',(52.5957844650742,13.0340065728056,15.6486157179124));
#69745=CARTESIAN_POINT('Ctrl Pts',(51.7275322899413,14.1451788297802,15.5701102075356));
#69746=CARTESIAN_POINT('Ctrl Pts',(52.1754619743441,15.482311827054,15.4916046971588));
#69747=CARTESIAN_POINT('Ctrl Pts',(53.5378595250824,15.8462328751838,15.413099186782));
#69748=CARTESIAN_POINT('Ctrl Pts',(54.5928944361861,14.9105689849469,15.3345936764052));
#69749=CARTESIAN_POINT('Ctrl Pts',(54.3943863038764,13.5144456592424,15.2560881660285));
#69750=CARTESIAN_POINT('Ctrl Pts',(53.120361967679,12.9099397256483,15.1775826556517));
#69751=CARTESIAN_POINT('Ctrl Pts',(51.9133966855747,13.6391859960657,15.0990771452749));
#69752=CARTESIAN_POINT('Ctrl Pts',(51.8559257273451,15.0481800484177,15.0205716348981));
#69753=CARTESIAN_POINT('Ctrl Pts',(52.9994901909361,15.8733005618024,14.9420661245214));
#69754=CARTESIAN_POINT('Ctrl Pts',(54.3185147301667,15.3745637950836,14.8635606141446));
#69755=CARTESIAN_POINT('Ctrl Pts',(54.6300658690945,13.9992407625991,14.7850551037678));
#69756=CARTESIAN_POINT('Ctrl Pts',(53.654738978538,12.980769951465,14.706549593391));
#69757=CARTESIAN_POINT('Ctrl Pts',(52.2672266896493,13.2325077139822,14.6280440830142));
#69758=CARTESIAN_POINT('Ctrl Pts',(51.7118904997504,14.5287552002895,14.5495385726374));
#69759=CARTESIAN_POINT('Ctrl Pts',(52.4867539888634,15.7068745316113,14.4710330622607));
#69760=CARTESIAN_POINT('Ctrl Pts',(53.8969316686011,15.7105673317642,14.3925275518839));
#69761=CARTESIAN_POINT('Ctrl Pts',(54.6776811042154,14.5359828160102,14.3140220415071));
#69762=CARTESIAN_POINT('Ctrl Pts',(54.1289317688846,13.2376044810286,14.2355165311303));
#69763=CARTESIAN_POINT('Ctrl Pts',(52.742566960956,12.9776469313721,14.1570110207535));
#69764=CARTESIAN_POINT('Ctrl Pts',(51.7623952451565,13.9937555684777,14.0785055103768));
#69765=CARTESIAN_POINT('Ctrl Pts',(51.9656547514336,14.9072768995629,14.0261685034589));
#69766=CARTESIAN_POINT('Ctrl Pts',(52.2370198037663,15.2223467977324,14.));
#69767=CARTESIAN_POINT('Ctrl Pts',(51.9314271328212,14.3981451355535,17.5565803263806));
#69768=CARTESIAN_POINT('Ctrl Pts',(51.9304449349957,14.5245552242527,17.5486362065721));
#69769=CARTESIAN_POINT('Ctrl Pts',(51.9479261083582,14.6507002121319,17.5406920867636));
#69770=CARTESIAN_POINT('Ctrl Pts',(51.9850067205755,14.7707929443901,17.5327479669551));
#69771=CARTESIAN_POINT('Ctrl Pts',(52.107152930912,15.1663870637192,17.5065794634962));
#69772=CARTESIAN_POINT('Ctrl Pts',(52.4419709085405,15.4963086957616,17.4804109600372));
#69773=CARTESIAN_POINT('Ctrl Pts',(52.8393171043614,15.6126253826987,17.4542424565783));
#69774=CARTESIAN_POINT('Ctrl Pts',(53.2366633001824,15.7289420696358,17.4280739531194));
#69775=CARTESIAN_POINT('Ctrl Pts',(53.6965377141958,15.6316538114677,17.4019054496604));
#69776=CARTESIAN_POINT('Ctrl Pts',(54.0127307542372,15.3643816953651,17.3757369462015));
#69777=CARTESIAN_POINT('Ctrl Pts',(54.3289237942786,15.0971095792624,17.3495684427426));
#69778=CARTESIAN_POINT('Ctrl Pts',(54.5014354603479,14.6598536052254,17.3233999392837));
#69779=CARTESIAN_POINT('Ctrl Pts',(54.452907706097,14.248686593078,17.2972314358247));
#69780=CARTESIAN_POINT('Ctrl Pts',(54.4043799518461,13.8375195809306,17.2710629323658));
#69781=CARTESIAN_POINT('Ctrl Pts',(54.134812777275,13.4524415306728,17.2448944289069));
#69782=CARTESIAN_POINT('Ctrl Pts',(53.7650841821172,13.2661250048862,17.218725925448));
#69783=CARTESIAN_POINT('Ctrl Pts',(53.3953555869595,13.0798084790996,17.192557421989));
#69784=CARTESIAN_POINT('Ctrl Pts',(52.9254655712151,13.0922534777843,17.1663889185301));
#69785=CARTESIAN_POINT('Ctrl Pts',(52.5661179702131,13.2978800172768,17.1402204150712));
#69786=CARTESIAN_POINT('Ctrl Pts',(52.206770369211,13.5035065567693,17.1140519116122));
#69787=CARTESIAN_POINT('Ctrl Pts',(51.9579651829513,13.9023146370697,17.0878834081533));
#69788=CARTESIAN_POINT('Ctrl Pts',(51.9312698291118,14.3154737258394,17.0617149046944));
#69789=CARTESIAN_POINT('Ctrl Pts',(51.9295238448586,14.3424960034753,17.0600033785898));
#69790=CARTESIAN_POINT('Ctrl Pts',(51.9287279775559,14.3695796702729,17.0582918524852));
#69791=CARTESIAN_POINT('Ctrl Pts',(51.9288577112775,14.3966710926088,17.0565803263806));
#69792=CARTESIAN_POINT('Origin',(53.1951359564886,14.3971354987959,15.5));
#69793=CARTESIAN_POINT('Origin',(53.1951359564886,14.3971354987959,13.));
#69794=CARTESIAN_POINT('',(53.1951359564886,14.3971354987959,13.));
#69795=CARTESIAN_POINT('Origin',(53.1951359564886,14.3971354987959,13.));
#69796=CARTESIAN_POINT('',(53.1951359564886,14.3971354987959,13.));
#69797=CARTESIAN_POINT('Origin',(38.7910352698572,-39.2874736104613,10.));
#69798=CARTESIAN_POINT('',(37.4169463095016,-41.3759849293267,8.5));
#69799=CARTESIAN_POINT('Origin',(37.4169463095016,-41.3759849293267,10.));
#69800=CARTESIAN_POINT('',(36.8673107253594,-42.2113894568729,8.5));
#69801=CARTESIAN_POINT('',(38.7910352698572,-39.2874736104613,8.5));
#69802=CARTESIAN_POINT('Origin',(36.8673107253594,-42.2113894568729,10.));
#69803=CARTESIAN_POINT('Origin',(39.0658530619283,-38.8697713466882,10.));
#69804=CARTESIAN_POINT('',(40.714759814355,-36.3635577640498,7.));
#69805=CARTESIAN_POINT('Origin',(40.714759814355,-36.3635577640498,10.));
#69806=CARTESIAN_POINT('',(39.0658530619283,-38.8697713466882,7.));
#69807=CARTESIAN_POINT('',(37.4169463095016,-41.3759849293267,7.));
#69808=CARTESIAN_POINT('',(39.0658530619283,-38.8697713466882,7.));
#69809=CARTESIAN_POINT('Origin',(37.4169463095016,-41.3759849293267,10.));
#69810=CARTESIAN_POINT('Origin',(37.4169463095016,-41.3759849293267,10.));
#69811=CARTESIAN_POINT('Origin',(-14.6284325622417,-53.2377587880251,10.));
#69812=CARTESIAN_POINT('',(-17.2116250730252,-54.5894675037741,10.));
#69813=CARTESIAN_POINT('Origin',(-17.1241809006482,-53.0920185007302,10.));
#69814=CARTESIAN_POINT('',(-18.2099244083879,-54.5311713888561,10.));
#69815=CARTESIAN_POINT('',(-14.7158767346186,-54.7352077910691,10.));
#69816=CARTESIAN_POINT('Origin',(-18.1224802360109,-53.0337223858122,10.));
#69817=CARTESIAN_POINT('Origin',(-14.1292828945603,-53.2669068454841,10.));
#69818=CARTESIAN_POINT('',(-11.1343848884725,-53.4417951902381,7.));
#69819=CARTESIAN_POINT('Origin',(-11.1343848884725,-53.4417951902381,10.));
#69820=CARTESIAN_POINT('',(-14.1292828945603,-53.2669068454841,7.));
#69821=CARTESIAN_POINT('',(-17.1241809006482,-53.0920185007302,7.));
#69822=CARTESIAN_POINT('',(-14.1292828945603,-53.2669068454841,7.));
#69823=CARTESIAN_POINT('Origin',(-17.1241809006482,-53.0920185007302,10.));
#69824=CARTESIAN_POINT('Origin',(-17.1241809006482,-53.0920185007302,10.));
#69825=CARTESIAN_POINT('Origin',(-53.4194678320988,-13.9502851775638,10.));
#69826=CARTESIAN_POINT('',(-54.5411272101499,-11.7160335714034,11.5));
#69827=CARTESIAN_POINT('Origin',(-54.5411272101499,-11.7160335714034,10.));
#69828=CARTESIAN_POINT('',(-54.9897909613702,-10.8223329289393,11.5));
#69829=CARTESIAN_POINT('',(-53.4194678320988,-13.9502851775638,11.5));
#69830=CARTESIAN_POINT('Origin',(-54.9897909613702,-10.8223329289393,10.));
#69831=CARTESIAN_POINT('Origin',(-53.1951359564886,-14.3971354987959,10.));
#69832=CARTESIAN_POINT('',(-51.8491447028274,-17.0782374261884,7.));
#69833=CARTESIAN_POINT('Origin',(-51.8491447028274,-17.0782374261884,10.));
#69834=CARTESIAN_POINT('',(-53.1951359564886,-14.3971354987959,7.));
#69835=CARTESIAN_POINT('',(-54.5411272101499,-11.7160335714034,7.));
#69836=CARTESIAN_POINT('',(-53.1951359564886,-14.3971354987959,7.));
#69837=CARTESIAN_POINT('Origin',(-54.5411272101499,-11.7160335714034,10.));
#69838=CARTESIAN_POINT('Origin',(-54.5411272101499,-11.7160335714034,10.));
#69839=CARTESIAN_POINT('Origin',(-38.7910352698572,39.2874736104613,10.));
#69840=CARTESIAN_POINT('',(-37.4169463095016,41.3759849293267,11.5));
#69841=CARTESIAN_POINT('Origin',(-37.4169463095016,41.3759849293267,10.));
#69842=CARTESIAN_POINT('',(-36.8673107253594,42.2113894568729,11.5));
#69843=CARTESIAN_POINT('',(-38.7910352698572,39.2874736104613,11.5));
#69844=CARTESIAN_POINT('Origin',(-36.8673107253594,42.2113894568729,10.));
#69845=CARTESIAN_POINT('Origin',(-39.0658530619283,38.8697713466882,10.));
#69846=CARTESIAN_POINT('',(-40.714759814355,36.3635577640498,7.));
#69847=CARTESIAN_POINT('Origin',(-40.714759814355,36.3635577640498,10.));
#69848=CARTESIAN_POINT('',(-39.0658530619283,38.8697713466882,7.));
#69849=CARTESIAN_POINT('',(-37.4169463095016,41.3759849293267,7.));
#69850=CARTESIAN_POINT('',(-39.0658530619283,38.8697713466882,7.));
#69851=CARTESIAN_POINT('Origin',(-37.4169463095016,41.3759849293267,10.));
#69852=CARTESIAN_POINT('Origin',(-37.4169463095016,41.3759849293267,10.));
#69853=CARTESIAN_POINT('Origin',(14.6284325622417,53.2377587880251,10.));
#69854=CARTESIAN_POINT('',(17.2116250730252,54.5894675037741,10.));
#69855=CARTESIAN_POINT('Origin',(17.1241809006482,53.0920185007302,10.));
#69856=CARTESIAN_POINT('',(18.2099244083878,54.5311713888561,10.));
#69857=CARTESIAN_POINT('',(14.7158767346186,54.7352077910691,10.));
#69858=CARTESIAN_POINT('Origin',(18.1224802360108,53.0337223858122,10.));
#69859=CARTESIAN_POINT('Origin',(14.1292828945603,53.2669068454841,10.));
#69860=CARTESIAN_POINT('',(11.1343848884724,53.4417951902381,7.));
#69861=CARTESIAN_POINT('Origin',(11.1343848884724,53.4417951902381,10.));
#69862=CARTESIAN_POINT('',(14.1292828945603,53.2669068454841,7.));
#69863=CARTESIAN_POINT('',(17.1241809006482,53.0920185007302,7.));
#69864=CARTESIAN_POINT('',(14.1292828945603,53.2669068454841,7.));
#69865=CARTESIAN_POINT('Origin',(17.1241809006482,53.0920185007302,10.));
#69866=CARTESIAN_POINT('Origin',(17.1241809006482,53.0920185007302,10.));
#69867=CARTESIAN_POINT('Origin',(53.4194678320988,13.9502851775638,10.));
#69868=CARTESIAN_POINT('',(54.5411272101499,11.7160335714034,8.5));
#69869=CARTESIAN_POINT('Origin',(54.5411272101499,11.7160335714034,10.));
#69870=CARTESIAN_POINT('',(54.9897909613702,10.8223329289393,8.5));
#69871=CARTESIAN_POINT('',(53.4194678320988,13.9502851775638,8.5));
#69872=CARTESIAN_POINT('Origin',(54.9897909613702,10.8223329289393,10.));
#69873=CARTESIAN_POINT('Origin',(53.1951359564886,14.3971354987959,10.));
#69874=CARTESIAN_POINT('',(51.8491447028274,17.0782374261884,7.));
#69875=CARTESIAN_POINT('Origin',(51.8491447028274,17.0782374261884,10.));
#69876=CARTESIAN_POINT('',(53.1951359564886,14.3971354987959,7.));
#69877=CARTESIAN_POINT('',(54.5411272101499,11.7160335714034,7.));
#69878=CARTESIAN_POINT('',(53.1951359564886,14.3971354987959,7.));
#69879=CARTESIAN_POINT('Origin',(54.5411272101499,11.7160335714034,10.));
#69880=CARTESIAN_POINT('Origin',(54.5411272101499,11.7160335714034,10.));
#69881=CARTESIAN_POINT('Origin',(32.7784168026664,-31.1420197146986,2.));
#69882=CARTESIAN_POINT('',(29.4485343854062,-36.2031892017778,2.));
#69883=CARTESIAN_POINT('Ctrl Pts',(29.4485343857591,-36.2031892014269,2.));
#69884=CARTESIAN_POINT('Ctrl Pts',(29.4485343857591,-36.2031892014269,4.66666666666667));
#69885=CARTESIAN_POINT('Ctrl Pts',(29.4485343857591,-36.2031892014269,7.33333333333333));
#69886=CARTESIAN_POINT('Ctrl Pts',(29.4485343857591,-36.2031892014269,12.6666666666667));
#69887=CARTESIAN_POINT('Ctrl Pts',(29.4485343857591,-36.2031892014269,15.3333333333333));
#69888=CARTESIAN_POINT('Ctrl Pts',(29.4485343857591,-36.2031892014269,18.));
#69889=CARTESIAN_POINT('',(28.9309677136708,-36.9898514075217,2.));
#69890=CARTESIAN_POINT('',(32.7784168026664,-31.1420197146986,2.));
#69891=CARTESIAN_POINT('',(28.9309677136708,-36.9898514075217,2.));
#69892=CARTESIAN_POINT('Origin',(43.6386756607666,-38.2872823085476,2.));
#69893=CARTESIAN_POINT('',(34.5017338047181,-32.2758373034865,2.));
#69894=CARTESIAN_POINT('Ctrl Pts',(34.5017338047181,-32.2758373034865,18.));
#69895=CARTESIAN_POINT('Ctrl Pts',(34.5017338047181,-32.2758373034865,15.3333333333333));
#69896=CARTESIAN_POINT('Ctrl Pts',(34.5017338047181,-32.2758373034865,12.6666666666667));
#69897=CARTESIAN_POINT('Ctrl Pts',(34.5017338047181,-32.2758373034865,7.33333333333333));
#69898=CARTESIAN_POINT('Ctrl Pts',(34.5017338047181,-32.2758373034865,4.66666666666667));
#69899=CARTESIAN_POINT('Ctrl Pts',(34.5017338047181,-32.2758373034865,2.));
#69900=CARTESIAN_POINT('',(43.6386756607666,-38.2872823085476,2.));
#69901=CARTESIAN_POINT('',(43.6386756607666,-38.2872823085476,2.));
#69902=CARTESIAN_POINT('',(43.6386756607666,-38.2872823085476,2.));
#69903=CARTESIAN_POINT('Origin',(39.7912265717709,-44.1351140013707,2.));
#69904=CARTESIAN_POINT('',(39.7912265717709,-44.1351140013707,2.));
#69905=CARTESIAN_POINT('',(39.7912265717709,-44.1351140013707,2.));
#69906=CARTESIAN_POINT('',(39.7912265717709,-44.1351140013707,2.));
#69907=CARTESIAN_POINT('Origin',(28.9309677136708,-36.9898514075217,2.));
#69908=CARTESIAN_POINT('',(28.9309677136708,-36.9898514075217,2.));
#69909=CARTESIAN_POINT('Origin',(-11.3384212906854,-56.9358428640073,2.));
#69910=CARTESIAN_POINT('',(-10.7008281308737,-46.0172966012375,2.));
#69911=CARTESIAN_POINT('Ctrl Pts',(-10.7008281308737,-46.0172966012375,
18.));
#69912=CARTESIAN_POINT('Ctrl Pts',(-10.7008281308737,-46.0172966012375,
15.3333333333333));
#69913=CARTESIAN_POINT('Ctrl Pts',(-10.7008281308737,-46.0172966012375,
12.6666666666667));
#69914=CARTESIAN_POINT('Ctrl Pts',(-10.7008281308737,-46.0172966012375,
7.33333333333333));
#69915=CARTESIAN_POINT('Ctrl Pts',(-10.7008281308737,-46.0172966012375,
4.66666666666667));
#69916=CARTESIAN_POINT('Ctrl Pts',(-10.7008281308737,-46.0172966012375,
2.));
#69917=CARTESIAN_POINT('',(-11.3384212906854,-56.9358428640073,2.));
#69918=CARTESIAN_POINT('',(-11.3384212906854,-56.9358428640073,2.));
#69919=CARTESIAN_POINT('',(-11.3384212906854,-56.9358428640073,2.));
#69920=CARTESIAN_POINT('Origin',(-18.3265166382238,-56.5277700595814,2.));
#69921=CARTESIAN_POINT('',(-18.3265166382238,-56.5277700595814,2.));
#69922=CARTESIAN_POINT('',(-18.3265166382238,-56.5277700595814,2.));
#69923=CARTESIAN_POINT('',(-18.3265166382238,-56.5277700595814,2.));
#69924=CARTESIAN_POINT('Origin',(-17.56866714429,-43.5498786998672,2.));
#69925=CARTESIAN_POINT('',(-17.56866714429,-43.5498786998672,2.));
#69926=CARTESIAN_POINT('',(-17.56866714429,-43.5498786998672,2.));
#69927=CARTESIAN_POINT('',(-17.56866714429,-43.5498786998672,2.));
#69928=CARTESIAN_POINT('Origin',(-10.5805717967516,-43.9579515042931,2.));
#69929=CARTESIAN_POINT('',(-16.6286143535706,-43.6047734830004,2.));
#69930=CARTESIAN_POINT('Ctrl Pts',(-16.6286143535706,-43.6047734830004,
2.));
#69931=CARTESIAN_POINT('Ctrl Pts',(-16.6286143535706,-43.6047734830004,
4.66666666666667));
#69932=CARTESIAN_POINT('Ctrl Pts',(-16.6286143535706,-43.6047734830004,
7.33333333333333));
#69933=CARTESIAN_POINT('Ctrl Pts',(-16.6286143535706,-43.6047734830004,
12.6666666666667));
#69934=CARTESIAN_POINT('Ctrl Pts',(-16.6286143535706,-43.6047734830004,
15.3333333333333));
#69935=CARTESIAN_POINT('Ctrl Pts',(-16.6286143535706,-43.6047734830004,
18.));
#69936=CARTESIAN_POINT('',(-10.5805717967516,-43.9579515042931,2.));
#69937=CARTESIAN_POINT('Origin',(-54.977096951452,-18.6485605554598,2.));
#69938=CARTESIAN_POINT('',(-45.2025619355918,-13.741459297751,2.));
#69939=CARTESIAN_POINT('Ctrl Pts',(-45.2025619355918,-13.741459297751,18.));
#69940=CARTESIAN_POINT('Ctrl Pts',(-45.2025619355918,-13.741459297751,15.3333333333333));
#69941=CARTESIAN_POINT('Ctrl Pts',(-45.2025619355918,-13.741459297751,12.6666666666667));
#69942=CARTESIAN_POINT('Ctrl Pts',(-45.2025619355918,-13.741459297751,7.33333333333333));
#69943=CARTESIAN_POINT('Ctrl Pts',(-45.2025619355918,-13.741459297751,4.66666666666667));
#69944=CARTESIAN_POINT('Ctrl Pts',(-45.2025619355918,-13.741459297751,2.));
#69945=CARTESIAN_POINT('',(-54.977096951452,-18.6485605554598,2.));
#69946=CARTESIAN_POINT('',(-54.977096951452,-18.6485605554598,2.));
#69947=CARTESIAN_POINT('',(-54.977096951452,-18.6485605554598,2.));
#69948=CARTESIAN_POINT('Origin',(-58.1177432099948,-12.3926560582107,2.));
#69949=CARTESIAN_POINT('',(-58.1177432099948,-12.3926560582107,2.));
#69950=CARTESIAN_POINT('',(-58.1177432099948,-12.3926560582107,2.));
#69951=CARTESIAN_POINT('',(-58.1177432099948,-12.3926560582107,2.));
#69952=CARTESIAN_POINT('Origin',(-46.4996348579608,-6.56002729234549,2.));
#69953=CARTESIAN_POINT('',(-46.4996348579608,-6.56002729234549,2.));
#69954=CARTESIAN_POINT('',(-46.4996348579608,-6.56002729234549,2.));
#69955=CARTESIAN_POINT('',(-46.4996348579608,-6.56002729234549,2.));
#69956=CARTESIAN_POINT('Origin',(-43.358988599418,-12.8159317895946,2.));
#69957=CARTESIAN_POINT('',(-46.0771487393297,-7.40158428157358,2.));
#69958=CARTESIAN_POINT('Ctrl Pts',(-46.0771487393297,-7.40158428157357,
2.));
#69959=CARTESIAN_POINT('Ctrl Pts',(-46.0771487393297,-7.40158428157357,
4.66666666666667));
#69960=CARTESIAN_POINT('Ctrl Pts',(-46.0771487393297,-7.40158428157357,
7.33333333333333));
#69961=CARTESIAN_POINT('Ctrl Pts',(-46.0771487393297,-7.40158428157357,
12.6666666666667));
#69962=CARTESIAN_POINT('Ctrl Pts',(-46.0771487393297,-7.40158428157357,
15.3333333333333));
#69963=CARTESIAN_POINT('Ctrl Pts',(-46.0771487393297,-7.40158428157357,
18.));
#69964=CARTESIAN_POINT('',(-43.358988599418,-12.8159317895946,2.));
#69965=CARTESIAN_POINT('Origin',(-43.6386756607666,38.2872823085476,2.));
#69966=CARTESIAN_POINT('',(-34.5017338047182,32.2758373034865,2.));
#69967=CARTESIAN_POINT('Ctrl Pts',(-34.5017338047182,32.2758373034865,18.));
#69968=CARTESIAN_POINT('Ctrl Pts',(-34.5017338047182,32.2758373034865,15.3333333333333));
#69969=CARTESIAN_POINT('Ctrl Pts',(-34.5017338047182,32.2758373034865,12.6666666666667));
#69970=CARTESIAN_POINT('Ctrl Pts',(-34.5017338047182,32.2758373034865,7.33333333333333));
#69971=CARTESIAN_POINT('Ctrl Pts',(-34.5017338047182,32.2758373034865,4.66666666666667));
#69972=CARTESIAN_POINT('Ctrl Pts',(-34.5017338047182,32.2758373034865,2.));
#69973=CARTESIAN_POINT('',(-43.6386756607666,38.2872823085476,2.));
#69974=CARTESIAN_POINT('',(-43.6386756607666,38.2872823085476,2.));
#69975=CARTESIAN_POINT('',(-43.6386756607666,38.2872823085476,2.));
#69976=CARTESIAN_POINT('Origin',(-39.791226571771,44.1351140013707,2.));
#69977=CARTESIAN_POINT('',(-39.791226571771,44.1351140013707,2.));
#69978=CARTESIAN_POINT('',(-39.791226571771,44.1351140013707,2.));
#69979=CARTESIAN_POINT('',(-39.791226571771,44.1351140013707,2.));
#69980=CARTESIAN_POINT('Origin',(-28.9309677136708,36.9898514075217,2.));
#69981=CARTESIAN_POINT('',(-28.9309677136708,36.9898514075217,2.));
#69982=CARTESIAN_POINT('',(-28.9309677136708,36.9898514075217,2.));
#69983=CARTESIAN_POINT('',(-28.9309677136708,36.9898514075217,2.));
#69984=CARTESIAN_POINT('Origin',(-32.7784168026664,31.1420197146986,2.));
#69985=CARTESIAN_POINT('',(-29.4485343857591,36.2031892014269,2.));
#69986=CARTESIAN_POINT('Ctrl Pts',(-29.4485343857591,36.2031892014269,2.));
#69987=CARTESIAN_POINT('Ctrl Pts',(-29.4485343857591,36.2031892014269,4.66666666666667));
#69988=CARTESIAN_POINT('Ctrl Pts',(-29.4485343857591,36.2031892014269,7.33333333333333));
#69989=CARTESIAN_POINT('Ctrl Pts',(-29.4485343857591,36.2031892014269,12.6666666666667));
#69990=CARTESIAN_POINT('Ctrl Pts',(-29.4485343857591,36.2031892014269,15.3333333333333));
#69991=CARTESIAN_POINT('Ctrl Pts',(-29.4485343857591,36.2031892014269,18.));
#69992=CARTESIAN_POINT('',(-32.7784168026664,31.1420197146986,2.));
#69993=CARTESIAN_POINT('Origin',(10.5805717967515,43.9579515042931,2.));
#69994=CARTESIAN_POINT('',(16.6286143540509,43.6047734828703,2.));
#69995=CARTESIAN_POINT('Ctrl Pts',(16.6286143535706,43.6047734830004,2.));
#69996=CARTESIAN_POINT('Ctrl Pts',(16.6286143535706,43.6047734830004,4.66666666666667));
#69997=CARTESIAN_POINT('Ctrl Pts',(16.6286143535706,43.6047734830004,7.33333333333333));
#69998=CARTESIAN_POINT('Ctrl Pts',(16.6286143535706,43.6047734830004,12.6666666666667));
#69999=CARTESIAN_POINT('Ctrl Pts',(16.6286143535706,43.6047734830004,15.3333333333333));
#70000=CARTESIAN_POINT('Ctrl Pts',(16.6286143535706,43.6047734830004,18.));
#70001=CARTESIAN_POINT('',(17.56866714429,43.5498786998672,2.));
#70002=CARTESIAN_POINT('',(10.5805717967515,43.9579515042931,2.));
#70003=CARTESIAN_POINT('',(17.56866714429,43.5498786998672,2.));
#70004=CARTESIAN_POINT('Origin',(11.3384212906854,56.9358428640073,2.));
#70005=CARTESIAN_POINT('',(10.7008281308737,46.0172966012375,2.));
#70006=CARTESIAN_POINT('Ctrl Pts',(10.7008281308737,46.0172966012375,18.));
#70007=CARTESIAN_POINT('Ctrl Pts',(10.7008281308737,46.0172966012375,15.3333333333333));
#70008=CARTESIAN_POINT('Ctrl Pts',(10.7008281308737,46.0172966012375,12.6666666666667));
#70009=CARTESIAN_POINT('Ctrl Pts',(10.7008281308737,46.0172966012375,7.33333333333333));
#70010=CARTESIAN_POINT('Ctrl Pts',(10.7008281308737,46.0172966012375,4.66666666666667));
#70011=CARTESIAN_POINT('Ctrl Pts',(10.7008281308737,46.0172966012375,2.));
#70012=CARTESIAN_POINT('',(11.3384212906854,56.9358428640073,2.));
#70013=CARTESIAN_POINT('',(11.3384212906854,56.9358428640073,2.));
#70014=CARTESIAN_POINT('',(11.3384212906854,56.9358428640073,2.));
#70015=CARTESIAN_POINT('Origin',(18.3265166382238,56.5277700595814,2.));
#70016=CARTESIAN_POINT('',(18.3265166382238,56.5277700595814,2.));
#70017=CARTESIAN_POINT('',(18.3265166382238,56.5277700595814,2.));
#70018=CARTESIAN_POINT('',(18.3265166382238,56.5277700595814,2.));
#70019=CARTESIAN_POINT('Origin',(17.56866714429,43.5498786998672,2.));
#70020=CARTESIAN_POINT('',(17.56866714429,43.5498786998672,2.));
#70021=CARTESIAN_POINT('Ctrl Pts',(46.0449384185095,-16.7589870229578,0.));
#70022=CARTESIAN_POINT('Ctrl Pts',(46.0449384185095,-16.7589870229578,20.));
#70023=CARTESIAN_POINT('Ctrl Pts',(46.0420594924752,-16.7651130917503,0.));
#70024=CARTESIAN_POINT('Ctrl Pts',(46.0420594924752,-16.7651130917503,20.));
#70025=CARTESIAN_POINT('Ctrl Pts',(46.0362995834799,-16.7773641333857,0.));
#70026=CARTESIAN_POINT('Ctrl Pts',(46.0362995834799,-16.7773641333857,20.));
#70027=CARTESIAN_POINT('Ctrl Pts',(46.0276535492064,-16.79573740799,0.));
#70028=CARTESIAN_POINT('Ctrl Pts',(46.0276535492064,-16.79573740799,20.));
#70029=CARTESIAN_POINT('Ctrl Pts',(46.0161131619282,-16.8202285317553,0.));
#70030=CARTESIAN_POINT('Ctrl Pts',(46.0161131619282,-16.8202285317553,20.));
#70031=CARTESIAN_POINT('Ctrl Pts',(46.0016671088634,-16.8508314760754,0.));
#70032=CARTESIAN_POINT('Ctrl Pts',(46.0016671088634,-16.8508314760754,20.));
#70033=CARTESIAN_POINT('Ctrl Pts',(45.9872004880192,-16.8814234574889,0.));
#70034=CARTESIAN_POINT('Ctrl Pts',(45.9872004880192,-16.8814234574889,20.));
#70035=CARTESIAN_POINT('Ctrl Pts',(45.9727133019197,-16.9120044710149,0.));
#70036=CARTESIAN_POINT('Ctrl Pts',(45.9727133019197,-16.9120044710149,20.));
#70037=CARTESIAN_POINT('Ctrl Pts',(45.9582055548827,-16.9425745084438,0.));
#70038=CARTESIAN_POINT('Ctrl Pts',(45.9582055548827,-16.9425745084438,20.));
#70039=CARTESIAN_POINT('Ctrl Pts',(45.9436772535459,-16.9731335574459,0.));
#70040=CARTESIAN_POINT('Ctrl Pts',(45.9436772535459,-16.9731335574459,20.));
#70041=CARTESIAN_POINT('Ctrl Pts',(45.9291284062576,-17.0036816026634,0.));
#70042=CARTESIAN_POINT('Ctrl Pts',(45.9291284062576,-17.0036816026634,20.));
#70043=CARTESIAN_POINT('Ctrl Pts',(45.91455902239,-17.0342186269342,0.));
#70044=CARTESIAN_POINT('Ctrl Pts',(45.91455902239,-17.0342186269342,20.));
#70045=CARTESIAN_POINT('Ctrl Pts',(45.8999691116666,-17.0647446124944,0.));
#70046=CARTESIAN_POINT('Ctrl Pts',(45.8999691116666,-17.0647446124944,20.));
#70047=CARTESIAN_POINT('Ctrl Pts',(45.8853586835176,-17.09525954213,0.));
#70048=CARTESIAN_POINT('Ctrl Pts',(45.8853586835176,-17.09525954213,20.));
#70049=CARTESIAN_POINT('Ctrl Pts',(45.8707277463338,-17.1257634005084,0.));
#70050=CARTESIAN_POINT('Ctrl Pts',(45.8707277463338,-17.1257634005084,20.));
#70051=CARTESIAN_POINT('Ctrl Pts',(45.8560763076625,-17.1562561738292,0.));
#70052=CARTESIAN_POINT('Ctrl Pts',(45.8560763076625,-17.1562561738292,20.));
#70053=CARTESIAN_POINT('Ctrl Pts',(45.8414043745501,-17.1867378492105,0.));
#70054=CARTESIAN_POINT('Ctrl Pts',(45.8414043745501,-17.1867378492105,20.));
#70055=CARTESIAN_POINT('Ctrl Pts',(45.8267119538424,-17.2172084141516,0.));
#70056=CARTESIAN_POINT('Ctrl Pts',(45.8267119538424,-17.2172084141516,20.));
#70057=CARTESIAN_POINT('Ctrl Pts',(45.8119990524823,-17.247667856,0.));
#70058=CARTESIAN_POINT('Ctrl Pts',(45.8119990524823,-17.247667856,20.));
#70059=CARTESIAN_POINT('Ctrl Pts',(45.7972656778619,-17.2781161613228,0.));
#70060=CARTESIAN_POINT('Ctrl Pts',(45.7972656778619,-17.2781161613228,20.));
#70061=CARTESIAN_POINT('Ctrl Pts',(45.7825118377706,-17.3085533159982,0.));
#70062=CARTESIAN_POINT('Ctrl Pts',(45.7825118377706,-17.3085533159982,20.));
#70063=CARTESIAN_POINT('Ctrl Pts',(45.7677375402375,-17.3389793054985,0.));
#70064=CARTESIAN_POINT('Ctrl Pts',(45.7677375402375,-17.3389793054985,20.));
#70065=CARTESIAN_POINT('Ctrl Pts',(45.7529427934047,-17.3693941151172,0.));
#70066=CARTESIAN_POINT('Ctrl Pts',(45.7529427934047,-17.3693941151172,20.));
#70067=CARTESIAN_POINT('Ctrl Pts',(45.7381276053971,-17.3997977302007,0.));
#70068=CARTESIAN_POINT('Ctrl Pts',(45.7381276053971,-17.3997977302007,20.));
#70069=CARTESIAN_POINT('Ctrl Pts',(45.7232919841685,-17.4301901364248,0.));
#70070=CARTESIAN_POINT('Ctrl Pts',(45.7232919841685,-17.4301901364248,20.));
#70071=CARTESIAN_POINT('Ctrl Pts',(45.7084359375081,-17.460571319782,0.));
#70072=CARTESIAN_POINT('Ctrl Pts',(45.7084359375081,-17.460571319782,20.));
#70073=CARTESIAN_POINT('Ctrl Pts',(45.6935594731126,-17.490941266452,0.));
#70074=CARTESIAN_POINT('Ctrl Pts',(45.6935594731126,-17.490941266452,20.));
#70075=CARTESIAN_POINT('Ctrl Pts',(45.67866259864,-17.5212999627071,0.));
#70076=CARTESIAN_POINT('Ctrl Pts',(45.67866259864,-17.5212999627071,20.));
#70077=CARTESIAN_POINT('Ctrl Pts',(45.6637453217655,-17.5516473948116,0.));
#70078=CARTESIAN_POINT('Ctrl Pts',(45.6637453217655,-17.5516473948116,20.));
#70079=CARTESIAN_POINT('Ctrl Pts',(45.6488076502485,-17.5819835489016,0.));
#70080=CARTESIAN_POINT('Ctrl Pts',(45.6488076502485,-17.5819835489016,20.));
#70081=CARTESIAN_POINT('Ctrl Pts',(45.6338495919363,-17.6123084109794,0.));
#70082=CARTESIAN_POINT('Ctrl Pts',(45.6338495919363,-17.6123084109794,20.));
#70083=CARTESIAN_POINT('Ctrl Pts',(45.6188711547313,-17.6426219669712,0.));
#70084=CARTESIAN_POINT('Ctrl Pts',(45.6188711547313,-17.6426219669712,20.));
#70085=CARTESIAN_POINT('Ctrl Pts',(45.6038723465685,-17.672924202767,0.));
#70086=CARTESIAN_POINT('Ctrl Pts',(45.6038723465685,-17.672924202767,20.));
#70087=CARTESIAN_POINT('Ctrl Pts',(45.5888531753911,-17.7032151042646,0.));
#70088=CARTESIAN_POINT('Ctrl Pts',(45.5888531753911,-17.7032151042646,20.));
#70089=CARTESIAN_POINT('Ctrl Pts',(45.5738136491221,-17.7334946574206,0.));
#70090=CARTESIAN_POINT('Ctrl Pts',(45.5738136491221,-17.7334946574206,20.));
#70091=CARTESIAN_POINT('Ctrl Pts',(45.5587537756595,-17.7637628482589,0.));
#70092=CARTESIAN_POINT('Ctrl Pts',(45.5587537756595,-17.7637628482589,20.));
#70093=CARTESIAN_POINT('Ctrl Pts',(45.5436735628911,-17.7940196628443,0.));
#70094=CARTESIAN_POINT('Ctrl Pts',(45.5436735628911,-17.7940196628443,20.));
#70095=CARTESIAN_POINT('Ctrl Pts',(45.528573018704,-17.8242650872661,0.));
#70096=CARTESIAN_POINT('Ctrl Pts',(45.528573018704,-17.8242650872661,20.));
#70097=CARTESIAN_POINT('Ctrl Pts',(45.5134521509949,-17.8544991076192,0.));
#70098=CARTESIAN_POINT('Ctrl Pts',(45.5134521509949,-17.8544991076192,20.));
#70099=CARTESIAN_POINT('Ctrl Pts',(45.498310967683,-17.8847217099814,0.));
#70100=CARTESIAN_POINT('Ctrl Pts',(45.498310967683,-17.8847217099814,20.));
#70101=CARTESIAN_POINT('Ctrl Pts',(45.4831494767122,-17.9149328804084,0.));
#70102=CARTESIAN_POINT('Ctrl Pts',(45.4831494767122,-17.9149328804084,20.));
#70103=CARTESIAN_POINT('Ctrl Pts',(45.4679676860453,-17.9451326049449,0.));
#70104=CARTESIAN_POINT('Ctrl Pts',(45.4679676860453,-17.9451326049449,20.));
#70105=CARTESIAN_POINT('Ctrl Pts',(45.4527656036598,-17.9753208696316,0.));
#70106=CARTESIAN_POINT('Ctrl Pts',(45.4527656036598,-17.9753208696316,20.));
#70107=CARTESIAN_POINT('Ctrl Pts',(45.4375432375433,-18.0054976605138,0.));
#70108=CARTESIAN_POINT('Ctrl Pts',(45.4375432375433,-18.0054976605138,20.));
#70109=CARTESIAN_POINT('Ctrl Pts',(45.4223005956881,-18.0356629636502,0.));
#70110=CARTESIAN_POINT('Ctrl Pts',(45.4223005956881,-18.0356629636502,20.));
#70111=CARTESIAN_POINT('Ctrl Pts',(45.4070376860893,-18.0658167651176,0.));
#70112=CARTESIAN_POINT('Ctrl Pts',(45.4070376860893,-18.0658167651176,20.));
#70113=CARTESIAN_POINT('Ctrl Pts',(45.3917545167484,-18.0959590510046,0.));
#70114=CARTESIAN_POINT('Ctrl Pts',(45.3917545167484,-18.0959590510046,20.));
#70115=CARTESIAN_POINT('Ctrl Pts',(45.3764510956741,-18.1260898074095,0.));
#70116=CARTESIAN_POINT('Ctrl Pts',(45.3764510956741,-18.1260898074095,20.));
#70117=CARTESIAN_POINT('Ctrl Pts',(45.3611274308852,-18.156209020436,0.));
#70118=CARTESIAN_POINT('Ctrl Pts',(45.3611274308852,-18.156209020436,20.));
#70119=CARTESIAN_POINT('Ctrl Pts',(45.3457835304119,-18.1863166761898,0.));
#70120=CARTESIAN_POINT('Ctrl Pts',(45.3457835304119,-18.1863166761898,20.));
#70121=CARTESIAN_POINT('Ctrl Pts',(45.3304194022976,-18.2164127607761,0.));
#70122=CARTESIAN_POINT('Ctrl Pts',(45.3304194022976,-18.2164127607761,20.));
#70123=CARTESIAN_POINT('Ctrl Pts',(45.3150350545965,-18.2464972603023,0.));
#70124=CARTESIAN_POINT('Ctrl Pts',(45.3150350545965,-18.2464972603023,20.));
#70125=CARTESIAN_POINT('Ctrl Pts',(45.299630495374,-18.276570160879,0.));
#70126=CARTESIAN_POINT('Ctrl Pts',(45.299630495374,-18.276570160879,20.));
#70127=CARTESIAN_POINT('Ctrl Pts',(45.2842057327048,-18.3066314486215,0.));
#70128=CARTESIAN_POINT('Ctrl Pts',(45.2842057327048,-18.3066314486215,20.));
#70129=CARTESIAN_POINT('Ctrl Pts',(45.2687607746732,-18.3366811096519,0.));
#70130=CARTESIAN_POINT('Ctrl Pts',(45.2687607746732,-18.3366811096519,20.));
#70131=CARTESIAN_POINT('Ctrl Pts',(45.2532956293718,-18.3667191300999,0.));
#70132=CARTESIAN_POINT('Ctrl Pts',(45.2532956293718,-18.3667191300999,20.));
#70133=CARTESIAN_POINT('Ctrl Pts',(45.2378103049022,-18.3967454961017,0.));
#70134=CARTESIAN_POINT('Ctrl Pts',(45.2378103049022,-18.3967454961017,20.));
#70135=CARTESIAN_POINT('Ctrl Pts',(45.2223048093755,-18.4267601937997,0.));
#70136=CARTESIAN_POINT('Ctrl Pts',(45.2223048093755,-18.4267601937997,20.));
#70137=CARTESIAN_POINT('Ctrl Pts',(45.2067791509123,-18.456763209342,0.));
#70138=CARTESIAN_POINT('Ctrl Pts',(45.2067791509123,-18.456763209342,20.));
#70139=CARTESIAN_POINT('Ctrl Pts',(45.1912333376434,-18.4867545288811,0.));
#70140=CARTESIAN_POINT('Ctrl Pts',(45.1912333376434,-18.4867545288811,20.));
#70141=CARTESIAN_POINT('Ctrl Pts',(45.1756673777099,-18.5167341385735,0.));
#70142=CARTESIAN_POINT('Ctrl Pts',(45.1756673777099,-18.5167341385735,20.));
#70143=CARTESIAN_POINT('Ctrl Pts',(45.1600812792631,-18.5467020245809,0.));
#70144=CARTESIAN_POINT('Ctrl Pts',(45.1600812792631,-18.5467020245809,20.));
#70145=CARTESIAN_POINT('Ctrl Pts',(45.144475050464,-18.5766581730695,0.));
#70146=CARTESIAN_POINT('Ctrl Pts',(45.144475050464,-18.5766581730695,20.));
#70147=CARTESIAN_POINT('Ctrl Pts',(45.1288486994834,-18.6066025702107,0.));
#70148=CARTESIAN_POINT('Ctrl Pts',(45.1288486994834,-18.6066025702107,20.));
#70149=CARTESIAN_POINT('Ctrl Pts',(45.1132022345013,-18.6365352021814,0.));
#70150=CARTESIAN_POINT('Ctrl Pts',(45.1132022345013,-18.6365352021814,20.));
#70151=CARTESIAN_POINT('Ctrl Pts',(45.097535663708,-18.6664560551643,0.));
#70152=CARTESIAN_POINT('Ctrl Pts',(45.097535663708,-18.6664560551643,20.));
#70153=CARTESIAN_POINT('Ctrl Pts',(45.081848995303,-18.6963651153477,0.));
#70154=CARTESIAN_POINT('Ctrl Pts',(45.081848995303,-18.6963651153477,20.));
#70155=CARTESIAN_POINT('Ctrl Pts',(45.0661422374956,-18.7262623689254,0.));
#70156=CARTESIAN_POINT('Ctrl Pts',(45.0661422374956,-18.7262623689254,20.));
#70157=CARTESIAN_POINT('Ctrl Pts',(45.050415398505,-18.7561478020964,0.));
#70158=CARTESIAN_POINT('Ctrl Pts',(45.050415398505,-18.7561478020964,20.));
#70159=CARTESIAN_POINT('Ctrl Pts',(45.0346684865594,-18.7860214010651,0.));
#70160=CARTESIAN_POINT('Ctrl Pts',(45.0346684865594,-18.7860214010651,20.));
#70161=CARTESIAN_POINT('Ctrl Pts',(45.0189015098976,-18.815883152041,0.));
#70162=CARTESIAN_POINT('Ctrl Pts',(45.0189015098976,-18.815883152041,20.));
#70163=CARTESIAN_POINT('Ctrl Pts',(45.0031144767678,-18.8457330412389,0.));
#70164=CARTESIAN_POINT('Ctrl Pts',(45.0031144767678,-18.8457330412389,20.));
#70165=CARTESIAN_POINT('Ctrl Pts',(44.987307395428,-18.8755710548788,0.));
#70166=CARTESIAN_POINT('Ctrl Pts',(44.987307395428,-18.8755710548788,20.));
#70167=CARTESIAN_POINT('Ctrl Pts',(44.971480274146,-18.9053971791858,0.));
#70168=CARTESIAN_POINT('Ctrl Pts',(44.971480274146,-18.9053971791858,20.));
#70169=CARTESIAN_POINT('Ctrl Pts',(44.9556331211993,-18.9352114003906,0.));
#70170=CARTESIAN_POINT('Ctrl Pts',(44.9556331211993,-18.9352114003906,20.));
#70171=CARTESIAN_POINT('Ctrl Pts',(44.9397659448752,-18.9650137047294,0.));
#70172=CARTESIAN_POINT('Ctrl Pts',(44.9397659448752,-18.9650137047294,20.));
#70173=CARTESIAN_POINT('Ctrl Pts',(44.9238787534705,-18.9948040784434,0.));
#70174=CARTESIAN_POINT('Ctrl Pts',(44.9238787534705,-18.9948040784434,20.));
#70175=CARTESIAN_POINT('Ctrl Pts',(44.9079715552916,-19.0245825077798,0.));
#70176=CARTESIAN_POINT('Ctrl Pts',(44.9079715552916,-19.0245825077798,20.));
#70177=CARTESIAN_POINT('Ctrl Pts',(44.8920443586544,-19.0543489789907,0.));
#70178=CARTESIAN_POINT('Ctrl Pts',(44.8920443586544,-19.0543489789907,20.));
#70179=CARTESIAN_POINT('Ctrl Pts',(44.8760971718851,-19.0841034783341,0.));
#70180=CARTESIAN_POINT('Ctrl Pts',(44.8760971718851,-19.0841034783341,20.));
#70181=CARTESIAN_POINT('Ctrl Pts',(44.8601300033192,-19.1138459920731,0.));
#70182=CARTESIAN_POINT('Ctrl Pts',(44.8601300033192,-19.1138459920731,20.));
#70183=CARTESIAN_POINT('Ctrl Pts',(44.8441428613021,-19.143576506476,0.));
#70184=CARTESIAN_POINT('Ctrl Pts',(44.8441428613021,-19.143576506476,20.));
#70185=CARTESIAN_POINT('Ctrl Pts',(44.8281357541891,-19.1732950078169,0.));
#70186=CARTESIAN_POINT('Ctrl Pts',(44.8281357541891,-19.1732950078169,20.));
#70187=CARTESIAN_POINT('Ctrl Pts',(44.8121086903447,-19.2030014823748,0.));
#70188=CARTESIAN_POINT('Ctrl Pts',(44.8121086903447,-19.2030014823748,20.));
#70189=CARTESIAN_POINT('Ctrl Pts',(44.7960616781431,-19.2326959164344,0.));
#70190=CARTESIAN_POINT('Ctrl Pts',(44.7960616781431,-19.2326959164344,20.));
#70191=CARTESIAN_POINT('Ctrl Pts',(44.7799947259683,-19.2623782962859,0.));
#70192=CARTESIAN_POINT('Ctrl Pts',(44.7799947259683,-19.2623782962859,20.));
#70193=CARTESIAN_POINT('Ctrl Pts',(44.7639078422139,-19.2920486082247,0.));
#70194=CARTESIAN_POINT('Ctrl Pts',(44.7639078422139,-19.2920486082247,20.));
#70195=CARTESIAN_POINT('Ctrl Pts',(44.7478010352831,-19.321706838552,0.));
#70196=CARTESIAN_POINT('Ctrl Pts',(44.7478010352831,-19.321706838552,20.));
#70197=CARTESIAN_POINT('Ctrl Pts',(44.731674313589,-19.3513529735741,0.));
#70198=CARTESIAN_POINT('Ctrl Pts',(44.731674313589,-19.3513529735741,20.));
#70199=CARTESIAN_POINT('Ctrl Pts',(44.7155276855546,-19.3809869996033,0.));
#70200=CARTESIAN_POINT('Ctrl Pts',(44.7155276855546,-19.3809869996033,20.));
#70201=CARTESIAN_POINT('Ctrl Pts',(44.6993611596123,-19.4106089029568,0.));
#70202=CARTESIAN_POINT('Ctrl Pts',(44.6993611596123,-19.4106089029568,20.));
#70203=CARTESIAN_POINT('Ctrl Pts',(44.6831747442042,-19.4402186699576,0.));
#70204=CARTESIAN_POINT('Ctrl Pts',(44.6831747442042,-19.4402186699576,20.));
#70205=CARTESIAN_POINT('Ctrl Pts',(44.6669684477819,-19.4698162869338,0.));
#70206=CARTESIAN_POINT('Ctrl Pts',(44.6669684477819,-19.4698162869338,20.));
#70207=CARTESIAN_POINT('Ctrl Pts',(44.6507422788067,-19.4994017402193,0.));
#70208=CARTESIAN_POINT('Ctrl Pts',(44.6507422788067,-19.4994017402193,20.));
#70209=CARTESIAN_POINT('Ctrl Pts',(44.6344962457493,-19.5289750161534,0.));
#70210=CARTESIAN_POINT('Ctrl Pts',(44.6344962457493,-19.5289750161534,20.));
#70211=CARTESIAN_POINT('Ctrl Pts',(44.6182303570903,-19.5585361010809,0.));
#70212=CARTESIAN_POINT('Ctrl Pts',(44.6182303570903,-19.5585361010809,20.));
#70213=CARTESIAN_POINT('Ctrl Pts',(44.60194462132,-19.5880849813526,0.));
#70214=CARTESIAN_POINT('Ctrl Pts',(44.60194462132,-19.5880849813526,20.));
#70215=CARTESIAN_POINT('Ctrl Pts',(44.5856390469384,-19.6176216433241,0.));
#70216=CARTESIAN_POINT('Ctrl Pts',(44.5856390469384,-19.6176216433241,20.));
#70217=CARTESIAN_POINT('Ctrl Pts',(44.5693136424548,-19.6471460733569,0.));
#70218=CARTESIAN_POINT('Ctrl Pts',(44.5693136424548,-19.6471460733569,20.));
#70219=CARTESIAN_POINT('Ctrl Pts',(44.5529684163885,-19.6766582578175,0.));
#70220=CARTESIAN_POINT('Ctrl Pts',(44.5529684163885,-19.6766582578175,20.));
#70221=CARTESIAN_POINT('Ctrl Pts',(44.5366033772681,-19.7061581830785,0.));
#70222=CARTESIAN_POINT('Ctrl Pts',(44.5366033772681,-19.7061581830785,20.));
#70223=CARTESIAN_POINT('Ctrl Pts',(44.5202185336324,-19.7356458355178,0.));
#70224=CARTESIAN_POINT('Ctrl Pts',(44.5202185336324,-19.7356458355178,20.));
#70225=CARTESIAN_POINT('Ctrl Pts',(44.5038138940293,-19.7651212015191,0.));
#70226=CARTESIAN_POINT('Ctrl Pts',(44.5038138940293,-19.7651212015191,20.));
#70227=CARTESIAN_POINT('Ctrl Pts',(44.4873894670167,-19.7945842674717,0.));
#70228=CARTESIAN_POINT('Ctrl Pts',(44.4873894670167,-19.7945842674717,20.));
#70229=CARTESIAN_POINT('Ctrl Pts',(44.4709452611615,-19.8240350197702,0.));
#70230=CARTESIAN_POINT('Ctrl Pts',(44.4709452611615,-19.8240350197702,20.));
#70231=CARTESIAN_POINT('Ctrl Pts',(44.4544812850403,-19.8534734448147,0.));
#70232=CARTESIAN_POINT('Ctrl Pts',(44.4544812850403,-19.8534734448147,20.));
#70233=CARTESIAN_POINT('Ctrl Pts',(44.4379975472397,-19.8828995290107,0.));
#70234=CARTESIAN_POINT('Ctrl Pts',(44.4379975472397,-19.8828995290107,20.));
#70235=CARTESIAN_POINT('Ctrl Pts',(44.4214940563556,-19.9123132587698,0.));
#70236=CARTESIAN_POINT('Ctrl Pts',(44.4214940563556,-19.9123132587698,20.));
#70237=CARTESIAN_POINT('Ctrl Pts',(44.4049708209939,-19.9417146205087,0.));
#70238=CARTESIAN_POINT('Ctrl Pts',(44.4049708209939,-19.9417146205087,20.));
#70239=CARTESIAN_POINT('Ctrl Pts',(44.3884278497697,-19.9711036006504,0.));
#70240=CARTESIAN_POINT('Ctrl Pts',(44.3884278497697,-19.9711036006504,20.));
#70241=CARTESIAN_POINT('Ctrl Pts',(44.371865151308,-20.0004801856229,0.));
#70242=CARTESIAN_POINT('Ctrl Pts',(44.371865151308,-20.0004801856229,20.));
#70243=CARTESIAN_POINT('Ctrl Pts',(44.3552827342435,-20.0298443618602,0.));
#70244=CARTESIAN_POINT('Ctrl Pts',(44.3552827342435,-20.0298443618602,20.));
#70245=CARTESIAN_POINT('Ctrl Pts',(44.3386806072204,-20.0591961158019,0.));
#70246=CARTESIAN_POINT('Ctrl Pts',(44.3386806072204,-20.0591961158019,20.));
#70247=CARTESIAN_POINT('Ctrl Pts',(44.3220587788923,-20.0885354338929,0.));
#70248=CARTESIAN_POINT('Ctrl Pts',(44.3220587788923,-20.0885354338929,20.));
#70249=CARTESIAN_POINT('Ctrl Pts',(44.3054172579221,-20.117862302584,0.));
#70250=CARTESIAN_POINT('Ctrl Pts',(44.3054172579221,-20.117862302584,20.));
#70251=CARTESIAN_POINT('Ctrl Pts',(44.2887560529826,-20.1471767083313,0.));
#70252=CARTESIAN_POINT('Ctrl Pts',(44.2887560529826,-20.1471767083313,20.));
#70253=CARTESIAN_POINT('Ctrl Pts',(44.2720751727557,-20.1764786375963,0.));
#70254=CARTESIAN_POINT('Ctrl Pts',(44.2720751727557,-20.1764786375963,20.));
#70255=CARTESIAN_POINT('Ctrl Pts',(44.2553746259333,-20.2057680768465,0.));
#70256=CARTESIAN_POINT('Ctrl Pts',(44.2553746259333,-20.2057680768465,20.));
#70257=CARTESIAN_POINT('Ctrl Pts',(44.238654421217,-20.2350450125552,0.));
#70258=CARTESIAN_POINT('Ctrl Pts',(44.238654421217,-20.2350450125552,20.));
#70259=CARTESIAN_POINT('Ctrl Pts',(44.221914567318,-20.2643094312016,0.));
#70260=CARTESIAN_POINT('Ctrl Pts',(44.221914567318,-20.2643094312016,20.));
#70261=CARTESIAN_POINT('Ctrl Pts',(44.205155072957,-20.2935613192706,0.));
#70262=CARTESIAN_POINT('Ctrl Pts',(44.205155072957,-20.2935613192706,20.));
#70263=CARTESIAN_POINT('Ctrl Pts',(44.1883759468646,-20.3228006632528,0.));
#70264=CARTESIAN_POINT('Ctrl Pts',(44.1883759468646,-20.3228006632528,20.));
#70265=CARTESIAN_POINT('Ctrl Pts',(44.1715771977807,-20.3520274496444,0.));
#70266=CARTESIAN_POINT('Ctrl Pts',(44.1715771977807,-20.3520274496444,20.));
#70267=CARTESIAN_POINT('Ctrl Pts',(44.1547588344544,-20.3812416649468,0.));
#70268=CARTESIAN_POINT('Ctrl Pts',(44.1547588344544,-20.3812416649468,20.));
#70269=CARTESIAN_POINT('Ctrl Pts',(44.1379208656442,-20.4104432956673,0.));
#70270=CARTESIAN_POINT('Ctrl Pts',(44.1379208656442,-20.4104432956673,20.));
#70271=CARTESIAN_POINT('Ctrl Pts',(44.1210633001184,-20.4396323283186,0.));
#70272=CARTESIAN_POINT('Ctrl Pts',(44.1210633001184,-20.4396323283186,20.));
#70273=CARTESIAN_POINT('Ctrl Pts',(44.1041861466545,-20.4688087494191,0.));
#70274=CARTESIAN_POINT('Ctrl Pts',(44.1041861466545,-20.4688087494191,20.));
#70275=CARTESIAN_POINT('Ctrl Pts',(44.0872894140398,-20.4979725454933,0.));
#70276=CARTESIAN_POINT('Ctrl Pts',(44.0872894140398,-20.4979725454933,20.));
#70277=CARTESIAN_POINT('Ctrl Pts',(44.0703731110714,-20.5271237030716,0.));
#70278=CARTESIAN_POINT('Ctrl Pts',(44.0703731110714,-20.5271237030716,20.));
#70279=CARTESIAN_POINT('Ctrl Pts',(44.053437246556,-20.5562622086905,0.));
#70280=CARTESIAN_POINT('Ctrl Pts',(44.053437246556,-20.5562622086905,20.));
#70281=CARTESIAN_POINT('Ctrl Pts',(44.03648182931,-20.5853880488919,0.));
#70282=CARTESIAN_POINT('Ctrl Pts',(44.03648182931,-20.5853880488919,20.));
#70283=CARTESIAN_POINT('Ctrl Pts',(44.0195068681592,-20.6145012102233,0.));
#70284=CARTESIAN_POINT('Ctrl Pts',(44.0195068681592,-20.6145012102233,20.));
#70285=CARTESIAN_POINT('Ctrl Pts',(44.0025123719387,-20.6436016792381,0.));
#70286=CARTESIAN_POINT('Ctrl Pts',(44.0025123719387,-20.6436016792381,20.));
#70287=CARTESIAN_POINT('Ctrl Pts',(43.9854983494929,-20.6726894424949,0.));
#70288=CARTESIAN_POINT('Ctrl Pts',(43.9854983494929,-20.6726894424949,20.));
#70289=CARTESIAN_POINT('Ctrl Pts',(43.9684648096756,-20.7017644865585,0.));
#70290=CARTESIAN_POINT('Ctrl Pts',(43.9684648096756,-20.7017644865585,20.));
#70291=CARTESIAN_POINT('Ctrl Pts',(43.9514117613501,-20.7308267979991,0.));
#70292=CARTESIAN_POINT('Ctrl Pts',(43.9514117613501,-20.7308267979991,20.));
#70293=CARTESIAN_POINT('Ctrl Pts',(43.9343392133895,-20.7598763633934,0.));
#70294=CARTESIAN_POINT('Ctrl Pts',(43.9343392133895,-20.7598763633934,20.));
#70295=CARTESIAN_POINT('Ctrl Pts',(43.9172471746767,-20.7889131693233,0.));
#70296=CARTESIAN_POINT('Ctrl Pts',(43.9172471746767,-20.7889131693233,20.));
#70297=CARTESIAN_POINT('Ctrl Pts',(43.9001356541037,-20.817937202377,0.));
#70298=CARTESIAN_POINT('Ctrl Pts',(43.9001356541037,-20.817937202377,20.));
#70299=CARTESIAN_POINT('Ctrl Pts',(43.8830046605723,-20.8469484491482,0.));
#70300=CARTESIAN_POINT('Ctrl Pts',(43.8830046605723,-20.8469484491482,20.));
#70301=CARTESIAN_POINT('Ctrl Pts',(43.8658542029936,-20.8759468962364,0.));
#70302=CARTESIAN_POINT('Ctrl Pts',(43.8658542029936,-20.8759468962364,20.));
#70303=CARTESIAN_POINT('Ctrl Pts',(43.8486842902882,-20.9049325302471,0.));
#70304=CARTESIAN_POINT('Ctrl Pts',(43.8486842902882,-20.9049325302471,20.));
#70305=CARTESIAN_POINT('Ctrl Pts',(43.8314949313861,-20.9339053377914,0.));
#70306=CARTESIAN_POINT('Ctrl Pts',(43.8314949313861,-20.9339053377914,20.));
#70307=CARTESIAN_POINT('Ctrl Pts',(43.8142861352268,-20.9628653054863,0.));
#70308=CARTESIAN_POINT('Ctrl Pts',(43.8142861352268,-20.9628653054863,20.));
#70309=CARTESIAN_POINT('Ctrl Pts',(43.7970579107591,-20.9918124199547,0.));
#70310=CARTESIAN_POINT('Ctrl Pts',(43.7970579107591,-20.9918124199547,20.));
#70311=CARTESIAN_POINT('Ctrl Pts',(43.7798102669417,-21.0207466678254,0.));
#70312=CARTESIAN_POINT('Ctrl Pts',(43.7798102669417,-21.0207466678254,20.));
#70313=CARTESIAN_POINT('Ctrl Pts',(43.7625432127426,-21.0496680357328,0.));
#70314=CARTESIAN_POINT('Ctrl Pts',(43.7625432127426,-21.0496680357328,20.));
#70315=CARTESIAN_POINT('Ctrl Pts',(43.7452567571393,-21.0785765103173,0.));
#70316=CARTESIAN_POINT('Ctrl Pts',(43.7452567571393,-21.0785765103173,20.));
#70317=CARTESIAN_POINT('Ctrl Pts',(43.7279509091188,-21.1074720782252,0.));
#70318=CARTESIAN_POINT('Ctrl Pts',(43.7279509091188,-21.1074720782252,20.));
#70319=CARTESIAN_POINT('Ctrl Pts',(43.7106256776774,-21.1363547261089,0.));
#70320=CARTESIAN_POINT('Ctrl Pts',(43.7106256776774,-21.1363547261089,20.));
#70321=CARTESIAN_POINT('Ctrl Pts',(43.6932810718209,-21.1652244406266,0.));
#70322=CARTESIAN_POINT('Ctrl Pts',(43.6932810718209,-21.1652244406266,20.));
#70323=CARTESIAN_POINT('Ctrl Pts',(43.6759171005641,-21.1940812084419,0.));
#70324=CARTESIAN_POINT('Ctrl Pts',(43.6759171005641,-21.1940812084419,20.));
#70325=CARTESIAN_POINT('Ctrl Pts',(43.658533772932,-21.2229250162246,0.));
#70326=CARTESIAN_POINT('Ctrl Pts',(43.658533772932,-21.2229250162246,20.));
#70327=CARTESIAN_POINT('Ctrl Pts',(43.6411310979584,-21.2517558506503,0.));
#70328=CARTESIAN_POINT('Ctrl Pts',(43.6411310979584,-21.2517558506503,20.));
#70329=CARTESIAN_POINT('Ctrl Pts',(43.6237090846874,-21.2805736984008,0.));
#70330=CARTESIAN_POINT('Ctrl Pts',(43.6237090846874,-21.2805736984008,20.));
#70331=CARTESIAN_POINT('Ctrl Pts',(43.6062677421718,-21.3093785461635,0.));
#70332=CARTESIAN_POINT('Ctrl Pts',(43.6062677421718,-21.3093785461635,20.));
#70333=CARTESIAN_POINT('Ctrl Pts',(43.5888070794743,-21.3381703806324,0.));
#70334=CARTESIAN_POINT('Ctrl Pts',(43.5888070794743,-21.3381703806324,20.));
#70335=CARTESIAN_POINT('Ctrl Pts',(43.571327105667,-21.3669491885068,0.));
#70336=CARTESIAN_POINT('Ctrl Pts',(43.571327105667,-21.3669491885068,20.));
#70337=CARTESIAN_POINT('Ctrl Pts',(43.5538278298311,-21.3957149564922,0.));
#70338=CARTESIAN_POINT('Ctrl Pts',(43.5538278298311,-21.3957149564922,20.));
#70339=CARTESIAN_POINT('Ctrl Pts',(43.5363092610574,-21.4244676712999,0.));
#70340=CARTESIAN_POINT('Ctrl Pts',(43.5363092610574,-21.4244676712999,20.));
#70341=CARTESIAN_POINT('Ctrl Pts',(43.5187714084458,-21.4532073196468,0.));
#70342=CARTESIAN_POINT('Ctrl Pts',(43.5187714084458,-21.4532073196468,20.));
#70343=CARTESIAN_POINT('Ctrl Pts',(43.5012142811058,-21.4819338882558,0.));
#70344=CARTESIAN_POINT('Ctrl Pts',(43.5012142811058,-21.4819338882558,20.));
#70345=CARTESIAN_POINT('Ctrl Pts',(43.4836378881563,-21.5106473638561,0.));
#70346=CARTESIAN_POINT('Ctrl Pts',(43.4836378881563,-21.5106473638561,20.));
#70347=CARTESIAN_POINT('Ctrl Pts',(43.4660422387257,-21.5393477331829,0.));
#70348=CARTESIAN_POINT('Ctrl Pts',(43.4660422387257,-21.5393477331829,20.));
#70349=CARTESIAN_POINT('Ctrl Pts',(43.4484273419519,-21.5680349829774,0.));
#70350=CARTESIAN_POINT('Ctrl Pts',(43.4484273419519,-21.5680349829774,20.));
#70351=CARTESIAN_POINT('Ctrl Pts',(43.4307932069823,-21.5967090999869,0.));
#70352=CARTESIAN_POINT('Ctrl Pts',(43.4307932069823,-21.5967090999869,20.));
#70353=CARTESIAN_POINT('Ctrl Pts',(43.4131398429739,-21.6253700709647,0.));
#70354=CARTESIAN_POINT('Ctrl Pts',(43.4131398429739,-21.6253700709647,20.));
#70355=CARTESIAN_POINT('Ctrl Pts',(43.3954672590924,-21.6540178826698,0.));
#70356=CARTESIAN_POINT('Ctrl Pts',(43.3954672590924,-21.6540178826698,20.));
#70357=CARTESIAN_POINT('Ctrl Pts',(43.3777754645132,-21.682652521867,0.));
#70358=CARTESIAN_POINT('Ctrl Pts',(43.3777754645132,-21.682652521867,20.));
#70359=CARTESIAN_POINT('Ctrl Pts',(43.3600644684208,-21.7112739753274,0.));
#70360=CARTESIAN_POINT('Ctrl Pts',(43.3600644684208,-21.7112739753274,20.));
#70361=CARTESIAN_POINT('Ctrl Pts',(43.3423342800096,-21.7398822298281,0.));
#70362=CARTESIAN_POINT('Ctrl Pts',(43.3423342800096,-21.7398822298281,20.));
#70363=CARTESIAN_POINT('Ctrl Pts',(43.3245849084831,-21.7684772721522,0.));
#70364=CARTESIAN_POINT('Ctrl Pts',(43.3245849084831,-21.7684772721522,20.));
#70365=CARTESIAN_POINT('Ctrl Pts',(43.3068163630542,-21.7970590890891,0.));
#70366=CARTESIAN_POINT('Ctrl Pts',(43.3068163630542,-21.7970590890891,20.));
#70367=CARTESIAN_POINT('Ctrl Pts',(43.2890286529453,-21.825627667434,0.));
#70368=CARTESIAN_POINT('Ctrl Pts',(43.2890286529453,-21.825627667434,20.));
#70369=CARTESIAN_POINT('Ctrl Pts',(43.271221787388,-21.854182993988,0.));
#70370=CARTESIAN_POINT('Ctrl Pts',(43.271221787388,-21.854182993988,20.));
#70371=CARTESIAN_POINT('Ctrl Pts',(43.2533957756234,-21.8827250555584,0.));
#70372=CARTESIAN_POINT('Ctrl Pts',(43.2533957756234,-21.8827250555584,20.));
#70373=CARTESIAN_POINT('Ctrl Pts',(43.2355506269018,-21.9112538389586,0.));
#70374=CARTESIAN_POINT('Ctrl Pts',(43.2355506269018,-21.9112538389586,20.));
#70375=CARTESIAN_POINT('Ctrl Pts',(43.217686350483,-21.939769331008,0.));
#70376=CARTESIAN_POINT('Ctrl Pts',(43.217686350483,-21.939769331008,20.));
#70377=CARTESIAN_POINT('Ctrl Pts',(43.1998029556363,-21.9682715185322,0.));
#70378=CARTESIAN_POINT('Ctrl Pts',(43.1998029556363,-21.9682715185322,20.));
#70379=CARTESIAN_POINT('Ctrl Pts',(43.1819004516401,-21.9967603883628,0.));
#70380=CARTESIAN_POINT('Ctrl Pts',(43.1819004516401,-21.9967603883628,20.));
#70381=CARTESIAN_POINT('Ctrl Pts',(43.1639788477821,-22.0252359273374,0.));
#70382=CARTESIAN_POINT('Ctrl Pts',(43.1639788477821,-22.0252359273374,20.));
#70383=CARTESIAN_POINT('Ctrl Pts',(43.1460381533593,-22.0536981222997,0.));
#70384=CARTESIAN_POINT('Ctrl Pts',(43.1460381533593,-22.0536981222997,20.));
#70385=CARTESIAN_POINT('Ctrl Pts',(43.1280783776784,-22.0821469600998,0.));
#70386=CARTESIAN_POINT('Ctrl Pts',(43.1280783776784,-22.0821469600998,20.));
#70387=CARTESIAN_POINT('Ctrl Pts',(43.1100995300552,-22.1105824275933,0.));
#70388=CARTESIAN_POINT('Ctrl Pts',(43.1100995300552,-22.1105824275933,20.));
#70389=CARTESIAN_POINT('Ctrl Pts',(43.0921016198148,-22.1390045116426,0.));
#70390=CARTESIAN_POINT('Ctrl Pts',(43.0921016198148,-22.1390045116426,20.));
#70391=CARTESIAN_POINT('Ctrl Pts',(43.0740846562917,-22.1674131991155,0.));
#70392=CARTESIAN_POINT('Ctrl Pts',(43.0740846562917,-22.1674131991155,20.));
#70393=CARTESIAN_POINT('Ctrl Pts',(43.0560486488298,-22.1958084768868,0.));
#70394=CARTESIAN_POINT('Ctrl Pts',(43.0560486488298,-22.1958084768868,20.));
#70395=CARTESIAN_POINT('Ctrl Pts',(43.0379936067822,-22.2241903318366,0.));
#70396=CARTESIAN_POINT('Ctrl Pts',(43.0379936067822,-22.2241903318366,20.));
#70397=CARTESIAN_POINT('Ctrl Pts',(43.0199195395114,-22.252558750852,0.));
#70398=CARTESIAN_POINT('Ctrl Pts',(43.0199195395114,-22.252558750852,20.));
#70399=CARTESIAN_POINT('Ctrl Pts',(43.0018264563892,-22.2809137208256,0.));
#70400=CARTESIAN_POINT('Ctrl Pts',(43.0018264563892,-22.2809137208256,20.));
#70401=CARTESIAN_POINT('Ctrl Pts',(42.9837143667967,-22.3092552286565,0.));
#70402=CARTESIAN_POINT('Ctrl Pts',(42.9837143667967,-22.3092552286565,20.));
#70403=CARTESIAN_POINT('Ctrl Pts',(42.965583280124,-22.3375832612492,0.));
#70404=CARTESIAN_POINT('Ctrl Pts',(42.965583280124,-22.3375832612492,20.));
#70405=CARTESIAN_POINT('Ctrl Pts',(42.947433205771,-22.3658978055149,0.));
#70406=CARTESIAN_POINT('Ctrl Pts',(42.947433205771,-22.3658978055149,20.));
#70407=CARTESIAN_POINT('Ctrl Pts',(42.9292641531465,-22.3941988483709,0.));
#70408=CARTESIAN_POINT('Ctrl Pts',(42.9292641531465,-22.3941988483709,20.));
#70409=CARTESIAN_POINT('Ctrl Pts',(42.9110761316689,-22.4224863767407,0.));
#70410=CARTESIAN_POINT('Ctrl Pts',(42.9110761316689,-22.4224863767407,20.));
#70411=CARTESIAN_POINT('Ctrl Pts',(42.8928691507659,-22.4507603775546,0.));
#70412=CARTESIAN_POINT('Ctrl Pts',(42.8928691507659,-22.4507603775546,20.));
#70413=CARTESIAN_POINT('Ctrl Pts',(42.8746432198743,-22.4790208377489,0.));
#70414=CARTESIAN_POINT('Ctrl Pts',(42.8746432198743,-22.4790208377489,20.));
#70415=CARTESIAN_POINT('Ctrl Pts',(42.8563983484404,-22.5072677442656,0.));
#70416=CARTESIAN_POINT('Ctrl Pts',(42.8563983484404,-22.5072677442656,20.));
#70417=CARTESIAN_POINT('Ctrl Pts',(42.8381345459193,-22.5355010840531,0.));
#70418=CARTESIAN_POINT('Ctrl Pts',(42.8381345459193,-22.5355010840531,20.));
#70419=CARTESIAN_POINT('Ctrl Pts',(42.8198518217756,-22.5637208440656,0.));
#70420=CARTESIAN_POINT('Ctrl Pts',(42.8198518217756,-22.5637208440656,20.));
#70421=CARTESIAN_POINT('Ctrl Pts',(42.8015501854832,-22.5919270112639,0.));
#70422=CARTESIAN_POINT('Ctrl Pts',(42.8015501854832,-22.5919270112639,20.));
#70423=CARTESIAN_POINT('Ctrl Pts',(42.7832296465255,-22.6201195726151,0.));
#70424=CARTESIAN_POINT('Ctrl Pts',(42.7832296465255,-22.6201195726151,20.));
#70425=CARTESIAN_POINT('Ctrl Pts',(42.7648902143955,-22.6482985150925,0.));
#70426=CARTESIAN_POINT('Ctrl Pts',(42.7648902143955,-22.6482985150925,20.));
#70427=CARTESIAN_POINT('Ctrl Pts',(42.7465318985949,-22.6764638256759,0.));
#70428=CARTESIAN_POINT('Ctrl Pts',(42.7465318985949,-22.6764638256759,20.));
#70429=CARTESIAN_POINT('Ctrl Pts',(42.7281547086347,-22.7046154913512,0.));
#70430=CARTESIAN_POINT('Ctrl Pts',(42.7281547086347,-22.7046154913512,20.));
#70431=CARTESIAN_POINT('Ctrl Pts',(42.7097586540349,-22.7327534991101,0.));
#70432=CARTESIAN_POINT('Ctrl Pts',(42.7097586540349,-22.7327534991101,20.));
#70433=CARTESIAN_POINT('Ctrl Pts',(42.6913437443248,-22.7608778359508,0.));
#70434=CARTESIAN_POINT('Ctrl Pts',(42.6913437443248,-22.7608778359508,20.));
#70435=CARTESIAN_POINT('Ctrl Pts',(42.6729099890431,-22.788988488878,0.));
#70436=CARTESIAN_POINT('Ctrl Pts',(42.6729099890431,-22.788988488878,20.));
#70437=CARTESIAN_POINT('Ctrl Pts',(42.6544573977378,-22.8170854449024,0.));
#70438=CARTESIAN_POINT('Ctrl Pts',(42.6544573977378,-22.8170854449024,20.));
#70439=CARTESIAN_POINT('Ctrl Pts',(42.6359859799663,-22.845168691041,0.));
#70440=CARTESIAN_POINT('Ctrl Pts',(42.6359859799663,-22.845168691041,20.));
#70441=CARTESIAN_POINT('Ctrl Pts',(42.6174957452953,-22.8732382143175,0.));
#70442=CARTESIAN_POINT('Ctrl Pts',(42.6174957452953,-22.8732382143175,20.));
#70443=CARTESIAN_POINT('Ctrl Pts',(42.5989867033005,-22.9012940017616,0.));
#70444=CARTESIAN_POINT('Ctrl Pts',(42.5989867033005,-22.9012940017616,20.));
#70445=CARTESIAN_POINT('Ctrl Pts',(42.5804588635669,-22.9293360404095,0.));
#70446=CARTESIAN_POINT('Ctrl Pts',(42.5804588635669,-22.9293360404095,20.));
#70447=CARTESIAN_POINT('Ctrl Pts',(42.5619122356886,-22.9573643173034,0.));
#70448=CARTESIAN_POINT('Ctrl Pts',(42.5619122356886,-22.9573643173034,20.));
#70449=CARTESIAN_POINT('Ctrl Pts',(42.5433468292689,-22.9853788194919,0.));
#70450=CARTESIAN_POINT('Ctrl Pts',(42.5433468292689,-22.9853788194919,20.));
#70451=CARTESIAN_POINT('Ctrl Pts',(42.5247626539203,-23.0133795340299,0.));
#70452=CARTESIAN_POINT('Ctrl Pts',(42.5247626539203,-23.0133795340299,20.));
#70453=CARTESIAN_POINT('Ctrl Pts',(42.5061597192647,-23.0413664479785,0.));
#70454=CARTESIAN_POINT('Ctrl Pts',(42.5061597192647,-23.0413664479785,20.));
#70455=CARTESIAN_POINT('Ctrl Pts',(42.4875380349329,-23.0693395484056,0.));
#70456=CARTESIAN_POINT('Ctrl Pts',(42.4875380349329,-23.0693395484056,20.));
#70457=CARTESIAN_POINT('Ctrl Pts',(42.4688976105654,-23.097298822385,0.));
#70458=CARTESIAN_POINT('Ctrl Pts',(42.4688976105654,-23.097298822385,20.));
#70459=CARTESIAN_POINT('Ctrl Pts',(42.4502384558115,-23.1252442569971,0.));
#70460=CARTESIAN_POINT('Ctrl Pts',(42.4502384558115,-23.1252442569971,20.));
#70461=CARTESIAN_POINT('Ctrl Pts',(42.4315605803297,-23.1531758393284,0.));
#70462=CARTESIAN_POINT('Ctrl Pts',(42.4315605803297,-23.1531758393284,20.));
#70463=CARTESIAN_POINT('Ctrl Pts',(42.4128639937879,-23.1810935564721,0.));
#70464=CARTESIAN_POINT('Ctrl Pts',(42.4128639937879,-23.1810935564721,20.));
#70465=CARTESIAN_POINT('Ctrl Pts',(42.3941487058631,-23.2089973955278,0.));
#70466=CARTESIAN_POINT('Ctrl Pts',(42.3941487058631,-23.2089973955278,20.));
#70467=CARTESIAN_POINT('Ctrl Pts',(42.3754147262417,-23.2368873436013,0.));
#70468=CARTESIAN_POINT('Ctrl Pts',(42.3754147262417,-23.2368873436013,20.));
#70469=CARTESIAN_POINT('Ctrl Pts',(42.3566620646188,-23.2647633878047,0.));
#70470=CARTESIAN_POINT('Ctrl Pts',(42.3566620646188,-23.2647633878047,20.));
#70471=CARTESIAN_POINT('Ctrl Pts',(42.3378907306988,-23.2926255152563,0.));
#70472=CARTESIAN_POINT('Ctrl Pts',(42.3378907306988,-23.2926255152563,20.));
#70473=CARTESIAN_POINT('Ctrl Pts',(42.3191007341954,-23.320473713081,0.));
#70474=CARTESIAN_POINT('Ctrl Pts',(42.3191007341954,-23.320473713081,20.));
#70475=CARTESIAN_POINT('Ctrl Pts',(42.3002920848317,-23.3483079684104,0.));
#70476=CARTESIAN_POINT('Ctrl Pts',(42.3002920848317,-23.3483079684104,20.));
#70477=CARTESIAN_POINT('Ctrl Pts',(42.2814647923395,-23.3761282683822,0.));
#70478=CARTESIAN_POINT('Ctrl Pts',(42.2814647923395,-23.3761282683822,20.));
#70479=CARTESIAN_POINT('Ctrl Pts',(42.2626188664603,-23.4039346001409,0.));
#70480=CARTESIAN_POINT('Ctrl Pts',(42.2626188664603,-23.4039346001409,20.));
#70481=CARTESIAN_POINT('Ctrl Pts',(42.2437543169442,-23.4317269508371,0.));
#70482=CARTESIAN_POINT('Ctrl Pts',(42.2437543169442,-23.4317269508371,20.));
#70483=CARTESIAN_POINT('Ctrl Pts',(42.2248711535508,-23.4595053076278,0.));
#70484=CARTESIAN_POINT('Ctrl Pts',(42.2248711535508,-23.4595053076278,20.));
#70485=CARTESIAN_POINT('Ctrl Pts',(42.2059693860486,-23.4872696576759,0.));
#70486=CARTESIAN_POINT('Ctrl Pts',(42.2059693860486,-23.4872696576759,20.));
#70487=CARTESIAN_POINT('Ctrl Pts',(42.1870490242153,-23.5150199881515,0.));
#70488=CARTESIAN_POINT('Ctrl Pts',(42.1870490242153,-23.5150199881515,20.));
#70489=CARTESIAN_POINT('Ctrl Pts',(42.1681100778379,-23.5427562862308,0.));
#70490=CARTESIAN_POINT('Ctrl Pts',(42.1681100778379,-23.5427562862308,20.));
#70491=CARTESIAN_POINT('Ctrl Pts',(42.1491525567126,-23.5704785390969,0.));
#70492=CARTESIAN_POINT('Ctrl Pts',(42.1491525567126,-23.5704785390969,20.));
#70493=CARTESIAN_POINT('Ctrl Pts',(42.1301764706447,-23.5981867339395,0.));
#70494=CARTESIAN_POINT('Ctrl Pts',(42.1301764706447,-23.5981867339395,20.));
#70495=CARTESIAN_POINT('Ctrl Pts',(42.1111818294483,-23.6258808579543,0.));
#70496=CARTESIAN_POINT('Ctrl Pts',(42.1111818294483,-23.6258808579543,20.));
#70497=CARTESIAN_POINT('Ctrl Pts',(42.0921686429469,-23.6535608983436,0.));
#70498=CARTESIAN_POINT('Ctrl Pts',(42.0921686429469,-23.6535608983436,20.));
#70499=CARTESIAN_POINT('Ctrl Pts',(42.0731369209731,-23.6812268423159,0.));
#70500=CARTESIAN_POINT('Ctrl Pts',(42.0731369209731,-23.6812268423159,20.));
#70501=CARTESIAN_POINT('Ctrl Pts',(42.0540866733685,-23.7088786770864,0.));
#70502=CARTESIAN_POINT('Ctrl Pts',(42.0540866733685,-23.7088786770864,20.));
#70503=CARTESIAN_POINT('Ctrl Pts',(42.0350179099839,-23.7365163898768,0.));
#70504=CARTESIAN_POINT('Ctrl Pts',(42.0350179099839,-23.7365163898768,20.));
#70505=CARTESIAN_POINT('Ctrl Pts',(42.0159306406794,-23.7641399679152,0.));
#70506=CARTESIAN_POINT('Ctrl Pts',(42.0159306406794,-23.7641399679152,20.));
#70507=CARTESIAN_POINT('Ctrl Pts',(41.9968248753238,-23.7917493984363,0.));
#70508=CARTESIAN_POINT('Ctrl Pts',(41.9968248753238,-23.7917493984363,20.));
#70509=CARTESIAN_POINT('Ctrl Pts',(41.9777006237952,-23.8193446686815,0.));
#70510=CARTESIAN_POINT('Ctrl Pts',(41.9777006237952,-23.8193446686815,20.));
#70511=CARTESIAN_POINT('Ctrl Pts',(41.9585578959806,-23.8469257658985,0.));
#70512=CARTESIAN_POINT('Ctrl Pts',(41.9585578959806,-23.8469257658985,20.));
#70513=CARTESIAN_POINT('Ctrl Pts',(41.9393967017767,-23.8744926773418,0.));
#70514=CARTESIAN_POINT('Ctrl Pts',(41.9393967017767,-23.8744926773418,20.));
#70515=CARTESIAN_POINT('Ctrl Pts',(41.9202170510888,-23.9020453902722,0.));
#70516=CARTESIAN_POINT('Ctrl Pts',(41.9202170510888,-23.9020453902722,20.));
#70517=CARTESIAN_POINT('Ctrl Pts',(41.9010189538314,-23.9295838919573,0.));
#70518=CARTESIAN_POINT('Ctrl Pts',(41.9010189538314,-23.9295838919573,20.));
#70519=CARTESIAN_POINT('Ctrl Pts',(41.8818024199281,-23.9571081696708,0.));
#70520=CARTESIAN_POINT('Ctrl Pts',(41.8818024199281,-23.9571081696708,20.));
#70521=CARTESIAN_POINT('Ctrl Pts',(41.8625674593112,-23.9846182106931,0.));
#70522=CARTESIAN_POINT('Ctrl Pts',(41.8625674593112,-23.9846182106931,20.));
#70523=CARTESIAN_POINT('Ctrl Pts',(41.8433140819226,-24.0121140023113,0.));
#70524=CARTESIAN_POINT('Ctrl Pts',(41.8433140819226,-24.0121140023113,20.));
#70525=CARTESIAN_POINT('Ctrl Pts',(41.824042297713,-24.0395955318191,0.));
#70526=CARTESIAN_POINT('Ctrl Pts',(41.824042297713,-24.0395955318191,20.));
#70527=CARTESIAN_POINT('Ctrl Pts',(41.8047521166422,-24.0670627865166,0.));
#70528=CARTESIAN_POINT('Ctrl Pts',(41.8047521166422,-24.0670627865166,20.));
#70529=CARTESIAN_POINT('Ctrl Pts',(41.785443548679,-24.0945157537107,0.));
#70530=CARTESIAN_POINT('Ctrl Pts',(41.785443548679,-24.0945157537107,20.));
#70531=CARTESIAN_POINT('Ctrl Pts',(41.7661166038015,-24.1219544207148,0.));
#70532=CARTESIAN_POINT('Ctrl Pts',(41.7661166038015,-24.1219544207148,20.));
#70533=CARTESIAN_POINT('Ctrl Pts',(41.7467712919966,-24.1493787748488,0.));
#70534=CARTESIAN_POINT('Ctrl Pts',(41.7467712919966,-24.1493787748488,20.));
#70535=CARTESIAN_POINT('Ctrl Pts',(41.7274076232604,-24.1767888034393,0.));
#70536=CARTESIAN_POINT('Ctrl Pts',(41.7274076232604,-24.1767888034393,20.));
#70537=CARTESIAN_POINT('Ctrl Pts',(41.7080256075983,-24.2041844938197,0.));
#70538=CARTESIAN_POINT('Ctrl Pts',(41.7080256075983,-24.2041844938197,20.));
#70539=CARTESIAN_POINT('Ctrl Pts',(41.688625255024,-24.2315658333297,0.));
#70540=CARTESIAN_POINT('Ctrl Pts',(41.688625255024,-24.2315658333297,20.));
#70541=CARTESIAN_POINT('Ctrl Pts',(41.6692065755608,-24.2589328093159,0.));
#70542=CARTESIAN_POINT('Ctrl Pts',(41.6692065755608,-24.2589328093159,20.));
#70543=CARTESIAN_POINT('Ctrl Pts',(41.6497695792407,-24.2862854091312,0.));
#70544=CARTESIAN_POINT('Ctrl Pts',(41.6497695792407,-24.2862854091312,20.));
#70545=CARTESIAN_POINT('Ctrl Pts',(41.630314276105,-24.3136236201351,0.));
#70546=CARTESIAN_POINT('Ctrl Pts',(41.630314276105,-24.3136236201351,20.));
#70547=CARTESIAN_POINT('Ctrl Pts',(41.610840676204,-24.3409474296941,0.));
#70548=CARTESIAN_POINT('Ctrl Pts',(41.610840676204,-24.3409474296941,20.));
#70549=CARTESIAN_POINT('Ctrl Pts',(41.5913487895971,-24.368256825181,0.));
#70550=CARTESIAN_POINT('Ctrl Pts',(41.5913487895971,-24.368256825181,20.));
#70551=CARTESIAN_POINT('Ctrl Pts',(41.5718386263526,-24.3955517939757,0.));
#70552=CARTESIAN_POINT('Ctrl Pts',(41.5718386263526,-24.3955517939757,20.));
#70553=CARTESIAN_POINT('Ctrl Pts',(41.5523101965477,-24.4228323234645,0.));
#70554=CARTESIAN_POINT('Ctrl Pts',(41.5523101965477,-24.4228323234645,20.));
#70555=CARTESIAN_POINT('Ctrl Pts',(41.5327635102685,-24.4500984010406,0.));
#70556=CARTESIAN_POINT('Ctrl Pts',(41.5327635102685,-24.4500984010406,20.));
#70557=CARTESIAN_POINT('Ctrl Pts',(41.5131985776101,-24.4773500141037,0.));
#70558=CARTESIAN_POINT('Ctrl Pts',(41.5131985776101,-24.4773500141037,20.));
#70559=CARTESIAN_POINT('Ctrl Pts',(41.4936154086768,-24.5045871500598,0.));
#70560=CARTESIAN_POINT('Ctrl Pts',(41.4936154086768,-24.5045871500598,20.));
#70561=CARTESIAN_POINT('Ctrl Pts',(41.4740140135823,-24.5318097963223,0.));
#70562=CARTESIAN_POINT('Ctrl Pts',(41.4740140135823,-24.5318097963223,20.));
#70563=CARTESIAN_POINT('Ctrl Pts',(41.4543944024488,-24.5590179403106,0.));
#70564=CARTESIAN_POINT('Ctrl Pts',(41.4543944024488,-24.5590179403106,20.));
#70565=CARTESIAN_POINT('Ctrl Pts',(41.4347565854076,-24.5862115694513,0.));
#70566=CARTESIAN_POINT('Ctrl Pts',(41.4347565854076,-24.5862115694513,20.));
#70567=CARTESIAN_POINT('Ctrl Pts',(41.4151005725989,-24.6133906711774,0.));
#70568=CARTESIAN_POINT('Ctrl Pts',(41.4151005725989,-24.6133906711774,20.));
#70569=CARTESIAN_POINT('Ctrl Pts',(41.3954263741717,-24.6405552329289,0.));
#70570=CARTESIAN_POINT('Ctrl Pts',(41.3954263741717,-24.6405552329289,20.));
#70571=CARTESIAN_POINT('Ctrl Pts',(41.3757340002844,-24.6677052421523,0.));
#70572=CARTESIAN_POINT('Ctrl Pts',(41.3757340002844,-24.6677052421523,20.));
#70573=CARTESIAN_POINT('Ctrl Pts',(41.3560234611038,-24.694840686301,0.));
#70574=CARTESIAN_POINT('Ctrl Pts',(41.3560234611038,-24.694840686301,20.));
#70575=CARTESIAN_POINT('Ctrl Pts',(41.3362947668064,-24.7219615528352,0.));
#70576=CARTESIAN_POINT('Ctrl Pts',(41.3362947668064,-24.7219615528352,20.));
#70577=CARTESIAN_POINT('Ctrl Pts',(41.3165479275773,-24.7490678292217,0.));
#70578=CARTESIAN_POINT('Ctrl Pts',(41.3165479275773,-24.7490678292217,20.));
#70579=CARTESIAN_POINT('Ctrl Pts',(41.2967829536105,-24.7761595029341,0.));
#70580=CARTESIAN_POINT('Ctrl Pts',(41.2967829536105,-24.7761595029341,20.));
#70581=CARTESIAN_POINT('Ctrl Pts',(41.276999855109,-24.8032365614526,0.));
#70582=CARTESIAN_POINT('Ctrl Pts',(41.276999855109,-24.8032365614526,20.));
#70583=CARTESIAN_POINT('Ctrl Pts',(41.2571986422843,-24.8302989922639,0.));
#70584=CARTESIAN_POINT('Ctrl Pts',(41.2571986422843,-24.8302989922639,20.));
#70585=CARTESIAN_POINT('Ctrl Pts',(41.2373793253577,-24.8573467828623,0.));
#70586=CARTESIAN_POINT('Ctrl Pts',(41.2373793253577,-24.8573467828623,20.));
#70587=CARTESIAN_POINT('Ctrl Pts',(41.2175419145588,-24.8843799207483,0.));
#70588=CARTESIAN_POINT('Ctrl Pts',(41.2175419145588,-24.8843799207483,20.));
#70589=CARTESIAN_POINT('Ctrl Pts',(41.1976864201268,-24.9113983934294,0.));
#70590=CARTESIAN_POINT('Ctrl Pts',(41.1976864201268,-24.9113983934294,20.));
#70591=CARTESIAN_POINT('Ctrl Pts',(41.1778128523092,-24.9384021884197,0.));
#70592=CARTESIAN_POINT('Ctrl Pts',(41.1778128523092,-24.9384021884197,20.));
#70593=CARTESIAN_POINT('Ctrl Pts',(41.1579212213625,-24.9653912932403,0.));
#70594=CARTESIAN_POINT('Ctrl Pts',(41.1579212213625,-24.9653912932403,20.));
#70595=CARTESIAN_POINT('Ctrl Pts',(41.1380115375521,-24.9923656954187,0.));
#70596=CARTESIAN_POINT('Ctrl Pts',(41.1380115375521,-24.9923656954187,20.));
#70597=CARTESIAN_POINT('Ctrl Pts',(41.1180838111525,-25.0193253824897,0.));
#70598=CARTESIAN_POINT('Ctrl Pts',(41.1180838111525,-25.0193253824897,20.));
#70599=CARTESIAN_POINT('Ctrl Pts',(41.0981380524472,-25.0462703419947,0.));
#70600=CARTESIAN_POINT('Ctrl Pts',(41.0981380524472,-25.0462703419947,20.));
#70601=CARTESIAN_POINT('Ctrl Pts',(41.0781742717283,-25.0732005614819,0.));
#70602=CARTESIAN_POINT('Ctrl Pts',(41.0781742717283,-25.0732005614819,20.));
#70603=CARTESIAN_POINT('Ctrl Pts',(41.058192479297,-25.1001160285063,0.));
#70604=CARTESIAN_POINT('Ctrl Pts',(41.058192479297,-25.1001160285063,20.));
#70605=CARTESIAN_POINT('Ctrl Pts',(41.0381926854635,-25.1270167306298,0.));
#70606=CARTESIAN_POINT('Ctrl Pts',(41.0381926854635,-25.1270167306298,20.));
#70607=CARTESIAN_POINT('Ctrl Pts',(41.0181749005471,-25.1539026554213,0.));
#70608=CARTESIAN_POINT('Ctrl Pts',(41.0181749005471,-25.1539026554213,20.));
#70609=CARTESIAN_POINT('Ctrl Pts',(40.9981391348755,-25.1807737904566,0.));
#70610=CARTESIAN_POINT('Ctrl Pts',(40.9981391348755,-25.1807737904566,20.));
#70611=CARTESIAN_POINT('Ctrl Pts',(40.9780853987856,-25.2076301233182,0.));
#70612=CARTESIAN_POINT('Ctrl Pts',(40.9780853987856,-25.2076301233182,20.));
#70613=CARTESIAN_POINT('Ctrl Pts',(40.9580137026228,-25.2344716415952,0.));
#70614=CARTESIAN_POINT('Ctrl Pts',(40.9580137026228,-25.2344716415952,20.));
#70615=CARTESIAN_POINT('Ctrl Pts',(40.9379240567416,-25.2612983328836,0.));
#70616=CARTESIAN_POINT('Ctrl Pts',(40.9379240567416,-25.2612983328836,20.));
#70617=CARTESIAN_POINT('Ctrl Pts',(40.9178164715051,-25.2881101847862,0.));
#70618=CARTESIAN_POINT('Ctrl Pts',(40.9178164715051,-25.2881101847862,20.));
#70619=CARTESIAN_POINT('Ctrl Pts',(40.8976909572856,-25.3149071849127,0.));
#70620=CARTESIAN_POINT('Ctrl Pts',(40.8976909572856,-25.3149071849127,20.));
#70621=CARTESIAN_POINT('Ctrl Pts',(40.8775475244644,-25.3416893208803,0.));
#70622=CARTESIAN_POINT('Ctrl Pts',(40.8775475244644,-25.3416893208803,20.));
#70623=CARTESIAN_POINT('Ctrl Pts',(40.8573861834315,-25.3684565803126,0.));
#70624=CARTESIAN_POINT('Ctrl Pts',(40.8573861834315,-25.3684565803126,20.));
#70625=CARTESIAN_POINT('Ctrl Pts',(40.8372069445861,-25.3952089508407,0.));
#70626=CARTESIAN_POINT('Ctrl Pts',(40.8372069445861,-25.3952089508407,20.));
#70627=CARTESIAN_POINT('Ctrl Pts',(40.8170098183361,-25.4219464201024,0.));
#70628=CARTESIAN_POINT('Ctrl Pts',(40.8170098183361,-25.4219464201024,20.));
#70629=CARTESIAN_POINT('Ctrl Pts',(40.796794815098,-25.4486689757422,0.));
#70630=CARTESIAN_POINT('Ctrl Pts',(40.796794815098,-25.4486689757422,20.));
#70631=CARTESIAN_POINT('Ctrl Pts',(40.7765619452973,-25.4753766054114,0.));
#70632=CARTESIAN_POINT('Ctrl Pts',(40.7765619452973,-25.4753766054114,20.));
#70633=CARTESIAN_POINT('Ctrl Pts',(40.7563112193678,-25.5020692967677,0.));
#70634=CARTESIAN_POINT('Ctrl Pts',(40.7563112193678,-25.5020692967677,20.));
#70635=CARTESIAN_POINT('Ctrl Pts',(40.7360426477524,-25.528747037476,0.));
#70636=CARTESIAN_POINT('Ctrl Pts',(40.7360426477524,-25.528747037476,20.));
#70637=CARTESIAN_POINT('Ctrl Pts',(40.715756240903,-25.5554098152083,0.));
#70638=CARTESIAN_POINT('Ctrl Pts',(40.715756240903,-25.5554098152083,20.));
#70639=CARTESIAN_POINT('Ctrl Pts',(40.6954520092804,-25.5820576176439,0.));
#70640=CARTESIAN_POINT('Ctrl Pts',(40.6954520092804,-25.5820576176439,20.));
#70641=CARTESIAN_POINT('Ctrl Pts',(40.6751299633542,-25.6086904324689,0.));
#70642=CARTESIAN_POINT('Ctrl Pts',(40.6751299633542,-25.6086904324689,20.));
#70643=CARTESIAN_POINT('Ctrl Pts',(40.6547901136033,-25.6353082473769,0.));
#70644=CARTESIAN_POINT('Ctrl Pts',(40.6547901136033,-25.6353082473769,20.));
#70645=CARTESIAN_POINT('Ctrl Pts',(40.6344324705148,-25.6619110500678,0.));
#70646=CARTESIAN_POINT('Ctrl Pts',(40.6344324705148,-25.6619110500678,20.));
#70647=CARTESIAN_POINT('Ctrl Pts',(40.6140570445846,-25.6884988282486,0.));
#70648=CARTESIAN_POINT('Ctrl Pts',(40.6140570445846,-25.6884988282486,20.));
#70649=CARTESIAN_POINT('Ctrl Pts',(40.5936638463177,-25.7150715696333,0.));
#70650=CARTESIAN_POINT('Ctrl Pts',(40.5936638463177,-25.7150715696333,20.));
#70651=CARTESIAN_POINT('Ctrl Pts',(40.5732528862276,-25.7416292619425,0.));
#70652=CARTESIAN_POINT('Ctrl Pts',(40.5732528862276,-25.7416292619425,20.));
#70653=CARTESIAN_POINT('Ctrl Pts',(40.5528241748366,-25.768171892904,0.));
#70654=CARTESIAN_POINT('Ctrl Pts',(40.5528241748366,-25.768171892904,20.));
#70655=CARTESIAN_POINT('Ctrl Pts',(40.5323777226757,-25.7946994502526,0.));
#70656=CARTESIAN_POINT('Ctrl Pts',(40.5323777226757,-25.7946994502526,20.));
#70657=CARTESIAN_POINT('Ctrl Pts',(40.5119135402852,-25.8212119217304,0.));
#70658=CARTESIAN_POINT('Ctrl Pts',(40.5119135402852,-25.8212119217304,20.));
#70659=CARTESIAN_POINT('Ctrl Pts',(40.491431638214,-25.8477092950863,0.));
#70660=CARTESIAN_POINT('Ctrl Pts',(40.491431638214,-25.8477092950863,20.));
#70661=CARTESIAN_POINT('Ctrl Pts',(40.4709320270197,-25.8741915580762,0.));
#70662=CARTESIAN_POINT('Ctrl Pts',(40.4709320270197,-25.8741915580762,20.));
#70663=CARTESIAN_POINT('Ctrl Pts',(40.4504147172684,-25.9006586984631,0.));
#70664=CARTESIAN_POINT('Ctrl Pts',(40.4504147172684,-25.9006586984631,20.));
#70665=CARTESIAN_POINT('Ctrl Pts',(40.4298797195352,-25.9271107040169,0.));
#70666=CARTESIAN_POINT('Ctrl Pts',(40.4298797195352,-25.9271107040169,20.));
#70667=CARTESIAN_POINT('Ctrl Pts',(40.4093270444043,-25.953547562515,0.));
#70668=CARTESIAN_POINT('Ctrl Pts',(40.4093270444043,-25.953547562515,20.));
#70669=CARTESIAN_POINT('Ctrl Pts',(40.3887567024682,-25.9799692617416,0.));
#70670=CARTESIAN_POINT('Ctrl Pts',(40.3887567024682,-25.9799692617416,20.));
#70671=CARTESIAN_POINT('Ctrl Pts',(40.3681687043283,-26.0063757894875,0.));
#70672=CARTESIAN_POINT('Ctrl Pts',(40.3681687043283,-26.0063757894875,20.));
#70673=CARTESIAN_POINT('Ctrl Pts',(40.347563060595,-26.0327671335511,0.));
#70674=CARTESIAN_POINT('Ctrl Pts',(40.347563060595,-26.0327671335511,20.));
#70675=CARTESIAN_POINT('Ctrl Pts',(40.326939781887,-26.0591432817373,0.));
#70676=CARTESIAN_POINT('Ctrl Pts',(40.326939781887,-26.0591432817373,20.));
#70677=CARTESIAN_POINT('Ctrl Pts',(40.3062988788318,-26.0855042218584,0.));
#70678=CARTESIAN_POINT('Ctrl Pts',(40.3062988788318,-26.0855042218584,20.));
#70679=CARTESIAN_POINT('Ctrl Pts',(40.2856403620657,-26.1118499417334,0.));
#70680=CARTESIAN_POINT('Ctrl Pts',(40.2856403620657,-26.1118499417334,20.));
#70681=CARTESIAN_POINT('Ctrl Pts',(40.2649642422341,-26.1381804291893,0.));
#70682=CARTESIAN_POINT('Ctrl Pts',(40.2649642422341,-26.1381804291893,20.));
#70683=CARTESIAN_POINT('Ctrl Pts',(40.2442705299908,-26.1644956720595,0.));
#70684=CARTESIAN_POINT('Ctrl Pts',(40.2442705299908,-26.1644956720595,20.));
#70685=CARTESIAN_POINT('Ctrl Pts',(40.2235592359986,-26.1907956581852,0.));
#70686=CARTESIAN_POINT('Ctrl Pts',(40.2235592359986,-26.1907956581852,20.));
#70687=CARTESIAN_POINT('Ctrl Pts',(40.2028303709288,-26.217080375414,0.));
#70688=CARTESIAN_POINT('Ctrl Pts',(40.2028303709288,-26.217080375414,20.));
#70689=CARTESIAN_POINT('Ctrl Pts',(40.1820839454613,-26.2433498116008,0.));
#70690=CARTESIAN_POINT('Ctrl Pts',(40.1820839454613,-26.2433498116008,20.));
#70691=CARTESIAN_POINT('Ctrl Pts',(40.161319970285,-26.2696039546074,0.));
#70692=CARTESIAN_POINT('Ctrl Pts',(40.161319970285,-26.2696039546074,20.));
#70693=CARTESIAN_POINT('Ctrl Pts',(40.1405384560971,-26.2958427923028,0.));
#70694=CARTESIAN_POINT('Ctrl Pts',(40.1405384560971,-26.2958427923028,20.));
#70695=CARTESIAN_POINT('Ctrl Pts',(40.1197394136039,-26.3220663125631,0.));
#70696=CARTESIAN_POINT('Ctrl Pts',(40.1197394136039,-26.3220663125631,20.));
#70697=CARTESIAN_POINT('Ctrl Pts',(40.0989228535202,-26.3482745032719,0.));
#70698=CARTESIAN_POINT('Ctrl Pts',(40.0989228535202,-26.3482745032719,20.));
#70699=CARTESIAN_POINT('Ctrl Pts',(40.0780887865696,-26.3744673523197,0.));
#70700=CARTESIAN_POINT('Ctrl Pts',(40.0780887865696,-26.3744673523197,20.));
#70701=CARTESIAN_POINT('Ctrl Pts',(40.0572372234843,-26.4006448476042,0.));
#70702=CARTESIAN_POINT('Ctrl Pts',(40.0572372234843,-26.4006448476042,20.));
#70703=CARTESIAN_POINT('Ctrl Pts',(40.0363681750052,-26.4268069770299,0.));
#70704=CARTESIAN_POINT('Ctrl Pts',(40.0363681750052,-26.4268069770299,20.));
#70705=CARTESIAN_POINT('Ctrl Pts',(40.015481651882,-26.4529537285089,0.));
#70706=CARTESIAN_POINT('Ctrl Pts',(40.015481651882,-26.4529537285089,20.));
#70707=CARTESIAN_POINT('Ctrl Pts',(39.994577664873,-26.4790850899607,0.));
#70708=CARTESIAN_POINT('Ctrl Pts',(39.994577664873,-26.4790850899607,20.));
#70709=CARTESIAN_POINT('Ctrl Pts',(39.9736562247456,-26.5052010493117,0.));
#70710=CARTESIAN_POINT('Ctrl Pts',(39.9736562247456,-26.5052010493117,20.));
#70711=CARTESIAN_POINT('Ctrl Pts',(39.9527173422752,-26.5313015944953,0.));
#70712=CARTESIAN_POINT('Ctrl Pts',(39.9527173422752,-26.5313015944953,20.));
#70713=CARTESIAN_POINT('Ctrl Pts',(39.9317610282459,-26.5573867134521,0.));
#70714=CARTESIAN_POINT('Ctrl Pts',(39.9317610282459,-26.5573867134521,20.));
#70715=CARTESIAN_POINT('Ctrl Pts',(39.9107872934506,-26.5834563941296,0.));
#70716=CARTESIAN_POINT('Ctrl Pts',(39.9107872934506,-26.5834563941296,20.));
#70717=CARTESIAN_POINT('Ctrl Pts',(39.8897961486907,-26.6095106244829,0.));
#70718=CARTESIAN_POINT('Ctrl Pts',(39.8897961486907,-26.6095106244829,20.));
#70719=CARTESIAN_POINT('Ctrl Pts',(39.8687876047769,-26.6355493924744,0.));
#70720=CARTESIAN_POINT('Ctrl Pts',(39.8687876047769,-26.6355493924744,20.));
#70721=CARTESIAN_POINT('Ctrl Pts',(39.847761672528,-26.6615726860735,0.));
#70722=CARTESIAN_POINT('Ctrl Pts',(39.847761672528,-26.6615726860735,20.));
#70723=CARTESIAN_POINT('Ctrl Pts',(39.8267183627717,-26.687580493257,0.));
#70724=CARTESIAN_POINT('Ctrl Pts',(39.8267183627717,-26.687580493257,20.));
#70725=CARTESIAN_POINT('Ctrl Pts',(39.8056576863443,-26.713572802009,0.));
#70726=CARTESIAN_POINT('Ctrl Pts',(39.8056576863443,-26.713572802009,20.));
#70727=CARTESIAN_POINT('Ctrl Pts',(39.7845796540903,-26.7395496003209,0.));
#70728=CARTESIAN_POINT('Ctrl Pts',(39.7845796540903,-26.7395496003209,20.));
#70729=CARTESIAN_POINT('Ctrl Pts',(39.7634842768631,-26.7655108761908,0.));
#70730=CARTESIAN_POINT('Ctrl Pts',(39.7634842768631,-26.7655108761908,20.));
#70731=CARTESIAN_POINT('Ctrl Pts',(39.7423715655248,-26.7914566176244,0.));
#70732=CARTESIAN_POINT('Ctrl Pts',(39.7423715655248,-26.7914566176244,20.));
#70733=CARTESIAN_POINT('Ctrl Pts',(39.7212415309462,-26.8173868126345,0.));
#70734=CARTESIAN_POINT('Ctrl Pts',(39.7212415309462,-26.8173868126345,20.));
#70735=CARTESIAN_POINT('Ctrl Pts',(39.7000941840065,-26.843301449241,0.));
#70736=CARTESIAN_POINT('Ctrl Pts',(39.7000941840065,-26.843301449241,20.));
#70737=CARTESIAN_POINT('Ctrl Pts',(39.6789295355942,-26.8692005154716,0.));
#70738=CARTESIAN_POINT('Ctrl Pts',(39.6789295355942,-26.8692005154716,20.));
#70739=CARTESIAN_POINT('Ctrl Pts',(39.6577475966055,-26.8950839993609,0.));
#70740=CARTESIAN_POINT('Ctrl Pts',(39.6577475966055,-26.8950839993609,20.));
#70741=CARTESIAN_POINT('Ctrl Pts',(39.6365483779457,-26.9209518889509,0.));
#70742=CARTESIAN_POINT('Ctrl Pts',(39.6365483779457,-26.9209518889509,20.));
#70743=CARTESIAN_POINT('Ctrl Pts',(39.6153318905282,-26.9468041722907,0.));
#70744=CARTESIAN_POINT('Ctrl Pts',(39.6153318905282,-26.9468041722907,20.));
#70745=CARTESIAN_POINT('Ctrl Pts',(39.5940981452753,-26.9726408374371,0.));
#70746=CARTESIAN_POINT('Ctrl Pts',(39.5940981452753,-26.9726408374371,20.));
#70747=CARTESIAN_POINT('Ctrl Pts',(39.5728471531177,-26.9984618724537,0.));
#70748=CARTESIAN_POINT('Ctrl Pts',(39.5728471531177,-26.9984618724537,20.));
#70749=CARTESIAN_POINT('Ctrl Pts',(39.5515789249952,-27.0242672654118,0.));
#70750=CARTESIAN_POINT('Ctrl Pts',(39.5515789249952,-27.0242672654118,20.));
#70751=CARTESIAN_POINT('Ctrl Pts',(39.5302934718558,-27.0500570043898,0.));
#70752=CARTESIAN_POINT('Ctrl Pts',(39.5302934718558,-27.0500570043898,20.));
#70753=CARTESIAN_POINT('Ctrl Pts',(39.5089908046561,-27.0758310774732,0.));
#70754=CARTESIAN_POINT('Ctrl Pts',(39.5089908046561,-27.0758310774732,20.));
#70755=CARTESIAN_POINT('Ctrl Pts',(39.4876709343614,-27.1015894727552,0.));
#70756=CARTESIAN_POINT('Ctrl Pts',(39.4876709343614,-27.1015894727552,20.));
#70757=CARTESIAN_POINT('Ctrl Pts',(39.4663338719455,-27.1273321783362,0.));
#70758=CARTESIAN_POINT('Ctrl Pts',(39.4663338719455,-27.1273321783362,20.));
#70759=CARTESIAN_POINT('Ctrl Pts',(39.4449796283908,-27.153059182324,0.));
#70760=CARTESIAN_POINT('Ctrl Pts',(39.4449796283908,-27.153059182324,20.));
#70761=CARTESIAN_POINT('Ctrl Pts',(39.4236082146882,-27.1787704728337,0.));
#70762=CARTESIAN_POINT('Ctrl Pts',(39.4236082146882,-27.1787704728337,20.));
#70763=CARTESIAN_POINT('Ctrl Pts',(39.4022196418372,-27.2044660379877,0.));
#70764=CARTESIAN_POINT('Ctrl Pts',(39.4022196418372,-27.2044660379877,20.));
#70765=CARTESIAN_POINT('Ctrl Pts',(39.3808139208456,-27.2301458659158,0.));
#70766=CARTESIAN_POINT('Ctrl Pts',(39.3808139208456,-27.2301458659158,20.));
#70767=CARTESIAN_POINT('Ctrl Pts',(39.3593910627297,-27.2558099447548,0.));
#70768=CARTESIAN_POINT('Ctrl Pts',(39.3593910627297,-27.2558099447548,20.));
#70769=CARTESIAN_POINT('Ctrl Pts',(39.3379510785145,-27.2814582626493,0.));
#70770=CARTESIAN_POINT('Ctrl Pts',(39.3379510785145,-27.2814582626493,20.));
#70771=CARTESIAN_POINT('Ctrl Pts',(39.3164939792334,-27.3070908077508,0.));
#70772=CARTESIAN_POINT('Ctrl Pts',(39.3164939792334,-27.3070908077508,20.));
#70773=CARTESIAN_POINT('Ctrl Pts',(39.2950197759285,-27.3327075682187,0.));
#70774=CARTESIAN_POINT('Ctrl Pts',(39.2950197759285,-27.3327075682187,20.));
#70775=CARTESIAN_POINT('Ctrl Pts',(39.2735284796508,-27.3583085322198,0.));
#70776=CARTESIAN_POINT('Ctrl Pts',(39.2735284796508,-27.3583085322198,20.));
#70777=CARTESIAN_POINT('Ctrl Pts',(39.25202010146,-27.3838936879286,0.));
#70778=CARTESIAN_POINT('Ctrl Pts',(39.25202010146,-27.3838936879286,20.));
#70779=CARTESIAN_POINT('Ctrl Pts',(39.2304946524241,-27.4094630235266,0.));
#70780=CARTESIAN_POINT('Ctrl Pts',(39.2304946524241,-27.4094630235266,20.));
#70781=CARTESIAN_POINT('Ctrl Pts',(39.2089521436188,-27.4350165272023,0.));
#70782=CARTESIAN_POINT('Ctrl Pts',(39.2089521436188,-27.4350165272023,20.));
#70783=CARTESIAN_POINT('Ctrl Pts',(39.1873925861285,-27.4605541871518,0.));
#70784=CARTESIAN_POINT('Ctrl Pts',(39.1873925861285,-27.4605541871518,20.));
#70785=CARTESIAN_POINT('Ctrl Pts',(39.1658159910457,-27.4860759915783,0.));
#70786=CARTESIAN_POINT('Ctrl Pts',(39.1658159910457,-27.4860759915783,20.));
#70787=CARTESIAN_POINT('Ctrl Pts',(39.1442223694722,-27.5115819286927,0.));
#70788=CARTESIAN_POINT('Ctrl Pts',(39.1442223694722,-27.5115819286927,20.));
#70789=CARTESIAN_POINT('Ctrl Pts',(39.1226117325183,-27.5370719867137,0.));
#70790=CARTESIAN_POINT('Ctrl Pts',(39.1226117325183,-27.5370719867137,20.));
#70791=CARTESIAN_POINT('Ctrl Pts',(39.100984091303,-27.5625461538676,0.));
#70792=CARTESIAN_POINT('Ctrl Pts',(39.100984091303,-27.5625461538676,20.));
#70793=CARTESIAN_POINT('Ctrl Pts',(39.0793394569537,-27.5880044183879,0.));
#70794=CARTESIAN_POINT('Ctrl Pts',(39.0793394569537,-27.5880044183879,20.));
#70795=CARTESIAN_POINT('Ctrl Pts',(39.057677840606,-27.6134467685156,0.));
#70796=CARTESIAN_POINT('Ctrl Pts',(39.057677840606,-27.6134467685156,20.));
#70797=CARTESIAN_POINT('Ctrl Pts',(39.0359992534037,-27.6388731924983,0.));
#70798=CARTESIAN_POINT('Ctrl Pts',(39.0359992534037,-27.6388731924983,20.));
#70799=CARTESIAN_POINT('Ctrl Pts',(39.0143037064988,-27.6642836785915,0.));
#70800=CARTESIAN_POINT('Ctrl Pts',(39.0143037064988,-27.6642836785915,20.));
#70801=CARTESIAN_POINT('Ctrl Pts',(38.9925912110523,-27.6896782150583,0.));
#70802=CARTESIAN_POINT('Ctrl Pts',(38.9925912110523,-27.6896782150583,20.));
#70803=CARTESIAN_POINT('Ctrl Pts',(38.9708617782339,-27.7150567901695,0.));
#70804=CARTESIAN_POINT('Ctrl Pts',(38.9708617782339,-27.7150567901695,20.));
#70805=CARTESIAN_POINT('Ctrl Pts',(38.9491154192216,-27.7404193922036,0.));
#70806=CARTESIAN_POINT('Ctrl Pts',(38.9491154192216,-27.7404193922036,20.));
#70807=CARTESIAN_POINT('Ctrl Pts',(38.9273521452022,-27.7657660094467,0.));
#70808=CARTESIAN_POINT('Ctrl Pts',(38.9273521452022,-27.7657660094467,20.));
#70809=CARTESIAN_POINT('Ctrl Pts',(38.9055719673706,-27.7910966301919,0.));
#70810=CARTESIAN_POINT('Ctrl Pts',(38.9055719673706,-27.7910966301919,20.));
#70811=CARTESIAN_POINT('Ctrl Pts',(38.8837748969299,-27.8164112427396,0.));
#70812=CARTESIAN_POINT('Ctrl Pts',(38.8837748969299,-27.8164112427396,20.));
#70813=CARTESIAN_POINT('Ctrl Pts',(38.8619609450912,-27.8417098353976,0.));
#70814=CARTESIAN_POINT('Ctrl Pts',(38.8619609450912,-27.8417098353976,20.));
#70815=CARTESIAN_POINT('Ctrl Pts',(38.8401301230745,-27.866992396481,0.));
#70816=CARTESIAN_POINT('Ctrl Pts',(38.8401301230745,-27.866992396481,20.));
#70817=CARTESIAN_POINT('Ctrl Pts',(38.8182824421081,-27.8922589143132,0.));
#70818=CARTESIAN_POINT('Ctrl Pts',(38.8182824421081,-27.8922589143132,20.));
#70819=CARTESIAN_POINT('Ctrl Pts',(38.7964179134294,-27.917509377225,0.));
#70820=CARTESIAN_POINT('Ctrl Pts',(38.7964179134294,-27.917509377225,20.));
#70821=CARTESIAN_POINT('Ctrl Pts',(38.7745365482837,-27.9427437735547,0.));
#70822=CARTESIAN_POINT('Ctrl Pts',(38.7745365482837,-27.9427437735547,20.));
#70823=CARTESIAN_POINT('Ctrl Pts',(38.752638357925,-27.9679620916479,0.));
#70824=CARTESIAN_POINT('Ctrl Pts',(38.752638357925,-27.9679620916479,20.));
#70825=CARTESIAN_POINT('Ctrl Pts',(38.7307233536152,-27.9931643198581,0.));
#70826=CARTESIAN_POINT('Ctrl Pts',(38.7307233536152,-27.9931643198581,20.));
#70827=CARTESIAN_POINT('Ctrl Pts',(38.7087915466246,-28.0183504465459,0.));
#70828=CARTESIAN_POINT('Ctrl Pts',(38.7087915466246,-28.0183504465459,20.));
#70829=CARTESIAN_POINT('Ctrl Pts',(38.6868429482324,-28.0435204600798,0.));
#70830=CARTESIAN_POINT('Ctrl Pts',(38.6868429482324,-28.0435204600798,20.));
#70831=CARTESIAN_POINT('Ctrl Pts',(38.6648775697261,-28.0686743488362,0.));
#70832=CARTESIAN_POINT('Ctrl Pts',(38.6648775697261,-28.0686743488362,20.));
#70833=CARTESIAN_POINT('Ctrl Pts',(38.6428954224012,-28.0938121011982,0.));
#70834=CARTESIAN_POINT('Ctrl Pts',(38.6428954224012,-28.0938121011982,20.));
#70835=CARTESIAN_POINT('Ctrl Pts',(38.6208965175619,-28.1189337055566,0.));
#70836=CARTESIAN_POINT('Ctrl Pts',(38.6208965175619,-28.1189337055566,20.));
#70837=CARTESIAN_POINT('Ctrl Pts',(38.5988808665205,-28.14403915031,0.));
#70838=CARTESIAN_POINT('Ctrl Pts',(38.5988808665205,-28.14403915031,20.));
#70839=CARTESIAN_POINT('Ctrl Pts',(38.5768484805978,-28.1691284238645,0.));
#70840=CARTESIAN_POINT('Ctrl Pts',(38.5768484805978,-28.1691284238645,20.));
#70841=CARTESIAN_POINT('Ctrl Pts',(38.5547993711231,-28.1942015146341,0.));
#70842=CARTESIAN_POINT('Ctrl Pts',(38.5547993711231,-28.1942015146341,20.));
#70843=CARTESIAN_POINT('Ctrl Pts',(38.5327335494334,-28.2192584110398,0.));
#70844=CARTESIAN_POINT('Ctrl Pts',(38.5327335494334,-28.2192584110398,20.));
#70845=CARTESIAN_POINT('Ctrl Pts',(38.5106510268752,-28.2442991015113,0.));
#70846=CARTESIAN_POINT('Ctrl Pts',(38.5106510268752,-28.2442991015113,20.));
#70847=CARTESIAN_POINT('Ctrl Pts',(38.4885518148031,-28.2693235744854,0.));
#70848=CARTESIAN_POINT('Ctrl Pts',(38.4885518148031,-28.2693235744854,20.));
#70849=CARTESIAN_POINT('Ctrl Pts',(38.4664359245797,-28.2943318184066,0.));
#70850=CARTESIAN_POINT('Ctrl Pts',(38.4664359245797,-28.2943318184066,20.));
#70851=CARTESIAN_POINT('Ctrl Pts',(38.4443033675759,-28.3193238217266,0.));
#70852=CARTESIAN_POINT('Ctrl Pts',(38.4443033675759,-28.3193238217266,20.));
#70853=CARTESIAN_POINT('Ctrl Pts',(38.4221541551709,-28.344299572905,0.));
#70854=CARTESIAN_POINT('Ctrl Pts',(38.4221541551709,-28.344299572905,20.));
#70855=CARTESIAN_POINT('Ctrl Pts',(38.3999882987522,-28.3692590604082,0.));
#70856=CARTESIAN_POINT('Ctrl Pts',(38.3999882987522,-28.3692590604082,20.));
#70857=CARTESIAN_POINT('Ctrl Pts',(38.3778058097152,-28.3942022727108,0.));
#70858=CARTESIAN_POINT('Ctrl Pts',(38.3778058097152,-28.3942022727108,20.));
#70859=CARTESIAN_POINT('Ctrl Pts',(38.3556066994642,-28.4191291982951,0.));
#70860=CARTESIAN_POINT('Ctrl Pts',(38.3556066994642,-28.4191291982951,20.));
#70861=CARTESIAN_POINT('Ctrl Pts',(38.3333909794119,-28.4440398256512,0.));
#70862=CARTESIAN_POINT('Ctrl Pts',(38.3333909794119,-28.4440398256512,20.));
#70863=CARTESIAN_POINT('Ctrl Pts',(38.3111586609794,-28.4689341432774,0.));
#70864=CARTESIAN_POINT('Ctrl Pts',(38.3111586609794,-28.4689341432774,20.));
#70865=CARTESIAN_POINT('Ctrl Pts',(38.2889097555964,-28.4938121396793,0.));
#70866=CARTESIAN_POINT('Ctrl Pts',(38.2889097555964,-28.4938121396793,20.));
#70867=CARTESIAN_POINT('Ctrl Pts',(38.2666442747002,-28.5186738033704,0.));
#70868=CARTESIAN_POINT('Ctrl Pts',(38.2666442747002,-28.5186738033704,20.));
#70869=CARTESIAN_POINT('Ctrl Pts',(38.2443622297368,-28.5435191228711,0.));
#70870=CARTESIAN_POINT('Ctrl Pts',(38.2443622297368,-28.5435191228711,20.));
#70871=CARTESIAN_POINT('Ctrl Pts',(38.2220636321601,-28.5683480867098,0.));
#70872=CARTESIAN_POINT('Ctrl Pts',(38.2220636321601,-28.5683480867098,20.));
#70873=CARTESIAN_POINT('Ctrl Pts',(38.1997484934321,-28.5931606834224,0.));
#70874=CARTESIAN_POINT('Ctrl Pts',(38.1997484934321,-28.5931606834224,20.));
#70875=CARTESIAN_POINT('Ctrl Pts',(38.1774168250235,-28.6179569015525,0.));
#70876=CARTESIAN_POINT('Ctrl Pts',(38.1774168250235,-28.6179569015525,20.));
#70877=CARTESIAN_POINT('Ctrl Pts',(38.1550686384134,-28.6427367296518,0.));
#70878=CARTESIAN_POINT('Ctrl Pts',(38.1550686384134,-28.6427367296518,20.));
#70879=CARTESIAN_POINT('Ctrl Pts',(38.1327039450889,-28.6675001562794,0.));
#70880=CARTESIAN_POINT('Ctrl Pts',(38.1327039450889,-28.6675001562794,20.));
#70881=CARTESIAN_POINT('Ctrl Pts',(38.1103227565456,-28.6922471700024,0.));
#70882=CARTESIAN_POINT('Ctrl Pts',(38.1103227565456,-28.6922471700024,20.));
#70883=CARTESIAN_POINT('Ctrl Pts',(38.0879250842874,-28.7169777593956,0.));
#70884=CARTESIAN_POINT('Ctrl Pts',(38.0879250842874,-28.7169777593956,20.));
#70885=CARTESIAN_POINT('Ctrl Pts',(38.0655109398262,-28.7416919130413,0.));
#70886=CARTESIAN_POINT('Ctrl Pts',(38.0655109398262,-28.7416919130413,20.));
#70887=CARTESIAN_POINT('Ctrl Pts',(38.0430803346823,-28.76638961953,0.));
#70888=CARTESIAN_POINT('Ctrl Pts',(38.0430803346823,-28.76638961953,20.));
#70889=CARTESIAN_POINT('Ctrl Pts',(38.020633280384,-28.7910708674595,0.));
#70890=CARTESIAN_POINT('Ctrl Pts',(38.020633280384,-28.7910708674595,20.));
#70891=CARTESIAN_POINT('Ctrl Pts',(37.9981697884679,-28.8157356454354,0.));
#70892=CARTESIAN_POINT('Ctrl Pts',(37.9981697884679,-28.8157356454354,20.));
#70893=CARTESIAN_POINT('Ctrl Pts',(37.975689870479,-28.8403839420709,0.));
#70894=CARTESIAN_POINT('Ctrl Pts',(37.975689870479,-28.8403839420709,20.));
#70895=CARTESIAN_POINT('Ctrl Pts',(37.9531935379708,-28.8650157459872,0.));
#70896=CARTESIAN_POINT('Ctrl Pts',(37.9531935379708,-28.8650157459872,20.));
#70897=CARTESIAN_POINT('Ctrl Pts',(37.9306808025048,-28.8896310458131,0.));
#70898=CARTESIAN_POINT('Ctrl Pts',(37.9306808025048,-28.8896310458131,20.));
#70899=CARTESIAN_POINT('Ctrl Pts',(37.9081516756509,-28.9142298301853,0.));
#70900=CARTESIAN_POINT('Ctrl Pts',(37.9081516756509,-28.9142298301853,20.));
#70901=CARTESIAN_POINT('Ctrl Pts',(37.8856061689868,-28.9388120877484,0.));
#70902=CARTESIAN_POINT('Ctrl Pts',(37.8856061689868,-28.9388120877484,20.));
#70903=CARTESIAN_POINT('Ctrl Pts',(37.8630442940985,-28.9633778071544,0.));
#70904=CARTESIAN_POINT('Ctrl Pts',(37.8630442940985,-28.9633778071544,20.));
#70905=CARTESIAN_POINT('Ctrl Pts',(37.8404660625803,-28.9879269770638,0.));
#70906=CARTESIAN_POINT('Ctrl Pts',(37.8404660625803,-28.9879269770638,20.));
#70907=CARTESIAN_POINT('Ctrl Pts',(37.8178714860345,-29.0124595861442,0.));
#70908=CARTESIAN_POINT('Ctrl Pts',(37.8178714860345,-29.0124595861442,20.));
#70909=CARTESIAN_POINT('Ctrl Pts',(37.7952605760716,-29.0369756230713,0.));
#70910=CARTESIAN_POINT('Ctrl Pts',(37.7952605760716,-29.0369756230713,20.));
#70911=CARTESIAN_POINT('Ctrl Pts',(37.7726333443105,-29.0614750765285,0.));
#70912=CARTESIAN_POINT('Ctrl Pts',(37.7726333443105,-29.0614750765285,20.));
#70913=CARTESIAN_POINT('Ctrl Pts',(37.7499898023784,-29.0859579352069,0.));
#70914=CARTESIAN_POINT('Ctrl Pts',(37.7499898023784,-29.0859579352069,20.));
#70915=CARTESIAN_POINT('Ctrl Pts',(37.7273299619109,-29.1104241878056,0.));
#70916=CARTESIAN_POINT('Ctrl Pts',(37.7273299619109,-29.1104241878056,20.));
#70917=CARTESIAN_POINT('Ctrl Pts',(37.7046538345516,-29.1348738230316,0.));
#70918=CARTESIAN_POINT('Ctrl Pts',(37.7046538345516,-29.1348738230316,20.));
#70919=CARTESIAN_POINT('Ctrl Pts',(37.6819614319522,-29.1593068295998,0.));
#70920=CARTESIAN_POINT('Ctrl Pts',(37.6819614319522,-29.1593068295998,20.));
#70921=CARTESIAN_POINT('Ctrl Pts',(37.6592527657727,-29.1837231962329,0.));
#70922=CARTESIAN_POINT('Ctrl Pts',(37.6592527657727,-29.1837231962329,20.));
#70923=CARTESIAN_POINT('Ctrl Pts',(37.6365278476807,-29.208122911661,0.));
#70924=CARTESIAN_POINT('Ctrl Pts',(37.6365278476807,-29.208122911661,20.));
#70925=CARTESIAN_POINT('Ctrl Pts',(37.6137866893519,-29.2325059646225,0.));
#70926=CARTESIAN_POINT('Ctrl Pts',(37.6137866893519,-29.2325059646225,20.));
#70927=CARTESIAN_POINT('Ctrl Pts',(37.5910293024705,-29.2568723438632,0.));
#70928=CARTESIAN_POINT('Ctrl Pts',(37.5910293024705,-29.2568723438632,20.));
#70929=CARTESIAN_POINT('Ctrl Pts',(37.5682556987287,-29.2812220381373,0.));
#70930=CARTESIAN_POINT('Ctrl Pts',(37.5682556987287,-29.2812220381373,20.));
#70931=CARTESIAN_POINT('Ctrl Pts',(37.5454658898273,-29.3055550362068,0.));
#70932=CARTESIAN_POINT('Ctrl Pts',(37.5454658898273,-29.3055550362068,20.));
#70933=CARTESIAN_POINT('Ctrl Pts',(37.5226598874754,-29.3298713268414,0.));
#70934=CARTESIAN_POINT('Ctrl Pts',(37.5226598874754,-29.3298713268414,20.));
#70935=CARTESIAN_POINT('Ctrl Pts',(37.4998377033899,-29.3541708988191,0.));
#70936=CARTESIAN_POINT('Ctrl Pts',(37.4998377033899,-29.3541708988191,20.));
#70937=CARTESIAN_POINT('Ctrl Pts',(37.4769993492958,-29.3784537409251,0.));
#70938=CARTESIAN_POINT('Ctrl Pts',(37.4769993492958,-29.3784537409251,20.));
#70939=CARTESIAN_POINT('Ctrl Pts',(37.4541448369259,-29.4027198419524,0.));
#70940=CARTESIAN_POINT('Ctrl Pts',(37.4541448369259,-29.4027198419524,20.));
#70941=CARTESIAN_POINT('Ctrl Pts',(37.4312741780212,-29.4269691907023,0.));
#70942=CARTESIAN_POINT('Ctrl Pts',(37.4312741780212,-29.4269691907023,20.));
#70943=CARTESIAN_POINT('Ctrl Pts',(37.4083873843312,-29.4512017759842,0.));
#70944=CARTESIAN_POINT('Ctrl Pts',(37.4083873843312,-29.4512017759842,20.));
#70945=CARTESIAN_POINT('Ctrl Pts',(37.3854844676135,-29.4754175866156,0.));
#70946=CARTESIAN_POINT('Ctrl Pts',(37.3854844676135,-29.4754175866156,20.));
#70947=CARTESIAN_POINT('Ctrl Pts',(37.3625654396334,-29.4996166114217,0.));
#70948=CARTESIAN_POINT('Ctrl Pts',(37.3625654396334,-29.4996166114217,20.));
#70949=CARTESIAN_POINT('Ctrl Pts',(37.3396303121646,-29.5237988392353,0.));
#70950=CARTESIAN_POINT('Ctrl Pts',(37.3396303121646,-29.5237988392353,20.));
#70951=CARTESIAN_POINT('Ctrl Pts',(37.3166790969884,-29.5479642588972,0.));
#70952=CARTESIAN_POINT('Ctrl Pts',(37.3166790969884,-29.5479642588972,20.));
#70953=CARTESIAN_POINT('Ctrl Pts',(37.2937118058947,-29.5721128592559,0.));
#70954=CARTESIAN_POINT('Ctrl Pts',(37.2937118058947,-29.5721128592559,20.));
#70955=CARTESIAN_POINT('Ctrl Pts',(37.2707284506814,-29.5962446291683,0.));
#70956=CARTESIAN_POINT('Ctrl Pts',(37.2707284506814,-29.5962446291683,20.));
#70957=CARTESIAN_POINT('Ctrl Pts',(37.2477290431548,-29.6203595574991,0.));
#70958=CARTESIAN_POINT('Ctrl Pts',(37.2477290431548,-29.6203595574991,20.));
#70959=CARTESIAN_POINT('Ctrl Pts',(37.2247135951292,-29.6444576331215,0.));
#70960=CARTESIAN_POINT('Ctrl Pts',(37.2247135951292,-29.6444576331215,20.));
#70961=CARTESIAN_POINT('Ctrl Pts',(37.2016821184267,-29.668538844916,0.));
#70962=CARTESIAN_POINT('Ctrl Pts',(37.2016821184267,-29.668538844916,20.));
#70963=CARTESIAN_POINT('Ctrl Pts',(37.1786346248774,-29.6926031817715,0.));
#70964=CARTESIAN_POINT('Ctrl Pts',(37.1786346248774,-29.6926031817715,20.));
#70965=CARTESIAN_POINT('Ctrl Pts',(37.155571126319,-29.7166506325841,0.));
#70966=CARTESIAN_POINT('Ctrl Pts',(37.155571126319,-29.7166506325841,20.));
#70967=CARTESIAN_POINT('Ctrl Pts',(37.1324916345976,-29.7406811862582,0.));
#70968=CARTESIAN_POINT('Ctrl Pts',(37.1324916345976,-29.7406811862582,20.));
#70969=CARTESIAN_POINT('Ctrl Pts',(37.1093961615672,-29.7646948317062,0.));
#70970=CARTESIAN_POINT('Ctrl Pts',(37.1093961615672,-29.7646948317062,20.));
#70971=CARTESIAN_POINT('Ctrl Pts',(37.0862847190902,-29.7886915578486,0.));
#70972=CARTESIAN_POINT('Ctrl Pts',(37.0862847190902,-29.7886915578486,20.));
#70973=CARTESIAN_POINT('Ctrl Pts',(37.0631573190373,-29.8126713536142,0.));
#70974=CARTESIAN_POINT('Ctrl Pts',(37.0631573190373,-29.8126713536142,20.));
#70975=CARTESIAN_POINT('Ctrl Pts',(37.0400139732874,-29.8366342079401,0.));
#70976=CARTESIAN_POINT('Ctrl Pts',(37.0400139732874,-29.8366342079401,20.));
#70977=CARTESIAN_POINT('Ctrl Pts',(37.0168546937273,-29.8605801097708,0.));
#70978=CARTESIAN_POINT('Ctrl Pts',(37.0168546937273,-29.8605801097708,20.));
#70979=CARTESIAN_POINT('Ctrl Pts',(36.9936794922513,-29.884509048059,0.));
#70980=CARTESIAN_POINT('Ctrl Pts',(36.9936794922513,-29.884509048059,20.));
#70981=CARTESIAN_POINT('Ctrl Pts',(36.9704883807614,-29.9084210117647,0.));
#70982=CARTESIAN_POINT('Ctrl Pts',(36.9704883807614,-29.9084210117647,20.));
#70983=CARTESIAN_POINT('Ctrl Pts',(36.9472813711676,-29.9323159898562,0.));
#70984=CARTESIAN_POINT('Ctrl Pts',(36.9472813711676,-29.9323159898562,20.));
#70985=CARTESIAN_POINT('Ctrl Pts',(36.9240584753882,-29.9561939713103,0.));
#70986=CARTESIAN_POINT('Ctrl Pts',(36.9240584753882,-29.9561939713103,20.));
#70987=CARTESIAN_POINT('Ctrl Pts',(36.9008197053507,-29.9800549451122,0.));
#70988=CARTESIAN_POINT('Ctrl Pts',(36.9008197053507,-29.9800549451122,20.));
#70989=CARTESIAN_POINT('Ctrl Pts',(36.8775650729895,-30.003898900255,0.));
#70990=CARTESIAN_POINT('Ctrl Pts',(36.8775650729895,-30.003898900255,20.));
#70991=CARTESIAN_POINT('Ctrl Pts',(36.8542945902472,-30.0277258257394,0.));
#70992=CARTESIAN_POINT('Ctrl Pts',(36.8542945902472,-30.0277258257394,20.));
#70993=CARTESIAN_POINT('Ctrl Pts',(36.8310082690741,-30.051535710574,0.));
#70994=CARTESIAN_POINT('Ctrl Pts',(36.8310082690741,-30.051535710574,20.));
#70995=CARTESIAN_POINT('Ctrl Pts',(36.8077061214283,-30.0753285437754,0.));
#70996=CARTESIAN_POINT('Ctrl Pts',(36.8077061214283,-30.0753285437754,20.));
#70997=CARTESIAN_POINT('Ctrl Pts',(36.7843881592759,-30.0991043143685,0.));
#70998=CARTESIAN_POINT('Ctrl Pts',(36.7843881592759,-30.0991043143685,20.));
#70999=CARTESIAN_POINT('Ctrl Pts',(36.7610543945915,-30.1228630113862,0.));
#71000=CARTESIAN_POINT('Ctrl Pts',(36.7610543945915,-30.1228630113862,20.));
#71001=CARTESIAN_POINT('Ctrl Pts',(36.7377048393574,-30.1466046238701,0.));
#71002=CARTESIAN_POINT('Ctrl Pts',(36.7377048393574,-30.1466046238701,20.));
#71003=CARTESIAN_POINT('Ctrl Pts',(36.7143395055641,-30.1703291408693,0.));
#71004=CARTESIAN_POINT('Ctrl Pts',(36.7143395055641,-30.1703291408693,20.));
#71005=CARTESIAN_POINT('Ctrl Pts',(36.6909584052099,-30.1940365514414,0.));
#71006=CARTESIAN_POINT('Ctrl Pts',(36.6909584052099,-30.1940365514414,20.));
#71007=CARTESIAN_POINT('Ctrl Pts',(36.6675615503012,-30.2177268446518,0.));
#71008=CARTESIAN_POINT('Ctrl Pts',(36.6675615503012,-30.2177268446518,20.));
#71009=CARTESIAN_POINT('Ctrl Pts',(36.6441489528521,-30.2414000095742,0.));
#71010=CARTESIAN_POINT('Ctrl Pts',(36.6441489528521,-30.2414000095742,20.));
#71011=CARTESIAN_POINT('Ctrl Pts',(36.6207206248848,-30.2650560352902,0.));
#71012=CARTESIAN_POINT('Ctrl Pts',(36.6207206248848,-30.2650560352902,20.));
#71013=CARTESIAN_POINT('Ctrl Pts',(36.5972765784293,-30.2886949108895,0.));
#71014=CARTESIAN_POINT('Ctrl Pts',(36.5972765784293,-30.2886949108895,20.));
#71015=CARTESIAN_POINT('Ctrl Pts',(36.5738168255233,-30.3123166254701,0.));
#71016=CARTESIAN_POINT('Ctrl Pts',(36.5738168255233,-30.3123166254701,20.));
#71017=CARTESIAN_POINT('Ctrl Pts',(36.5503413782123,-30.3359211681376,0.));
#71018=CARTESIAN_POINT('Ctrl Pts',(36.5503413782123,-30.3359211681376,20.));
#71019=CARTESIAN_POINT('Ctrl Pts',(36.5268502485502,-30.3595085280059,0.));
#71020=CARTESIAN_POINT('Ctrl Pts',(36.5268502485502,-30.3595085280059,20.));
#71021=CARTESIAN_POINT('Ctrl Pts',(36.5033434485984,-30.3830786941972,0.));
#71022=CARTESIAN_POINT('Ctrl Pts',(36.5033434485984,-30.3830786941972,20.));
#71023=CARTESIAN_POINT('Ctrl Pts',(36.4798209904267,-30.4066316558424,0.));
#71024=CARTESIAN_POINT('Ctrl Pts',(36.4798209904267,-30.4066316558424,20.));
#71025=CARTESIAN_POINT('Ctrl Pts',(36.456282886113,-30.4301674020802,0.));
#71026=CARTESIAN_POINT('Ctrl Pts',(36.456282886113,-30.4301674020802,20.));
#71027=CARTESIAN_POINT('Ctrl Pts',(36.4327291477428,-30.4536859220576,0.));
#71028=CARTESIAN_POINT('Ctrl Pts',(36.4327291477428,-30.4536859220576,20.));
#71029=CARTESIAN_POINT('Ctrl Pts',(36.4091597874097,-30.4771872049299,0.));
#71030=CARTESIAN_POINT('Ctrl Pts',(36.4091597874097,-30.4771872049299,20.));
#71031=CARTESIAN_POINT('Ctrl Pts',(36.3855748172148,-30.5006712398601,0.));
#71032=CARTESIAN_POINT('Ctrl Pts',(36.3855748172148,-30.5006712398601,20.));
#71033=CARTESIAN_POINT('Ctrl Pts',(36.3619742492671,-30.5241380160195,0.));
#71034=CARTESIAN_POINT('Ctrl Pts',(36.3619742492671,-30.5241380160195,20.));
#71035=CARTESIAN_POINT('Ctrl Pts',(36.3383580956832,-30.5475875225872,0.));
#71036=CARTESIAN_POINT('Ctrl Pts',(36.3383580956832,-30.5475875225872,20.));
#71037=CARTESIAN_POINT('Ctrl Pts',(36.3147263685874,-30.5710197487502,0.));
#71038=CARTESIAN_POINT('Ctrl Pts',(36.3147263685874,-30.5710197487502,20.));
#71039=CARTESIAN_POINT('Ctrl Pts',(36.2910790801119,-30.5944346837039,0.));
#71040=CARTESIAN_POINT('Ctrl Pts',(36.2910790801119,-30.5944346837039,20.));
#71041=CARTESIAN_POINT('Ctrl Pts',(36.2674162423973,-30.6178323166527,0.));
#71042=CARTESIAN_POINT('Ctrl Pts',(36.2674162423973,-30.6178323166527,20.));
#71043=CARTESIAN_POINT('Ctrl Pts',(36.2437378675924,-30.6412126368095,0.));
#71044=CARTESIAN_POINT('Ctrl Pts',(36.2437378675924,-30.6412126368095,20.));
#71045=CARTESIAN_POINT('Ctrl Pts',(36.2200439678542,-30.6645756333955,0.));
#71046=CARTESIAN_POINT('Ctrl Pts',(36.2200439678542,-30.6645756333955,20.));
#71047=CARTESIAN_POINT('Ctrl Pts',(36.196334555347,-30.6879212956392,0.));
#71048=CARTESIAN_POINT('Ctrl Pts',(36.196334555347,-30.6879212956392,20.));
#71049=CARTESIAN_POINT('Ctrl Pts',(36.1726096422428,-30.7112496127774,0.));
#71050=CARTESIAN_POINT('Ctrl Pts',(36.1726096422428,-30.7112496127774,20.));
#71051=CARTESIAN_POINT('Ctrl Pts',(36.1488692407204,-30.7345605740545,0.));
#71052=CARTESIAN_POINT('Ctrl Pts',(36.1488692407204,-30.7345605740545,20.));
#71053=CARTESIAN_POINT('Ctrl Pts',(36.1251133629669,-30.7578541687236,0.));
#71054=CARTESIAN_POINT('Ctrl Pts',(36.1251133629669,-30.7578541687236,20.));
#71055=CARTESIAN_POINT('Ctrl Pts',(36.1013420211777,-30.7811303860468,0.));
#71056=CARTESIAN_POINT('Ctrl Pts',(36.1013420211777,-30.7811303860468,20.));
#71057=CARTESIAN_POINT('Ctrl Pts',(36.0775552275565,-30.8043892152943,0.));
#71058=CARTESIAN_POINT('Ctrl Pts',(36.0775552275565,-30.8043892152943,20.));
#71059=CARTESIAN_POINT('Ctrl Pts',(36.0537529943146,-30.8276306457446,0.));
#71060=CARTESIAN_POINT('Ctrl Pts',(36.0537529943146,-30.8276306457446,20.));
#71061=CARTESIAN_POINT('Ctrl Pts',(36.0299353336712,-30.8508546666841,0.));
#71062=CARTESIAN_POINT('Ctrl Pts',(36.0299353336712,-30.8508546666841,20.));
#71063=CARTESIAN_POINT('Ctrl Pts',(36.0061022578528,-30.8740612674075,0.));
#71064=CARTESIAN_POINT('Ctrl Pts',(36.0061022578528,-30.8740612674075,20.));
#71065=CARTESIAN_POINT('Ctrl Pts',(35.9822537790931,-30.8972504372171,0.));
#71066=CARTESIAN_POINT('Ctrl Pts',(35.9822537790931,-30.8972504372171,20.));
#71067=CARTESIAN_POINT('Ctrl Pts',(35.9583899096339,-30.9204221654236,0.));
#71068=CARTESIAN_POINT('Ctrl Pts',(35.9583899096339,-30.9204221654236,20.));
#71069=CARTESIAN_POINT('Ctrl Pts',(35.9345106617251,-30.9435764413467,0.));
#71070=CARTESIAN_POINT('Ctrl Pts',(35.9345106617251,-30.9435764413467,20.));
#71071=CARTESIAN_POINT('Ctrl Pts',(35.9106160476245,-30.9667132543142,0.));
#71072=CARTESIAN_POINT('Ctrl Pts',(35.9106160476245,-30.9667132543142,20.));
#71073=CARTESIAN_POINT('Ctrl Pts',(35.886706079598,-30.9898325936627,0.));
#71074=CARTESIAN_POINT('Ctrl Pts',(35.886706079598,-30.9898325936627,20.));
#71075=CARTESIAN_POINT('Ctrl Pts',(35.8627807699193,-31.0129344487367,0.));
#71076=CARTESIAN_POINT('Ctrl Pts',(35.8627807699193,-31.0129344487367,20.));
#71077=CARTESIAN_POINT('Ctrl Pts',(35.8388401308696,-31.036018808889,0.));
#71078=CARTESIAN_POINT('Ctrl Pts',(35.8388401308696,-31.036018808889,20.));
#71079=CARTESIAN_POINT('Ctrl Pts',(35.8148841747376,-31.0590856634804,0.));
#71080=CARTESIAN_POINT('Ctrl Pts',(35.8148841747376,-31.0590856634804,20.));
#71081=CARTESIAN_POINT('Ctrl Pts',(35.7909129138202,-31.082135001881,0.));
#71082=CARTESIAN_POINT('Ctrl Pts',(35.7909129138202,-31.082135001881,20.));
#71083=CARTESIAN_POINT('Ctrl Pts',(35.7669263604212,-31.1051668134678,0.));
#71084=CARTESIAN_POINT('Ctrl Pts',(35.7669263604212,-31.1051668134678,20.));
#71085=CARTESIAN_POINT('Ctrl Pts',(35.7429245268523,-31.1281810876267,0.));
#71086=CARTESIAN_POINT('Ctrl Pts',(35.7429245268523,-31.1281810876267,20.));
#71087=CARTESIAN_POINT('Ctrl Pts',(35.7189074254331,-31.1511778137516,0.));
#71088=CARTESIAN_POINT('Ctrl Pts',(35.7189074254331,-31.1511778137516,20.));
#71089=CARTESIAN_POINT('Ctrl Pts',(35.6948750684911,-31.1741569812451,0.));
#71090=CARTESIAN_POINT('Ctrl Pts',(35.6948750684911,-31.1741569812451,20.));
#71091=CARTESIAN_POINT('Ctrl Pts',(35.6708274683619,-31.1971185795181,0.));
#71092=CARTESIAN_POINT('Ctrl Pts',(35.6708274683619,-31.1971185795181,20.));
#71093=CARTESIAN_POINT('Ctrl Pts',(35.6467646373883,-31.2200625979904,0.));
#71094=CARTESIAN_POINT('Ctrl Pts',(35.6467646373883,-31.2200625979904,20.));
#71095=CARTESIAN_POINT('Ctrl Pts',(35.6226865879214,-31.24298902609,0.));
#71096=CARTESIAN_POINT('Ctrl Pts',(35.6226865879214,-31.24298902609,20.));
#71097=CARTESIAN_POINT('Ctrl Pts',(35.5985933323194,-31.2658978532533,0.));
#71098=CARTESIAN_POINT('Ctrl Pts',(35.5985933323194,-31.2658978532533,20.));
#71099=CARTESIAN_POINT('Ctrl Pts',(35.5744848829487,-31.288789068925,0.));
#71100=CARTESIAN_POINT('Ctrl Pts',(35.5744848829487,-31.288789068925,20.));
#71101=CARTESIAN_POINT('Ctrl Pts',(35.5503612521832,-31.3116626625581,0.));
#71102=CARTESIAN_POINT('Ctrl Pts',(35.5503612521832,-31.3116626625581,20.));
#71103=CARTESIAN_POINT('Ctrl Pts',(35.5262224524039,-31.3345186236135,0.));
#71104=CARTESIAN_POINT('Ctrl Pts',(35.5262224524039,-31.3345186236135,20.));
#71105=CARTESIAN_POINT('Ctrl Pts',(35.502068496,-31.3573569415606,0.));
#71106=CARTESIAN_POINT('Ctrl Pts',(35.502068496,-31.3573569415606,20.));
#71107=CARTESIAN_POINT('Ctrl Pts',(35.4778993953681,-31.3801776058768,0.));
#71108=CARTESIAN_POINT('Ctrl Pts',(35.4778993953681,-31.3801776058768,20.));
#71109=CARTESIAN_POINT('Ctrl Pts',(35.4537151629126,-31.4029806060482,0.));
#71110=CARTESIAN_POINT('Ctrl Pts',(35.4537151629126,-31.4029806060482,20.));
#71111=CARTESIAN_POINT('Ctrl Pts',(35.4295158110454,-31.4257659315696,0.));
#71112=CARTESIAN_POINT('Ctrl Pts',(35.4295158110454,-31.4257659315696,20.));
#71113=CARTESIAN_POINT('Ctrl Pts',(35.4053013521866,-31.4485335719447,0.));
#71114=CARTESIAN_POINT('Ctrl Pts',(35.4053013521866,-31.4485335719447,20.));
#71115=CARTESIAN_POINT('Ctrl Pts',(35.3810717987641,-31.4712835166857,0.));
#71116=CARTESIAN_POINT('Ctrl Pts',(35.3810717987641,-31.4712835166857,20.));
#71117=CARTESIAN_POINT('Ctrl Pts',(35.3568271632136,-31.4940157553136,0.));
#71118=CARTESIAN_POINT('Ctrl Pts',(35.3568271632136,-31.4940157553136,20.));
#71119=CARTESIAN_POINT('Ctrl Pts',(35.3325674579779,-31.516730277357,0.));
#71120=CARTESIAN_POINT('Ctrl Pts',(35.3325674579779,-31.516730277357,20.));
#71121=CARTESIAN_POINT('Ctrl Pts',(35.3082926955072,-31.5394270723526,0.));
#71122=CARTESIAN_POINT('Ctrl Pts',(35.3082926955072,-31.5394270723526,20.));
#71123=CARTESIAN_POINT('Ctrl Pts',(35.2840028882593,-31.5621061298453,0.));
#71124=CARTESIAN_POINT('Ctrl Pts',(35.2840028882593,-31.5621061298453,20.));
#71125=CARTESIAN_POINT('Ctrl Pts',(35.2596980486996,-31.5847674393885,0.));
#71126=CARTESIAN_POINT('Ctrl Pts',(35.2596980486996,-31.5847674393885,20.));
#71127=CARTESIAN_POINT('Ctrl Pts',(35.2353781893014,-31.6074109905439,0.));
#71128=CARTESIAN_POINT('Ctrl Pts',(35.2353781893014,-31.6074109905439,20.));
#71129=CARTESIAN_POINT('Ctrl Pts',(35.2110433225458,-31.6300367728827,0.));
#71130=CARTESIAN_POINT('Ctrl Pts',(35.2110433225458,-31.6300367728827,20.));
#71131=CARTESIAN_POINT('Ctrl Pts',(35.1866934609214,-31.652644775984,0.));
#71132=CARTESIAN_POINT('Ctrl Pts',(35.1866934609214,-31.652644775984,20.));
#71133=CARTESIAN_POINT('Ctrl Pts',(35.1623286169245,-31.6752349894358,0.));
#71134=CARTESIAN_POINT('Ctrl Pts',(35.1623286169245,-31.6752349894358,20.));
#71135=CARTESIAN_POINT('Ctrl Pts',(35.1379488030591,-31.6978074028349,0.));
#71136=CARTESIAN_POINT('Ctrl Pts',(35.1379488030591,-31.6978074028349,20.));
#71137=CARTESIAN_POINT('Ctrl Pts',(35.1135540318367,-31.7203620057864,0.));
#71138=CARTESIAN_POINT('Ctrl Pts',(35.1135540318367,-31.7203620057864,20.));
#71139=CARTESIAN_POINT('Ctrl Pts',(35.0891443157764,-31.7428987879035,0.));
#71140=CARTESIAN_POINT('Ctrl Pts',(35.0891443157764,-31.7428987879035,20.));
#71141=CARTESIAN_POINT('Ctrl Pts',(35.0647196674043,-31.7654177388073,0.));
#71142=CARTESIAN_POINT('Ctrl Pts',(35.0647196674043,-31.7654177388073,20.));
#71143=CARTESIAN_POINT('Ctrl Pts',(35.0402800992547,-31.7879188481278,0.));
#71144=CARTESIAN_POINT('Ctrl Pts',(35.0402800992547,-31.7879188481278,20.));
#71145=CARTESIAN_POINT('Ctrl Pts',(35.0158256238691,-31.8104021055033,0.));
#71146=CARTESIAN_POINT('Ctrl Pts',(35.0158256238691,-31.8104021055033,20.));
#71147=CARTESIAN_POINT('Ctrl Pts',(34.991356253797,-31.8328675005809,0.));
#71148=CARTESIAN_POINT('Ctrl Pts',(34.991356253797,-31.8328675005809,20.));
#71149=CARTESIAN_POINT('Ctrl Pts',(34.9668720015954,-31.8553150230168,0.));
#71150=CARTESIAN_POINT('Ctrl Pts',(34.9668720015954,-31.8553150230168,20.));
#71151=CARTESIAN_POINT('Ctrl Pts',(34.9423728798289,-31.8777446624754,0.));
#71152=CARTESIAN_POINT('Ctrl Pts',(34.9423728798289,-31.8777446624754,20.));
#71153=CARTESIAN_POINT('Ctrl Pts',(34.9178589010694,-31.9001564086295,0.));
#71154=CARTESIAN_POINT('Ctrl Pts',(34.9178589010694,-31.9001564086295,20.));
#71155=CARTESIAN_POINT('Ctrl Pts',(34.8933300778963,-31.9225502511603,0.));
#71156=CARTESIAN_POINT('Ctrl Pts',(34.8933300778963,-31.9225502511603,20.));
#71157=CARTESIAN_POINT('Ctrl Pts',(34.8687864228965,-31.9449261797574,0.));
#71158=CARTESIAN_POINT('Ctrl Pts',(34.8687864228965,-31.9449261797574,20.));
#71159=CARTESIAN_POINT('Ctrl Pts',(34.8442279486644,-31.967284184119,0.));
#71160=CARTESIAN_POINT('Ctrl Pts',(34.8442279486644,-31.967284184119,20.));
#71161=CARTESIAN_POINT('Ctrl Pts',(34.8196546678026,-31.9896242539524,0.));
#71162=CARTESIAN_POINT('Ctrl Pts',(34.8196546678026,-31.9896242539524,20.));
#71163=CARTESIAN_POINT('Ctrl Pts',(34.7950665929206,-32.011946378973,0.));
#71164=CARTESIAN_POINT('Ctrl Pts',(34.7950665929206,-32.011946378973,20.));
#71165=CARTESIAN_POINT('Ctrl Pts',(34.7704637366357,-32.0342505489048,0.));
#71166=CARTESIAN_POINT('Ctrl Pts',(34.7704637366357,-32.0342505489048,20.));
#71167=CARTESIAN_POINT('Ctrl Pts',(34.7458461115727,-32.0565367534806,0.));
#71168=CARTESIAN_POINT('Ctrl Pts',(34.7458461115727,-32.0565367534806,20.));
#71169=CARTESIAN_POINT('Ctrl Pts',(34.7212137303638,-32.0788049824416,0.));
#71170=CARTESIAN_POINT('Ctrl Pts',(34.7212137303638,-32.0788049824416,20.));
#71171=CARTESIAN_POINT('Ctrl Pts',(34.6965666056491,-32.1010552255379,0.));
#71172=CARTESIAN_POINT('Ctrl Pts',(34.6965666056491,-32.1010552255379,20.));
#71173=CARTESIAN_POINT('Ctrl Pts',(34.6719047500757,-32.1232874725277,0.));
#71174=CARTESIAN_POINT('Ctrl Pts',(34.6719047500757,-32.1232874725277,20.));
#71175=CARTESIAN_POINT('Ctrl Pts',(34.6472281762982,-32.145501713178,0.));
#71176=CARTESIAN_POINT('Ctrl Pts',(34.6472281762982,-32.145501713178,20.));
#71177=CARTESIAN_POINT('Ctrl Pts',(34.6225368969784,-32.167697937264,0.));
#71178=CARTESIAN_POINT('Ctrl Pts',(34.6225368969784,-32.167697937264,20.));
#71179=CARTESIAN_POINT('Ctrl Pts',(34.5978309247855,-32.1898761345694,0.));
#71180=CARTESIAN_POINT('Ctrl Pts',(34.5978309247855,-32.1898761345694,20.));
#71181=CARTESIAN_POINT('Ctrl Pts',(34.5731102723969,-32.212036294887,0.));
#71182=CARTESIAN_POINT('Ctrl Pts',(34.5731102723969,-32.212036294887,20.));
#71183=CARTESIAN_POINT('Ctrl Pts',(34.5483749524972,-32.2341784080184,0.));
#71184=CARTESIAN_POINT('Ctrl Pts',(34.5483749524972,-32.2341784080184,20.));
#71185=CARTESIAN_POINT('Ctrl Pts',(34.5236249777791,-32.2563024637739,0.));
#71186=CARTESIAN_POINT('Ctrl Pts',(34.5236249777791,-32.2563024637739,20.));
#71187=CARTESIAN_POINT('Ctrl Pts',(34.4988603609426,-32.2784084519728,0.));
#71188=CARTESIAN_POINT('Ctrl Pts',(34.4988603609426,-32.2784084519728,20.));
#71189=CARTESIAN_POINT('Ctrl Pts',(34.474081114695,-32.3004963624427,0.));
#71190=CARTESIAN_POINT('Ctrl Pts',(34.474081114695,-32.3004963624427,20.));
#71191=CARTESIAN_POINT('Ctrl Pts',(34.4492872517507,-32.3225661850195,0.));
#71192=CARTESIAN_POINT('Ctrl Pts',(34.4492872517507,-32.3225661850195,20.));
#71193=CARTESIAN_POINT('Ctrl Pts',(34.4244787848311,-32.3446179095474,0.));
#71194=CARTESIAN_POINT('Ctrl Pts',(34.4244787848311,-32.3446179095474,20.));
#71195=CARTESIAN_POINT('Ctrl Pts',(34.3996557266651,-32.3666515258788,0.));
#71196=CARTESIAN_POINT('Ctrl Pts',(34.3996557266651,-32.3666515258788,20.));
#71197=CARTESIAN_POINT('Ctrl Pts',(34.3748180899889,-32.388667023875,0.));
#71198=CARTESIAN_POINT('Ctrl Pts',(34.3748180899889,-32.388667023875,20.));
#71199=CARTESIAN_POINT('Ctrl Pts',(34.3499658875467,-32.4106643934066,0.));
#71200=CARTESIAN_POINT('Ctrl Pts',(34.3499658875467,-32.4106643934066,20.));
#71201=CARTESIAN_POINT('Ctrl Pts',(34.3250991320904,-32.4326436243533,0.));
#71202=CARTESIAN_POINT('Ctrl Pts',(34.3250991320904,-32.4326436243533,20.));
#71203=CARTESIAN_POINT('Ctrl Pts',(34.3002178363797,-32.4546047066034,0.));
#71204=CARTESIAN_POINT('Ctrl Pts',(34.3002178363797,-32.4546047066034,20.));
#71205=CARTESIAN_POINT('Ctrl Pts',(34.2753220131812,-32.4765476300538,0.));
#71206=CARTESIAN_POINT('Ctrl Pts',(34.2753220131812,-32.4765476300538,20.));
#71207=CARTESIAN_POINT('Ctrl Pts',(34.2504116752689,-32.4984723846098,0.));
#71208=CARTESIAN_POINT('Ctrl Pts',(34.2504116752689,-32.4984723846098,20.));
#71209=CARTESIAN_POINT('Ctrl Pts',(34.2254868354237,-32.5203789601849,0.));
#71210=CARTESIAN_POINT('Ctrl Pts',(34.2254868354237,-32.5203789601849,20.));
#71211=CARTESIAN_POINT('Ctrl Pts',(34.2005475064343,-32.542267346702,0.));
#71212=CARTESIAN_POINT('Ctrl Pts',(34.2005475064343,-32.542267346702,20.));
#71213=CARTESIAN_POINT('Ctrl Pts',(34.1755937010962,-32.564137534092,0.));
#71214=CARTESIAN_POINT('Ctrl Pts',(34.1755937010962,-32.564137534092,20.));
#71215=CARTESIAN_POINT('Ctrl Pts',(34.1506254322131,-32.585989512295,0.));
#71216=CARTESIAN_POINT('Ctrl Pts',(34.1506254322131,-32.585989512295,20.));
#71217=CARTESIAN_POINT('Ctrl Pts',(34.1256427125955,-32.6078232712594,0.));
#71218=CARTESIAN_POINT('Ctrl Pts',(34.1256427125955,-32.6078232712594,20.));
#71219=CARTESIAN_POINT('Ctrl Pts',(34.1006455550618,-32.6296388009428,0.));
#71220=CARTESIAN_POINT('Ctrl Pts',(34.1006455550618,-32.6296388009428,20.));
#71221=CARTESIAN_POINT('Ctrl Pts',(34.0756339724376,-32.6514360913116,0.));
#71222=CARTESIAN_POINT('Ctrl Pts',(34.0756339724376,-32.6514360913116,20.));
#71223=CARTESIAN_POINT('Ctrl Pts',(34.0506079775557,-32.6732151323407,0.));
#71224=CARTESIAN_POINT('Ctrl Pts',(34.0506079775557,-32.6732151323407,20.));
#71225=CARTESIAN_POINT('Ctrl Pts',(34.0255675832564,-32.694975914014,0.));
#71226=CARTESIAN_POINT('Ctrl Pts',(34.0255675832564,-32.694975914014,20.));
#71227=CARTESIAN_POINT('Ctrl Pts',(34.0005128023871,-32.7167184263237,0.));
#71228=CARTESIAN_POINT('Ctrl Pts',(34.0005128023871,-32.7167184263237,20.));
#71229=CARTESIAN_POINT('Ctrl Pts',(33.9754436478026,-32.7384426592708,0.));
#71230=CARTESIAN_POINT('Ctrl Pts',(33.9754436478026,-32.7384426592708,20.));
#71231=CARTESIAN_POINT('Ctrl Pts',(33.950360132365,-32.7601486028652,0.));
#71232=CARTESIAN_POINT('Ctrl Pts',(33.950360132365,-32.7601486028652,20.));
#71233=CARTESIAN_POINT('Ctrl Pts',(33.9252622689445,-32.781836247126,0.));
#71234=CARTESIAN_POINT('Ctrl Pts',(33.9252622689445,-32.781836247126,20.));
#71235=CARTESIAN_POINT('Ctrl Pts',(33.9001500704179,-32.8035055820806,0.));
#71236=CARTESIAN_POINT('Ctrl Pts',(33.9001500704179,-32.8035055820806,20.));
#71237=CARTESIAN_POINT('Ctrl Pts',(33.8750235496691,-32.8251565977646,0.));
#71238=CARTESIAN_POINT('Ctrl Pts',(33.8750235496691,-32.8251565977646,20.));
#71239=CARTESIAN_POINT('Ctrl Pts',(33.8498827195893,-32.8467892842227,0.));
#71240=CARTESIAN_POINT('Ctrl Pts',(33.8498827195893,-32.8467892842227,20.));
#71241=CARTESIAN_POINT('Ctrl Pts',(33.8247275930774,-32.8684036315086,0.));
#71242=CARTESIAN_POINT('Ctrl Pts',(33.8247275930774,-32.8684036315086,20.));
#71243=CARTESIAN_POINT('Ctrl Pts',(33.7995581830395,-32.8899996296849,0.));
#71244=CARTESIAN_POINT('Ctrl Pts',(33.7995581830395,-32.8899996296849,20.));
#71245=CARTESIAN_POINT('Ctrl Pts',(33.7743745023893,-32.9115772688235,0.));
#71246=CARTESIAN_POINT('Ctrl Pts',(33.7743745023893,-32.9115772688235,20.));
#71247=CARTESIAN_POINT('Ctrl Pts',(33.7491765640476,-32.9331365390046,0.));
#71248=CARTESIAN_POINT('Ctrl Pts',(33.7491765640476,-32.9331365390046,20.));
#71249=CARTESIAN_POINT('Ctrl Pts',(33.723964380943,-32.9546774303179,0.));
#71250=CARTESIAN_POINT('Ctrl Pts',(33.723964380943,-32.9546774303179,20.));
#71251=CARTESIAN_POINT('Ctrl Pts',(33.6987379660104,-32.9761999328605,0.));
#71252=CARTESIAN_POINT('Ctrl Pts',(33.6987379660104,-32.9761999328605,20.));
#71253=CARTESIAN_POINT('Ctrl Pts',(33.6734973321919,-32.9977040367383,0.));
#71254=CARTESIAN_POINT('Ctrl Pts',(33.6734973321919,-32.9977040367383,20.));
#71255=CARTESIAN_POINT('Ctrl Pts',(33.6482424924372,-33.0191897320665,0.));
#71256=CARTESIAN_POINT('Ctrl Pts',(33.6482424924372,-33.0191897320665,20.));
#71257=CARTESIAN_POINT('Ctrl Pts',(33.6229734597032,-33.0406570089692,0.));
#71258=CARTESIAN_POINT('Ctrl Pts',(33.6229734597032,-33.0406570089692,20.));
#71259=CARTESIAN_POINT('Ctrl Pts',(33.5976902469543,-33.0621058575797,0.));
#71260=CARTESIAN_POINT('Ctrl Pts',(33.5976902469543,-33.0621058575797,20.));
#71261=CARTESIAN_POINT('Ctrl Pts',(33.572392867162,-33.0835362680399,0.));
#71262=CARTESIAN_POINT('Ctrl Pts',(33.572392867162,-33.0835362680399,20.));
#71263=CARTESIAN_POINT('Ctrl Pts',(33.5470813333053,-33.1049482305004,0.));
#71264=CARTESIAN_POINT('Ctrl Pts',(33.5470813333053,-33.1049482305004,20.));
#71265=CARTESIAN_POINT('Ctrl Pts',(33.5217556583703,-33.1263417351208,0.));
#71266=CARTESIAN_POINT('Ctrl Pts',(33.5217556583703,-33.1263417351208,20.));
#71267=CARTESIAN_POINT('Ctrl Pts',(33.4964158553505,-33.1477167720697,0.));
#71268=CARTESIAN_POINT('Ctrl Pts',(33.4964158553505,-33.1477167720697,20.));
#71269=CARTESIAN_POINT('Ctrl Pts',(33.4710619372468,-33.1690733315248,0.));
#71270=CARTESIAN_POINT('Ctrl Pts',(33.4710619372468,-33.1690733315248,20.));
#71271=CARTESIAN_POINT('Ctrl Pts',(33.4456939170666,-33.1904114036721,0.));
#71272=CARTESIAN_POINT('Ctrl Pts',(33.4456939170666,-33.1904114036721,20.));
#71273=CARTESIAN_POINT('Ctrl Pts',(33.4203118078248,-33.2117309787064,0.));
#71274=CARTESIAN_POINT('Ctrl Pts',(33.4203118078248,-33.2117309787064,20.));
#71275=CARTESIAN_POINT('Ctrl Pts',(33.3949156225429,-33.233032046831,0.));
#71276=CARTESIAN_POINT('Ctrl Pts',(33.3949156225429,-33.233032046831,20.));
#71277=CARTESIAN_POINT('Ctrl Pts',(33.3695053742505,-33.2543145982587,0.));
#71278=CARTESIAN_POINT('Ctrl Pts',(33.3695053742505,-33.2543145982587,20.));
#71279=CARTESIAN_POINT('Ctrl Pts',(33.3440810759838,-33.2755786232108,0.));
#71280=CARTESIAN_POINT('Ctrl Pts',(33.3440810759838,-33.2755786232108,20.));
#71281=CARTESIAN_POINT('Ctrl Pts',(33.3186427407863,-33.2968241119177,0.));
#71282=CARTESIAN_POINT('Ctrl Pts',(33.3186427407863,-33.2968241119177,20.));
#71283=CARTESIAN_POINT('Ctrl Pts',(33.2931903817093,-33.318051054619,0.));
#71284=CARTESIAN_POINT('Ctrl Pts',(33.2931903817093,-33.318051054619,20.));
#71285=CARTESIAN_POINT('Ctrl Pts',(33.2677240118112,-33.3392594415636,0.));
#71286=CARTESIAN_POINT('Ctrl Pts',(33.2677240118112,-33.3392594415636,20.));
#71287=CARTESIAN_POINT('Ctrl Pts',(33.2422436441578,-33.3604492630093,0.));
#71288=CARTESIAN_POINT('Ctrl Pts',(33.2422436441578,-33.3604492630093,20.));
#71289=CARTESIAN_POINT('Ctrl Pts',(33.2167492918215,-33.3816205092222,0.));
#71290=CARTESIAN_POINT('Ctrl Pts',(33.2167492918215,-33.3816205092222,20.));
#71291=CARTESIAN_POINT('Ctrl Pts',(33.1912409678819,-33.4027731704774,0.));
#71292=CARTESIAN_POINT('Ctrl Pts',(33.1912409678819,-33.4027731704774,20.));
#71293=CARTESIAN_POINT('Ctrl Pts',(33.1657186854252,-33.4239072370581,0.));
#71294=CARTESIAN_POINT('Ctrl Pts',(33.1657186854252,-33.4239072370581,20.));
#71295=CARTESIAN_POINT('Ctrl Pts',(33.1401824575448,-33.4450226992568,0.));
#71296=CARTESIAN_POINT('Ctrl Pts',(33.1401824575448,-33.4450226992568,20.));
#71297=CARTESIAN_POINT('Ctrl Pts',(33.1146322973416,-33.4661195473749,0.));
#71298=CARTESIAN_POINT('Ctrl Pts',(33.1146322973416,-33.4661195473749,20.));
#71299=CARTESIAN_POINT('Ctrl Pts',(33.0890682179238,-33.4871977717238,0.));
#71300=CARTESIAN_POINT('Ctrl Pts',(33.0890682179238,-33.4871977717238,20.));
#71301=CARTESIAN_POINT('Ctrl Pts',(33.063490232407,-33.5082573626235,0.));
#71302=CARTESIAN_POINT('Ctrl Pts',(33.063490232407,-33.5082573626235,20.));
#71303=CARTESIAN_POINT('Ctrl Pts',(33.0378983539137,-33.5292983104032,0.));
#71304=CARTESIAN_POINT('Ctrl Pts',(33.0378983539137,-33.5292983104032,20.));
#71305=CARTESIAN_POINT('Ctrl Pts',(33.0122925955738,-33.5503206054004,0.));
#71306=CARTESIAN_POINT('Ctrl Pts',(33.0122925955738,-33.5503206054004,20.));
#71307=CARTESIAN_POINT('Ctrl Pts',(32.986672970524,-33.5713242379612,0.));
#71308=CARTESIAN_POINT('Ctrl Pts',(32.986672970524,-33.5713242379612,20.));
#71309=CARTESIAN_POINT('Ctrl Pts',(32.9610394919081,-33.5923091984411,0.));
#71310=CARTESIAN_POINT('Ctrl Pts',(32.9610394919081,-33.5923091984411,20.));
#71311=CARTESIAN_POINT('Ctrl Pts',(32.935392172877,-33.6132754772046,0.));
#71312=CARTESIAN_POINT('Ctrl Pts',(32.935392172877,-33.6132754772046,20.));
#71313=CARTESIAN_POINT('Ctrl Pts',(32.9097310265884,-33.6342230646254,0.));
#71314=CARTESIAN_POINT('Ctrl Pts',(32.9097310265884,-33.6342230646254,20.));
#71315=CARTESIAN_POINT('Ctrl Pts',(32.8840560662069,-33.6551519510862,0.));
#71316=CARTESIAN_POINT('Ctrl Pts',(32.8840560662069,-33.6551519510862,20.));
#71317=CARTESIAN_POINT('Ctrl Pts',(32.8583673049046,-33.6760621269785,0.));
#71318=CARTESIAN_POINT('Ctrl Pts',(32.8583673049046,-33.6760621269785,20.));
#71319=CARTESIAN_POINT('Ctrl Pts',(32.8326647558605,-33.6969535827028,0.));
#71320=CARTESIAN_POINT('Ctrl Pts',(32.8326647558605,-33.6969535827028,20.));
#71321=CARTESIAN_POINT('Ctrl Pts',(32.8069484322617,-33.717826308669,0.));
#71322=CARTESIAN_POINT('Ctrl Pts',(32.8069484322617,-33.717826308669,20.));
#71323=CARTESIAN_POINT('Ctrl Pts',(32.7812183473018,-33.7386802952956,0.));
#71324=CARTESIAN_POINT('Ctrl Pts',(32.7812183473018,-33.7386802952956,20.));
#71325=CARTESIAN_POINT('Ctrl Pts',(32.755474514181,-33.7595155330097,0.));
#71326=CARTESIAN_POINT('Ctrl Pts',(32.755474514181,-33.7595155330097,20.));
#71327=CARTESIAN_POINT('Ctrl Pts',(32.7297169461064,-33.7803320122473,0.));
#71328=CARTESIAN_POINT('Ctrl Pts',(32.7297169461064,-33.7803320122473,20.));
#71329=CARTESIAN_POINT('Ctrl Pts',(32.7039456562922,-33.8011297234537,0.));
#71330=CARTESIAN_POINT('Ctrl Pts',(32.7039456562922,-33.8011297234537,20.));
#71331=CARTESIAN_POINT('Ctrl Pts',(32.6781606579597,-33.8219086570836,0.));
#71332=CARTESIAN_POINT('Ctrl Pts',(32.6781606579597,-33.8219086570836,20.));
#71333=CARTESIAN_POINT('Ctrl Pts',(32.652361964338,-33.8426688036011,0.));
#71334=CARTESIAN_POINT('Ctrl Pts',(32.652361964338,-33.8426688036011,20.));
#71335=CARTESIAN_POINT('Ctrl Pts',(32.6265495886629,-33.8634101534794,0.));
#71336=CARTESIAN_POINT('Ctrl Pts',(32.6265495886629,-33.8634101534794,20.));
#71337=CARTESIAN_POINT('Ctrl Pts',(32.6007235441777,-33.8841326972008,0.));
#71338=CARTESIAN_POINT('Ctrl Pts',(32.6007235441777,-33.8841326972008,20.));
#71339=CARTESIAN_POINT('Ctrl Pts',(32.5748838441319,-33.9048364252556,0.));
#71340=CARTESIAN_POINT('Ctrl Pts',(32.5748838441319,-33.9048364252556,20.));
#71341=CARTESIAN_POINT('Ctrl Pts',(32.5490305017817,-33.9255213281434,0.));
#71342=CARTESIAN_POINT('Ctrl Pts',(32.5490305017817,-33.9255213281434,20.));
#71343=CARTESIAN_POINT('Ctrl Pts',(32.5231635303904,-33.9461873963724,0.));
#71344=CARTESIAN_POINT('Ctrl Pts',(32.5231635303904,-33.9461873963724,20.));
#71345=CARTESIAN_POINT('Ctrl Pts',(32.4972829432285,-33.9668346204605,0.));
#71346=CARTESIAN_POINT('Ctrl Pts',(32.4972829432285,-33.9668346204605,20.));
#71347=CARTESIAN_POINT('Ctrl Pts',(32.4713887535741,-33.987462990935,0.));
#71348=CARTESIAN_POINT('Ctrl Pts',(32.4713887535741,-33.987462990935,20.));
#71349=CARTESIAN_POINT('Ctrl Pts',(32.4454809747123,-34.0080724983324,0.));
#71350=CARTESIAN_POINT('Ctrl Pts',(32.4454809747123,-34.0080724983324,20.));
#71351=CARTESIAN_POINT('Ctrl Pts',(32.4195596199344,-34.0286631331978,0.));
#71352=CARTESIAN_POINT('Ctrl Pts',(32.4195596199344,-34.0286631331978,20.));
#71353=CARTESIAN_POINT('Ctrl Pts',(32.3936247025392,-34.0492348860855,0.));
#71354=CARTESIAN_POINT('Ctrl Pts',(32.3936247025392,-34.0492348860855,20.));
#71355=CARTESIAN_POINT('Ctrl Pts',(32.3676762358321,-34.0697877475586,0.));
#71356=CARTESIAN_POINT('Ctrl Pts',(32.3676762358321,-34.0697877475586,20.));
#71357=CARTESIAN_POINT('Ctrl Pts',(32.3417142331256,-34.0903217081898,0.));
#71358=CARTESIAN_POINT('Ctrl Pts',(32.3417142331256,-34.0903217081898,20.));
#71359=CARTESIAN_POINT('Ctrl Pts',(32.3157387077392,-34.1108367585604,0.));
#71360=CARTESIAN_POINT('Ctrl Pts',(32.3157387077392,-34.1108367585604,20.));
#71361=CARTESIAN_POINT('Ctrl Pts',(32.289749672999,-34.131332889261,0.));
#71362=CARTESIAN_POINT('Ctrl Pts',(32.289749672999,-34.131332889261,20.));
#71363=CARTESIAN_POINT('Ctrl Pts',(32.2637471422388,-34.1518100908915,0.));
#71364=CARTESIAN_POINT('Ctrl Pts',(32.2637471422388,-34.1518100908915,20.));
#71365=CARTESIAN_POINT('Ctrl Pts',(32.2377311287994,-34.1722683540613,0.));
#71366=CARTESIAN_POINT('Ctrl Pts',(32.2377311287994,-34.1722683540613,20.));
#71367=CARTESIAN_POINT('Ctrl Pts',(32.2117016460282,-34.1927076693884,0.));
#71368=CARTESIAN_POINT('Ctrl Pts',(32.2117016460282,-34.1927076693884,20.));
#71369=CARTESIAN_POINT('Ctrl Pts',(32.1856587072789,-34.2131280274994,0.));
#71370=CARTESIAN_POINT('Ctrl Pts',(32.1856587072789,-34.2131280274994,20.));
#71371=CARTESIAN_POINT('Ctrl Pts',(32.1596023259127,-34.233529419031,0.));
#71372=CARTESIAN_POINT('Ctrl Pts',(32.1596023259127,-34.233529419031,20.));
#71373=CARTESIAN_POINT('Ctrl Pts',(32.1335325152974,-34.2539118346284,0.));
#71374=CARTESIAN_POINT('Ctrl Pts',(32.1335325152974,-34.2539118346284,20.));
#71375=CARTESIAN_POINT('Ctrl Pts',(32.1074492888083,-34.2742752649465,0.));
#71376=CARTESIAN_POINT('Ctrl Pts',(32.1074492888083,-34.2742752649465,20.));
#71377=CARTESIAN_POINT('Ctrl Pts',(32.081352659827,-34.2946197006486,0.));
#71378=CARTESIAN_POINT('Ctrl Pts',(32.081352659827,-34.2946197006486,20.));
#71379=CARTESIAN_POINT('Ctrl Pts',(32.0552426417428,-34.3149451324082,0.));
#71380=CARTESIAN_POINT('Ctrl Pts',(32.0552426417428,-34.3149451324082,20.));
#71381=CARTESIAN_POINT('Ctrl Pts',(32.0291192479513,-34.335251550907,0.));
#71382=CARTESIAN_POINT('Ctrl Pts',(32.0291192479513,-34.335251550907,20.));
#71383=CARTESIAN_POINT('Ctrl Pts',(32.0029824918551,-34.3555389468366,0.));
#71384=CARTESIAN_POINT('Ctrl Pts',(32.0029824918551,-34.3555389468366,20.));
#71385=CARTESIAN_POINT('Ctrl Pts',(31.9768323868632,-34.3758073108972,0.));
#71386=CARTESIAN_POINT('Ctrl Pts',(31.9768323868632,-34.3758073108972,20.));
#71387=CARTESIAN_POINT('Ctrl Pts',(31.9506689463919,-34.3960566337983,0.));
#71388=CARTESIAN_POINT('Ctrl Pts',(31.9506689463919,-34.3960566337983,20.));
#71389=CARTESIAN_POINT('Ctrl Pts',(31.9244921838641,-34.4162869062584,0.));
#71390=CARTESIAN_POINT('Ctrl Pts',(31.9244921838641,-34.4162869062584,20.));
#71391=CARTESIAN_POINT('Ctrl Pts',(31.8983021127101,-34.4364981190057,0.));
#71392=CARTESIAN_POINT('Ctrl Pts',(31.8983021127101,-34.4364981190057,20.));
#71393=CARTESIAN_POINT('Ctrl Pts',(31.8720987463673,-34.4566902627777,0.));
#71394=CARTESIAN_POINT('Ctrl Pts',(31.8720987463673,-34.4566902627777,20.));
#71395=CARTESIAN_POINT('Ctrl Pts',(31.8458820982794,-34.4768633283209,0.));
#71396=CARTESIAN_POINT('Ctrl Pts',(31.8458820982794,-34.4768633283209,20.));
#71397=CARTESIAN_POINT('Ctrl Pts',(31.819652181897,-34.4970173063908,0.));
#71398=CARTESIAN_POINT('Ctrl Pts',(31.819652181897,-34.4970173063908,20.));
#71399=CARTESIAN_POINT('Ctrl Pts',(31.7934090106771,-34.5171521877519,0.));
#71400=CARTESIAN_POINT('Ctrl Pts',(31.7934090106771,-34.5171521877519,20.));
#71401=CARTESIAN_POINT('Ctrl Pts',(31.7671525980837,-34.5372679631778,0.));
#71402=CARTESIAN_POINT('Ctrl Pts',(31.7671525980837,-34.5372679631778,20.));
#71403=CARTESIAN_POINT('Ctrl Pts',(31.7408829575878,-34.5573646234518,0.));
#71404=CARTESIAN_POINT('Ctrl Pts',(31.7408829575878,-34.5573646234518,20.));
#71405=CARTESIAN_POINT('Ctrl Pts',(31.7146001026678,-34.5774421593669,0.));
#71406=CARTESIAN_POINT('Ctrl Pts',(31.7146001026678,-34.5774421593669,20.));
#71407=CARTESIAN_POINT('Ctrl Pts',(31.6883040468088,-34.5975005617252,0.));
#71408=CARTESIAN_POINT('Ctrl Pts',(31.6883040468088,-34.5975005617252,20.));
#71409=CARTESIAN_POINT('Ctrl Pts',(31.6619948035026,-34.6175398213376,0.));
#71410=CARTESIAN_POINT('Ctrl Pts',(31.6619948035026,-34.6175398213376,20.));
#71411=CARTESIAN_POINT('Ctrl Pts',(31.6356723862475,-34.6375599290243,0.));
#71412=CARTESIAN_POINT('Ctrl Pts',(31.6356723862475,-34.6375599290243,20.));
#71413=CARTESIAN_POINT('Ctrl Pts',(31.609336808548,-34.6575608756141,0.));
#71414=CARTESIAN_POINT('Ctrl Pts',(31.609336808548,-34.6575608756141,20.));
#71415=CARTESIAN_POINT('Ctrl Pts',(31.5829880839157,-34.6775426519456,0.));
#71416=CARTESIAN_POINT('Ctrl Pts',(31.5829880839157,-34.6775426519456,20.));
#71417=CARTESIAN_POINT('Ctrl Pts',(31.556626225869,-34.6975052488666,0.));
#71418=CARTESIAN_POINT('Ctrl Pts',(31.556626225869,-34.6975052488666,20.));
#71419=CARTESIAN_POINT('Ctrl Pts',(31.5302512479332,-34.7174486572342,0.));
#71420=CARTESIAN_POINT('Ctrl Pts',(31.5302512479332,-34.7174486572342,20.));
#71421=CARTESIAN_POINT('Ctrl Pts',(31.5038631636409,-34.7373728679152,0.));
#71422=CARTESIAN_POINT('Ctrl Pts',(31.5038631636409,-34.7373728679152,20.));
#71423=CARTESIAN_POINT('Ctrl Pts',(31.4774619865312,-34.7572778717853,0.));
#71424=CARTESIAN_POINT('Ctrl Pts',(31.4774619865312,-34.7572778717853,20.));
#71425=CARTESIAN_POINT('Ctrl Pts',(31.4510477301503,-34.7771636597296,0.));
#71426=CARTESIAN_POINT('Ctrl Pts',(31.4510477301503,-34.7771636597296,20.));
#71427=CARTESIAN_POINT('Ctrl Pts',(31.4246204080513,-34.7970302226433,0.));
#71428=CARTESIAN_POINT('Ctrl Pts',(31.4246204080513,-34.7970302226433,20.));
#71429=CARTESIAN_POINT('Ctrl Pts',(31.3981800337935,-34.8168775514299,0.));
#71430=CARTESIAN_POINT('Ctrl Pts',(31.3981800337935,-34.8168775514299,20.));
#71431=CARTESIAN_POINT('Ctrl Pts',(31.3717266209433,-34.8367056370027,0.));
#71432=CARTESIAN_POINT('Ctrl Pts',(31.3717266209433,-34.8367056370027,20.));
#71433=CARTESIAN_POINT('Ctrl Pts',(31.3452601830725,-34.856514470283,0.));
#71434=CARTESIAN_POINT('Ctrl Pts',(31.3452601830725,-34.856514470283,20.));
#71435=CARTESIAN_POINT('Ctrl Pts',(31.3187807337598,-34.8763040422018,0.));
#71436=CARTESIAN_POINT('Ctrl Pts',(31.3187807337598,-34.8763040422018,20.));
#71437=CARTESIAN_POINT('Ctrl Pts',(31.2922882865907,-34.8960743436995,0.));
#71438=CARTESIAN_POINT('Ctrl Pts',(31.2922882865907,-34.8960743436995,20.));
#71439=CARTESIAN_POINT('Ctrl Pts',(31.2657828551579,-34.9158253657263,0.));
#71440=CARTESIAN_POINT('Ctrl Pts',(31.2657828551579,-34.9158253657263,20.));
#71441=CARTESIAN_POINT('Ctrl Pts',(31.2392644530613,-34.9355570992414,0.));
#71442=CARTESIAN_POINT('Ctrl Pts',(31.2392644530613,-34.9355570992414,20.));
#71443=CARTESIAN_POINT('Ctrl Pts',(31.2127330939085,-34.9552695352152,0.));
#71444=CARTESIAN_POINT('Ctrl Pts',(31.2127330939085,-34.9552695352152,20.));
#71445=CARTESIAN_POINT('Ctrl Pts',(31.1861887913133,-34.974962664626,0.));
#71446=CARTESIAN_POINT('Ctrl Pts',(31.1861887913133,-34.974962664626,20.));
#71447=CARTESIAN_POINT('Ctrl Pts',(31.1596315588953,-34.9946364784612,0.));
#71448=CARTESIAN_POINT('Ctrl Pts',(31.1596315588953,-34.9946364784612,20.));
#71449=CARTESIAN_POINT('Ctrl Pts',(31.1330614102809,-35.0142909677175,0.));
#71450=CARTESIAN_POINT('Ctrl Pts',(31.1330614102809,-35.0142909677175,20.));
#71451=CARTESIAN_POINT('Ctrl Pts',(31.1064783591027,-35.0339261234013,0.));
#71452=CARTESIAN_POINT('Ctrl Pts',(31.1064783591027,-35.0339261234013,20.));
#71453=CARTESIAN_POINT('Ctrl Pts',(31.0798824190003,-35.0535419365277,0.));
#71454=CARTESIAN_POINT('Ctrl Pts',(31.0798824190003,-35.0535419365277,20.));
#71455=CARTESIAN_POINT('Ctrl Pts',(31.0532736036193,-35.0731383981212,0.));
#71456=CARTESIAN_POINT('Ctrl Pts',(31.0532736036193,-35.0731383981212,20.));
#71457=CARTESIAN_POINT('Ctrl Pts',(31.026651926612,-35.0927154992152,0.));
#71458=CARTESIAN_POINT('Ctrl Pts',(31.026651926612,-35.0927154992152,20.));
#71459=CARTESIAN_POINT('Ctrl Pts',(31.0000174016378,-35.1122732308527,0.));
#71460=CARTESIAN_POINT('Ctrl Pts',(31.0000174016378,-35.1122732308527,20.));
#71461=CARTESIAN_POINT('Ctrl Pts',(30.9733700423633,-35.131811584087,0.));
#71462=CARTESIAN_POINT('Ctrl Pts',(30.9733700423633,-35.131811584087,20.));
#71463=CARTESIAN_POINT('Ctrl Pts',(30.9467098624624,-35.1513305499814,0.));
#71464=CARTESIAN_POINT('Ctrl Pts',(30.9467098624624,-35.1513305499814,20.));
#71465=CARTESIAN_POINT('Ctrl Pts',(30.9200368756162,-35.170830119609,0.));
#71466=CARTESIAN_POINT('Ctrl Pts',(30.9200368756162,-35.170830119609,20.));
#71467=CARTESIAN_POINT('Ctrl Pts',(30.8933510955115,-35.1903102840519,0.));
#71468=CARTESIAN_POINT('Ctrl Pts',(30.8933510955115,-35.1903102840519,20.));
#71469=CARTESIAN_POINT('Ctrl Pts',(30.8666525358408,-35.2097710343998,0.));
#71470=CARTESIAN_POINT('Ctrl Pts',(30.8666525358408,-35.2097710343998,20.));
#71471=CARTESIAN_POINT('Ctrl Pts',(30.8399412103026,-35.2292123617517,0.));
#71472=CARTESIAN_POINT('Ctrl Pts',(30.8399412103026,-35.2292123617517,20.));
#71473=CARTESIAN_POINT('Ctrl Pts',(30.8132171326021,-35.2486342572162,0.));
#71474=CARTESIAN_POINT('Ctrl Pts',(30.8132171326021,-35.2486342572162,20.));
#71475=CARTESIAN_POINT('Ctrl Pts',(30.786480316451,-35.2680367119112,0.));
#71476=CARTESIAN_POINT('Ctrl Pts',(30.786480316451,-35.2680367119112,20.));
#71477=CARTESIAN_POINT('Ctrl Pts',(30.7597307755696,-35.2874197169657,0.));
#71478=CARTESIAN_POINT('Ctrl Pts',(30.7597307755696,-35.2874197169657,20.));
#71479=CARTESIAN_POINT('Ctrl Pts',(30.732968523684,-35.3067832635177,0.));
#71480=CARTESIAN_POINT('Ctrl Pts',(30.732968523684,-35.3067832635177,20.));
#71481=CARTESIAN_POINT('Ctrl Pts',(30.7061935745273,-35.3261273427148,0.));
#71482=CARTESIAN_POINT('Ctrl Pts',(30.7061935745273,-35.3261273427148,20.));
#71483=CARTESIAN_POINT('Ctrl Pts',(30.6794059418388,-35.3454519457137,0.));
#71484=CARTESIAN_POINT('Ctrl Pts',(30.6794059418388,-35.3454519457137,20.));
#71485=CARTESIAN_POINT('Ctrl Pts',(30.6526056393638,-35.3647570636798,0.));
#71486=CARTESIAN_POINT('Ctrl Pts',(30.6526056393638,-35.3647570636798,20.));
#71487=CARTESIAN_POINT('Ctrl Pts',(30.6257926808541,-35.3840426877879,0.));
#71488=CARTESIAN_POINT('Ctrl Pts',(30.6257926808541,-35.3840426877879,20.));
#71489=CARTESIAN_POINT('Ctrl Pts',(30.5989670800681,-35.4033088092226,0.));
#71490=CARTESIAN_POINT('Ctrl Pts',(30.5989670800681,-35.4033088092226,20.));
#71491=CARTESIAN_POINT('Ctrl Pts',(30.5721288507715,-35.4225554191786,0.));
#71492=CARTESIAN_POINT('Ctrl Pts',(30.5721288507715,-35.4225554191786,20.));
#71493=CARTESIAN_POINT('Ctrl Pts',(30.5452780067368,-35.4417825088605,0.));
#71494=CARTESIAN_POINT('Ctrl Pts',(30.5452780067368,-35.4417825088605,20.));
#71495=CARTESIAN_POINT('Ctrl Pts',(30.5184145617424,-35.4609900694812,0.));
#71496=CARTESIAN_POINT('Ctrl Pts',(30.5184145617424,-35.4609900694812,20.));
#71497=CARTESIAN_POINT('Ctrl Pts',(30.4915385295724,-35.4801780922626,0.));
#71498=CARTESIAN_POINT('Ctrl Pts',(30.4915385295724,-35.4801780922626,20.));
#71499=CARTESIAN_POINT('Ctrl Pts',(30.4646499240177,-35.4993465684362,0.));
#71500=CARTESIAN_POINT('Ctrl Pts',(30.4646499240177,-35.4993465684362,20.));
#71501=CARTESIAN_POINT('Ctrl Pts',(30.437748758876,-35.518495489243,0.));
#71502=CARTESIAN_POINT('Ctrl Pts',(30.437748758876,-35.518495489243,20.));
#71503=CARTESIAN_POINT('Ctrl Pts',(30.4108350479521,-35.5376248459348,0.));
#71504=CARTESIAN_POINT('Ctrl Pts',(30.4108350479521,-35.5376248459348,20.));
#71505=CARTESIAN_POINT('Ctrl Pts',(30.3839088050584,-35.5567346297737,0.));
#71506=CARTESIAN_POINT('Ctrl Pts',(30.3839088050584,-35.5567346297737,20.));
#71507=CARTESIAN_POINT('Ctrl Pts',(30.3569700440131,-35.5758248320301,0.));
#71508=CARTESIAN_POINT('Ctrl Pts',(30.3569700440131,-35.5758248320301,20.));
#71509=CARTESIAN_POINT('Ctrl Pts',(30.3300187786403,-35.5948954439837,0.));
#71510=CARTESIAN_POINT('Ctrl Pts',(30.3300187786403,-35.5948954439837,20.));
#71511=CARTESIAN_POINT('Ctrl Pts',(30.3030550227693,-35.6139464569223,0.));
#71512=CARTESIAN_POINT('Ctrl Pts',(30.3030550227693,-35.6139464569223,20.));
#71513=CARTESIAN_POINT('Ctrl Pts',(30.2760787902362,-35.6329778621436,0.));
#71514=CARTESIAN_POINT('Ctrl Pts',(30.2760787902362,-35.6329778621436,20.));
#71515=CARTESIAN_POINT('Ctrl Pts',(30.2490900948838,-35.6519896509552,0.));
#71516=CARTESIAN_POINT('Ctrl Pts',(30.2490900948838,-35.6519896509552,20.));
#71517=CARTESIAN_POINT('Ctrl Pts',(30.2220889505625,-35.6709818146751,0.));
#71518=CARTESIAN_POINT('Ctrl Pts',(30.2220889505625,-35.6709818146751,20.));
#71519=CARTESIAN_POINT('Ctrl Pts',(30.1950753711288,-35.6899543446309,0.));
#71520=CARTESIAN_POINT('Ctrl Pts',(30.1950753711288,-35.6899543446309,20.));
#71521=CARTESIAN_POINT('Ctrl Pts',(30.1680493704465,-35.7089072321597,0.));
#71522=CARTESIAN_POINT('Ctrl Pts',(30.1680493704465,-35.7089072321597,20.));
#71523=CARTESIAN_POINT('Ctrl Pts',(30.141010962385,-35.727840468608,0.));
#71524=CARTESIAN_POINT('Ctrl Pts',(30.141010962385,-35.727840468608,20.));
#71525=CARTESIAN_POINT('Ctrl Pts',(30.1139601608197,-35.7467540453308,0.));
#71526=CARTESIAN_POINT('Ctrl Pts',(30.1139601608197,-35.7467540453308,20.));
#71527=CARTESIAN_POINT('Ctrl Pts',(30.0868969796328,-35.7656479536939,0.));
#71528=CARTESIAN_POINT('Ctrl Pts',(30.0868969796328,-35.7656479536939,20.));
#71529=CARTESIAN_POINT('Ctrl Pts',(30.0598214327127,-35.7845221850715,0.));
#71530=CARTESIAN_POINT('Ctrl Pts',(30.0598214327127,-35.7845221850715,20.));
#71531=CARTESIAN_POINT('Ctrl Pts',(30.0327335339539,-35.8033767308478,0.));
#71532=CARTESIAN_POINT('Ctrl Pts',(30.0327335339539,-35.8033767308478,20.));
#71533=CARTESIAN_POINT('Ctrl Pts',(30.005633297258,-35.8222115824167,0.));
#71534=CARTESIAN_POINT('Ctrl Pts',(30.005633297258,-35.8222115824167,20.));
#71535=CARTESIAN_POINT('Ctrl Pts',(29.9785207365333,-35.841026731182,0.));
#71536=CARTESIAN_POINT('Ctrl Pts',(29.9785207365333,-35.841026731182,20.));
#71537=CARTESIAN_POINT('Ctrl Pts',(29.9513958656946,-35.8598221685576,0.));
#71538=CARTESIAN_POINT('Ctrl Pts',(29.9513958656946,-35.8598221685576,20.));
#71539=CARTESIAN_POINT('Ctrl Pts',(29.9242586986624,-35.8785978859658,0.));
#71540=CARTESIAN_POINT('Ctrl Pts',(29.9242586986624,-35.8785978859658,20.));
#71541=CARTESIAN_POINT('Ctrl Pts',(29.8971092493634,-35.8973538748387,0.));
#71542=CARTESIAN_POINT('Ctrl Pts',(29.8971092493634,-35.8973538748387,20.));
#71543=CARTESIAN_POINT('Ctrl Pts',(29.869947531731,-35.9160901266177,0.));
#71544=CARTESIAN_POINT('Ctrl Pts',(29.869947531731,-35.9160901266177,20.));
#71545=CARTESIAN_POINT('Ctrl Pts',(29.8427735597048,-35.934806632754,0.));
#71546=CARTESIAN_POINT('Ctrl Pts',(29.8427735597048,-35.934806632754,20.));
#71547=CARTESIAN_POINT('Ctrl Pts',(29.8155873472308,-35.9535033847082,0.));
#71548=CARTESIAN_POINT('Ctrl Pts',(29.8155873472308,-35.9535033847082,20.));
#71549=CARTESIAN_POINT('Ctrl Pts',(29.7883889082614,-35.9721803739509,0.));
#71550=CARTESIAN_POINT('Ctrl Pts',(29.7883889082614,-35.9721803739509,20.));
#71551=CARTESIAN_POINT('Ctrl Pts',(29.7611782567557,-35.9908375919623,0.));
#71552=CARTESIAN_POINT('Ctrl Pts',(29.7611782567557,-35.9908375919623,20.));
#71553=CARTESIAN_POINT('Ctrl Pts',(29.7339554066796,-36.0094750302331,0.));
#71554=CARTESIAN_POINT('Ctrl Pts',(29.7339554066796,-36.0094750302331,20.));
#71555=CARTESIAN_POINT('Ctrl Pts',(29.7067203720053,-36.0280926802632,0.));
#71556=CARTESIAN_POINT('Ctrl Pts',(29.7067203720053,-36.0280926802632,20.));
#71557=CARTESIAN_POINT('Ctrl Pts',(29.6794731667106,-36.0466905335617,0.));
#71558=CARTESIAN_POINT('Ctrl Pts',(29.6794731667106,-36.0466905335617,20.));
#71559=CARTESIAN_POINT('Ctrl Pts',(29.6522138047793,-36.0652685816464,0.));
#71560=CARTESIAN_POINT('Ctrl Pts',(29.6522138047793,-36.0652685816464,20.));
#71561=CARTESIAN_POINT('Ctrl Pts',(29.6249423002017,-36.0838268160451,0.));
#71562=CARTESIAN_POINT('Ctrl Pts',(29.6249423002017,-36.0838268160451,20.));
#71563=CARTESIAN_POINT('Ctrl Pts',(29.5976586669748,-36.1023652282957,0.));
#71564=CARTESIAN_POINT('Ctrl Pts',(29.5976586669748,-36.1023652282957,20.));
#71565=CARTESIAN_POINT('Ctrl Pts',(29.5703629191022,-36.1208838099461,0.));
#71566=CARTESIAN_POINT('Ctrl Pts',(29.5703629191022,-36.1208838099461,20.));
#71567=CARTESIAN_POINT('Ctrl Pts',(29.5430550705937,-36.1393825525541,0.));
#71568=CARTESIAN_POINT('Ctrl Pts',(29.5430550705937,-36.1393825525541,20.));
#71569=CARTESIAN_POINT('Ctrl Pts',(29.5157351354651,-36.1578614476865,0.));
#71570=CARTESIAN_POINT('Ctrl Pts',(29.5157351354651,-36.1578614476865,20.));
#71571=CARTESIAN_POINT('Ctrl Pts',(29.4884031277381,-36.1763204869193,0.));
#71572=CARTESIAN_POINT('Ctrl Pts',(29.4884031277381,-36.1763204869193,20.));
#71573=CARTESIAN_POINT('Ctrl Pts',(29.4610590614411,-36.1947596618382,0.));
#71574=CARTESIAN_POINT('Ctrl Pts',(29.4610590614411,-36.1947596618382,20.));
#71575=CARTESIAN_POINT('Ctrl Pts',(29.4337029506094,-36.2131789640397,0.));
#71576=CARTESIAN_POINT('Ctrl Pts',(29.4337029506094,-36.2131789640397,20.));
#71577=CARTESIAN_POINT('Ctrl Pts',(29.4063348092849,-36.2315783851295,0.));
#71578=CARTESIAN_POINT('Ctrl Pts',(29.4063348092849,-36.2315783851295,20.));
#71579=CARTESIAN_POINT('Ctrl Pts',(29.3789546515147,-36.2499579167227,0.));
#71580=CARTESIAN_POINT('Ctrl Pts',(29.3789546515147,-36.2499579167227,20.));
#71581=CARTESIAN_POINT('Ctrl Pts',(29.3515624913523,-36.2683175504441,0.));
#71582=CARTESIAN_POINT('Ctrl Pts',(29.3515624913523,-36.2683175504441,20.));
#71583=CARTESIAN_POINT('Ctrl Pts',(29.3241583428569,-36.286657277928,0.));
#71584=CARTESIAN_POINT('Ctrl Pts',(29.3241583428569,-36.286657277928,20.));
#71585=CARTESIAN_POINT('Ctrl Pts',(29.2967422200943,-36.3049770908188,0.));
#71586=CARTESIAN_POINT('Ctrl Pts',(29.2967422200943,-36.3049770908188,20.));
#71587=CARTESIAN_POINT('Ctrl Pts',(29.2693141371364,-36.3232769807701,0.));
#71588=CARTESIAN_POINT('Ctrl Pts',(29.2693141371364,-36.3232769807701,20.));
#71589=CARTESIAN_POINT('Ctrl Pts',(29.241874108062,-36.3415569394456,0.));
#71590=CARTESIAN_POINT('Ctrl Pts',(29.241874108062,-36.3415569394456,20.));
#71591=CARTESIAN_POINT('Ctrl Pts',(29.2144221469562,-36.3598169585187,0.));
#71592=CARTESIAN_POINT('Ctrl Pts',(29.2144221469562,-36.3598169585187,20.));
#71593=CARTESIAN_POINT('Ctrl Pts',(29.186958267911,-36.3780570296726,0.));
#71594=CARTESIAN_POINT('Ctrl Pts',(29.186958267911,-36.3780570296726,20.));
#71595=CARTESIAN_POINT('Ctrl Pts',(29.1594824850239,-36.3962771446002,0.));
#71596=CARTESIAN_POINT('Ctrl Pts',(29.1594824850239,-36.3962771446002,20.));
#71597=CARTESIAN_POINT('Ctrl Pts',(29.1319948123985,-36.4144772950043,0.));
#71598=CARTESIAN_POINT('Ctrl Pts',(29.1319948123985,-36.4144772950043,20.));
#71599=CARTESIAN_POINT('Ctrl Pts',(29.1044952641442,-36.4326574725969,0.));
#71600=CARTESIAN_POINT('Ctrl Pts',(29.1044952641442,-36.4326574725969,20.));
#71601=CARTESIAN_POINT('Ctrl Pts',(29.0769838543763,-36.4508176690994,0.));
#71602=CARTESIAN_POINT('Ctrl Pts',(29.0769838543763,-36.4508176690994,20.));
#71603=CARTESIAN_POINT('Ctrl Pts',(29.0494605972165,-36.4689578762435,0.));
#71604=CARTESIAN_POINT('Ctrl Pts',(29.0494605972165,-36.4689578762435,20.));
#71605=CARTESIAN_POINT('Ctrl Pts',(29.0219255067927,-36.4870780857703,0.));
#71606=CARTESIAN_POINT('Ctrl Pts',(29.0219255067927,-36.4870780857703,20.));
#71607=CARTESIAN_POINT('Ctrl Pts',(28.99437859724,-36.5051782894317,0.));
#71608=CARTESIAN_POINT('Ctrl Pts',(28.99437859724,-36.5051782894317,20.));
#71609=CARTESIAN_POINT('Ctrl Pts',(28.9668198826995,-36.5232584789886,0.));
#71610=CARTESIAN_POINT('Ctrl Pts',(28.9668198826995,-36.5232584789886,20.));
#71611=CARTESIAN_POINT('Ctrl Pts',(28.9392493773185,-36.5413186462123,0.));
#71612=CARTESIAN_POINT('Ctrl Pts',(28.9392493773185,-36.5413186462123,20.));
#71613=CARTESIAN_POINT('Ctrl Pts',(28.9116670952497,-36.5593587828826,0.));
#71614=CARTESIAN_POINT('Ctrl Pts',(28.9116670952497,-36.5593587828826,20.));
#71615=CARTESIAN_POINT('Ctrl Pts',(28.8840730506515,-36.577378880789,0.));
#71616=CARTESIAN_POINT('Ctrl Pts',(28.8840730506515,-36.577378880789,20.));
#71617=CARTESIAN_POINT('Ctrl Pts',(28.8564672576885,-36.5953789317306,0.));
#71618=CARTESIAN_POINT('Ctrl Pts',(28.8564672576885,-36.5953789317306,20.));
#71619=CARTESIAN_POINT('Ctrl Pts',(28.8288497305324,-36.6133589275174,0.));
#71620=CARTESIAN_POINT('Ctrl Pts',(28.8288497305324,-36.6133589275174,20.));
#71621=CARTESIAN_POINT('Ctrl Pts',(28.8012204833609,-36.6313188599694,0.));
#71622=CARTESIAN_POINT('Ctrl Pts',(28.8012204833609,-36.6313188599694,20.));
#71623=CARTESIAN_POINT('Ctrl Pts',(28.7735795303585,-36.6492587209168,0.));
#71624=CARTESIAN_POINT('Ctrl Pts',(28.7735795303585,-36.6492587209168,20.));
#71625=CARTESIAN_POINT('Ctrl Pts',(28.7459268857152,-36.6671785021988,0.));
#71626=CARTESIAN_POINT('Ctrl Pts',(28.7459268857152,-36.6671785021988,20.));
#71627=CARTESIAN_POINT('Ctrl Pts',(28.7182625636274,-36.6850781956649,0.));
#71628=CARTESIAN_POINT('Ctrl Pts',(28.7182625636274,-36.6850781956649,20.));
#71629=CARTESIAN_POINT('Ctrl Pts',(28.6905865782966,-36.7029577931733,0.));
#71630=CARTESIAN_POINT('Ctrl Pts',(28.6905865782966,-36.7029577931733,20.));
#71631=CARTESIAN_POINT('Ctrl Pts',(28.6628989439305,-36.7208172865919,0.));
#71632=CARTESIAN_POINT('Ctrl Pts',(28.6628989439305,-36.7208172865919,20.));
#71633=CARTESIAN_POINT('Ctrl Pts',(28.6351996747428,-36.7386566677981,0.));
#71634=CARTESIAN_POINT('Ctrl Pts',(28.6351996747428,-36.7386566677981,20.));
#71635=CARTESIAN_POINT('Ctrl Pts',(28.6074887849535,-36.7564759286795,0.));
#71636=CARTESIAN_POINT('Ctrl Pts',(28.6074887849535,-36.7564759286795,20.));
#71637=CARTESIAN_POINT('Ctrl Pts',(28.5797662887891,-36.774275061134,0.));
#71638=CARTESIAN_POINT('Ctrl Pts',(28.5797662887891,-36.774275061134,20.));
#71639=CARTESIAN_POINT('Ctrl Pts',(28.5520322004824,-36.7920540570698,0.));
#71640=CARTESIAN_POINT('Ctrl Pts',(28.5520322004824,-36.7920540570698,20.));
#71641=CARTESIAN_POINT('Ctrl Pts',(28.5242865342724,-36.8098129084051,0.));
#71642=CARTESIAN_POINT('Ctrl Pts',(28.5242865342724,-36.8098129084051,20.));
#71643=CARTESIAN_POINT('Ctrl Pts',(28.496529304404,-36.8275516070676,0.));
#71644=CARTESIAN_POINT('Ctrl Pts',(28.496529304404,-36.8275516070676,20.));
#71645=CARTESIAN_POINT('Ctrl Pts',(28.4687605251277,-36.8452701449948,0.));
#71646=CARTESIAN_POINT('Ctrl Pts',(28.4687605251277,-36.8452701449948,20.));
#71647=CARTESIAN_POINT('Ctrl Pts',(28.4409802107002,-36.8629685141338,0.));
#71648=CARTESIAN_POINT('Ctrl Pts',(28.4409802107002,-36.8629685141338,20.));
#71649=CARTESIAN_POINT('Ctrl Pts',(28.413188375384,-36.8806467064409,0.));
#71650=CARTESIAN_POINT('Ctrl Pts',(28.413188375384,-36.8806467064409,20.));
#71651=CARTESIAN_POINT('Ctrl Pts',(28.3853850334475,-36.8983047138822,0.));
#71652=CARTESIAN_POINT('Ctrl Pts',(28.3853850334475,-36.8983047138822,20.));
#71653=CARTESIAN_POINT('Ctrl Pts',(28.3575701991656,-36.9159425284342,0.));
#71654=CARTESIAN_POINT('Ctrl Pts',(28.3575701991656,-36.9159425284342,20.));
#71655=CARTESIAN_POINT('Ctrl Pts',(28.3297438868192,-36.9335601420835,0.));
#71656=CARTESIAN_POINT('Ctrl Pts',(28.3297438868192,-36.9335601420835,20.));
#71657=CARTESIAN_POINT('Ctrl Pts',(28.3019061106957,-36.9511575468269,0.));
#71658=CARTESIAN_POINT('Ctrl Pts',(28.3019061106957,-36.9511575468269,20.));
#71659=CARTESIAN_POINT('Ctrl Pts',(28.2740568850881,-36.968734734671,0.));
#71660=CARTESIAN_POINT('Ctrl Pts',(28.2740568850881,-36.968734734671,20.));
#71661=CARTESIAN_POINT('Ctrl Pts',(28.2461962242955,-36.9862916976318,0.));
#71662=CARTESIAN_POINT('Ctrl Pts',(28.2461962242955,-36.9862916976318,20.));
#71663=CARTESIAN_POINT('Ctrl Pts',(28.2183241426219,-37.0038284277349,0.));
#71664=CARTESIAN_POINT('Ctrl Pts',(28.2183241426219,-37.0038284277349,20.));
#71665=CARTESIAN_POINT('Ctrl Pts',(28.1904406543778,-37.0213449170157,0.));
#71666=CARTESIAN_POINT('Ctrl Pts',(28.1904406543778,-37.0213449170157,20.));
#71667=CARTESIAN_POINT('Ctrl Pts',(28.1625457738797,-37.0388411575197,0.));
#71668=CARTESIAN_POINT('Ctrl Pts',(28.1625457738797,-37.0388411575197,20.));
#71669=CARTESIAN_POINT('Ctrl Pts',(28.1346395154506,-37.0563171413026,0.));
#71670=CARTESIAN_POINT('Ctrl Pts',(28.1346395154506,-37.0563171413026,20.));
#71671=CARTESIAN_POINT('Ctrl Pts',(28.1067218934195,-37.0737728604298,0.));
#71672=CARTESIAN_POINT('Ctrl Pts',(28.1067218934195,-37.0737728604298,20.));
#71673=CARTESIAN_POINT('Ctrl Pts',(28.0787929221219,-37.0912083069772,0.));
#71674=CARTESIAN_POINT('Ctrl Pts',(28.0787929221219,-37.0912083069772,20.));
#71675=CARTESIAN_POINT('Ctrl Pts',(28.0508526158994,-37.1086234730312,0.));
#71676=CARTESIAN_POINT('Ctrl Pts',(28.0508526158994,-37.1086234730312,20.));
#71677=CARTESIAN_POINT('Ctrl Pts',(28.0229009890985,-37.1260183506872,0.));
#71678=CARTESIAN_POINT('Ctrl Pts',(28.0229009890985,-37.1260183506872,20.));
#71679=CARTESIAN_POINT('Ctrl Pts',(27.994938056072,-37.1433929320507,0.));
#71680=CARTESIAN_POINT('Ctrl Pts',(27.994938056072,-37.1433929320507,20.));
#71681=CARTESIAN_POINT('Ctrl Pts',(27.9669638311771,-37.1607472092352,0.));
#71682=CARTESIAN_POINT('Ctrl Pts',(27.9669638311771,-37.1607472092352,20.));
#71683=CARTESIAN_POINT('Ctrl Pts',(27.9389783287777,-37.1780811743652,0.));
#71684=CARTESIAN_POINT('Ctrl Pts',(27.9389783287777,-37.1780811743652,20.));
#71685=CARTESIAN_POINT('Ctrl Pts',(27.9109815632437,-37.1953948195748,0.));
#71686=CARTESIAN_POINT('Ctrl Pts',(27.9109815632437,-37.1953948195748,20.));
#71687=CARTESIAN_POINT('Ctrl Pts',(27.8829735489517,-37.2126881370093,0.));
#71688=CARTESIAN_POINT('Ctrl Pts',(27.8829735489517,-37.2126881370093,20.));
#71689=CARTESIAN_POINT('Ctrl Pts',(27.8549543002843,-37.2299611188238,0.));
#71690=CARTESIAN_POINT('Ctrl Pts',(27.8549543002843,-37.2299611188238,20.));
#71691=CARTESIAN_POINT('Ctrl Pts',(27.8269238316305,-37.2472137571842,0.));
#71692=CARTESIAN_POINT('Ctrl Pts',(27.8269238316305,-37.2472137571842,20.));
#71693=CARTESIAN_POINT('Ctrl Pts',(27.7988821573846,-37.2644460442654,0.));
#71694=CARTESIAN_POINT('Ctrl Pts',(27.7988821573846,-37.2644460442654,20.));
#71695=CARTESIAN_POINT('Ctrl Pts',(27.7708292919468,-37.2816579722525,0.));
#71696=CARTESIAN_POINT('Ctrl Pts',(27.7708292919468,-37.2816579722525,20.));
#71697=CARTESIAN_POINT('Ctrl Pts',(27.7427652497224,-37.2988495333397,0.));
#71698=CARTESIAN_POINT('Ctrl Pts',(27.7427652497224,-37.2988495333397,20.));
#71699=CARTESIAN_POINT('Ctrl Pts',(27.7146900451228,-37.3160207197314,0.));
#71700=CARTESIAN_POINT('Ctrl Pts',(27.7146900451228,-37.3160207197314,20.));
#71701=CARTESIAN_POINT('Ctrl Pts',(27.6866036925651,-37.3331715236414,0.));
#71702=CARTESIAN_POINT('Ctrl Pts',(27.6866036925651,-37.3331715236414,20.));
#71703=CARTESIAN_POINT('Ctrl Pts',(27.6585062064726,-37.3503019372939,0.));
#71704=CARTESIAN_POINT('Ctrl Pts',(27.6585062064726,-37.3503019372939,20.));
#71705=CARTESIAN_POINT('Ctrl Pts',(27.6303976012744,-37.3674119529234,0.));
#71706=CARTESIAN_POINT('Ctrl Pts',(27.6303976012744,-37.3674119529234,20.));
#71707=CARTESIAN_POINT('Ctrl Pts',(27.6022778914064,-37.384501562775,0.));
#71708=CARTESIAN_POINT('Ctrl Pts',(27.6022778914064,-37.384501562775,20.));
#71709=CARTESIAN_POINT('Ctrl Pts',(27.5741470913094,-37.4015707591036,0.));
#71710=CARTESIAN_POINT('Ctrl Pts',(27.5741470913094,-37.4015707591036,20.));
#71711=CARTESIAN_POINT('Ctrl Pts',(27.5460052154308,-37.4186195341741,0.));
#71712=CARTESIAN_POINT('Ctrl Pts',(27.5460052154308,-37.4186195341741,20.));
#71713=CARTESIAN_POINT('Ctrl Pts',(27.5178522782226,-37.4356478802604,0.));
#71714=CARTESIAN_POINT('Ctrl Pts',(27.5178522782226,-37.4356478802604,20.));
#71715=CARTESIAN_POINT('Ctrl Pts',(27.4896882941429,-37.4526557896465,0.));
#71716=CARTESIAN_POINT('Ctrl Pts',(27.4896882941429,-37.4526557896465,20.));
#71717=CARTESIAN_POINT('Ctrl Pts',(27.4615132776558,-37.4696432546267,0.));
#71718=CARTESIAN_POINT('Ctrl Pts',(27.4615132776558,-37.4696432546267,20.));
#71719=CARTESIAN_POINT('Ctrl Pts',(27.4333272432311,-37.4866102675048,0.));
#71720=CARTESIAN_POINT('Ctrl Pts',(27.4333272432311,-37.4866102675048,20.));
#71721=CARTESIAN_POINT('Ctrl Pts',(27.4051302053449,-37.5035568205959,0.));
#71722=CARTESIAN_POINT('Ctrl Pts',(27.4051302053449,-37.5035568205959,20.));
#71723=CARTESIAN_POINT('Ctrl Pts',(27.3769221784798,-37.5204829062256,0.));
#71724=CARTESIAN_POINT('Ctrl Pts',(27.3769221784798,-37.5204829062256,20.));
#71725=CARTESIAN_POINT('Ctrl Pts',(27.3487031771241,-37.5373885167297,0.));
#71726=CARTESIAN_POINT('Ctrl Pts',(27.3487031771241,-37.5373885167297,20.));
#71727=CARTESIAN_POINT('Ctrl Pts',(27.3204732157704,-37.5542736444521,0.));
#71728=CARTESIAN_POINT('Ctrl Pts',(27.3204732157704,-37.5542736444521,20.));
#71729=CARTESIAN_POINT('Ctrl Pts',(27.2922323089174,-37.571138281747,0.));
#71730=CARTESIAN_POINT('Ctrl Pts',(27.2922323089174,-37.571138281747,20.));
#71731=CARTESIAN_POINT('Ctrl Pts',(27.2639804710687,-37.5879824209777,0.));
#71732=CARTESIAN_POINT('Ctrl Pts',(27.2639804710687,-37.5879824209777,20.));
#71733=CARTESIAN_POINT('Ctrl Pts',(27.2357177167352,-37.6048060545189,0.));
#71734=CARTESIAN_POINT('Ctrl Pts',(27.2357177167352,-37.6048060545189,20.));
#71735=CARTESIAN_POINT('Ctrl Pts',(27.2074440604332,-37.6216091747552,0.));
#71736=CARTESIAN_POINT('Ctrl Pts',(27.2074440604332,-37.6216091747552,20.));
#71737=CARTESIAN_POINT('Ctrl Pts',(27.1791595166855,-37.6383917740821,0.));
#71738=CARTESIAN_POINT('Ctrl Pts',(27.1791595166855,-37.6383917740821,20.));
#71739=CARTESIAN_POINT('Ctrl Pts',(27.15086410002,-37.6551538449046,0.));
#71740=CARTESIAN_POINT('Ctrl Pts',(27.15086410002,-37.6551538449046,20.));
#71741=CARTESIAN_POINT('Ctrl Pts',(27.1225578249702,-37.6718953796384,0.));
#71742=CARTESIAN_POINT('Ctrl Pts',(27.1225578249702,-37.6718953796384,20.));
#71743=CARTESIAN_POINT('Ctrl Pts',(27.0942407060752,-37.6886163707084,0.));
#71744=CARTESIAN_POINT('Ctrl Pts',(27.0942407060752,-37.6886163707084,20.));
#71745=CARTESIAN_POINT('Ctrl Pts',(27.0659127578793,-37.705316810549,0.));
#71746=CARTESIAN_POINT('Ctrl Pts',(27.0659127578793,-37.705316810549,20.));
#71747=CARTESIAN_POINT('Ctrl Pts',(27.0375739949332,-37.7219966916053,0.));
#71748=CARTESIAN_POINT('Ctrl Pts',(27.0375739949332,-37.7219966916053,20.));
#71749=CARTESIAN_POINT('Ctrl Pts',(27.0092244317933,-37.7386560063324,0.));
#71750=CARTESIAN_POINT('Ctrl Pts',(27.0092244317933,-37.7386560063324,20.));
#71751=CARTESIAN_POINT('Ctrl Pts',(26.9808640830224,-37.755294747196,0.));
#71752=CARTESIAN_POINT('Ctrl Pts',(26.9808640830224,-37.755294747196,20.));
#71753=CARTESIAN_POINT('Ctrl Pts',(26.9524929631885,-37.7719129066716,0.));
#71754=CARTESIAN_POINT('Ctrl Pts',(26.9524929631885,-37.7719129066716,20.));
#71755=CARTESIAN_POINT('Ctrl Pts',(26.9241110868652,-37.7885104772446,0.));
#71756=CARTESIAN_POINT('Ctrl Pts',(26.9241110868652,-37.7885104772446,20.));
#71757=CARTESIAN_POINT('Ctrl Pts',(26.8957184686315,-37.8050874514106,0.));
#71758=CARTESIAN_POINT('Ctrl Pts',(26.8957184686315,-37.8050874514106,20.));
#71759=CARTESIAN_POINT('Ctrl Pts',(26.8673151230714,-37.8216438216745,0.));
#71760=CARTESIAN_POINT('Ctrl Pts',(26.8673151230714,-37.8216438216745,20.));
#71761=CARTESIAN_POINT('Ctrl Pts',(26.8389010647754,-37.8381795805523,0.));
#71762=CARTESIAN_POINT('Ctrl Pts',(26.8389010647754,-37.8381795805523,20.));
#71763=CARTESIAN_POINT('Ctrl Pts',(26.8104763083398,-37.8546947205707,0.));
#71764=CARTESIAN_POINT('Ctrl Pts',(26.8104763083398,-37.8546947205707,20.));
#71765=CARTESIAN_POINT('Ctrl Pts',(26.7820408683669,-37.8711892342661,0.));
#71766=CARTESIAN_POINT('Ctrl Pts',(26.7820408683669,-37.8711892342661,20.));
#71767=CARTESIAN_POINT('Ctrl Pts',(26.7535947594648,-37.887663114185,0.));
#71768=CARTESIAN_POINT('Ctrl Pts',(26.7535947594648,-37.887663114185,20.));
#71769=CARTESIAN_POINT('Ctrl Pts',(26.7251379962461,-37.904116352883,0.));
#71770=CARTESIAN_POINT('Ctrl Pts',(26.7251379962461,-37.904116352883,20.));
#71771=CARTESIAN_POINT('Ctrl Pts',(26.6966705933291,-37.9205489429259,0.));
#71772=CARTESIAN_POINT('Ctrl Pts',(26.6966705933291,-37.9205489429259,20.));
#71773=CARTESIAN_POINT('Ctrl Pts',(26.6681925653377,-37.9369608768897,0.));
#71774=CARTESIAN_POINT('Ctrl Pts',(26.6681925653377,-37.9369608768897,20.));
#71775=CARTESIAN_POINT('Ctrl Pts',(26.6397039269022,-37.9533521473617,0.));
#71776=CARTESIAN_POINT('Ctrl Pts',(26.6397039269022,-37.9533521473617,20.));
#71777=CARTESIAN_POINT('Ctrl Pts',(26.6112046926582,-37.9697227469389,0.));
#71778=CARTESIAN_POINT('Ctrl Pts',(26.6112046926582,-37.9697227469389,20.));
#71779=CARTESIAN_POINT('Ctrl Pts',(26.5826948772471,-37.9860726682287,0.));
#71780=CARTESIAN_POINT('Ctrl Pts',(26.5826948772471,-37.9860726682287,20.));
#71781=CARTESIAN_POINT('Ctrl Pts',(26.5541744953162,-38.0024019038486,0.));
#71782=CARTESIAN_POINT('Ctrl Pts',(26.5541744953162,-38.0024019038486,20.));
#71783=CARTESIAN_POINT('Ctrl Pts',(26.5256435615177,-38.0187104464255,0.));
#71784=CARTESIAN_POINT('Ctrl Pts',(26.5256435615177,-38.0187104464255,20.));
#71785=CARTESIAN_POINT('Ctrl Pts',(26.4971020905092,-38.0349982885963,0.));
#71786=CARTESIAN_POINT('Ctrl Pts',(26.4971020905092,-38.0349982885963,20.));
#71787=CARTESIAN_POINT('Ctrl Pts',(26.4685500969542,-38.0512654230086,0.));
#71788=CARTESIAN_POINT('Ctrl Pts',(26.4685500969542,-38.0512654230086,20.));
#71789=CARTESIAN_POINT('Ctrl Pts',(26.4399875955219,-38.0675118423201,0.));
#71790=CARTESIAN_POINT('Ctrl Pts',(26.4399875955219,-38.0675118423201,20.));
#71791=CARTESIAN_POINT('Ctrl Pts',(26.4114146008872,-38.0837375391992,0.));
#71792=CARTESIAN_POINT('Ctrl Pts',(26.4114146008872,-38.0837375391992,20.));
#71793=CARTESIAN_POINT('Ctrl Pts',(26.38283112773,-38.0999425063245,0.));
#71794=CARTESIAN_POINT('Ctrl Pts',(26.38283112773,-38.0999425063245,20.));
#71795=CARTESIAN_POINT('Ctrl Pts',(26.3542371907363,-38.1161267363846,0.));
#71796=CARTESIAN_POINT('Ctrl Pts',(26.3542371907363,-38.1161267363846,20.));
#71797=CARTESIAN_POINT('Ctrl Pts',(26.3256328045975,-38.1322902220784,0.));
#71798=CARTESIAN_POINT('Ctrl Pts',(26.3256328045975,-38.1322902220784,20.));
#71799=CARTESIAN_POINT('Ctrl Pts',(26.2970179840108,-38.1484329561142,0.));
#71800=CARTESIAN_POINT('Ctrl Pts',(26.2970179840108,-38.1484329561142,20.));
#71801=CARTESIAN_POINT('Ctrl Pts',(26.2683927436784,-38.1645549312104,0.));
#71802=CARTESIAN_POINT('Ctrl Pts',(26.2683927436784,-38.1645549312104,20.));
#71803=CARTESIAN_POINT('Ctrl Pts',(26.2397570983077,-38.1806561400953,0.));
#71804=CARTESIAN_POINT('Ctrl Pts',(26.2397570983077,-38.1806561400953,20.));
#71805=CARTESIAN_POINT('Ctrl Pts',(26.2111110626121,-38.1967365755081,0.));
#71806=CARTESIAN_POINT('Ctrl Pts',(26.2111110626121,-38.1967365755081,20.));
#71807=CARTESIAN_POINT('Ctrl Pts',(26.1824546513102,-38.2127962301983,0.));
#71808=CARTESIAN_POINT('Ctrl Pts',(26.1824546513102,-38.2127962301983,20.));
#71809=CARTESIAN_POINT('Ctrl Pts',(26.1537878791271,-38.2288350969267,0.));
#71810=CARTESIAN_POINT('Ctrl Pts',(26.1537878791271,-38.2288350969267,20.));
#71811=CARTESIAN_POINT('Ctrl Pts',(26.1251107607929,-38.244853168464,0.));
#71812=CARTESIAN_POINT('Ctrl Pts',(26.1251107607929,-38.244853168464,20.));
#71813=CARTESIAN_POINT('Ctrl Pts',(26.0964233110434,-38.2608504375907,0.));
#71814=CARTESIAN_POINT('Ctrl Pts',(26.0964233110434,-38.2608504375907,20.));
#71815=CARTESIAN_POINT('Ctrl Pts',(26.0677255446196,-38.276826897097,0.));
#71816=CARTESIAN_POINT('Ctrl Pts',(26.0677255446196,-38.276826897097,20.));
#71817=CARTESIAN_POINT('Ctrl Pts',(26.0390174762675,-38.2927825397833,0.));
#71818=CARTESIAN_POINT('Ctrl Pts',(26.0390174762675,-38.2927825397833,20.));
#71819=CARTESIAN_POINT('Ctrl Pts',(26.0102991207387,-38.30871735846,0.));
#71820=CARTESIAN_POINT('Ctrl Pts',(26.0102991207387,-38.30871735846,20.));
#71821=CARTESIAN_POINT('Ctrl Pts',(25.9815704927901,-38.3246313459476,0.));
#71822=CARTESIAN_POINT('Ctrl Pts',(25.9815704927901,-38.3246313459476,20.));
#71823=CARTESIAN_POINT('Ctrl Pts',(25.9528316071847,-38.3405244950781,0.));
#71824=CARTESIAN_POINT('Ctrl Pts',(25.9528316071847,-38.3405244950781,20.));
#71825=CARTESIAN_POINT('Ctrl Pts',(25.9240824786908,-38.3563967986932,0.));
#71826=CARTESIAN_POINT('Ctrl Pts',(25.9240824786908,-38.3563967986932,20.));
#71827=CARTESIAN_POINT('Ctrl Pts',(25.8953231220827,-38.3722482496454,0.));
#71828=CARTESIAN_POINT('Ctrl Pts',(25.8953231220827,-38.3722482496454,20.));
#71829=CARTESIAN_POINT('Ctrl Pts',(25.8665535521392,-38.3880788407969,0.));
#71830=CARTESIAN_POINT('Ctrl Pts',(25.8665535521392,-38.3880788407969,20.));
#71831=CARTESIAN_POINT('Ctrl Pts',(25.8377737836446,-38.4038885650199,0.));
#71832=CARTESIAN_POINT('Ctrl Pts',(25.8377737836446,-38.4038885650199,20.));
#71833=CARTESIAN_POINT('Ctrl Pts',(25.8089838313888,-38.419677415197,0.));
#71834=CARTESIAN_POINT('Ctrl Pts',(25.8089838313888,-38.419677415197,20.));
#71835=CARTESIAN_POINT('Ctrl Pts',(25.7801837101667,-38.4354453842206,0.));
#71836=CARTESIAN_POINT('Ctrl Pts',(25.7801837101667,-38.4354453842206,20.));
#71837=CARTESIAN_POINT('Ctrl Pts',(25.7513734347795,-38.4511924649945,0.));
#71838=CARTESIAN_POINT('Ctrl Pts',(25.7513734347795,-38.4511924649945,20.));
#71839=CARTESIAN_POINT('Ctrl Pts',(25.7225530200331,-38.4669186504318,0.));
#71840=CARTESIAN_POINT('Ctrl Pts',(25.7225530200331,-38.4669186504318,20.));
#71841=CARTESIAN_POINT('Ctrl Pts',(25.6937224807392,-38.4826239334567,0.));
#71842=CARTESIAN_POINT('Ctrl Pts',(25.6937224807392,-38.4826239334567,20.));
#71843=CARTESIAN_POINT('Ctrl Pts',(25.6648818317151,-38.4983083070042,0.));
#71844=CARTESIAN_POINT('Ctrl Pts',(25.6648818317151,-38.4983083070042,20.));
#71845=CARTESIAN_POINT('Ctrl Pts',(25.6360310877836,-38.5139717640192,0.));
#71846=CARTESIAN_POINT('Ctrl Pts',(25.6360310877836,-38.5139717640192,20.));
#71847=CARTESIAN_POINT('Ctrl Pts',(25.6071702637723,-38.5296142974561,0.));
#71848=CARTESIAN_POINT('Ctrl Pts',(25.6071702637723,-38.5296142974561,20.));
#71849=CARTESIAN_POINT('Ctrl Pts',(25.5782993745137,-38.5452359002793,0.));
#71850=CARTESIAN_POINT('Ctrl Pts',(25.5782993745137,-38.5452359002793,20.));
#71851=CARTESIAN_POINT('Ctrl Pts',(25.5494184348456,-38.5608365654634,0.));
#71852=CARTESIAN_POINT('Ctrl Pts',(25.5494184348456,-38.5608365654634,20.));
#71853=CARTESIAN_POINT('Ctrl Pts',(25.5205274596115,-38.576416285994,0.));
#71854=CARTESIAN_POINT('Ctrl Pts',(25.5205274596115,-38.576416285994,20.));
#71855=CARTESIAN_POINT('Ctrl Pts',(25.4916264636604,-38.591975054867,0.));
#71856=CARTESIAN_POINT('Ctrl Pts',(25.4916264636604,-38.591975054867,20.));
#71857=CARTESIAN_POINT('Ctrl Pts',(25.462715461847,-38.6075128650891,0.));
#71858=CARTESIAN_POINT('Ctrl Pts',(25.462715461847,-38.6075128650891,20.));
#71859=CARTESIAN_POINT('Ctrl Pts',(25.4337944690316,-38.6230297096774,0.));
#71860=CARTESIAN_POINT('Ctrl Pts',(25.4337944690316,-38.6230297096774,20.));
#71861=CARTESIAN_POINT('Ctrl Pts',(25.4048635000794,-38.6385255816593,0.));
#71862=CARTESIAN_POINT('Ctrl Pts',(25.4048635000794,-38.6385255816593,20.));
#71863=CARTESIAN_POINT('Ctrl Pts',(25.3759225698613,-38.6540004740723,0.));
#71864=CARTESIAN_POINT('Ctrl Pts',(25.3759225698613,-38.6540004740723,20.));
#71865=CARTESIAN_POINT('Ctrl Pts',(25.3469716932528,-38.6694543799641,0.));
#71866=CARTESIAN_POINT('Ctrl Pts',(25.3469716932528,-38.6694543799641,20.));
#71867=CARTESIAN_POINT('Ctrl Pts',(25.318010885134,-38.6848872923919,0.));
#71868=CARTESIAN_POINT('Ctrl Pts',(25.318010885134,-38.6848872923919,20.));
#71869=CARTESIAN_POINT('Ctrl Pts',(25.2890401603912,-38.7002992044242,0.));
#71870=CARTESIAN_POINT('Ctrl Pts',(25.2890401603912,-38.7002992044242,20.));
#71871=CARTESIAN_POINT('Ctrl Pts',(25.2600595339159,-38.7156901091392,0.));
#71872=CARTESIAN_POINT('Ctrl Pts',(25.2600595339159,-38.7156901091392,20.));
#71873=CARTESIAN_POINT('Ctrl Pts',(25.2310690206049,-38.7310599996258,0.));
#71874=CARTESIAN_POINT('Ctrl Pts',(25.2310690206049,-38.7310599996258,20.));
#71875=CARTESIAN_POINT('Ctrl Pts',(25.2020686353608,-38.7464088689837,0.));
#71876=CARTESIAN_POINT('Ctrl Pts',(25.2020686353608,-38.7464088689837,20.));
#71877=CARTESIAN_POINT('Ctrl Pts',(25.1730583930911,-38.7617367103229,0.));
#71878=CARTESIAN_POINT('Ctrl Pts',(25.1730583930911,-38.7617367103229,20.));
#71879=CARTESIAN_POINT('Ctrl Pts',(25.1440383087084,-38.7770435167639,0.));
#71880=CARTESIAN_POINT('Ctrl Pts',(25.1440383087084,-38.7770435167639,20.));
#71881=CARTESIAN_POINT('Ctrl Pts',(25.1150083971302,-38.7923292814368,0.));
#71882=CARTESIAN_POINT('Ctrl Pts',(25.1150083971302,-38.7923292814368,20.));
#71883=CARTESIAN_POINT('Ctrl Pts',(25.0859686732794,-38.8075939974829,0.));
#71884=CARTESIAN_POINT('Ctrl Pts',(25.0859686732794,-38.8075939974829,20.));
#71885=CARTESIAN_POINT('Ctrl Pts',(25.0569191520845,-38.8228376580533,0.));
#71886=CARTESIAN_POINT('Ctrl Pts',(25.0569191520845,-38.8228376580533,20.));
#71887=CARTESIAN_POINT('Ctrl Pts',(25.0278598484791,-38.8380602563098,0.));
#71888=CARTESIAN_POINT('Ctrl Pts',(25.0278598484791,-38.8380602563098,20.));
#71889=CARTESIAN_POINT('Ctrl Pts',(24.9987907774025,-38.8532617854245,0.));
#71890=CARTESIAN_POINT('Ctrl Pts',(24.9987907774025,-38.8532617854245,20.));
#71891=CARTESIAN_POINT('Ctrl Pts',(24.9697119537988,-38.8684422385799,0.));
#71892=CARTESIAN_POINT('Ctrl Pts',(24.9697119537988,-38.8684422385799,20.));
#71893=CARTESIAN_POINT('Ctrl Pts',(24.9406233926168,-38.883601608968,0.));
#71894=CARTESIAN_POINT('Ctrl Pts',(24.9406233926168,-38.883601608968,20.));
#71895=CARTESIAN_POINT('Ctrl Pts',(24.9115251088107,-38.8987398897918,0.));
#71896=CARTESIAN_POINT('Ctrl Pts',(24.9115251088107,-38.8987398897918,20.));
#71897=CARTESIAN_POINT('Ctrl Pts',(24.8824171173401,-38.9138570742648,0.));
#71898=CARTESIAN_POINT('Ctrl Pts',(24.8824171173401,-38.9138570742648,20.));
#71899=CARTESIAN_POINT('Ctrl Pts',(24.8532994331703,-38.9289531556118,0.));
#71900=CARTESIAN_POINT('Ctrl Pts',(24.8532994331703,-38.9289531556118,20.));
#71901=CARTESIAN_POINT('Ctrl Pts',(24.8241720712716,-38.9440281270684,0.));
#71902=CARTESIAN_POINT('Ctrl Pts',(24.8241720712716,-38.9440281270684,20.));
#71903=CARTESIAN_POINT('Ctrl Pts',(24.7950350466188,-38.9590819818798,0.));
#71904=CARTESIAN_POINT('Ctrl Pts',(24.7950350466188,-38.9590819818798,20.));
#71905=CARTESIAN_POINT('Ctrl Pts',(24.7658883741919,-38.9741147133012,0.));
#71906=CARTESIAN_POINT('Ctrl Pts',(24.7658883741919,-38.9741147133012,20.));
#71907=CARTESIAN_POINT('Ctrl Pts',(24.736732068976,-38.989126314598,0.));
#71908=CARTESIAN_POINT('Ctrl Pts',(24.736732068976,-38.989126314598,20.));
#71909=CARTESIAN_POINT('Ctrl Pts',(24.7075661459616,-39.0041167790461,0.));
#71910=CARTESIAN_POINT('Ctrl Pts',(24.7075661459616,-39.0041167790461,20.));
#71911=CARTESIAN_POINT('Ctrl Pts',(24.6783906201452,-39.019086099931,0.));
#71912=CARTESIAN_POINT('Ctrl Pts',(24.6783906201452,-39.019086099931,20.));
#71913=CARTESIAN_POINT('Ctrl Pts',(24.6492055065285,-39.0340342705498,0.));
#71914=CARTESIAN_POINT('Ctrl Pts',(24.6492055065285,-39.0340342705498,20.));
#71915=CARTESIAN_POINT('Ctrl Pts',(24.6200108201182,-39.0489612842096,0.));
#71916=CARTESIAN_POINT('Ctrl Pts',(24.6200108201182,-39.0489612842096,20.));
#71917=CARTESIAN_POINT('Ctrl Pts',(24.5908065759258,-39.0638671342286,0.));
#71918=CARTESIAN_POINT('Ctrl Pts',(24.5908065759258,-39.0638671342286,20.));
#71919=CARTESIAN_POINT('Ctrl Pts',(24.5615927889669,-39.0787518139362,0.));
#71920=CARTESIAN_POINT('Ctrl Pts',(24.5615927889669,-39.0787518139362,20.));
#71921=CARTESIAN_POINT('Ctrl Pts',(24.5323694742616,-39.0936153166722,0.));
#71922=CARTESIAN_POINT('Ctrl Pts',(24.5323694742616,-39.0936153166722,20.));
#71923=CARTESIAN_POINT('Ctrl Pts',(24.5031366468345,-39.1084576357872,0.));
#71924=CARTESIAN_POINT('Ctrl Pts',(24.5031366468345,-39.1084576357872,20.));
#71925=CARTESIAN_POINT('Ctrl Pts',(24.4738943217155,-39.1232787646414,0.));
#71926=CARTESIAN_POINT('Ctrl Pts',(24.4738943217155,-39.1232787646414,20.));
#71927=CARTESIAN_POINT('Ctrl Pts',(24.4446425139409,-39.1380786966047,0.));
#71928=CARTESIAN_POINT('Ctrl Pts',(24.4446425139409,-39.1380786966047,20.));
#71929=CARTESIAN_POINT('Ctrl Pts',(24.4153812385543,-39.1528574250569,0.));
#71930=CARTESIAN_POINT('Ctrl Pts',(24.4153812385543,-39.1528574250569,20.));
#71931=CARTESIAN_POINT('Ctrl Pts',(24.3861105106067,-39.1676149433869,0.));
#71932=CARTESIAN_POINT('Ctrl Pts',(24.3861105106067,-39.1676149433869,20.));
#71933=CARTESIAN_POINT('Ctrl Pts',(24.3568303451549,-39.1823512449951,0.));
#71934=CARTESIAN_POINT('Ctrl Pts',(24.3568303451549,-39.1823512449951,20.));
#71935=CARTESIAN_POINT('Ctrl Pts',(24.3275407572587,-39.197066323292,0.));
#71936=CARTESIAN_POINT('Ctrl Pts',(24.3275407572587,-39.197066323292,20.));
#71937=CARTESIAN_POINT('Ctrl Pts',(24.2982417619806,-39.2117601717005,0.));
#71938=CARTESIAN_POINT('Ctrl Pts',(24.2982417619806,-39.2117601717005,20.));
#71939=CARTESIAN_POINT('Ctrl Pts',(24.2689333743822,-39.2264327836562,0.));
#71940=CARTESIAN_POINT('Ctrl Pts',(24.2689333743822,-39.2264327836562,20.));
#71941=CARTESIAN_POINT('Ctrl Pts',(24.239615609526,-39.2410841526078,0.));
#71942=CARTESIAN_POINT('Ctrl Pts',(24.239615609526,-39.2410841526078,20.));
#71943=CARTESIAN_POINT('Ctrl Pts',(24.2102884824784,-39.2557142720138,0.));
#71944=CARTESIAN_POINT('Ctrl Pts',(24.2102884824784,-39.2557142720138,20.));
#71945=CARTESIAN_POINT('Ctrl Pts',(24.1809520083146,-39.2703231353422,0.));
#71946=CARTESIAN_POINT('Ctrl Pts',(24.1809520083146,-39.2703231353422,20.));
#71947=CARTESIAN_POINT('Ctrl Pts',(24.1516062021224,-39.2849107360681,0.));
#71948=CARTESIAN_POINT('Ctrl Pts',(24.1516062021224,-39.2849107360681,20.));
#71949=CARTESIAN_POINT('Ctrl Pts',(24.1222510790066,-39.2994770676712,0.));
#71950=CARTESIAN_POINT('Ctrl Pts',(24.1222510790066,-39.2994770676712,20.));
#71951=CARTESIAN_POINT('Ctrl Pts',(24.0928866540881,-39.3140221236369,0.));
#71952=CARTESIAN_POINT('Ctrl Pts',(24.0928866540881,-39.3140221236369,20.));
#71953=CARTESIAN_POINT('Ctrl Pts',(24.0635129424931,-39.3285458974613,0.));
#71954=CARTESIAN_POINT('Ctrl Pts',(24.0635129424931,-39.3285458974613,20.));
#71955=CARTESIAN_POINT('Ctrl Pts',(24.0341299593437,-39.3430483826555,0.));
#71956=CARTESIAN_POINT('Ctrl Pts',(24.0341299593437,-39.3430483826555,20.));
#71957=CARTESIAN_POINT('Ctrl Pts',(24.0047377197503,-39.3575295727493,0.));
#71958=CARTESIAN_POINT('Ctrl Pts',(24.0047377197503,-39.3575295727493,20.));
#71959=CARTESIAN_POINT('Ctrl Pts',(23.9753362387978,-39.3719894612957,0.));
#71960=CARTESIAN_POINT('Ctrl Pts',(23.9753362387978,-39.3719894612957,20.));
#71961=CARTESIAN_POINT('Ctrl Pts',(23.9459255315518,-39.3864280418676,0.));
#71962=CARTESIAN_POINT('Ctrl Pts',(23.9459255315518,-39.3864280418676,20.));
#71963=CARTESIAN_POINT('Ctrl Pts',(23.9165056130837,-39.4008453080481,0.));
#71964=CARTESIAN_POINT('Ctrl Pts',(23.9165056130837,-39.4008453080481,20.));
#71965=CARTESIAN_POINT('Ctrl Pts',(23.8870764984925,-39.4152412534209,0.));
#71966=CARTESIAN_POINT('Ctrl Pts',(23.8870764984925,-39.4152412534209,20.));
#71967=CARTESIAN_POINT('Ctrl Pts',(23.8576382029237,-39.4296158715627,0.));
#71968=CARTESIAN_POINT('Ctrl Pts',(23.8576382029237,-39.4296158715627,20.));
#71969=CARTESIAN_POINT('Ctrl Pts',(23.8281907416004,-39.4439691560298,0.));
#71970=CARTESIAN_POINT('Ctrl Pts',(23.8281907416004,-39.4439691560298,20.));
#71971=CARTESIAN_POINT('Ctrl Pts',(23.7987341298022,-39.4583011003674,0.));
#71972=CARTESIAN_POINT('Ctrl Pts',(23.7987341298022,-39.4583011003674,20.));
#71973=CARTESIAN_POINT('Ctrl Pts',(23.769268382808,-39.4726116981337,0.));
#71974=CARTESIAN_POINT('Ctrl Pts',(23.769268382808,-39.4726116981337,20.));
#71975=CARTESIAN_POINT('Ctrl Pts',(23.7397935158457,-39.4869009429217,0.));
#71976=CARTESIAN_POINT('Ctrl Pts',(23.7397935158457,-39.4869009429217,20.));
#71977=CARTESIAN_POINT('Ctrl Pts',(23.7103095440476,-39.5011688283778,0.));
#71978=CARTESIAN_POINT('Ctrl Pts',(23.7103095440476,-39.5011688283778,20.));
#71979=CARTESIAN_POINT('Ctrl Pts',(23.6808164823786,-39.5154153482324,0.));
#71980=CARTESIAN_POINT('Ctrl Pts',(23.6808164823786,-39.5154153482324,20.));
#71981=CARTESIAN_POINT('Ctrl Pts',(23.651314345698,-39.5296404962722,0.));
#71982=CARTESIAN_POINT('Ctrl Pts',(23.651314345698,-39.5296404962722,20.));
#71983=CARTESIAN_POINT('Ctrl Pts',(23.6218031488904,-39.5438442662853,0.));
#71984=CARTESIAN_POINT('Ctrl Pts',(23.6218031488904,-39.5438442662853,20.));
#71985=CARTESIAN_POINT('Ctrl Pts',(23.5922829069852,-39.5580266520107,0.));
#71986=CARTESIAN_POINT('Ctrl Pts',(23.5922829069852,-39.5580266520107,20.));
#71987=CARTESIAN_POINT('Ctrl Pts',(23.5627536352592,-39.5721876470956,0.));
#71988=CARTESIAN_POINT('Ctrl Pts',(23.5627536352592,-39.5721876470956,20.));
#71989=CARTESIAN_POINT('Ctrl Pts',(23.5332153494019,-39.5863272450268,0.));
#71990=CARTESIAN_POINT('Ctrl Pts',(23.5332153494019,-39.5863272450268,20.));
#71991=CARTESIAN_POINT('Ctrl Pts',(23.5036680653391,-39.6004454392038,0.));
#71992=CARTESIAN_POINT('Ctrl Pts',(23.5036680653391,-39.6004454392038,20.));
#71993=CARTESIAN_POINT('Ctrl Pts',(23.4741117989348,-39.6145422230651,0.));
#71994=CARTESIAN_POINT('Ctrl Pts',(23.4741117989348,-39.6145422230651,20.));
#71995=CARTESIAN_POINT('Ctrl Pts',(23.4445465657147,-39.6286175902046,0.));
#71996=CARTESIAN_POINT('Ctrl Pts',(23.4445465657147,-39.6286175902046,20.));
#71997=CARTESIAN_POINT('Ctrl Pts',(23.414972380622,-39.6426715344742,0.));
#71998=CARTESIAN_POINT('Ctrl Pts',(23.414972380622,-39.6426715344742,20.));
#71999=CARTESIAN_POINT('Ctrl Pts',(23.385389257652,-39.6567040501382,0.));
#72000=CARTESIAN_POINT('Ctrl Pts',(23.385389257652,-39.6567040501382,20.));
#72001=CARTESIAN_POINT('Ctrl Pts',(23.3557972103217,-39.6707151316771,0.));
#72002=CARTESIAN_POINT('Ctrl Pts',(23.3557972103217,-39.6707151316771,20.));
#72003=CARTESIAN_POINT('Ctrl Pts',(23.3261962523444,-39.6847047735001,0.));
#72004=CARTESIAN_POINT('Ctrl Pts',(23.3261962523444,-39.6847047735001,20.));
#72005=CARTESIAN_POINT('Ctrl Pts',(23.2965863982648,-39.6986729696788,0.));
#72006=CARTESIAN_POINT('Ctrl Pts',(23.2965863982648,-39.6986729696788,20.));
#72007=CARTESIAN_POINT('Ctrl Pts',(23.2669676640418,-39.7126197136991,0.));
#72008=CARTESIAN_POINT('Ctrl Pts',(23.2669676640418,-39.7126197136991,20.));
#72009=CARTESIAN_POINT('Ctrl Pts',(23.2373400678346,-39.7265449981305,0.));
#72010=CARTESIAN_POINT('Ctrl Pts',(23.2373400678346,-39.7265449981305,20.));
#72011=CARTESIAN_POINT('Ctrl Pts',(23.2077036288597,-39.7404488151086,0.));
#72012=CARTESIAN_POINT('Ctrl Pts',(23.2077036288597,-39.7404488151086,20.));
#72013=CARTESIAN_POINT('Ctrl Pts',(23.1780583659508,-39.7543311569459,0.));
#72014=CARTESIAN_POINT('Ctrl Pts',(23.1780583659508,-39.7543311569459,20.));
#72015=CARTESIAN_POINT('Ctrl Pts',(23.1484042962029,-39.7681920167058,0.));
#72016=CARTESIAN_POINT('Ctrl Pts',(23.1484042962029,-39.7681920167058,20.));
#72017=CARTESIAN_POINT('Ctrl Pts',(23.118741433625,-39.7820313887737,0.));
#72018=CARTESIAN_POINT('Ctrl Pts',(23.118741433625,-39.7820313887737,20.));
#72019=CARTESIAN_POINT('Ctrl Pts',(23.089069787673,-39.7958492694787,0.));
#72020=CARTESIAN_POINT('Ctrl Pts',(23.089069787673,-39.7958492694787,20.));
#72021=CARTESIAN_POINT('Ctrl Pts',(23.0593893640427,-39.8096456567259,0.));
#72022=CARTESIAN_POINT('Ctrl Pts',(23.0593893640427,-39.8096456567259,20.));
#72023=CARTESIAN_POINT('Ctrl Pts',(23.0356380053138,-39.8206655709904,0.));
#72024=CARTESIAN_POINT('Ctrl Pts',(23.0356380053138,-39.8206655709904,20.));
#72025=CARTESIAN_POINT('Ctrl Pts',(23.0178205380655,-39.8289208340947,0.));
#72026=CARTESIAN_POINT('Ctrl Pts',(23.0178205380655,-39.8289208340947,20.));
#72027=CARTESIAN_POINT('Ctrl Pts',(23.0059404718139,-39.8344200439082,0.));
#72028=CARTESIAN_POINT('Ctrl Pts',(23.0059404718139,-39.8344200439082,20.));
#72029=CARTESIAN_POINT('Ctrl Pts',(23.,-39.8371685740842,0.));
#72030=CARTESIAN_POINT('Ctrl Pts',(23.,-39.8371685740842,20.));
#72031=CARTESIAN_POINT('',(46.0449384185095,-16.7589870229578,2.));
#72032=CARTESIAN_POINT('Ctrl Pts',(34.5017338047269,-32.2758373034788,2.));
#72033=CARTESIAN_POINT('Ctrl Pts',(35.1012599438994,-31.7409631286146,2.));
#72034=CARTESIAN_POINT('Ctrl Pts',(35.6879267845883,-31.1902015741136,2.));
#72035=CARTESIAN_POINT('Ctrl Pts',(36.260940923753,-30.624221206043,2.));
#72036=CARTESIAN_POINT('Ctrl Pts',(36.8331140520758,-30.0590715253732,2.));
#72037=CARTESIAN_POINT('Ctrl Pts',(37.3916744157871,-29.4787478132684,2.));
#72038=CARTESIAN_POINT('Ctrl Pts',(37.9358682563863,-28.8839535575986,2.));
#72039=CARTESIAN_POINT('Ctrl Pts',(38.4805324906895,-28.2886451699188,2.));
#72040=CARTESIAN_POINT('Ctrl Pts',(39.0108052381929,-27.6788413440332,2.));
#72041=CARTESIAN_POINT('Ctrl Pts',(39.5259687462372,-27.0552833125806,2.));
#72042=CARTESIAN_POINT('Ctrl Pts',(40.0415783150755,-26.4311853655743,2.));
#72043=CARTESIAN_POINT('Ctrl Pts',(40.5420523586309,-25.793309522113,2.));
#72044=CARTESIAN_POINT('Ctrl Pts',(41.0267109660362,-25.1424328771062,2.));
#72045=CARTESIAN_POINT('Ctrl Pts',(41.5120532707873,-24.4906380545866,2.));
#72046=CARTESIAN_POINT('Ctrl Pts',(41.9815353808389,-23.8258058651361,2.));
#72047=CARTESIAN_POINT('Ctrl Pts',(42.4345159310068,-23.1487486269677,2.));
#72048=CARTESIAN_POINT('Ctrl Pts',(42.8878234627796,-22.4712026586269,2.));
#72049=CARTESIAN_POINT('Ctrl Pts',(43.32460550914,-21.7814141347634,2.));
#72050=CARTESIAN_POINT('Ctrl Pts',(43.7442622667776,-21.0802269103741,2.));
#72051=CARTESIAN_POINT('Ctrl Pts',(44.1624443435522,-20.3815036696152,2.));
#72052=CARTESIAN_POINT('Ctrl Pts',(44.5636212234609,-19.671461867878,2.));
#72053=CARTESIAN_POINT('Ctrl Pts',(44.9472430970921,-18.9509636362294,2.));
#72054=CARTESIAN_POINT('Ctrl Pts',(45.1999134416925,-18.47641161251,2.));
#72055=CARTESIAN_POINT('Ctrl Pts',(45.4449691102617,-17.9973240026997,2.));
#72056=CARTESIAN_POINT('Ctrl Pts',(45.6822635680233,-17.5139530963398,2.));
#72057=CARTESIAN_POINT('Ctrl Pts',(45.8052462319505,-17.2634363236775,2.));
#72058=CARTESIAN_POINT('Ctrl Pts',(45.9261440619272,-17.01176962033,2.));
#72059=CARTESIAN_POINT('Ctrl Pts',(46.0449384185095,-16.7589870229578,2.));
#72060=CARTESIAN_POINT('',(46.0449384185095,-16.7589870229578,0.));
#72061=CARTESIAN_POINT('Ctrl Pts',(8.50876070567956,-48.2555798975982,0.));
#72062=CARTESIAN_POINT('Ctrl Pts',(8.50876070567956,-48.2555798975982,20.));
#72063=CARTESIAN_POINT('Ctrl Pts',(8.5020159114628,-48.2561497089132,0.));
#72064=CARTESIAN_POINT('Ctrl Pts',(8.5020159114628,-48.2561497089132,20.));
#72065=CARTESIAN_POINT('Ctrl Pts',(8.48852624368607,-48.2572870022174,0.));
#72066=CARTESIAN_POINT('Ctrl Pts',(8.48852624368607,-48.2572870022174,20.));
#72067=CARTESIAN_POINT('Ctrl Pts',(8.46829150399132,-48.2589859541967,0.));
#72068=CARTESIAN_POINT('Ctrl Pts',(8.46829150399132,-48.2589859541967,20.));
#72069=CARTESIAN_POINT('Ctrl Pts',(8.4413113750042,-48.2612372475269,0.));
#72070=CARTESIAN_POINT('Ctrl Pts',(8.4413113750042,-48.2612372475269,20.));
#72071=CARTESIAN_POINT('Ctrl Pts',(8.40758542125999,-48.2640280707484,0.));
#72072=CARTESIAN_POINT('Ctrl Pts',(8.40758542125999,-48.2640280707484,20.));
#72073=CARTESIAN_POINT('Ctrl Pts',(8.37385867778169,-48.2667956002972,0.));
#72074=CARTESIAN_POINT('Ctrl Pts',(8.37385867778169,-48.2667956002972,20.));
#72075=CARTESIAN_POINT('Ctrl Pts',(8.34013115014496,-48.2695398358687,0.));
#72076=CARTESIAN_POINT('Ctrl Pts',(8.34013115014496,-48.2695398358687,20.));
#72077=CARTESIAN_POINT('Ctrl Pts',(8.30640284761835,-48.2722607770974,0.));
#72078=CARTESIAN_POINT('Ctrl Pts',(8.30640284761835,-48.2722607770974,20.));
#72079=CARTESIAN_POINT('Ctrl Pts',(8.27267378419868,-48.274958423567,0.));
#72080=CARTESIAN_POINT('Ctrl Pts',(8.27267378419868,-48.274958423567,20.));
#72081=CARTESIAN_POINT('Ctrl Pts',(8.23894397736021,-48.2776327748283,0.));
#72082=CARTESIAN_POINT('Ctrl Pts',(8.23894397736021,-48.2776327748283,20.));
#72083=CARTESIAN_POINT('Ctrl Pts',(8.20521344665193,-48.2802838304168,0.));
#72084=CARTESIAN_POINT('Ctrl Pts',(8.20521344665193,-48.2802838304168,20.));
#72085=CARTESIAN_POINT('Ctrl Pts',(8.17148221231953,-48.2829115898716,0.));
#72086=CARTESIAN_POINT('Ctrl Pts',(8.17148221231953,-48.2829115898716,20.));
#72087=CARTESIAN_POINT('Ctrl Pts',(8.13775029398593,-48.2855160527521,0.));
#72088=CARTESIAN_POINT('Ctrl Pts',(8.13775029398593,-48.2855160527521,20.));
#72089=CARTESIAN_POINT('Ctrl Pts',(8.10401770912491,-48.288097218659,0.));
#72090=CARTESIAN_POINT('Ctrl Pts',(8.10401770912491,-48.288097218659,20.));
#72091=CARTESIAN_POINT('Ctrl Pts',(8.07028447346157,-48.2906550872281,0.));
#72092=CARTESIAN_POINT('Ctrl Pts',(8.07028447346157,-48.2906550872281,20.));
#72093=CARTESIAN_POINT('Ctrl Pts',(8.03655060167523,-48.2931896581208,0.));
#72094=CARTESIAN_POINT('Ctrl Pts',(8.03655060167523,-48.2931896581208,20.));
#72095=CARTESIAN_POINT('Ctrl Pts',(8.00281610801472,-48.2957009310153,0.));
#72096=CARTESIAN_POINT('Ctrl Pts',(8.00281610801472,-48.2957009310153,20.));
#72097=CARTESIAN_POINT('Ctrl Pts',(7.96908100690892,-48.2981889055984,0.));
#72098=CARTESIAN_POINT('Ctrl Pts',(7.96908100690892,-48.2981889055984,20.));
#72099=CARTESIAN_POINT('Ctrl Pts',(7.93534531368689,-48.300653581555,0.));
#72100=CARTESIAN_POINT('Ctrl Pts',(7.93534531368689,-48.300653581555,20.));
#72101=CARTESIAN_POINT('Ctrl Pts',(7.90160904447351,-48.3030949585702,0.));
#72102=CARTESIAN_POINT('Ctrl Pts',(7.90160904447351,-48.3030949585702,20.));
#72103=CARTESIAN_POINT('Ctrl Pts',(7.86787221586445,-48.3055130363337,0.));
#72104=CARTESIAN_POINT('Ctrl Pts',(7.86787221586445,-48.3055130363337,20.));
#72105=CARTESIAN_POINT('Ctrl Pts',(7.83413484466693,-48.3079078145432,0.));
#72106=CARTESIAN_POINT('Ctrl Pts',(7.83413484466693,-48.3079078145432,20.));
#72107=CARTESIAN_POINT('Ctrl Pts',(7.80039694763397,-48.3102792929086,0.));
#72108=CARTESIAN_POINT('Ctrl Pts',(7.80039694763397,-48.3102792929086,20.));
#72109=CARTESIAN_POINT('Ctrl Pts',(7.76665854114745,-48.3126274711557,0.));
#72110=CARTESIAN_POINT('Ctrl Pts',(7.76665854114745,-48.3126274711557,20.));
#72111=CARTESIAN_POINT('Ctrl Pts',(7.73291964123288,-48.3149523490266,0.));
#72112=CARTESIAN_POINT('Ctrl Pts',(7.73291964123288,-48.3149523490266,20.));
#72113=CARTESIAN_POINT('Ctrl Pts',(7.69918026370735,-48.3172539262766,0.));
#72114=CARTESIAN_POINT('Ctrl Pts',(7.69918026370735,-48.3172539262766,20.));
#72115=CARTESIAN_POINT('Ctrl Pts',(7.66544042428832,-48.3195322026739,0.));
#72116=CARTESIAN_POINT('Ctrl Pts',(7.66544042428832,-48.3195322026739,20.));
#72117=CARTESIAN_POINT('Ctrl Pts',(7.63170013870892,-48.3217871779975,0.));
#72118=CARTESIAN_POINT('Ctrl Pts',(7.63170013870892,-48.3217871779975,20.));
#72119=CARTESIAN_POINT('Ctrl Pts',(7.59795942285539,-48.3240188520354,0.));
#72120=CARTESIAN_POINT('Ctrl Pts',(7.59795942285539,-48.3240188520354,20.));
#72121=CARTESIAN_POINT('Ctrl Pts',(7.56421829277369,-48.3262272245847,0.));
#72122=CARTESIAN_POINT('Ctrl Pts',(7.56421829277369,-48.3262272245847,20.));
#72123=CARTESIAN_POINT('Ctrl Pts',(7.53047676460326,-48.328412295452,0.));
#72124=CARTESIAN_POINT('Ctrl Pts',(7.53047676460326,-48.328412295452,20.));
#72125=CARTESIAN_POINT('Ctrl Pts',(7.49673485453118,-48.3305740644544,0.));
#72126=CARTESIAN_POINT('Ctrl Pts',(7.49673485453118,-48.3305740644544,20.));
#72127=CARTESIAN_POINT('Ctrl Pts',(7.46299257874208,-48.3327125314199,0.));
#72128=CARTESIAN_POINT('Ctrl Pts',(7.46299257874208,-48.3327125314199,20.));
#72129=CARTESIAN_POINT('Ctrl Pts',(7.42924995335917,-48.3348276961881,0.));
#72130=CARTESIAN_POINT('Ctrl Pts',(7.42924995335917,-48.3348276961881,20.));
#72131=CARTESIAN_POINT('Ctrl Pts',(7.39550699443533,-48.3369195586108,0.));
#72132=CARTESIAN_POINT('Ctrl Pts',(7.39550699443533,-48.3369195586108,20.));
#72133=CARTESIAN_POINT('Ctrl Pts',(7.36176371798261,-48.3389881185516,0.));
#72134=CARTESIAN_POINT('Ctrl Pts',(7.36176371798261,-48.3389881185516,20.));
#72135=CARTESIAN_POINT('Ctrl Pts',(7.32802013999146,-48.3410333758855,0.));
#72136=CARTESIAN_POINT('Ctrl Pts',(7.32802013999146,-48.3410333758855,20.));
#72137=CARTESIAN_POINT('Ctrl Pts',(7.29427627645269,-48.3430553304987,0.));
#72138=CARTESIAN_POINT('Ctrl Pts',(7.29427627645269,-48.3430553304987,20.));
#72139=CARTESIAN_POINT('Ctrl Pts',(7.26053214338256,-48.3450539822883,0.));
#72140=CARTESIAN_POINT('Ctrl Pts',(7.26053214338256,-48.3450539822883,20.));
#72141=CARTESIAN_POINT('Ctrl Pts',(7.22678775682931,-48.3470293311619,0.));
#72142=CARTESIAN_POINT('Ctrl Pts',(7.22678775682931,-48.3470293311619,20.));
#72143=CARTESIAN_POINT('Ctrl Pts',(7.19304313285997,-48.3489813770376,0.));
#72144=CARTESIAN_POINT('Ctrl Pts',(7.19304313285997,-48.3489813770376,20.));
#72145=CARTESIAN_POINT('Ctrl Pts',(7.15929828755239,-48.3509101198447,0.));
#72146=CARTESIAN_POINT('Ctrl Pts',(7.15929828755239,-48.3509101198447,20.));
#72147=CARTESIAN_POINT('Ctrl Pts',(7.12555323698548,-48.3528155595232,0.));
#72148=CARTESIAN_POINT('Ctrl Pts',(7.12555323698548,-48.3528155595232,20.));
#72149=CARTESIAN_POINT('Ctrl Pts',(7.0918079972288,-48.354697696024,0.));
#72150=CARTESIAN_POINT('Ctrl Pts',(7.0918079972288,-48.354697696024,20.));
#72151=CARTESIAN_POINT('Ctrl Pts',(7.05806258433801,-48.3565565293095,0.));
#72152=CARTESIAN_POINT('Ctrl Pts',(7.05806258433801,-48.3565565293095,20.));
#72153=CARTESIAN_POINT('Ctrl Pts',(7.02431701436125,-48.3583920593534,0.));
#72154=CARTESIAN_POINT('Ctrl Pts',(7.02431701436125,-48.3583920593534,20.));
#72155=CARTESIAN_POINT('Ctrl Pts',(6.99057130334226,-48.3602042861407,0.));
#72156=CARTESIAN_POINT('Ctrl Pts',(6.99057130334226,-48.3602042861407,20.));
#72157=CARTESIAN_POINT('Ctrl Pts',(6.95682546732483,-48.3619932096677,0.));
#72158=CARTESIAN_POINT('Ctrl Pts',(6.95682546732483,-48.3619932096677,20.));
#72159=CARTESIAN_POINT('Ctrl Pts',(6.92307952235708,-48.3637588299416,0.));
#72160=CARTESIAN_POINT('Ctrl Pts',(6.92307952235708,-48.3637588299416,20.));
#72161=CARTESIAN_POINT('Ctrl Pts',(6.8893334844937,-48.3655011469807,0.));
#72162=CARTESIAN_POINT('Ctrl Pts',(6.8893334844937,-48.3655011469807,20.));
#72163=CARTESIAN_POINT('Ctrl Pts',(6.85558736979328,-48.3672201608141,0.));
#72164=CARTESIAN_POINT('Ctrl Pts',(6.85558736979328,-48.3672201608141,20.));
#72165=CARTESIAN_POINT('Ctrl Pts',(6.82184119431717,-48.3689158714816,0.));
#72166=CARTESIAN_POINT('Ctrl Pts',(6.82184119431717,-48.3689158714816,20.));
#72167=CARTESIAN_POINT('Ctrl Pts',(6.78809497412713,-48.370588279034,0.));
#72168=CARTESIAN_POINT('Ctrl Pts',(6.78809497412713,-48.370588279034,20.));
#72169=CARTESIAN_POINT('Ctrl Pts',(6.75434872528384,-48.3722373835335,0.));
#72170=CARTESIAN_POINT('Ctrl Pts',(6.75434872528384,-48.3722373835335,20.));
#72171=CARTESIAN_POINT('Ctrl Pts',(6.72060246384579,-48.3738631850533,0.));
#72172=CARTESIAN_POINT('Ctrl Pts',(6.72060246384579,-48.3738631850533,20.));
#72173=CARTESIAN_POINT('Ctrl Pts',(6.68685620587014,-48.3754656836776,0.));
#72174=CARTESIAN_POINT('Ctrl Pts',(6.68685620587014,-48.3754656836776,20.));
#72175=CARTESIAN_POINT('Ctrl Pts',(6.65310996741333,-48.3770448795022,0.));
#72176=CARTESIAN_POINT('Ctrl Pts',(6.65310996741333,-48.3770448795022,20.));
#72177=CARTESIAN_POINT('Ctrl Pts',(6.61936376453194,-48.3786007726338,0.));
#72178=CARTESIAN_POINT('Ctrl Pts',(6.61936376453194,-48.3786007726338,20.));
#72179=CARTESIAN_POINT('Ctrl Pts',(6.58561761328367,-48.3801333631899,0.));
#72180=CARTESIAN_POINT('Ctrl Pts',(6.58561761328367,-48.3801333631899,20.));
#72181=CARTESIAN_POINT('Ctrl Pts',(6.55187152972771,-48.3816426512995,0.));
#72182=CARTESIAN_POINT('Ctrl Pts',(6.55187152972771,-48.3816426512995,20.));
#72183=CARTESIAN_POINT('Ctrl Pts',(6.51812552992423,-48.3831286371024,0.));
#72184=CARTESIAN_POINT('Ctrl Pts',(6.51812552992423,-48.3831286371024,20.));
#72185=CARTESIAN_POINT('Ctrl Pts',(6.48437962993405,-48.3845913207494,0.));
#72186=CARTESIAN_POINT('Ctrl Pts',(6.48437962993405,-48.3845913207494,20.));
#72187=CARTESIAN_POINT('Ctrl Pts',(6.45063384581844,-48.3860307024022,0.));
#72188=CARTESIAN_POINT('Ctrl Pts',(6.45063384581844,-48.3860307024022,20.));
#72189=CARTESIAN_POINT('Ctrl Pts',(6.41688819363864,-48.3874467822337,0.));
#72190=CARTESIAN_POINT('Ctrl Pts',(6.41688819363864,-48.3874467822337,20.));
#72191=CARTESIAN_POINT('Ctrl Pts',(6.38314268945587,-48.388839560428,0.));
#72192=CARTESIAN_POINT('Ctrl Pts',(6.38314268945587,-48.388839560428,20.));
#72193=CARTESIAN_POINT('Ctrl Pts',(6.34939734933121,-48.3902090371802,0.));
#72194=CARTESIAN_POINT('Ctrl Pts',(6.34939734933121,-48.3902090371802,20.));
#72195=CARTESIAN_POINT('Ctrl Pts',(6.31565218932588,-48.3915552126968,0.));
#72196=CARTESIAN_POINT('Ctrl Pts',(6.31565218932588,-48.3915552126968,20.));
#72197=CARTESIAN_POINT('Ctrl Pts',(6.28190722550132,-48.3928780871951,0.));
#72198=CARTESIAN_POINT('Ctrl Pts',(6.28190722550132,-48.3928780871951,20.));
#72199=CARTESIAN_POINT('Ctrl Pts',(6.24816247391919,-48.3941776609035,0.));
#72200=CARTESIAN_POINT('Ctrl Pts',(6.24816247391919,-48.3941776609035,20.));
#72201=CARTESIAN_POINT('Ctrl Pts',(6.21441795064167,-48.3954539340615,0.));
#72202=CARTESIAN_POINT('Ctrl Pts',(6.21441795064167,-48.3954539340615,20.));
#72203=CARTESIAN_POINT('Ctrl Pts',(6.18067367173123,-48.3967069069196,0.));
#72204=CARTESIAN_POINT('Ctrl Pts',(6.18067367173123,-48.3967069069196,20.));
#72205=CARTESIAN_POINT('Ctrl Pts',(6.14692965325078,-48.3979365797396,0.));
#72206=CARTESIAN_POINT('Ctrl Pts',(6.14692965325078,-48.3979365797396,20.));
#72207=CARTESIAN_POINT('Ctrl Pts',(6.11318591126342,-48.3991429527941,0.));
#72208=CARTESIAN_POINT('Ctrl Pts',(6.11318591126342,-48.3991429527941,20.));
#72209=CARTESIAN_POINT('Ctrl Pts',(6.07944246183266,-48.400326026367,0.));
#72210=CARTESIAN_POINT('Ctrl Pts',(6.07944246183266,-48.400326026367,20.));
#72211=CARTESIAN_POINT('Ctrl Pts',(6.04569932102199,-48.4014858007534,0.));
#72212=CARTESIAN_POINT('Ctrl Pts',(6.04569932102199,-48.4014858007534,20.));
#72213=CARTESIAN_POINT('Ctrl Pts',(6.01195650489504,-48.4026222762592,0.));
#72214=CARTESIAN_POINT('Ctrl Pts',(6.01195650489504,-48.4026222762592,20.));
#72215=CARTESIAN_POINT('Ctrl Pts',(5.97821402951547,-48.4037354532014,0.));
#72216=CARTESIAN_POINT('Ctrl Pts',(5.97821402951547,-48.4037354532014,20.));
#72217=CARTESIAN_POINT('Ctrl Pts',(5.94447191094721,-48.404825331908,0.));
#72218=CARTESIAN_POINT('Ctrl Pts',(5.94447191094721,-48.404825331908,20.));
#72219=CARTESIAN_POINT('Ctrl Pts',(5.91073016525425,-48.4058919127185,0.));
#72220=CARTESIAN_POINT('Ctrl Pts',(5.91073016525425,-48.4058919127185,20.));
#72221=CARTESIAN_POINT('Ctrl Pts',(5.87698880850095,-48.4069351959835,0.));
#72222=CARTESIAN_POINT('Ctrl Pts',(5.87698880850095,-48.4069351959835,20.));
#72223=CARTESIAN_POINT('Ctrl Pts',(5.84324785675189,-48.4079551820643,0.));
#72224=CARTESIAN_POINT('Ctrl Pts',(5.84324785675189,-48.4079551820643,20.));
#72225=CARTESIAN_POINT('Ctrl Pts',(5.80950732607177,-48.4089518713337,0.));
#72226=CARTESIAN_POINT('Ctrl Pts',(5.80950732607177,-48.4089518713337,20.));
#72227=CARTESIAN_POINT('Ctrl Pts',(5.77576723252552,-48.4099252641753,0.));
#72228=CARTESIAN_POINT('Ctrl Pts',(5.77576723252552,-48.4099252641753,20.));
#72229=CARTESIAN_POINT('Ctrl Pts',(5.74202759217812,-48.4108753609837,0.));
#72230=CARTESIAN_POINT('Ctrl Pts',(5.74202759217812,-48.4108753609837,20.));
#72231=CARTESIAN_POINT('Ctrl Pts',(5.70828842109459,-48.4118021621647,0.));
#72232=CARTESIAN_POINT('Ctrl Pts',(5.70828842109459,-48.4118021621647,20.));
#72233=CARTESIAN_POINT('Ctrl Pts',(5.67454973534013,-48.412705668135,0.));
#72234=CARTESIAN_POINT('Ctrl Pts',(5.67454973534013,-48.412705668135,20.));
#72235=CARTESIAN_POINT('Ctrl Pts',(5.64081155098004,-48.4135858793227,0.));
#72236=CARTESIAN_POINT('Ctrl Pts',(5.64081155098004,-48.4135858793227,20.));
#72237=CARTESIAN_POINT('Ctrl Pts',(5.6070738840798,-48.414442796167,0.));
#72238=CARTESIAN_POINT('Ctrl Pts',(5.6070738840798,-48.414442796167,20.));
#72239=CARTESIAN_POINT('Ctrl Pts',(5.57333675070491,-48.4152764191183,0.));
#72240=CARTESIAN_POINT('Ctrl Pts',(5.57333675070491,-48.4152764191183,20.));
#72241=CARTESIAN_POINT('Ctrl Pts',(5.53960016692117,-48.4160867486381,0.));
#72242=CARTESIAN_POINT('Ctrl Pts',(5.53960016692117,-48.4160867486381,20.));
#72243=CARTESIAN_POINT('Ctrl Pts',(5.50586414879429,-48.4168737851989,0.));
#72244=CARTESIAN_POINT('Ctrl Pts',(5.50586414879429,-48.4168737851989,20.));
#72245=CARTESIAN_POINT('Ctrl Pts',(5.47212871239029,-48.417637529284,0.));
#72246=CARTESIAN_POINT('Ctrl Pts',(5.47212871239029,-48.417637529284,20.));
#72247=CARTESIAN_POINT('Ctrl Pts',(5.43839387377497,-48.4183779813881,0.));
#72248=CARTESIAN_POINT('Ctrl Pts',(5.43839387377497,-48.4183779813881,20.));
#72249=CARTESIAN_POINT('Ctrl Pts',(5.40465964901424,-48.4190951420167,0.));
#72250=CARTESIAN_POINT('Ctrl Pts',(5.40465964901424,-48.4190951420167,20.));
#72251=CARTESIAN_POINT('Ctrl Pts',(5.37092605417401,-48.4197890116867,0.));
#72252=CARTESIAN_POINT('Ctrl Pts',(5.37092605417401,-48.4197890116867,20.));
#72253=CARTESIAN_POINT('Ctrl Pts',(5.33719310532026,-48.4204595909261,0.));
#72254=CARTESIAN_POINT('Ctrl Pts',(5.33719310532026,-48.4204595909261,20.));
#72255=CARTESIAN_POINT('Ctrl Pts',(5.30346081851908,-48.4211068802741,0.));
#72256=CARTESIAN_POINT('Ctrl Pts',(5.30346081851908,-48.4211068802741,20.));
#72257=CARTESIAN_POINT('Ctrl Pts',(5.26972920983669,-48.4217308802807,0.));
#72258=CARTESIAN_POINT('Ctrl Pts',(5.26972920983669,-48.4217308802807,20.));
#72259=CARTESIAN_POINT('Ctrl Pts',(5.23599829533944,-48.4223315915069,0.));
#72260=CARTESIAN_POINT('Ctrl Pts',(5.23599829533944,-48.4223315915069,20.));
#72261=CARTESIAN_POINT('Ctrl Pts',(5.2022680910935,-48.4229090145253,0.));
#72262=CARTESIAN_POINT('Ctrl Pts',(5.2022680910935,-48.4229090145253,20.));
#72263=CARTESIAN_POINT('Ctrl Pts',(5.1685386131652,-48.4234631499194,0.));
#72264=CARTESIAN_POINT('Ctrl Pts',(5.1685386131652,-48.4234631499194,20.));
#72265=CARTESIAN_POINT('Ctrl Pts',(5.1348098776207,-48.4239939982838,0.));
#72266=CARTESIAN_POINT('Ctrl Pts',(5.1348098776207,-48.4239939982838,20.));
#72267=CARTESIAN_POINT('Ctrl Pts',(5.10108190052607,-48.4245015602246,0.));
#72268=CARTESIAN_POINT('Ctrl Pts',(5.10108190052607,-48.4245015602246,20.));
#72269=CARTESIAN_POINT('Ctrl Pts',(5.06735469794741,-48.4249858363582,0.));
#72270=CARTESIAN_POINT('Ctrl Pts',(5.06735469794741,-48.4249858363582,20.));
#72271=CARTESIAN_POINT('Ctrl Pts',(5.03362828595092,-48.4254468273122,0.));
#72272=CARTESIAN_POINT('Ctrl Pts',(5.03362828595092,-48.4254468273122,20.));
#72273=CARTESIAN_POINT('Ctrl Pts',(4.99990268060291,-48.4258845337255,0.));
#72274=CARTESIAN_POINT('Ctrl Pts',(4.99990268060291,-48.4258845337255,20.));
#72275=CARTESIAN_POINT('Ctrl Pts',(4.96617789796952,-48.4262989562483,0.));
#72276=CARTESIAN_POINT('Ctrl Pts',(4.96617789796952,-48.4262989562483,20.));
#72277=CARTESIAN_POINT('Ctrl Pts',(4.93245395411684,-48.4266900955418,0.));
#72278=CARTESIAN_POINT('Ctrl Pts',(4.93245395411684,-48.4266900955418,20.));
#72279=CARTESIAN_POINT('Ctrl Pts',(4.89873086511076,-48.4270579522784,0.));
#72280=CARTESIAN_POINT('Ctrl Pts',(4.89873086511076,-48.4270579522784,20.));
#72281=CARTESIAN_POINT('Ctrl Pts',(4.8650086470173,-48.4274025271416,0.));
#72282=CARTESIAN_POINT('Ctrl Pts',(4.8650086470173,-48.4274025271416,20.));
#72283=CARTESIAN_POINT('Ctrl Pts',(4.83128731590228,-48.4277238208263,0.));
#72284=CARTESIAN_POINT('Ctrl Pts',(4.83128731590228,-48.4277238208263,20.));
#72285=CARTESIAN_POINT('Ctrl Pts',(4.79756688783168,-48.4280218340382,0.));
#72286=CARTESIAN_POINT('Ctrl Pts',(4.79756688783168,-48.4280218340382,20.));
#72287=CARTESIAN_POINT('Ctrl Pts',(4.76384737887105,-48.4282965674942,0.));
#72288=CARTESIAN_POINT('Ctrl Pts',(4.76384737887105,-48.4282965674942,20.));
#72289=CARTESIAN_POINT('Ctrl Pts',(4.730128805086,-48.4285480219221,0.));
#72290=CARTESIAN_POINT('Ctrl Pts',(4.730128805086,-48.4285480219221,20.));
#72291=CARTESIAN_POINT('Ctrl Pts',(4.69641118254225,-48.4287761980604,0.));
#72292=CARTESIAN_POINT('Ctrl Pts',(4.69641118254225,-48.4287761980604,20.));
#72293=CARTESIAN_POINT('Ctrl Pts',(4.66269452730542,-48.4289810966589,0.));
#72294=CARTESIAN_POINT('Ctrl Pts',(4.66269452730542,-48.4289810966589,20.));
#72295=CARTESIAN_POINT('Ctrl Pts',(4.62897885544097,-48.4291627184787,0.));
#72296=CARTESIAN_POINT('Ctrl Pts',(4.62897885544097,-48.4291627184787,20.));
#72297=CARTESIAN_POINT('Ctrl Pts',(4.59526418301408,-48.4293210642923,0.));
#72298=CARTESIAN_POINT('Ctrl Pts',(4.59526418301408,-48.4293210642923,20.));
#72299=CARTESIAN_POINT('Ctrl Pts',(4.5615505260898,-48.4294561348833,0.));
#72300=CARTESIAN_POINT('Ctrl Pts',(4.5615505260898,-48.4294561348833,20.));
#72301=CARTESIAN_POINT('Ctrl Pts',(4.52783790073293,-48.4295679310466,0.));
#72302=CARTESIAN_POINT('Ctrl Pts',(4.52783790073293,-48.4295679310466,20.));
#72303=CARTESIAN_POINT('Ctrl Pts',(4.49412632300814,-48.4296564535884,0.));
#72304=CARTESIAN_POINT('Ctrl Pts',(4.49412632300814,-48.4296564535884,20.));
#72305=CARTESIAN_POINT('Ctrl Pts',(4.46041580898011,-48.4297217033257,0.));
#72306=CARTESIAN_POINT('Ctrl Pts',(4.46041580898011,-48.4297217033257,20.));
#72307=CARTESIAN_POINT('Ctrl Pts',(4.4267063747134,-48.4297636810863,0.));
#72308=CARTESIAN_POINT('Ctrl Pts',(4.4267063747134,-48.4297636810863,20.));
#72309=CARTESIAN_POINT('Ctrl Pts',(4.39299803627246,-48.4297823877088,0.));
#72310=CARTESIAN_POINT('Ctrl Pts',(4.39299803627246,-48.4297823877088,20.));
#72311=CARTESIAN_POINT('Ctrl Pts',(4.35929080972166,-48.4297778240431,0.));
#72312=CARTESIAN_POINT('Ctrl Pts',(4.35929080972166,-48.4297778240431,20.));
#72313=CARTESIAN_POINT('Ctrl Pts',(4.32558471112516,-48.42974999095,0.));
#72314=CARTESIAN_POINT('Ctrl Pts',(4.32558471112516,-48.42974999095,20.));
#72315=CARTESIAN_POINT('Ctrl Pts',(4.29187975654677,-48.4296988893018,0.));
#72316=CARTESIAN_POINT('Ctrl Pts',(4.29187975654677,-48.4296988893018,20.));
#72317=CARTESIAN_POINT('Ctrl Pts',(4.25817596205,-48.4296245199823,0.));
#72318=CARTESIAN_POINT('Ctrl Pts',(4.25817596205,-48.4296245199823,20.));
#72319=CARTESIAN_POINT('Ctrl Pts',(4.22447334369801,-48.4295268838864,0.));
#72320=CARTESIAN_POINT('Ctrl Pts',(4.22447334369801,-48.4295268838864,20.));
#72321=CARTESIAN_POINT('Ctrl Pts',(4.19077191755405,-48.4294059819202,0.));
#72322=CARTESIAN_POINT('Ctrl Pts',(4.19077191755405,-48.4294059819202,20.));
#72323=CARTESIAN_POINT('Ctrl Pts',(4.15707169968115,-48.4292618150011,0.));
#72324=CARTESIAN_POINT('Ctrl Pts',(4.15707169968115,-48.4292618150011,20.));
#72325=CARTESIAN_POINT('Ctrl Pts',(4.1233727061421,-48.429094384057,0.));
#72326=CARTESIAN_POINT('Ctrl Pts',(4.1233727061421,-48.429094384057,20.));
#72327=CARTESIAN_POINT('Ctrl Pts',(4.08967495299951,-48.4289036900268,0.));
#72328=CARTESIAN_POINT('Ctrl Pts',(4.08967495299951,-48.4289036900268,20.));
#72329=CARTESIAN_POINT('Ctrl Pts',(4.05597845631568,-48.4286897338604,0.));
#72330=CARTESIAN_POINT('Ctrl Pts',(4.05597845631568,-48.4286897338604,20.));
#72331=CARTESIAN_POINT('Ctrl Pts',(4.02228323215259,-48.4284525165189,0.));
#72332=CARTESIAN_POINT('Ctrl Pts',(4.02228323215259,-48.4284525165189,20.));
#72333=CARTESIAN_POINT('Ctrl Pts',(3.988589296572,-48.4281920389749,0.));
#72334=CARTESIAN_POINT('Ctrl Pts',(3.988589296572,-48.4281920389749,20.));
#72335=CARTESIAN_POINT('Ctrl Pts',(3.95489666563548,-48.427908302212,0.));
#72336=CARTESIAN_POINT('Ctrl Pts',(3.95489666563548,-48.427908302212,20.));
#72337=CARTESIAN_POINT('Ctrl Pts',(3.9212053554042,-48.4276013072253,0.));
#72338=CARTESIAN_POINT('Ctrl Pts',(3.9212053554042,-48.4276013072253,20.));
#72339=CARTESIAN_POINT('Ctrl Pts',(3.88751538193919,-48.4272710550207,0.));
#72340=CARTESIAN_POINT('Ctrl Pts',(3.88751538193919,-48.4272710550207,20.));
#72341=CARTESIAN_POINT('Ctrl Pts',(3.85382676130114,-48.4269175466151,0.));
#72342=CARTESIAN_POINT('Ctrl Pts',(3.85382676130114,-48.4269175466151,20.));
#72343=CARTESIAN_POINT('Ctrl Pts',(3.82013950955042,-48.4265407830367,0.));
#72344=CARTESIAN_POINT('Ctrl Pts',(3.82013950955042,-48.4265407830367,20.));
#72345=CARTESIAN_POINT('Ctrl Pts',(3.78645364274706,-48.4261407653249,0.));
#72346=CARTESIAN_POINT('Ctrl Pts',(3.78645364274706,-48.4261407653249,20.));
#72347=CARTESIAN_POINT('Ctrl Pts',(3.75276917695084,-48.4257174945298,0.));
#72348=CARTESIAN_POINT('Ctrl Pts',(3.75276917695084,-48.4257174945298,20.));
#72349=CARTESIAN_POINT('Ctrl Pts',(3.71908612822108,-48.4252709717129,0.));
#72350=CARTESIAN_POINT('Ctrl Pts',(3.71908612822108,-48.4252709717129,20.));
#72351=CARTESIAN_POINT('Ctrl Pts',(3.68540451261695,-48.424801197947,0.));
#72352=CARTESIAN_POINT('Ctrl Pts',(3.68540451261695,-48.424801197947,20.));
#72353=CARTESIAN_POINT('Ctrl Pts',(3.6517243461974,-48.4243081743158,0.));
#72354=CARTESIAN_POINT('Ctrl Pts',(3.6517243461974,-48.4243081743158,20.));
#72355=CARTESIAN_POINT('Ctrl Pts',(3.61804564502096,-48.4237919019141,0.));
#72356=CARTESIAN_POINT('Ctrl Pts',(3.61804564502096,-48.4237919019141,20.));
#72357=CARTESIAN_POINT('Ctrl Pts',(3.58436842514564,-48.4232523818483,0.));
#72358=CARTESIAN_POINT('Ctrl Pts',(3.58436842514564,-48.4232523818483,20.));
#72359=CARTESIAN_POINT('Ctrl Pts',(3.55069270262907,-48.4226896152354,0.));
#72360=CARTESIAN_POINT('Ctrl Pts',(3.55069270262907,-48.4226896152354,20.));
#72361=CARTESIAN_POINT('Ctrl Pts',(3.51701849352853,-48.422103603204,0.));
#72362=CARTESIAN_POINT('Ctrl Pts',(3.51701849352853,-48.422103603204,20.));
#72363=CARTESIAN_POINT('Ctrl Pts',(3.483345813901,-48.4214943468927,0.));
#72364=CARTESIAN_POINT('Ctrl Pts',(3.483345813901,-48.4214943468927,20.));
#72365=CARTESIAN_POINT('Ctrl Pts',(3.44967467980323,-48.4208618474523,0.));
#72366=CARTESIAN_POINT('Ctrl Pts',(3.44967467980323,-48.4208618474523,20.));
#72367=CARTESIAN_POINT('Ctrl Pts',(3.41600510729148,-48.4202061060442,0.));
#72368=CARTESIAN_POINT('Ctrl Pts',(3.41600510729148,-48.4202061060442,20.));
#72369=CARTESIAN_POINT('Ctrl Pts',(3.38233711242167,-48.4195271238417,0.));
#72370=CARTESIAN_POINT('Ctrl Pts',(3.38233711242167,-48.4195271238417,20.));
#72371=CARTESIAN_POINT('Ctrl Pts',(3.34867071124917,-48.4188249020284,0.));
#72372=CARTESIAN_POINT('Ctrl Pts',(3.34867071124917,-48.4188249020284,20.));
#72373=CARTESIAN_POINT('Ctrl Pts',(3.31500591982887,-48.4180994417999,0.));
#72374=CARTESIAN_POINT('Ctrl Pts',(3.31500591982887,-48.4180994417999,20.));
#72375=CARTESIAN_POINT('Ctrl Pts',(3.28134275421531,-48.4173507443625,0.));
#72376=CARTESIAN_POINT('Ctrl Pts',(3.28134275421531,-48.4173507443625,20.));
#72377=CARTESIAN_POINT('Ctrl Pts',(3.24768123046264,-48.4165788109335,0.));
#72378=CARTESIAN_POINT('Ctrl Pts',(3.24768123046264,-48.4165788109335,20.));
#72379=CARTESIAN_POINT('Ctrl Pts',(3.21402136462457,-48.4157836427414,0.));
#72380=CARTESIAN_POINT('Ctrl Pts',(3.21402136462457,-48.4157836427414,20.));
#72381=CARTESIAN_POINT('Ctrl Pts',(3.18036317275453,-48.4149652410254,0.));
#72382=CARTESIAN_POINT('Ctrl Pts',(3.18036317275453,-48.4149652410254,20.));
#72383=CARTESIAN_POINT('Ctrl Pts',(3.14670667090555,-48.414123607036,0.));
#72384=CARTESIAN_POINT('Ctrl Pts',(3.14670667090555,-48.414123607036,20.));
#72385=CARTESIAN_POINT('Ctrl Pts',(3.11305187512999,-48.4132587420349,0.));
#72386=CARTESIAN_POINT('Ctrl Pts',(3.11305187512999,-48.4132587420349,20.));
#72387=CARTESIAN_POINT('Ctrl Pts',(3.07939880147968,-48.4123706472953,0.));
#72388=CARTESIAN_POINT('Ctrl Pts',(3.07939880147968,-48.4123706472953,20.));
#72389=CARTESIAN_POINT('Ctrl Pts',(3.04574746600607,-48.4114593241014,0.));
#72390=CARTESIAN_POINT('Ctrl Pts',(3.04574746600607,-48.4114593241014,20.));
#72391=CARTESIAN_POINT('Ctrl Pts',(3.01209788475993,-48.4105247737488,0.));
#72392=CARTESIAN_POINT('Ctrl Pts',(3.01209788475993,-48.4105247737488,20.));
#72393=CARTESIAN_POINT('Ctrl Pts',(2.97845007379181,-48.4095669975441,0.));
#72394=CARTESIAN_POINT('Ctrl Pts',(2.97845007379181,-48.4095669975441,20.));
#72395=CARTESIAN_POINT('Ctrl Pts',(2.94480404915164,-48.4085859968048,0.));
#72396=CARTESIAN_POINT('Ctrl Pts',(2.94480404915164,-48.4085859968048,20.));
#72397=CARTESIAN_POINT('Ctrl Pts',(2.91115982688903,-48.4075817728593,0.));
#72398=CARTESIAN_POINT('Ctrl Pts',(2.91115982688903,-48.4075817728593,20.));
#72399=CARTESIAN_POINT('Ctrl Pts',(2.87751742305292,-48.4065543270471,0.));
#72400=CARTESIAN_POINT('Ctrl Pts',(2.87751742305292,-48.4065543270471,20.));
#72401=CARTESIAN_POINT('Ctrl Pts',(2.8438768536918,-48.4055036607195,0.));
#72402=CARTESIAN_POINT('Ctrl Pts',(2.8438768536918,-48.4055036607195,20.));
#72403=CARTESIAN_POINT('Ctrl Pts',(2.81023813485355,-48.4044297752383,0.));
#72404=CARTESIAN_POINT('Ctrl Pts',(2.81023813485355,-48.4044297752383,20.));
#72405=CARTESIAN_POINT('Ctrl Pts',(2.77660128258546,-48.4033326719771,0.));
#72406=CARTESIAN_POINT('Ctrl Pts',(2.77660128258546,-48.4033326719771,20.));
#72407=CARTESIAN_POINT('Ctrl Pts',(2.74296631293436,-48.4022123523201,0.));
#72408=CARTESIAN_POINT('Ctrl Pts',(2.74296631293436,-48.4022123523201,20.));
#72409=CARTESIAN_POINT('Ctrl Pts',(2.7093332419466,-48.4010688176627,0.));
#72410=CARTESIAN_POINT('Ctrl Pts',(2.7093332419466,-48.4010688176627,20.));
#72411=CARTESIAN_POINT('Ctrl Pts',(2.67570208566793,-48.3999020694116,0.));
#72412=CARTESIAN_POINT('Ctrl Pts',(2.67570208566793,-48.3999020694116,20.));
#72413=CARTESIAN_POINT('Ctrl Pts',(2.64207286014349,-48.3987121089844,0.));
#72414=CARTESIAN_POINT('Ctrl Pts',(2.64207286014349,-48.3987121089844,20.));
#72415=CARTESIAN_POINT('Ctrl Pts',(2.60844558141789,-48.3974989378103,0.));
#72416=CARTESIAN_POINT('Ctrl Pts',(2.60844558141789,-48.3974989378103,20.));
#72417=CARTESIAN_POINT('Ctrl Pts',(2.57482026553515,-48.3962625573292,0.));
#72418=CARTESIAN_POINT('Ctrl Pts',(2.57482026553515,-48.3962625573292,20.));
#72419=CARTESIAN_POINT('Ctrl Pts',(2.5411969285386,-48.3950029689925,0.));
#72420=CARTESIAN_POINT('Ctrl Pts',(2.5411969285386,-48.3950029689925,20.));
#72421=CARTESIAN_POINT('Ctrl Pts',(2.50757558647119,-48.3937201742621,0.));
#72422=CARTESIAN_POINT('Ctrl Pts',(2.50757558647119,-48.3937201742621,20.));
#72423=CARTESIAN_POINT('Ctrl Pts',(2.47395625537494,-48.3924141746117,0.));
#72424=CARTESIAN_POINT('Ctrl Pts',(2.47395625537494,-48.3924141746117,20.));
#72425=CARTESIAN_POINT('Ctrl Pts',(2.44033895129153,-48.3910849715258,0.));
#72426=CARTESIAN_POINT('Ctrl Pts',(2.44033895129153,-48.3910849715258,20.));
#72427=CARTESIAN_POINT('Ctrl Pts',(2.40672369026195,-48.3897325665,0.));
#72428=CARTESIAN_POINT('Ctrl Pts',(2.40672369026195,-48.3897325665,20.));
#72429=CARTESIAN_POINT('Ctrl Pts',(2.37311048832664,-48.3883569610415,0.));
#72430=CARTESIAN_POINT('Ctrl Pts',(2.37311048832664,-48.3883569610415,20.));
#72431=CARTESIAN_POINT('Ctrl Pts',(2.33949936152533,-48.3869581566679,0.));
#72432=CARTESIAN_POINT('Ctrl Pts',(2.33949936152533,-48.3869581566679,20.));
#72433=CARTESIAN_POINT('Ctrl Pts',(2.30589032589699,-48.3855361549086,0.));
#72434=CARTESIAN_POINT('Ctrl Pts',(2.30589032589699,-48.3855361549086,20.));
#72435=CARTESIAN_POINT('Ctrl Pts',(2.27228339748008,-48.3840909573039,0.));
#72436=CARTESIAN_POINT('Ctrl Pts',(2.27228339748008,-48.3840909573039,20.));
#72437=CARTESIAN_POINT('Ctrl Pts',(2.2386785923122,-48.3826225654054,0.));
#72438=CARTESIAN_POINT('Ctrl Pts',(2.2386785923122,-48.3826225654054,20.));
#72439=CARTESIAN_POINT('Ctrl Pts',(2.20507592643041,-48.3811309807756,0.));
#72440=CARTESIAN_POINT('Ctrl Pts',(2.20507592643041,-48.3811309807756,20.));
#72441=CARTESIAN_POINT('Ctrl Pts',(2.17147541587102,-48.3796162049883,0.));
#72442=CARTESIAN_POINT('Ctrl Pts',(2.17147541587102,-48.3796162049883,20.));
#72443=CARTESIAN_POINT('Ctrl Pts',(2.13787707667012,-48.3780782396279,0.));
#72444=CARTESIAN_POINT('Ctrl Pts',(2.13787707667012,-48.3780782396279,20.));
#72445=CARTESIAN_POINT('Ctrl Pts',(2.10428092486293,-48.3765170862905,0.));
#72446=CARTESIAN_POINT('Ctrl Pts',(2.10428092486293,-48.3765170862905,20.));
#72447=CARTESIAN_POINT('Ctrl Pts',(2.07068697648387,-48.374932746583,0.));
#72448=CARTESIAN_POINT('Ctrl Pts',(2.07068697648387,-48.374932746583,20.));
#72449=CARTESIAN_POINT('Ctrl Pts',(2.03709524756654,-48.3733252221237,0.));
#72450=CARTESIAN_POINT('Ctrl Pts',(2.03709524756654,-48.3733252221237,20.));
#72451=CARTESIAN_POINT('Ctrl Pts',(2.00350575414355,-48.3716945145424,0.));
#72452=CARTESIAN_POINT('Ctrl Pts',(2.00350575414355,-48.3716945145424,20.));
#72453=CARTESIAN_POINT('Ctrl Pts',(1.96991851224691,-48.3700406254798,0.));
#72454=CARTESIAN_POINT('Ctrl Pts',(1.96991851224691,-48.3700406254798,20.));
#72455=CARTESIAN_POINT('Ctrl Pts',(1.93633353790811,-48.3683635565876,0.));
#72456=CARTESIAN_POINT('Ctrl Pts',(1.93633353790811,-48.3683635565876,20.));
#72457=CARTESIAN_POINT('Ctrl Pts',(1.90275084715795,-48.3666633095284,0.));
#72458=CARTESIAN_POINT('Ctrl Pts',(1.90275084715795,-48.3666633095284,20.));
#72459=CARTESIAN_POINT('Ctrl Pts',(1.86917045602651,-48.3649398859758,0.));
#72460=CARTESIAN_POINT('Ctrl Pts',(1.86917045602651,-48.3649398859758,20.));
#72461=CARTESIAN_POINT('Ctrl Pts',(1.83559238054322,-48.3631932876149,0.));
#72462=CARTESIAN_POINT('Ctrl Pts',(1.83559238054322,-48.3631932876149,20.));
#72463=CARTESIAN_POINT('Ctrl Pts',(1.80201663673655,-48.3614235161422,0.));
#72464=CARTESIAN_POINT('Ctrl Pts',(1.80201663673655,-48.3614235161422,20.));
#72465=CARTESIAN_POINT('Ctrl Pts',(1.76844324063425,-48.3596305732653,0.));
#72466=CARTESIAN_POINT('Ctrl Pts',(1.76844324063425,-48.3596305732653,20.));
#72467=CARTESIAN_POINT('Ctrl Pts',(1.73487220826325,-48.357814460703,0.));
#72468=CARTESIAN_POINT('Ctrl Pts',(1.73487220826325,-48.357814460703,20.));
#72469=CARTESIAN_POINT('Ctrl Pts',(1.70130355564956,-48.3559751801849,0.));
#72470=CARTESIAN_POINT('Ctrl Pts',(1.70130355564956,-48.3559751801849,20.));
#72471=CARTESIAN_POINT('Ctrl Pts',(1.66773729881855,-48.3541127334515,0.));
#72472=CARTESIAN_POINT('Ctrl Pts',(1.66773729881855,-48.3541127334515,20.));
#72473=CARTESIAN_POINT('Ctrl Pts',(1.63417345379481,-48.3522271222546,0.));
#72474=CARTESIAN_POINT('Ctrl Pts',(1.63417345379481,-48.3522271222546,20.));
#72475=CARTESIAN_POINT('Ctrl Pts',(1.60061203660205,-48.350318348357,0.));
#72476=CARTESIAN_POINT('Ctrl Pts',(1.60061203660205,-48.350318348357,20.));
#72477=CARTESIAN_POINT('Ctrl Pts',(1.56705306326331,-48.3483864135332,0.));
#72478=CARTESIAN_POINT('Ctrl Pts',(1.56705306326331,-48.3483864135332,20.));
#72479=CARTESIAN_POINT('Ctrl Pts',(1.53349654980076,-48.3464313195685,0.));
#72480=CARTESIAN_POINT('Ctrl Pts',(1.53349654980076,-48.3464313195685,20.));
#72481=CARTESIAN_POINT('Ctrl Pts',(1.4999425122357,-48.3444530682597,0.));
#72482=CARTESIAN_POINT('Ctrl Pts',(1.4999425122357,-48.3444530682597,20.));
#72483=CARTESIAN_POINT('Ctrl Pts',(1.46639096658851,-48.3424516614145,0.));
#72484=CARTESIAN_POINT('Ctrl Pts',(1.46639096658851,-48.3424516614145,20.));
#72485=CARTESIAN_POINT('Ctrl Pts',(1.43284192887878,-48.3404271008519,0.));
#72486=CARTESIAN_POINT('Ctrl Pts',(1.43284192887878,-48.3404271008519,20.));
#72487=CARTESIAN_POINT('Ctrl Pts',(1.39929541512519,-48.3383793884017,0.));
#72488=CARTESIAN_POINT('Ctrl Pts',(1.39929541512519,-48.3383793884017,20.));
#72489=CARTESIAN_POINT('Ctrl Pts',(1.3657514413457,-48.336308525905,0.));
#72490=CARTESIAN_POINT('Ctrl Pts',(1.3657514413457,-48.336308525905,20.));
#72491=CARTESIAN_POINT('Ctrl Pts',(1.33221002355742,-48.3342145152137,0.));
#72492=CARTESIAN_POINT('Ctrl Pts',(1.33221002355742,-48.3342145152137,20.));
#72493=CARTESIAN_POINT('Ctrl Pts',(1.29867117777651,-48.3320973581913,0.));
#72494=CARTESIAN_POINT('Ctrl Pts',(1.29867117777651,-48.3320973581913,20.));
#72495=CARTESIAN_POINT('Ctrl Pts',(1.26513492001821,-48.3299570567123,0.));
#72496=CARTESIAN_POINT('Ctrl Pts',(1.26513492001821,-48.3299570567123,20.));
#72497=CARTESIAN_POINT('Ctrl Pts',(1.23160126629692,-48.3277936126623,0.));
#72498=CARTESIAN_POINT('Ctrl Pts',(1.23160126629692,-48.3277936126623,20.));
#72499=CARTESIAN_POINT('Ctrl Pts',(1.19807023262611,-48.3256070279384,0.));
#72500=CARTESIAN_POINT('Ctrl Pts',(1.19807023262611,-48.3256070279384,20.));
#72501=CARTESIAN_POINT('Ctrl Pts',(1.16454183501838,-48.3233973044482,0.));
#72502=CARTESIAN_POINT('Ctrl Pts',(1.16454183501838,-48.3233973044482,20.));
#72503=CARTESIAN_POINT('Ctrl Pts',(1.13101608948534,-48.3211644441107,0.));
#72504=CARTESIAN_POINT('Ctrl Pts',(1.13101608948534,-48.3211644441107,20.));
#72505=CARTESIAN_POINT('Ctrl Pts',(1.09749301203762,-48.3189084488565,0.));
#72506=CARTESIAN_POINT('Ctrl Pts',(1.09749301203762,-48.3189084488565,20.));
#72507=CARTESIAN_POINT('Ctrl Pts',(1.063972618685,-48.3166293206271,0.));
#72508=CARTESIAN_POINT('Ctrl Pts',(1.063972618685,-48.3166293206271,20.));
#72509=CARTESIAN_POINT('Ctrl Pts',(1.0304549254364,-48.3143270613748,0.));
#72510=CARTESIAN_POINT('Ctrl Pts',(1.0304549254364,-48.3143270613748,20.));
#72511=CARTESIAN_POINT('Ctrl Pts',(0.996939948299849,-48.312001673063,0.));
#72512=CARTESIAN_POINT('Ctrl Pts',(0.996939948299849,-48.312001673063,20.));
#72513=CARTESIAN_POINT('Ctrl Pts',(0.963427703282353,-48.3096531576664,
0.));
#72514=CARTESIAN_POINT('Ctrl Pts',(0.963427703282353,-48.3096531576664,
20.));
#72515=CARTESIAN_POINT('Ctrl Pts',(0.929918206389826,-48.3072815171712,
0.));
#72516=CARTESIAN_POINT('Ctrl Pts',(0.929918206389826,-48.3072815171712,
20.));
#72517=CARTESIAN_POINT('Ctrl Pts',(0.896411473627223,-48.3048867535744,
0.));
#72518=CARTESIAN_POINT('Ctrl Pts',(0.896411473627223,-48.3048867535744,
20.));
#72519=CARTESIAN_POINT('Ctrl Pts',(0.862907520998486,-48.3024688688845,
0.));
#72520=CARTESIAN_POINT('Ctrl Pts',(0.862907520998486,-48.3024688688845,
20.));
#72521=CARTESIAN_POINT('Ctrl Pts',(0.829406364506662,-48.3000278651208,
0.));
#72522=CARTESIAN_POINT('Ctrl Pts',(0.829406364506662,-48.3000278651208,
20.));
#72523=CARTESIAN_POINT('Ctrl Pts',(0.795908020153888,-48.2975637443136,
0.));
#72524=CARTESIAN_POINT('Ctrl Pts',(0.795908020153888,-48.2975637443136,
20.));
#72525=CARTESIAN_POINT('Ctrl Pts',(0.762412503941521,-48.2950765085043,
0.));
#72526=CARTESIAN_POINT('Ctrl Pts',(0.762412503941521,-48.2950765085043,
20.));
#72527=CARTESIAN_POINT('Ctrl Pts',(0.728919831869645,-48.2925661597457,
0.));
#72528=CARTESIAN_POINT('Ctrl Pts',(0.728919831869645,-48.2925661597457,
20.));
#72529=CARTESIAN_POINT('Ctrl Pts',(0.69543001993734,-48.2900327001016,0.));
#72530=CARTESIAN_POINT('Ctrl Pts',(0.69543001993734,-48.2900327001016,20.));
#72531=CARTESIAN_POINT('Ctrl Pts',(0.661943084142442,-48.2874761316474,
0.));
#72532=CARTESIAN_POINT('Ctrl Pts',(0.661943084142442,-48.2874761316474,
20.));
#72533=CARTESIAN_POINT('Ctrl Pts',(0.628459040481828,-48.2848964564694,
0.));
#72534=CARTESIAN_POINT('Ctrl Pts',(0.628459040481828,-48.2848964564694,
20.));
#72535=CARTESIAN_POINT('Ctrl Pts',(0.594977904951266,-48.282293676665,0.));
#72536=CARTESIAN_POINT('Ctrl Pts',(0.594977904951266,-48.282293676665,20.));
#72537=CARTESIAN_POINT('Ctrl Pts',(0.561499693545673,-48.2796677943426,
0.));
#72538=CARTESIAN_POINT('Ctrl Pts',(0.561499693545673,-48.2796677943426,
20.));
#72539=CARTESIAN_POINT('Ctrl Pts',(0.528024422259019,-48.2770188116216,
0.));
#72540=CARTESIAN_POINT('Ctrl Pts',(0.528024422259019,-48.2770188116216,
20.));
#72541=CARTESIAN_POINT('Ctrl Pts',(0.49455210708421,-48.2743467306329,0.));
#72542=CARTESIAN_POINT('Ctrl Pts',(0.49455210708421,-48.2743467306329,20.));
#72543=CARTESIAN_POINT('Ctrl Pts',(0.461082764012986,-48.2716515535183,
0.));
#72544=CARTESIAN_POINT('Ctrl Pts',(0.461082764012986,-48.2716515535183,
20.));
#72545=CARTESIAN_POINT('Ctrl Pts',(0.427616409036036,-48.2689332824309,
0.));
#72546=CARTESIAN_POINT('Ctrl Pts',(0.427616409036036,-48.2689332824309,
20.));
#72547=CARTESIAN_POINT('Ctrl Pts',(0.394153058142903,-48.2661919195348,
0.));
#72548=CARTESIAN_POINT('Ctrl Pts',(0.394153058142903,-48.2661919195348,
20.));
#72549=CARTESIAN_POINT('Ctrl Pts',(0.360692727321981,-48.2634274670053,
0.));
#72550=CARTESIAN_POINT('Ctrl Pts',(0.360692727321981,-48.2634274670053,
20.));
#72551=CARTESIAN_POINT('Ctrl Pts',(0.327235432560538,-48.2606399270286,
0.));
#72552=CARTESIAN_POINT('Ctrl Pts',(0.327235432560538,-48.2606399270286,
20.));
#72553=CARTESIAN_POINT('Ctrl Pts',(0.293781189844817,-48.2578293018028,
0.));
#72554=CARTESIAN_POINT('Ctrl Pts',(0.293781189844817,-48.2578293018028,
20.));
#72555=CARTESIAN_POINT('Ctrl Pts',(0.260330015159931,-48.2549955935366,
0.));
#72556=CARTESIAN_POINT('Ctrl Pts',(0.260330015159931,-48.2549955935366,
20.));
#72557=CARTESIAN_POINT('Ctrl Pts',(0.226881924489848,-48.2521388044499,
0.));
#72558=CARTESIAN_POINT('Ctrl Pts',(0.226881924489848,-48.2521388044499,
20.));
#72559=CARTESIAN_POINT('Ctrl Pts',(0.193436933817455,-48.2492589367737,
0.));
#72560=CARTESIAN_POINT('Ctrl Pts',(0.193436933817455,-48.2492589367737,
20.));
#72561=CARTESIAN_POINT('Ctrl Pts',(0.159995059124558,-48.2463559927498,
0.));
#72562=CARTESIAN_POINT('Ctrl Pts',(0.159995059124558,-48.2463559927498,
20.));
#72563=CARTESIAN_POINT('Ctrl Pts',(0.126556316391659,-48.2434299746318,
0.));
#72564=CARTESIAN_POINT('Ctrl Pts',(0.126556316391659,-48.2434299746318,
20.));
#72565=CARTESIAN_POINT('Ctrl Pts',(0.0931207215982655,-48.2404808846839,
0.));
#72566=CARTESIAN_POINT('Ctrl Pts',(0.0931207215982655,-48.2404808846839,
20.));
#72567=CARTESIAN_POINT('Ctrl Pts',(0.0596882907225815,-48.2375087251817,
0.));
#72568=CARTESIAN_POINT('Ctrl Pts',(0.0596882907225815,-48.2375087251817,
20.));
#72569=CARTESIAN_POINT('Ctrl Pts',(0.0262590397416584,-48.234513498412,
0.));
#72570=CARTESIAN_POINT('Ctrl Pts',(0.0262590397416584,-48.234513498412,
20.));
#72571=CARTESIAN_POINT('Ctrl Pts',(-0.00716701536858544,-48.2314952066725,
0.));
#72572=CARTESIAN_POINT('Ctrl Pts',(-0.00716701536858544,-48.2314952066725,
20.));
#72573=CARTESIAN_POINT('Ctrl Pts',(-0.040589858633453,-48.2284538522724,
0.));
#72574=CARTESIAN_POINT('Ctrl Pts',(-0.040589858633453,-48.2284538522724,
20.));
#72575=CARTESIAN_POINT('Ctrl Pts',(-0.0740094740794106,-48.2253894375317,
0.));
#72576=CARTESIAN_POINT('Ctrl Pts',(-0.0740094740794106,-48.2253894375317,
20.));
#72577=CARTESIAN_POINT('Ctrl Pts',(-0.107425845734137,-48.2223019647818,
0.));
#72578=CARTESIAN_POINT('Ctrl Pts',(-0.107425845734137,-48.2223019647818,
20.));
#72579=CARTESIAN_POINT('Ctrl Pts',(-0.140838957626559,-48.2191914363652,
0.));
#72580=CARTESIAN_POINT('Ctrl Pts',(-0.140838957626559,-48.2191914363652,
20.));
#72581=CARTESIAN_POINT('Ctrl Pts',(-0.174248793786917,-48.2160578546352,
0.));
#72582=CARTESIAN_POINT('Ctrl Pts',(-0.174248793786917,-48.2160578546352,
20.));
#72583=CARTESIAN_POINT('Ctrl Pts',(-0.207655338246577,-48.2129012219564,
0.));
#72584=CARTESIAN_POINT('Ctrl Pts',(-0.207655338246577,-48.2129012219564,
20.));
#72585=CARTESIAN_POINT('Ctrl Pts',(-0.241058575037889,-48.2097215407045,
0.));
#72586=CARTESIAN_POINT('Ctrl Pts',(-0.241058575037889,-48.2097215407045,
20.));
#72587=CARTESIAN_POINT('Ctrl Pts',(-0.274458488194607,-48.2065188132665,
0.));
#72588=CARTESIAN_POINT('Ctrl Pts',(-0.274458488194607,-48.2065188132665,
20.));
#72589=CARTESIAN_POINT('Ctrl Pts',(-0.307855061751732,-48.2032930420408,
0.));
#72590=CARTESIAN_POINT('Ctrl Pts',(-0.307855061751732,-48.2032930420408,
20.));
#72591=CARTESIAN_POINT('Ctrl Pts',(-0.341248279745661,-48.2000442294364,
0.));
#72592=CARTESIAN_POINT('Ctrl Pts',(-0.341248279745661,-48.2000442294364,
20.));
#72593=CARTESIAN_POINT('Ctrl Pts',(-0.374638126214117,-48.1967723778737,
0.));
#72594=CARTESIAN_POINT('Ctrl Pts',(-0.374638126214117,-48.1967723778737,
20.));
#72595=CARTESIAN_POINT('Ctrl Pts',(-0.408024585196243,-48.1934774897842,
0.));
#72596=CARTESIAN_POINT('Ctrl Pts',(-0.408024585196243,-48.1934774897842,
20.));
#72597=CARTESIAN_POINT('Ctrl Pts',(-0.441407640732114,-48.1901595676102,
0.));
#72598=CARTESIAN_POINT('Ctrl Pts',(-0.441407640732114,-48.1901595676102,
20.));
#72599=CARTESIAN_POINT('Ctrl Pts',(-0.474787276863089,-48.1868186138054,
0.));
#72600=CARTESIAN_POINT('Ctrl Pts',(-0.474787276863089,-48.1868186138054,
20.));
#72601=CARTESIAN_POINT('Ctrl Pts',(-0.508163477631873,-48.1834546308352,
0.));
#72602=CARTESIAN_POINT('Ctrl Pts',(-0.508163477631873,-48.1834546308352,
20.));
#72603=CARTESIAN_POINT('Ctrl Pts',(-0.541536227082378,-48.1800676211754,
0.));
#72604=CARTESIAN_POINT('Ctrl Pts',(-0.541536227082378,-48.1800676211754,
20.));
#72605=CARTESIAN_POINT('Ctrl Pts',(-0.574905509259906,-48.1766575873132,
0.));
#72606=CARTESIAN_POINT('Ctrl Pts',(-0.574905509259906,-48.1766575873132,
20.));
#72607=CARTESIAN_POINT('Ctrl Pts',(-0.608271308211115,-48.1732245317468,
0.));
#72608=CARTESIAN_POINT('Ctrl Pts',(-0.608271308211115,-48.1732245317468,
20.));
#72609=CARTESIAN_POINT('Ctrl Pts',(-0.641633607984118,-48.1697684569855,
0.));
#72610=CARTESIAN_POINT('Ctrl Pts',(-0.641633607984118,-48.1697684569855,
20.));
#72611=CARTESIAN_POINT('Ctrl Pts',(-0.674992392628253,-48.16628936555,0.));
#72612=CARTESIAN_POINT('Ctrl Pts',(-0.674992392628253,-48.16628936555,20.));
#72613=CARTESIAN_POINT('Ctrl Pts',(-0.708347646194296,-48.1627872599717,
0.));
#72614=CARTESIAN_POINT('Ctrl Pts',(-0.708347646194296,-48.1627872599717,
20.));
#72615=CARTESIAN_POINT('Ctrl Pts',(-0.741699352734275,-48.1592621427937,
0.));
#72616=CARTESIAN_POINT('Ctrl Pts',(-0.741699352734275,-48.1592621427937,
20.));
#72617=CARTESIAN_POINT('Ctrl Pts',(-0.775047496301551,-48.1557140165701,
0.));
#72618=CARTESIAN_POINT('Ctrl Pts',(-0.775047496301551,-48.1557140165701,
20.));
#72619=CARTESIAN_POINT('Ctrl Pts',(-0.808392060950887,-48.1521428838659,
0.));
#72620=CARTESIAN_POINT('Ctrl Pts',(-0.808392060950887,-48.1521428838659,
20.));
#72621=CARTESIAN_POINT('Ctrl Pts',(-0.84173303073841,-48.1485487472572,
0.));
#72622=CARTESIAN_POINT('Ctrl Pts',(-0.84173303073841,-48.1485487472572,
20.));
#72623=CARTESIAN_POINT('Ctrl Pts',(-0.875070389721544,-48.144931609331,
0.));
#72624=CARTESIAN_POINT('Ctrl Pts',(-0.875070389721544,-48.144931609331,
20.));
#72625=CARTESIAN_POINT('Ctrl Pts',(-0.908404121959303,-48.1412914726861,
0.));
#72626=CARTESIAN_POINT('Ctrl Pts',(-0.908404121959303,-48.1412914726861,
20.));
#72627=CARTESIAN_POINT('Ctrl Pts',(-0.941734211511966,-48.137628339932,
0.));
#72628=CARTESIAN_POINT('Ctrl Pts',(-0.941734211511966,-48.137628339932,
20.));
#72629=CARTESIAN_POINT('Ctrl Pts',(-0.975060642441261,-48.1339422136897,
0.));
#72630=CARTESIAN_POINT('Ctrl Pts',(-0.975060642441261,-48.1339422136897,
20.));
#72631=CARTESIAN_POINT('Ctrl Pts',(-1.00838339881034,-48.130233096591,0.));
#72632=CARTESIAN_POINT('Ctrl Pts',(-1.00838339881034,-48.130233096591,20.));
#72633=CARTESIAN_POINT('Ctrl Pts',(-1.04170246468366,-48.1265009912787,
0.));
#72634=CARTESIAN_POINT('Ctrl Pts',(-1.04170246468366,-48.1265009912787,
20.));
#72635=CARTESIAN_POINT('Ctrl Pts',(-1.0750178241273,-48.1227459004068,0.));
#72636=CARTESIAN_POINT('Ctrl Pts',(-1.0750178241273,-48.1227459004068,20.));
#72637=CARTESIAN_POINT('Ctrl Pts',(-1.10832946120863,-48.1189678266406,
0.));
#72638=CARTESIAN_POINT('Ctrl Pts',(-1.10832946120863,-48.1189678266406,
20.));
#72639=CARTESIAN_POINT('Ctrl Pts',(-1.14163735999659,-48.1151667726565,
0.));
#72640=CARTESIAN_POINT('Ctrl Pts',(-1.14163735999659,-48.1151667726565,
20.));
#72641=CARTESIAN_POINT('Ctrl Pts',(-1.17494150456147,-48.111342741142,0.));
#72642=CARTESIAN_POINT('Ctrl Pts',(-1.17494150456147,-48.111342741142,20.));
#72643=CARTESIAN_POINT('Ctrl Pts',(-1.20824187897491,-48.1074957347955,
0.));
#72644=CARTESIAN_POINT('Ctrl Pts',(-1.20824187897491,-48.1074957347955,
20.));
#72645=CARTESIAN_POINT('Ctrl Pts',(-1.24153846731024,-48.1036257563271,
0.));
#72646=CARTESIAN_POINT('Ctrl Pts',(-1.24153846731024,-48.1036257563271,
20.));
#72647=CARTESIAN_POINT('Ctrl Pts',(-1.27483125364217,-48.0997328084577,
0.));
#72648=CARTESIAN_POINT('Ctrl Pts',(-1.27483125364217,-48.0997328084577,
20.));
#72649=CARTESIAN_POINT('Ctrl Pts',(-1.30812022204706,-48.0958168939195,
0.));
#72650=CARTESIAN_POINT('Ctrl Pts',(-1.30812022204706,-48.0958168939195,
20.));
#72651=CARTESIAN_POINT('Ctrl Pts',(-1.34140535660262,-48.0918780154556,
0.));
#72652=CARTESIAN_POINT('Ctrl Pts',(-1.34140535660262,-48.0918780154556,
20.));
#72653=CARTESIAN_POINT('Ctrl Pts',(-1.37468664138803,-48.0879161758201,
0.));
#72654=CARTESIAN_POINT('Ctrl Pts',(-1.37468664138803,-48.0879161758201,
20.));
#72655=CARTESIAN_POINT('Ctrl Pts',(-1.40796406048389,-48.0839313777781,
0.));
#72656=CARTESIAN_POINT('Ctrl Pts',(-1.40796406048389,-48.0839313777781,
20.));
#72657=CARTESIAN_POINT('Ctrl Pts',(-1.44123759797226,-48.0799236241059,
0.));
#72658=CARTESIAN_POINT('Ctrl Pts',(-1.44123759797226,-48.0799236241059,
20.));
#72659=CARTESIAN_POINT('Ctrl Pts',(-1.47450723793683,-48.0758929175908,
0.));
#72660=CARTESIAN_POINT('Ctrl Pts',(-1.47450723793683,-48.0758929175908,
20.));
#72661=CARTESIAN_POINT('Ctrl Pts',(-1.50777296446293,-48.071839261032,0.));
#72662=CARTESIAN_POINT('Ctrl Pts',(-1.50777296446293,-48.071839261032,20.));
#72663=CARTESIAN_POINT('Ctrl Pts',(-1.54103476163745,-48.0677626572394,
0.));
#72664=CARTESIAN_POINT('Ctrl Pts',(-1.54103476163745,-48.0677626572394,
20.));
#72665=CARTESIAN_POINT('Ctrl Pts',(-1.57429261354891,-48.0636631090342,
0.));
#72666=CARTESIAN_POINT('Ctrl Pts',(-1.57429261354891,-48.0636631090342,
20.));
#72667=CARTESIAN_POINT('Ctrl Pts',(-1.60754650428747,-48.0595406192492,
0.));
#72668=CARTESIAN_POINT('Ctrl Pts',(-1.60754650428747,-48.0595406192492,
20.));
#72669=CARTESIAN_POINT('Ctrl Pts',(-1.64079641794463,-48.0553951907273,
0.));
#72670=CARTESIAN_POINT('Ctrl Pts',(-1.64079641794463,-48.0553951907273,
20.));
#72671=CARTESIAN_POINT('Ctrl Pts',(-1.67404233861339,-48.0512268263229,
0.));
#72672=CARTESIAN_POINT('Ctrl Pts',(-1.67404233861339,-48.0512268263229,
20.));
#72673=CARTESIAN_POINT('Ctrl Pts',(-1.70728425038806,-48.0470355289011,
0.));
#72674=CARTESIAN_POINT('Ctrl Pts',(-1.70728425038806,-48.0470355289011,
20.));
#72675=CARTESIAN_POINT('Ctrl Pts',(-1.74052213736473,-48.0428213013379,
0.));
#72676=CARTESIAN_POINT('Ctrl Pts',(-1.74052213736473,-48.0428213013379,
20.));
#72677=CARTESIAN_POINT('Ctrl Pts',(-1.77375598364111,-48.038584146521,0.));
#72678=CARTESIAN_POINT('Ctrl Pts',(-1.77375598364111,-48.038584146521,20.));
#72679=CARTESIAN_POINT('Ctrl Pts',(-1.80698577331665,-48.0343240673492,
0.));
#72680=CARTESIAN_POINT('Ctrl Pts',(-1.80698577331665,-48.0343240673492,
20.));
#72681=CARTESIAN_POINT('Ctrl Pts',(-1.84021149049247,-48.0300410667328,
0.));
#72682=CARTESIAN_POINT('Ctrl Pts',(-1.84021149049247,-48.0300410667328,
20.));
#72683=CARTESIAN_POINT('Ctrl Pts',(-1.87343311927143,-48.0257351475934,
0.));
#72684=CARTESIAN_POINT('Ctrl Pts',(-1.87343311927143,-48.0257351475934,
20.));
#72685=CARTESIAN_POINT('Ctrl Pts',(-1.90665064375788,-48.0214063128629,
0.));
#72686=CARTESIAN_POINT('Ctrl Pts',(-1.90665064375788,-48.0214063128629,
20.));
#72687=CARTESIAN_POINT('Ctrl Pts',(-1.93986404805774,-48.0170545654849,
0.));
#72688=CARTESIAN_POINT('Ctrl Pts',(-1.93986404805774,-48.0170545654849,
20.));
#72689=CARTESIAN_POINT('Ctrl Pts',(-1.97307331627851,-48.0126799084137,
0.));
#72690=CARTESIAN_POINT('Ctrl Pts',(-1.97307331627851,-48.0126799084137,
20.));
#72691=CARTESIAN_POINT('Ctrl Pts',(-2.00627843252927,-48.0082823446147,
0.));
#72692=CARTESIAN_POINT('Ctrl Pts',(-2.00627843252927,-48.0082823446147,
20.));
#72693=CARTESIAN_POINT('Ctrl Pts',(-2.03947938092069,-48.0038618770642,
0.));
#72694=CARTESIAN_POINT('Ctrl Pts',(-2.03947938092069,-48.0038618770642,
20.));
#72695=CARTESIAN_POINT('Ctrl Pts',(-2.07267614556538,-47.9994185087499,
0.));
#72696=CARTESIAN_POINT('Ctrl Pts',(-2.07267614556538,-47.9994185087499,
20.));
#72697=CARTESIAN_POINT('Ctrl Pts',(-2.1058687105775,-47.994952242671,0.));
#72698=CARTESIAN_POINT('Ctrl Pts',(-2.1058687105775,-47.994952242671,20.));
#72699=CARTESIAN_POINT('Ctrl Pts',(-2.13905706007287,-47.9904630818375,
0.));
#72700=CARTESIAN_POINT('Ctrl Pts',(-2.13905706007287,-47.9904630818375,
20.));
#72701=CARTESIAN_POINT('Ctrl Pts',(-2.172241178169,-47.9859510292704,0.));
#72702=CARTESIAN_POINT('Ctrl Pts',(-2.172241178169,-47.9859510292704,20.));
#72703=CARTESIAN_POINT('Ctrl Pts',(-2.20542104898522,-47.9814160880019,
0.));
#72704=CARTESIAN_POINT('Ctrl Pts',(-2.20542104898522,-47.9814160880019,
20.));
#72705=CARTESIAN_POINT('Ctrl Pts',(-2.23859665664241,-47.9768582610752,
0.));
#72706=CARTESIAN_POINT('Ctrl Pts',(-2.23859665664241,-47.9768582610752,
20.));
#72707=CARTESIAN_POINT('Ctrl Pts',(-2.27176798526354,-47.9722775515452,
0.));
#72708=CARTESIAN_POINT('Ctrl Pts',(-2.27176798526354,-47.9722775515452,
20.));
#72709=CARTESIAN_POINT('Ctrl Pts',(-2.30493501897296,-47.9676739624772,
0.));
#72710=CARTESIAN_POINT('Ctrl Pts',(-2.30493501897296,-47.9676739624772,
20.));
#72711=CARTESIAN_POINT('Ctrl Pts',(-2.33809774189659,-47.9630474969481,
0.));
#72712=CARTESIAN_POINT('Ctrl Pts',(-2.33809774189659,-47.9630474969481,
20.));
#72713=CARTESIAN_POINT('Ctrl Pts',(-2.37125613816232,-47.9583981580454,
0.));
#72714=CARTESIAN_POINT('Ctrl Pts',(-2.37125613816232,-47.9583981580454,
20.));
#72715=CARTESIAN_POINT('Ctrl Pts',(-2.40441019189961,-47.9537259488681,
0.));
#72716=CARTESIAN_POINT('Ctrl Pts',(-2.40441019189961,-47.9537259488681,
20.));
#72717=CARTESIAN_POINT('Ctrl Pts',(-2.43755988723967,-47.9490308725257,
0.));
#72718=CARTESIAN_POINT('Ctrl Pts',(-2.43755988723967,-47.9490308725257,
20.));
#72719=CARTESIAN_POINT('Ctrl Pts',(-2.4707052083155,-47.9443129321394,0.));
#72720=CARTESIAN_POINT('Ctrl Pts',(-2.4707052083155,-47.9443129321394,20.));
#72721=CARTESIAN_POINT('Ctrl Pts',(-2.5038461392621,-47.9395721308414,0.));
#72722=CARTESIAN_POINT('Ctrl Pts',(-2.5038461392621,-47.9395721308414,20.));
#72723=CARTESIAN_POINT('Ctrl Pts',(-2.53698266421615,-47.9348084717752,
0.));
#72724=CARTESIAN_POINT('Ctrl Pts',(-2.53698266421615,-47.9348084717752,
20.));
#72725=CARTESIAN_POINT('Ctrl Pts',(-2.57011476731624,-47.9300219580955,
0.));
#72726=CARTESIAN_POINT('Ctrl Pts',(-2.57011476731624,-47.9300219580955,
20.));
#72727=CARTESIAN_POINT('Ctrl Pts',(-2.60324243270259,-47.9252125929679,
0.));
#72728=CARTESIAN_POINT('Ctrl Pts',(-2.60324243270259,-47.9252125929679,
20.));
#72729=CARTESIAN_POINT('Ctrl Pts',(-2.6363656445172,-47.9203803795688,0.));
#72730=CARTESIAN_POINT('Ctrl Pts',(-2.6363656445172,-47.9203803795688,20.));
#72731=CARTESIAN_POINT('Ctrl Pts',(-2.66948438690367,-47.9155253210858,
0.));
#72732=CARTESIAN_POINT('Ctrl Pts',(-2.66948438690367,-47.9155253210858,
20.));
#72733=CARTESIAN_POINT('Ctrl Pts',(-2.70259864400759,-47.9106474207177,
0.));
#72734=CARTESIAN_POINT('Ctrl Pts',(-2.70259864400759,-47.9106474207177,
20.));
#72735=CARTESIAN_POINT('Ctrl Pts',(-2.7357083999763,-47.9057466816743,0.));
#72736=CARTESIAN_POINT('Ctrl Pts',(-2.7357083999763,-47.9057466816743,20.));
#72737=CARTESIAN_POINT('Ctrl Pts',(-2.76881363895919,-47.9008231071768,
0.));
#72738=CARTESIAN_POINT('Ctrl Pts',(-2.76881363895919,-47.9008231071768,
20.));
#72739=CARTESIAN_POINT('Ctrl Pts',(-2.80191434510735,-47.8958767004573,
0.));
#72740=CARTESIAN_POINT('Ctrl Pts',(-2.80191434510735,-47.8958767004573,
20.));
#72741=CARTESIAN_POINT('Ctrl Pts',(-2.83501050257377,-47.8909074647592,
0.));
#72742=CARTESIAN_POINT('Ctrl Pts',(-2.83501050257377,-47.8909074647592,
20.));
#72743=CARTESIAN_POINT('Ctrl Pts',(-2.86810209551309,-47.8859154033363,
0.));
#72744=CARTESIAN_POINT('Ctrl Pts',(-2.86810209551309,-47.8859154033363,
20.));
#72745=CARTESIAN_POINT('Ctrl Pts',(-2.90118910808201,-47.8809005194543,
0.));
#72746=CARTESIAN_POINT('Ctrl Pts',(-2.90118910808201,-47.8809005194543,
20.));
#72747=CARTESIAN_POINT('Ctrl Pts',(-2.93427152443919,-47.8758628163901,
0.));
#72748=CARTESIAN_POINT('Ctrl Pts',(-2.93427152443919,-47.8758628163901,
20.));
#72749=CARTESIAN_POINT('Ctrl Pts',(-2.96734932874506,-47.8708022974315,
0.));
#72750=CARTESIAN_POINT('Ctrl Pts',(-2.96734932874506,-47.8708022974315,
20.));
#72751=CARTESIAN_POINT('Ctrl Pts',(-3.00042250516194,-47.8657189658771,
0.));
#72752=CARTESIAN_POINT('Ctrl Pts',(-3.00042250516194,-47.8657189658771,
20.));
#72753=CARTESIAN_POINT('Ctrl Pts',(-3.03349103785389,-47.8606128250365,
0.));
#72754=CARTESIAN_POINT('Ctrl Pts',(-3.03349103785389,-47.8606128250365,
20.));
#72755=CARTESIAN_POINT('Ctrl Pts',(-3.06655491098683,-47.8554838782302,
0.));
#72756=CARTESIAN_POINT('Ctrl Pts',(-3.06655491098683,-47.8554838782302,
20.));
#72757=CARTESIAN_POINT('Ctrl Pts',(-3.09961410872877,-47.8503321287903,
0.));
#72758=CARTESIAN_POINT('Ctrl Pts',(-3.09961410872877,-47.8503321287903,
20.));
#72759=CARTESIAN_POINT('Ctrl Pts',(-3.13266861524955,-47.8451575800601,
0.));
#72760=CARTESIAN_POINT('Ctrl Pts',(-3.13266861524955,-47.8451575800601,
20.));
#72761=CARTESIAN_POINT('Ctrl Pts',(-3.16571841472091,-47.8399602353939,
0.));
#72762=CARTESIAN_POINT('Ctrl Pts',(-3.16571841472091,-47.8399602353939,
20.));
#72763=CARTESIAN_POINT('Ctrl Pts',(-3.19876349131676,-47.834740098157,0.));
#72764=CARTESIAN_POINT('Ctrl Pts',(-3.19876349131676,-47.834740098157,20.));
#72765=CARTESIAN_POINT('Ctrl Pts',(-3.23180382921274,-47.829497171726,0.));
#72766=CARTESIAN_POINT('Ctrl Pts',(-3.23180382921274,-47.829497171726,20.));
#72767=CARTESIAN_POINT('Ctrl Pts',(-3.26483941258678,-47.8242314594881,
0.));
#72768=CARTESIAN_POINT('Ctrl Pts',(-3.26483941258678,-47.8242314594881,
20.));
#72769=CARTESIAN_POINT('Ctrl Pts',(-3.29787022561837,-47.818942964842,0.));
#72770=CARTESIAN_POINT('Ctrl Pts',(-3.29787022561837,-47.818942964842,20.));
#72771=CARTESIAN_POINT('Ctrl Pts',(-3.33089625248904,-47.813631691197,0.));
#72772=CARTESIAN_POINT('Ctrl Pts',(-3.33089625248904,-47.813631691197,20.));
#72773=CARTESIAN_POINT('Ctrl Pts',(-3.36391747738215,-47.8082976419741,
0.));
#72774=CARTESIAN_POINT('Ctrl Pts',(-3.36391747738215,-47.8082976419741,
20.));
#72775=CARTESIAN_POINT('Ctrl Pts',(-3.39693388448307,-47.802940820605,0.));
#72776=CARTESIAN_POINT('Ctrl Pts',(-3.39693388448307,-47.802940820605,20.));
#72777=CARTESIAN_POINT('Ctrl Pts',(-3.42994545797923,-47.797561230533,0.));
#72778=CARTESIAN_POINT('Ctrl Pts',(-3.42994545797923,-47.797561230533,20.));
#72779=CARTESIAN_POINT('Ctrl Pts',(-3.46295218206013,-47.7921588752121,
0.));
#72780=CARTESIAN_POINT('Ctrl Pts',(-3.46295218206013,-47.7921588752121,
20.));
#72781=CARTESIAN_POINT('Ctrl Pts',(-3.49595404091729,-47.7867337581073,
0.));
#72782=CARTESIAN_POINT('Ctrl Pts',(-3.49595404091729,-47.7867337581073,
20.));
#72783=CARTESIAN_POINT('Ctrl Pts',(-3.52895101874416,-47.7812858826946,
0.));
#72784=CARTESIAN_POINT('Ctrl Pts',(-3.52895101874416,-47.7812858826946,
20.));
#72785=CARTESIAN_POINT('Ctrl Pts',(-3.56194309973643,-47.7758152524613,
0.));
#72786=CARTESIAN_POINT('Ctrl Pts',(-3.56194309973643,-47.7758152524613,
20.));
#72787=CARTESIAN_POINT('Ctrl Pts',(-3.59493026809159,-47.7703218709055,
0.));
#72788=CARTESIAN_POINT('Ctrl Pts',(-3.59493026809159,-47.7703218709055,
20.));
#72789=CARTESIAN_POINT('Ctrl Pts',(-3.62791250800925,-47.764805741537,0.));
#72790=CARTESIAN_POINT('Ctrl Pts',(-3.62791250800925,-47.764805741537,20.));
#72791=CARTESIAN_POINT('Ctrl Pts',(-3.66088980369085,-47.7592668678762,
0.));
#72792=CARTESIAN_POINT('Ctrl Pts',(-3.66088980369085,-47.7592668678762,
20.));
#72793=CARTESIAN_POINT('Ctrl Pts',(-3.69386213933995,-47.7537052534546,
0.));
#72794=CARTESIAN_POINT('Ctrl Pts',(-3.69386213933995,-47.7537052534546,
20.));
#72795=CARTESIAN_POINT('Ctrl Pts',(-3.72682949916223,-47.7481209018149,
0.));
#72796=CARTESIAN_POINT('Ctrl Pts',(-3.72682949916223,-47.7481209018149,
20.));
#72797=CARTESIAN_POINT('Ctrl Pts',(-3.75979186736546,-47.7425138165111,
0.));
#72798=CARTESIAN_POINT('Ctrl Pts',(-3.75979186736546,-47.7425138165111,
20.));
#72799=CARTESIAN_POINT('Ctrl Pts',(-3.7927492281595,-47.7368840011081,0.));
#72800=CARTESIAN_POINT('Ctrl Pts',(-3.7927492281595,-47.7368840011081,20.));
#72801=CARTESIAN_POINT('Ctrl Pts',(-3.82570156575624,-47.7312314591817,
0.));
#72802=CARTESIAN_POINT('Ctrl Pts',(-3.82570156575624,-47.7312314591817,
20.));
#72803=CARTESIAN_POINT('Ctrl Pts',(-3.85864886436974,-47.7255561943191,
0.));
#72804=CARTESIAN_POINT('Ctrl Pts',(-3.85864886436974,-47.7255561943191,
20.));
#72805=CARTESIAN_POINT('Ctrl Pts',(-3.89159110821606,-47.719858210118,0.));
#72806=CARTESIAN_POINT('Ctrl Pts',(-3.89159110821606,-47.719858210118,20.));
#72807=CARTESIAN_POINT('Ctrl Pts',(-3.92452828151334,-47.7141375101875,
0.));
#72808=CARTESIAN_POINT('Ctrl Pts',(-3.92452828151334,-47.7141375101875,
20.));
#72809=CARTESIAN_POINT('Ctrl Pts',(-3.95746036848188,-47.7083940981477,
0.));
#72810=CARTESIAN_POINT('Ctrl Pts',(-3.95746036848188,-47.7083940981477,
20.));
#72811=CARTESIAN_POINT('Ctrl Pts',(-3.99038735334402,-47.7026279776294,
0.));
#72812=CARTESIAN_POINT('Ctrl Pts',(-3.99038735334402,-47.7026279776294,
20.));
#72813=CARTESIAN_POINT('Ctrl Pts',(-4.02330922032434,-47.6968391522753,
0.));
#72814=CARTESIAN_POINT('Ctrl Pts',(-4.02330922032434,-47.6968391522753,
20.));
#72815=CARTESIAN_POINT('Ctrl Pts',(-4.05622595364953,-47.6910276257391,
0.));
#72816=CARTESIAN_POINT('Ctrl Pts',(-4.05622595364953,-47.6910276257391,
20.));
#72817=CARTESIAN_POINT('Ctrl Pts',(-4.0891375375485,-47.6851934016861,0.));
#72818=CARTESIAN_POINT('Ctrl Pts',(-4.0891375375485,-47.6851934016861,20.));
#72819=CARTESIAN_POINT('Ctrl Pts',(-4.1220439562522,-47.6793364837921,0.));
#72820=CARTESIAN_POINT('Ctrl Pts',(-4.1220439562522,-47.6793364837921,20.));
#72821=CARTESIAN_POINT('Ctrl Pts',(-4.15494519399371,-47.6734568757434,
0.));
#72822=CARTESIAN_POINT('Ctrl Pts',(-4.15494519399371,-47.6734568757434,
20.));
#72823=CARTESIAN_POINT('Ctrl Pts',(-4.18784123500837,-47.6675545812371,
0.));
#72824=CARTESIAN_POINT('Ctrl Pts',(-4.18784123500837,-47.6675545812371,
20.));
#72825=CARTESIAN_POINT('Ctrl Pts',(-4.22073206353346,-47.6616296039816,
0.));
#72826=CARTESIAN_POINT('Ctrl Pts',(-4.22073206353346,-47.6616296039816,
20.));
#72827=CARTESIAN_POINT('Ctrl Pts',(-4.25361766380861,-47.6556819476964,
0.));
#72828=CARTESIAN_POINT('Ctrl Pts',(-4.25361766380861,-47.6556819476964,
20.));
#72829=CARTESIAN_POINT('Ctrl Pts',(-4.28649802007568,-47.6497116161128,
0.));
#72830=CARTESIAN_POINT('Ctrl Pts',(-4.28649802007568,-47.6497116161128,
20.));
#72831=CARTESIAN_POINT('Ctrl Pts',(-4.31937311657887,-47.6437186129734,
0.));
#72832=CARTESIAN_POINT('Ctrl Pts',(-4.31937311657887,-47.6437186129734,
20.));
#72833=CARTESIAN_POINT('Ctrl Pts',(-4.35224293756441,-47.6377029420315,
0.));
#72834=CARTESIAN_POINT('Ctrl Pts',(-4.35224293756441,-47.6377029420315,
20.));
#72835=CARTESIAN_POINT('Ctrl Pts',(-4.38510746728076,-47.6316646070511,
0.));
#72836=CARTESIAN_POINT('Ctrl Pts',(-4.38510746728076,-47.6316646070511,
20.));
#72837=CARTESIAN_POINT('Ctrl Pts',(-4.41796668997837,-47.6256036118071,
0.));
#72838=CARTESIAN_POINT('Ctrl Pts',(-4.41796668997837,-47.6256036118071,
20.));
#72839=CARTESIAN_POINT('Ctrl Pts',(-4.45082058991005,-47.6195199600851,
0.));
#72840=CARTESIAN_POINT('Ctrl Pts',(-4.45082058991005,-47.6195199600851,
20.));
#72841=CARTESIAN_POINT('Ctrl Pts',(-4.48366915133085,-47.6134136556823,
0.));
#72842=CARTESIAN_POINT('Ctrl Pts',(-4.48366915133085,-47.6134136556823,
20.));
#72843=CARTESIAN_POINT('Ctrl Pts',(-4.51651235849824,-47.6072847024073,
0.));
#72844=CARTESIAN_POINT('Ctrl Pts',(-4.51651235849824,-47.6072847024073,
20.));
#72845=CARTESIAN_POINT('Ctrl Pts',(-4.54935019567199,-47.6011331040799,
0.));
#72846=CARTESIAN_POINT('Ctrl Pts',(-4.54935019567199,-47.6011331040799,
20.));
#72847=CARTESIAN_POINT('Ctrl Pts',(-4.5821826471142,-47.5949588645311,0.));
#72848=CARTESIAN_POINT('Ctrl Pts',(-4.5821826471142,-47.5949588645311,20.));
#72849=CARTESIAN_POINT('Ctrl Pts',(-4.61500969708897,-47.5887619876026,
0.));
#72850=CARTESIAN_POINT('Ctrl Pts',(-4.61500969708897,-47.5887619876026,
20.));
#72851=CARTESIAN_POINT('Ctrl Pts',(-4.64783132986261,-47.5825424771468,
0.));
#72852=CARTESIAN_POINT('Ctrl Pts',(-4.64783132986261,-47.5825424771468,
20.));
#72853=CARTESIAN_POINT('Ctrl Pts',(-4.68064752970371,-47.5763003370265,
0.));
#72854=CARTESIAN_POINT('Ctrl Pts',(-4.68064752970371,-47.5763003370265,
20.));
#72855=CARTESIAN_POINT('Ctrl Pts',(-4.7134582808831,-47.5700355711162,0.));
#72856=CARTESIAN_POINT('Ctrl Pts',(-4.7134582808831,-47.5700355711162,20.));
#72857=CARTESIAN_POINT('Ctrl Pts',(-4.74626356767414,-47.5637481833017,
0.));
#72858=CARTESIAN_POINT('Ctrl Pts',(-4.74626356767414,-47.5637481833017,
20.));
#72859=CARTESIAN_POINT('Ctrl Pts',(-4.77906337435245,-47.5574381774801,
0.));
#72860=CARTESIAN_POINT('Ctrl Pts',(-4.77906337435245,-47.5574381774801,
20.));
#72861=CARTESIAN_POINT('Ctrl Pts',(-4.8118576851959,-47.5511055575592,0.));
#72862=CARTESIAN_POINT('Ctrl Pts',(-4.8118576851959,-47.5511055575592,20.));
#72863=CARTESIAN_POINT('Ctrl Pts',(-4.84464648448476,-47.5447503274583,
0.));
#72864=CARTESIAN_POINT('Ctrl Pts',(-4.84464648448476,-47.5447503274583,
20.));
#72865=CARTESIAN_POINT('Ctrl Pts',(-4.87742975650163,-47.538372491107,0.));
#72866=CARTESIAN_POINT('Ctrl Pts',(-4.87742975650163,-47.538372491107,20.));
#72867=CARTESIAN_POINT('Ctrl Pts',(-4.91020748553146,-47.5319720524462,
0.));
#72868=CARTESIAN_POINT('Ctrl Pts',(-4.91020748553146,-47.5319720524462,
20.));
#72869=CARTESIAN_POINT('Ctrl Pts',(-4.94297965586158,-47.5255490154281,
0.));
#72870=CARTESIAN_POINT('Ctrl Pts',(-4.94297965586158,-47.5255490154281,
20.));
#72871=CARTESIAN_POINT('Ctrl Pts',(-4.97574625178171,-47.519103384016,0.));
#72872=CARTESIAN_POINT('Ctrl Pts',(-4.97574625178171,-47.519103384016,20.));
#72873=CARTESIAN_POINT('Ctrl Pts',(-5.00850725758369,-47.5126351621839,
0.));
#72874=CARTESIAN_POINT('Ctrl Pts',(-5.00850725758369,-47.5126351621839,
20.));
#72875=CARTESIAN_POINT('Ctrl Pts',(-5.04126265756156,-47.5061443539168,
0.));
#72876=CARTESIAN_POINT('Ctrl Pts',(-5.04126265756156,-47.5061443539168,
20.));
#72877=CARTESIAN_POINT('Ctrl Pts',(-5.074012436012,-47.4996309632108,0.));
#72878=CARTESIAN_POINT('Ctrl Pts',(-5.074012436012,-47.4996309632108,20.));
#72879=CARTESIAN_POINT('Ctrl Pts',(-5.10675657723404,-47.4930949940731,
0.));
#72880=CARTESIAN_POINT('Ctrl Pts',(-5.10675657723404,-47.4930949940731,
20.));
#72881=CARTESIAN_POINT('Ctrl Pts',(-5.13949506552924,-47.4865364505219,
0.));
#72882=CARTESIAN_POINT('Ctrl Pts',(-5.13949506552924,-47.4865364505219,
20.));
#72883=CARTESIAN_POINT('Ctrl Pts',(-5.17222788520145,-47.4799553365862,
0.));
#72884=CARTESIAN_POINT('Ctrl Pts',(-5.17222788520145,-47.4799553365862,
20.));
#72885=CARTESIAN_POINT('Ctrl Pts',(-5.20495502055715,-47.4733516563069,
0.));
#72886=CARTESIAN_POINT('Ctrl Pts',(-5.20495502055715,-47.4733516563069,
20.));
#72887=CARTESIAN_POINT('Ctrl Pts',(-5.23767645590512,-47.4667254137359,
0.));
#72888=CARTESIAN_POINT('Ctrl Pts',(-5.23767645590512,-47.4667254137359,
20.));
#72889=CARTESIAN_POINT('Ctrl Pts',(-5.27039217555657,-47.4600766129357,
0.));
#72890=CARTESIAN_POINT('Ctrl Pts',(-5.27039217555657,-47.4600766129357,
20.));
#72891=CARTESIAN_POINT('Ctrl Pts',(-5.30310216382507,-47.4534052579797,
0.));
#72892=CARTESIAN_POINT('Ctrl Pts',(-5.30310216382507,-47.4534052579797,
20.));
#72893=CARTESIAN_POINT('Ctrl Pts',(-5.33580640502662,-47.4467113529523,
0.));
#72894=CARTESIAN_POINT('Ctrl Pts',(-5.33580640502662,-47.4467113529523,
20.));
#72895=CARTESIAN_POINT('Ctrl Pts',(-5.36850488347925,-47.4399949019487,
0.));
#72896=CARTESIAN_POINT('Ctrl Pts',(-5.36850488347925,-47.4399949019487,
20.));
#72897=CARTESIAN_POINT('Ctrl Pts',(-5.4011975835038,-47.4332559090748,0.));
#72898=CARTESIAN_POINT('Ctrl Pts',(-5.4011975835038,-47.4332559090748,20.));
#72899=CARTESIAN_POINT('Ctrl Pts',(-5.43388448942351,-47.4264943784481,
0.));
#72900=CARTESIAN_POINT('Ctrl Pts',(-5.43388448942351,-47.4264943784481,
20.));
#72901=CARTESIAN_POINT('Ctrl Pts',(-5.46656558556427,-47.4197103141976,
0.));
#72902=CARTESIAN_POINT('Ctrl Pts',(-5.46656558556427,-47.4197103141976,
20.));
#72903=CARTESIAN_POINT('Ctrl Pts',(-5.49924085625465,-47.4129037204631,
0.));
#72904=CARTESIAN_POINT('Ctrl Pts',(-5.49924085625465,-47.4129037204631,
20.));
#72905=CARTESIAN_POINT('Ctrl Pts',(-5.53191028582555,-47.4060746013959,
0.));
#72906=CARTESIAN_POINT('Ctrl Pts',(-5.53191028582555,-47.4060746013959,
20.));
#72907=CARTESIAN_POINT('Ctrl Pts',(-5.56457385861038,-47.3992229611579,
0.));
#72908=CARTESIAN_POINT('Ctrl Pts',(-5.56457385861038,-47.3992229611579,
20.));
#72909=CARTESIAN_POINT('Ctrl Pts',(-5.59723155894484,-47.3923488039217,
0.));
#72910=CARTESIAN_POINT('Ctrl Pts',(-5.59723155894484,-47.3923488039217,
20.));
#72911=CARTESIAN_POINT('Ctrl Pts',(-5.62988337116716,-47.3854521338708,
0.));
#72912=CARTESIAN_POINT('Ctrl Pts',(-5.62988337116716,-47.3854521338708,
20.));
#72913=CARTESIAN_POINT('Ctrl Pts',(-5.66252927961812,-47.3785329551997,
0.));
#72914=CARTESIAN_POINT('Ctrl Pts',(-5.66252927961812,-47.3785329551997,
20.));
#72915=CARTESIAN_POINT('Ctrl Pts',(-5.69516926864089,-47.3715912721141,
0.));
#72916=CARTESIAN_POINT('Ctrl Pts',(-5.69516926864089,-47.3715912721141,
20.));
#72917=CARTESIAN_POINT('Ctrl Pts',(-5.72780332258136,-47.3646270888308,
0.));
#72918=CARTESIAN_POINT('Ctrl Pts',(-5.72780332258136,-47.3646270888308,
20.));
#72919=CARTESIAN_POINT('Ctrl Pts',(-5.76043142578787,-47.3576404095777,
0.));
#72920=CARTESIAN_POINT('Ctrl Pts',(-5.76043142578787,-47.3576404095777,
20.));
#72921=CARTESIAN_POINT('Ctrl Pts',(-5.79305356261143,-47.3506312385939,
0.));
#72922=CARTESIAN_POINT('Ctrl Pts',(-5.79305356261143,-47.3506312385939,
20.));
#72923=CARTESIAN_POINT('Ctrl Pts',(-5.82566971740557,-47.3435995801292,
0.));
#72924=CARTESIAN_POINT('Ctrl Pts',(-5.82566971740557,-47.3435995801292,
20.));
#72925=CARTESIAN_POINT('Ctrl Pts',(-5.85827987452641,-47.3365454384446,
0.));
#72926=CARTESIAN_POINT('Ctrl Pts',(-5.85827987452641,-47.3365454384446,
20.));
#72927=CARTESIAN_POINT('Ctrl Pts',(-5.89088401833278,-47.3294688178121,
0.));
#72928=CARTESIAN_POINT('Ctrl Pts',(-5.89088401833278,-47.3294688178121,
20.));
#72929=CARTESIAN_POINT('Ctrl Pts',(-5.92348213318599,-47.3223697225143,
0.));
#72930=CARTESIAN_POINT('Ctrl Pts',(-5.92348213318599,-47.3223697225143,
20.));
#72931=CARTESIAN_POINT('Ctrl Pts',(-5.95607420344987,-47.3152481568452,
0.));
#72932=CARTESIAN_POINT('Ctrl Pts',(-5.95607420344987,-47.3152481568452,
20.));
#72933=CARTESIAN_POINT('Ctrl Pts',(-5.98866021349068,-47.3081041251096,
0.));
#72934=CARTESIAN_POINT('Ctrl Pts',(-5.98866021349068,-47.3081041251096,
20.));
#72935=CARTESIAN_POINT('Ctrl Pts',(-6.02124014767731,-47.3009376316237,
0.));
#72936=CARTESIAN_POINT('Ctrl Pts',(-6.02124014767731,-47.3009376316237,
20.));
#72937=CARTESIAN_POINT('Ctrl Pts',(-6.0538139903813,-47.2937486807145,0.));
#72938=CARTESIAN_POINT('Ctrl Pts',(-6.0538139903813,-47.2937486807145,20.));
#72939=CARTESIAN_POINT('Ctrl Pts',(-6.08638172597685,-47.2865372767199,
0.));
#72940=CARTESIAN_POINT('Ctrl Pts',(-6.08638172597685,-47.2865372767199,
20.));
#72941=CARTESIAN_POINT('Ctrl Pts',(-6.11894333884089,-47.2793034239892,
0.));
#72942=CARTESIAN_POINT('Ctrl Pts',(-6.11894333884089,-47.2793034239892,
20.));
#72943=CARTESIAN_POINT('Ctrl Pts',(-6.15149881335291,-47.272047126882,0.));
#72944=CARTESIAN_POINT('Ctrl Pts',(-6.15149881335291,-47.272047126882,20.));
#72945=CARTESIAN_POINT('Ctrl Pts',(-6.1840481338953,-47.2647683897693,0.));
#72946=CARTESIAN_POINT('Ctrl Pts',(-6.1840481338953,-47.2647683897693,20.));
#72947=CARTESIAN_POINT('Ctrl Pts',(-6.21659128485297,-47.2574672170331,
0.));
#72948=CARTESIAN_POINT('Ctrl Pts',(-6.21659128485297,-47.2574672170331,
20.));
#72949=CARTESIAN_POINT('Ctrl Pts',(-6.24912825061344,-47.2501436130661,
0.));
#72950=CARTESIAN_POINT('Ctrl Pts',(-6.24912825061344,-47.2501436130661,
20.));
#72951=CARTESIAN_POINT('Ctrl Pts',(-6.28165901556677,-47.2427975822723,
0.));
#72952=CARTESIAN_POINT('Ctrl Pts',(-6.28165901556677,-47.2427975822723,
20.));
#72953=CARTESIAN_POINT('Ctrl Pts',(-6.31418356410551,-47.2354291290667,
0.));
#72954=CARTESIAN_POINT('Ctrl Pts',(-6.31418356410551,-47.2354291290667,
20.));
#72955=CARTESIAN_POINT('Ctrl Pts',(-6.34670188062517,-47.2280382578755,
0.));
#72956=CARTESIAN_POINT('Ctrl Pts',(-6.34670188062517,-47.2280382578755,
20.));
#72957=CARTESIAN_POINT('Ctrl Pts',(-6.37921394952381,-47.2206249731358,
0.));
#72958=CARTESIAN_POINT('Ctrl Pts',(-6.37921394952381,-47.2206249731358,
20.));
#72959=CARTESIAN_POINT('Ctrl Pts',(-6.41171975520235,-47.213189279296,0.));
#72960=CARTESIAN_POINT('Ctrl Pts',(-6.41171975520235,-47.213189279296,20.));
#72961=CARTESIAN_POINT('Ctrl Pts',(-6.44421928206447,-47.205731180815,0.));
#72962=CARTESIAN_POINT('Ctrl Pts',(-6.44421928206447,-47.205731180815,20.));
#72963=CARTESIAN_POINT('Ctrl Pts',(-6.47671251451639,-47.1982506821625,
0.));
#72964=CARTESIAN_POINT('Ctrl Pts',(-6.47671251451639,-47.1982506821625,
20.));
#72965=CARTESIAN_POINT('Ctrl Pts',(-6.50919943696718,-47.190747787819,0.));
#72966=CARTESIAN_POINT('Ctrl Pts',(-6.50919943696718,-47.190747787819,20.));
#72967=CARTESIAN_POINT('Ctrl Pts',(-6.54168003382863,-47.1832225022762,
0.));
#72968=CARTESIAN_POINT('Ctrl Pts',(-6.54168003382863,-47.1832225022762,
20.));
#72969=CARTESIAN_POINT('Ctrl Pts',(-6.57415428951526,-47.1756748300372,
0.));
#72970=CARTESIAN_POINT('Ctrl Pts',(-6.57415428951526,-47.1756748300372,
20.));
#72971=CARTESIAN_POINT('Ctrl Pts',(-6.60662218844436,-47.168104775616,0.));
#72972=CARTESIAN_POINT('Ctrl Pts',(-6.60662218844436,-47.168104775616,20.));
#72973=CARTESIAN_POINT('Ctrl Pts',(-6.63908371503578,-47.1605123435378,
0.));
#72974=CARTESIAN_POINT('Ctrl Pts',(-6.63908371503578,-47.1605123435378,
20.));
#72975=CARTESIAN_POINT('Ctrl Pts',(-6.67153885371228,-47.1528975383387,
0.));
#72976=CARTESIAN_POINT('Ctrl Pts',(-6.67153885371228,-47.1528975383387,
20.));
#72977=CARTESIAN_POINT('Ctrl Pts',(-6.70398758889918,-47.1452603645656,
0.));
#72978=CARTESIAN_POINT('Ctrl Pts',(-6.70398758889918,-47.1452603645656,
20.));
#72979=CARTESIAN_POINT('Ctrl Pts',(-6.7364299050246,-47.1376008267758,0.));
#72980=CARTESIAN_POINT('Ctrl Pts',(-6.7364299050246,-47.1376008267758,20.));
#72981=CARTESIAN_POINT('Ctrl Pts',(-6.76886578651956,-47.129918929538,0.));
#72982=CARTESIAN_POINT('Ctrl Pts',(-6.76886578651956,-47.129918929538,20.));
#72983=CARTESIAN_POINT('Ctrl Pts',(-6.80129521781809,-47.1222146774323,
0.));
#72984=CARTESIAN_POINT('Ctrl Pts',(-6.80129521781809,-47.1222146774323,
20.));
#72985=CARTESIAN_POINT('Ctrl Pts',(-6.83371818335699,-47.1144880750497,
0.));
#72986=CARTESIAN_POINT('Ctrl Pts',(-6.83371818335699,-47.1144880750497,
20.));
#72987=CARTESIAN_POINT('Ctrl Pts',(-6.8661346675759,-47.1067391269919,0.));
#72988=CARTESIAN_POINT('Ctrl Pts',(-6.8661346675759,-47.1067391269919,20.));
#72989=CARTESIAN_POINT('Ctrl Pts',(-6.89854465491704,-47.0989678378717,
0.));
#72990=CARTESIAN_POINT('Ctrl Pts',(-6.89854465491704,-47.0989678378717,
20.));
#72991=CARTESIAN_POINT('Ctrl Pts',(-6.93094812982543,-47.0911742123123,
0.));
#72992=CARTESIAN_POINT('Ctrl Pts',(-6.93094812982543,-47.0911742123123,
20.));
#72993=CARTESIAN_POINT('Ctrl Pts',(-6.96334507674875,-47.0833582549484,
0.));
#72994=CARTESIAN_POINT('Ctrl Pts',(-6.96334507674875,-47.0833582549484,
20.));
#72995=CARTESIAN_POINT('Ctrl Pts',(-6.99573548013778,-47.0755199704256,
0.));
#72996=CARTESIAN_POINT('Ctrl Pts',(-6.99573548013778,-47.0755199704256,
20.));
#72997=CARTESIAN_POINT('Ctrl Pts',(-7.02811932444603,-47.0676593634011,
0.));
#72998=CARTESIAN_POINT('Ctrl Pts',(-7.02811932444603,-47.0676593634011,
20.));
#72999=CARTESIAN_POINT('Ctrl Pts',(-7.06049659413009,-47.0597764385426,
0.));
#73000=CARTESIAN_POINT('Ctrl Pts',(-7.06049659413009,-47.0597764385426,
20.));
#73001=CARTESIAN_POINT('Ctrl Pts',(-7.09286727364934,-47.0518712005288,
0.));
#73002=CARTESIAN_POINT('Ctrl Pts',(-7.09286727364934,-47.0518712005288,
20.));
#73003=CARTESIAN_POINT('Ctrl Pts',(-7.12523134746605,-47.0439436540493,
0.));
#73004=CARTESIAN_POINT('Ctrl Pts',(-7.12523134746605,-47.0439436540493,
20.));
#73005=CARTESIAN_POINT('Ctrl Pts',(-7.15758880004523,-47.0359938038039,
0.));
#73006=CARTESIAN_POINT('Ctrl Pts',(-7.15758880004523,-47.0359938038039,
20.));
#73007=CARTESIAN_POINT('Ctrl Pts',(-7.18993961585471,-47.0280216545038,
0.));
#73008=CARTESIAN_POINT('Ctrl Pts',(-7.18993961585471,-47.0280216545038,
20.));
#73009=CARTESIAN_POINT('Ctrl Pts',(-7.22228377936531,-47.020027210871,0.));
#73010=CARTESIAN_POINT('Ctrl Pts',(-7.22228377936531,-47.020027210871,20.));
#73011=CARTESIAN_POINT('Ctrl Pts',(-7.25462127505078,-47.012010477639,0.));
#73012=CARTESIAN_POINT('Ctrl Pts',(-7.25462127505078,-47.012010477639,20.));
#73013=CARTESIAN_POINT('Ctrl Pts',(-7.28695208738785,-47.0039714595526,
0.));
#73014=CARTESIAN_POINT('Ctrl Pts',(-7.28695208738785,-47.0039714595526,
20.));
#73015=CARTESIAN_POINT('Ctrl Pts',(-7.31927620085615,-46.9959101613675,
0.));
#73016=CARTESIAN_POINT('Ctrl Pts',(-7.31927620085615,-46.9959101613675,
20.));
#73017=CARTESIAN_POINT('Ctrl Pts',(-7.35159359993819,-46.9878265878505,
0.));
#73018=CARTESIAN_POINT('Ctrl Pts',(-7.35159359993819,-46.9878265878505,
20.));
#73019=CARTESIAN_POINT('Ctrl Pts',(-7.38390426911933,-46.9797207437786,
0.));
#73020=CARTESIAN_POINT('Ctrl Pts',(-7.38390426911933,-46.9797207437786,
20.));
#73021=CARTESIAN_POINT('Ctrl Pts',(-7.41620819288779,-46.9715926339391,
0.));
#73022=CARTESIAN_POINT('Ctrl Pts',(-7.41620819288779,-46.9715926339391,
20.));
#73023=CARTESIAN_POINT('Ctrl Pts',(-7.44850535573483,-46.9634422631307,
0.));
#73024=CARTESIAN_POINT('Ctrl Pts',(-7.44850535573483,-46.9634422631307,
20.));
#73025=CARTESIAN_POINT('Ctrl Pts',(-7.4807957421548,-46.9552696361634,0.));
#73026=CARTESIAN_POINT('Ctrl Pts',(-7.4807957421548,-46.9552696361634,20.));
#73027=CARTESIAN_POINT('Ctrl Pts',(-7.51307933664513,-46.9470747578592,
0.));
#73028=CARTESIAN_POINT('Ctrl Pts',(-7.51307933664513,-46.9470747578592,
20.));
#73029=CARTESIAN_POINT('Ctrl Pts',(-7.54535612370603,-46.9388576330501,
0.));
#73030=CARTESIAN_POINT('Ctrl Pts',(-7.54535612370603,-46.9388576330501,
20.));
#73031=CARTESIAN_POINT('Ctrl Pts',(-7.5776260878407,-46.9306182665792,0.));
#73032=CARTESIAN_POINT('Ctrl Pts',(-7.5776260878407,-46.9306182665792,20.));
#73033=CARTESIAN_POINT('Ctrl Pts',(-7.60988921355522,-46.9223566632999,
0.));
#73034=CARTESIAN_POINT('Ctrl Pts',(-7.60988921355522,-46.9223566632999,
20.));
#73035=CARTESIAN_POINT('Ctrl Pts',(-7.64214548535858,-46.9140728280766,
0.));
#73036=CARTESIAN_POINT('Ctrl Pts',(-7.64214548535858,-46.9140728280766,
20.));
#73037=CARTESIAN_POINT('Ctrl Pts',(-7.67439488776289,-46.9057667657847,
0.));
#73038=CARTESIAN_POINT('Ctrl Pts',(-7.67439488776289,-46.9057667657847,
20.));
#73039=CARTESIAN_POINT('Ctrl Pts',(-7.70663740528332,-46.8974384813109,
0.));
#73040=CARTESIAN_POINT('Ctrl Pts',(-7.70663740528332,-46.8974384813109,
20.));
#73041=CARTESIAN_POINT('Ctrl Pts',(-7.73887302243817,-46.8890879795531,
0.));
#73042=CARTESIAN_POINT('Ctrl Pts',(-7.73887302243817,-46.8890879795531,
20.));
#73043=CARTESIAN_POINT('Ctrl Pts',(-7.77110172374869,-46.8807152654198,
0.));
#73044=CARTESIAN_POINT('Ctrl Pts',(-7.77110172374869,-46.8807152654198,
20.));
#73045=CARTESIAN_POINT('Ctrl Pts',(-7.80332349373919,-46.8723203438306,
0.));
#73046=CARTESIAN_POINT('Ctrl Pts',(-7.80332349373919,-46.8723203438306,
20.));
#73047=CARTESIAN_POINT('Ctrl Pts',(-7.83553831693688,-46.8639032197162,
0.));
#73048=CARTESIAN_POINT('Ctrl Pts',(-7.83553831693688,-46.8639032197162,
20.));
#73049=CARTESIAN_POINT('Ctrl Pts',(-7.86774617787214,-46.855463898018,0.));
#73050=CARTESIAN_POINT('Ctrl Pts',(-7.86774617787214,-46.855463898018,20.));
#73051=CARTESIAN_POINT('Ctrl Pts',(-7.8999470610784,-46.8470023836881,0.));
#73052=CARTESIAN_POINT('Ctrl Pts',(-7.8999470610784,-46.8470023836881,20.));
#73053=CARTESIAN_POINT('Ctrl Pts',(-7.93214095109212,-46.8385186816898,
0.));
#73054=CARTESIAN_POINT('Ctrl Pts',(-7.93214095109212,-46.8385186816898,
20.));
#73055=CARTESIAN_POINT('Ctrl Pts',(-7.96432783245287,-46.8300127969969,
0.));
#73056=CARTESIAN_POINT('Ctrl Pts',(-7.96432783245287,-46.8300127969969,
20.));
#73057=CARTESIAN_POINT('Ctrl Pts',(-7.99650768970305,-46.8214847345942,
0.));
#73058=CARTESIAN_POINT('Ctrl Pts',(-7.99650768970305,-46.8214847345942,
20.));
#73059=CARTESIAN_POINT('Ctrl Pts',(-8.02868050738829,-46.8129344994773,
0.));
#73060=CARTESIAN_POINT('Ctrl Pts',(-8.02868050738829,-46.8129344994773,
20.));
#73061=CARTESIAN_POINT('Ctrl Pts',(-8.0608462700573,-46.8043620966531,0.));
#73062=CARTESIAN_POINT('Ctrl Pts',(-8.0608462700573,-46.8043620966531,20.));
#73063=CARTESIAN_POINT('Ctrl Pts',(-8.09300496226221,-46.7957675311395,
0.));
#73064=CARTESIAN_POINT('Ctrl Pts',(-8.09300496226221,-46.7957675311395,
20.));
#73065=CARTESIAN_POINT('Ctrl Pts',(-8.12515656855803,-46.7871508079658,
0.));
#73066=CARTESIAN_POINT('Ctrl Pts',(-8.12515656855803,-46.7871508079658,
20.));
#73067=CARTESIAN_POINT('Ctrl Pts',(-8.15730107350296,-46.7785119321719,
0.));
#73068=CARTESIAN_POINT('Ctrl Pts',(-8.15730107350296,-46.7785119321719,
20.));
#73069=CARTESIAN_POINT('Ctrl Pts',(-8.18943846165846,-46.7698509088086,
0.));
#73070=CARTESIAN_POINT('Ctrl Pts',(-8.18943846165846,-46.7698509088086,
20.));
#73071=CARTESIAN_POINT('Ctrl Pts',(-8.22156871758883,-46.7611677429374,
0.));
#73072=CARTESIAN_POINT('Ctrl Pts',(-8.22156871758883,-46.7611677429374,
20.));
#73073=CARTESIAN_POINT('Ctrl Pts',(-8.2536918258617,-46.7524624396307,0.));
#73074=CARTESIAN_POINT('Ctrl Pts',(-8.2536918258617,-46.7524624396307,20.));
#73075=CARTESIAN_POINT('Ctrl Pts',(-8.28580777104746,-46.7437350039712,
0.));
#73076=CARTESIAN_POINT('Ctrl Pts',(-8.28580777104746,-46.7437350039712,
20.));
#73077=CARTESIAN_POINT('Ctrl Pts',(-8.31791653771974,-46.7349854410525,
0.));
#73078=CARTESIAN_POINT('Ctrl Pts',(-8.31791653771974,-46.7349854410525,
20.));
#73079=CARTESIAN_POINT('Ctrl Pts',(-8.35001811045537,-46.7262137559789,
0.));
#73080=CARTESIAN_POINT('Ctrl Pts',(-8.35001811045537,-46.7262137559789,
20.));
#73081=CARTESIAN_POINT('Ctrl Pts',(-8.38211247383477,-46.7174199538668,
0.));
#73082=CARTESIAN_POINT('Ctrl Pts',(-8.38211247383477,-46.7174199538668,
20.));
#73083=CARTESIAN_POINT('Ctrl Pts',(-8.41419961244156,-46.7086040398438,
0.));
#73084=CARTESIAN_POINT('Ctrl Pts',(-8.41419961244156,-46.7086040398438,
20.));
#73085=CARTESIAN_POINT('Ctrl Pts',(-8.44627951086263,-46.6997660190488,
0.));
#73086=CARTESIAN_POINT('Ctrl Pts',(-8.44627951086263,-46.6997660190488,
20.));
#73087=CARTESIAN_POINT('Ctrl Pts',(-8.47835215368745,-46.6909058966306,
0.));
#73088=CARTESIAN_POINT('Ctrl Pts',(-8.47835215368745,-46.6909058966306,
20.));
#73089=CARTESIAN_POINT('Ctrl Pts',(-8.51041752550882,-46.6820236777489,
0.));
#73090=CARTESIAN_POINT('Ctrl Pts',(-8.51041752550882,-46.6820236777489,
20.));
#73091=CARTESIAN_POINT('Ctrl Pts',(-8.54247561092259,-46.673119367573,0.));
#73092=CARTESIAN_POINT('Ctrl Pts',(-8.54247561092259,-46.673119367573,20.));
#73093=CARTESIAN_POINT('Ctrl Pts',(-8.57452639452829,-46.6641929712839,
0.));
#73094=CARTESIAN_POINT('Ctrl Pts',(-8.57452639452829,-46.6641929712839,
20.));
#73095=CARTESIAN_POINT('Ctrl Pts',(-8.60656986092879,-46.6552444940739,
0.));
#73096=CARTESIAN_POINT('Ctrl Pts',(-8.60656986092879,-46.6552444940739,
20.));
#73097=CARTESIAN_POINT('Ctrl Pts',(-8.63860599473004,-46.6462739411471,
0.));
#73098=CARTESIAN_POINT('Ctrl Pts',(-8.63860599473004,-46.6462739411471,
20.));
#73099=CARTESIAN_POINT('Ctrl Pts',(-8.67063478054117,-46.6372813177181,
0.));
#73100=CARTESIAN_POINT('Ctrl Pts',(-8.67063478054117,-46.6372813177181,
20.));
#73101=CARTESIAN_POINT('Ctrl Pts',(-8.70265620297455,-46.6282666290119,
0.));
#73102=CARTESIAN_POINT('Ctrl Pts',(-8.70265620297455,-46.6282666290119,
20.));
#73103=CARTESIAN_POINT('Ctrl Pts',(-8.73467024664571,-46.6192298802645,
0.));
#73104=CARTESIAN_POINT('Ctrl Pts',(-8.73467024664571,-46.6192298802645,
20.));
#73105=CARTESIAN_POINT('Ctrl Pts',(-8.76667689617331,-46.6101710767218,
0.));
#73106=CARTESIAN_POINT('Ctrl Pts',(-8.76667689617331,-46.6101710767218,
20.));
#73107=CARTESIAN_POINT('Ctrl Pts',(-8.79867613617934,-46.6010902236408,
0.));
#73108=CARTESIAN_POINT('Ctrl Pts',(-8.79867613617934,-46.6010902236408,
20.));
#73109=CARTESIAN_POINT('Ctrl Pts',(-8.83066795128935,-46.59198732629,0.));
#73110=CARTESIAN_POINT('Ctrl Pts',(-8.83066795128935,-46.59198732629,20.));
#73111=CARTESIAN_POINT('Ctrl Pts',(-8.86265232613216,-46.582862389949,0.));
#73112=CARTESIAN_POINT('Ctrl Pts',(-8.86265232613216,-46.582862389949,20.));
#73113=CARTESIAN_POINT('Ctrl Pts',(-8.8946292453399,-46.5737154199087,0.));
#73114=CARTESIAN_POINT('Ctrl Pts',(-8.8946292453399,-46.5737154199087,20.));
#73115=CARTESIAN_POINT('Ctrl Pts',(-8.92659869354789,-46.5645464214705,
0.));
#73116=CARTESIAN_POINT('Ctrl Pts',(-8.92659869354789,-46.5645464214705,
20.));
#73117=CARTESIAN_POINT('Ctrl Pts',(-8.95856065539471,-46.5553553999467,
0.));
#73118=CARTESIAN_POINT('Ctrl Pts',(-8.95856065539471,-46.5553553999467,
20.));
#73119=CARTESIAN_POINT('Ctrl Pts',(-8.9905151155223,-46.5461423606602,0.));
#73120=CARTESIAN_POINT('Ctrl Pts',(-8.9905151155223,-46.5461423606602,20.));
#73121=CARTESIAN_POINT('Ctrl Pts',(-9.02246205857629,-46.5369073089453,
0.));
#73122=CARTESIAN_POINT('Ctrl Pts',(-9.02246205857629,-46.5369073089453,
20.));
#73123=CARTESIAN_POINT('Ctrl Pts',(-9.05440146920516,-46.5276502501459,
0.));
#73124=CARTESIAN_POINT('Ctrl Pts',(-9.05440146920516,-46.5276502501459,
20.));
#73125=CARTESIAN_POINT('Ctrl Pts',(-9.08633333206091,-46.5183711896174,
0.));
#73126=CARTESIAN_POINT('Ctrl Pts',(-9.08633333206091,-46.5183711896174,
20.));
#73127=CARTESIAN_POINT('Ctrl Pts',(-9.11825763179854,-46.5090701327255,
0.));
#73128=CARTESIAN_POINT('Ctrl Pts',(-9.11825763179854,-46.5090701327255,
20.));
#73129=CARTESIAN_POINT('Ctrl Pts',(-9.15017435307667,-46.4997470848477,
0.));
#73130=CARTESIAN_POINT('Ctrl Pts',(-9.15017435307667,-46.4997470848477,
20.));
#73131=CARTESIAN_POINT('Ctrl Pts',(-9.18208348055726,-46.4904020513722,
0.));
#73132=CARTESIAN_POINT('Ctrl Pts',(-9.18208348055726,-46.4904020513722,
20.));
#73133=CARTESIAN_POINT('Ctrl Pts',(-9.21398499890594,-46.4810350376983,
0.));
#73134=CARTESIAN_POINT('Ctrl Pts',(-9.21398499890594,-46.4810350376983,
20.));
#73135=CARTESIAN_POINT('Ctrl Pts',(-9.24587889279172,-46.4716460492361,
0.));
#73136=CARTESIAN_POINT('Ctrl Pts',(-9.24587889279172,-46.4716460492361,
20.));
#73137=CARTESIAN_POINT('Ctrl Pts',(-9.277765146887,-46.4622350914066,0.));
#73138=CARTESIAN_POINT('Ctrl Pts',(-9.277765146887,-46.4622350914066,20.));
#73139=CARTESIAN_POINT('Ctrl Pts',(-9.30964374586753,-46.4528021696416,
0.));
#73140=CARTESIAN_POINT('Ctrl Pts',(-9.30964374586753,-46.4528021696416,
20.));
#73141=CARTESIAN_POINT('Ctrl Pts',(-9.34151467441242,-46.4433472893837,
0.));
#73142=CARTESIAN_POINT('Ctrl Pts',(-9.34151467441242,-46.4433472893837,
20.));
#73143=CARTESIAN_POINT('Ctrl Pts',(-9.37337791720394,-46.4338704560856,
0.));
#73144=CARTESIAN_POINT('Ctrl Pts',(-9.37337791720394,-46.4338704560856,
20.));
#73145=CARTESIAN_POINT('Ctrl Pts',(-9.40523345892774,-46.4243716752115,
0.));
#73146=CARTESIAN_POINT('Ctrl Pts',(-9.40523345892774,-46.4243716752115,
20.));
#73147=CARTESIAN_POINT('Ctrl Pts',(-9.43708128427275,-46.4148509522358,
0.));
#73148=CARTESIAN_POINT('Ctrl Pts',(-9.43708128427275,-46.4148509522358,
20.));
#73149=CARTESIAN_POINT('Ctrl Pts',(-9.46892137793149,-46.405308292644,0.));
#73150=CARTESIAN_POINT('Ctrl Pts',(-9.46892137793149,-46.405308292644,20.));
#73151=CARTESIAN_POINT('Ctrl Pts',(-9.5007537246001,-46.3957437019326,0.));
#73152=CARTESIAN_POINT('Ctrl Pts',(-9.5007537246001,-46.3957437019326,20.));
#73153=CARTESIAN_POINT('Ctrl Pts',(-9.53257830897852,-46.3861571856095,
0.));
#73154=CARTESIAN_POINT('Ctrl Pts',(-9.53257830897852,-46.3861571856095,
20.));
#73155=CARTESIAN_POINT('Ctrl Pts',(-9.56439511577024,-46.3765487491938,
0.));
#73156=CARTESIAN_POINT('Ctrl Pts',(-9.56439511577024,-46.3765487491938,
20.));
#73157=CARTESIAN_POINT('Ctrl Pts',(-9.59620412968214,-46.3669183982155,
0.));
#73158=CARTESIAN_POINT('Ctrl Pts',(-9.59620412968214,-46.3669183982155,
20.));
#73159=CARTESIAN_POINT('Ctrl Pts',(-9.62800533542437,-46.3572661382147,
0.));
#73160=CARTESIAN_POINT('Ctrl Pts',(-9.62800533542437,-46.3572661382147,
20.));
#73161=CARTESIAN_POINT('Ctrl Pts',(-9.6597987177104,-46.347591974742,0.));
#73162=CARTESIAN_POINT('Ctrl Pts',(-9.6597987177104,-46.347591974742,20.));
#73163=CARTESIAN_POINT('Ctrl Pts',(-9.69158426125693,-46.3378959133587,
0.));
#73164=CARTESIAN_POINT('Ctrl Pts',(-9.69158426125693,-46.3378959133587,
20.));
#73165=CARTESIAN_POINT('Ctrl Pts',(-9.72336195078415,-46.3281779596367,
0.));
#73166=CARTESIAN_POINT('Ctrl Pts',(-9.72336195078415,-46.3281779596367,
20.));
#73167=CARTESIAN_POINT('Ctrl Pts',(-9.75513177101578,-46.3184381191592,
0.));
#73168=CARTESIAN_POINT('Ctrl Pts',(-9.75513177101578,-46.3184381191592,
20.));
#73169=CARTESIAN_POINT('Ctrl Pts',(-9.78689370667941,-46.3086763975205,
0.));
#73170=CARTESIAN_POINT('Ctrl Pts',(-9.78689370667941,-46.3086763975205,
20.));
#73171=CARTESIAN_POINT('Ctrl Pts',(-9.8186477425062,-46.2988928003257,0.));
#73172=CARTESIAN_POINT('Ctrl Pts',(-9.8186477425062,-46.2988928003257,20.));
#73173=CARTESIAN_POINT('Ctrl Pts',(-9.85039386323086,-46.289087333191,0.));
#73174=CARTESIAN_POINT('Ctrl Pts',(-9.85039386323086,-46.289087333191,20.));
#73175=CARTESIAN_POINT('Ctrl Pts',(-9.88213205359192,-46.2792600017436,
0.));
#73176=CARTESIAN_POINT('Ctrl Pts',(-9.88213205359192,-46.2792600017436,
20.));
#73177=CARTESIAN_POINT('Ctrl Pts',(-9.91386229833138,-46.2694108116213,
0.));
#73178=CARTESIAN_POINT('Ctrl Pts',(-9.91386229833138,-46.2694108116213,
20.));
#73179=CARTESIAN_POINT('Ctrl Pts',(-9.94558458219447,-46.2595397684724,
0.));
#73180=CARTESIAN_POINT('Ctrl Pts',(-9.94558458219447,-46.2595397684724,
20.));
#73181=CARTESIAN_POINT('Ctrl Pts',(-9.97729888992981,-46.2496468779557,
0.));
#73182=CARTESIAN_POINT('Ctrl Pts',(-9.97729888992981,-46.2496468779557,
20.));
#73183=CARTESIAN_POINT('Ctrl Pts',(-10.0090052062895,-46.2397321457408,
0.));
#73184=CARTESIAN_POINT('Ctrl Pts',(-10.0090052062895,-46.2397321457408,
20.));
#73185=CARTESIAN_POINT('Ctrl Pts',(-10.0407035160293,-46.2297955775084,
0.));
#73186=CARTESIAN_POINT('Ctrl Pts',(-10.0407035160293,-46.2297955775084,
20.));
#73187=CARTESIAN_POINT('Ctrl Pts',(-10.0723938039086,-46.2198371789501,
0.));
#73188=CARTESIAN_POINT('Ctrl Pts',(-10.0723938039086,-46.2198371789501,
20.));
#73189=CARTESIAN_POINT('Ctrl Pts',(-10.1040760546909,-46.2098569557688,
0.));
#73190=CARTESIAN_POINT('Ctrl Pts',(-10.1040760546909,-46.2098569557688,
20.));
#73191=CARTESIAN_POINT('Ctrl Pts',(-10.1357502531431,-46.1998549136779,
0.));
#73192=CARTESIAN_POINT('Ctrl Pts',(-10.1357502531431,-46.1998549136779,
20.));
#73193=CARTESIAN_POINT('Ctrl Pts',(-10.1674163840354,-46.1898310584014,
0.));
#73194=CARTESIAN_POINT('Ctrl Pts',(-10.1674163840354,-46.1898310584014,
20.));
#73195=CARTESIAN_POINT('Ctrl Pts',(-10.199074432142,-46.179785395674,0.));
#73196=CARTESIAN_POINT('Ctrl Pts',(-10.199074432142,-46.179785395674,20.));
#73197=CARTESIAN_POINT('Ctrl Pts',(-10.2307243822402,-46.169717931241,0.));
#73198=CARTESIAN_POINT('Ctrl Pts',(-10.2307243822402,-46.169717931241,20.));
#73199=CARTESIAN_POINT('Ctrl Pts',(-10.2623662191114,-46.1596286708586,
0.));
#73200=CARTESIAN_POINT('Ctrl Pts',(-10.2623662191114,-46.1596286708586,
20.));
#73201=CARTESIAN_POINT('Ctrl Pts',(-10.2939999275403,-46.1495176202946,
0.));
#73202=CARTESIAN_POINT('Ctrl Pts',(-10.2939999275403,-46.1495176202946,
20.));
#73203=CARTESIAN_POINT('Ctrl Pts',(-10.3256254923156,-46.139384785327,0.));
#73204=CARTESIAN_POINT('Ctrl Pts',(-10.3256254923156,-46.139384785327,20.));
#73205=CARTESIAN_POINT('Ctrl Pts',(-10.3572428982293,-46.1292301717445,
0.));
#73206=CARTESIAN_POINT('Ctrl Pts',(-10.3572428982293,-46.1292301717445,
20.));
#73207=CARTESIAN_POINT('Ctrl Pts',(-10.3888521300774,-46.119053785347,0.));
#73208=CARTESIAN_POINT('Ctrl Pts',(-10.3888521300774,-46.119053785347,20.));
#73209=CARTESIAN_POINT('Ctrl Pts',(-10.4204531726593,-46.1088556319449,
0.));
#73210=CARTESIAN_POINT('Ctrl Pts',(-10.4204531726593,-46.1088556319449,
20.));
#73211=CARTESIAN_POINT('Ctrl Pts',(-10.4520460107784,-46.0986357173598,
0.));
#73212=CARTESIAN_POINT('Ctrl Pts',(-10.4520460107784,-46.0986357173598,
20.));
#73213=CARTESIAN_POINT('Ctrl Pts',(-10.4836306292415,-46.0883940474237,
0.));
#73214=CARTESIAN_POINT('Ctrl Pts',(-10.4836306292415,-46.0883940474237,
20.));
#73215=CARTESIAN_POINT('Ctrl Pts',(-10.5152070128593,-46.0781306279792,
0.));
#73216=CARTESIAN_POINT('Ctrl Pts',(-10.5152070128593,-46.0781306279792,
20.));
#73217=CARTESIAN_POINT('Ctrl Pts',(-10.5467751464457,-46.0678454648793,
0.));
#73218=CARTESIAN_POINT('Ctrl Pts',(-10.5467751464457,-46.0678454648793,
20.));
#73219=CARTESIAN_POINT('Ctrl Pts',(-10.5783350148188,-46.0575385639878,
0.));
#73220=CARTESIAN_POINT('Ctrl Pts',(-10.5783350148188,-46.0575385639878,
20.));
#73221=CARTESIAN_POINT('Ctrl Pts',(-10.6098866028001,-46.0472099311799,
0.));
#73222=CARTESIAN_POINT('Ctrl Pts',(-10.6098866028001,-46.0472099311799,
20.));
#73223=CARTESIAN_POINT('Ctrl Pts',(-10.6414298952151,-46.0368595723418,
0.));
#73224=CARTESIAN_POINT('Ctrl Pts',(-10.6414298952151,-46.0368595723418,
20.));
#73225=CARTESIAN_POINT('Ctrl Pts',(-10.6729648768932,-46.0264874933706,
0.));
#73226=CARTESIAN_POINT('Ctrl Pts',(-10.6729648768932,-46.0264874933706,
20.));
#73227=CARTESIAN_POINT('Ctrl Pts',(-10.7044915326674,-46.0160937001747,
0.));
#73228=CARTESIAN_POINT('Ctrl Pts',(-10.7044915326674,-46.0160937001747,
20.));
#73229=CARTESIAN_POINT('Ctrl Pts',(-10.7360098473747,-46.0056781986726,
0.));
#73230=CARTESIAN_POINT('Ctrl Pts',(-10.7360098473747,-46.0056781986726,
20.));
#73231=CARTESIAN_POINT('Ctrl Pts',(-10.7675198058554,-45.9952409947932,
0.));
#73232=CARTESIAN_POINT('Ctrl Pts',(-10.7675198058554,-45.9952409947932,
20.));
#73233=CARTESIAN_POINT('Ctrl Pts',(-10.7990213929536,-45.9847820944759,
0.));
#73234=CARTESIAN_POINT('Ctrl Pts',(-10.7990213929536,-45.9847820944759,
20.));
#73235=CARTESIAN_POINT('Ctrl Pts',(-10.8305145935168,-45.9743015036702,
0.));
#73236=CARTESIAN_POINT('Ctrl Pts',(-10.8305145935168,-45.9743015036702,
20.));
#73237=CARTESIAN_POINT('Ctrl Pts',(-10.8619993923967,-45.9637992283368,
0.));
#73238=CARTESIAN_POINT('Ctrl Pts',(-10.8619993923967,-45.9637992283368,
20.));
#73239=CARTESIAN_POINT('Ctrl Pts',(-10.8934757744485,-45.9532752744476,
0.));
#73240=CARTESIAN_POINT('Ctrl Pts',(-10.8934757744485,-45.9532752744476,
20.));
#73241=CARTESIAN_POINT('Ctrl Pts',(-10.9249437245321,-45.9427296479861,
0.));
#73242=CARTESIAN_POINT('Ctrl Pts',(-10.9249437245321,-45.9427296479861,
20.));
#73243=CARTESIAN_POINT('Ctrl Pts',(-10.9564032275107,-45.9321623549466,
0.));
#73244=CARTESIAN_POINT('Ctrl Pts',(-10.9564032275107,-45.9321623549466,
20.));
#73245=CARTESIAN_POINT('Ctrl Pts',(-10.9878542682513,-45.9215734013338,
0.));
#73246=CARTESIAN_POINT('Ctrl Pts',(-10.9878542682513,-45.9215734013338,
20.));
#73247=CARTESIAN_POINT('Ctrl Pts',(-11.0192968316247,-45.9109627931629,
0.));
#73248=CARTESIAN_POINT('Ctrl Pts',(-11.0192968316247,-45.9109627931629,
20.));
#73249=CARTESIAN_POINT('Ctrl Pts',(-11.0507309025053,-45.9003305364593,
0.));
#73250=CARTESIAN_POINT('Ctrl Pts',(-11.0507309025053,-45.9003305364593,
20.));
#73251=CARTESIAN_POINT('Ctrl Pts',(-11.0821564657716,-45.8896766372596,
0.));
#73252=CARTESIAN_POINT('Ctrl Pts',(-11.0821564657716,-45.8896766372596,
20.));
#73253=CARTESIAN_POINT('Ctrl Pts',(-11.1135735063059,-45.8790011016108,
0.));
#73254=CARTESIAN_POINT('Ctrl Pts',(-11.1135735063059,-45.8790011016108,
20.));
#73255=CARTESIAN_POINT('Ctrl Pts',(-11.1449820089942,-45.868303935571,0.));
#73256=CARTESIAN_POINT('Ctrl Pts',(-11.1449820089942,-45.868303935571,20.));
#73257=CARTESIAN_POINT('Ctrl Pts',(-11.1763819587263,-45.8575851452088,
0.));
#73258=CARTESIAN_POINT('Ctrl Pts',(-11.1763819587263,-45.8575851452088,
20.));
#73259=CARTESIAN_POINT('Ctrl Pts',(-11.207773340396,-45.8468447366038,0.));
#73260=CARTESIAN_POINT('Ctrl Pts',(-11.207773340396,-45.8468447366038,20.));
#73261=CARTESIAN_POINT('Ctrl Pts',(-11.2391561389011,-45.8360827158468,
0.));
#73262=CARTESIAN_POINT('Ctrl Pts',(-11.2391561389011,-45.8360827158468,
20.));
#73263=CARTESIAN_POINT('Ctrl Pts',(-11.2705303391434,-45.8252990890386,
0.));
#73264=CARTESIAN_POINT('Ctrl Pts',(-11.2705303391434,-45.8252990890386,
20.));
#73265=CARTESIAN_POINT('Ctrl Pts',(-11.3018959260283,-45.8144938622913,
0.));
#73266=CARTESIAN_POINT('Ctrl Pts',(-11.3018959260283,-45.8144938622913,
20.));
#73267=CARTESIAN_POINT('Ctrl Pts',(-11.3332528844652,-45.8036670417272,
0.));
#73268=CARTESIAN_POINT('Ctrl Pts',(-11.3332528844652,-45.8036670417272,
20.));
#73269=CARTESIAN_POINT('Ctrl Pts',(-11.3646011993674,-45.7928186334791,
0.));
#73270=CARTESIAN_POINT('Ctrl Pts',(-11.3646011993674,-45.7928186334791,
20.));
#73271=CARTESIAN_POINT('Ctrl Pts',(-11.395940855652,-45.7819486436912,0.));
#73272=CARTESIAN_POINT('Ctrl Pts',(-11.395940855652,-45.7819486436912,20.));
#73273=CARTESIAN_POINT('Ctrl Pts',(-11.4272718382404,-45.7710570785186,
0.));
#73274=CARTESIAN_POINT('Ctrl Pts',(-11.4272718382404,-45.7710570785186,
20.));
#73275=CARTESIAN_POINT('Ctrl Pts',(-11.4585941320575,-45.760143944127,0.));
#73276=CARTESIAN_POINT('Ctrl Pts',(-11.4585941320575,-45.760143944127,20.));
#73277=CARTESIAN_POINT('Ctrl Pts',(-11.489907722032,-45.7492092466918,0.));
#73278=CARTESIAN_POINT('Ctrl Pts',(-11.489907722032,-45.7492092466918,20.));
#73279=CARTESIAN_POINT('Ctrl Pts',(-11.5212125930967,-45.7382529923996,
0.));
#73280=CARTESIAN_POINT('Ctrl Pts',(-11.5212125930967,-45.7382529923996,
20.));
#73281=CARTESIAN_POINT('Ctrl Pts',(-11.5525087301884,-45.7272751874478,
0.));
#73282=CARTESIAN_POINT('Ctrl Pts',(-11.5525087301884,-45.7272751874478,
20.));
#73283=CARTESIAN_POINT('Ctrl Pts',(-11.5837961182482,-45.7162758380449,
0.));
#73284=CARTESIAN_POINT('Ctrl Pts',(-11.5837961182482,-45.7162758380449,
20.));
#73285=CARTESIAN_POINT('Ctrl Pts',(-11.615074742221,-45.7052549504103,0.));
#73286=CARTESIAN_POINT('Ctrl Pts',(-11.615074742221,-45.7052549504103,20.));
#73287=CARTESIAN_POINT('Ctrl Pts',(-11.6463445870557,-45.694212530774,0.));
#73288=CARTESIAN_POINT('Ctrl Pts',(-11.6463445870557,-45.694212530774,20.));
#73289=CARTESIAN_POINT('Ctrl Pts',(-11.6776056377055,-45.6831485853771,
0.));
#73290=CARTESIAN_POINT('Ctrl Pts',(-11.6776056377055,-45.6831485853771,
20.));
#73291=CARTESIAN_POINT('Ctrl Pts',(-11.7088578791267,-45.6720631204703,
0.));
#73292=CARTESIAN_POINT('Ctrl Pts',(-11.7088578791267,-45.6720631204703,
20.));
#73293=CARTESIAN_POINT('Ctrl Pts',(-11.7401012962797,-45.6609561423149,
0.));
#73294=CARTESIAN_POINT('Ctrl Pts',(-11.7401012962797,-45.6609561423149,
20.));
#73295=CARTESIAN_POINT('Ctrl Pts',(-11.7713358741293,-45.6498276571829,
0.));
#73296=CARTESIAN_POINT('Ctrl Pts',(-11.7713358741293,-45.6498276571829,
20.));
#73297=CARTESIAN_POINT('Ctrl Pts',(-11.8025615976441,-45.6386776713575,
0.));
#73298=CARTESIAN_POINT('Ctrl Pts',(-11.8025615976441,-45.6386776713575,
20.));
#73299=CARTESIAN_POINT('Ctrl Pts',(-11.8337784517972,-45.627506191133,0.));
#73300=CARTESIAN_POINT('Ctrl Pts',(-11.8337784517972,-45.627506191133,20.));
#73301=CARTESIAN_POINT('Ctrl Pts',(-11.8649864215653,-45.6163132228138,
0.));
#73302=CARTESIAN_POINT('Ctrl Pts',(-11.8649864215653,-45.6163132228138,
20.));
#73303=CARTESIAN_POINT('Ctrl Pts',(-11.8961854919294,-45.6050987727153,
0.));
#73304=CARTESIAN_POINT('Ctrl Pts',(-11.8961854919294,-45.6050987727153,
20.));
#73305=CARTESIAN_POINT('Ctrl Pts',(-11.9273756478741,-45.5938628471638,
0.));
#73306=CARTESIAN_POINT('Ctrl Pts',(-11.9273756478741,-45.5938628471638,
20.));
#73307=CARTESIAN_POINT('Ctrl Pts',(-11.9585568743886,-45.5826054524963,
0.));
#73308=CARTESIAN_POINT('Ctrl Pts',(-11.9585568743886,-45.5826054524963,
20.));
#73309=CARTESIAN_POINT('Ctrl Pts',(-11.989729156466,-45.5713265950605,0.));
#73310=CARTESIAN_POINT('Ctrl Pts',(-11.989729156466,-45.5713265950605,20.));
#73311=CARTESIAN_POINT('Ctrl Pts',(-12.0208924791035,-45.5600262812144,
0.));
#73312=CARTESIAN_POINT('Ctrl Pts',(-12.0208924791035,-45.5600262812144,
20.));
#73313=CARTESIAN_POINT('Ctrl Pts',(-12.0520468273019,-45.5487045173265,
0.));
#73314=CARTESIAN_POINT('Ctrl Pts',(-12.0520468273019,-45.5487045173265,
20.));
#73315=CARTESIAN_POINT('Ctrl Pts',(-12.0831921860666,-45.5373613097755,
0.));
#73316=CARTESIAN_POINT('Ctrl Pts',(-12.0831921860666,-45.5373613097755,
20.));
#73317=CARTESIAN_POINT('Ctrl Pts',(-12.1143285404065,-45.5259966649516,
0.));
#73318=CARTESIAN_POINT('Ctrl Pts',(-12.1143285404065,-45.5259966649516,
20.));
#73319=CARTESIAN_POINT('Ctrl Pts',(-12.1454558753351,-45.5146105892553,
0.));
#73320=CARTESIAN_POINT('Ctrl Pts',(-12.1454558753351,-45.5146105892553,
20.));
#73321=CARTESIAN_POINT('Ctrl Pts',(-12.1765741758697,-45.5032030890978,
0.));
#73322=CARTESIAN_POINT('Ctrl Pts',(-12.1765741758697,-45.5032030890978,
20.));
#73323=CARTESIAN_POINT('Ctrl Pts',(-12.2076834270323,-45.4917741709015,
0.));
#73324=CARTESIAN_POINT('Ctrl Pts',(-12.2076834270323,-45.4917741709015,
20.));
#73325=CARTESIAN_POINT('Ctrl Pts',(-12.2387836138487,-45.4803238410999,
0.));
#73326=CARTESIAN_POINT('Ctrl Pts',(-12.2387836138487,-45.4803238410999,
20.));
#73327=CARTESIAN_POINT('Ctrl Pts',(-12.269874721349,-45.4688521061371,0.));
#73328=CARTESIAN_POINT('Ctrl Pts',(-12.269874721349,-45.4688521061371,20.));
#73329=CARTESIAN_POINT('Ctrl Pts',(-12.3009567345673,-45.4573589724673,
0.));
#73330=CARTESIAN_POINT('Ctrl Pts',(-12.3009567345673,-45.4573589724673,
20.));
#73331=CARTESIAN_POINT('Ctrl Pts',(-12.3320296385418,-45.4458444465552,
0.));
#73332=CARTESIAN_POINT('Ctrl Pts',(-12.3320296385418,-45.4458444465552,
20.));
#73333=CARTESIAN_POINT('Ctrl Pts',(-12.3630934183143,-45.4343085348755,
0.));
#73334=CARTESIAN_POINT('Ctrl Pts',(-12.3630934183143,-45.4343085348755,
20.));
#73335=CARTESIAN_POINT('Ctrl Pts',(-12.3941480589311,-45.4227512439136,
0.));
#73336=CARTESIAN_POINT('Ctrl Pts',(-12.3941480589311,-45.4227512439136,
20.));
#73337=CARTESIAN_POINT('Ctrl Pts',(-12.4251935454428,-45.4111725801659,
0.));
#73338=CARTESIAN_POINT('Ctrl Pts',(-12.4251935454428,-45.4111725801659,
20.));
#73339=CARTESIAN_POINT('Ctrl Pts',(-12.4562298629045,-45.3995725501402,
0.));
#73340=CARTESIAN_POINT('Ctrl Pts',(-12.4562298629045,-45.3995725501402,
20.));
#73341=CARTESIAN_POINT('Ctrl Pts',(-12.4872569963754,-45.3879511603549,
0.));
#73342=CARTESIAN_POINT('Ctrl Pts',(-12.4872569963754,-45.3879511603549,
20.));
#73343=CARTESIAN_POINT('Ctrl Pts',(-12.5182749309189,-45.376308417339,0.));
#73344=CARTESIAN_POINT('Ctrl Pts',(-12.5182749309189,-45.376308417339,20.));
#73345=CARTESIAN_POINT('Ctrl Pts',(-12.5492836516023,-45.364644327632,0.));
#73346=CARTESIAN_POINT('Ctrl Pts',(-12.5492836516023,-45.364644327632,20.));
#73347=CARTESIAN_POINT('Ctrl Pts',(-12.5802831434966,-45.3529588977839,
0.));
#73348=CARTESIAN_POINT('Ctrl Pts',(-12.5802831434966,-45.3529588977839,
20.));
#73349=CARTESIAN_POINT('Ctrl Pts',(-12.6112733916776,-45.3412521343551,
0.));
#73350=CARTESIAN_POINT('Ctrl Pts',(-12.6112733916776,-45.3412521343551,
20.));
#73351=CARTESIAN_POINT('Ctrl Pts',(-12.6422543812252,-45.3295240439169,
0.));
#73352=CARTESIAN_POINT('Ctrl Pts',(-12.6422543812252,-45.3295240439169,
20.));
#73353=CARTESIAN_POINT('Ctrl Pts',(-12.6732260972239,-45.3177746330512,
0.));
#73354=CARTESIAN_POINT('Ctrl Pts',(-12.6732260972239,-45.3177746330512,
20.));
#73355=CARTESIAN_POINT('Ctrl Pts',(-12.7041885247626,-45.3060039083501,
0.));
#73356=CARTESIAN_POINT('Ctrl Pts',(-12.7041885247626,-45.3060039083501,
20.));
#73357=CARTESIAN_POINT('Ctrl Pts',(-12.7351416489341,-45.2942118764167,
0.));
#73358=CARTESIAN_POINT('Ctrl Pts',(-12.7351416489341,-45.2942118764167,
20.));
#73359=CARTESIAN_POINT('Ctrl Pts',(-12.7660854548354,-45.2823985438647,
0.));
#73360=CARTESIAN_POINT('Ctrl Pts',(-12.7660854548354,-45.2823985438647,
20.));
#73361=CARTESIAN_POINT('Ctrl Pts',(-12.7970199275678,-45.2705639173192,
0.));
#73362=CARTESIAN_POINT('Ctrl Pts',(-12.7970199275678,-45.2705639173192,
20.));
#73363=CARTESIAN_POINT('Ctrl Pts',(-12.8279450522366,-45.2587080034157,
0.));
#73364=CARTESIAN_POINT('Ctrl Pts',(-12.8279450522366,-45.2587080034157,
20.));
#73365=CARTESIAN_POINT('Ctrl Pts',(-12.8588608139512,-45.2468308087994,
0.));
#73366=CARTESIAN_POINT('Ctrl Pts',(-12.8588608139512,-45.2468308087994,
20.));
#73367=CARTESIAN_POINT('Ctrl Pts',(-12.8897671978257,-45.2349323401259,
0.));
#73368=CARTESIAN_POINT('Ctrl Pts',(-12.8897671978257,-45.2349323401259,
20.));
#73369=CARTESIAN_POINT('Ctrl Pts',(-12.9206641889781,-45.2230126040617,
0.));
#73370=CARTESIAN_POINT('Ctrl Pts',(-12.9206641889781,-45.2230126040617,
20.));
#73371=CARTESIAN_POINT('Ctrl Pts',(-12.9515517725313,-45.2110716072841,
0.));
#73372=CARTESIAN_POINT('Ctrl Pts',(-12.9515517725313,-45.2110716072841,
20.));
#73373=CARTESIAN_POINT('Ctrl Pts',(-12.9824299336127,-45.199109356482,0.));
#73374=CARTESIAN_POINT('Ctrl Pts',(-12.9824299336127,-45.199109356482,20.));
#73375=CARTESIAN_POINT('Ctrl Pts',(-13.0132986573536,-45.1871258583545,
0.));
#73376=CARTESIAN_POINT('Ctrl Pts',(-13.0132986573536,-45.1871258583545,
20.));
#73377=CARTESIAN_POINT('Ctrl Pts',(-13.0441579288899,-45.1751211196118,
0.));
#73378=CARTESIAN_POINT('Ctrl Pts',(-13.0441579288899,-45.1751211196118,
20.));
#73379=CARTESIAN_POINT('Ctrl Pts',(-13.0750077333614,-45.1630951469733,
0.));
#73380=CARTESIAN_POINT('Ctrl Pts',(-13.0750077333614,-45.1630951469733,
20.));
#73381=CARTESIAN_POINT('Ctrl Pts',(-13.1058480559121,-45.1510479471692,
0.));
#73382=CARTESIAN_POINT('Ctrl Pts',(-13.1058480559121,-45.1510479471692,
20.));
#73383=CARTESIAN_POINT('Ctrl Pts',(-13.1366788816904,-45.1389795269399,
0.));
#73384=CARTESIAN_POINT('Ctrl Pts',(-13.1366788816904,-45.1389795269399,
20.));
#73385=CARTESIAN_POINT('Ctrl Pts',(-13.1675001958493,-45.1268898930368,
0.));
#73386=CARTESIAN_POINT('Ctrl Pts',(-13.1675001958493,-45.1268898930368,
20.));
#73387=CARTESIAN_POINT('Ctrl Pts',(-13.198311983546,-45.114779052223,0.));
#73388=CARTESIAN_POINT('Ctrl Pts',(-13.198311983546,-45.114779052223,20.));
#73389=CARTESIAN_POINT('Ctrl Pts',(-13.2291142299426,-45.1026470112717,
0.));
#73390=CARTESIAN_POINT('Ctrl Pts',(-13.2291142299426,-45.1026470112717,
20.));
#73391=CARTESIAN_POINT('Ctrl Pts',(-13.259906920205,-45.0904937769663,0.));
#73392=CARTESIAN_POINT('Ctrl Pts',(-13.259906920205,-45.0904937769663,20.));
#73393=CARTESIAN_POINT('Ctrl Pts',(-13.2906900395037,-45.0783193561008,
0.));
#73394=CARTESIAN_POINT('Ctrl Pts',(-13.2906900395037,-45.0783193561008,
20.));
#73395=CARTESIAN_POINT('Ctrl Pts',(-13.3214635730135,-45.0661237554798,
0.));
#73396=CARTESIAN_POINT('Ctrl Pts',(-13.3214635730135,-45.0661237554798,
20.));
#73397=CARTESIAN_POINT('Ctrl Pts',(-13.3522275059137,-45.0539069819185,
0.));
#73398=CARTESIAN_POINT('Ctrl Pts',(-13.3522275059137,-45.0539069819185,
20.));
#73399=CARTESIAN_POINT('Ctrl Pts',(-13.3829818233878,-45.0416690422424,
0.));
#73400=CARTESIAN_POINT('Ctrl Pts',(-13.3829818233878,-45.0416690422424,
20.));
#73401=CARTESIAN_POINT('Ctrl Pts',(-13.4137265106238,-45.0294099432879,
0.));
#73402=CARTESIAN_POINT('Ctrl Pts',(-13.4137265106238,-45.0294099432879,
20.));
#73403=CARTESIAN_POINT('Ctrl Pts',(-13.4444615528144,-45.0171296919022,
0.));
#73404=CARTESIAN_POINT('Ctrl Pts',(-13.4444615528144,-45.0171296919022,
20.));
#73405=CARTESIAN_POINT('Ctrl Pts',(-13.4751869351564,-45.0048282949433,
0.));
#73406=CARTESIAN_POINT('Ctrl Pts',(-13.4751869351564,-45.0048282949433,
20.));
#73407=CARTESIAN_POINT('Ctrl Pts',(-13.5059026428512,-44.9925057592796,
0.));
#73408=CARTESIAN_POINT('Ctrl Pts',(-13.5059026428512,-44.9925057592796,
20.));
#73409=CARTESIAN_POINT('Ctrl Pts',(-13.5366086611044,-44.9801620917891,
0.));
#73410=CARTESIAN_POINT('Ctrl Pts',(-13.5366086611044,-44.9801620917891,
20.));
#73411=CARTESIAN_POINT('Ctrl Pts',(-13.5673049751264,-44.967797299361,0.));
#73412=CARTESIAN_POINT('Ctrl Pts',(-13.5673049751264,-44.967797299361,20.));
#73413=CARTESIAN_POINT('Ctrl Pts',(-13.5979915701319,-44.955411388895,0.));
#73414=CARTESIAN_POINT('Ctrl Pts',(-13.5979915701319,-44.955411388895,20.));
#73415=CARTESIAN_POINT('Ctrl Pts',(-13.6286684313402,-44.9430043673018,
0.));
#73416=CARTESIAN_POINT('Ctrl Pts',(-13.6286684313402,-44.9430043673018,
20.));
#73417=CARTESIAN_POINT('Ctrl Pts',(-13.6593355439745,-44.9305762415019,
0.));
#73418=CARTESIAN_POINT('Ctrl Pts',(-13.6593355439745,-44.9305762415019,
20.));
#73419=CARTESIAN_POINT('Ctrl Pts',(-13.6899928932632,-44.9181270184275,
0.));
#73420=CARTESIAN_POINT('Ctrl Pts',(-13.6899928932632,-44.9181270184275,
20.));
#73421=CARTESIAN_POINT('Ctrl Pts',(-13.7206404644388,-44.9056567050204,
0.));
#73422=CARTESIAN_POINT('Ctrl Pts',(-13.7206404644388,-44.9056567050204,
20.));
#73423=CARTESIAN_POINT('Ctrl Pts',(-13.7512782427386,-44.8931653082334,
0.));
#73424=CARTESIAN_POINT('Ctrl Pts',(-13.7512782427386,-44.8931653082334,
20.));
#73425=CARTESIAN_POINT('Ctrl Pts',(-13.7819062134042,-44.8806528350291,
0.));
#73426=CARTESIAN_POINT('Ctrl Pts',(-13.7819062134042,-44.8806528350291,
20.));
#73427=CARTESIAN_POINT('Ctrl Pts',(-13.8125243616816,-44.8681192923811,
0.));
#73428=CARTESIAN_POINT('Ctrl Pts',(-13.8125243616816,-44.8681192923811,
20.));
#73429=CARTESIAN_POINT('Ctrl Pts',(-13.8431326728214,-44.8555646872732,
0.));
#73430=CARTESIAN_POINT('Ctrl Pts',(-13.8431326728214,-44.8555646872732,
20.));
#73431=CARTESIAN_POINT('Ctrl Pts',(-13.8737311320789,-44.8429890267007,
0.));
#73432=CARTESIAN_POINT('Ctrl Pts',(-13.8737311320789,-44.8429890267007,
20.));
#73433=CARTESIAN_POINT('Ctrl Pts',(-13.9043197247138,-44.8303923176691,
0.));
#73434=CARTESIAN_POINT('Ctrl Pts',(-13.9043197247138,-44.8303923176691,
20.));
#73435=CARTESIAN_POINT('Ctrl Pts',(-13.9348984359903,-44.8177745671945,
0.));
#73436=CARTESIAN_POINT('Ctrl Pts',(-13.9348984359903,-44.8177745671945,
20.));
#73437=CARTESIAN_POINT('Ctrl Pts',(-13.9654672511774,-44.8051357823031,
0.));
#73438=CARTESIAN_POINT('Ctrl Pts',(-13.9654672511774,-44.8051357823031,
20.));
#73439=CARTESIAN_POINT('Ctrl Pts',(-13.9960261555481,-44.7924759700314,
0.));
#73440=CARTESIAN_POINT('Ctrl Pts',(-13.9960261555481,-44.7924759700314,
20.));
#73441=CARTESIAN_POINT('Ctrl Pts',(-14.0265751343805,-44.7797951374262,
0.));
#73442=CARTESIAN_POINT('Ctrl Pts',(-14.0265751343805,-44.7797951374262,
20.));
#73443=CARTESIAN_POINT('Ctrl Pts',(-14.057114172957,-44.7670932915455,0.));
#73444=CARTESIAN_POINT('Ctrl Pts',(-14.057114172957,-44.7670932915455,20.));
#73445=CARTESIAN_POINT('Ctrl Pts',(-14.0876432565649,-44.7543704394583,
0.));
#73446=CARTESIAN_POINT('Ctrl Pts',(-14.0876432565649,-44.7543704394583,
20.));
#73447=CARTESIAN_POINT('Ctrl Pts',(-14.118162370496,-44.7416265882442,0.));
#73448=CARTESIAN_POINT('Ctrl Pts',(-14.118162370496,-44.7416265882442,20.));
#73449=CARTESIAN_POINT('Ctrl Pts',(-14.1486715000464,-44.728861744993,0.));
#73450=CARTESIAN_POINT('Ctrl Pts',(-14.1486715000464,-44.728861744993,20.));
#73451=CARTESIAN_POINT('Ctrl Pts',(-14.1791706305171,-44.7160759168044,
0.));
#73452=CARTESIAN_POINT('Ctrl Pts',(-14.1791706305171,-44.7160759168044,
20.));
#73453=CARTESIAN_POINT('Ctrl Pts',(-14.2096597472134,-44.7032691107881,
0.));
#73454=CARTESIAN_POINT('Ctrl Pts',(-14.2096597472134,-44.7032691107881,
20.));
#73455=CARTESIAN_POINT('Ctrl Pts',(-14.2401388354454,-44.690441334065,0.));
#73456=CARTESIAN_POINT('Ctrl Pts',(-14.2401388354454,-44.690441334065,20.));
#73457=CARTESIAN_POINT('Ctrl Pts',(-14.2706078805279,-44.6775925937661,
0.));
#73458=CARTESIAN_POINT('Ctrl Pts',(-14.2706078805279,-44.6775925937661,
20.));
#73459=CARTESIAN_POINT('Ctrl Pts',(-14.3010668677802,-44.6647228970333,
0.));
#73460=CARTESIAN_POINT('Ctrl Pts',(-14.3010668677802,-44.6647228970333,
20.));
#73461=CARTESIAN_POINT('Ctrl Pts',(-14.3315157825264,-44.6518322510194,
0.));
#73462=CARTESIAN_POINT('Ctrl Pts',(-14.3315157825264,-44.6518322510194,
20.));
#73463=CARTESIAN_POINT('Ctrl Pts',(-14.3619546100951,-44.6389206628876,
0.));
#73464=CARTESIAN_POINT('Ctrl Pts',(-14.3619546100951,-44.6389206628876,
20.));
#73465=CARTESIAN_POINT('Ctrl Pts',(-14.3923833358197,-44.6259881398118,
0.));
#73466=CARTESIAN_POINT('Ctrl Pts',(-14.3923833358197,-44.6259881398118,
20.));
#73467=CARTESIAN_POINT('Ctrl Pts',(-14.4228019450383,-44.6130346889769,
0.));
#73468=CARTESIAN_POINT('Ctrl Pts',(-14.4228019450383,-44.6130346889769,
20.));
#73469=CARTESIAN_POINT('Ctrl Pts',(-14.4532104230937,-44.6000603175775,
0.));
#73470=CARTESIAN_POINT('Ctrl Pts',(-14.4532104230937,-44.6000603175775,
20.));
#73471=CARTESIAN_POINT('Ctrl Pts',(-14.4836087553332,-44.5870650328188,
0.));
#73472=CARTESIAN_POINT('Ctrl Pts',(-14.4836087553332,-44.5870650328188,
20.));
#73473=CARTESIAN_POINT('Ctrl Pts',(-14.5139969271087,-44.5740488419152,
0.));
#73474=CARTESIAN_POINT('Ctrl Pts',(-14.5139969271087,-44.5740488419152,
20.));
#73475=CARTESIAN_POINT('Ctrl Pts',(-14.5443749237768,-44.5610117520915,
0.));
#73476=CARTESIAN_POINT('Ctrl Pts',(-14.5443749237768,-44.5610117520915,
20.));
#73477=CARTESIAN_POINT('Ctrl Pts',(-14.5747427306988,-44.5479537705835,
0.));
#73478=CARTESIAN_POINT('Ctrl Pts',(-14.5747427306988,-44.5479537705835,
20.));
#73479=CARTESIAN_POINT('Ctrl Pts',(-14.6051003332411,-44.5348749046378,
0.));
#73480=CARTESIAN_POINT('Ctrl Pts',(-14.6051003332411,-44.5348749046378,
20.));
#73481=CARTESIAN_POINT('Ctrl Pts',(-14.6354477167742,-44.521775161512,0.));
#73482=CARTESIAN_POINT('Ctrl Pts',(-14.6354477167742,-44.521775161512,20.));
#73483=CARTESIAN_POINT('Ctrl Pts',(-14.6657848666744,-44.5086545484757,
0.));
#73484=CARTESIAN_POINT('Ctrl Pts',(-14.6657848666744,-44.5086545484757,
20.));
#73485=CARTESIAN_POINT('Ctrl Pts',(-14.6961117683217,-44.4955130728078,
0.));
#73486=CARTESIAN_POINT('Ctrl Pts',(-14.6961117683217,-44.4955130728078,
20.));
#73487=CARTESIAN_POINT('Ctrl Pts',(-14.7264284071013,-44.4823507417973,
0.));
#73488=CARTESIAN_POINT('Ctrl Pts',(-14.7264284071013,-44.4823507417973,
20.));
#73489=CARTESIAN_POINT('Ctrl Pts',(-14.756734768403,-44.469167562743,0.));
#73490=CARTESIAN_POINT('Ctrl Pts',(-14.756734768403,-44.469167562743,20.));
#73491=CARTESIAN_POINT('Ctrl Pts',(-14.7870308376214,-44.4559635429545,
0.));
#73492=CARTESIAN_POINT('Ctrl Pts',(-14.7870308376214,-44.4559635429545,
20.));
#73493=CARTESIAN_POINT('Ctrl Pts',(-14.817316600156,-44.4427386897515,0.));
#73494=CARTESIAN_POINT('Ctrl Pts',(-14.817316600156,-44.4427386897515,20.));
#73495=CARTESIAN_POINT('Ctrl Pts',(-14.8475920414108,-44.4294930104636,
0.));
#73496=CARTESIAN_POINT('Ctrl Pts',(-14.8475920414108,-44.4294930104636,
20.));
#73497=CARTESIAN_POINT('Ctrl Pts',(-14.8778571467943,-44.416226512431,0.));
#73498=CARTESIAN_POINT('Ctrl Pts',(-14.8778571467943,-44.416226512431,20.));
#73499=CARTESIAN_POINT('Ctrl Pts',(-14.9081119017199,-44.4029392030043,
0.));
#73500=CARTESIAN_POINT('Ctrl Pts',(-14.9081119017199,-44.4029392030043,
20.));
#73501=CARTESIAN_POINT('Ctrl Pts',(-14.9383562916061,-44.389631089546,0.));
#73502=CARTESIAN_POINT('Ctrl Pts',(-14.9383562916061,-44.389631089546,20.));
#73503=CARTESIAN_POINT('Ctrl Pts',(-14.9685903018767,-44.3763021794296,
0.));
#73504=CARTESIAN_POINT('Ctrl Pts',(-14.9685903018767,-44.3763021794296,
20.));
#73505=CARTESIAN_POINT('Ctrl Pts',(-14.9988139179602,-44.3629524800397,
0.));
#73506=CARTESIAN_POINT('Ctrl Pts',(-14.9988139179602,-44.3629524800397,
20.));
#73507=CARTESIAN_POINT('Ctrl Pts',(-15.0290271252899,-44.3495819987707,
0.));
#73508=CARTESIAN_POINT('Ctrl Pts',(-15.0290271252899,-44.3495819987707,
20.));
#73509=CARTESIAN_POINT('Ctrl Pts',(-15.0592299093033,-44.3361907430254,
0.));
#73510=CARTESIAN_POINT('Ctrl Pts',(-15.0592299093033,-44.3361907430254,
20.));
#73511=CARTESIAN_POINT('Ctrl Pts',(-15.0894222554425,-44.3227787202166,
0.));
#73512=CARTESIAN_POINT('Ctrl Pts',(-15.0894222554425,-44.3227787202166,
20.));
#73513=CARTESIAN_POINT('Ctrl Pts',(-15.1196041491546,-44.3093459377674,
0.));
#73514=CARTESIAN_POINT('Ctrl Pts',(-15.1196041491546,-44.3093459377674,
20.));
#73515=CARTESIAN_POINT('Ctrl Pts',(-15.1497755758918,-44.2958924031118,
0.));
#73516=CARTESIAN_POINT('Ctrl Pts',(-15.1497755758918,-44.2958924031118,
20.));
#73517=CARTESIAN_POINT('Ctrl Pts',(-15.1799365211114,-44.2824181236961,
0.));
#73518=CARTESIAN_POINT('Ctrl Pts',(-15.1799365211114,-44.2824181236961,
20.));
#73519=CARTESIAN_POINT('Ctrl Pts',(-15.2100869702755,-44.2689231069767,
0.));
#73520=CARTESIAN_POINT('Ctrl Pts',(-15.2100869702755,-44.2689231069767,
20.));
#73521=CARTESIAN_POINT('Ctrl Pts',(-15.2402269088514,-44.2554073604206,
0.));
#73522=CARTESIAN_POINT('Ctrl Pts',(-15.2402269088514,-44.2554073604206,
20.));
#73523=CARTESIAN_POINT('Ctrl Pts',(-15.2703563223108,-44.2418708915045,
0.));
#73524=CARTESIAN_POINT('Ctrl Pts',(-15.2703563223108,-44.2418708915045,
20.));
#73525=CARTESIAN_POINT('Ctrl Pts',(-15.30047519613,-44.2283137077152,0.));
#73526=CARTESIAN_POINT('Ctrl Pts',(-15.30047519613,-44.2283137077152,20.));
#73527=CARTESIAN_POINT('Ctrl Pts',(-15.3305835157903,-44.2147358165492,
0.));
#73528=CARTESIAN_POINT('Ctrl Pts',(-15.3305835157903,-44.2147358165492,
20.));
#73529=CARTESIAN_POINT('Ctrl Pts',(-15.3606812667781,-44.201137225514,0.));
#73530=CARTESIAN_POINT('Ctrl Pts',(-15.3606812667781,-44.201137225514,20.));
#73531=CARTESIAN_POINT('Ctrl Pts',(-15.390768434585,-44.1875179421286,0.));
#73532=CARTESIAN_POINT('Ctrl Pts',(-15.390768434585,-44.1875179421286,20.));
#73533=CARTESIAN_POINT('Ctrl Pts',(-15.4208450047077,-44.1738779739224,
0.));
#73534=CARTESIAN_POINT('Ctrl Pts',(-15.4208450047077,-44.1738779739224,
20.));
#73535=CARTESIAN_POINT('Ctrl Pts',(-15.4509109626472,-44.1602173284345,
0.));
#73536=CARTESIAN_POINT('Ctrl Pts',(-15.4509109626472,-44.1602173284345,
20.));
#73537=CARTESIAN_POINT('Ctrl Pts',(-15.4809662939093,-44.146536013213,0.));
#73538=CARTESIAN_POINT('Ctrl Pts',(-15.4809662939093,-44.146536013213,20.));
#73539=CARTESIAN_POINT('Ctrl Pts',(-15.5110109840048,-44.1328340358171,
0.));
#73540=CARTESIAN_POINT('Ctrl Pts',(-15.5110109840048,-44.1328340358171,
20.));
#73541=CARTESIAN_POINT('Ctrl Pts',(-15.5410450184494,-44.1191114038164,
0.));
#73542=CARTESIAN_POINT('Ctrl Pts',(-15.5410450184494,-44.1191114038164,
20.));
#73543=CARTESIAN_POINT('Ctrl Pts',(-15.5710683827646,-44.1053681247921,
0.));
#73544=CARTESIAN_POINT('Ctrl Pts',(-15.5710683827646,-44.1053681247921,
20.));
#73545=CARTESIAN_POINT('Ctrl Pts',(-15.6010810624766,-44.0916042063371,
0.));
#73546=CARTESIAN_POINT('Ctrl Pts',(-15.6010810624766,-44.0916042063371,
20.));
#73547=CARTESIAN_POINT('Ctrl Pts',(-15.6310830431167,-44.0778196560536,
0.));
#73548=CARTESIAN_POINT('Ctrl Pts',(-15.6310830431167,-44.0778196560536,
20.));
#73549=CARTESIAN_POINT('Ctrl Pts',(-15.6610743102207,-44.0640144815534,
0.));
#73550=CARTESIAN_POINT('Ctrl Pts',(-15.6610743102207,-44.0640144815534,
20.));
#73551=CARTESIAN_POINT('Ctrl Pts',(-15.6910548493289,-44.050188690457,0.));
#73552=CARTESIAN_POINT('Ctrl Pts',(-15.6910548493289,-44.050188690457,20.));
#73553=CARTESIAN_POINT('Ctrl Pts',(-15.7210246459868,-44.0363422903955,
0.));
#73554=CARTESIAN_POINT('Ctrl Pts',(-15.7210246459868,-44.0363422903955,
20.));
#73555=CARTESIAN_POINT('Ctrl Pts',(-15.7509836857452,-44.0224752890112,
0.));
#73556=CARTESIAN_POINT('Ctrl Pts',(-15.7509836857452,-44.0224752890112,
20.));
#73557=CARTESIAN_POINT('Ctrl Pts',(-15.7809319541602,-44.0085876939576,
0.));
#73558=CARTESIAN_POINT('Ctrl Pts',(-15.7809319541602,-44.0085876939576,
20.));
#73559=CARTESIAN_POINT('Ctrl Pts',(-15.8108694367927,-43.9946795128988,
0.));
#73560=CARTESIAN_POINT('Ctrl Pts',(-15.8108694367927,-43.9946795128988,
20.));
#73561=CARTESIAN_POINT('Ctrl Pts',(-15.8407961192089,-43.9807507535096,
0.));
#73562=CARTESIAN_POINT('Ctrl Pts',(-15.8407961192089,-43.9807507535096,
20.));
#73563=CARTESIAN_POINT('Ctrl Pts',(-15.8707119869797,-43.9668014234746,
0.));
#73564=CARTESIAN_POINT('Ctrl Pts',(-15.8707119869797,-43.9668014234746,
20.));
#73565=CARTESIAN_POINT('Ctrl Pts',(-15.9006170256808,-43.9528315304878,
0.));
#73566=CARTESIAN_POINT('Ctrl Pts',(-15.9006170256808,-43.9528315304878,
20.));
#73567=CARTESIAN_POINT('Ctrl Pts',(-15.9305112208934,-43.9388410822542,
0.));
#73568=CARTESIAN_POINT('Ctrl Pts',(-15.9305112208934,-43.9388410822542,
20.));
#73569=CARTESIAN_POINT('Ctrl Pts',(-15.9603945582034,-43.9248300864889,
0.));
#73570=CARTESIAN_POINT('Ctrl Pts',(-15.9603945582034,-43.9248300864889,
20.));
#73571=CARTESIAN_POINT('Ctrl Pts',(-15.9902670232019,-43.9107985509168,
0.));
#73572=CARTESIAN_POINT('Ctrl Pts',(-15.9902670232019,-43.9107985509168,
20.));
#73573=CARTESIAN_POINT('Ctrl Pts',(-16.020128601485,-43.896746483274,0.));
#73574=CARTESIAN_POINT('Ctrl Pts',(-16.020128601485,-43.896746483274,20.));
#73575=CARTESIAN_POINT('Ctrl Pts',(-16.0499792786541,-43.8826738913074,
0.));
#73576=CARTESIAN_POINT('Ctrl Pts',(-16.0499792786541,-43.8826738913074,
20.));
#73577=CARTESIAN_POINT('Ctrl Pts',(-16.0798190403159,-43.8685807827745,
0.));
#73578=CARTESIAN_POINT('Ctrl Pts',(-16.0798190403159,-43.8685807827745,
20.));
#73579=CARTESIAN_POINT('Ctrl Pts',(-16.1096478720818,-43.854467165442,0.));
#73580=CARTESIAN_POINT('Ctrl Pts',(-16.1096478720818,-43.854467165442,20.));
#73581=CARTESIAN_POINT('Ctrl Pts',(-16.1394657595683,-43.8403330470868,
0.));
#73582=CARTESIAN_POINT('Ctrl Pts',(-16.1394657595683,-43.8403330470868,
20.));
#73583=CARTESIAN_POINT('Ctrl Pts',(-16.1692726883968,-43.8261784354962,
0.));
#73584=CARTESIAN_POINT('Ctrl Pts',(-16.1692726883968,-43.8261784354962,
20.));
#73585=CARTESIAN_POINT('Ctrl Pts',(-16.199068644194,-43.8120033384679,0.));
#73586=CARTESIAN_POINT('Ctrl Pts',(-16.199068644194,-43.8120033384679,20.));
#73587=CARTESIAN_POINT('Ctrl Pts',(-16.2288536125917,-43.7978077638098,
0.));
#73588=CARTESIAN_POINT('Ctrl Pts',(-16.2288536125917,-43.7978077638098,
20.));
#73589=CARTESIAN_POINT('Ctrl Pts',(-16.2586275792268,-43.7835917193404,
0.));
#73590=CARTESIAN_POINT('Ctrl Pts',(-16.2586275792268,-43.7835917193404,
20.));
#73591=CARTESIAN_POINT('Ctrl Pts',(-16.2883905297415,-43.7693552128887,
0.));
#73592=CARTESIAN_POINT('Ctrl Pts',(-16.2883905297415,-43.7693552128887,
20.));
#73593=CARTESIAN_POINT('Ctrl Pts',(-16.3181424497834,-43.7550982522947,
0.));
#73594=CARTESIAN_POINT('Ctrl Pts',(-16.3181424497834,-43.7550982522947,
20.));
#73595=CARTESIAN_POINT('Ctrl Pts',(-16.3478833250055,-43.7408208454089,
0.));
#73596=CARTESIAN_POINT('Ctrl Pts',(-16.3478833250055,-43.7408208454089,
20.));
#73597=CARTESIAN_POINT('Ctrl Pts',(-16.3776131410651,-43.7265230000909,
0.));
#73598=CARTESIAN_POINT('Ctrl Pts',(-16.3776131410651,-43.7265230000909,
20.));
#73599=CARTESIAN_POINT('Ctrl Pts',(-16.4073318836249,-43.7122047242097,
0.));
#73600=CARTESIAN_POINT('Ctrl Pts',(-16.4073318836249,-43.7122047242097,
20.));
#73601=CARTESIAN_POINT('Ctrl Pts',(-16.4370395383524,-43.6978660256455,
0.));
#73602=CARTESIAN_POINT('Ctrl Pts',(-16.4370395383524,-43.6978660256455,
20.));
#73603=CARTESIAN_POINT('Ctrl Pts',(-16.4667360909207,-43.6835069122887,
0.));
#73604=CARTESIAN_POINT('Ctrl Pts',(-16.4667360909207,-43.6835069122887,
20.));
#73605=CARTESIAN_POINT('Ctrl Pts',(-16.4964215270082,-43.6691273920409,
0.));
#73606=CARTESIAN_POINT('Ctrl Pts',(-16.4964215270082,-43.6691273920409,
20.));
#73607=CARTESIAN_POINT('Ctrl Pts',(-16.5260958322991,-43.6547274728139,
0.));
#73608=CARTESIAN_POINT('Ctrl Pts',(-16.5260958322991,-43.6547274728139,
20.));
#73609=CARTESIAN_POINT('Ctrl Pts',(-16.5557589924819,-43.640307162529,0.));
#73610=CARTESIAN_POINT('Ctrl Pts',(-16.5557589924819,-43.640307162529,20.));
#73611=CARTESIAN_POINT('Ctrl Pts',(-16.5854109932504,-43.6258664691173,
0.));
#73612=CARTESIAN_POINT('Ctrl Pts',(-16.5854109932504,-43.6258664691173,
20.));
#73613=CARTESIAN_POINT('Ctrl Pts',(-16.6150518203036,-43.6114054005208,
0.));
#73614=CARTESIAN_POINT('Ctrl Pts',(-16.6150518203036,-43.6114054005208,
20.));
#73615=CARTESIAN_POINT('Ctrl Pts',(-16.6446814593459,-43.5969239646926,
0.));
#73616=CARTESIAN_POINT('Ctrl Pts',(-16.6446814593459,-43.5969239646926,
20.));
#73617=CARTESIAN_POINT('Ctrl Pts',(-16.6742998960869,-43.5824221695961,
0.));
#73618=CARTESIAN_POINT('Ctrl Pts',(-16.6742998960869,-43.5824221695961,
20.));
#73619=CARTESIAN_POINT('Ctrl Pts',(-16.7039071162413,-43.5679000232041,
0.));
#73620=CARTESIAN_POINT('Ctrl Pts',(-16.7039071162413,-43.5679000232041,
20.));
#73621=CARTESIAN_POINT('Ctrl Pts',(-16.7335031055295,-43.5533575334996,
0.));
#73622=CARTESIAN_POINT('Ctrl Pts',(-16.7335031055295,-43.5533575334996,
20.));
#73623=CARTESIAN_POINT('Ctrl Pts',(-16.7630878496767,-43.5387947084755,
0.));
#73624=CARTESIAN_POINT('Ctrl Pts',(-16.7630878496767,-43.5387947084755,
20.));
#73625=CARTESIAN_POINT('Ctrl Pts',(-16.792661334414,-43.5242115561352,0.));
#73626=CARTESIAN_POINT('Ctrl Pts',(-16.792661334414,-43.5242115561352,20.));
#73627=CARTESIAN_POINT('Ctrl Pts',(-16.8222235454772,-43.5096080844922,
0.));
#73628=CARTESIAN_POINT('Ctrl Pts',(-16.8222235454772,-43.5096080844922,
20.));
#73629=CARTESIAN_POINT('Ctrl Pts',(-16.8517744686076,-43.4949843015709,
0.));
#73630=CARTESIAN_POINT('Ctrl Pts',(-16.8517744686076,-43.4949843015709,
20.));
#73631=CARTESIAN_POINT('Ctrl Pts',(-16.8813140895513,-43.4803402154062,
0.));
#73632=CARTESIAN_POINT('Ctrl Pts',(-16.8813140895513,-43.4803402154062,
20.));
#73633=CARTESIAN_POINT('Ctrl Pts',(-16.91084239406,-43.4656758340435,0.));
#73634=CARTESIAN_POINT('Ctrl Pts',(-16.91084239406,-43.4656758340435,20.));
#73635=CARTESIAN_POINT('Ctrl Pts',(-16.9403593678908,-43.4509911655382,
0.));
#73636=CARTESIAN_POINT('Ctrl Pts',(-16.9403593678908,-43.4509911655382,
20.));
#73637=CARTESIAN_POINT('Ctrl Pts',(-16.9698649968061,-43.4362862179557,
0.));
#73638=CARTESIAN_POINT('Ctrl Pts',(-16.9698649968061,-43.4362862179557,
20.));
#73639=CARTESIAN_POINT('Ctrl Pts',(-16.9993592665737,-43.4215609993712,
0.));
#73640=CARTESIAN_POINT('Ctrl Pts',(-16.9993592665737,-43.4215609993712,
20.));
#73641=CARTESIAN_POINT('Ctrl Pts',(-17.0288421629666,-43.4068155178695,
0.));
#73642=CARTESIAN_POINT('Ctrl Pts',(-17.0288421629666,-43.4068155178695,
20.));
#73643=CARTESIAN_POINT('Ctrl Pts',(-17.0583136717632,-43.3920497815463,
0.));
#73644=CARTESIAN_POINT('Ctrl Pts',(-17.0583136717632,-43.3920497815463,
20.));
#73645=CARTESIAN_POINT('Ctrl Pts',(-17.0877737787472,-43.3772637985072,
0.));
#73646=CARTESIAN_POINT('Ctrl Pts',(-17.0877737787472,-43.3772637985072,
20.));
#73647=CARTESIAN_POINT('Ctrl Pts',(-17.1172224697079,-43.3624575768695,
0.));
#73648=CARTESIAN_POINT('Ctrl Pts',(-17.1172224697079,-43.3624575768695,
20.));
#73649=CARTESIAN_POINT('Ctrl Pts',(-17.1466597304397,-43.3476311247602,
0.));
#73650=CARTESIAN_POINT('Ctrl Pts',(-17.1466597304397,-43.3476311247602,
20.));
#73651=CARTESIAN_POINT('Ctrl Pts',(-17.1760855467426,-43.332784450317,0.));
#73652=CARTESIAN_POINT('Ctrl Pts',(-17.1760855467426,-43.332784450317,20.));
#73653=CARTESIAN_POINT('Ctrl Pts',(-17.2054999044213,-43.3179175616862,
0.));
#73654=CARTESIAN_POINT('Ctrl Pts',(-17.2054999044213,-43.3179175616862,
20.));
#73655=CARTESIAN_POINT('Ctrl Pts',(-17.2349027892859,-43.3030304670242,
0.));
#73656=CARTESIAN_POINT('Ctrl Pts',(-17.2349027892859,-43.3030304670242,
20.));
#73657=CARTESIAN_POINT('Ctrl Pts',(-17.2642941871522,-43.2881231744974,
0.));
#73658=CARTESIAN_POINT('Ctrl Pts',(-17.2642941871522,-43.2881231744974,
20.));
#73659=CARTESIAN_POINT('Ctrl Pts',(-17.2936740838416,-43.2731956922839,
0.));
#73660=CARTESIAN_POINT('Ctrl Pts',(-17.2936740838416,-43.2731956922839,
20.));
#73661=CARTESIAN_POINT('Ctrl Pts',(-17.3230424651811,-43.258248028572,0.));
#73662=CARTESIAN_POINT('Ctrl Pts',(-17.3230424651811,-43.258248028572,20.));
#73663=CARTESIAN_POINT('Ctrl Pts',(-17.3523993170031,-43.2432801915607,
0.));
#73664=CARTESIAN_POINT('Ctrl Pts',(-17.3523993170031,-43.2432801915607,
20.));
#73665=CARTESIAN_POINT('Ctrl Pts',(-17.3817446251452,-43.2282921894589,
0.));
#73666=CARTESIAN_POINT('Ctrl Pts',(-17.3817446251452,-43.2282921894589,
20.));
#73667=CARTESIAN_POINT('Ctrl Pts',(-17.4110783754507,-43.2132840304854,
0.));
#73668=CARTESIAN_POINT('Ctrl Pts',(-17.4110783754507,-43.2132840304854,
20.));
#73669=CARTESIAN_POINT('Ctrl Pts',(-17.4404005537678,-43.1982557228684,
0.));
#73670=CARTESIAN_POINT('Ctrl Pts',(-17.4404005537678,-43.1982557228684,
20.));
#73671=CARTESIAN_POINT('Ctrl Pts',(-17.4697111459501,-43.1832072748459,
0.));
#73672=CARTESIAN_POINT('Ctrl Pts',(-17.4697111459501,-43.1832072748459,
20.));
#73673=CARTESIAN_POINT('Ctrl Pts',(-17.4990101378563,-43.1681386946662,
0.));
#73674=CARTESIAN_POINT('Ctrl Pts',(-17.4990101378563,-43.1681386946662,
20.));
#73675=CARTESIAN_POINT('Ctrl Pts',(-17.5282975153509,-43.1530499905879,
0.));
#73676=CARTESIAN_POINT('Ctrl Pts',(-17.5282975153509,-43.1530499905879,
20.));
#73677=CARTESIAN_POINT('Ctrl Pts',(-17.557573264304,-43.1379411708804,0.));
#73678=CARTESIAN_POINT('Ctrl Pts',(-17.557573264304,-43.1379411708804,20.));
#73679=CARTESIAN_POINT('Ctrl Pts',(-17.5868373705916,-43.122812243824,0.));
#73680=CARTESIAN_POINT('Ctrl Pts',(-17.5868373705916,-43.122812243824,20.));
#73681=CARTESIAN_POINT('Ctrl Pts',(-17.6160898200949,-43.1076632177088,
0.));
#73682=CARTESIAN_POINT('Ctrl Pts',(-17.6160898200949,-43.1076632177088,
20.));
#73683=CARTESIAN_POINT('Ctrl Pts',(-17.645330598701,-43.0924941008354,0.));
#73684=CARTESIAN_POINT('Ctrl Pts',(-17.645330598701,-43.0924941008354,20.));
#73685=CARTESIAN_POINT('Ctrl Pts',(-17.674559692302,-43.0773049015136,0.));
#73686=CARTESIAN_POINT('Ctrl Pts',(-17.674559692302,-43.0773049015136,20.));
#73687=CARTESIAN_POINT('Ctrl Pts',(-17.7037770867956,-43.0620956280638,
0.));
#73688=CARTESIAN_POINT('Ctrl Pts',(-17.7037770867956,-43.0620956280638,
20.));
#73689=CARTESIAN_POINT('Ctrl Pts',(-17.7329827680847,-43.0468662888157,
0.));
#73690=CARTESIAN_POINT('Ctrl Pts',(-17.7329827680847,-43.0468662888157,
20.));
#73691=CARTESIAN_POINT('Ctrl Pts',(-17.7621767220773,-43.0316168921093,
0.));
#73692=CARTESIAN_POINT('Ctrl Pts',(-17.7621767220773,-43.0316168921093,
20.));
#73693=CARTESIAN_POINT('Ctrl Pts',(-17.7913589346876,-43.0163474462951,
0.));
#73694=CARTESIAN_POINT('Ctrl Pts',(-17.7913589346876,-43.0163474462951,
20.));
#73695=CARTESIAN_POINT('Ctrl Pts',(-17.8205293918351,-43.0010579597341,
0.));
#73696=CARTESIAN_POINT('Ctrl Pts',(-17.8205293918351,-43.0010579597341,
20.));
#73697=CARTESIAN_POINT('Ctrl Pts',(-17.8496880794454,-42.9857484407979,
0.));
#73698=CARTESIAN_POINT('Ctrl Pts',(-17.8496880794454,-42.9857484407979,
20.));
#73699=CARTESIAN_POINT('Ctrl Pts',(-17.8788349834491,-42.9704188978681,
0.));
#73700=CARTESIAN_POINT('Ctrl Pts',(-17.8788349834491,-42.9704188978681,
20.));
#73701=CARTESIAN_POINT('Ctrl Pts',(-17.9079700897828,-42.9550693393359,
0.));
#73702=CARTESIAN_POINT('Ctrl Pts',(-17.9079700897828,-42.9550693393359,
20.));
#73703=CARTESIAN_POINT('Ctrl Pts',(-17.9370933843882,-42.9396997736018,
0.));
#73704=CARTESIAN_POINT('Ctrl Pts',(-17.9370933843882,-42.9396997736018,
20.));
#73705=CARTESIAN_POINT('Ctrl Pts',(-17.9662048532126,-42.9243102090766,
0.));
#73706=CARTESIAN_POINT('Ctrl Pts',(-17.9662048532126,-42.9243102090766,
20.));
#73707=CARTESIAN_POINT('Ctrl Pts',(-17.9953044822088,-42.9089006541818,
0.));
#73708=CARTESIAN_POINT('Ctrl Pts',(-17.9953044822088,-42.9089006541818,
20.));
#73709=CARTESIAN_POINT('Ctrl Pts',(-18.0243922573354,-42.893471117349,0.));
#73710=CARTESIAN_POINT('Ctrl Pts',(-18.0243922573354,-42.893471117349,20.));
#73711=CARTESIAN_POINT('Ctrl Pts',(-18.0534681645565,-42.8780216070204,
0.));
#73712=CARTESIAN_POINT('Ctrl Pts',(-18.0534681645565,-42.8780216070204,
20.));
#73713=CARTESIAN_POINT('Ctrl Pts',(-18.0825321898416,-42.8625521316488,
0.));
#73714=CARTESIAN_POINT('Ctrl Pts',(-18.0825321898416,-42.8625521316488,
20.));
#73715=CARTESIAN_POINT('Ctrl Pts',(-18.1115843191668,-42.8470626996976,
0.));
#73716=CARTESIAN_POINT('Ctrl Pts',(-18.1115843191668,-42.8470626996976,
20.));
#73717=CARTESIAN_POINT('Ctrl Pts',(-18.1406245385131,-42.831553319639,0.));
#73718=CARTESIAN_POINT('Ctrl Pts',(-18.1406245385131,-42.831553319639,20.));
#73719=CARTESIAN_POINT('Ctrl Pts',(-18.1696528338673,-42.8160239999555,
0.));
#73720=CARTESIAN_POINT('Ctrl Pts',(-18.1696528338673,-42.8160239999555,
20.));
#73721=CARTESIAN_POINT('Ctrl Pts',(-18.1986691912208,-42.8004747491375,
0.));
#73722=CARTESIAN_POINT('Ctrl Pts',(-18.1986691912208,-42.8004747491375,
20.));
#73723=CARTESIAN_POINT('Ctrl Pts',(-18.2276735965714,-42.7849055756869,
0.));
#73724=CARTESIAN_POINT('Ctrl Pts',(-18.2276735965714,-42.7849055756869,
20.));
#73725=CARTESIAN_POINT('Ctrl Pts',(-18.256666035922,-42.7693164881155,0.));
#73726=CARTESIAN_POINT('Ctrl Pts',(-18.256666035922,-42.7693164881155,20.));
#73727=CARTESIAN_POINT('Ctrl Pts',(-18.285646495282,-42.7537074949463,0.));
#73728=CARTESIAN_POINT('Ctrl Pts',(-18.285646495282,-42.7537074949463,20.));
#73729=CARTESIAN_POINT('Ctrl Pts',(-18.3146149606662,-42.7380786047127,
0.));
#73730=CARTESIAN_POINT('Ctrl Pts',(-18.3146149606662,-42.7380786047127,
20.));
#73731=CARTESIAN_POINT('Ctrl Pts',(-18.3435714180954,-42.7224298259587,
0.));
#73732=CARTESIAN_POINT('Ctrl Pts',(-18.3435714180954,-42.7224298259587,
20.));
#73733=CARTESIAN_POINT('Ctrl Pts',(-18.372515853596,-42.7067611672378,0.));
#73734=CARTESIAN_POINT('Ctrl Pts',(-18.372515853596,-42.7067611672378,20.));
#73735=CARTESIAN_POINT('Ctrl Pts',(-18.4014482531999,-42.6910726371132,
0.));
#73736=CARTESIAN_POINT('Ctrl Pts',(-18.4014482531999,-42.6910726371132,
20.));
#73737=CARTESIAN_POINT('Ctrl Pts',(-18.4303686029444,-42.6753642441576,
0.));
#73738=CARTESIAN_POINT('Ctrl Pts',(-18.4303686029444,-42.6753642441576,
20.));
#73739=CARTESIAN_POINT('Ctrl Pts',(-18.4592768888724,-42.6596359969538,
0.));
#73740=CARTESIAN_POINT('Ctrl Pts',(-18.4592768888724,-42.6596359969538,
20.));
#73741=CARTESIAN_POINT('Ctrl Pts',(-18.4881730970326,-42.6438879040941,
0.));
#73742=CARTESIAN_POINT('Ctrl Pts',(-18.4881730970326,-42.6438879040941,
20.));
#73743=CARTESIAN_POINT('Ctrl Pts',(-18.5170572134793,-42.6281199741818,
0.));
#73744=CARTESIAN_POINT('Ctrl Pts',(-18.5170572134793,-42.6281199741818,
20.));
#73745=CARTESIAN_POINT('Ctrl Pts',(-18.5459292242727,-42.61233221583,0.));
#73746=CARTESIAN_POINT('Ctrl Pts',(-18.5459292242727,-42.61233221583,20.));
#73747=CARTESIAN_POINT('Ctrl Pts',(-18.574789115479,-42.596524637663,0.));
#73748=CARTESIAN_POINT('Ctrl Pts',(-18.574789115479,-42.596524637663,20.));
#73749=CARTESIAN_POINT('Ctrl Pts',(-18.6036368731702,-42.5806972483146,
0.));
#73750=CARTESIAN_POINT('Ctrl Pts',(-18.6036368731702,-42.5806972483146,
20.));
#73751=CARTESIAN_POINT('Ctrl Pts',(-18.632472483424,-42.5648500564287,0.));
#73752=CARTESIAN_POINT('Ctrl Pts',(-18.632472483424,-42.5648500564287,20.));
#73753=CARTESIAN_POINT('Ctrl Pts',(-18.6612959323233,-42.5489830706585,
0.));
#73754=CARTESIAN_POINT('Ctrl Pts',(-18.6612959323233,-42.5489830706585,
20.));
#73755=CARTESIAN_POINT('Ctrl Pts',(-18.6901072059568,-42.5330962996668,
0.));
#73756=CARTESIAN_POINT('Ctrl Pts',(-18.6901072059568,-42.5330962996668,
20.));
#73757=CARTESIAN_POINT('Ctrl Pts',(-18.718906290419,-42.5171897521269,0.));
#73758=CARTESIAN_POINT('Ctrl Pts',(-18.718906290419,-42.5171897521269,20.));
#73759=CARTESIAN_POINT('Ctrl Pts',(-18.7476931718101,-42.5012634367222,
0.));
#73760=CARTESIAN_POINT('Ctrl Pts',(-18.7476931718101,-42.5012634367222,
20.));
#73761=CARTESIAN_POINT('Ctrl Pts',(-18.7764678362368,-42.4853173621469,
0.));
#73762=CARTESIAN_POINT('Ctrl Pts',(-18.7764678362368,-42.4853173621469,
20.));
#73763=CARTESIAN_POINT('Ctrl Pts',(-18.8052302698113,-42.4693515371059,
0.));
#73764=CARTESIAN_POINT('Ctrl Pts',(-18.8052302698113,-42.4693515371059,
20.));
#73765=CARTESIAN_POINT('Ctrl Pts',(-18.8339804586522,-42.4533659703145,
0.));
#73766=CARTESIAN_POINT('Ctrl Pts',(-18.8339804586522,-42.4533659703145,
20.));
#73767=CARTESIAN_POINT('Ctrl Pts',(-18.8627183888827,-42.4373606704956,
0.));
#73768=CARTESIAN_POINT('Ctrl Pts',(-18.8627183888827,-42.4373606704956,
20.));
#73769=CARTESIAN_POINT('Ctrl Pts',(-18.8914440466322,-42.4213356463824,
0.));
#73770=CARTESIAN_POINT('Ctrl Pts',(-18.8914440466322,-42.4213356463824,
20.));
#73771=CARTESIAN_POINT('Ctrl Pts',(-18.9201574180352,-42.4052909067172,
0.));
#73772=CARTESIAN_POINT('Ctrl Pts',(-18.9201574180352,-42.4052909067172,
20.));
#73773=CARTESIAN_POINT('Ctrl Pts',(-18.9488584892326,-42.389226460254,0.));
#73774=CARTESIAN_POINT('Ctrl Pts',(-18.9488584892326,-42.389226460254,20.));
#73775=CARTESIAN_POINT('Ctrl Pts',(-18.9775472463711,-42.3731423157568,
0.));
#73776=CARTESIAN_POINT('Ctrl Pts',(-18.9775472463711,-42.3731423157568,
20.));
#73777=CARTESIAN_POINT('Ctrl Pts',(-19.0062236756035,-42.3570384820003,
0.));
#73778=CARTESIAN_POINT('Ctrl Pts',(-19.0062236756035,-42.3570384820003,
20.));
#73779=CARTESIAN_POINT('Ctrl Pts',(-19.0348877630887,-42.3409149677685,
0.));
#73780=CARTESIAN_POINT('Ctrl Pts',(-19.0348877630887,-42.3409149677685,
20.));
#73781=CARTESIAN_POINT('Ctrl Pts',(-19.0635394949913,-42.3247717818558,
0.));
#73782=CARTESIAN_POINT('Ctrl Pts',(-19.0635394949913,-42.3247717818558,
20.));
#73783=CARTESIAN_POINT('Ctrl Pts',(-19.0921788574819,-42.3086089330657,
0.));
#73784=CARTESIAN_POINT('Ctrl Pts',(-19.0921788574819,-42.3086089330657,
20.));
#73785=CARTESIAN_POINT('Ctrl Pts',(-19.1208058367362,-42.2924264302113,
0.));
#73786=CARTESIAN_POINT('Ctrl Pts',(-19.1208058367362,-42.2924264302113,
20.));
#73787=CARTESIAN_POINT('Ctrl Pts',(-19.1494204189361,-42.2762242821163,
0.));
#73788=CARTESIAN_POINT('Ctrl Pts',(-19.1494204189361,-42.2762242821163,
20.));
#73789=CARTESIAN_POINT('Ctrl Pts',(-19.1780225902694,-42.2600024976146,
0.));
#73790=CARTESIAN_POINT('Ctrl Pts',(-19.1780225902694,-42.2600024976146,
20.));
#73791=CARTESIAN_POINT('Ctrl Pts',(-19.2066123369297,-42.2437610855506,
0.));
#73792=CARTESIAN_POINT('Ctrl Pts',(-19.2066123369297,-42.2437610855506,
20.));
#73793=CARTESIAN_POINT('Ctrl Pts',(-19.2351896451166,-42.2275000547783,
0.));
#73794=CARTESIAN_POINT('Ctrl Pts',(-19.2351896451166,-42.2275000547783,
20.));
#73795=CARTESIAN_POINT('Ctrl Pts',(-19.2637545010356,-42.2112194141618,
0.));
#73796=CARTESIAN_POINT('Ctrl Pts',(-19.2637545010356,-42.2112194141618,
20.));
#73797=CARTESIAN_POINT('Ctrl Pts',(-19.2923068908981,-42.1949191725745,
0.));
#73798=CARTESIAN_POINT('Ctrl Pts',(-19.2923068908981,-42.1949191725745,
20.));
#73799=CARTESIAN_POINT('Ctrl Pts',(-19.3208468009212,-42.1785993388989,
0.));
#73800=CARTESIAN_POINT('Ctrl Pts',(-19.3208468009212,-42.1785993388989,
20.));
#73801=CARTESIAN_POINT('Ctrl Pts',(-19.3493742173283,-42.1622599220289,
0.));
#73802=CARTESIAN_POINT('Ctrl Pts',(-19.3493742173283,-42.1622599220289,
20.));
#73803=CARTESIAN_POINT('Ctrl Pts',(-19.377889126349,-42.1459009308685,0.));
#73804=CARTESIAN_POINT('Ctrl Pts',(-19.377889126349,-42.1459009308685,20.));
#73805=CARTESIAN_POINT('Ctrl Pts',(-19.4063915142187,-42.1295223743319,
0.));
#73806=CARTESIAN_POINT('Ctrl Pts',(-19.4063915142187,-42.1295223743319,
20.));
#73807=CARTESIAN_POINT('Ctrl Pts',(-19.4348813671785,-42.1131242613432,
0.));
#73808=CARTESIAN_POINT('Ctrl Pts',(-19.4348813671785,-42.1131242613432,
20.));
#73809=CARTESIAN_POINT('Ctrl Pts',(-19.4633586714748,-42.0967066008354,
0.));
#73810=CARTESIAN_POINT('Ctrl Pts',(-19.4633586714748,-42.0967066008354,
20.));
#73811=CARTESIAN_POINT('Ctrl Pts',(-19.4918234133604,-42.080269401751,0.));
#73812=CARTESIAN_POINT('Ctrl Pts',(-19.4918234133604,-42.080269401751,20.));
#73813=CARTESIAN_POINT('Ctrl Pts',(-19.520275579094,-42.0638126730426,0.));
#73814=CARTESIAN_POINT('Ctrl Pts',(-19.520275579094,-42.0638126730426,20.));
#73815=CARTESIAN_POINT('Ctrl Pts',(-19.5487151549408,-42.0473364236742,
0.));
#73816=CARTESIAN_POINT('Ctrl Pts',(-19.5487151549408,-42.0473364236742,
20.));
#73817=CARTESIAN_POINT('Ctrl Pts',(-19.5771421271718,-42.0308406626191,
0.));
#73818=CARTESIAN_POINT('Ctrl Pts',(-19.5771421271718,-42.0308406626191,
20.));
#73819=CARTESIAN_POINT('Ctrl Pts',(-19.6055564820642,-42.0143253988608,
0.));
#73820=CARTESIAN_POINT('Ctrl Pts',(-19.6055564820642,-42.0143253988608,
20.));
#73821=CARTESIAN_POINT('Ctrl Pts',(-19.6339582059009,-41.997790641393,0.));
#73822=CARTESIAN_POINT('Ctrl Pts',(-19.6339582059009,-41.997790641393,20.));
#73823=CARTESIAN_POINT('Ctrl Pts',(-19.6623472849704,-41.9812363992182,
0.));
#73824=CARTESIAN_POINT('Ctrl Pts',(-19.6623472849704,-41.9812363992182,
20.));
#73825=CARTESIAN_POINT('Ctrl Pts',(-19.6907237055675,-41.9646626813489,
0.));
#73826=CARTESIAN_POINT('Ctrl Pts',(-19.6907237055675,-41.9646626813489,
20.));
#73827=CARTESIAN_POINT('Ctrl Pts',(-19.7190874539927,-41.9480694968077,
0.));
#73828=CARTESIAN_POINT('Ctrl Pts',(-19.7190874539927,-41.9480694968077,
20.));
#73829=CARTESIAN_POINT('Ctrl Pts',(-19.7474385165532,-41.9314568546275,
0.));
#73830=CARTESIAN_POINT('Ctrl Pts',(-19.7474385165532,-41.9314568546275,
20.));
#73831=CARTESIAN_POINT('Ctrl Pts',(-19.775776879562,-41.9148247638512,0.));
#73832=CARTESIAN_POINT('Ctrl Pts',(-19.775776879562,-41.9148247638512,20.));
#73833=CARTESIAN_POINT('Ctrl Pts',(-19.8041025293385,-41.8981732335313,
0.));
#73834=CARTESIAN_POINT('Ctrl Pts',(-19.8041025293385,-41.8981732335313,
20.));
#73835=CARTESIAN_POINT('Ctrl Pts',(-19.8324154522082,-41.8815022727306,
0.));
#73836=CARTESIAN_POINT('Ctrl Pts',(-19.8324154522082,-41.8815022727306,
20.));
#73837=CARTESIAN_POINT('Ctrl Pts',(-19.8607156345021,-41.8648118905217,
0.));
#73838=CARTESIAN_POINT('Ctrl Pts',(-19.8607156345021,-41.8648118905217,
20.));
#73839=CARTESIAN_POINT('Ctrl Pts',(-19.889003062557,-41.8481020959867,0.));
#73840=CARTESIAN_POINT('Ctrl Pts',(-19.889003062557,-41.8481020959867,20.));
#73841=CARTESIAN_POINT('Ctrl Pts',(-19.9172777227157,-41.8313728982175,
0.));
#73842=CARTESIAN_POINT('Ctrl Pts',(-19.9172777227157,-41.8313728982175,
20.));
#73843=CARTESIAN_POINT('Ctrl Pts',(-19.945539601327,-41.8146243063151,0.));
#73844=CARTESIAN_POINT('Ctrl Pts',(-19.945539601327,-41.8146243063151,20.));
#73845=CARTESIAN_POINT('Ctrl Pts',(-19.9737886847462,-41.7978563293914,
0.));
#73846=CARTESIAN_POINT('Ctrl Pts',(-19.9737886847462,-41.7978563293914,
20.));
#73847=CARTESIAN_POINT('Ctrl Pts',(-20.0020249593348,-41.7810689765678,
0.));
#73848=CARTESIAN_POINT('Ctrl Pts',(-20.0020249593348,-41.7810689765678,
20.));
#73849=CARTESIAN_POINT('Ctrl Pts',(-20.0302484114611,-41.7642622569769,
0.));
#73850=CARTESIAN_POINT('Ctrl Pts',(-20.0302484114611,-41.7642622569769,
20.));
#73851=CARTESIAN_POINT('Ctrl Pts',(-20.0584590274992,-41.7474361797609,
0.));
#73852=CARTESIAN_POINT('Ctrl Pts',(-20.0584590274992,-41.7474361797609,
20.));
#73853=CARTESIAN_POINT('Ctrl Pts',(-20.0866567938288,-41.7305907540713,
0.));
#73854=CARTESIAN_POINT('Ctrl Pts',(-20.0866567938288,-41.7305907540713,
20.));
#73855=CARTESIAN_POINT('Ctrl Pts',(-20.1148416968357,-41.7137259890696,
0.));
#73856=CARTESIAN_POINT('Ctrl Pts',(-20.1148416968357,-41.7137259890696,
20.));
#73857=CARTESIAN_POINT('Ctrl Pts',(-20.1430137229118,-41.6968418939263,
0.));
#73858=CARTESIAN_POINT('Ctrl Pts',(-20.1430137229118,-41.6968418939263,
20.));
#73859=CARTESIAN_POINT('Ctrl Pts',(-20.1711728584549,-41.6799384778218,
0.));
#73860=CARTESIAN_POINT('Ctrl Pts',(-20.1711728584549,-41.6799384778218,
20.));
#73861=CARTESIAN_POINT('Ctrl Pts',(-20.199319089869,-41.6630157499462,0.));
#73862=CARTESIAN_POINT('Ctrl Pts',(-20.199319089869,-41.6630157499462,20.));
#73863=CARTESIAN_POINT('Ctrl Pts',(-20.2274524035648,-41.6460737195007,
0.));
#73864=CARTESIAN_POINT('Ctrl Pts',(-20.2274524035648,-41.6460737195007,
20.));
#73865=CARTESIAN_POINT('Ctrl Pts',(-20.2555727859589,-41.6291123956959,
0.));
#73866=CARTESIAN_POINT('Ctrl Pts',(-20.2555727859589,-41.6291123956959,
20.));
#73867=CARTESIAN_POINT('Ctrl Pts',(-20.2836802234745,-41.6121317877528,
0.));
#73868=CARTESIAN_POINT('Ctrl Pts',(-20.2836802234745,-41.6121317877528,
20.));
#73869=CARTESIAN_POINT('Ctrl Pts',(-20.3117747025404,-41.5951319049016,
0.));
#73870=CARTESIAN_POINT('Ctrl Pts',(-20.3117747025404,-41.5951319049016,
20.));
#73871=CARTESIAN_POINT('Ctrl Pts',(-20.3398562095917,-41.5781127563818,
0.));
#73872=CARTESIAN_POINT('Ctrl Pts',(-20.3398562095917,-41.5781127563818,
20.));
#73873=CARTESIAN_POINT('Ctrl Pts',(-20.3679247310694,-41.561074351443,0.));
#73874=CARTESIAN_POINT('Ctrl Pts',(-20.3679247310694,-41.561074351443,20.));
#73875=CARTESIAN_POINT('Ctrl Pts',(-20.3959802534211,-41.5440166993445,
0.));
#73876=CARTESIAN_POINT('Ctrl Pts',(-20.3959802534211,-41.5440166993445,
20.));
#73877=CARTESIAN_POINT('Ctrl Pts',(-20.4240227631002,-41.5269398093561,
0.));
#73878=CARTESIAN_POINT('Ctrl Pts',(-20.4240227631002,-41.5269398093561,
20.));
#73879=CARTESIAN_POINT('Ctrl Pts',(-20.4520522465668,-41.5098436907568,
0.));
#73880=CARTESIAN_POINT('Ctrl Pts',(-20.4520522465668,-41.5098436907568,
20.));
#73881=CARTESIAN_POINT('Ctrl Pts',(-20.4800686902869,-41.4927283528358,
0.));
#73882=CARTESIAN_POINT('Ctrl Pts',(-20.4800686902869,-41.4927283528358,
20.));
#73883=CARTESIAN_POINT('Ctrl Pts',(-20.5080720807336,-41.4755938048931,
0.));
#73884=CARTESIAN_POINT('Ctrl Pts',(-20.5080720807336,-41.4755938048931,
20.));
#73885=CARTESIAN_POINT('Ctrl Pts',(-20.5360624043854,-41.4584400562379,
0.));
#73886=CARTESIAN_POINT('Ctrl Pts',(-20.5360624043854,-41.4584400562379,
20.));
#73887=CARTESIAN_POINT('Ctrl Pts',(-20.564039647727,-41.4412671161883,0.));
#73888=CARTESIAN_POINT('Ctrl Pts',(-20.564039647727,-41.4412671161883,20.));
#73889=CARTESIAN_POINT('Ctrl Pts',(-20.592003797249,-41.4240749940721,0.));
#73890=CARTESIAN_POINT('Ctrl Pts',(-20.592003797249,-41.4240749940721,20.));
#73891=CARTESIAN_POINT('Ctrl Pts',(-20.6199548394484,-41.4068636992265,
0.));
#73892=CARTESIAN_POINT('Ctrl Pts',(-20.6199548394484,-41.4068636992265,
20.));
#73893=CARTESIAN_POINT('Ctrl Pts',(-20.6478927608288,-41.3896332409988,
0.));
#73894=CARTESIAN_POINT('Ctrl Pts',(-20.6478927608288,-41.3896332409988,
20.));
#73895=CARTESIAN_POINT('Ctrl Pts',(-20.6758175479,-41.372383628747,0.));
#73896=CARTESIAN_POINT('Ctrl Pts',(-20.6758175479,-41.372383628747,20.));
#73897=CARTESIAN_POINT('Ctrl Pts',(-20.7037291871782,-41.3551148718389,
0.));
#73898=CARTESIAN_POINT('Ctrl Pts',(-20.7037291871782,-41.3551148718389,
20.));
#73899=CARTESIAN_POINT('Ctrl Pts',(-20.731627665186,-41.3378269796522,0.));
#73900=CARTESIAN_POINT('Ctrl Pts',(-20.731627665186,-41.3378269796522,20.));
#73901=CARTESIAN_POINT('Ctrl Pts',(-20.7595129684521,-41.3205199615745,
0.));
#73902=CARTESIAN_POINT('Ctrl Pts',(-20.7595129684521,-41.3205199615745,
20.));
#73903=CARTESIAN_POINT('Ctrl Pts',(-20.7873850835117,-41.303193827003,0.));
#73904=CARTESIAN_POINT('Ctrl Pts',(-20.7873850835117,-41.303193827003,20.));
#73905=CARTESIAN_POINT('Ctrl Pts',(-20.8152439969059,-41.285848585344,0.));
#73906=CARTESIAN_POINT('Ctrl Pts',(-20.8152439969059,-41.285848585344,20.));
#73907=CARTESIAN_POINT('Ctrl Pts',(-20.8430896951822,-41.268484246013,0.));
#73908=CARTESIAN_POINT('Ctrl Pts',(-20.8430896951822,-41.268484246013,20.));
#73909=CARTESIAN_POINT('Ctrl Pts',(-20.8709221648944,-41.2511008184358,
0.));
#73910=CARTESIAN_POINT('Ctrl Pts',(-20.8709221648944,-41.2511008184358,
20.));
#73911=CARTESIAN_POINT('Ctrl Pts',(-20.8987413926025,-41.2336983120481,
0.));
#73912=CARTESIAN_POINT('Ctrl Pts',(-20.8987413926025,-41.2336983120481,
20.));
#73913=CARTESIAN_POINT('Ctrl Pts',(-20.9265473648728,-41.2162767362953,
0.));
#73914=CARTESIAN_POINT('Ctrl Pts',(-20.9265473648728,-41.2162767362953,
20.));
#73915=CARTESIAN_POINT('Ctrl Pts',(-20.9543400682781,-41.1988361006333,
0.));
#73916=CARTESIAN_POINT('Ctrl Pts',(-20.9543400682781,-41.1988361006333,
20.));
#73917=CARTESIAN_POINT('Ctrl Pts',(-20.9821194893979,-41.1813764145274,
0.));
#73918=CARTESIAN_POINT('Ctrl Pts',(-20.9821194893979,-41.1813764145274,
20.));
#73919=CARTESIAN_POINT('Ctrl Pts',(-21.009885614818,-41.1638976874526,0.));
#73920=CARTESIAN_POINT('Ctrl Pts',(-21.009885614818,-41.1638976874526,20.));
#73921=CARTESIAN_POINT('Ctrl Pts',(-21.0376384311301,-41.1463999288927,
0.));
#73922=CARTESIAN_POINT('Ctrl Pts',(-21.0376384311301,-41.1463999288927,
20.));
#73923=CARTESIAN_POINT('Ctrl Pts',(-21.0653779249329,-41.128883148342,0.));
#73924=CARTESIAN_POINT('Ctrl Pts',(-21.0653779249329,-41.128883148342,20.));
#73925=CARTESIAN_POINT('Ctrl Pts',(-21.0931040828311,-41.1113473553046,
0.));
#73926=CARTESIAN_POINT('Ctrl Pts',(-21.0931040828311,-41.1113473553046,
20.));
#73927=CARTESIAN_POINT('Ctrl Pts',(-21.1208168914355,-41.0937925592943,
0.));
#73928=CARTESIAN_POINT('Ctrl Pts',(-21.1208168914355,-41.0937925592943,
20.));
#73929=CARTESIAN_POINT('Ctrl Pts',(-21.1485163373635,-41.076218769835,0.));
#73930=CARTESIAN_POINT('Ctrl Pts',(-21.1485163373635,-41.076218769835,20.));
#73931=CARTESIAN_POINT('Ctrl Pts',(-21.1762024072388,-41.0586259964597,
0.));
#73932=CARTESIAN_POINT('Ctrl Pts',(-21.1762024072388,-41.0586259964597,
20.));
#73933=CARTESIAN_POINT('Ctrl Pts',(-21.2038750876913,-41.0410142487106,
0.));
#73934=CARTESIAN_POINT('Ctrl Pts',(-21.2038750876913,-41.0410142487106,
20.));
#73935=CARTESIAN_POINT('Ctrl Pts',(-21.2315343653574,-41.0233835361399,
0.));
#73936=CARTESIAN_POINT('Ctrl Pts',(-21.2315343653574,-41.0233835361399,
20.));
#73937=CARTESIAN_POINT('Ctrl Pts',(-21.25918022688,-41.0057338683097,0.));
#73938=CARTESIAN_POINT('Ctrl Pts',(-21.25918022688,-41.0057338683097,20.));
#73939=CARTESIAN_POINT('Ctrl Pts',(-21.286812658909,-40.9880652547927,0.));
#73940=CARTESIAN_POINT('Ctrl Pts',(-21.286812658909,-40.9880652547927,20.));
#73941=CARTESIAN_POINT('Ctrl Pts',(-21.3144316481012,-40.9703777051716,
0.));
#73942=CARTESIAN_POINT('Ctrl Pts',(-21.3144316481012,-40.9703777051716,
20.));
#73943=CARTESIAN_POINT('Ctrl Pts',(-21.342037181119,-40.9526712290373,0.));
#73944=CARTESIAN_POINT('Ctrl Pts',(-21.342037181119,-40.9526712290373,20.));
#73945=CARTESIAN_POINT('Ctrl Pts',(-21.3696292446317,-40.9349458359905,
0.));
#73946=CARTESIAN_POINT('Ctrl Pts',(-21.3696292446317,-40.9349458359905,
20.));
#73947=CARTESIAN_POINT('Ctrl Pts',(-21.3972078253142,-40.9172015356414,
0.));
#73948=CARTESIAN_POINT('Ctrl Pts',(-21.3972078253142,-40.9172015356414,
20.));
#73949=CARTESIAN_POINT('Ctrl Pts',(-21.424772909848,-40.8994383376102,0.));
#73950=CARTESIAN_POINT('Ctrl Pts',(-21.424772909848,-40.8994383376102,20.));
#73951=CARTESIAN_POINT('Ctrl Pts',(-21.45232448492,-40.8816562515268,0.));
#73952=CARTESIAN_POINT('Ctrl Pts',(-21.45232448492,-40.8816562515268,20.));
#73953=CARTESIAN_POINT('Ctrl Pts',(-21.4798625372243,-40.8638552870319,
0.));
#73954=CARTESIAN_POINT('Ctrl Pts',(-21.4798625372243,-40.8638552870319,
20.));
#73955=CARTESIAN_POINT('Ctrl Pts',(-21.5073870534614,-40.8460354537749,
0.));
#73956=CARTESIAN_POINT('Ctrl Pts',(-21.5073870534614,-40.8460354537749,
20.));
#73957=CARTESIAN_POINT('Ctrl Pts',(-21.5348980203391,-40.8281967614155,
0.));
#73958=CARTESIAN_POINT('Ctrl Pts',(-21.5348980203391,-40.8281967614155,
20.));
#73959=CARTESIAN_POINT('Ctrl Pts',(-21.5623954245725,-40.8103392196221,
0.));
#73960=CARTESIAN_POINT('Ctrl Pts',(-21.5623954245725,-40.8103392196221,
20.));
#73961=CARTESIAN_POINT('Ctrl Pts',(-21.5898792528837,-40.7924628380726,
0.));
#73962=CARTESIAN_POINT('Ctrl Pts',(-21.5898792528837,-40.7924628380726,
20.));
#73963=CARTESIAN_POINT('Ctrl Pts',(-21.6173494920019,-40.7745676264537,
0.));
#73964=CARTESIAN_POINT('Ctrl Pts',(-21.6173494920019,-40.7745676264537,
20.));
#73965=CARTESIAN_POINT('Ctrl Pts',(-21.6448061286619,-40.7566535944621,
0.));
#73966=CARTESIAN_POINT('Ctrl Pts',(-21.6448061286619,-40.7566535944621,
20.));
#73967=CARTESIAN_POINT('Ctrl Pts',(-21.6722491496038,-40.7387207518043,
0.));
#73968=CARTESIAN_POINT('Ctrl Pts',(-21.6722491496038,-40.7387207518043,
20.));
#73969=CARTESIAN_POINT('Ctrl Pts',(-21.6996785415723,-40.7207691081984,
0.));
#73970=CARTESIAN_POINT('Ctrl Pts',(-21.6996785415723,-40.7207691081984,
20.));
#73971=CARTESIAN_POINT('Ctrl Pts',(-21.7270942913167,-40.7027986733736,
0.));
#73972=CARTESIAN_POINT('Ctrl Pts',(-21.7270942913167,-40.7027986733736,
20.));
#73973=CARTESIAN_POINT('Ctrl Pts',(-21.7544963855931,-40.6848094570694,
0.));
#73974=CARTESIAN_POINT('Ctrl Pts',(-21.7544963855931,-40.6848094570694,
20.));
#73975=CARTESIAN_POINT('Ctrl Pts',(-21.781884811165,-40.6668014690334,0.));
#73976=CARTESIAN_POINT('Ctrl Pts',(-21.781884811165,-40.6668014690334,20.));
#73977=CARTESIAN_POINT('Ctrl Pts',(-21.8092595548052,-40.6487747190214,
0.));
#73978=CARTESIAN_POINT('Ctrl Pts',(-21.8092595548052,-40.6487747190214,
20.));
#73979=CARTESIAN_POINT('Ctrl Pts',(-21.8366206032979,-40.6307292167951,
0.));
#73980=CARTESIAN_POINT('Ctrl Pts',(-21.8366206032979,-40.6307292167951,
20.));
#73981=CARTESIAN_POINT('Ctrl Pts',(-21.8639679434382,-40.6126649721233,
0.));
#73982=CARTESIAN_POINT('Ctrl Pts',(-21.8639679434382,-40.6126649721233,
20.));
#73983=CARTESIAN_POINT('Ctrl Pts',(-21.8913015620281,-40.594581994783,0.));
#73984=CARTESIAN_POINT('Ctrl Pts',(-21.8913015620281,-40.594581994783,20.));
#73985=CARTESIAN_POINT('Ctrl Pts',(-21.9186214458728,-40.5764802945639,
0.));
#73986=CARTESIAN_POINT('Ctrl Pts',(-21.9186214458728,-40.5764802945639,
20.));
#73987=CARTESIAN_POINT('Ctrl Pts',(-21.9459275817778,-40.5583598812699,
0.));
#73988=CARTESIAN_POINT('Ctrl Pts',(-21.9459275817778,-40.5583598812699,
20.));
#73989=CARTESIAN_POINT('Ctrl Pts',(-21.9732199565439,-40.5402207647219,
0.));
#73990=CARTESIAN_POINT('Ctrl Pts',(-21.9732199565439,-40.5402207647219,
20.));
#73991=CARTESIAN_POINT('Ctrl Pts',(-22.0004985569689,-40.5220629547578,
0.));
#73992=CARTESIAN_POINT('Ctrl Pts',(-22.0004985569689,-40.5220629547578,
20.));
#73993=CARTESIAN_POINT('Ctrl Pts',(-22.0277633698572,-40.5038864612252,
0.));
#73994=CARTESIAN_POINT('Ctrl Pts',(-22.0277633698572,-40.5038864612252,
20.));
#73995=CARTESIAN_POINT('Ctrl Pts',(-22.0550143820281,-40.485691293976,0.));
#73996=CARTESIAN_POINT('Ctrl Pts',(-22.0550143820281,-40.485691293976,20.));
#73997=CARTESIAN_POINT('Ctrl Pts',(-22.0822515803231,-40.4674774628609,
0.));
#73998=CARTESIAN_POINT('Ctrl Pts',(-22.0822515803231,-40.4674774628609,
20.));
#73999=CARTESIAN_POINT('Ctrl Pts',(-22.1094749516164,-40.4492449777204,
0.));
#74000=CARTESIAN_POINT('Ctrl Pts',(-22.1094749516164,-40.4492449777204,
20.));
#74001=CARTESIAN_POINT('Ctrl Pts',(-22.1366844828092,-40.4309938483881,
0.));
#74002=CARTESIAN_POINT('Ctrl Pts',(-22.1366844828092,-40.4309938483881,
20.));
#74003=CARTESIAN_POINT('Ctrl Pts',(-22.1638801608087,-40.4127240847076,
0.));
#74004=CARTESIAN_POINT('Ctrl Pts',(-22.1638801608087,-40.4127240847076,
20.));
#74005=CARTESIAN_POINT('Ctrl Pts',(-22.1910619725087,-40.3944356965472,
0.));
#74006=CARTESIAN_POINT('Ctrl Pts',(-22.1910619725087,-40.3944356965472,
20.));
#74007=CARTESIAN_POINT('Ctrl Pts',(-22.2182299047735,-40.3761286938114,
0.));
#74008=CARTESIAN_POINT('Ctrl Pts',(-22.2182299047735,-40.3761286938114,
20.));
#74009=CARTESIAN_POINT('Ctrl Pts',(-22.2453839444114,-40.357803086462,0.));
#74010=CARTESIAN_POINT('Ctrl Pts',(-22.2453839444114,-40.357803086462,20.));
#74011=CARTESIAN_POINT('Ctrl Pts',(-22.2725240781926,-40.3394588845042,
0.));
#74012=CARTESIAN_POINT('Ctrl Pts',(-22.2725240781926,-40.3394588845042,
20.));
#74013=CARTESIAN_POINT('Ctrl Pts',(-22.2996502928986,-40.3210960979489,
0.));
#74014=CARTESIAN_POINT('Ctrl Pts',(-22.2996502928986,-40.3210960979489,
20.));
#74015=CARTESIAN_POINT('Ctrl Pts',(-22.3267625753671,-40.3027147367803,
0.));
#74016=CARTESIAN_POINT('Ctrl Pts',(-22.3267625753671,-40.3027147367803,
20.));
#74017=CARTESIAN_POINT('Ctrl Pts',(-22.3538609125294,-40.2843148109267,
0.));
#74018=CARTESIAN_POINT('Ctrl Pts',(-22.3538609125294,-40.2843148109267,
20.));
#74019=CARTESIAN_POINT('Ctrl Pts',(-22.3809452914735,-40.2658963302133,
0.));
#74020=CARTESIAN_POINT('Ctrl Pts',(-22.3809452914735,-40.2658963302133,
20.));
#74021=CARTESIAN_POINT('Ctrl Pts',(-22.4080156993888,-40.2474593044019,
0.));
#74022=CARTESIAN_POINT('Ctrl Pts',(-22.4080156993888,-40.2474593044019,
20.));
#74023=CARTESIAN_POINT('Ctrl Pts',(-22.4350721234534,-40.229003743277,0.));
#74024=CARTESIAN_POINT('Ctrl Pts',(-22.4350721234534,-40.229003743277,20.));
#74025=CARTESIAN_POINT('Ctrl Pts',(-22.4621145507305,-40.2105296567239,
0.));
#74026=CARTESIAN_POINT('Ctrl Pts',(-22.4621145507305,-40.2105296567239,
20.));
#74027=CARTESIAN_POINT('Ctrl Pts',(-22.4891429680799,-40.1920370547964,
0.));
#74028=CARTESIAN_POINT('Ctrl Pts',(-22.4891429680799,-40.1920370547964,
20.));
#74029=CARTESIAN_POINT('Ctrl Pts',(-22.5161573620162,-40.1735259478254,
0.));
#74030=CARTESIAN_POINT('Ctrl Pts',(-22.5161573620162,-40.1735259478254,
20.));
#74031=CARTESIAN_POINT('Ctrl Pts',(-22.5431577188606,-40.1549963463026,
0.));
#74032=CARTESIAN_POINT('Ctrl Pts',(-22.5431577188606,-40.1549963463026,
20.));
#74033=CARTESIAN_POINT('Ctrl Pts',(-22.5701440249982,-40.1364482606861,
0.));
#74034=CARTESIAN_POINT('Ctrl Pts',(-22.5701440249982,-40.1364482606861,
20.));
#74035=CARTESIAN_POINT('Ctrl Pts',(-22.5971162671187,-40.1178817012184,
0.));
#74036=CARTESIAN_POINT('Ctrl Pts',(-22.5971162671187,-40.1178817012184,
20.));
#74037=CARTESIAN_POINT('Ctrl Pts',(-22.6240744324259,-40.0992966777668,
0.));
#74038=CARTESIAN_POINT('Ctrl Pts',(-22.6240744324259,-40.0992966777668,
20.));
#74039=CARTESIAN_POINT('Ctrl Pts',(-22.6510185089549,-40.0806931995834,
0.));
#74040=CARTESIAN_POINT('Ctrl Pts',(-22.6510185089549,-40.0806931995834,
20.));
#74041=CARTESIAN_POINT('Ctrl Pts',(-22.6779484851672,-40.0620712756149,
0.));
#74042=CARTESIAN_POINT('Ctrl Pts',(-22.6779484851672,-40.0620712756149,
20.));
#74043=CARTESIAN_POINT('Ctrl Pts',(-22.7048643493645,-40.0434309149416,
0.));
#74044=CARTESIAN_POINT('Ctrl Pts',(-22.7048643493645,-40.0434309149416,
20.));
#74045=CARTESIAN_POINT('Ctrl Pts',(-22.73176608914,-40.0247721271957,0.));
#74046=CARTESIAN_POINT('Ctrl Pts',(-22.73176608914,-40.0247721271957,20.));
#74047=CARTESIAN_POINT('Ctrl Pts',(-22.7586536908732,-40.0060949229408,
0.));
#74048=CARTESIAN_POINT('Ctrl Pts',(-22.7586536908732,-40.0060949229408,
20.));
#74049=CARTESIAN_POINT('Ctrl Pts',(-22.7855271390494,-39.987399314188,0.));
#74050=CARTESIAN_POINT('Ctrl Pts',(-22.7855271390494,-39.987399314188,20.));
#74051=CARTESIAN_POINT('Ctrl Pts',(-22.8123864172494,-39.9686853136472,
0.));
#74052=CARTESIAN_POINT('Ctrl Pts',(-22.8123864172494,-39.9686853136472,
20.));
#74053=CARTESIAN_POINT('Ctrl Pts',(-22.839231509399,-39.9499529337848,0.));
#74054=CARTESIAN_POINT('Ctrl Pts',(-22.839231509399,-39.9499529337848,20.));
#74055=CARTESIAN_POINT('Ctrl Pts',(-22.8660624009432,-39.9312021859374,
0.));
#74056=CARTESIAN_POINT('Ctrl Pts',(-22.8660624009432,-39.9312021859374,
20.));
#74057=CARTESIAN_POINT('Ctrl Pts',(-22.8928790800155,-39.91243307943,0.));
#74058=CARTESIAN_POINT('Ctrl Pts',(-22.8928790800155,-39.91243307943,20.));
#74059=CARTESIAN_POINT('Ctrl Pts',(-22.9196815387084,-39.8936456206159,
0.));
#74060=CARTESIAN_POINT('Ctrl Pts',(-22.9196815387084,-39.8936456206159,
20.));
#74061=CARTESIAN_POINT('Ctrl Pts',(-22.9464697723601,-39.8748398133807,
0.));
#74062=CARTESIAN_POINT('Ctrl Pts',(-22.9464697723601,-39.8748398133807,
20.));
#74063=CARTESIAN_POINT('Ctrl Pts',(-22.9678889774251,-39.8597804904793,
0.));
#74064=CARTESIAN_POINT('Ctrl Pts',(-22.9678889774251,-39.8597804904793,
20.));
#74065=CARTESIAN_POINT('Ctrl Pts',(-22.9839469786126,-39.8484777427633,
0.));
#74066=CARTESIAN_POINT('Ctrl Pts',(-22.9839469786126,-39.8484777427633,
20.));
#74067=CARTESIAN_POINT('Ctrl Pts',(-22.9946494671375,-39.8409389084975,
0.));
#74068=CARTESIAN_POINT('Ctrl Pts',(-22.9946494671375,-39.8409389084975,
20.));
#74069=CARTESIAN_POINT('Ctrl Pts',(-23.,-39.8371685740842,0.));
#74070=CARTESIAN_POINT('Ctrl Pts',(-23.,-39.8371685740842,20.));
#74071=CARTESIAN_POINT('',(8.50876070567956,-48.2555798975982,2.));
#74072=CARTESIAN_POINT('Ctrl Pts',(-10.7008281308626,-46.0172966012412,
2.));
#74073=CARTESIAN_POINT('Ctrl Pts',(-9.9378504380159,-46.269064380565,2.));
#74074=CARTESIAN_POINT('Ctrl Pts',(-9.16754352004547,-46.5017519909094,
2.));
#74075=CARTESIAN_POINT('Ctrl Pts',(-8.39088307367083,-46.7150066081184,
2.));
#74076=CARTESIAN_POINT('Ctrl Pts',(-7.61536245946424,-46.9279482513967,
2.));
#74077=CARTESIAN_POINT('Ctrl Pts',(-6.83350712972477,-47.1215138755074,
2.));
#74078=CARTESIAN_POINT('Ctrl Pts',(-6.04630320233569,-47.295402450297,2.));
#74079=CARTESIAN_POINT('Ctrl Pts',(-5.25842029857172,-47.4694410068512,
2.));
#74080=CARTESIAN_POINT('Ctrl Pts',(-4.46517973963092,-47.6237685212337,
2.));
#74081=CARTESIAN_POINT('Ctrl Pts',(-3.66758232279066,-47.7581340190259,
2.));
#74082=CARTESIAN_POINT('Ctrl Pts',(-2.86929259445598,-47.8926161455541,
2.));
#74083=CARTESIAN_POINT('Ctrl Pts',(-2.06663861563481,-48.0071015607066,
2.));
#74084=CARTESIAN_POINT('Ctrl Pts',(-1.26063332675557,-48.1013899915641,
2.));
#74085=CARTESIAN_POINT('Ctrl Pts',(-0.453491517294757,-48.1958113753237,
2.));
#74086=CARTESIAN_POINT('Ctrl Pts',(0.35701088540252,-48.2699787547905,2.));
#74087=CARTESIAN_POINT('Ctrl Pts',(1.16984971133678,-48.3237428505666,2.));
#74088=CARTESIAN_POINT('Ctrl Pts',(1.98327626216417,-48.3775458205899,2.));
#74089=CARTESIAN_POINT('Ctrl Pts',(2.79904244044949,-48.4109159841017,2.));
#74090=CARTESIAN_POINT('Ctrl Pts',(3.61611754174313,-48.4237558233583,2.));
#74091=CARTESIAN_POINT('Ctrl Pts',(4.43032091679204,-48.4365505351801,2.));
#74092=CARTESIAN_POINT('Ctrl Pts',(5.24582385624142,-48.4289590209732,2.));
#74093=CARTESIAN_POINT('Ctrl Pts',(6.06160482699488,-48.4009361972841,2.));
#74094=CARTESIAN_POINT('Ctrl Pts',(6.59891438315241,-48.3824791217963,2.));
#74095=CARTESIAN_POINT('Ctrl Pts',(7.13634453433625,-48.3551597412747,2.));
#74096=CARTESIAN_POINT('Ctrl Pts',(7.67360352355697,-48.3189772976484,2.));
#74097=CARTESIAN_POINT('Ctrl Pts',(7.95204873082741,-48.3002250232013,2.));
#74098=CARTESIAN_POINT('Ctrl Pts',(8.23044739031116,-48.2790922644854,2.));
#74099=CARTESIAN_POINT('Ctrl Pts',(8.50876070567956,-48.2555798975982,2.));
#74100=CARTESIAN_POINT('',(8.50876070567956,-48.2555798975982,0.));
#74101=CARTESIAN_POINT('Ctrl Pts',(8.50876070567956,-48.2555798975982,0.));
#74102=CARTESIAN_POINT('Ctrl Pts',(8.50876070567956,-48.2555798975982,20.));
#74103=CARTESIAN_POINT('Ctrl Pts',(8.5020159114628,-48.2561497089132,0.));
#74104=CARTESIAN_POINT('Ctrl Pts',(8.5020159114628,-48.2561497089132,20.));
#74105=CARTESIAN_POINT('Ctrl Pts',(8.48852624368607,-48.2572870022174,0.));
#74106=CARTESIAN_POINT('Ctrl Pts',(8.48852624368607,-48.2572870022174,20.));
#74107=CARTESIAN_POINT('Ctrl Pts',(8.46829150399132,-48.2589859541967,0.));
#74108=CARTESIAN_POINT('Ctrl Pts',(8.46829150399132,-48.2589859541967,20.));
#74109=CARTESIAN_POINT('Ctrl Pts',(8.4413113750042,-48.2612372475269,0.));
#74110=CARTESIAN_POINT('Ctrl Pts',(8.4413113750042,-48.2612372475269,20.));
#74111=CARTESIAN_POINT('Ctrl Pts',(8.40758542125999,-48.2640280707484,0.));
#74112=CARTESIAN_POINT('Ctrl Pts',(8.40758542125999,-48.2640280707484,20.));
#74113=CARTESIAN_POINT('Ctrl Pts',(8.37385867778169,-48.2667956002972,0.));
#74114=CARTESIAN_POINT('Ctrl Pts',(8.37385867778169,-48.2667956002972,20.));
#74115=CARTESIAN_POINT('Ctrl Pts',(8.34013115014496,-48.2695398358687,0.));
#74116=CARTESIAN_POINT('Ctrl Pts',(8.34013115014496,-48.2695398358687,20.));
#74117=CARTESIAN_POINT('Ctrl Pts',(8.30640284761835,-48.2722607770974,0.));
#74118=CARTESIAN_POINT('Ctrl Pts',(8.30640284761835,-48.2722607770974,20.));
#74119=CARTESIAN_POINT('Ctrl Pts',(8.27267378419868,-48.274958423567,0.));
#74120=CARTESIAN_POINT('Ctrl Pts',(8.27267378419868,-48.274958423567,20.));
#74121=CARTESIAN_POINT('Ctrl Pts',(8.23894397736021,-48.2776327748283,0.));
#74122=CARTESIAN_POINT('Ctrl Pts',(8.23894397736021,-48.2776327748283,20.));
#74123=CARTESIAN_POINT('Ctrl Pts',(8.20521344665193,-48.2802838304168,0.));
#74124=CARTESIAN_POINT('Ctrl Pts',(8.20521344665193,-48.2802838304168,20.));
#74125=CARTESIAN_POINT('Ctrl Pts',(8.17148221231953,-48.2829115898716,0.));
#74126=CARTESIAN_POINT('Ctrl Pts',(8.17148221231953,-48.2829115898716,20.));
#74127=CARTESIAN_POINT('Ctrl Pts',(8.13775029398593,-48.2855160527521,0.));
#74128=CARTESIAN_POINT('Ctrl Pts',(8.13775029398593,-48.2855160527521,20.));
#74129=CARTESIAN_POINT('Ctrl Pts',(8.10401770912491,-48.288097218659,0.));
#74130=CARTESIAN_POINT('Ctrl Pts',(8.10401770912491,-48.288097218659,20.));
#74131=CARTESIAN_POINT('Ctrl Pts',(8.07028447346157,-48.2906550872281,0.));
#74132=CARTESIAN_POINT('Ctrl Pts',(8.07028447346157,-48.2906550872281,20.));
#74133=CARTESIAN_POINT('Ctrl Pts',(8.03655060167523,-48.2931896581208,0.));
#74134=CARTESIAN_POINT('Ctrl Pts',(8.03655060167523,-48.2931896581208,20.));
#74135=CARTESIAN_POINT('Ctrl Pts',(8.00281610801472,-48.2957009310153,0.));
#74136=CARTESIAN_POINT('Ctrl Pts',(8.00281610801472,-48.2957009310153,20.));
#74137=CARTESIAN_POINT('Ctrl Pts',(7.96908100690892,-48.2981889055984,0.));
#74138=CARTESIAN_POINT('Ctrl Pts',(7.96908100690892,-48.2981889055984,20.));
#74139=CARTESIAN_POINT('Ctrl Pts',(7.93534531368689,-48.300653581555,0.));
#74140=CARTESIAN_POINT('Ctrl Pts',(7.93534531368689,-48.300653581555,20.));
#74141=CARTESIAN_POINT('Ctrl Pts',(7.90160904447351,-48.3030949585702,0.));
#74142=CARTESIAN_POINT('Ctrl Pts',(7.90160904447351,-48.3030949585702,20.));
#74143=CARTESIAN_POINT('Ctrl Pts',(7.86787221586445,-48.3055130363337,0.));
#74144=CARTESIAN_POINT('Ctrl Pts',(7.86787221586445,-48.3055130363337,20.));
#74145=CARTESIAN_POINT('Ctrl Pts',(7.83413484466693,-48.3079078145432,0.));
#74146=CARTESIAN_POINT('Ctrl Pts',(7.83413484466693,-48.3079078145432,20.));
#74147=CARTESIAN_POINT('Ctrl Pts',(7.80039694763397,-48.3102792929086,0.));
#74148=CARTESIAN_POINT('Ctrl Pts',(7.80039694763397,-48.3102792929086,20.));
#74149=CARTESIAN_POINT('Ctrl Pts',(7.76665854114745,-48.3126274711557,0.));
#74150=CARTESIAN_POINT('Ctrl Pts',(7.76665854114745,-48.3126274711557,20.));
#74151=CARTESIAN_POINT('Ctrl Pts',(7.73291964123288,-48.3149523490266,0.));
#74152=CARTESIAN_POINT('Ctrl Pts',(7.73291964123288,-48.3149523490266,20.));
#74153=CARTESIAN_POINT('Ctrl Pts',(7.69918026370735,-48.3172539262766,0.));
#74154=CARTESIAN_POINT('Ctrl Pts',(7.69918026370735,-48.3172539262766,20.));
#74155=CARTESIAN_POINT('Ctrl Pts',(7.66544042428832,-48.3195322026739,0.));
#74156=CARTESIAN_POINT('Ctrl Pts',(7.66544042428832,-48.3195322026739,20.));
#74157=CARTESIAN_POINT('Ctrl Pts',(7.63170013870892,-48.3217871779975,0.));
#74158=CARTESIAN_POINT('Ctrl Pts',(7.63170013870892,-48.3217871779975,20.));
#74159=CARTESIAN_POINT('Ctrl Pts',(7.59795942285539,-48.3240188520354,0.));
#74160=CARTESIAN_POINT('Ctrl Pts',(7.59795942285539,-48.3240188520354,20.));
#74161=CARTESIAN_POINT('Ctrl Pts',(7.56421829277369,-48.3262272245847,0.));
#74162=CARTESIAN_POINT('Ctrl Pts',(7.56421829277369,-48.3262272245847,20.));
#74163=CARTESIAN_POINT('Ctrl Pts',(7.53047676460326,-48.328412295452,0.));
#74164=CARTESIAN_POINT('Ctrl Pts',(7.53047676460326,-48.328412295452,20.));
#74165=CARTESIAN_POINT('Ctrl Pts',(7.49673485453118,-48.3305740644544,0.));
#74166=CARTESIAN_POINT('Ctrl Pts',(7.49673485453118,-48.3305740644544,20.));
#74167=CARTESIAN_POINT('Ctrl Pts',(7.46299257874208,-48.3327125314199,0.));
#74168=CARTESIAN_POINT('Ctrl Pts',(7.46299257874208,-48.3327125314199,20.));
#74169=CARTESIAN_POINT('Ctrl Pts',(7.42924995335917,-48.3348276961881,0.));
#74170=CARTESIAN_POINT('Ctrl Pts',(7.42924995335917,-48.3348276961881,20.));
#74171=CARTESIAN_POINT('Ctrl Pts',(7.39550699443533,-48.3369195586108,0.));
#74172=CARTESIAN_POINT('Ctrl Pts',(7.39550699443533,-48.3369195586108,20.));
#74173=CARTESIAN_POINT('Ctrl Pts',(7.36176371798261,-48.3389881185516,0.));
#74174=CARTESIAN_POINT('Ctrl Pts',(7.36176371798261,-48.3389881185516,20.));
#74175=CARTESIAN_POINT('Ctrl Pts',(7.32802013999146,-48.3410333758855,0.));
#74176=CARTESIAN_POINT('Ctrl Pts',(7.32802013999146,-48.3410333758855,20.));
#74177=CARTESIAN_POINT('Ctrl Pts',(7.29427627645269,-48.3430553304987,0.));
#74178=CARTESIAN_POINT('Ctrl Pts',(7.29427627645269,-48.3430553304987,20.));
#74179=CARTESIAN_POINT('Ctrl Pts',(7.26053214338256,-48.3450539822883,0.));
#74180=CARTESIAN_POINT('Ctrl Pts',(7.26053214338256,-48.3450539822883,20.));
#74181=CARTESIAN_POINT('Ctrl Pts',(7.22678775682931,-48.3470293311619,0.));
#74182=CARTESIAN_POINT('Ctrl Pts',(7.22678775682931,-48.3470293311619,20.));
#74183=CARTESIAN_POINT('Ctrl Pts',(7.19304313285997,-48.3489813770376,0.));
#74184=CARTESIAN_POINT('Ctrl Pts',(7.19304313285997,-48.3489813770376,20.));
#74185=CARTESIAN_POINT('Ctrl Pts',(7.15929828755239,-48.3509101198447,0.));
#74186=CARTESIAN_POINT('Ctrl Pts',(7.15929828755239,-48.3509101198447,20.));
#74187=CARTESIAN_POINT('Ctrl Pts',(7.12555323698548,-48.3528155595232,0.));
#74188=CARTESIAN_POINT('Ctrl Pts',(7.12555323698548,-48.3528155595232,20.));
#74189=CARTESIAN_POINT('Ctrl Pts',(7.0918079972288,-48.354697696024,0.));
#74190=CARTESIAN_POINT('Ctrl Pts',(7.0918079972288,-48.354697696024,20.));
#74191=CARTESIAN_POINT('Ctrl Pts',(7.05806258433801,-48.3565565293095,0.));
#74192=CARTESIAN_POINT('Ctrl Pts',(7.05806258433801,-48.3565565293095,20.));
#74193=CARTESIAN_POINT('Ctrl Pts',(7.02431701436125,-48.3583920593534,0.));
#74194=CARTESIAN_POINT('Ctrl Pts',(7.02431701436125,-48.3583920593534,20.));
#74195=CARTESIAN_POINT('Ctrl Pts',(6.99057130334226,-48.3602042861407,0.));
#74196=CARTESIAN_POINT('Ctrl Pts',(6.99057130334226,-48.3602042861407,20.));
#74197=CARTESIAN_POINT('Ctrl Pts',(6.95682546732483,-48.3619932096677,0.));
#74198=CARTESIAN_POINT('Ctrl Pts',(6.95682546732483,-48.3619932096677,20.));
#74199=CARTESIAN_POINT('Ctrl Pts',(6.92307952235708,-48.3637588299416,0.));
#74200=CARTESIAN_POINT('Ctrl Pts',(6.92307952235708,-48.3637588299416,20.));
#74201=CARTESIAN_POINT('Ctrl Pts',(6.8893334844937,-48.3655011469807,0.));
#74202=CARTESIAN_POINT('Ctrl Pts',(6.8893334844937,-48.3655011469807,20.));
#74203=CARTESIAN_POINT('Ctrl Pts',(6.85558736979328,-48.3672201608141,0.));
#74204=CARTESIAN_POINT('Ctrl Pts',(6.85558736979328,-48.3672201608141,20.));
#74205=CARTESIAN_POINT('Ctrl Pts',(6.82184119431717,-48.3689158714816,0.));
#74206=CARTESIAN_POINT('Ctrl Pts',(6.82184119431717,-48.3689158714816,20.));
#74207=CARTESIAN_POINT('Ctrl Pts',(6.78809497412713,-48.370588279034,0.));
#74208=CARTESIAN_POINT('Ctrl Pts',(6.78809497412713,-48.370588279034,20.));
#74209=CARTESIAN_POINT('Ctrl Pts',(6.75434872528384,-48.3722373835335,0.));
#74210=CARTESIAN_POINT('Ctrl Pts',(6.75434872528384,-48.3722373835335,20.));
#74211=CARTESIAN_POINT('Ctrl Pts',(6.72060246384579,-48.3738631850533,0.));
#74212=CARTESIAN_POINT('Ctrl Pts',(6.72060246384579,-48.3738631850533,20.));
#74213=CARTESIAN_POINT('Ctrl Pts',(6.68685620587014,-48.3754656836776,0.));
#74214=CARTESIAN_POINT('Ctrl Pts',(6.68685620587014,-48.3754656836776,20.));
#74215=CARTESIAN_POINT('Ctrl Pts',(6.65310996741333,-48.3770448795022,0.));
#74216=CARTESIAN_POINT('Ctrl Pts',(6.65310996741333,-48.3770448795022,20.));
#74217=CARTESIAN_POINT('Ctrl Pts',(6.61936376453194,-48.3786007726338,0.));
#74218=CARTESIAN_POINT('Ctrl Pts',(6.61936376453194,-48.3786007726338,20.));
#74219=CARTESIAN_POINT('Ctrl Pts',(6.58561761328367,-48.3801333631899,0.));
#74220=CARTESIAN_POINT('Ctrl Pts',(6.58561761328367,-48.3801333631899,20.));
#74221=CARTESIAN_POINT('Ctrl Pts',(6.55187152972771,-48.3816426512995,0.));
#74222=CARTESIAN_POINT('Ctrl Pts',(6.55187152972771,-48.3816426512995,20.));
#74223=CARTESIAN_POINT('Ctrl Pts',(6.51812552992423,-48.3831286371024,0.));
#74224=CARTESIAN_POINT('Ctrl Pts',(6.51812552992423,-48.3831286371024,20.));
#74225=CARTESIAN_POINT('Ctrl Pts',(6.48437962993405,-48.3845913207494,0.));
#74226=CARTESIAN_POINT('Ctrl Pts',(6.48437962993405,-48.3845913207494,20.));
#74227=CARTESIAN_POINT('Ctrl Pts',(6.45063384581844,-48.3860307024022,0.));
#74228=CARTESIAN_POINT('Ctrl Pts',(6.45063384581844,-48.3860307024022,20.));
#74229=CARTESIAN_POINT('Ctrl Pts',(6.41688819363864,-48.3874467822337,0.));
#74230=CARTESIAN_POINT('Ctrl Pts',(6.41688819363864,-48.3874467822337,20.));
#74231=CARTESIAN_POINT('Ctrl Pts',(6.38314268945587,-48.388839560428,0.));
#74232=CARTESIAN_POINT('Ctrl Pts',(6.38314268945587,-48.388839560428,20.));
#74233=CARTESIAN_POINT('Ctrl Pts',(6.34939734933121,-48.3902090371802,0.));
#74234=CARTESIAN_POINT('Ctrl Pts',(6.34939734933121,-48.3902090371802,20.));
#74235=CARTESIAN_POINT('Ctrl Pts',(6.31565218932588,-48.3915552126968,0.));
#74236=CARTESIAN_POINT('Ctrl Pts',(6.31565218932588,-48.3915552126968,20.));
#74237=CARTESIAN_POINT('Ctrl Pts',(6.28190722550132,-48.3928780871951,0.));
#74238=CARTESIAN_POINT('Ctrl Pts',(6.28190722550132,-48.3928780871951,20.));
#74239=CARTESIAN_POINT('Ctrl Pts',(6.24816247391919,-48.3941776609035,0.));
#74240=CARTESIAN_POINT('Ctrl Pts',(6.24816247391919,-48.3941776609035,20.));
#74241=CARTESIAN_POINT('Ctrl Pts',(6.21441795064167,-48.3954539340615,0.));
#74242=CARTESIAN_POINT('Ctrl Pts',(6.21441795064167,-48.3954539340615,20.));
#74243=CARTESIAN_POINT('Ctrl Pts',(6.18067367173123,-48.3967069069196,0.));
#74244=CARTESIAN_POINT('Ctrl Pts',(6.18067367173123,-48.3967069069196,20.));
#74245=CARTESIAN_POINT('Ctrl Pts',(6.14692965325078,-48.3979365797396,0.));
#74246=CARTESIAN_POINT('Ctrl Pts',(6.14692965325078,-48.3979365797396,20.));
#74247=CARTESIAN_POINT('Ctrl Pts',(6.11318591126342,-48.3991429527941,0.));
#74248=CARTESIAN_POINT('Ctrl Pts',(6.11318591126342,-48.3991429527941,20.));
#74249=CARTESIAN_POINT('Ctrl Pts',(6.07944246183266,-48.400326026367,0.));
#74250=CARTESIAN_POINT('Ctrl Pts',(6.07944246183266,-48.400326026367,20.));
#74251=CARTESIAN_POINT('Ctrl Pts',(6.04569932102199,-48.4014858007534,0.));
#74252=CARTESIAN_POINT('Ctrl Pts',(6.04569932102199,-48.4014858007534,20.));
#74253=CARTESIAN_POINT('Ctrl Pts',(6.01195650489504,-48.4026222762592,0.));
#74254=CARTESIAN_POINT('Ctrl Pts',(6.01195650489504,-48.4026222762592,20.));
#74255=CARTESIAN_POINT('Ctrl Pts',(5.97821402951547,-48.4037354532014,0.));
#74256=CARTESIAN_POINT('Ctrl Pts',(5.97821402951547,-48.4037354532014,20.));
#74257=CARTESIAN_POINT('Ctrl Pts',(5.94447191094721,-48.404825331908,0.));
#74258=CARTESIAN_POINT('Ctrl Pts',(5.94447191094721,-48.404825331908,20.));
#74259=CARTESIAN_POINT('Ctrl Pts',(5.91073016525425,-48.4058919127185,0.));
#74260=CARTESIAN_POINT('Ctrl Pts',(5.91073016525425,-48.4058919127185,20.));
#74261=CARTESIAN_POINT('Ctrl Pts',(5.87698880850095,-48.4069351959835,0.));
#74262=CARTESIAN_POINT('Ctrl Pts',(5.87698880850095,-48.4069351959835,20.));
#74263=CARTESIAN_POINT('Ctrl Pts',(5.84324785675189,-48.4079551820643,0.));
#74264=CARTESIAN_POINT('Ctrl Pts',(5.84324785675189,-48.4079551820643,20.));
#74265=CARTESIAN_POINT('Ctrl Pts',(5.80950732607177,-48.4089518713337,0.));
#74266=CARTESIAN_POINT('Ctrl Pts',(5.80950732607177,-48.4089518713337,20.));
#74267=CARTESIAN_POINT('Ctrl Pts',(5.77576723252552,-48.4099252641753,0.));
#74268=CARTESIAN_POINT('Ctrl Pts',(5.77576723252552,-48.4099252641753,20.));
#74269=CARTESIAN_POINT('Ctrl Pts',(5.74202759217812,-48.4108753609837,0.));
#74270=CARTESIAN_POINT('Ctrl Pts',(5.74202759217812,-48.4108753609837,20.));
#74271=CARTESIAN_POINT('Ctrl Pts',(5.70828842109459,-48.4118021621647,0.));
#74272=CARTESIAN_POINT('Ctrl Pts',(5.70828842109459,-48.4118021621647,20.));
#74273=CARTESIAN_POINT('Ctrl Pts',(5.67454973534013,-48.412705668135,0.));
#74274=CARTESIAN_POINT('Ctrl Pts',(5.67454973534013,-48.412705668135,20.));
#74275=CARTESIAN_POINT('Ctrl Pts',(5.64081155098004,-48.4135858793227,0.));
#74276=CARTESIAN_POINT('Ctrl Pts',(5.64081155098004,-48.4135858793227,20.));
#74277=CARTESIAN_POINT('Ctrl Pts',(5.6070738840798,-48.414442796167,0.));
#74278=CARTESIAN_POINT('Ctrl Pts',(5.6070738840798,-48.414442796167,20.));
#74279=CARTESIAN_POINT('Ctrl Pts',(5.57333675070491,-48.4152764191183,0.));
#74280=CARTESIAN_POINT('Ctrl Pts',(5.57333675070491,-48.4152764191183,20.));
#74281=CARTESIAN_POINT('Ctrl Pts',(5.53960016692117,-48.4160867486381,0.));
#74282=CARTESIAN_POINT('Ctrl Pts',(5.53960016692117,-48.4160867486381,20.));
#74283=CARTESIAN_POINT('Ctrl Pts',(5.50586414879429,-48.4168737851989,0.));
#74284=CARTESIAN_POINT('Ctrl Pts',(5.50586414879429,-48.4168737851989,20.));
#74285=CARTESIAN_POINT('Ctrl Pts',(5.47212871239029,-48.417637529284,0.));
#74286=CARTESIAN_POINT('Ctrl Pts',(5.47212871239029,-48.417637529284,20.));
#74287=CARTESIAN_POINT('Ctrl Pts',(5.43839387377497,-48.4183779813881,0.));
#74288=CARTESIAN_POINT('Ctrl Pts',(5.43839387377497,-48.4183779813881,20.));
#74289=CARTESIAN_POINT('Ctrl Pts',(5.40465964901424,-48.4190951420167,0.));
#74290=CARTESIAN_POINT('Ctrl Pts',(5.40465964901424,-48.4190951420167,20.));
#74291=CARTESIAN_POINT('Ctrl Pts',(5.37092605417401,-48.4197890116867,0.));
#74292=CARTESIAN_POINT('Ctrl Pts',(5.37092605417401,-48.4197890116867,20.));
#74293=CARTESIAN_POINT('Ctrl Pts',(5.33719310532026,-48.4204595909261,0.));
#74294=CARTESIAN_POINT('Ctrl Pts',(5.33719310532026,-48.4204595909261,20.));
#74295=CARTESIAN_POINT('Ctrl Pts',(5.30346081851908,-48.4211068802741,0.));
#74296=CARTESIAN_POINT('Ctrl Pts',(5.30346081851908,-48.4211068802741,20.));
#74297=CARTESIAN_POINT('Ctrl Pts',(5.26972920983669,-48.4217308802807,0.));
#74298=CARTESIAN_POINT('Ctrl Pts',(5.26972920983669,-48.4217308802807,20.));
#74299=CARTESIAN_POINT('Ctrl Pts',(5.23599829533944,-48.4223315915069,0.));
#74300=CARTESIAN_POINT('Ctrl Pts',(5.23599829533944,-48.4223315915069,20.));
#74301=CARTESIAN_POINT('Ctrl Pts',(5.2022680910935,-48.4229090145253,0.));
#74302=CARTESIAN_POINT('Ctrl Pts',(5.2022680910935,-48.4229090145253,20.));
#74303=CARTESIAN_POINT('Ctrl Pts',(5.1685386131652,-48.4234631499194,0.));
#74304=CARTESIAN_POINT('Ctrl Pts',(5.1685386131652,-48.4234631499194,20.));
#74305=CARTESIAN_POINT('Ctrl Pts',(5.1348098776207,-48.4239939982838,0.));
#74306=CARTESIAN_POINT('Ctrl Pts',(5.1348098776207,-48.4239939982838,20.));
#74307=CARTESIAN_POINT('Ctrl Pts',(5.10108190052607,-48.4245015602246,0.));
#74308=CARTESIAN_POINT('Ctrl Pts',(5.10108190052607,-48.4245015602246,20.));
#74309=CARTESIAN_POINT('Ctrl Pts',(5.06735469794741,-48.4249858363582,0.));
#74310=CARTESIAN_POINT('Ctrl Pts',(5.06735469794741,-48.4249858363582,20.));
#74311=CARTESIAN_POINT('Ctrl Pts',(5.03362828595092,-48.4254468273122,0.));
#74312=CARTESIAN_POINT('Ctrl Pts',(5.03362828595092,-48.4254468273122,20.));
#74313=CARTESIAN_POINT('Ctrl Pts',(4.99990268060291,-48.4258845337255,0.));
#74314=CARTESIAN_POINT('Ctrl Pts',(4.99990268060291,-48.4258845337255,20.));
#74315=CARTESIAN_POINT('Ctrl Pts',(4.96617789796952,-48.4262989562483,0.));
#74316=CARTESIAN_POINT('Ctrl Pts',(4.96617789796952,-48.4262989562483,20.));
#74317=CARTESIAN_POINT('Ctrl Pts',(4.93245395411684,-48.4266900955418,0.));
#74318=CARTESIAN_POINT('Ctrl Pts',(4.93245395411684,-48.4266900955418,20.));
#74319=CARTESIAN_POINT('Ctrl Pts',(4.89873086511076,-48.4270579522784,0.));
#74320=CARTESIAN_POINT('Ctrl Pts',(4.89873086511076,-48.4270579522784,20.));
#74321=CARTESIAN_POINT('Ctrl Pts',(4.8650086470173,-48.4274025271416,0.));
#74322=CARTESIAN_POINT('Ctrl Pts',(4.8650086470173,-48.4274025271416,20.));
#74323=CARTESIAN_POINT('Ctrl Pts',(4.83128731590228,-48.4277238208263,0.));
#74324=CARTESIAN_POINT('Ctrl Pts',(4.83128731590228,-48.4277238208263,20.));
#74325=CARTESIAN_POINT('Ctrl Pts',(4.79756688783168,-48.4280218340382,0.));
#74326=CARTESIAN_POINT('Ctrl Pts',(4.79756688783168,-48.4280218340382,20.));
#74327=CARTESIAN_POINT('Ctrl Pts',(4.76384737887105,-48.4282965674942,0.));
#74328=CARTESIAN_POINT('Ctrl Pts',(4.76384737887105,-48.4282965674942,20.));
#74329=CARTESIAN_POINT('Ctrl Pts',(4.730128805086,-48.4285480219221,0.));
#74330=CARTESIAN_POINT('Ctrl Pts',(4.730128805086,-48.4285480219221,20.));
#74331=CARTESIAN_POINT('Ctrl Pts',(4.69641118254225,-48.4287761980604,0.));
#74332=CARTESIAN_POINT('Ctrl Pts',(4.69641118254225,-48.4287761980604,20.));
#74333=CARTESIAN_POINT('Ctrl Pts',(4.66269452730542,-48.4289810966589,0.));
#74334=CARTESIAN_POINT('Ctrl Pts',(4.66269452730542,-48.4289810966589,20.));
#74335=CARTESIAN_POINT('Ctrl Pts',(4.62897885544097,-48.4291627184787,0.));
#74336=CARTESIAN_POINT('Ctrl Pts',(4.62897885544097,-48.4291627184787,20.));
#74337=CARTESIAN_POINT('Ctrl Pts',(4.59526418301408,-48.4293210642923,0.));
#74338=CARTESIAN_POINT('Ctrl Pts',(4.59526418301408,-48.4293210642923,20.));
#74339=CARTESIAN_POINT('Ctrl Pts',(4.5615505260898,-48.4294561348833,0.));
#74340=CARTESIAN_POINT('Ctrl Pts',(4.5615505260898,-48.4294561348833,20.));
#74341=CARTESIAN_POINT('Ctrl Pts',(4.52783790073293,-48.4295679310466,0.));
#74342=CARTESIAN_POINT('Ctrl Pts',(4.52783790073293,-48.4295679310466,20.));
#74343=CARTESIAN_POINT('Ctrl Pts',(4.49412632300814,-48.4296564535884,0.));
#74344=CARTESIAN_POINT('Ctrl Pts',(4.49412632300814,-48.4296564535884,20.));
#74345=CARTESIAN_POINT('Ctrl Pts',(4.46041580898011,-48.4297217033257,0.));
#74346=CARTESIAN_POINT('Ctrl Pts',(4.46041580898011,-48.4297217033257,20.));
#74347=CARTESIAN_POINT('Ctrl Pts',(4.4267063747134,-48.4297636810863,0.));
#74348=CARTESIAN_POINT('Ctrl Pts',(4.4267063747134,-48.4297636810863,20.));
#74349=CARTESIAN_POINT('Ctrl Pts',(4.39299803627246,-48.4297823877088,0.));
#74350=CARTESIAN_POINT('Ctrl Pts',(4.39299803627246,-48.4297823877088,20.));
#74351=CARTESIAN_POINT('Ctrl Pts',(4.35929080972166,-48.4297778240431,0.));
#74352=CARTESIAN_POINT('Ctrl Pts',(4.35929080972166,-48.4297778240431,20.));
#74353=CARTESIAN_POINT('Ctrl Pts',(4.32558471112516,-48.42974999095,0.));
#74354=CARTESIAN_POINT('Ctrl Pts',(4.32558471112516,-48.42974999095,20.));
#74355=CARTESIAN_POINT('Ctrl Pts',(4.29187975654677,-48.4296988893018,0.));
#74356=CARTESIAN_POINT('Ctrl Pts',(4.29187975654677,-48.4296988893018,20.));
#74357=CARTESIAN_POINT('Ctrl Pts',(4.25817596205,-48.4296245199823,0.));
#74358=CARTESIAN_POINT('Ctrl Pts',(4.25817596205,-48.4296245199823,20.));
#74359=CARTESIAN_POINT('Ctrl Pts',(4.22447334369801,-48.4295268838864,0.));
#74360=CARTESIAN_POINT('Ctrl Pts',(4.22447334369801,-48.4295268838864,20.));
#74361=CARTESIAN_POINT('Ctrl Pts',(4.19077191755405,-48.4294059819202,0.));
#74362=CARTESIAN_POINT('Ctrl Pts',(4.19077191755405,-48.4294059819202,20.));
#74363=CARTESIAN_POINT('Ctrl Pts',(4.15707169968115,-48.4292618150011,0.));
#74364=CARTESIAN_POINT('Ctrl Pts',(4.15707169968115,-48.4292618150011,20.));
#74365=CARTESIAN_POINT('Ctrl Pts',(4.1233727061421,-48.429094384057,0.));
#74366=CARTESIAN_POINT('Ctrl Pts',(4.1233727061421,-48.429094384057,20.));
#74367=CARTESIAN_POINT('Ctrl Pts',(4.08967495299951,-48.4289036900268,0.));
#74368=CARTESIAN_POINT('Ctrl Pts',(4.08967495299951,-48.4289036900268,20.));
#74369=CARTESIAN_POINT('Ctrl Pts',(4.05597845631568,-48.4286897338604,0.));
#74370=CARTESIAN_POINT('Ctrl Pts',(4.05597845631568,-48.4286897338604,20.));
#74371=CARTESIAN_POINT('Ctrl Pts',(4.02228323215259,-48.4284525165189,0.));
#74372=CARTESIAN_POINT('Ctrl Pts',(4.02228323215259,-48.4284525165189,20.));
#74373=CARTESIAN_POINT('Ctrl Pts',(3.988589296572,-48.4281920389749,0.));
#74374=CARTESIAN_POINT('Ctrl Pts',(3.988589296572,-48.4281920389749,20.));
#74375=CARTESIAN_POINT('Ctrl Pts',(3.95489666563548,-48.427908302212,0.));
#74376=CARTESIAN_POINT('Ctrl Pts',(3.95489666563548,-48.427908302212,20.));
#74377=CARTESIAN_POINT('Ctrl Pts',(3.9212053554042,-48.4276013072253,0.));
#74378=CARTESIAN_POINT('Ctrl Pts',(3.9212053554042,-48.4276013072253,20.));
#74379=CARTESIAN_POINT('Ctrl Pts',(3.88751538193919,-48.4272710550207,0.));
#74380=CARTESIAN_POINT('Ctrl Pts',(3.88751538193919,-48.4272710550207,20.));
#74381=CARTESIAN_POINT('Ctrl Pts',(3.85382676130114,-48.4269175466151,0.));
#74382=CARTESIAN_POINT('Ctrl Pts',(3.85382676130114,-48.4269175466151,20.));
#74383=CARTESIAN_POINT('Ctrl Pts',(3.82013950955042,-48.4265407830367,0.));
#74384=CARTESIAN_POINT('Ctrl Pts',(3.82013950955042,-48.4265407830367,20.));
#74385=CARTESIAN_POINT('Ctrl Pts',(3.78645364274706,-48.4261407653249,0.));
#74386=CARTESIAN_POINT('Ctrl Pts',(3.78645364274706,-48.4261407653249,20.));
#74387=CARTESIAN_POINT('Ctrl Pts',(3.75276917695084,-48.4257174945298,0.));
#74388=CARTESIAN_POINT('Ctrl Pts',(3.75276917695084,-48.4257174945298,20.));
#74389=CARTESIAN_POINT('Ctrl Pts',(3.71908612822108,-48.4252709717129,0.));
#74390=CARTESIAN_POINT('Ctrl Pts',(3.71908612822108,-48.4252709717129,20.));
#74391=CARTESIAN_POINT('Ctrl Pts',(3.68540451261695,-48.424801197947,0.));
#74392=CARTESIAN_POINT('Ctrl Pts',(3.68540451261695,-48.424801197947,20.));
#74393=CARTESIAN_POINT('Ctrl Pts',(3.6517243461974,-48.4243081743158,0.));
#74394=CARTESIAN_POINT('Ctrl Pts',(3.6517243461974,-48.4243081743158,20.));
#74395=CARTESIAN_POINT('Ctrl Pts',(3.61804564502096,-48.4237919019141,0.));
#74396=CARTESIAN_POINT('Ctrl Pts',(3.61804564502096,-48.4237919019141,20.));
#74397=CARTESIAN_POINT('Ctrl Pts',(3.58436842514564,-48.4232523818483,0.));
#74398=CARTESIAN_POINT('Ctrl Pts',(3.58436842514564,-48.4232523818483,20.));
#74399=CARTESIAN_POINT('Ctrl Pts',(3.55069270262907,-48.4226896152354,0.));
#74400=CARTESIAN_POINT('Ctrl Pts',(3.55069270262907,-48.4226896152354,20.));
#74401=CARTESIAN_POINT('Ctrl Pts',(3.51701849352853,-48.422103603204,0.));
#74402=CARTESIAN_POINT('Ctrl Pts',(3.51701849352853,-48.422103603204,20.));
#74403=CARTESIAN_POINT('Ctrl Pts',(3.483345813901,-48.4214943468927,0.));
#74404=CARTESIAN_POINT('Ctrl Pts',(3.483345813901,-48.4214943468927,20.));
#74405=CARTESIAN_POINT('Ctrl Pts',(3.44967467980323,-48.4208618474523,0.));
#74406=CARTESIAN_POINT('Ctrl Pts',(3.44967467980323,-48.4208618474523,20.));
#74407=CARTESIAN_POINT('Ctrl Pts',(3.41600510729148,-48.4202061060442,0.));
#74408=CARTESIAN_POINT('Ctrl Pts',(3.41600510729148,-48.4202061060442,20.));
#74409=CARTESIAN_POINT('Ctrl Pts',(3.38233711242167,-48.4195271238417,0.));
#74410=CARTESIAN_POINT('Ctrl Pts',(3.38233711242167,-48.4195271238417,20.));
#74411=CARTESIAN_POINT('Ctrl Pts',(3.34867071124917,-48.4188249020284,0.));
#74412=CARTESIAN_POINT('Ctrl Pts',(3.34867071124917,-48.4188249020284,20.));
#74413=CARTESIAN_POINT('Ctrl Pts',(3.31500591982887,-48.4180994417999,0.));
#74414=CARTESIAN_POINT('Ctrl Pts',(3.31500591982887,-48.4180994417999,20.));
#74415=CARTESIAN_POINT('Ctrl Pts',(3.28134275421531,-48.4173507443625,0.));
#74416=CARTESIAN_POINT('Ctrl Pts',(3.28134275421531,-48.4173507443625,20.));
#74417=CARTESIAN_POINT('Ctrl Pts',(3.24768123046264,-48.4165788109335,0.));
#74418=CARTESIAN_POINT('Ctrl Pts',(3.24768123046264,-48.4165788109335,20.));
#74419=CARTESIAN_POINT('Ctrl Pts',(3.21402136462457,-48.4157836427414,0.));
#74420=CARTESIAN_POINT('Ctrl Pts',(3.21402136462457,-48.4157836427414,20.));
#74421=CARTESIAN_POINT('Ctrl Pts',(3.18036317275453,-48.4149652410254,0.));
#74422=CARTESIAN_POINT('Ctrl Pts',(3.18036317275453,-48.4149652410254,20.));
#74423=CARTESIAN_POINT('Ctrl Pts',(3.14670667090555,-48.414123607036,0.));
#74424=CARTESIAN_POINT('Ctrl Pts',(3.14670667090555,-48.414123607036,20.));
#74425=CARTESIAN_POINT('Ctrl Pts',(3.11305187512999,-48.4132587420349,0.));
#74426=CARTESIAN_POINT('Ctrl Pts',(3.11305187512999,-48.4132587420349,20.));
#74427=CARTESIAN_POINT('Ctrl Pts',(3.07939880147968,-48.4123706472953,0.));
#74428=CARTESIAN_POINT('Ctrl Pts',(3.07939880147968,-48.4123706472953,20.));
#74429=CARTESIAN_POINT('Ctrl Pts',(3.04574746600607,-48.4114593241014,0.));
#74430=CARTESIAN_POINT('Ctrl Pts',(3.04574746600607,-48.4114593241014,20.));
#74431=CARTESIAN_POINT('Ctrl Pts',(3.01209788475993,-48.4105247737488,0.));
#74432=CARTESIAN_POINT('Ctrl Pts',(3.01209788475993,-48.4105247737488,20.));
#74433=CARTESIAN_POINT('Ctrl Pts',(2.97845007379181,-48.4095669975441,0.));
#74434=CARTESIAN_POINT('Ctrl Pts',(2.97845007379181,-48.4095669975441,20.));
#74435=CARTESIAN_POINT('Ctrl Pts',(2.94480404915164,-48.4085859968048,0.));
#74436=CARTESIAN_POINT('Ctrl Pts',(2.94480404915164,-48.4085859968048,20.));
#74437=CARTESIAN_POINT('Ctrl Pts',(2.91115982688903,-48.4075817728593,0.));
#74438=CARTESIAN_POINT('Ctrl Pts',(2.91115982688903,-48.4075817728593,20.));
#74439=CARTESIAN_POINT('Ctrl Pts',(2.87751742305292,-48.4065543270471,0.));
#74440=CARTESIAN_POINT('Ctrl Pts',(2.87751742305292,-48.4065543270471,20.));
#74441=CARTESIAN_POINT('Ctrl Pts',(2.8438768536918,-48.4055036607195,0.));
#74442=CARTESIAN_POINT('Ctrl Pts',(2.8438768536918,-48.4055036607195,20.));
#74443=CARTESIAN_POINT('Ctrl Pts',(2.81023813485355,-48.4044297752383,0.));
#74444=CARTESIAN_POINT('Ctrl Pts',(2.81023813485355,-48.4044297752383,20.));
#74445=CARTESIAN_POINT('Ctrl Pts',(2.77660128258546,-48.4033326719771,0.));
#74446=CARTESIAN_POINT('Ctrl Pts',(2.77660128258546,-48.4033326719771,20.));
#74447=CARTESIAN_POINT('Ctrl Pts',(2.74296631293436,-48.4022123523201,0.));
#74448=CARTESIAN_POINT('Ctrl Pts',(2.74296631293436,-48.4022123523201,20.));
#74449=CARTESIAN_POINT('Ctrl Pts',(2.7093332419466,-48.4010688176627,0.));
#74450=CARTESIAN_POINT('Ctrl Pts',(2.7093332419466,-48.4010688176627,20.));
#74451=CARTESIAN_POINT('Ctrl Pts',(2.67570208566793,-48.3999020694116,0.));
#74452=CARTESIAN_POINT('Ctrl Pts',(2.67570208566793,-48.3999020694116,20.));
#74453=CARTESIAN_POINT('Ctrl Pts',(2.64207286014349,-48.3987121089844,0.));
#74454=CARTESIAN_POINT('Ctrl Pts',(2.64207286014349,-48.3987121089844,20.));
#74455=CARTESIAN_POINT('Ctrl Pts',(2.60844558141789,-48.3974989378103,0.));
#74456=CARTESIAN_POINT('Ctrl Pts',(2.60844558141789,-48.3974989378103,20.));
#74457=CARTESIAN_POINT('Ctrl Pts',(2.57482026553515,-48.3962625573292,0.));
#74458=CARTESIAN_POINT('Ctrl Pts',(2.57482026553515,-48.3962625573292,20.));
#74459=CARTESIAN_POINT('Ctrl Pts',(2.5411969285386,-48.3950029689925,0.));
#74460=CARTESIAN_POINT('Ctrl Pts',(2.5411969285386,-48.3950029689925,20.));
#74461=CARTESIAN_POINT('Ctrl Pts',(2.50757558647119,-48.3937201742621,0.));
#74462=CARTESIAN_POINT('Ctrl Pts',(2.50757558647119,-48.3937201742621,20.));
#74463=CARTESIAN_POINT('Ctrl Pts',(2.47395625537494,-48.3924141746117,0.));
#74464=CARTESIAN_POINT('Ctrl Pts',(2.47395625537494,-48.3924141746117,20.));
#74465=CARTESIAN_POINT('Ctrl Pts',(2.44033895129153,-48.3910849715258,0.));
#74466=CARTESIAN_POINT('Ctrl Pts',(2.44033895129153,-48.3910849715258,20.));
#74467=CARTESIAN_POINT('Ctrl Pts',(2.40672369026195,-48.3897325665,0.));
#74468=CARTESIAN_POINT('Ctrl Pts',(2.40672369026195,-48.3897325665,20.));
#74469=CARTESIAN_POINT('Ctrl Pts',(2.37311048832664,-48.3883569610415,0.));
#74470=CARTESIAN_POINT('Ctrl Pts',(2.37311048832664,-48.3883569610415,20.));
#74471=CARTESIAN_POINT('Ctrl Pts',(2.33949936152533,-48.3869581566679,0.));
#74472=CARTESIAN_POINT('Ctrl Pts',(2.33949936152533,-48.3869581566679,20.));
#74473=CARTESIAN_POINT('Ctrl Pts',(2.30589032589699,-48.3855361549086,0.));
#74474=CARTESIAN_POINT('Ctrl Pts',(2.30589032589699,-48.3855361549086,20.));
#74475=CARTESIAN_POINT('Ctrl Pts',(2.27228339748008,-48.3840909573039,0.));
#74476=CARTESIAN_POINT('Ctrl Pts',(2.27228339748008,-48.3840909573039,20.));
#74477=CARTESIAN_POINT('Ctrl Pts',(2.2386785923122,-48.3826225654054,0.));
#74478=CARTESIAN_POINT('Ctrl Pts',(2.2386785923122,-48.3826225654054,20.));
#74479=CARTESIAN_POINT('Ctrl Pts',(2.20507592643041,-48.3811309807756,0.));
#74480=CARTESIAN_POINT('Ctrl Pts',(2.20507592643041,-48.3811309807756,20.));
#74481=CARTESIAN_POINT('Ctrl Pts',(2.17147541587102,-48.3796162049883,0.));
#74482=CARTESIAN_POINT('Ctrl Pts',(2.17147541587102,-48.3796162049883,20.));
#74483=CARTESIAN_POINT('Ctrl Pts',(2.13787707667012,-48.3780782396279,0.));
#74484=CARTESIAN_POINT('Ctrl Pts',(2.13787707667012,-48.3780782396279,20.));
#74485=CARTESIAN_POINT('Ctrl Pts',(2.10428092486293,-48.3765170862905,0.));
#74486=CARTESIAN_POINT('Ctrl Pts',(2.10428092486293,-48.3765170862905,20.));
#74487=CARTESIAN_POINT('Ctrl Pts',(2.07068697648387,-48.374932746583,0.));
#74488=CARTESIAN_POINT('Ctrl Pts',(2.07068697648387,-48.374932746583,20.));
#74489=CARTESIAN_POINT('Ctrl Pts',(2.03709524756654,-48.3733252221237,0.));
#74490=CARTESIAN_POINT('Ctrl Pts',(2.03709524756654,-48.3733252221237,20.));
#74491=CARTESIAN_POINT('Ctrl Pts',(2.00350575414355,-48.3716945145424,0.));
#74492=CARTESIAN_POINT('Ctrl Pts',(2.00350575414355,-48.3716945145424,20.));
#74493=CARTESIAN_POINT('Ctrl Pts',(1.96991851224691,-48.3700406254798,0.));
#74494=CARTESIAN_POINT('Ctrl Pts',(1.96991851224691,-48.3700406254798,20.));
#74495=CARTESIAN_POINT('Ctrl Pts',(1.93633353790811,-48.3683635565876,0.));
#74496=CARTESIAN_POINT('Ctrl Pts',(1.93633353790811,-48.3683635565876,20.));
#74497=CARTESIAN_POINT('Ctrl Pts',(1.90275084715795,-48.3666633095284,0.));
#74498=CARTESIAN_POINT('Ctrl Pts',(1.90275084715795,-48.3666633095284,20.));
#74499=CARTESIAN_POINT('Ctrl Pts',(1.86917045602651,-48.3649398859758,0.));
#74500=CARTESIAN_POINT('Ctrl Pts',(1.86917045602651,-48.3649398859758,20.));
#74501=CARTESIAN_POINT('Ctrl Pts',(1.83559238054322,-48.3631932876149,0.));
#74502=CARTESIAN_POINT('Ctrl Pts',(1.83559238054322,-48.3631932876149,20.));
#74503=CARTESIAN_POINT('Ctrl Pts',(1.80201663673655,-48.3614235161422,0.));
#74504=CARTESIAN_POINT('Ctrl Pts',(1.80201663673655,-48.3614235161422,20.));
#74505=CARTESIAN_POINT('Ctrl Pts',(1.76844324063425,-48.3596305732653,0.));
#74506=CARTESIAN_POINT('Ctrl Pts',(1.76844324063425,-48.3596305732653,20.));
#74507=CARTESIAN_POINT('Ctrl Pts',(1.73487220826325,-48.357814460703,0.));
#74508=CARTESIAN_POINT('Ctrl Pts',(1.73487220826325,-48.357814460703,20.));
#74509=CARTESIAN_POINT('Ctrl Pts',(1.70130355564956,-48.3559751801849,0.));
#74510=CARTESIAN_POINT('Ctrl Pts',(1.70130355564956,-48.3559751801849,20.));
#74511=CARTESIAN_POINT('Ctrl Pts',(1.66773729881855,-48.3541127334515,0.));
#74512=CARTESIAN_POINT('Ctrl Pts',(1.66773729881855,-48.3541127334515,20.));
#74513=CARTESIAN_POINT('Ctrl Pts',(1.63417345379481,-48.3522271222546,0.));
#74514=CARTESIAN_POINT('Ctrl Pts',(1.63417345379481,-48.3522271222546,20.));
#74515=CARTESIAN_POINT('Ctrl Pts',(1.60061203660205,-48.350318348357,0.));
#74516=CARTESIAN_POINT('Ctrl Pts',(1.60061203660205,-48.350318348357,20.));
#74517=CARTESIAN_POINT('Ctrl Pts',(1.56705306326331,-48.3483864135332,0.));
#74518=CARTESIAN_POINT('Ctrl Pts',(1.56705306326331,-48.3483864135332,20.));
#74519=CARTESIAN_POINT('Ctrl Pts',(1.53349654980076,-48.3464313195685,0.));
#74520=CARTESIAN_POINT('Ctrl Pts',(1.53349654980076,-48.3464313195685,20.));
#74521=CARTESIAN_POINT('Ctrl Pts',(1.4999425122357,-48.3444530682597,0.));
#74522=CARTESIAN_POINT('Ctrl Pts',(1.4999425122357,-48.3444530682597,20.));
#74523=CARTESIAN_POINT('Ctrl Pts',(1.46639096658851,-48.3424516614145,0.));
#74524=CARTESIAN_POINT('Ctrl Pts',(1.46639096658851,-48.3424516614145,20.));
#74525=CARTESIAN_POINT('Ctrl Pts',(1.43284192887878,-48.3404271008519,0.));
#74526=CARTESIAN_POINT('Ctrl Pts',(1.43284192887878,-48.3404271008519,20.));
#74527=CARTESIAN_POINT('Ctrl Pts',(1.39929541512519,-48.3383793884017,0.));
#74528=CARTESIAN_POINT('Ctrl Pts',(1.39929541512519,-48.3383793884017,20.));
#74529=CARTESIAN_POINT('Ctrl Pts',(1.3657514413457,-48.336308525905,0.));
#74530=CARTESIAN_POINT('Ctrl Pts',(1.3657514413457,-48.336308525905,20.));
#74531=CARTESIAN_POINT('Ctrl Pts',(1.33221002355742,-48.3342145152137,0.));
#74532=CARTESIAN_POINT('Ctrl Pts',(1.33221002355742,-48.3342145152137,20.));
#74533=CARTESIAN_POINT('Ctrl Pts',(1.29867117777651,-48.3320973581913,0.));
#74534=CARTESIAN_POINT('Ctrl Pts',(1.29867117777651,-48.3320973581913,20.));
#74535=CARTESIAN_POINT('Ctrl Pts',(1.26513492001821,-48.3299570567123,0.));
#74536=CARTESIAN_POINT('Ctrl Pts',(1.26513492001821,-48.3299570567123,20.));
#74537=CARTESIAN_POINT('Ctrl Pts',(1.23160126629692,-48.3277936126623,0.));
#74538=CARTESIAN_POINT('Ctrl Pts',(1.23160126629692,-48.3277936126623,20.));
#74539=CARTESIAN_POINT('Ctrl Pts',(1.19807023262611,-48.3256070279384,0.));
#74540=CARTESIAN_POINT('Ctrl Pts',(1.19807023262611,-48.3256070279384,20.));
#74541=CARTESIAN_POINT('Ctrl Pts',(1.16454183501838,-48.3233973044482,0.));
#74542=CARTESIAN_POINT('Ctrl Pts',(1.16454183501838,-48.3233973044482,20.));
#74543=CARTESIAN_POINT('Ctrl Pts',(1.13101608948534,-48.3211644441107,0.));
#74544=CARTESIAN_POINT('Ctrl Pts',(1.13101608948534,-48.3211644441107,20.));
#74545=CARTESIAN_POINT('Ctrl Pts',(1.09749301203762,-48.3189084488565,0.));
#74546=CARTESIAN_POINT('Ctrl Pts',(1.09749301203762,-48.3189084488565,20.));
#74547=CARTESIAN_POINT('Ctrl Pts',(1.063972618685,-48.3166293206271,0.));
#74548=CARTESIAN_POINT('Ctrl Pts',(1.063972618685,-48.3166293206271,20.));
#74549=CARTESIAN_POINT('Ctrl Pts',(1.0304549254364,-48.3143270613748,0.));
#74550=CARTESIAN_POINT('Ctrl Pts',(1.0304549254364,-48.3143270613748,20.));
#74551=CARTESIAN_POINT('Ctrl Pts',(0.996939948299849,-48.312001673063,0.));
#74552=CARTESIAN_POINT('Ctrl Pts',(0.996939948299849,-48.312001673063,20.));
#74553=CARTESIAN_POINT('Ctrl Pts',(0.963427703282353,-48.3096531576664,
0.));
#74554=CARTESIAN_POINT('Ctrl Pts',(0.963427703282353,-48.3096531576664,
20.));
#74555=CARTESIAN_POINT('Ctrl Pts',(0.929918206389826,-48.3072815171712,
0.));
#74556=CARTESIAN_POINT('Ctrl Pts',(0.929918206389826,-48.3072815171712,
20.));
#74557=CARTESIAN_POINT('Ctrl Pts',(0.896411473627223,-48.3048867535744,
0.));
#74558=CARTESIAN_POINT('Ctrl Pts',(0.896411473627223,-48.3048867535744,
20.));
#74559=CARTESIAN_POINT('Ctrl Pts',(0.862907520998486,-48.3024688688845,
0.));
#74560=CARTESIAN_POINT('Ctrl Pts',(0.862907520998486,-48.3024688688845,
20.));
#74561=CARTESIAN_POINT('Ctrl Pts',(0.829406364506662,-48.3000278651208,
0.));
#74562=CARTESIAN_POINT('Ctrl Pts',(0.829406364506662,-48.3000278651208,
20.));
#74563=CARTESIAN_POINT('Ctrl Pts',(0.795908020153888,-48.2975637443136,
0.));
#74564=CARTESIAN_POINT('Ctrl Pts',(0.795908020153888,-48.2975637443136,
20.));
#74565=CARTESIAN_POINT('Ctrl Pts',(0.762412503941521,-48.2950765085043,
0.));
#74566=CARTESIAN_POINT('Ctrl Pts',(0.762412503941521,-48.2950765085043,
20.));
#74567=CARTESIAN_POINT('Ctrl Pts',(0.728919831869645,-48.2925661597457,
0.));
#74568=CARTESIAN_POINT('Ctrl Pts',(0.728919831869645,-48.2925661597457,
20.));
#74569=CARTESIAN_POINT('Ctrl Pts',(0.69543001993734,-48.2900327001016,0.));
#74570=CARTESIAN_POINT('Ctrl Pts',(0.69543001993734,-48.2900327001016,20.));
#74571=CARTESIAN_POINT('Ctrl Pts',(0.661943084142442,-48.2874761316474,
0.));
#74572=CARTESIAN_POINT('Ctrl Pts',(0.661943084142442,-48.2874761316474,
20.));
#74573=CARTESIAN_POINT('Ctrl Pts',(0.628459040481828,-48.2848964564694,
0.));
#74574=CARTESIAN_POINT('Ctrl Pts',(0.628459040481828,-48.2848964564694,
20.));
#74575=CARTESIAN_POINT('Ctrl Pts',(0.594977904951266,-48.282293676665,0.));
#74576=CARTESIAN_POINT('Ctrl Pts',(0.594977904951266,-48.282293676665,20.));
#74577=CARTESIAN_POINT('Ctrl Pts',(0.561499693545673,-48.2796677943426,
0.));
#74578=CARTESIAN_POINT('Ctrl Pts',(0.561499693545673,-48.2796677943426,
20.));
#74579=CARTESIAN_POINT('Ctrl Pts',(0.528024422259019,-48.2770188116216,
0.));
#74580=CARTESIAN_POINT('Ctrl Pts',(0.528024422259019,-48.2770188116216,
20.));
#74581=CARTESIAN_POINT('Ctrl Pts',(0.49455210708421,-48.2743467306329,0.));
#74582=CARTESIAN_POINT('Ctrl Pts',(0.49455210708421,-48.2743467306329,20.));
#74583=CARTESIAN_POINT('Ctrl Pts',(0.461082764012986,-48.2716515535183,
0.));
#74584=CARTESIAN_POINT('Ctrl Pts',(0.461082764012986,-48.2716515535183,
20.));
#74585=CARTESIAN_POINT('Ctrl Pts',(0.427616409036036,-48.2689332824309,
0.));
#74586=CARTESIAN_POINT('Ctrl Pts',(0.427616409036036,-48.2689332824309,
20.));
#74587=CARTESIAN_POINT('Ctrl Pts',(0.394153058142903,-48.2661919195348,
0.));
#74588=CARTESIAN_POINT('Ctrl Pts',(0.394153058142903,-48.2661919195348,
20.));
#74589=CARTESIAN_POINT('Ctrl Pts',(0.360692727321981,-48.2634274670053,
0.));
#74590=CARTESIAN_POINT('Ctrl Pts',(0.360692727321981,-48.2634274670053,
20.));
#74591=CARTESIAN_POINT('Ctrl Pts',(0.327235432560538,-48.2606399270286,
0.));
#74592=CARTESIAN_POINT('Ctrl Pts',(0.327235432560538,-48.2606399270286,
20.));
#74593=CARTESIAN_POINT('Ctrl Pts',(0.293781189844817,-48.2578293018028,
0.));
#74594=CARTESIAN_POINT('Ctrl Pts',(0.293781189844817,-48.2578293018028,
20.));
#74595=CARTESIAN_POINT('Ctrl Pts',(0.260330015159931,-48.2549955935366,
0.));
#74596=CARTESIAN_POINT('Ctrl Pts',(0.260330015159931,-48.2549955935366,
20.));
#74597=CARTESIAN_POINT('Ctrl Pts',(0.226881924489848,-48.2521388044499,
0.));
#74598=CARTESIAN_POINT('Ctrl Pts',(0.226881924489848,-48.2521388044499,
20.));
#74599=CARTESIAN_POINT('Ctrl Pts',(0.193436933817455,-48.2492589367737,
0.));
#74600=CARTESIAN_POINT('Ctrl Pts',(0.193436933817455,-48.2492589367737,
20.));
#74601=CARTESIAN_POINT('Ctrl Pts',(0.159995059124558,-48.2463559927498,
0.));
#74602=CARTESIAN_POINT('Ctrl Pts',(0.159995059124558,-48.2463559927498,
20.));
#74603=CARTESIAN_POINT('Ctrl Pts',(0.126556316391659,-48.2434299746318,
0.));
#74604=CARTESIAN_POINT('Ctrl Pts',(0.126556316391659,-48.2434299746318,
20.));
#74605=CARTESIAN_POINT('Ctrl Pts',(0.0931207215982655,-48.2404808846839,
0.));
#74606=CARTESIAN_POINT('Ctrl Pts',(0.0931207215982655,-48.2404808846839,
20.));
#74607=CARTESIAN_POINT('Ctrl Pts',(0.0596882907225815,-48.2375087251817,
0.));
#74608=CARTESIAN_POINT('Ctrl Pts',(0.0596882907225815,-48.2375087251817,
20.));
#74609=CARTESIAN_POINT('Ctrl Pts',(0.0262590397416584,-48.234513498412,
0.));
#74610=CARTESIAN_POINT('Ctrl Pts',(0.0262590397416584,-48.234513498412,
20.));
#74611=CARTESIAN_POINT('Ctrl Pts',(-0.00716701536858544,-48.2314952066725,
0.));
#74612=CARTESIAN_POINT('Ctrl Pts',(-0.00716701536858544,-48.2314952066725,
20.));
#74613=CARTESIAN_POINT('Ctrl Pts',(-0.040589858633453,-48.2284538522724,
0.));
#74614=CARTESIAN_POINT('Ctrl Pts',(-0.040589858633453,-48.2284538522724,
20.));
#74615=CARTESIAN_POINT('Ctrl Pts',(-0.0740094740794106,-48.2253894375317,
0.));
#74616=CARTESIAN_POINT('Ctrl Pts',(-0.0740094740794106,-48.2253894375317,
20.));
#74617=CARTESIAN_POINT('Ctrl Pts',(-0.107425845734137,-48.2223019647818,
0.));
#74618=CARTESIAN_POINT('Ctrl Pts',(-0.107425845734137,-48.2223019647818,
20.));
#74619=CARTESIAN_POINT('Ctrl Pts',(-0.140838957626559,-48.2191914363652,
0.));
#74620=CARTESIAN_POINT('Ctrl Pts',(-0.140838957626559,-48.2191914363652,
20.));
#74621=CARTESIAN_POINT('Ctrl Pts',(-0.174248793786917,-48.2160578546352,
0.));
#74622=CARTESIAN_POINT('Ctrl Pts',(-0.174248793786917,-48.2160578546352,
20.));
#74623=CARTESIAN_POINT('Ctrl Pts',(-0.207655338246577,-48.2129012219564,
0.));
#74624=CARTESIAN_POINT('Ctrl Pts',(-0.207655338246577,-48.2129012219564,
20.));
#74625=CARTESIAN_POINT('Ctrl Pts',(-0.241058575037889,-48.2097215407045,
0.));
#74626=CARTESIAN_POINT('Ctrl Pts',(-0.241058575037889,-48.2097215407045,
20.));
#74627=CARTESIAN_POINT('Ctrl Pts',(-0.274458488194607,-48.2065188132665,
0.));
#74628=CARTESIAN_POINT('Ctrl Pts',(-0.274458488194607,-48.2065188132665,
20.));
#74629=CARTESIAN_POINT('Ctrl Pts',(-0.307855061751732,-48.2032930420408,
0.));
#74630=CARTESIAN_POINT('Ctrl Pts',(-0.307855061751732,-48.2032930420408,
20.));
#74631=CARTESIAN_POINT('Ctrl Pts',(-0.341248279745661,-48.2000442294364,
0.));
#74632=CARTESIAN_POINT('Ctrl Pts',(-0.341248279745661,-48.2000442294364,
20.));
#74633=CARTESIAN_POINT('Ctrl Pts',(-0.374638126214117,-48.1967723778737,
0.));
#74634=CARTESIAN_POINT('Ctrl Pts',(-0.374638126214117,-48.1967723778737,
20.));
#74635=CARTESIAN_POINT('Ctrl Pts',(-0.408024585196243,-48.1934774897842,
0.));
#74636=CARTESIAN_POINT('Ctrl Pts',(-0.408024585196243,-48.1934774897842,
20.));
#74637=CARTESIAN_POINT('Ctrl Pts',(-0.441407640732114,-48.1901595676102,
0.));
#74638=CARTESIAN_POINT('Ctrl Pts',(-0.441407640732114,-48.1901595676102,
20.));
#74639=CARTESIAN_POINT('Ctrl Pts',(-0.474787276863089,-48.1868186138054,
0.));
#74640=CARTESIAN_POINT('Ctrl Pts',(-0.474787276863089,-48.1868186138054,
20.));
#74641=CARTESIAN_POINT('Ctrl Pts',(-0.508163477631873,-48.1834546308352,
0.));
#74642=CARTESIAN_POINT('Ctrl Pts',(-0.508163477631873,-48.1834546308352,
20.));
#74643=CARTESIAN_POINT('Ctrl Pts',(-0.541536227082378,-48.1800676211754,
0.));
#74644=CARTESIAN_POINT('Ctrl Pts',(-0.541536227082378,-48.1800676211754,
20.));
#74645=CARTESIAN_POINT('Ctrl Pts',(-0.574905509259906,-48.1766575873132,
0.));
#74646=CARTESIAN_POINT('Ctrl Pts',(-0.574905509259906,-48.1766575873132,
20.));
#74647=CARTESIAN_POINT('Ctrl Pts',(-0.608271308211115,-48.1732245317468,
0.));
#74648=CARTESIAN_POINT('Ctrl Pts',(-0.608271308211115,-48.1732245317468,
20.));
#74649=CARTESIAN_POINT('Ctrl Pts',(-0.641633607984118,-48.1697684569855,
0.));
#74650=CARTESIAN_POINT('Ctrl Pts',(-0.641633607984118,-48.1697684569855,
20.));
#74651=CARTESIAN_POINT('Ctrl Pts',(-0.674992392628253,-48.16628936555,0.));
#74652=CARTESIAN_POINT('Ctrl Pts',(-0.674992392628253,-48.16628936555,20.));
#74653=CARTESIAN_POINT('Ctrl Pts',(-0.708347646194296,-48.1627872599717,
0.));
#74654=CARTESIAN_POINT('Ctrl Pts',(-0.708347646194296,-48.1627872599717,
20.));
#74655=CARTESIAN_POINT('Ctrl Pts',(-0.741699352734275,-48.1592621427937,
0.));
#74656=CARTESIAN_POINT('Ctrl Pts',(-0.741699352734275,-48.1592621427937,
20.));
#74657=CARTESIAN_POINT('Ctrl Pts',(-0.775047496301551,-48.1557140165701,
0.));
#74658=CARTESIAN_POINT('Ctrl Pts',(-0.775047496301551,-48.1557140165701,
20.));
#74659=CARTESIAN_POINT('Ctrl Pts',(-0.808392060950887,-48.1521428838659,
0.));
#74660=CARTESIAN_POINT('Ctrl Pts',(-0.808392060950887,-48.1521428838659,
20.));
#74661=CARTESIAN_POINT('Ctrl Pts',(-0.84173303073841,-48.1485487472572,
0.));
#74662=CARTESIAN_POINT('Ctrl Pts',(-0.84173303073841,-48.1485487472572,
20.));
#74663=CARTESIAN_POINT('Ctrl Pts',(-0.875070389721544,-48.144931609331,
0.));
#74664=CARTESIAN_POINT('Ctrl Pts',(-0.875070389721544,-48.144931609331,
20.));
#74665=CARTESIAN_POINT('Ctrl Pts',(-0.908404121959303,-48.1412914726861,
0.));
#74666=CARTESIAN_POINT('Ctrl Pts',(-0.908404121959303,-48.1412914726861,
20.));
#74667=CARTESIAN_POINT('Ctrl Pts',(-0.941734211511966,-48.137628339932,
0.));
#74668=CARTESIAN_POINT('Ctrl Pts',(-0.941734211511966,-48.137628339932,
20.));
#74669=CARTESIAN_POINT('Ctrl Pts',(-0.975060642441261,-48.1339422136897,
0.));
#74670=CARTESIAN_POINT('Ctrl Pts',(-0.975060642441261,-48.1339422136897,
20.));
#74671=CARTESIAN_POINT('Ctrl Pts',(-1.00838339881034,-48.130233096591,0.));
#74672=CARTESIAN_POINT('Ctrl Pts',(-1.00838339881034,-48.130233096591,20.));
#74673=CARTESIAN_POINT('Ctrl Pts',(-1.04170246468366,-48.1265009912787,
0.));
#74674=CARTESIAN_POINT('Ctrl Pts',(-1.04170246468366,-48.1265009912787,
20.));
#74675=CARTESIAN_POINT('Ctrl Pts',(-1.0750178241273,-48.1227459004068,0.));
#74676=CARTESIAN_POINT('Ctrl Pts',(-1.0750178241273,-48.1227459004068,20.));
#74677=CARTESIAN_POINT('Ctrl Pts',(-1.10832946120863,-48.1189678266406,
0.));
#74678=CARTESIAN_POINT('Ctrl Pts',(-1.10832946120863,-48.1189678266406,
20.));
#74679=CARTESIAN_POINT('Ctrl Pts',(-1.14163735999659,-48.1151667726565,
0.));
#74680=CARTESIAN_POINT('Ctrl Pts',(-1.14163735999659,-48.1151667726565,
20.));
#74681=CARTESIAN_POINT('Ctrl Pts',(-1.17494150456147,-48.111342741142,0.));
#74682=CARTESIAN_POINT('Ctrl Pts',(-1.17494150456147,-48.111342741142,20.));
#74683=CARTESIAN_POINT('Ctrl Pts',(-1.20824187897491,-48.1074957347955,
0.));
#74684=CARTESIAN_POINT('Ctrl Pts',(-1.20824187897491,-48.1074957347955,
20.));
#74685=CARTESIAN_POINT('Ctrl Pts',(-1.24153846731024,-48.1036257563271,
0.));
#74686=CARTESIAN_POINT('Ctrl Pts',(-1.24153846731024,-48.1036257563271,
20.));
#74687=CARTESIAN_POINT('Ctrl Pts',(-1.27483125364217,-48.0997328084577,
0.));
#74688=CARTESIAN_POINT('Ctrl Pts',(-1.27483125364217,-48.0997328084577,
20.));
#74689=CARTESIAN_POINT('Ctrl Pts',(-1.30812022204706,-48.0958168939195,
0.));
#74690=CARTESIAN_POINT('Ctrl Pts',(-1.30812022204706,-48.0958168939195,
20.));
#74691=CARTESIAN_POINT('Ctrl Pts',(-1.34140535660262,-48.0918780154556,
0.));
#74692=CARTESIAN_POINT('Ctrl Pts',(-1.34140535660262,-48.0918780154556,
20.));
#74693=CARTESIAN_POINT('Ctrl Pts',(-1.37468664138803,-48.0879161758201,
0.));
#74694=CARTESIAN_POINT('Ctrl Pts',(-1.37468664138803,-48.0879161758201,
20.));
#74695=CARTESIAN_POINT('Ctrl Pts',(-1.40796406048389,-48.0839313777781,
0.));
#74696=CARTESIAN_POINT('Ctrl Pts',(-1.40796406048389,-48.0839313777781,
20.));
#74697=CARTESIAN_POINT('Ctrl Pts',(-1.44123759797226,-48.0799236241059,
0.));
#74698=CARTESIAN_POINT('Ctrl Pts',(-1.44123759797226,-48.0799236241059,
20.));
#74699=CARTESIAN_POINT('Ctrl Pts',(-1.47450723793683,-48.0758929175908,
0.));
#74700=CARTESIAN_POINT('Ctrl Pts',(-1.47450723793683,-48.0758929175908,
20.));
#74701=CARTESIAN_POINT('Ctrl Pts',(-1.50777296446293,-48.071839261032,0.));
#74702=CARTESIAN_POINT('Ctrl Pts',(-1.50777296446293,-48.071839261032,20.));
#74703=CARTESIAN_POINT('Ctrl Pts',(-1.54103476163745,-48.0677626572394,
0.));
#74704=CARTESIAN_POINT('Ctrl Pts',(-1.54103476163745,-48.0677626572394,
20.));
#74705=CARTESIAN_POINT('Ctrl Pts',(-1.57429261354891,-48.0636631090342,
0.));
#74706=CARTESIAN_POINT('Ctrl Pts',(-1.57429261354891,-48.0636631090342,
20.));
#74707=CARTESIAN_POINT('Ctrl Pts',(-1.60754650428747,-48.0595406192492,
0.));
#74708=CARTESIAN_POINT('Ctrl Pts',(-1.60754650428747,-48.0595406192492,
20.));
#74709=CARTESIAN_POINT('Ctrl Pts',(-1.64079641794463,-48.0553951907273,
0.));
#74710=CARTESIAN_POINT('Ctrl Pts',(-1.64079641794463,-48.0553951907273,
20.));
#74711=CARTESIAN_POINT('Ctrl Pts',(-1.67404233861339,-48.0512268263229,
0.));
#74712=CARTESIAN_POINT('Ctrl Pts',(-1.67404233861339,-48.0512268263229,
20.));
#74713=CARTESIAN_POINT('Ctrl Pts',(-1.70728425038806,-48.0470355289011,
0.));
#74714=CARTESIAN_POINT('Ctrl Pts',(-1.70728425038806,-48.0470355289011,
20.));
#74715=CARTESIAN_POINT('Ctrl Pts',(-1.74052213736473,-48.0428213013379,
0.));
#74716=CARTESIAN_POINT('Ctrl Pts',(-1.74052213736473,-48.0428213013379,
20.));
#74717=CARTESIAN_POINT('Ctrl Pts',(-1.77375598364111,-48.038584146521,0.));
#74718=CARTESIAN_POINT('Ctrl Pts',(-1.77375598364111,-48.038584146521,20.));
#74719=CARTESIAN_POINT('Ctrl Pts',(-1.80698577331665,-48.0343240673492,
0.));
#74720=CARTESIAN_POINT('Ctrl Pts',(-1.80698577331665,-48.0343240673492,
20.));
#74721=CARTESIAN_POINT('Ctrl Pts',(-1.84021149049247,-48.0300410667328,
0.));
#74722=CARTESIAN_POINT('Ctrl Pts',(-1.84021149049247,-48.0300410667328,
20.));
#74723=CARTESIAN_POINT('Ctrl Pts',(-1.87343311927143,-48.0257351475934,
0.));
#74724=CARTESIAN_POINT('Ctrl Pts',(-1.87343311927143,-48.0257351475934,
20.));
#74725=CARTESIAN_POINT('Ctrl Pts',(-1.90665064375788,-48.0214063128629,
0.));
#74726=CARTESIAN_POINT('Ctrl Pts',(-1.90665064375788,-48.0214063128629,
20.));
#74727=CARTESIAN_POINT('Ctrl Pts',(-1.93986404805774,-48.0170545654849,
0.));
#74728=CARTESIAN_POINT('Ctrl Pts',(-1.93986404805774,-48.0170545654849,
20.));
#74729=CARTESIAN_POINT('Ctrl Pts',(-1.97307331627851,-48.0126799084137,
0.));
#74730=CARTESIAN_POINT('Ctrl Pts',(-1.97307331627851,-48.0126799084137,
20.));
#74731=CARTESIAN_POINT('Ctrl Pts',(-2.00627843252927,-48.0082823446147,
0.));
#74732=CARTESIAN_POINT('Ctrl Pts',(-2.00627843252927,-48.0082823446147,
20.));
#74733=CARTESIAN_POINT('Ctrl Pts',(-2.03947938092069,-48.0038618770642,
0.));
#74734=CARTESIAN_POINT('Ctrl Pts',(-2.03947938092069,-48.0038618770642,
20.));
#74735=CARTESIAN_POINT('Ctrl Pts',(-2.07267614556538,-47.9994185087499,
0.));
#74736=CARTESIAN_POINT('Ctrl Pts',(-2.07267614556538,-47.9994185087499,
20.));
#74737=CARTESIAN_POINT('Ctrl Pts',(-2.1058687105775,-47.994952242671,0.));
#74738=CARTESIAN_POINT('Ctrl Pts',(-2.1058687105775,-47.994952242671,20.));
#74739=CARTESIAN_POINT('Ctrl Pts',(-2.13905706007287,-47.9904630818375,
0.));
#74740=CARTESIAN_POINT('Ctrl Pts',(-2.13905706007287,-47.9904630818375,
20.));
#74741=CARTESIAN_POINT('Ctrl Pts',(-2.172241178169,-47.9859510292704,0.));
#74742=CARTESIAN_POINT('Ctrl Pts',(-2.172241178169,-47.9859510292704,20.));
#74743=CARTESIAN_POINT('Ctrl Pts',(-2.20542104898522,-47.9814160880019,
0.));
#74744=CARTESIAN_POINT('Ctrl Pts',(-2.20542104898522,-47.9814160880019,
20.));
#74745=CARTESIAN_POINT('Ctrl Pts',(-2.23859665664241,-47.9768582610752,
0.));
#74746=CARTESIAN_POINT('Ctrl Pts',(-2.23859665664241,-47.9768582610752,
20.));
#74747=CARTESIAN_POINT('Ctrl Pts',(-2.27176798526354,-47.9722775515452,
0.));
#74748=CARTESIAN_POINT('Ctrl Pts',(-2.27176798526354,-47.9722775515452,
20.));
#74749=CARTESIAN_POINT('Ctrl Pts',(-2.30493501897296,-47.9676739624772,
0.));
#74750=CARTESIAN_POINT('Ctrl Pts',(-2.30493501897296,-47.9676739624772,
20.));
#74751=CARTESIAN_POINT('Ctrl Pts',(-2.33809774189659,-47.9630474969481,
0.));
#74752=CARTESIAN_POINT('Ctrl Pts',(-2.33809774189659,-47.9630474969481,
20.));
#74753=CARTESIAN_POINT('Ctrl Pts',(-2.37125613816232,-47.9583981580454,
0.));
#74754=CARTESIAN_POINT('Ctrl Pts',(-2.37125613816232,-47.9583981580454,
20.));
#74755=CARTESIAN_POINT('Ctrl Pts',(-2.40441019189961,-47.9537259488681,
0.));
#74756=CARTESIAN_POINT('Ctrl Pts',(-2.40441019189961,-47.9537259488681,
20.));
#74757=CARTESIAN_POINT('Ctrl Pts',(-2.43755988723967,-47.9490308725257,
0.));
#74758=CARTESIAN_POINT('Ctrl Pts',(-2.43755988723967,-47.9490308725257,
20.));
#74759=CARTESIAN_POINT('Ctrl Pts',(-2.4707052083155,-47.9443129321394,0.));
#74760=CARTESIAN_POINT('Ctrl Pts',(-2.4707052083155,-47.9443129321394,20.));
#74761=CARTESIAN_POINT('Ctrl Pts',(-2.5038461392621,-47.9395721308414,0.));
#74762=CARTESIAN_POINT('Ctrl Pts',(-2.5038461392621,-47.9395721308414,20.));
#74763=CARTESIAN_POINT('Ctrl Pts',(-2.53698266421615,-47.9348084717752,
0.));
#74764=CARTESIAN_POINT('Ctrl Pts',(-2.53698266421615,-47.9348084717752,
20.));
#74765=CARTESIAN_POINT('Ctrl Pts',(-2.57011476731624,-47.9300219580955,
0.));
#74766=CARTESIAN_POINT('Ctrl Pts',(-2.57011476731624,-47.9300219580955,
20.));
#74767=CARTESIAN_POINT('Ctrl Pts',(-2.60324243270259,-47.9252125929679,
0.));
#74768=CARTESIAN_POINT('Ctrl Pts',(-2.60324243270259,-47.9252125929679,
20.));
#74769=CARTESIAN_POINT('Ctrl Pts',(-2.6363656445172,-47.9203803795688,0.));
#74770=CARTESIAN_POINT('Ctrl Pts',(-2.6363656445172,-47.9203803795688,20.));
#74771=CARTESIAN_POINT('Ctrl Pts',(-2.66948438690367,-47.9155253210858,
0.));
#74772=CARTESIAN_POINT('Ctrl Pts',(-2.66948438690367,-47.9155253210858,
20.));
#74773=CARTESIAN_POINT('Ctrl Pts',(-2.70259864400759,-47.9106474207177,
0.));
#74774=CARTESIAN_POINT('Ctrl Pts',(-2.70259864400759,-47.9106474207177,
20.));
#74775=CARTESIAN_POINT('Ctrl Pts',(-2.7357083999763,-47.9057466816743,0.));
#74776=CARTESIAN_POINT('Ctrl Pts',(-2.7357083999763,-47.9057466816743,20.));
#74777=CARTESIAN_POINT('Ctrl Pts',(-2.76881363895919,-47.9008231071768,
0.));
#74778=CARTESIAN_POINT('Ctrl Pts',(-2.76881363895919,-47.9008231071768,
20.));
#74779=CARTESIAN_POINT('Ctrl Pts',(-2.80191434510735,-47.8958767004573,
0.));
#74780=CARTESIAN_POINT('Ctrl Pts',(-2.80191434510735,-47.8958767004573,
20.));
#74781=CARTESIAN_POINT('Ctrl Pts',(-2.83501050257377,-47.8909074647592,
0.));
#74782=CARTESIAN_POINT('Ctrl Pts',(-2.83501050257377,-47.8909074647592,
20.));
#74783=CARTESIAN_POINT('Ctrl Pts',(-2.86810209551309,-47.8859154033363,
0.));
#74784=CARTESIAN_POINT('Ctrl Pts',(-2.86810209551309,-47.8859154033363,
20.));
#74785=CARTESIAN_POINT('Ctrl Pts',(-2.90118910808201,-47.8809005194543,
0.));
#74786=CARTESIAN_POINT('Ctrl Pts',(-2.90118910808201,-47.8809005194543,
20.));
#74787=CARTESIAN_POINT('Ctrl Pts',(-2.93427152443919,-47.8758628163901,
0.));
#74788=CARTESIAN_POINT('Ctrl Pts',(-2.93427152443919,-47.8758628163901,
20.));
#74789=CARTESIAN_POINT('Ctrl Pts',(-2.96734932874506,-47.8708022974315,
0.));
#74790=CARTESIAN_POINT('Ctrl Pts',(-2.96734932874506,-47.8708022974315,
20.));
#74791=CARTESIAN_POINT('Ctrl Pts',(-3.00042250516194,-47.8657189658771,
0.));
#74792=CARTESIAN_POINT('Ctrl Pts',(-3.00042250516194,-47.8657189658771,
20.));
#74793=CARTESIAN_POINT('Ctrl Pts',(-3.03349103785389,-47.8606128250365,
0.));
#74794=CARTESIAN_POINT('Ctrl Pts',(-3.03349103785389,-47.8606128250365,
20.));
#74795=CARTESIAN_POINT('Ctrl Pts',(-3.06655491098683,-47.8554838782302,
0.));
#74796=CARTESIAN_POINT('Ctrl Pts',(-3.06655491098683,-47.8554838782302,
20.));
#74797=CARTESIAN_POINT('Ctrl Pts',(-3.09961410872877,-47.8503321287903,
0.));
#74798=CARTESIAN_POINT('Ctrl Pts',(-3.09961410872877,-47.8503321287903,
20.));
#74799=CARTESIAN_POINT('Ctrl Pts',(-3.13266861524955,-47.8451575800601,
0.));
#74800=CARTESIAN_POINT('Ctrl Pts',(-3.13266861524955,-47.8451575800601,
20.));
#74801=CARTESIAN_POINT('Ctrl Pts',(-3.16571841472091,-47.8399602353939,
0.));
#74802=CARTESIAN_POINT('Ctrl Pts',(-3.16571841472091,-47.8399602353939,
20.));
#74803=CARTESIAN_POINT('Ctrl Pts',(-3.19876349131676,-47.834740098157,0.));
#74804=CARTESIAN_POINT('Ctrl Pts',(-3.19876349131676,-47.834740098157,20.));
#74805=CARTESIAN_POINT('Ctrl Pts',(-3.23180382921274,-47.829497171726,0.));
#74806=CARTESIAN_POINT('Ctrl Pts',(-3.23180382921274,-47.829497171726,20.));
#74807=CARTESIAN_POINT('Ctrl Pts',(-3.26483941258678,-47.8242314594881,
0.));
#74808=CARTESIAN_POINT('Ctrl Pts',(-3.26483941258678,-47.8242314594881,
20.));
#74809=CARTESIAN_POINT('Ctrl Pts',(-3.29787022561837,-47.818942964842,0.));
#74810=CARTESIAN_POINT('Ctrl Pts',(-3.29787022561837,-47.818942964842,20.));
#74811=CARTESIAN_POINT('Ctrl Pts',(-3.33089625248904,-47.813631691197,0.));
#74812=CARTESIAN_POINT('Ctrl Pts',(-3.33089625248904,-47.813631691197,20.));
#74813=CARTESIAN_POINT('Ctrl Pts',(-3.36391747738215,-47.8082976419741,
0.));
#74814=CARTESIAN_POINT('Ctrl Pts',(-3.36391747738215,-47.8082976419741,
20.));
#74815=CARTESIAN_POINT('Ctrl Pts',(-3.39693388448307,-47.802940820605,0.));
#74816=CARTESIAN_POINT('Ctrl Pts',(-3.39693388448307,-47.802940820605,20.));
#74817=CARTESIAN_POINT('Ctrl Pts',(-3.42994545797923,-47.797561230533,0.));
#74818=CARTESIAN_POINT('Ctrl Pts',(-3.42994545797923,-47.797561230533,20.));
#74819=CARTESIAN_POINT('Ctrl Pts',(-3.46295218206013,-47.7921588752121,
0.));
#74820=CARTESIAN_POINT('Ctrl Pts',(-3.46295218206013,-47.7921588752121,
20.));
#74821=CARTESIAN_POINT('Ctrl Pts',(-3.49595404091729,-47.7867337581073,
0.));
#74822=CARTESIAN_POINT('Ctrl Pts',(-3.49595404091729,-47.7867337581073,
20.));
#74823=CARTESIAN_POINT('Ctrl Pts',(-3.52895101874416,-47.7812858826946,
0.));
#74824=CARTESIAN_POINT('Ctrl Pts',(-3.52895101874416,-47.7812858826946,
20.));
#74825=CARTESIAN_POINT('Ctrl Pts',(-3.56194309973643,-47.7758152524613,
0.));
#74826=CARTESIAN_POINT('Ctrl Pts',(-3.56194309973643,-47.7758152524613,
20.));
#74827=CARTESIAN_POINT('Ctrl Pts',(-3.59493026809159,-47.7703218709055,
0.));
#74828=CARTESIAN_POINT('Ctrl Pts',(-3.59493026809159,-47.7703218709055,
20.));
#74829=CARTESIAN_POINT('Ctrl Pts',(-3.62791250800925,-47.764805741537,0.));
#74830=CARTESIAN_POINT('Ctrl Pts',(-3.62791250800925,-47.764805741537,20.));
#74831=CARTESIAN_POINT('Ctrl Pts',(-3.66088980369085,-47.7592668678762,
0.));
#74832=CARTESIAN_POINT('Ctrl Pts',(-3.66088980369085,-47.7592668678762,
20.));
#74833=CARTESIAN_POINT('Ctrl Pts',(-3.69386213933995,-47.7537052534546,
0.));
#74834=CARTESIAN_POINT('Ctrl Pts',(-3.69386213933995,-47.7537052534546,
20.));
#74835=CARTESIAN_POINT('Ctrl Pts',(-3.72682949916223,-47.7481209018149,
0.));
#74836=CARTESIAN_POINT('Ctrl Pts',(-3.72682949916223,-47.7481209018149,
20.));
#74837=CARTESIAN_POINT('Ctrl Pts',(-3.75979186736546,-47.7425138165111,
0.));
#74838=CARTESIAN_POINT('Ctrl Pts',(-3.75979186736546,-47.7425138165111,
20.));
#74839=CARTESIAN_POINT('Ctrl Pts',(-3.7927492281595,-47.7368840011081,0.));
#74840=CARTESIAN_POINT('Ctrl Pts',(-3.7927492281595,-47.7368840011081,20.));
#74841=CARTESIAN_POINT('Ctrl Pts',(-3.82570156575624,-47.7312314591817,
0.));
#74842=CARTESIAN_POINT('Ctrl Pts',(-3.82570156575624,-47.7312314591817,
20.));
#74843=CARTESIAN_POINT('Ctrl Pts',(-3.85864886436974,-47.7255561943191,
0.));
#74844=CARTESIAN_POINT('Ctrl Pts',(-3.85864886436974,-47.7255561943191,
20.));
#74845=CARTESIAN_POINT('Ctrl Pts',(-3.89159110821606,-47.719858210118,0.));
#74846=CARTESIAN_POINT('Ctrl Pts',(-3.89159110821606,-47.719858210118,20.));
#74847=CARTESIAN_POINT('Ctrl Pts',(-3.92452828151334,-47.7141375101875,
0.));
#74848=CARTESIAN_POINT('Ctrl Pts',(-3.92452828151334,-47.7141375101875,
20.));
#74849=CARTESIAN_POINT('Ctrl Pts',(-3.95746036848188,-47.7083940981477,
0.));
#74850=CARTESIAN_POINT('Ctrl Pts',(-3.95746036848188,-47.7083940981477,
20.));
#74851=CARTESIAN_POINT('Ctrl Pts',(-3.99038735334402,-47.7026279776294,
0.));
#74852=CARTESIAN_POINT('Ctrl Pts',(-3.99038735334402,-47.7026279776294,
20.));
#74853=CARTESIAN_POINT('Ctrl Pts',(-4.02330922032434,-47.6968391522753,
0.));
#74854=CARTESIAN_POINT('Ctrl Pts',(-4.02330922032434,-47.6968391522753,
20.));
#74855=CARTESIAN_POINT('Ctrl Pts',(-4.05622595364953,-47.6910276257391,
0.));
#74856=CARTESIAN_POINT('Ctrl Pts',(-4.05622595364953,-47.6910276257391,
20.));
#74857=CARTESIAN_POINT('Ctrl Pts',(-4.0891375375485,-47.6851934016861,0.));
#74858=CARTESIAN_POINT('Ctrl Pts',(-4.0891375375485,-47.6851934016861,20.));
#74859=CARTESIAN_POINT('Ctrl Pts',(-4.1220439562522,-47.6793364837921,0.));
#74860=CARTESIAN_POINT('Ctrl Pts',(-4.1220439562522,-47.6793364837921,20.));
#74861=CARTESIAN_POINT('Ctrl Pts',(-4.15494519399371,-47.6734568757434,
0.));
#74862=CARTESIAN_POINT('Ctrl Pts',(-4.15494519399371,-47.6734568757434,
20.));
#74863=CARTESIAN_POINT('Ctrl Pts',(-4.18784123500837,-47.6675545812371,
0.));
#74864=CARTESIAN_POINT('Ctrl Pts',(-4.18784123500837,-47.6675545812371,
20.));
#74865=CARTESIAN_POINT('Ctrl Pts',(-4.22073206353346,-47.6616296039816,
0.));
#74866=CARTESIAN_POINT('Ctrl Pts',(-4.22073206353346,-47.6616296039816,
20.));
#74867=CARTESIAN_POINT('Ctrl Pts',(-4.25361766380861,-47.6556819476964,
0.));
#74868=CARTESIAN_POINT('Ctrl Pts',(-4.25361766380861,-47.6556819476964,
20.));
#74869=CARTESIAN_POINT('Ctrl Pts',(-4.28649802007568,-47.6497116161128,
0.));
#74870=CARTESIAN_POINT('Ctrl Pts',(-4.28649802007568,-47.6497116161128,
20.));
#74871=CARTESIAN_POINT('Ctrl Pts',(-4.31937311657887,-47.6437186129734,
0.));
#74872=CARTESIAN_POINT('Ctrl Pts',(-4.31937311657887,-47.6437186129734,
20.));
#74873=CARTESIAN_POINT('Ctrl Pts',(-4.35224293756441,-47.6377029420315,
0.));
#74874=CARTESIAN_POINT('Ctrl Pts',(-4.35224293756441,-47.6377029420315,
20.));
#74875=CARTESIAN_POINT('Ctrl Pts',(-4.38510746728076,-47.6316646070511,
0.));
#74876=CARTESIAN_POINT('Ctrl Pts',(-4.38510746728076,-47.6316646070511,
20.));
#74877=CARTESIAN_POINT('Ctrl Pts',(-4.41796668997837,-47.6256036118071,
0.));
#74878=CARTESIAN_POINT('Ctrl Pts',(-4.41796668997837,-47.6256036118071,
20.));
#74879=CARTESIAN_POINT('Ctrl Pts',(-4.45082058991005,-47.6195199600851,
0.));
#74880=CARTESIAN_POINT('Ctrl Pts',(-4.45082058991005,-47.6195199600851,
20.));
#74881=CARTESIAN_POINT('Ctrl Pts',(-4.48366915133085,-47.6134136556823,
0.));
#74882=CARTESIAN_POINT('Ctrl Pts',(-4.48366915133085,-47.6134136556823,
20.));
#74883=CARTESIAN_POINT('Ctrl Pts',(-4.51651235849824,-47.6072847024073,
0.));
#74884=CARTESIAN_POINT('Ctrl Pts',(-4.51651235849824,-47.6072847024073,
20.));
#74885=CARTESIAN_POINT('Ctrl Pts',(-4.54935019567199,-47.6011331040799,
0.));
#74886=CARTESIAN_POINT('Ctrl Pts',(-4.54935019567199,-47.6011331040799,
20.));
#74887=CARTESIAN_POINT('Ctrl Pts',(-4.5821826471142,-47.5949588645311,0.));
#74888=CARTESIAN_POINT('Ctrl Pts',(-4.5821826471142,-47.5949588645311,20.));
#74889=CARTESIAN_POINT('Ctrl Pts',(-4.61500969708897,-47.5887619876026,
0.));
#74890=CARTESIAN_POINT('Ctrl Pts',(-4.61500969708897,-47.5887619876026,
20.));
#74891=CARTESIAN_POINT('Ctrl Pts',(-4.64783132986261,-47.5825424771468,
0.));
#74892=CARTESIAN_POINT('Ctrl Pts',(-4.64783132986261,-47.5825424771468,
20.));
#74893=CARTESIAN_POINT('Ctrl Pts',(-4.68064752970371,-47.5763003370265,
0.));
#74894=CARTESIAN_POINT('Ctrl Pts',(-4.68064752970371,-47.5763003370265,
20.));
#74895=CARTESIAN_POINT('Ctrl Pts',(-4.7134582808831,-47.5700355711162,0.));
#74896=CARTESIAN_POINT('Ctrl Pts',(-4.7134582808831,-47.5700355711162,20.));
#74897=CARTESIAN_POINT('Ctrl Pts',(-4.74626356767414,-47.5637481833017,
0.));
#74898=CARTESIAN_POINT('Ctrl Pts',(-4.74626356767414,-47.5637481833017,
20.));
#74899=CARTESIAN_POINT('Ctrl Pts',(-4.77906337435245,-47.5574381774801,
0.));
#74900=CARTESIAN_POINT('Ctrl Pts',(-4.77906337435245,-47.5574381774801,
20.));
#74901=CARTESIAN_POINT('Ctrl Pts',(-4.8118576851959,-47.5511055575592,0.));
#74902=CARTESIAN_POINT('Ctrl Pts',(-4.8118576851959,-47.5511055575592,20.));
#74903=CARTESIAN_POINT('Ctrl Pts',(-4.84464648448476,-47.5447503274583,
0.));
#74904=CARTESIAN_POINT('Ctrl Pts',(-4.84464648448476,-47.5447503274583,
20.));
#74905=CARTESIAN_POINT('Ctrl Pts',(-4.87742975650163,-47.538372491107,0.));
#74906=CARTESIAN_POINT('Ctrl Pts',(-4.87742975650163,-47.538372491107,20.));
#74907=CARTESIAN_POINT('Ctrl Pts',(-4.91020748553146,-47.5319720524462,
0.));
#74908=CARTESIAN_POINT('Ctrl Pts',(-4.91020748553146,-47.5319720524462,
20.));
#74909=CARTESIAN_POINT('Ctrl Pts',(-4.94297965586158,-47.5255490154281,
0.));
#74910=CARTESIAN_POINT('Ctrl Pts',(-4.94297965586158,-47.5255490154281,
20.));
#74911=CARTESIAN_POINT('Ctrl Pts',(-4.97574625178171,-47.519103384016,0.));
#74912=CARTESIAN_POINT('Ctrl Pts',(-4.97574625178171,-47.519103384016,20.));
#74913=CARTESIAN_POINT('Ctrl Pts',(-5.00850725758369,-47.5126351621839,
0.));
#74914=CARTESIAN_POINT('Ctrl Pts',(-5.00850725758369,-47.5126351621839,
20.));
#74915=CARTESIAN_POINT('Ctrl Pts',(-5.04126265756156,-47.5061443539168,
0.));
#74916=CARTESIAN_POINT('Ctrl Pts',(-5.04126265756156,-47.5061443539168,
20.));
#74917=CARTESIAN_POINT('Ctrl Pts',(-5.074012436012,-47.4996309632108,0.));
#74918=CARTESIAN_POINT('Ctrl Pts',(-5.074012436012,-47.4996309632108,20.));
#74919=CARTESIAN_POINT('Ctrl Pts',(-5.10675657723404,-47.4930949940731,
0.));
#74920=CARTESIAN_POINT('Ctrl Pts',(-5.10675657723404,-47.4930949940731,
20.));
#74921=CARTESIAN_POINT('Ctrl Pts',(-5.13949506552924,-47.4865364505219,
0.));
#74922=CARTESIAN_POINT('Ctrl Pts',(-5.13949506552924,-47.4865364505219,
20.));
#74923=CARTESIAN_POINT('Ctrl Pts',(-5.17222788520145,-47.4799553365862,
0.));
#74924=CARTESIAN_POINT('Ctrl Pts',(-5.17222788520145,-47.4799553365862,
20.));
#74925=CARTESIAN_POINT('Ctrl Pts',(-5.20495502055715,-47.4733516563069,
0.));
#74926=CARTESIAN_POINT('Ctrl Pts',(-5.20495502055715,-47.4733516563069,
20.));
#74927=CARTESIAN_POINT('Ctrl Pts',(-5.23767645590512,-47.4667254137359,
0.));
#74928=CARTESIAN_POINT('Ctrl Pts',(-5.23767645590512,-47.4667254137359,
20.));
#74929=CARTESIAN_POINT('Ctrl Pts',(-5.27039217555657,-47.4600766129357,
0.));
#74930=CARTESIAN_POINT('Ctrl Pts',(-5.27039217555657,-47.4600766129357,
20.));
#74931=CARTESIAN_POINT('Ctrl Pts',(-5.30310216382507,-47.4534052579797,
0.));
#74932=CARTESIAN_POINT('Ctrl Pts',(-5.30310216382507,-47.4534052579797,
20.));
#74933=CARTESIAN_POINT('Ctrl Pts',(-5.33580640502662,-47.4467113529523,
0.));
#74934=CARTESIAN_POINT('Ctrl Pts',(-5.33580640502662,-47.4467113529523,
20.));
#74935=CARTESIAN_POINT('Ctrl Pts',(-5.36850488347925,-47.4399949019487,
0.));
#74936=CARTESIAN_POINT('Ctrl Pts',(-5.36850488347925,-47.4399949019487,
20.));
#74937=CARTESIAN_POINT('Ctrl Pts',(-5.4011975835038,-47.4332559090748,0.));
#74938=CARTESIAN_POINT('Ctrl Pts',(-5.4011975835038,-47.4332559090748,20.));
#74939=CARTESIAN_POINT('Ctrl Pts',(-5.43388448942351,-47.4264943784481,
0.));
#74940=CARTESIAN_POINT('Ctrl Pts',(-5.43388448942351,-47.4264943784481,
20.));
#74941=CARTESIAN_POINT('Ctrl Pts',(-5.46656558556427,-47.4197103141976,
0.));
#74942=CARTESIAN_POINT('Ctrl Pts',(-5.46656558556427,-47.4197103141976,
20.));
#74943=CARTESIAN_POINT('Ctrl Pts',(-5.49924085625465,-47.4129037204631,
0.));
#74944=CARTESIAN_POINT('Ctrl Pts',(-5.49924085625465,-47.4129037204631,
20.));
#74945=CARTESIAN_POINT('Ctrl Pts',(-5.53191028582555,-47.4060746013959,
0.));
#74946=CARTESIAN_POINT('Ctrl Pts',(-5.53191028582555,-47.4060746013959,
20.));
#74947=CARTESIAN_POINT('Ctrl Pts',(-5.56457385861038,-47.3992229611579,
0.));
#74948=CARTESIAN_POINT('Ctrl Pts',(-5.56457385861038,-47.3992229611579,
20.));
#74949=CARTESIAN_POINT('Ctrl Pts',(-5.59723155894484,-47.3923488039217,
0.));
#74950=CARTESIAN_POINT('Ctrl Pts',(-5.59723155894484,-47.3923488039217,
20.));
#74951=CARTESIAN_POINT('Ctrl Pts',(-5.62988337116716,-47.3854521338708,
0.));
#74952=CARTESIAN_POINT('Ctrl Pts',(-5.62988337116716,-47.3854521338708,
20.));
#74953=CARTESIAN_POINT('Ctrl Pts',(-5.66252927961812,-47.3785329551997,
0.));
#74954=CARTESIAN_POINT('Ctrl Pts',(-5.66252927961812,-47.3785329551997,
20.));
#74955=CARTESIAN_POINT('Ctrl Pts',(-5.69516926864089,-47.3715912721141,
0.));
#74956=CARTESIAN_POINT('Ctrl Pts',(-5.69516926864089,-47.3715912721141,
20.));
#74957=CARTESIAN_POINT('Ctrl Pts',(-5.72780332258136,-47.3646270888308,
0.));
#74958=CARTESIAN_POINT('Ctrl Pts',(-5.72780332258136,-47.3646270888308,
20.));
#74959=CARTESIAN_POINT('Ctrl Pts',(-5.76043142578787,-47.3576404095777,
0.));
#74960=CARTESIAN_POINT('Ctrl Pts',(-5.76043142578787,-47.3576404095777,
20.));
#74961=CARTESIAN_POINT('Ctrl Pts',(-5.79305356261143,-47.3506312385939,
0.));
#74962=CARTESIAN_POINT('Ctrl Pts',(-5.79305356261143,-47.3506312385939,
20.));
#74963=CARTESIAN_POINT('Ctrl Pts',(-5.82566971740557,-47.3435995801292,
0.));
#74964=CARTESIAN_POINT('Ctrl Pts',(-5.82566971740557,-47.3435995801292,
20.));
#74965=CARTESIAN_POINT('Ctrl Pts',(-5.85827987452641,-47.3365454384446,
0.));
#74966=CARTESIAN_POINT('Ctrl Pts',(-5.85827987452641,-47.3365454384446,
20.));
#74967=CARTESIAN_POINT('Ctrl Pts',(-5.89088401833278,-47.3294688178121,
0.));
#74968=CARTESIAN_POINT('Ctrl Pts',(-5.89088401833278,-47.3294688178121,
20.));
#74969=CARTESIAN_POINT('Ctrl Pts',(-5.92348213318599,-47.3223697225143,
0.));
#74970=CARTESIAN_POINT('Ctrl Pts',(-5.92348213318599,-47.3223697225143,
20.));
#74971=CARTESIAN_POINT('Ctrl Pts',(-5.95607420344987,-47.3152481568452,
0.));
#74972=CARTESIAN_POINT('Ctrl Pts',(-5.95607420344987,-47.3152481568452,
20.));
#74973=CARTESIAN_POINT('Ctrl Pts',(-5.98866021349068,-47.3081041251096,
0.));
#74974=CARTESIAN_POINT('Ctrl Pts',(-5.98866021349068,-47.3081041251096,
20.));
#74975=CARTESIAN_POINT('Ctrl Pts',(-6.02124014767731,-47.3009376316237,
0.));
#74976=CARTESIAN_POINT('Ctrl Pts',(-6.02124014767731,-47.3009376316237,
20.));
#74977=CARTESIAN_POINT('Ctrl Pts',(-6.0538139903813,-47.2937486807145,0.));
#74978=CARTESIAN_POINT('Ctrl Pts',(-6.0538139903813,-47.2937486807145,20.));
#74979=CARTESIAN_POINT('Ctrl Pts',(-6.08638172597685,-47.2865372767199,
0.));
#74980=CARTESIAN_POINT('Ctrl Pts',(-6.08638172597685,-47.2865372767199,
20.));
#74981=CARTESIAN_POINT('Ctrl Pts',(-6.11894333884089,-47.2793034239892,
0.));
#74982=CARTESIAN_POINT('Ctrl Pts',(-6.11894333884089,-47.2793034239892,
20.));
#74983=CARTESIAN_POINT('Ctrl Pts',(-6.15149881335291,-47.272047126882,0.));
#74984=CARTESIAN_POINT('Ctrl Pts',(-6.15149881335291,-47.272047126882,20.));
#74985=CARTESIAN_POINT('Ctrl Pts',(-6.1840481338953,-47.2647683897693,0.));
#74986=CARTESIAN_POINT('Ctrl Pts',(-6.1840481338953,-47.2647683897693,20.));
#74987=CARTESIAN_POINT('Ctrl Pts',(-6.21659128485297,-47.2574672170331,
0.));
#74988=CARTESIAN_POINT('Ctrl Pts',(-6.21659128485297,-47.2574672170331,
20.));
#74989=CARTESIAN_POINT('Ctrl Pts',(-6.24912825061344,-47.2501436130661,
0.));
#74990=CARTESIAN_POINT('Ctrl Pts',(-6.24912825061344,-47.2501436130661,
20.));
#74991=CARTESIAN_POINT('Ctrl Pts',(-6.28165901556677,-47.2427975822723,
0.));
#74992=CARTESIAN_POINT('Ctrl Pts',(-6.28165901556677,-47.2427975822723,
20.));
#74993=CARTESIAN_POINT('Ctrl Pts',(-6.31418356410551,-47.2354291290667,
0.));
#74994=CARTESIAN_POINT('Ctrl Pts',(-6.31418356410551,-47.2354291290667,
20.));
#74995=CARTESIAN_POINT('Ctrl Pts',(-6.34670188062517,-47.2280382578755,
0.));
#74996=CARTESIAN_POINT('Ctrl Pts',(-6.34670188062517,-47.2280382578755,
20.));
#74997=CARTESIAN_POINT('Ctrl Pts',(-6.37921394952381,-47.2206249731358,
0.));
#74998=CARTESIAN_POINT('Ctrl Pts',(-6.37921394952381,-47.2206249731358,
20.));
#74999=CARTESIAN_POINT('Ctrl Pts',(-6.41171975520235,-47.213189279296,0.));
#75000=CARTESIAN_POINT('Ctrl Pts',(-6.41171975520235,-47.213189279296,20.));
#75001=CARTESIAN_POINT('Ctrl Pts',(-6.44421928206447,-47.205731180815,0.));
#75002=CARTESIAN_POINT('Ctrl Pts',(-6.44421928206447,-47.205731180815,20.));
#75003=CARTESIAN_POINT('Ctrl Pts',(-6.47671251451639,-47.1982506821625,
0.));
#75004=CARTESIAN_POINT('Ctrl Pts',(-6.47671251451639,-47.1982506821625,
20.));
#75005=CARTESIAN_POINT('Ctrl Pts',(-6.50919943696718,-47.190747787819,0.));
#75006=CARTESIAN_POINT('Ctrl Pts',(-6.50919943696718,-47.190747787819,20.));
#75007=CARTESIAN_POINT('Ctrl Pts',(-6.54168003382863,-47.1832225022762,
0.));
#75008=CARTESIAN_POINT('Ctrl Pts',(-6.54168003382863,-47.1832225022762,
20.));
#75009=CARTESIAN_POINT('Ctrl Pts',(-6.57415428951526,-47.1756748300372,
0.));
#75010=CARTESIAN_POINT('Ctrl Pts',(-6.57415428951526,-47.1756748300372,
20.));
#75011=CARTESIAN_POINT('Ctrl Pts',(-6.60662218844436,-47.168104775616,0.));
#75012=CARTESIAN_POINT('Ctrl Pts',(-6.60662218844436,-47.168104775616,20.));
#75013=CARTESIAN_POINT('Ctrl Pts',(-6.63908371503578,-47.1605123435378,
0.));
#75014=CARTESIAN_POINT('Ctrl Pts',(-6.63908371503578,-47.1605123435378,
20.));
#75015=CARTESIAN_POINT('Ctrl Pts',(-6.67153885371228,-47.1528975383387,
0.));
#75016=CARTESIAN_POINT('Ctrl Pts',(-6.67153885371228,-47.1528975383387,
20.));
#75017=CARTESIAN_POINT('Ctrl Pts',(-6.70398758889918,-47.1452603645656,
0.));
#75018=CARTESIAN_POINT('Ctrl Pts',(-6.70398758889918,-47.1452603645656,
20.));
#75019=CARTESIAN_POINT('Ctrl Pts',(-6.7364299050246,-47.1376008267758,0.));
#75020=CARTESIAN_POINT('Ctrl Pts',(-6.7364299050246,-47.1376008267758,20.));
#75021=CARTESIAN_POINT('Ctrl Pts',(-6.76886578651956,-47.129918929538,0.));
#75022=CARTESIAN_POINT('Ctrl Pts',(-6.76886578651956,-47.129918929538,20.));
#75023=CARTESIAN_POINT('Ctrl Pts',(-6.80129521781809,-47.1222146774323,
0.));
#75024=CARTESIAN_POINT('Ctrl Pts',(-6.80129521781809,-47.1222146774323,
20.));
#75025=CARTESIAN_POINT('Ctrl Pts',(-6.83371818335699,-47.1144880750497,
0.));
#75026=CARTESIAN_POINT('Ctrl Pts',(-6.83371818335699,-47.1144880750497,
20.));
#75027=CARTESIAN_POINT('Ctrl Pts',(-6.8661346675759,-47.1067391269919,0.));
#75028=CARTESIAN_POINT('Ctrl Pts',(-6.8661346675759,-47.1067391269919,20.));
#75029=CARTESIAN_POINT('Ctrl Pts',(-6.89854465491704,-47.0989678378717,
0.));
#75030=CARTESIAN_POINT('Ctrl Pts',(-6.89854465491704,-47.0989678378717,
20.));
#75031=CARTESIAN_POINT('Ctrl Pts',(-6.93094812982543,-47.0911742123123,
0.));
#75032=CARTESIAN_POINT('Ctrl Pts',(-6.93094812982543,-47.0911742123123,
20.));
#75033=CARTESIAN_POINT('Ctrl Pts',(-6.96334507674875,-47.0833582549484,
0.));
#75034=CARTESIAN_POINT('Ctrl Pts',(-6.96334507674875,-47.0833582549484,
20.));
#75035=CARTESIAN_POINT('Ctrl Pts',(-6.99573548013778,-47.0755199704256,
0.));
#75036=CARTESIAN_POINT('Ctrl Pts',(-6.99573548013778,-47.0755199704256,
20.));
#75037=CARTESIAN_POINT('Ctrl Pts',(-7.02811932444603,-47.0676593634011,
0.));
#75038=CARTESIAN_POINT('Ctrl Pts',(-7.02811932444603,-47.0676593634011,
20.));
#75039=CARTESIAN_POINT('Ctrl Pts',(-7.06049659413009,-47.0597764385426,
0.));
#75040=CARTESIAN_POINT('Ctrl Pts',(-7.06049659413009,-47.0597764385426,
20.));
#75041=CARTESIAN_POINT('Ctrl Pts',(-7.09286727364934,-47.0518712005288,
0.));
#75042=CARTESIAN_POINT('Ctrl Pts',(-7.09286727364934,-47.0518712005288,
20.));
#75043=CARTESIAN_POINT('Ctrl Pts',(-7.12523134746605,-47.0439436540493,
0.));
#75044=CARTESIAN_POINT('Ctrl Pts',(-7.12523134746605,-47.0439436540493,
20.));
#75045=CARTESIAN_POINT('Ctrl Pts',(-7.15758880004523,-47.0359938038039,
0.));
#75046=CARTESIAN_POINT('Ctrl Pts',(-7.15758880004523,-47.0359938038039,
20.));
#75047=CARTESIAN_POINT('Ctrl Pts',(-7.18993961585471,-47.0280216545038,
0.));
#75048=CARTESIAN_POINT('Ctrl Pts',(-7.18993961585471,-47.0280216545038,
20.));
#75049=CARTESIAN_POINT('Ctrl Pts',(-7.22228377936531,-47.020027210871,0.));
#75050=CARTESIAN_POINT('Ctrl Pts',(-7.22228377936531,-47.020027210871,20.));
#75051=CARTESIAN_POINT('Ctrl Pts',(-7.25462127505078,-47.012010477639,0.));
#75052=CARTESIAN_POINT('Ctrl Pts',(-7.25462127505078,-47.012010477639,20.));
#75053=CARTESIAN_POINT('Ctrl Pts',(-7.28695208738785,-47.0039714595526,
0.));
#75054=CARTESIAN_POINT('Ctrl Pts',(-7.28695208738785,-47.0039714595526,
20.));
#75055=CARTESIAN_POINT('Ctrl Pts',(-7.31927620085615,-46.9959101613675,
0.));
#75056=CARTESIAN_POINT('Ctrl Pts',(-7.31927620085615,-46.9959101613675,
20.));
#75057=CARTESIAN_POINT('Ctrl Pts',(-7.35159359993819,-46.9878265878505,
0.));
#75058=CARTESIAN_POINT('Ctrl Pts',(-7.35159359993819,-46.9878265878505,
20.));
#75059=CARTESIAN_POINT('Ctrl Pts',(-7.38390426911933,-46.9797207437786,
0.));
#75060=CARTESIAN_POINT('Ctrl Pts',(-7.38390426911933,-46.9797207437786,
20.));
#75061=CARTESIAN_POINT('Ctrl Pts',(-7.41620819288779,-46.9715926339391,
0.));
#75062=CARTESIAN_POINT('Ctrl Pts',(-7.41620819288779,-46.9715926339391,
20.));
#75063=CARTESIAN_POINT('Ctrl Pts',(-7.44850535573483,-46.9634422631307,
0.));
#75064=CARTESIAN_POINT('Ctrl Pts',(-7.44850535573483,-46.9634422631307,
20.));
#75065=CARTESIAN_POINT('Ctrl Pts',(-7.4807957421548,-46.9552696361634,0.));
#75066=CARTESIAN_POINT('Ctrl Pts',(-7.4807957421548,-46.9552696361634,20.));
#75067=CARTESIAN_POINT('Ctrl Pts',(-7.51307933664513,-46.9470747578592,
0.));
#75068=CARTESIAN_POINT('Ctrl Pts',(-7.51307933664513,-46.9470747578592,
20.));
#75069=CARTESIAN_POINT('Ctrl Pts',(-7.54535612370603,-46.9388576330501,
0.));
#75070=CARTESIAN_POINT('Ctrl Pts',(-7.54535612370603,-46.9388576330501,
20.));
#75071=CARTESIAN_POINT('Ctrl Pts',(-7.5776260878407,-46.9306182665792,0.));
#75072=CARTESIAN_POINT('Ctrl Pts',(-7.5776260878407,-46.9306182665792,20.));
#75073=CARTESIAN_POINT('Ctrl Pts',(-7.60988921355522,-46.9223566632999,
0.));
#75074=CARTESIAN_POINT('Ctrl Pts',(-7.60988921355522,-46.9223566632999,
20.));
#75075=CARTESIAN_POINT('Ctrl Pts',(-7.64214548535858,-46.9140728280766,
0.));
#75076=CARTESIAN_POINT('Ctrl Pts',(-7.64214548535858,-46.9140728280766,
20.));
#75077=CARTESIAN_POINT('Ctrl Pts',(-7.67439488776289,-46.9057667657847,
0.));
#75078=CARTESIAN_POINT('Ctrl Pts',(-7.67439488776289,-46.9057667657847,
20.));
#75079=CARTESIAN_POINT('Ctrl Pts',(-7.70663740528332,-46.8974384813109,
0.));
#75080=CARTESIAN_POINT('Ctrl Pts',(-7.70663740528332,-46.8974384813109,
20.));
#75081=CARTESIAN_POINT('Ctrl Pts',(-7.73887302243817,-46.8890879795531,
0.));
#75082=CARTESIAN_POINT('Ctrl Pts',(-7.73887302243817,-46.8890879795531,
20.));
#75083=CARTESIAN_POINT('Ctrl Pts',(-7.77110172374869,-46.8807152654198,
0.));
#75084=CARTESIAN_POINT('Ctrl Pts',(-7.77110172374869,-46.8807152654198,
20.));
#75085=CARTESIAN_POINT('Ctrl Pts',(-7.80332349373919,-46.8723203438306,
0.));
#75086=CARTESIAN_POINT('Ctrl Pts',(-7.80332349373919,-46.8723203438306,
20.));
#75087=CARTESIAN_POINT('Ctrl Pts',(-7.83553831693688,-46.8639032197162,
0.));
#75088=CARTESIAN_POINT('Ctrl Pts',(-7.83553831693688,-46.8639032197162,
20.));
#75089=CARTESIAN_POINT('Ctrl Pts',(-7.86774617787214,-46.855463898018,0.));
#75090=CARTESIAN_POINT('Ctrl Pts',(-7.86774617787214,-46.855463898018,20.));
#75091=CARTESIAN_POINT('Ctrl Pts',(-7.8999470610784,-46.8470023836881,0.));
#75092=CARTESIAN_POINT('Ctrl Pts',(-7.8999470610784,-46.8470023836881,20.));
#75093=CARTESIAN_POINT('Ctrl Pts',(-7.93214095109212,-46.8385186816898,
0.));
#75094=CARTESIAN_POINT('Ctrl Pts',(-7.93214095109212,-46.8385186816898,
20.));
#75095=CARTESIAN_POINT('Ctrl Pts',(-7.96432783245287,-46.8300127969969,
0.));
#75096=CARTESIAN_POINT('Ctrl Pts',(-7.96432783245287,-46.8300127969969,
20.));
#75097=CARTESIAN_POINT('Ctrl Pts',(-7.99650768970305,-46.8214847345942,
0.));
#75098=CARTESIAN_POINT('Ctrl Pts',(-7.99650768970305,-46.8214847345942,
20.));
#75099=CARTESIAN_POINT('Ctrl Pts',(-8.02868050738829,-46.8129344994773,
0.));
#75100=CARTESIAN_POINT('Ctrl Pts',(-8.02868050738829,-46.8129344994773,
20.));
#75101=CARTESIAN_POINT('Ctrl Pts',(-8.0608462700573,-46.8043620966531,0.));
#75102=CARTESIAN_POINT('Ctrl Pts',(-8.0608462700573,-46.8043620966531,20.));
#75103=CARTESIAN_POINT('Ctrl Pts',(-8.09300496226221,-46.7957675311395,
0.));
#75104=CARTESIAN_POINT('Ctrl Pts',(-8.09300496226221,-46.7957675311395,
20.));
#75105=CARTESIAN_POINT('Ctrl Pts',(-8.12515656855803,-46.7871508079658,
0.));
#75106=CARTESIAN_POINT('Ctrl Pts',(-8.12515656855803,-46.7871508079658,
20.));
#75107=CARTESIAN_POINT('Ctrl Pts',(-8.15730107350296,-46.7785119321719,
0.));
#75108=CARTESIAN_POINT('Ctrl Pts',(-8.15730107350296,-46.7785119321719,
20.));
#75109=CARTESIAN_POINT('Ctrl Pts',(-8.18943846165846,-46.7698509088086,
0.));
#75110=CARTESIAN_POINT('Ctrl Pts',(-8.18943846165846,-46.7698509088086,
20.));
#75111=CARTESIAN_POINT('Ctrl Pts',(-8.22156871758883,-46.7611677429374,
0.));
#75112=CARTESIAN_POINT('Ctrl Pts',(-8.22156871758883,-46.7611677429374,
20.));
#75113=CARTESIAN_POINT('Ctrl Pts',(-8.2536918258617,-46.7524624396307,0.));
#75114=CARTESIAN_POINT('Ctrl Pts',(-8.2536918258617,-46.7524624396307,20.));
#75115=CARTESIAN_POINT('Ctrl Pts',(-8.28580777104746,-46.7437350039712,
0.));
#75116=CARTESIAN_POINT('Ctrl Pts',(-8.28580777104746,-46.7437350039712,
20.));
#75117=CARTESIAN_POINT('Ctrl Pts',(-8.31791653771974,-46.7349854410525,
0.));
#75118=CARTESIAN_POINT('Ctrl Pts',(-8.31791653771974,-46.7349854410525,
20.));
#75119=CARTESIAN_POINT('Ctrl Pts',(-8.35001811045537,-46.7262137559789,
0.));
#75120=CARTESIAN_POINT('Ctrl Pts',(-8.35001811045537,-46.7262137559789,
20.));
#75121=CARTESIAN_POINT('Ctrl Pts',(-8.38211247383477,-46.7174199538668,
0.));
#75122=CARTESIAN_POINT('Ctrl Pts',(-8.38211247383477,-46.7174199538668,
20.));
#75123=CARTESIAN_POINT('Ctrl Pts',(-8.41419961244156,-46.7086040398438,
0.));
#75124=CARTESIAN_POINT('Ctrl Pts',(-8.41419961244156,-46.7086040398438,
20.));
#75125=CARTESIAN_POINT('Ctrl Pts',(-8.44627951086263,-46.6997660190488,
0.));
#75126=CARTESIAN_POINT('Ctrl Pts',(-8.44627951086263,-46.6997660190488,
20.));
#75127=CARTESIAN_POINT('Ctrl Pts',(-8.47835215368745,-46.6909058966306,
0.));
#75128=CARTESIAN_POINT('Ctrl Pts',(-8.47835215368745,-46.6909058966306,
20.));
#75129=CARTESIAN_POINT('Ctrl Pts',(-8.51041752550882,-46.6820236777489,
0.));
#75130=CARTESIAN_POINT('Ctrl Pts',(-8.51041752550882,-46.6820236777489,
20.));
#75131=CARTESIAN_POINT('Ctrl Pts',(-8.54247561092259,-46.673119367573,0.));
#75132=CARTESIAN_POINT('Ctrl Pts',(-8.54247561092259,-46.673119367573,20.));
#75133=CARTESIAN_POINT('Ctrl Pts',(-8.57452639452829,-46.6641929712839,
0.));
#75134=CARTESIAN_POINT('Ctrl Pts',(-8.57452639452829,-46.6641929712839,
20.));
#75135=CARTESIAN_POINT('Ctrl Pts',(-8.60656986092879,-46.6552444940739,
0.));
#75136=CARTESIAN_POINT('Ctrl Pts',(-8.60656986092879,-46.6552444940739,
20.));
#75137=CARTESIAN_POINT('Ctrl Pts',(-8.63860599473004,-46.6462739411471,
0.));
#75138=CARTESIAN_POINT('Ctrl Pts',(-8.63860599473004,-46.6462739411471,
20.));
#75139=CARTESIAN_POINT('Ctrl Pts',(-8.67063478054117,-46.6372813177181,
0.));
#75140=CARTESIAN_POINT('Ctrl Pts',(-8.67063478054117,-46.6372813177181,
20.));
#75141=CARTESIAN_POINT('Ctrl Pts',(-8.70265620297455,-46.6282666290119,
0.));
#75142=CARTESIAN_POINT('Ctrl Pts',(-8.70265620297455,-46.6282666290119,
20.));
#75143=CARTESIAN_POINT('Ctrl Pts',(-8.73467024664571,-46.6192298802645,
0.));
#75144=CARTESIAN_POINT('Ctrl Pts',(-8.73467024664571,-46.6192298802645,
20.));
#75145=CARTESIAN_POINT('Ctrl Pts',(-8.76667689617331,-46.6101710767218,
0.));
#75146=CARTESIAN_POINT('Ctrl Pts',(-8.76667689617331,-46.6101710767218,
20.));
#75147=CARTESIAN_POINT('Ctrl Pts',(-8.79867613617934,-46.6010902236408,
0.));
#75148=CARTESIAN_POINT('Ctrl Pts',(-8.79867613617934,-46.6010902236408,
20.));
#75149=CARTESIAN_POINT('Ctrl Pts',(-8.83066795128935,-46.59198732629,0.));
#75150=CARTESIAN_POINT('Ctrl Pts',(-8.83066795128935,-46.59198732629,20.));
#75151=CARTESIAN_POINT('Ctrl Pts',(-8.86265232613216,-46.582862389949,0.));
#75152=CARTESIAN_POINT('Ctrl Pts',(-8.86265232613216,-46.582862389949,20.));
#75153=CARTESIAN_POINT('Ctrl Pts',(-8.8946292453399,-46.5737154199087,0.));
#75154=CARTESIAN_POINT('Ctrl Pts',(-8.8946292453399,-46.5737154199087,20.));
#75155=CARTESIAN_POINT('Ctrl Pts',(-8.92659869354789,-46.5645464214705,
0.));
#75156=CARTESIAN_POINT('Ctrl Pts',(-8.92659869354789,-46.5645464214705,
20.));
#75157=CARTESIAN_POINT('Ctrl Pts',(-8.95856065539471,-46.5553553999467,
0.));
#75158=CARTESIAN_POINT('Ctrl Pts',(-8.95856065539471,-46.5553553999467,
20.));
#75159=CARTESIAN_POINT('Ctrl Pts',(-8.9905151155223,-46.5461423606602,0.));
#75160=CARTESIAN_POINT('Ctrl Pts',(-8.9905151155223,-46.5461423606602,20.));
#75161=CARTESIAN_POINT('Ctrl Pts',(-9.02246205857629,-46.5369073089453,
0.));
#75162=CARTESIAN_POINT('Ctrl Pts',(-9.02246205857629,-46.5369073089453,
20.));
#75163=CARTESIAN_POINT('Ctrl Pts',(-9.05440146920516,-46.5276502501459,
0.));
#75164=CARTESIAN_POINT('Ctrl Pts',(-9.05440146920516,-46.5276502501459,
20.));
#75165=CARTESIAN_POINT('Ctrl Pts',(-9.08633333206091,-46.5183711896174,
0.));
#75166=CARTESIAN_POINT('Ctrl Pts',(-9.08633333206091,-46.5183711896174,
20.));
#75167=CARTESIAN_POINT('Ctrl Pts',(-9.11825763179854,-46.5090701327255,
0.));
#75168=CARTESIAN_POINT('Ctrl Pts',(-9.11825763179854,-46.5090701327255,
20.));
#75169=CARTESIAN_POINT('Ctrl Pts',(-9.15017435307667,-46.4997470848477,
0.));
#75170=CARTESIAN_POINT('Ctrl Pts',(-9.15017435307667,-46.4997470848477,
20.));
#75171=CARTESIAN_POINT('Ctrl Pts',(-9.18208348055726,-46.4904020513722,
0.));
#75172=CARTESIAN_POINT('Ctrl Pts',(-9.18208348055726,-46.4904020513722,
20.));
#75173=CARTESIAN_POINT('Ctrl Pts',(-9.21398499890594,-46.4810350376983,
0.));
#75174=CARTESIAN_POINT('Ctrl Pts',(-9.21398499890594,-46.4810350376983,
20.));
#75175=CARTESIAN_POINT('Ctrl Pts',(-9.24587889279172,-46.4716460492361,
0.));
#75176=CARTESIAN_POINT('Ctrl Pts',(-9.24587889279172,-46.4716460492361,
20.));
#75177=CARTESIAN_POINT('Ctrl Pts',(-9.277765146887,-46.4622350914066,0.));
#75178=CARTESIAN_POINT('Ctrl Pts',(-9.277765146887,-46.4622350914066,20.));
#75179=CARTESIAN_POINT('Ctrl Pts',(-9.30964374586753,-46.4528021696416,
0.));
#75180=CARTESIAN_POINT('Ctrl Pts',(-9.30964374586753,-46.4528021696416,
20.));
#75181=CARTESIAN_POINT('Ctrl Pts',(-9.34151467441242,-46.4433472893837,
0.));
#75182=CARTESIAN_POINT('Ctrl Pts',(-9.34151467441242,-46.4433472893837,
20.));
#75183=CARTESIAN_POINT('Ctrl Pts',(-9.37337791720394,-46.4338704560856,
0.));
#75184=CARTESIAN_POINT('Ctrl Pts',(-9.37337791720394,-46.4338704560856,
20.));
#75185=CARTESIAN_POINT('Ctrl Pts',(-9.40523345892774,-46.4243716752115,
0.));
#75186=CARTESIAN_POINT('Ctrl Pts',(-9.40523345892774,-46.4243716752115,
20.));
#75187=CARTESIAN_POINT('Ctrl Pts',(-9.43708128427275,-46.4148509522358,
0.));
#75188=CARTESIAN_POINT('Ctrl Pts',(-9.43708128427275,-46.4148509522358,
20.));
#75189=CARTESIAN_POINT('Ctrl Pts',(-9.46892137793149,-46.405308292644,0.));
#75190=CARTESIAN_POINT('Ctrl Pts',(-9.46892137793149,-46.405308292644,20.));
#75191=CARTESIAN_POINT('Ctrl Pts',(-9.5007537246001,-46.3957437019326,0.));
#75192=CARTESIAN_POINT('Ctrl Pts',(-9.5007537246001,-46.3957437019326,20.));
#75193=CARTESIAN_POINT('Ctrl Pts',(-9.53257830897852,-46.3861571856095,
0.));
#75194=CARTESIAN_POINT('Ctrl Pts',(-9.53257830897852,-46.3861571856095,
20.));
#75195=CARTESIAN_POINT('Ctrl Pts',(-9.56439511577024,-46.3765487491938,
0.));
#75196=CARTESIAN_POINT('Ctrl Pts',(-9.56439511577024,-46.3765487491938,
20.));
#75197=CARTESIAN_POINT('Ctrl Pts',(-9.59620412968214,-46.3669183982155,
0.));
#75198=CARTESIAN_POINT('Ctrl Pts',(-9.59620412968214,-46.3669183982155,
20.));
#75199=CARTESIAN_POINT('Ctrl Pts',(-9.62800533542437,-46.3572661382147,
0.));
#75200=CARTESIAN_POINT('Ctrl Pts',(-9.62800533542437,-46.3572661382147,
20.));
#75201=CARTESIAN_POINT('Ctrl Pts',(-9.6597987177104,-46.347591974742,0.));
#75202=CARTESIAN_POINT('Ctrl Pts',(-9.6597987177104,-46.347591974742,20.));
#75203=CARTESIAN_POINT('Ctrl Pts',(-9.69158426125693,-46.3378959133587,
0.));
#75204=CARTESIAN_POINT('Ctrl Pts',(-9.69158426125693,-46.3378959133587,
20.));
#75205=CARTESIAN_POINT('Ctrl Pts',(-9.72336195078415,-46.3281779596367,
0.));
#75206=CARTESIAN_POINT('Ctrl Pts',(-9.72336195078415,-46.3281779596367,
20.));
#75207=CARTESIAN_POINT('Ctrl Pts',(-9.75513177101578,-46.3184381191592,
0.));
#75208=CARTESIAN_POINT('Ctrl Pts',(-9.75513177101578,-46.3184381191592,
20.));
#75209=CARTESIAN_POINT('Ctrl Pts',(-9.78689370667941,-46.3086763975205,
0.));
#75210=CARTESIAN_POINT('Ctrl Pts',(-9.78689370667941,-46.3086763975205,
20.));
#75211=CARTESIAN_POINT('Ctrl Pts',(-9.8186477425062,-46.2988928003257,0.));
#75212=CARTESIAN_POINT('Ctrl Pts',(-9.8186477425062,-46.2988928003257,20.));
#75213=CARTESIAN_POINT('Ctrl Pts',(-9.85039386323086,-46.289087333191,0.));
#75214=CARTESIAN_POINT('Ctrl Pts',(-9.85039386323086,-46.289087333191,20.));
#75215=CARTESIAN_POINT('Ctrl Pts',(-9.88213205359192,-46.2792600017436,
0.));
#75216=CARTESIAN_POINT('Ctrl Pts',(-9.88213205359192,-46.2792600017436,
20.));
#75217=CARTESIAN_POINT('Ctrl Pts',(-9.91386229833138,-46.2694108116213,
0.));
#75218=CARTESIAN_POINT('Ctrl Pts',(-9.91386229833138,-46.2694108116213,
20.));
#75219=CARTESIAN_POINT('Ctrl Pts',(-9.94558458219447,-46.2595397684724,
0.));
#75220=CARTESIAN_POINT('Ctrl Pts',(-9.94558458219447,-46.2595397684724,
20.));
#75221=CARTESIAN_POINT('Ctrl Pts',(-9.97729888992981,-46.2496468779557,
0.));
#75222=CARTESIAN_POINT('Ctrl Pts',(-9.97729888992981,-46.2496468779557,
20.));
#75223=CARTESIAN_POINT('Ctrl Pts',(-10.0090052062895,-46.2397321457408,
0.));
#75224=CARTESIAN_POINT('Ctrl Pts',(-10.0090052062895,-46.2397321457408,
20.));
#75225=CARTESIAN_POINT('Ctrl Pts',(-10.0407035160293,-46.2297955775084,
0.));
#75226=CARTESIAN_POINT('Ctrl Pts',(-10.0407035160293,-46.2297955775084,
20.));
#75227=CARTESIAN_POINT('Ctrl Pts',(-10.0723938039086,-46.2198371789501,
0.));
#75228=CARTESIAN_POINT('Ctrl Pts',(-10.0723938039086,-46.2198371789501,
20.));
#75229=CARTESIAN_POINT('Ctrl Pts',(-10.1040760546909,-46.2098569557688,
0.));
#75230=CARTESIAN_POINT('Ctrl Pts',(-10.1040760546909,-46.2098569557688,
20.));
#75231=CARTESIAN_POINT('Ctrl Pts',(-10.1357502531431,-46.1998549136779,
0.));
#75232=CARTESIAN_POINT('Ctrl Pts',(-10.1357502531431,-46.1998549136779,
20.));
#75233=CARTESIAN_POINT('Ctrl Pts',(-10.1674163840354,-46.1898310584014,
0.));
#75234=CARTESIAN_POINT('Ctrl Pts',(-10.1674163840354,-46.1898310584014,
20.));
#75235=CARTESIAN_POINT('Ctrl Pts',(-10.199074432142,-46.179785395674,0.));
#75236=CARTESIAN_POINT('Ctrl Pts',(-10.199074432142,-46.179785395674,20.));
#75237=CARTESIAN_POINT('Ctrl Pts',(-10.2307243822402,-46.169717931241,0.));
#75238=CARTESIAN_POINT('Ctrl Pts',(-10.2307243822402,-46.169717931241,20.));
#75239=CARTESIAN_POINT('Ctrl Pts',(-10.2623662191114,-46.1596286708586,
0.));
#75240=CARTESIAN_POINT('Ctrl Pts',(-10.2623662191114,-46.1596286708586,
20.));
#75241=CARTESIAN_POINT('Ctrl Pts',(-10.2939999275403,-46.1495176202946,
0.));
#75242=CARTESIAN_POINT('Ctrl Pts',(-10.2939999275403,-46.1495176202946,
20.));
#75243=CARTESIAN_POINT('Ctrl Pts',(-10.3256254923156,-46.139384785327,0.));
#75244=CARTESIAN_POINT('Ctrl Pts',(-10.3256254923156,-46.139384785327,20.));
#75245=CARTESIAN_POINT('Ctrl Pts',(-10.3572428982293,-46.1292301717445,
0.));
#75246=CARTESIAN_POINT('Ctrl Pts',(-10.3572428982293,-46.1292301717445,
20.));
#75247=CARTESIAN_POINT('Ctrl Pts',(-10.3888521300774,-46.119053785347,0.));
#75248=CARTESIAN_POINT('Ctrl Pts',(-10.3888521300774,-46.119053785347,20.));
#75249=CARTESIAN_POINT('Ctrl Pts',(-10.4204531726593,-46.1088556319449,
0.));
#75250=CARTESIAN_POINT('Ctrl Pts',(-10.4204531726593,-46.1088556319449,
20.));
#75251=CARTESIAN_POINT('Ctrl Pts',(-10.4520460107784,-46.0986357173598,
0.));
#75252=CARTESIAN_POINT('Ctrl Pts',(-10.4520460107784,-46.0986357173598,
20.));
#75253=CARTESIAN_POINT('Ctrl Pts',(-10.4836306292415,-46.0883940474237,
0.));
#75254=CARTESIAN_POINT('Ctrl Pts',(-10.4836306292415,-46.0883940474237,
20.));
#75255=CARTESIAN_POINT('Ctrl Pts',(-10.5152070128593,-46.0781306279792,
0.));
#75256=CARTESIAN_POINT('Ctrl Pts',(-10.5152070128593,-46.0781306279792,
20.));
#75257=CARTESIAN_POINT('Ctrl Pts',(-10.5467751464457,-46.0678454648793,
0.));
#75258=CARTESIAN_POINT('Ctrl Pts',(-10.5467751464457,-46.0678454648793,
20.));
#75259=CARTESIAN_POINT('Ctrl Pts',(-10.5783350148188,-46.0575385639878,
0.));
#75260=CARTESIAN_POINT('Ctrl Pts',(-10.5783350148188,-46.0575385639878,
20.));
#75261=CARTESIAN_POINT('Ctrl Pts',(-10.6098866028001,-46.0472099311799,
0.));
#75262=CARTESIAN_POINT('Ctrl Pts',(-10.6098866028001,-46.0472099311799,
20.));
#75263=CARTESIAN_POINT('Ctrl Pts',(-10.6414298952151,-46.0368595723418,
0.));
#75264=CARTESIAN_POINT('Ctrl Pts',(-10.6414298952151,-46.0368595723418,
20.));
#75265=CARTESIAN_POINT('Ctrl Pts',(-10.6729648768932,-46.0264874933706,
0.));
#75266=CARTESIAN_POINT('Ctrl Pts',(-10.6729648768932,-46.0264874933706,
20.));
#75267=CARTESIAN_POINT('Ctrl Pts',(-10.7044915326674,-46.0160937001747,
0.));
#75268=CARTESIAN_POINT('Ctrl Pts',(-10.7044915326674,-46.0160937001747,
20.));
#75269=CARTESIAN_POINT('Ctrl Pts',(-10.7360098473747,-46.0056781986726,
0.));
#75270=CARTESIAN_POINT('Ctrl Pts',(-10.7360098473747,-46.0056781986726,
20.));
#75271=CARTESIAN_POINT('Ctrl Pts',(-10.7675198058554,-45.9952409947932,
0.));
#75272=CARTESIAN_POINT('Ctrl Pts',(-10.7675198058554,-45.9952409947932,
20.));
#75273=CARTESIAN_POINT('Ctrl Pts',(-10.7990213929536,-45.9847820944759,
0.));
#75274=CARTESIAN_POINT('Ctrl Pts',(-10.7990213929536,-45.9847820944759,
20.));
#75275=CARTESIAN_POINT('Ctrl Pts',(-10.8305145935168,-45.9743015036702,
0.));
#75276=CARTESIAN_POINT('Ctrl Pts',(-10.8305145935168,-45.9743015036702,
20.));
#75277=CARTESIAN_POINT('Ctrl Pts',(-10.8619993923967,-45.9637992283368,
0.));
#75278=CARTESIAN_POINT('Ctrl Pts',(-10.8619993923967,-45.9637992283368,
20.));
#75279=CARTESIAN_POINT('Ctrl Pts',(-10.8934757744485,-45.9532752744476,
0.));
#75280=CARTESIAN_POINT('Ctrl Pts',(-10.8934757744485,-45.9532752744476,
20.));
#75281=CARTESIAN_POINT('Ctrl Pts',(-10.9249437245321,-45.9427296479861,
0.));
#75282=CARTESIAN_POINT('Ctrl Pts',(-10.9249437245321,-45.9427296479861,
20.));
#75283=CARTESIAN_POINT('Ctrl Pts',(-10.9564032275107,-45.9321623549466,
0.));
#75284=CARTESIAN_POINT('Ctrl Pts',(-10.9564032275107,-45.9321623549466,
20.));
#75285=CARTESIAN_POINT('Ctrl Pts',(-10.9878542682513,-45.9215734013338,
0.));
#75286=CARTESIAN_POINT('Ctrl Pts',(-10.9878542682513,-45.9215734013338,
20.));
#75287=CARTESIAN_POINT('Ctrl Pts',(-11.0192968316247,-45.9109627931629,
0.));
#75288=CARTESIAN_POINT('Ctrl Pts',(-11.0192968316247,-45.9109627931629,
20.));
#75289=CARTESIAN_POINT('Ctrl Pts',(-11.0507309025053,-45.9003305364593,
0.));
#75290=CARTESIAN_POINT('Ctrl Pts',(-11.0507309025053,-45.9003305364593,
20.));
#75291=CARTESIAN_POINT('Ctrl Pts',(-11.0821564657716,-45.8896766372596,
0.));
#75292=CARTESIAN_POINT('Ctrl Pts',(-11.0821564657716,-45.8896766372596,
20.));
#75293=CARTESIAN_POINT('Ctrl Pts',(-11.1135735063059,-45.8790011016108,
0.));
#75294=CARTESIAN_POINT('Ctrl Pts',(-11.1135735063059,-45.8790011016108,
20.));
#75295=CARTESIAN_POINT('Ctrl Pts',(-11.1449820089942,-45.868303935571,0.));
#75296=CARTESIAN_POINT('Ctrl Pts',(-11.1449820089942,-45.868303935571,20.));
#75297=CARTESIAN_POINT('Ctrl Pts',(-11.1763819587263,-45.8575851452088,
0.));
#75298=CARTESIAN_POINT('Ctrl Pts',(-11.1763819587263,-45.8575851452088,
20.));
#75299=CARTESIAN_POINT('Ctrl Pts',(-11.207773340396,-45.8468447366038,0.));
#75300=CARTESIAN_POINT('Ctrl Pts',(-11.207773340396,-45.8468447366038,20.));
#75301=CARTESIAN_POINT('Ctrl Pts',(-11.2391561389011,-45.8360827158468,
0.));
#75302=CARTESIAN_POINT('Ctrl Pts',(-11.2391561389011,-45.8360827158468,
20.));
#75303=CARTESIAN_POINT('Ctrl Pts',(-11.2705303391434,-45.8252990890386,
0.));
#75304=CARTESIAN_POINT('Ctrl Pts',(-11.2705303391434,-45.8252990890386,
20.));
#75305=CARTESIAN_POINT('Ctrl Pts',(-11.3018959260283,-45.8144938622913,
0.));
#75306=CARTESIAN_POINT('Ctrl Pts',(-11.3018959260283,-45.8144938622913,
20.));
#75307=CARTESIAN_POINT('Ctrl Pts',(-11.3332528844652,-45.8036670417272,
0.));
#75308=CARTESIAN_POINT('Ctrl Pts',(-11.3332528844652,-45.8036670417272,
20.));
#75309=CARTESIAN_POINT('Ctrl Pts',(-11.3646011993674,-45.7928186334791,
0.));
#75310=CARTESIAN_POINT('Ctrl Pts',(-11.3646011993674,-45.7928186334791,
20.));
#75311=CARTESIAN_POINT('Ctrl Pts',(-11.395940855652,-45.7819486436912,0.));
#75312=CARTESIAN_POINT('Ctrl Pts',(-11.395940855652,-45.7819486436912,20.));
#75313=CARTESIAN_POINT('Ctrl Pts',(-11.4272718382404,-45.7710570785186,
0.));
#75314=CARTESIAN_POINT('Ctrl Pts',(-11.4272718382404,-45.7710570785186,
20.));
#75315=CARTESIAN_POINT('Ctrl Pts',(-11.4585941320575,-45.760143944127,0.));
#75316=CARTESIAN_POINT('Ctrl Pts',(-11.4585941320575,-45.760143944127,20.));
#75317=CARTESIAN_POINT('Ctrl Pts',(-11.489907722032,-45.7492092466918,0.));
#75318=CARTESIAN_POINT('Ctrl Pts',(-11.489907722032,-45.7492092466918,20.));
#75319=CARTESIAN_POINT('Ctrl Pts',(-11.5212125930967,-45.7382529923996,
0.));
#75320=CARTESIAN_POINT('Ctrl Pts',(-11.5212125930967,-45.7382529923996,
20.));
#75321=CARTESIAN_POINT('Ctrl Pts',(-11.5525087301884,-45.7272751874478,
0.));
#75322=CARTESIAN_POINT('Ctrl Pts',(-11.5525087301884,-45.7272751874478,
20.));
#75323=CARTESIAN_POINT('Ctrl Pts',(-11.5837961182482,-45.7162758380449,
0.));
#75324=CARTESIAN_POINT('Ctrl Pts',(-11.5837961182482,-45.7162758380449,
20.));
#75325=CARTESIAN_POINT('Ctrl Pts',(-11.615074742221,-45.7052549504103,0.));
#75326=CARTESIAN_POINT('Ctrl Pts',(-11.615074742221,-45.7052549504103,20.));
#75327=CARTESIAN_POINT('Ctrl Pts',(-11.6463445870557,-45.694212530774,0.));
#75328=CARTESIAN_POINT('Ctrl Pts',(-11.6463445870557,-45.694212530774,20.));
#75329=CARTESIAN_POINT('Ctrl Pts',(-11.6776056377055,-45.6831485853771,
0.));
#75330=CARTESIAN_POINT('Ctrl Pts',(-11.6776056377055,-45.6831485853771,
20.));
#75331=CARTESIAN_POINT('Ctrl Pts',(-11.7088578791267,-45.6720631204703,
0.));
#75332=CARTESIAN_POINT('Ctrl Pts',(-11.7088578791267,-45.6720631204703,
20.));
#75333=CARTESIAN_POINT('Ctrl Pts',(-11.7401012962797,-45.6609561423149,
0.));
#75334=CARTESIAN_POINT('Ctrl Pts',(-11.7401012962797,-45.6609561423149,
20.));
#75335=CARTESIAN_POINT('Ctrl Pts',(-11.7713358741293,-45.6498276571829,
0.));
#75336=CARTESIAN_POINT('Ctrl Pts',(-11.7713358741293,-45.6498276571829,
20.));
#75337=CARTESIAN_POINT('Ctrl Pts',(-11.8025615976441,-45.6386776713575,
0.));
#75338=CARTESIAN_POINT('Ctrl Pts',(-11.8025615976441,-45.6386776713575,
20.));
#75339=CARTESIAN_POINT('Ctrl Pts',(-11.8337784517972,-45.627506191133,0.));
#75340=CARTESIAN_POINT('Ctrl Pts',(-11.8337784517972,-45.627506191133,20.));
#75341=CARTESIAN_POINT('Ctrl Pts',(-11.8649864215653,-45.6163132228138,
0.));
#75342=CARTESIAN_POINT('Ctrl Pts',(-11.8649864215653,-45.6163132228138,
20.));
#75343=CARTESIAN_POINT('Ctrl Pts',(-11.8961854919294,-45.6050987727153,
0.));
#75344=CARTESIAN_POINT('Ctrl Pts',(-11.8961854919294,-45.6050987727153,
20.));
#75345=CARTESIAN_POINT('Ctrl Pts',(-11.9273756478741,-45.5938628471638,
0.));
#75346=CARTESIAN_POINT('Ctrl Pts',(-11.9273756478741,-45.5938628471638,
20.));
#75347=CARTESIAN_POINT('Ctrl Pts',(-11.9585568743886,-45.5826054524963,
0.));
#75348=CARTESIAN_POINT('Ctrl Pts',(-11.9585568743886,-45.5826054524963,
20.));
#75349=CARTESIAN_POINT('Ctrl Pts',(-11.989729156466,-45.5713265950605,0.));
#75350=CARTESIAN_POINT('Ctrl Pts',(-11.989729156466,-45.5713265950605,20.));
#75351=CARTESIAN_POINT('Ctrl Pts',(-12.0208924791035,-45.5600262812144,
0.));
#75352=CARTESIAN_POINT('Ctrl Pts',(-12.0208924791035,-45.5600262812144,
20.));
#75353=CARTESIAN_POINT('Ctrl Pts',(-12.0520468273019,-45.5487045173265,
0.));
#75354=CARTESIAN_POINT('Ctrl Pts',(-12.0520468273019,-45.5487045173265,
20.));
#75355=CARTESIAN_POINT('Ctrl Pts',(-12.0831921860666,-45.5373613097755,
0.));
#75356=CARTESIAN_POINT('Ctrl Pts',(-12.0831921860666,-45.5373613097755,
20.));
#75357=CARTESIAN_POINT('Ctrl Pts',(-12.1143285404065,-45.5259966649516,
0.));
#75358=CARTESIAN_POINT('Ctrl Pts',(-12.1143285404065,-45.5259966649516,
20.));
#75359=CARTESIAN_POINT('Ctrl Pts',(-12.1454558753351,-45.5146105892553,
0.));
#75360=CARTESIAN_POINT('Ctrl Pts',(-12.1454558753351,-45.5146105892553,
20.));
#75361=CARTESIAN_POINT('Ctrl Pts',(-12.1765741758697,-45.5032030890978,
0.));
#75362=CARTESIAN_POINT('Ctrl Pts',(-12.1765741758697,-45.5032030890978,
20.));
#75363=CARTESIAN_POINT('Ctrl Pts',(-12.2076834270323,-45.4917741709015,
0.));
#75364=CARTESIAN_POINT('Ctrl Pts',(-12.2076834270323,-45.4917741709015,
20.));
#75365=CARTESIAN_POINT('Ctrl Pts',(-12.2387836138487,-45.4803238410999,
0.));
#75366=CARTESIAN_POINT('Ctrl Pts',(-12.2387836138487,-45.4803238410999,
20.));
#75367=CARTESIAN_POINT('Ctrl Pts',(-12.269874721349,-45.4688521061371,0.));
#75368=CARTESIAN_POINT('Ctrl Pts',(-12.269874721349,-45.4688521061371,20.));
#75369=CARTESIAN_POINT('Ctrl Pts',(-12.3009567345673,-45.4573589724673,
0.));
#75370=CARTESIAN_POINT('Ctrl Pts',(-12.3009567345673,-45.4573589724673,
20.));
#75371=CARTESIAN_POINT('Ctrl Pts',(-12.3320296385418,-45.4458444465552,
0.));
#75372=CARTESIAN_POINT('Ctrl Pts',(-12.3320296385418,-45.4458444465552,
20.));
#75373=CARTESIAN_POINT('Ctrl Pts',(-12.3630934183143,-45.4343085348755,
0.));
#75374=CARTESIAN_POINT('Ctrl Pts',(-12.3630934183143,-45.4343085348755,
20.));
#75375=CARTESIAN_POINT('Ctrl Pts',(-12.3941480589311,-45.4227512439136,
0.));
#75376=CARTESIAN_POINT('Ctrl Pts',(-12.3941480589311,-45.4227512439136,
20.));
#75377=CARTESIAN_POINT('Ctrl Pts',(-12.4251935454428,-45.4111725801659,
0.));
#75378=CARTESIAN_POINT('Ctrl Pts',(-12.4251935454428,-45.4111725801659,
20.));
#75379=CARTESIAN_POINT('Ctrl Pts',(-12.4562298629045,-45.3995725501402,
0.));
#75380=CARTESIAN_POINT('Ctrl Pts',(-12.4562298629045,-45.3995725501402,
20.));
#75381=CARTESIAN_POINT('Ctrl Pts',(-12.4872569963754,-45.3879511603549,
0.));
#75382=CARTESIAN_POINT('Ctrl Pts',(-12.4872569963754,-45.3879511603549,
20.));
#75383=CARTESIAN_POINT('Ctrl Pts',(-12.5182749309189,-45.376308417339,0.));
#75384=CARTESIAN_POINT('Ctrl Pts',(-12.5182749309189,-45.376308417339,20.));
#75385=CARTESIAN_POINT('Ctrl Pts',(-12.5492836516023,-45.364644327632,0.));
#75386=CARTESIAN_POINT('Ctrl Pts',(-12.5492836516023,-45.364644327632,20.));
#75387=CARTESIAN_POINT('Ctrl Pts',(-12.5802831434966,-45.3529588977839,
0.));
#75388=CARTESIAN_POINT('Ctrl Pts',(-12.5802831434966,-45.3529588977839,
20.));
#75389=CARTESIAN_POINT('Ctrl Pts',(-12.6112733916776,-45.3412521343551,
0.));
#75390=CARTESIAN_POINT('Ctrl Pts',(-12.6112733916776,-45.3412521343551,
20.));
#75391=CARTESIAN_POINT('Ctrl Pts',(-12.6422543812252,-45.3295240439169,
0.));
#75392=CARTESIAN_POINT('Ctrl Pts',(-12.6422543812252,-45.3295240439169,
20.));
#75393=CARTESIAN_POINT('Ctrl Pts',(-12.6732260972239,-45.3177746330512,
0.));
#75394=CARTESIAN_POINT('Ctrl Pts',(-12.6732260972239,-45.3177746330512,
20.));
#75395=CARTESIAN_POINT('Ctrl Pts',(-12.7041885247626,-45.3060039083501,
0.));
#75396=CARTESIAN_POINT('Ctrl Pts',(-12.7041885247626,-45.3060039083501,
20.));
#75397=CARTESIAN_POINT('Ctrl Pts',(-12.7351416489341,-45.2942118764167,
0.));
#75398=CARTESIAN_POINT('Ctrl Pts',(-12.7351416489341,-45.2942118764167,
20.));
#75399=CARTESIAN_POINT('Ctrl Pts',(-12.7660854548354,-45.2823985438647,
0.));
#75400=CARTESIAN_POINT('Ctrl Pts',(-12.7660854548354,-45.2823985438647,
20.));
#75401=CARTESIAN_POINT('Ctrl Pts',(-12.7970199275678,-45.2705639173192,
0.));
#75402=CARTESIAN_POINT('Ctrl Pts',(-12.7970199275678,-45.2705639173192,
20.));
#75403=CARTESIAN_POINT('Ctrl Pts',(-12.8279450522366,-45.2587080034157,
0.));
#75404=CARTESIAN_POINT('Ctrl Pts',(-12.8279450522366,-45.2587080034157,
20.));
#75405=CARTESIAN_POINT('Ctrl Pts',(-12.8588608139512,-45.2468308087994,
0.));
#75406=CARTESIAN_POINT('Ctrl Pts',(-12.8588608139512,-45.2468308087994,
20.));
#75407=CARTESIAN_POINT('Ctrl Pts',(-12.8897671978257,-45.2349323401259,
0.));
#75408=CARTESIAN_POINT('Ctrl Pts',(-12.8897671978257,-45.2349323401259,
20.));
#75409=CARTESIAN_POINT('Ctrl Pts',(-12.9206641889781,-45.2230126040617,
0.));
#75410=CARTESIAN_POINT('Ctrl Pts',(-12.9206641889781,-45.2230126040617,
20.));
#75411=CARTESIAN_POINT('Ctrl Pts',(-12.9515517725313,-45.2110716072841,
0.));
#75412=CARTESIAN_POINT('Ctrl Pts',(-12.9515517725313,-45.2110716072841,
20.));
#75413=CARTESIAN_POINT('Ctrl Pts',(-12.9824299336127,-45.199109356482,0.));
#75414=CARTESIAN_POINT('Ctrl Pts',(-12.9824299336127,-45.199109356482,20.));
#75415=CARTESIAN_POINT('Ctrl Pts',(-13.0132986573536,-45.1871258583545,
0.));
#75416=CARTESIAN_POINT('Ctrl Pts',(-13.0132986573536,-45.1871258583545,
20.));
#75417=CARTESIAN_POINT('Ctrl Pts',(-13.0441579288899,-45.1751211196118,
0.));
#75418=CARTESIAN_POINT('Ctrl Pts',(-13.0441579288899,-45.1751211196118,
20.));
#75419=CARTESIAN_POINT('Ctrl Pts',(-13.0750077333614,-45.1630951469733,
0.));
#75420=CARTESIAN_POINT('Ctrl Pts',(-13.0750077333614,-45.1630951469733,
20.));
#75421=CARTESIAN_POINT('Ctrl Pts',(-13.1058480559121,-45.1510479471692,
0.));
#75422=CARTESIAN_POINT('Ctrl Pts',(-13.1058480559121,-45.1510479471692,
20.));
#75423=CARTESIAN_POINT('Ctrl Pts',(-13.1366788816904,-45.1389795269399,
0.));
#75424=CARTESIAN_POINT('Ctrl Pts',(-13.1366788816904,-45.1389795269399,
20.));
#75425=CARTESIAN_POINT('Ctrl Pts',(-13.1675001958493,-45.1268898930368,
0.));
#75426=CARTESIAN_POINT('Ctrl Pts',(-13.1675001958493,-45.1268898930368,
20.));
#75427=CARTESIAN_POINT('Ctrl Pts',(-13.198311983546,-45.114779052223,0.));
#75428=CARTESIAN_POINT('Ctrl Pts',(-13.198311983546,-45.114779052223,20.));
#75429=CARTESIAN_POINT('Ctrl Pts',(-13.2291142299426,-45.1026470112717,
0.));
#75430=CARTESIAN_POINT('Ctrl Pts',(-13.2291142299426,-45.1026470112717,
20.));
#75431=CARTESIAN_POINT('Ctrl Pts',(-13.259906920205,-45.0904937769663,0.));
#75432=CARTESIAN_POINT('Ctrl Pts',(-13.259906920205,-45.0904937769663,20.));
#75433=CARTESIAN_POINT('Ctrl Pts',(-13.2906900395037,-45.0783193561008,
0.));
#75434=CARTESIAN_POINT('Ctrl Pts',(-13.2906900395037,-45.0783193561008,
20.));
#75435=CARTESIAN_POINT('Ctrl Pts',(-13.3214635730135,-45.0661237554798,
0.));
#75436=CARTESIAN_POINT('Ctrl Pts',(-13.3214635730135,-45.0661237554798,
20.));
#75437=CARTESIAN_POINT('Ctrl Pts',(-13.3522275059137,-45.0539069819185,
0.));
#75438=CARTESIAN_POINT('Ctrl Pts',(-13.3522275059137,-45.0539069819185,
20.));
#75439=CARTESIAN_POINT('Ctrl Pts',(-13.3829818233878,-45.0416690422424,
0.));
#75440=CARTESIAN_POINT('Ctrl Pts',(-13.3829818233878,-45.0416690422424,
20.));
#75441=CARTESIAN_POINT('Ctrl Pts',(-13.4137265106238,-45.0294099432879,
0.));
#75442=CARTESIAN_POINT('Ctrl Pts',(-13.4137265106238,-45.0294099432879,
20.));
#75443=CARTESIAN_POINT('Ctrl Pts',(-13.4444615528144,-45.0171296919022,
0.));
#75444=CARTESIAN_POINT('Ctrl Pts',(-13.4444615528144,-45.0171296919022,
20.));
#75445=CARTESIAN_POINT('Ctrl Pts',(-13.4751869351564,-45.0048282949433,
0.));
#75446=CARTESIAN_POINT('Ctrl Pts',(-13.4751869351564,-45.0048282949433,
20.));
#75447=CARTESIAN_POINT('Ctrl Pts',(-13.5059026428512,-44.9925057592796,
0.));
#75448=CARTESIAN_POINT('Ctrl Pts',(-13.5059026428512,-44.9925057592796,
20.));
#75449=CARTESIAN_POINT('Ctrl Pts',(-13.5366086611044,-44.9801620917891,
0.));
#75450=CARTESIAN_POINT('Ctrl Pts',(-13.5366086611044,-44.9801620917891,
20.));
#75451=CARTESIAN_POINT('Ctrl Pts',(-13.5673049751264,-44.967797299361,0.));
#75452=CARTESIAN_POINT('Ctrl Pts',(-13.5673049751264,-44.967797299361,20.));
#75453=CARTESIAN_POINT('Ctrl Pts',(-13.5979915701319,-44.955411388895,0.));
#75454=CARTESIAN_POINT('Ctrl Pts',(-13.5979915701319,-44.955411388895,20.));
#75455=CARTESIAN_POINT('Ctrl Pts',(-13.6286684313402,-44.9430043673018,
0.));
#75456=CARTESIAN_POINT('Ctrl Pts',(-13.6286684313402,-44.9430043673018,
20.));
#75457=CARTESIAN_POINT('Ctrl Pts',(-13.6593355439745,-44.9305762415019,
0.));
#75458=CARTESIAN_POINT('Ctrl Pts',(-13.6593355439745,-44.9305762415019,
20.));
#75459=CARTESIAN_POINT('Ctrl Pts',(-13.6899928932632,-44.9181270184275,
0.));
#75460=CARTESIAN_POINT('Ctrl Pts',(-13.6899928932632,-44.9181270184275,
20.));
#75461=CARTESIAN_POINT('Ctrl Pts',(-13.7206404644388,-44.9056567050204,
0.));
#75462=CARTESIAN_POINT('Ctrl Pts',(-13.7206404644388,-44.9056567050204,
20.));
#75463=CARTESIAN_POINT('Ctrl Pts',(-13.7512782427386,-44.8931653082334,
0.));
#75464=CARTESIAN_POINT('Ctrl Pts',(-13.7512782427386,-44.8931653082334,
20.));
#75465=CARTESIAN_POINT('Ctrl Pts',(-13.7819062134042,-44.8806528350291,
0.));
#75466=CARTESIAN_POINT('Ctrl Pts',(-13.7819062134042,-44.8806528350291,
20.));
#75467=CARTESIAN_POINT('Ctrl Pts',(-13.8125243616816,-44.8681192923811,
0.));
#75468=CARTESIAN_POINT('Ctrl Pts',(-13.8125243616816,-44.8681192923811,
20.));
#75469=CARTESIAN_POINT('Ctrl Pts',(-13.8431326728214,-44.8555646872732,
0.));
#75470=CARTESIAN_POINT('Ctrl Pts',(-13.8431326728214,-44.8555646872732,
20.));
#75471=CARTESIAN_POINT('Ctrl Pts',(-13.8737311320789,-44.8429890267007,
0.));
#75472=CARTESIAN_POINT('Ctrl Pts',(-13.8737311320789,-44.8429890267007,
20.));
#75473=CARTESIAN_POINT('Ctrl Pts',(-13.9043197247138,-44.8303923176691,
0.));
#75474=CARTESIAN_POINT('Ctrl Pts',(-13.9043197247138,-44.8303923176691,
20.));
#75475=CARTESIAN_POINT('Ctrl Pts',(-13.9348984359903,-44.8177745671945,
0.));
#75476=CARTESIAN_POINT('Ctrl Pts',(-13.9348984359903,-44.8177745671945,
20.));
#75477=CARTESIAN_POINT('Ctrl Pts',(-13.9654672511774,-44.8051357823031,
0.));
#75478=CARTESIAN_POINT('Ctrl Pts',(-13.9654672511774,-44.8051357823031,
20.));
#75479=CARTESIAN_POINT('Ctrl Pts',(-13.9960261555481,-44.7924759700314,
0.));
#75480=CARTESIAN_POINT('Ctrl Pts',(-13.9960261555481,-44.7924759700314,
20.));
#75481=CARTESIAN_POINT('Ctrl Pts',(-14.0265751343805,-44.7797951374262,
0.));
#75482=CARTESIAN_POINT('Ctrl Pts',(-14.0265751343805,-44.7797951374262,
20.));
#75483=CARTESIAN_POINT('Ctrl Pts',(-14.057114172957,-44.7670932915455,0.));
#75484=CARTESIAN_POINT('Ctrl Pts',(-14.057114172957,-44.7670932915455,20.));
#75485=CARTESIAN_POINT('Ctrl Pts',(-14.0876432565649,-44.7543704394583,
0.));
#75486=CARTESIAN_POINT('Ctrl Pts',(-14.0876432565649,-44.7543704394583,
20.));
#75487=CARTESIAN_POINT('Ctrl Pts',(-14.118162370496,-44.7416265882442,0.));
#75488=CARTESIAN_POINT('Ctrl Pts',(-14.118162370496,-44.7416265882442,20.));
#75489=CARTESIAN_POINT('Ctrl Pts',(-14.1486715000464,-44.728861744993,0.));
#75490=CARTESIAN_POINT('Ctrl Pts',(-14.1486715000464,-44.728861744993,20.));
#75491=CARTESIAN_POINT('Ctrl Pts',(-14.1791706305171,-44.7160759168044,
0.));
#75492=CARTESIAN_POINT('Ctrl Pts',(-14.1791706305171,-44.7160759168044,
20.));
#75493=CARTESIAN_POINT('Ctrl Pts',(-14.2096597472134,-44.7032691107881,
0.));
#75494=CARTESIAN_POINT('Ctrl Pts',(-14.2096597472134,-44.7032691107881,
20.));
#75495=CARTESIAN_POINT('Ctrl Pts',(-14.2401388354454,-44.690441334065,0.));
#75496=CARTESIAN_POINT('Ctrl Pts',(-14.2401388354454,-44.690441334065,20.));
#75497=CARTESIAN_POINT('Ctrl Pts',(-14.2706078805279,-44.6775925937661,
0.));
#75498=CARTESIAN_POINT('Ctrl Pts',(-14.2706078805279,-44.6775925937661,
20.));
#75499=CARTESIAN_POINT('Ctrl Pts',(-14.3010668677802,-44.6647228970333,
0.));
#75500=CARTESIAN_POINT('Ctrl Pts',(-14.3010668677802,-44.6647228970333,
20.));
#75501=CARTESIAN_POINT('Ctrl Pts',(-14.3315157825264,-44.6518322510194,
0.));
#75502=CARTESIAN_POINT('Ctrl Pts',(-14.3315157825264,-44.6518322510194,
20.));
#75503=CARTESIAN_POINT('Ctrl Pts',(-14.3619546100951,-44.6389206628876,
0.));
#75504=CARTESIAN_POINT('Ctrl Pts',(-14.3619546100951,-44.6389206628876,
20.));
#75505=CARTESIAN_POINT('Ctrl Pts',(-14.3923833358197,-44.6259881398118,
0.));
#75506=CARTESIAN_POINT('Ctrl Pts',(-14.3923833358197,-44.6259881398118,
20.));
#75507=CARTESIAN_POINT('Ctrl Pts',(-14.4228019450383,-44.6130346889769,
0.));
#75508=CARTESIAN_POINT('Ctrl Pts',(-14.4228019450383,-44.6130346889769,
20.));
#75509=CARTESIAN_POINT('Ctrl Pts',(-14.4532104230937,-44.6000603175775,
0.));
#75510=CARTESIAN_POINT('Ctrl Pts',(-14.4532104230937,-44.6000603175775,
20.));
#75511=CARTESIAN_POINT('Ctrl Pts',(-14.4836087553332,-44.5870650328188,
0.));
#75512=CARTESIAN_POINT('Ctrl Pts',(-14.4836087553332,-44.5870650328188,
20.));
#75513=CARTESIAN_POINT('Ctrl Pts',(-14.5139969271087,-44.5740488419152,
0.));
#75514=CARTESIAN_POINT('Ctrl Pts',(-14.5139969271087,-44.5740488419152,
20.));
#75515=CARTESIAN_POINT('Ctrl Pts',(-14.5443749237768,-44.5610117520915,
0.));
#75516=CARTESIAN_POINT('Ctrl Pts',(-14.5443749237768,-44.5610117520915,
20.));
#75517=CARTESIAN_POINT('Ctrl Pts',(-14.5747427306988,-44.5479537705835,
0.));
#75518=CARTESIAN_POINT('Ctrl Pts',(-14.5747427306988,-44.5479537705835,
20.));
#75519=CARTESIAN_POINT('Ctrl Pts',(-14.6051003332411,-44.5348749046378,
0.));
#75520=CARTESIAN_POINT('Ctrl Pts',(-14.6051003332411,-44.5348749046378,
20.));
#75521=CARTESIAN_POINT('Ctrl Pts',(-14.6354477167742,-44.521775161512,0.));
#75522=CARTESIAN_POINT('Ctrl Pts',(-14.6354477167742,-44.521775161512,20.));
#75523=CARTESIAN_POINT('Ctrl Pts',(-14.6657848666744,-44.5086545484757,
0.));
#75524=CARTESIAN_POINT('Ctrl Pts',(-14.6657848666744,-44.5086545484757,
20.));
#75525=CARTESIAN_POINT('Ctrl Pts',(-14.6961117683217,-44.4955130728078,
0.));
#75526=CARTESIAN_POINT('Ctrl Pts',(-14.6961117683217,-44.4955130728078,
20.));
#75527=CARTESIAN_POINT('Ctrl Pts',(-14.7264284071013,-44.4823507417973,
0.));
#75528=CARTESIAN_POINT('Ctrl Pts',(-14.7264284071013,-44.4823507417973,
20.));
#75529=CARTESIAN_POINT('Ctrl Pts',(-14.756734768403,-44.469167562743,0.));
#75530=CARTESIAN_POINT('Ctrl Pts',(-14.756734768403,-44.469167562743,20.));
#75531=CARTESIAN_POINT('Ctrl Pts',(-14.7870308376214,-44.4559635429545,
0.));
#75532=CARTESIAN_POINT('Ctrl Pts',(-14.7870308376214,-44.4559635429545,
20.));
#75533=CARTESIAN_POINT('Ctrl Pts',(-14.817316600156,-44.4427386897515,0.));
#75534=CARTESIAN_POINT('Ctrl Pts',(-14.817316600156,-44.4427386897515,20.));
#75535=CARTESIAN_POINT('Ctrl Pts',(-14.8475920414108,-44.4294930104636,
0.));
#75536=CARTESIAN_POINT('Ctrl Pts',(-14.8475920414108,-44.4294930104636,
20.));
#75537=CARTESIAN_POINT('Ctrl Pts',(-14.8778571467943,-44.416226512431,0.));
#75538=CARTESIAN_POINT('Ctrl Pts',(-14.8778571467943,-44.416226512431,20.));
#75539=CARTESIAN_POINT('Ctrl Pts',(-14.9081119017199,-44.4029392030043,
0.));
#75540=CARTESIAN_POINT('Ctrl Pts',(-14.9081119017199,-44.4029392030043,
20.));
#75541=CARTESIAN_POINT('Ctrl Pts',(-14.9383562916061,-44.389631089546,0.));
#75542=CARTESIAN_POINT('Ctrl Pts',(-14.9383562916061,-44.389631089546,20.));
#75543=CARTESIAN_POINT('Ctrl Pts',(-14.9685903018767,-44.3763021794296,
0.));
#75544=CARTESIAN_POINT('Ctrl Pts',(-14.9685903018767,-44.3763021794296,
20.));
#75545=CARTESIAN_POINT('Ctrl Pts',(-14.9988139179602,-44.3629524800397,
0.));
#75546=CARTESIAN_POINT('Ctrl Pts',(-14.9988139179602,-44.3629524800397,
20.));
#75547=CARTESIAN_POINT('Ctrl Pts',(-15.0290271252899,-44.3495819987707,
0.));
#75548=CARTESIAN_POINT('Ctrl Pts',(-15.0290271252899,-44.3495819987707,
20.));
#75549=CARTESIAN_POINT('Ctrl Pts',(-15.0592299093033,-44.3361907430254,
0.));
#75550=CARTESIAN_POINT('Ctrl Pts',(-15.0592299093033,-44.3361907430254,
20.));
#75551=CARTESIAN_POINT('Ctrl Pts',(-15.0894222554425,-44.3227787202166,
0.));
#75552=CARTESIAN_POINT('Ctrl Pts',(-15.0894222554425,-44.3227787202166,
20.));
#75553=CARTESIAN_POINT('Ctrl Pts',(-15.1196041491546,-44.3093459377674,
0.));
#75554=CARTESIAN_POINT('Ctrl Pts',(-15.1196041491546,-44.3093459377674,
20.));
#75555=CARTESIAN_POINT('Ctrl Pts',(-15.1497755758918,-44.2958924031118,
0.));
#75556=CARTESIAN_POINT('Ctrl Pts',(-15.1497755758918,-44.2958924031118,
20.));
#75557=CARTESIAN_POINT('Ctrl Pts',(-15.1799365211114,-44.2824181236961,
0.));
#75558=CARTESIAN_POINT('Ctrl Pts',(-15.1799365211114,-44.2824181236961,
20.));
#75559=CARTESIAN_POINT('Ctrl Pts',(-15.2100869702755,-44.2689231069767,
0.));
#75560=CARTESIAN_POINT('Ctrl Pts',(-15.2100869702755,-44.2689231069767,
20.));
#75561=CARTESIAN_POINT('Ctrl Pts',(-15.2402269088514,-44.2554073604206,
0.));
#75562=CARTESIAN_POINT('Ctrl Pts',(-15.2402269088514,-44.2554073604206,
20.));
#75563=CARTESIAN_POINT('Ctrl Pts',(-15.2703563223108,-44.2418708915045,
0.));
#75564=CARTESIAN_POINT('Ctrl Pts',(-15.2703563223108,-44.2418708915045,
20.));
#75565=CARTESIAN_POINT('Ctrl Pts',(-15.30047519613,-44.2283137077152,0.));
#75566=CARTESIAN_POINT('Ctrl Pts',(-15.30047519613,-44.2283137077152,20.));
#75567=CARTESIAN_POINT('Ctrl Pts',(-15.3305835157903,-44.2147358165492,
0.));
#75568=CARTESIAN_POINT('Ctrl Pts',(-15.3305835157903,-44.2147358165492,
20.));
#75569=CARTESIAN_POINT('Ctrl Pts',(-15.3606812667781,-44.201137225514,0.));
#75570=CARTESIAN_POINT('Ctrl Pts',(-15.3606812667781,-44.201137225514,20.));
#75571=CARTESIAN_POINT('Ctrl Pts',(-15.390768434585,-44.1875179421286,0.));
#75572=CARTESIAN_POINT('Ctrl Pts',(-15.390768434585,-44.1875179421286,20.));
#75573=CARTESIAN_POINT('Ctrl Pts',(-15.4208450047077,-44.1738779739224,
0.));
#75574=CARTESIAN_POINT('Ctrl Pts',(-15.4208450047077,-44.1738779739224,
20.));
#75575=CARTESIAN_POINT('Ctrl Pts',(-15.4509109626472,-44.1602173284345,
0.));
#75576=CARTESIAN_POINT('Ctrl Pts',(-15.4509109626472,-44.1602173284345,
20.));
#75577=CARTESIAN_POINT('Ctrl Pts',(-15.4809662939093,-44.146536013213,0.));
#75578=CARTESIAN_POINT('Ctrl Pts',(-15.4809662939093,-44.146536013213,20.));
#75579=CARTESIAN_POINT('Ctrl Pts',(-15.5110109840048,-44.1328340358171,
0.));
#75580=CARTESIAN_POINT('Ctrl Pts',(-15.5110109840048,-44.1328340358171,
20.));
#75581=CARTESIAN_POINT('Ctrl Pts',(-15.5410450184494,-44.1191114038164,
0.));
#75582=CARTESIAN_POINT('Ctrl Pts',(-15.5410450184494,-44.1191114038164,
20.));
#75583=CARTESIAN_POINT('Ctrl Pts',(-15.5710683827646,-44.1053681247921,
0.));
#75584=CARTESIAN_POINT('Ctrl Pts',(-15.5710683827646,-44.1053681247921,
20.));
#75585=CARTESIAN_POINT('Ctrl Pts',(-15.6010810624766,-44.0916042063371,
0.));
#75586=CARTESIAN_POINT('Ctrl Pts',(-15.6010810624766,-44.0916042063371,
20.));
#75587=CARTESIAN_POINT('Ctrl Pts',(-15.6310830431167,-44.0778196560536,
0.));
#75588=CARTESIAN_POINT('Ctrl Pts',(-15.6310830431167,-44.0778196560536,
20.));
#75589=CARTESIAN_POINT('Ctrl Pts',(-15.6610743102207,-44.0640144815534,
0.));
#75590=CARTESIAN_POINT('Ctrl Pts',(-15.6610743102207,-44.0640144815534,
20.));
#75591=CARTESIAN_POINT('Ctrl Pts',(-15.6910548493289,-44.050188690457,0.));
#75592=CARTESIAN_POINT('Ctrl Pts',(-15.6910548493289,-44.050188690457,20.));
#75593=CARTESIAN_POINT('Ctrl Pts',(-15.7210246459868,-44.0363422903955,
0.));
#75594=CARTESIAN_POINT('Ctrl Pts',(-15.7210246459868,-44.0363422903955,
20.));
#75595=CARTESIAN_POINT('Ctrl Pts',(-15.7509836857452,-44.0224752890112,
0.));
#75596=CARTESIAN_POINT('Ctrl Pts',(-15.7509836857452,-44.0224752890112,
20.));
#75597=CARTESIAN_POINT('Ctrl Pts',(-15.7809319541602,-44.0085876939576,
0.));
#75598=CARTESIAN_POINT('Ctrl Pts',(-15.7809319541602,-44.0085876939576,
20.));
#75599=CARTESIAN_POINT('Ctrl Pts',(-15.8108694367927,-43.9946795128988,
0.));
#75600=CARTESIAN_POINT('Ctrl Pts',(-15.8108694367927,-43.9946795128988,
20.));
#75601=CARTESIAN_POINT('Ctrl Pts',(-15.8407961192089,-43.9807507535096,
0.));
#75602=CARTESIAN_POINT('Ctrl Pts',(-15.8407961192089,-43.9807507535096,
20.));
#75603=CARTESIAN_POINT('Ctrl Pts',(-15.8707119869797,-43.9668014234746,
0.));
#75604=CARTESIAN_POINT('Ctrl Pts',(-15.8707119869797,-43.9668014234746,
20.));
#75605=CARTESIAN_POINT('Ctrl Pts',(-15.9006170256808,-43.9528315304878,
0.));
#75606=CARTESIAN_POINT('Ctrl Pts',(-15.9006170256808,-43.9528315304878,
20.));
#75607=CARTESIAN_POINT('Ctrl Pts',(-15.9305112208934,-43.9388410822542,
0.));
#75608=CARTESIAN_POINT('Ctrl Pts',(-15.9305112208934,-43.9388410822542,
20.));
#75609=CARTESIAN_POINT('Ctrl Pts',(-15.9603945582034,-43.9248300864889,
0.));
#75610=CARTESIAN_POINT('Ctrl Pts',(-15.9603945582034,-43.9248300864889,
20.));
#75611=CARTESIAN_POINT('Ctrl Pts',(-15.9902670232019,-43.9107985509168,
0.));
#75612=CARTESIAN_POINT('Ctrl Pts',(-15.9902670232019,-43.9107985509168,
20.));
#75613=CARTESIAN_POINT('Ctrl Pts',(-16.020128601485,-43.896746483274,0.));
#75614=CARTESIAN_POINT('Ctrl Pts',(-16.020128601485,-43.896746483274,20.));
#75615=CARTESIAN_POINT('Ctrl Pts',(-16.0499792786541,-43.8826738913074,
0.));
#75616=CARTESIAN_POINT('Ctrl Pts',(-16.0499792786541,-43.8826738913074,
20.));
#75617=CARTESIAN_POINT('Ctrl Pts',(-16.0798190403159,-43.8685807827745,
0.));
#75618=CARTESIAN_POINT('Ctrl Pts',(-16.0798190403159,-43.8685807827745,
20.));
#75619=CARTESIAN_POINT('Ctrl Pts',(-16.1096478720818,-43.854467165442,0.));
#75620=CARTESIAN_POINT('Ctrl Pts',(-16.1096478720818,-43.854467165442,20.));
#75621=CARTESIAN_POINT('Ctrl Pts',(-16.1394657595683,-43.8403330470868,
0.));
#75622=CARTESIAN_POINT('Ctrl Pts',(-16.1394657595683,-43.8403330470868,
20.));
#75623=CARTESIAN_POINT('Ctrl Pts',(-16.1692726883968,-43.8261784354962,
0.));
#75624=CARTESIAN_POINT('Ctrl Pts',(-16.1692726883968,-43.8261784354962,
20.));
#75625=CARTESIAN_POINT('Ctrl Pts',(-16.199068644194,-43.8120033384679,0.));
#75626=CARTESIAN_POINT('Ctrl Pts',(-16.199068644194,-43.8120033384679,20.));
#75627=CARTESIAN_POINT('Ctrl Pts',(-16.2288536125917,-43.7978077638098,
0.));
#75628=CARTESIAN_POINT('Ctrl Pts',(-16.2288536125917,-43.7978077638098,
20.));
#75629=CARTESIAN_POINT('Ctrl Pts',(-16.2586275792268,-43.7835917193404,
0.));
#75630=CARTESIAN_POINT('Ctrl Pts',(-16.2586275792268,-43.7835917193404,
20.));
#75631=CARTESIAN_POINT('Ctrl Pts',(-16.2883905297415,-43.7693552128887,
0.));
#75632=CARTESIAN_POINT('Ctrl Pts',(-16.2883905297415,-43.7693552128887,
20.));
#75633=CARTESIAN_POINT('Ctrl Pts',(-16.3181424497834,-43.7550982522947,
0.));
#75634=CARTESIAN_POINT('Ctrl Pts',(-16.3181424497834,-43.7550982522947,
20.));
#75635=CARTESIAN_POINT('Ctrl Pts',(-16.3478833250055,-43.7408208454089,
0.));
#75636=CARTESIAN_POINT('Ctrl Pts',(-16.3478833250055,-43.7408208454089,
20.));
#75637=CARTESIAN_POINT('Ctrl Pts',(-16.3776131410651,-43.7265230000909,
0.));
#75638=CARTESIAN_POINT('Ctrl Pts',(-16.3776131410651,-43.7265230000909,
20.));
#75639=CARTESIAN_POINT('Ctrl Pts',(-16.4073318836249,-43.7122047242097,
0.));
#75640=CARTESIAN_POINT('Ctrl Pts',(-16.4073318836249,-43.7122047242097,
20.));
#75641=CARTESIAN_POINT('Ctrl Pts',(-16.4370395383524,-43.6978660256455,
0.));
#75642=CARTESIAN_POINT('Ctrl Pts',(-16.4370395383524,-43.6978660256455,
20.));
#75643=CARTESIAN_POINT('Ctrl Pts',(-16.4667360909207,-43.6835069122887,
0.));
#75644=CARTESIAN_POINT('Ctrl Pts',(-16.4667360909207,-43.6835069122887,
20.));
#75645=CARTESIAN_POINT('Ctrl Pts',(-16.4964215270082,-43.6691273920409,
0.));
#75646=CARTESIAN_POINT('Ctrl Pts',(-16.4964215270082,-43.6691273920409,
20.));
#75647=CARTESIAN_POINT('Ctrl Pts',(-16.5260958322991,-43.6547274728139,
0.));
#75648=CARTESIAN_POINT('Ctrl Pts',(-16.5260958322991,-43.6547274728139,
20.));
#75649=CARTESIAN_POINT('Ctrl Pts',(-16.5557589924819,-43.640307162529,0.));
#75650=CARTESIAN_POINT('Ctrl Pts',(-16.5557589924819,-43.640307162529,20.));
#75651=CARTESIAN_POINT('Ctrl Pts',(-16.5854109932504,-43.6258664691173,
0.));
#75652=CARTESIAN_POINT('Ctrl Pts',(-16.5854109932504,-43.6258664691173,
20.));
#75653=CARTESIAN_POINT('Ctrl Pts',(-16.6150518203036,-43.6114054005208,
0.));
#75654=CARTESIAN_POINT('Ctrl Pts',(-16.6150518203036,-43.6114054005208,
20.));
#75655=CARTESIAN_POINT('Ctrl Pts',(-16.6446814593459,-43.5969239646926,
0.));
#75656=CARTESIAN_POINT('Ctrl Pts',(-16.6446814593459,-43.5969239646926,
20.));
#75657=CARTESIAN_POINT('Ctrl Pts',(-16.6742998960869,-43.5824221695961,
0.));
#75658=CARTESIAN_POINT('Ctrl Pts',(-16.6742998960869,-43.5824221695961,
20.));
#75659=CARTESIAN_POINT('Ctrl Pts',(-16.7039071162413,-43.5679000232041,
0.));
#75660=CARTESIAN_POINT('Ctrl Pts',(-16.7039071162413,-43.5679000232041,
20.));
#75661=CARTESIAN_POINT('Ctrl Pts',(-16.7335031055295,-43.5533575334996,
0.));
#75662=CARTESIAN_POINT('Ctrl Pts',(-16.7335031055295,-43.5533575334996,
20.));
#75663=CARTESIAN_POINT('Ctrl Pts',(-16.7630878496767,-43.5387947084755,
0.));
#75664=CARTESIAN_POINT('Ctrl Pts',(-16.7630878496767,-43.5387947084755,
20.));
#75665=CARTESIAN_POINT('Ctrl Pts',(-16.792661334414,-43.5242115561352,0.));
#75666=CARTESIAN_POINT('Ctrl Pts',(-16.792661334414,-43.5242115561352,20.));
#75667=CARTESIAN_POINT('Ctrl Pts',(-16.8222235454772,-43.5096080844922,
0.));
#75668=CARTESIAN_POINT('Ctrl Pts',(-16.8222235454772,-43.5096080844922,
20.));
#75669=CARTESIAN_POINT('Ctrl Pts',(-16.8517744686076,-43.4949843015709,
0.));
#75670=CARTESIAN_POINT('Ctrl Pts',(-16.8517744686076,-43.4949843015709,
20.));
#75671=CARTESIAN_POINT('Ctrl Pts',(-16.8813140895513,-43.4803402154062,
0.));
#75672=CARTESIAN_POINT('Ctrl Pts',(-16.8813140895513,-43.4803402154062,
20.));
#75673=CARTESIAN_POINT('Ctrl Pts',(-16.91084239406,-43.4656758340435,0.));
#75674=CARTESIAN_POINT('Ctrl Pts',(-16.91084239406,-43.4656758340435,20.));
#75675=CARTESIAN_POINT('Ctrl Pts',(-16.9403593678908,-43.4509911655382,
0.));
#75676=CARTESIAN_POINT('Ctrl Pts',(-16.9403593678908,-43.4509911655382,
20.));
#75677=CARTESIAN_POINT('Ctrl Pts',(-16.9698649968061,-43.4362862179557,
0.));
#75678=CARTESIAN_POINT('Ctrl Pts',(-16.9698649968061,-43.4362862179557,
20.));
#75679=CARTESIAN_POINT('Ctrl Pts',(-16.9993592665737,-43.4215609993712,
0.));
#75680=CARTESIAN_POINT('Ctrl Pts',(-16.9993592665737,-43.4215609993712,
20.));
#75681=CARTESIAN_POINT('Ctrl Pts',(-17.0288421629666,-43.4068155178695,
0.));
#75682=CARTESIAN_POINT('Ctrl Pts',(-17.0288421629666,-43.4068155178695,
20.));
#75683=CARTESIAN_POINT('Ctrl Pts',(-17.0583136717632,-43.3920497815463,
0.));
#75684=CARTESIAN_POINT('Ctrl Pts',(-17.0583136717632,-43.3920497815463,
20.));
#75685=CARTESIAN_POINT('Ctrl Pts',(-17.0877737787472,-43.3772637985072,
0.));
#75686=CARTESIAN_POINT('Ctrl Pts',(-17.0877737787472,-43.3772637985072,
20.));
#75687=CARTESIAN_POINT('Ctrl Pts',(-17.1172224697079,-43.3624575768695,
0.));
#75688=CARTESIAN_POINT('Ctrl Pts',(-17.1172224697079,-43.3624575768695,
20.));
#75689=CARTESIAN_POINT('Ctrl Pts',(-17.1466597304397,-43.3476311247602,
0.));
#75690=CARTESIAN_POINT('Ctrl Pts',(-17.1466597304397,-43.3476311247602,
20.));
#75691=CARTESIAN_POINT('Ctrl Pts',(-17.1760855467426,-43.332784450317,0.));
#75692=CARTESIAN_POINT('Ctrl Pts',(-17.1760855467426,-43.332784450317,20.));
#75693=CARTESIAN_POINT('Ctrl Pts',(-17.2054999044213,-43.3179175616862,
0.));
#75694=CARTESIAN_POINT('Ctrl Pts',(-17.2054999044213,-43.3179175616862,
20.));
#75695=CARTESIAN_POINT('Ctrl Pts',(-17.2349027892859,-43.3030304670242,
0.));
#75696=CARTESIAN_POINT('Ctrl Pts',(-17.2349027892859,-43.3030304670242,
20.));
#75697=CARTESIAN_POINT('Ctrl Pts',(-17.2642941871522,-43.2881231744974,
0.));
#75698=CARTESIAN_POINT('Ctrl Pts',(-17.2642941871522,-43.2881231744974,
20.));
#75699=CARTESIAN_POINT('Ctrl Pts',(-17.2936740838416,-43.2731956922839,
0.));
#75700=CARTESIAN_POINT('Ctrl Pts',(-17.2936740838416,-43.2731956922839,
20.));
#75701=CARTESIAN_POINT('Ctrl Pts',(-17.3230424651811,-43.258248028572,0.));
#75702=CARTESIAN_POINT('Ctrl Pts',(-17.3230424651811,-43.258248028572,20.));
#75703=CARTESIAN_POINT('Ctrl Pts',(-17.3523993170031,-43.2432801915607,
0.));
#75704=CARTESIAN_POINT('Ctrl Pts',(-17.3523993170031,-43.2432801915607,
20.));
#75705=CARTESIAN_POINT('Ctrl Pts',(-17.3817446251452,-43.2282921894589,
0.));
#75706=CARTESIAN_POINT('Ctrl Pts',(-17.3817446251452,-43.2282921894589,
20.));
#75707=CARTESIAN_POINT('Ctrl Pts',(-17.4110783754507,-43.2132840304854,
0.));
#75708=CARTESIAN_POINT('Ctrl Pts',(-17.4110783754507,-43.2132840304854,
20.));
#75709=CARTESIAN_POINT('Ctrl Pts',(-17.4404005537678,-43.1982557228684,
0.));
#75710=CARTESIAN_POINT('Ctrl Pts',(-17.4404005537678,-43.1982557228684,
20.));
#75711=CARTESIAN_POINT('Ctrl Pts',(-17.4697111459501,-43.1832072748459,
0.));
#75712=CARTESIAN_POINT('Ctrl Pts',(-17.4697111459501,-43.1832072748459,
20.));
#75713=CARTESIAN_POINT('Ctrl Pts',(-17.4990101378563,-43.1681386946662,
0.));
#75714=CARTESIAN_POINT('Ctrl Pts',(-17.4990101378563,-43.1681386946662,
20.));
#75715=CARTESIAN_POINT('Ctrl Pts',(-17.5282975153509,-43.1530499905879,
0.));
#75716=CARTESIAN_POINT('Ctrl Pts',(-17.5282975153509,-43.1530499905879,
20.));
#75717=CARTESIAN_POINT('Ctrl Pts',(-17.557573264304,-43.1379411708804,0.));
#75718=CARTESIAN_POINT('Ctrl Pts',(-17.557573264304,-43.1379411708804,20.));
#75719=CARTESIAN_POINT('Ctrl Pts',(-17.5868373705916,-43.122812243824,0.));
#75720=CARTESIAN_POINT('Ctrl Pts',(-17.5868373705916,-43.122812243824,20.));
#75721=CARTESIAN_POINT('Ctrl Pts',(-17.6160898200949,-43.1076632177088,
0.));
#75722=CARTESIAN_POINT('Ctrl Pts',(-17.6160898200949,-43.1076632177088,
20.));
#75723=CARTESIAN_POINT('Ctrl Pts',(-17.645330598701,-43.0924941008354,0.));
#75724=CARTESIAN_POINT('Ctrl Pts',(-17.645330598701,-43.0924941008354,20.));
#75725=CARTESIAN_POINT('Ctrl Pts',(-17.674559692302,-43.0773049015136,0.));
#75726=CARTESIAN_POINT('Ctrl Pts',(-17.674559692302,-43.0773049015136,20.));
#75727=CARTESIAN_POINT('Ctrl Pts',(-17.7037770867956,-43.0620956280638,
0.));
#75728=CARTESIAN_POINT('Ctrl Pts',(-17.7037770867956,-43.0620956280638,
20.));
#75729=CARTESIAN_POINT('Ctrl Pts',(-17.7329827680847,-43.0468662888157,
0.));
#75730=CARTESIAN_POINT('Ctrl Pts',(-17.7329827680847,-43.0468662888157,
20.));
#75731=CARTESIAN_POINT('Ctrl Pts',(-17.7621767220773,-43.0316168921093,
0.));
#75732=CARTESIAN_POINT('Ctrl Pts',(-17.7621767220773,-43.0316168921093,
20.));
#75733=CARTESIAN_POINT('Ctrl Pts',(-17.7913589346876,-43.0163474462951,
0.));
#75734=CARTESIAN_POINT('Ctrl Pts',(-17.7913589346876,-43.0163474462951,
20.));
#75735=CARTESIAN_POINT('Ctrl Pts',(-17.8205293918351,-43.0010579597341,
0.));
#75736=CARTESIAN_POINT('Ctrl Pts',(-17.8205293918351,-43.0010579597341,
20.));
#75737=CARTESIAN_POINT('Ctrl Pts',(-17.8496880794454,-42.9857484407979,
0.));
#75738=CARTESIAN_POINT('Ctrl Pts',(-17.8496880794454,-42.9857484407979,
20.));
#75739=CARTESIAN_POINT('Ctrl Pts',(-17.8788349834491,-42.9704188978681,
0.));
#75740=CARTESIAN_POINT('Ctrl Pts',(-17.8788349834491,-42.9704188978681,
20.));
#75741=CARTESIAN_POINT('Ctrl Pts',(-17.9079700897828,-42.9550693393359,
0.));
#75742=CARTESIAN_POINT('Ctrl Pts',(-17.9079700897828,-42.9550693393359,
20.));
#75743=CARTESIAN_POINT('Ctrl Pts',(-17.9370933843882,-42.9396997736018,
0.));
#75744=CARTESIAN_POINT('Ctrl Pts',(-17.9370933843882,-42.9396997736018,
20.));
#75745=CARTESIAN_POINT('Ctrl Pts',(-17.9662048532126,-42.9243102090766,
0.));
#75746=CARTESIAN_POINT('Ctrl Pts',(-17.9662048532126,-42.9243102090766,
20.));
#75747=CARTESIAN_POINT('Ctrl Pts',(-17.9953044822088,-42.9089006541818,
0.));
#75748=CARTESIAN_POINT('Ctrl Pts',(-17.9953044822088,-42.9089006541818,
20.));
#75749=CARTESIAN_POINT('Ctrl Pts',(-18.0243922573354,-42.893471117349,0.));
#75750=CARTESIAN_POINT('Ctrl Pts',(-18.0243922573354,-42.893471117349,20.));
#75751=CARTESIAN_POINT('Ctrl Pts',(-18.0534681645565,-42.8780216070204,
0.));
#75752=CARTESIAN_POINT('Ctrl Pts',(-18.0534681645565,-42.8780216070204,
20.));
#75753=CARTESIAN_POINT('Ctrl Pts',(-18.0825321898416,-42.8625521316488,
0.));
#75754=CARTESIAN_POINT('Ctrl Pts',(-18.0825321898416,-42.8625521316488,
20.));
#75755=CARTESIAN_POINT('Ctrl Pts',(-18.1115843191668,-42.8470626996976,
0.));
#75756=CARTESIAN_POINT('Ctrl Pts',(-18.1115843191668,-42.8470626996976,
20.));
#75757=CARTESIAN_POINT('Ctrl Pts',(-18.1406245385131,-42.831553319639,0.));
#75758=CARTESIAN_POINT('Ctrl Pts',(-18.1406245385131,-42.831553319639,20.));
#75759=CARTESIAN_POINT('Ctrl Pts',(-18.1696528338673,-42.8160239999555,
0.));
#75760=CARTESIAN_POINT('Ctrl Pts',(-18.1696528338673,-42.8160239999555,
20.));
#75761=CARTESIAN_POINT('Ctrl Pts',(-18.1986691912208,-42.8004747491375,
0.));
#75762=CARTESIAN_POINT('Ctrl Pts',(-18.1986691912208,-42.8004747491375,
20.));
#75763=CARTESIAN_POINT('Ctrl Pts',(-18.2276735965714,-42.7849055756869,
0.));
#75764=CARTESIAN_POINT('Ctrl Pts',(-18.2276735965714,-42.7849055756869,
20.));
#75765=CARTESIAN_POINT('Ctrl Pts',(-18.256666035922,-42.7693164881155,0.));
#75766=CARTESIAN_POINT('Ctrl Pts',(-18.256666035922,-42.7693164881155,20.));
#75767=CARTESIAN_POINT('Ctrl Pts',(-18.285646495282,-42.7537074949463,0.));
#75768=CARTESIAN_POINT('Ctrl Pts',(-18.285646495282,-42.7537074949463,20.));
#75769=CARTESIAN_POINT('Ctrl Pts',(-18.3146149606662,-42.7380786047127,
0.));
#75770=CARTESIAN_POINT('Ctrl Pts',(-18.3146149606662,-42.7380786047127,
20.));
#75771=CARTESIAN_POINT('Ctrl Pts',(-18.3435714180954,-42.7224298259587,
0.));
#75772=CARTESIAN_POINT('Ctrl Pts',(-18.3435714180954,-42.7224298259587,
20.));
#75773=CARTESIAN_POINT('Ctrl Pts',(-18.372515853596,-42.7067611672378,0.));
#75774=CARTESIAN_POINT('Ctrl Pts',(-18.372515853596,-42.7067611672378,20.));
#75775=CARTESIAN_POINT('Ctrl Pts',(-18.4014482531999,-42.6910726371132,
0.));
#75776=CARTESIAN_POINT('Ctrl Pts',(-18.4014482531999,-42.6910726371132,
20.));
#75777=CARTESIAN_POINT('Ctrl Pts',(-18.4303686029444,-42.6753642441576,
0.));
#75778=CARTESIAN_POINT('Ctrl Pts',(-18.4303686029444,-42.6753642441576,
20.));
#75779=CARTESIAN_POINT('Ctrl Pts',(-18.4592768888724,-42.6596359969538,
0.));
#75780=CARTESIAN_POINT('Ctrl Pts',(-18.4592768888724,-42.6596359969538,
20.));
#75781=CARTESIAN_POINT('Ctrl Pts',(-18.4881730970326,-42.6438879040941,
0.));
#75782=CARTESIAN_POINT('Ctrl Pts',(-18.4881730970326,-42.6438879040941,
20.));
#75783=CARTESIAN_POINT('Ctrl Pts',(-18.5170572134793,-42.6281199741818,
0.));
#75784=CARTESIAN_POINT('Ctrl Pts',(-18.5170572134793,-42.6281199741818,
20.));
#75785=CARTESIAN_POINT('Ctrl Pts',(-18.5459292242727,-42.61233221583,0.));
#75786=CARTESIAN_POINT('Ctrl Pts',(-18.5459292242727,-42.61233221583,20.));
#75787=CARTESIAN_POINT('Ctrl Pts',(-18.574789115479,-42.596524637663,0.));
#75788=CARTESIAN_POINT('Ctrl Pts',(-18.574789115479,-42.596524637663,20.));
#75789=CARTESIAN_POINT('Ctrl Pts',(-18.6036368731702,-42.5806972483146,
0.));
#75790=CARTESIAN_POINT('Ctrl Pts',(-18.6036368731702,-42.5806972483146,
20.));
#75791=CARTESIAN_POINT('Ctrl Pts',(-18.632472483424,-42.5648500564287,0.));
#75792=CARTESIAN_POINT('Ctrl Pts',(-18.632472483424,-42.5648500564287,20.));
#75793=CARTESIAN_POINT('Ctrl Pts',(-18.6612959323233,-42.5489830706585,
0.));
#75794=CARTESIAN_POINT('Ctrl Pts',(-18.6612959323233,-42.5489830706585,
20.));
#75795=CARTESIAN_POINT('Ctrl Pts',(-18.6901072059568,-42.5330962996668,
0.));
#75796=CARTESIAN_POINT('Ctrl Pts',(-18.6901072059568,-42.5330962996668,
20.));
#75797=CARTESIAN_POINT('Ctrl Pts',(-18.718906290419,-42.5171897521269,0.));
#75798=CARTESIAN_POINT('Ctrl Pts',(-18.718906290419,-42.5171897521269,20.));
#75799=CARTESIAN_POINT('Ctrl Pts',(-18.7476931718101,-42.5012634367222,
0.));
#75800=CARTESIAN_POINT('Ctrl Pts',(-18.7476931718101,-42.5012634367222,
20.));
#75801=CARTESIAN_POINT('Ctrl Pts',(-18.7764678362368,-42.4853173621469,
0.));
#75802=CARTESIAN_POINT('Ctrl Pts',(-18.7764678362368,-42.4853173621469,
20.));
#75803=CARTESIAN_POINT('Ctrl Pts',(-18.8052302698113,-42.4693515371059,
0.));
#75804=CARTESIAN_POINT('Ctrl Pts',(-18.8052302698113,-42.4693515371059,
20.));
#75805=CARTESIAN_POINT('Ctrl Pts',(-18.8339804586522,-42.4533659703145,
0.));
#75806=CARTESIAN_POINT('Ctrl Pts',(-18.8339804586522,-42.4533659703145,
20.));
#75807=CARTESIAN_POINT('Ctrl Pts',(-18.8627183888827,-42.4373606704956,
0.));
#75808=CARTESIAN_POINT('Ctrl Pts',(-18.8627183888827,-42.4373606704956,
20.));
#75809=CARTESIAN_POINT('Ctrl Pts',(-18.8914440466322,-42.4213356463824,
0.));
#75810=CARTESIAN_POINT('Ctrl Pts',(-18.8914440466322,-42.4213356463824,
20.));
#75811=CARTESIAN_POINT('Ctrl Pts',(-18.9201574180352,-42.4052909067172,
0.));
#75812=CARTESIAN_POINT('Ctrl Pts',(-18.9201574180352,-42.4052909067172,
20.));
#75813=CARTESIAN_POINT('Ctrl Pts',(-18.9488584892326,-42.389226460254,0.));
#75814=CARTESIAN_POINT('Ctrl Pts',(-18.9488584892326,-42.389226460254,20.));
#75815=CARTESIAN_POINT('Ctrl Pts',(-18.9775472463711,-42.3731423157568,
0.));
#75816=CARTESIAN_POINT('Ctrl Pts',(-18.9775472463711,-42.3731423157568,
20.));
#75817=CARTESIAN_POINT('Ctrl Pts',(-19.0062236756035,-42.3570384820003,
0.));
#75818=CARTESIAN_POINT('Ctrl Pts',(-19.0062236756035,-42.3570384820003,
20.));
#75819=CARTESIAN_POINT('Ctrl Pts',(-19.0348877630887,-42.3409149677685,
0.));
#75820=CARTESIAN_POINT('Ctrl Pts',(-19.0348877630887,-42.3409149677685,
20.));
#75821=CARTESIAN_POINT('Ctrl Pts',(-19.0635394949913,-42.3247717818558,
0.));
#75822=CARTESIAN_POINT('Ctrl Pts',(-19.0635394949913,-42.3247717818558,
20.));
#75823=CARTESIAN_POINT('Ctrl Pts',(-19.0921788574819,-42.3086089330657,
0.));
#75824=CARTESIAN_POINT('Ctrl Pts',(-19.0921788574819,-42.3086089330657,
20.));
#75825=CARTESIAN_POINT('Ctrl Pts',(-19.1208058367362,-42.2924264302113,
0.));
#75826=CARTESIAN_POINT('Ctrl Pts',(-19.1208058367362,-42.2924264302113,
20.));
#75827=CARTESIAN_POINT('Ctrl Pts',(-19.1494204189361,-42.2762242821163,
0.));
#75828=CARTESIAN_POINT('Ctrl Pts',(-19.1494204189361,-42.2762242821163,
20.));
#75829=CARTESIAN_POINT('Ctrl Pts',(-19.1780225902694,-42.2600024976146,
0.));
#75830=CARTESIAN_POINT('Ctrl Pts',(-19.1780225902694,-42.2600024976146,
20.));
#75831=CARTESIAN_POINT('Ctrl Pts',(-19.2066123369297,-42.2437610855506,
0.));
#75832=CARTESIAN_POINT('Ctrl Pts',(-19.2066123369297,-42.2437610855506,
20.));
#75833=CARTESIAN_POINT('Ctrl Pts',(-19.2351896451166,-42.2275000547783,
0.));
#75834=CARTESIAN_POINT('Ctrl Pts',(-19.2351896451166,-42.2275000547783,
20.));
#75835=CARTESIAN_POINT('Ctrl Pts',(-19.2637545010356,-42.2112194141618,
0.));
#75836=CARTESIAN_POINT('Ctrl Pts',(-19.2637545010356,-42.2112194141618,
20.));
#75837=CARTESIAN_POINT('Ctrl Pts',(-19.2923068908981,-42.1949191725745,
0.));
#75838=CARTESIAN_POINT('Ctrl Pts',(-19.2923068908981,-42.1949191725745,
20.));
#75839=CARTESIAN_POINT('Ctrl Pts',(-19.3208468009212,-42.1785993388989,
0.));
#75840=CARTESIAN_POINT('Ctrl Pts',(-19.3208468009212,-42.1785993388989,
20.));
#75841=CARTESIAN_POINT('Ctrl Pts',(-19.3493742173283,-42.1622599220289,
0.));
#75842=CARTESIAN_POINT('Ctrl Pts',(-19.3493742173283,-42.1622599220289,
20.));
#75843=CARTESIAN_POINT('Ctrl Pts',(-19.377889126349,-42.1459009308685,0.));
#75844=CARTESIAN_POINT('Ctrl Pts',(-19.377889126349,-42.1459009308685,20.));
#75845=CARTESIAN_POINT('Ctrl Pts',(-19.4063915142187,-42.1295223743319,
0.));
#75846=CARTESIAN_POINT('Ctrl Pts',(-19.4063915142187,-42.1295223743319,
20.));
#75847=CARTESIAN_POINT('Ctrl Pts',(-19.4348813671785,-42.1131242613432,
0.));
#75848=CARTESIAN_POINT('Ctrl Pts',(-19.4348813671785,-42.1131242613432,
20.));
#75849=CARTESIAN_POINT('Ctrl Pts',(-19.4633586714748,-42.0967066008354,
0.));
#75850=CARTESIAN_POINT('Ctrl Pts',(-19.4633586714748,-42.0967066008354,
20.));
#75851=CARTESIAN_POINT('Ctrl Pts',(-19.4918234133604,-42.080269401751,0.));
#75852=CARTESIAN_POINT('Ctrl Pts',(-19.4918234133604,-42.080269401751,20.));
#75853=CARTESIAN_POINT('Ctrl Pts',(-19.520275579094,-42.0638126730426,0.));
#75854=CARTESIAN_POINT('Ctrl Pts',(-19.520275579094,-42.0638126730426,20.));
#75855=CARTESIAN_POINT('Ctrl Pts',(-19.5487151549408,-42.0473364236742,
0.));
#75856=CARTESIAN_POINT('Ctrl Pts',(-19.5487151549408,-42.0473364236742,
20.));
#75857=CARTESIAN_POINT('Ctrl Pts',(-19.5771421271718,-42.0308406626191,
0.));
#75858=CARTESIAN_POINT('Ctrl Pts',(-19.5771421271718,-42.0308406626191,
20.));
#75859=CARTESIAN_POINT('Ctrl Pts',(-19.6055564820642,-42.0143253988608,
0.));
#75860=CARTESIAN_POINT('Ctrl Pts',(-19.6055564820642,-42.0143253988608,
20.));
#75861=CARTESIAN_POINT('Ctrl Pts',(-19.6339582059009,-41.997790641393,0.));
#75862=CARTESIAN_POINT('Ctrl Pts',(-19.6339582059009,-41.997790641393,20.));
#75863=CARTESIAN_POINT('Ctrl Pts',(-19.6623472849704,-41.9812363992182,
0.));
#75864=CARTESIAN_POINT('Ctrl Pts',(-19.6623472849704,-41.9812363992182,
20.));
#75865=CARTESIAN_POINT('Ctrl Pts',(-19.6907237055675,-41.9646626813489,
0.));
#75866=CARTESIAN_POINT('Ctrl Pts',(-19.6907237055675,-41.9646626813489,
20.));
#75867=CARTESIAN_POINT('Ctrl Pts',(-19.7190874539927,-41.9480694968077,
0.));
#75868=CARTESIAN_POINT('Ctrl Pts',(-19.7190874539927,-41.9480694968077,
20.));
#75869=CARTESIAN_POINT('Ctrl Pts',(-19.7474385165532,-41.9314568546275,
0.));
#75870=CARTESIAN_POINT('Ctrl Pts',(-19.7474385165532,-41.9314568546275,
20.));
#75871=CARTESIAN_POINT('Ctrl Pts',(-19.775776879562,-41.9148247638512,0.));
#75872=CARTESIAN_POINT('Ctrl Pts',(-19.775776879562,-41.9148247638512,20.));
#75873=CARTESIAN_POINT('Ctrl Pts',(-19.8041025293385,-41.8981732335313,
0.));
#75874=CARTESIAN_POINT('Ctrl Pts',(-19.8041025293385,-41.8981732335313,
20.));
#75875=CARTESIAN_POINT('Ctrl Pts',(-19.8324154522082,-41.8815022727306,
0.));
#75876=CARTESIAN_POINT('Ctrl Pts',(-19.8324154522082,-41.8815022727306,
20.));
#75877=CARTESIAN_POINT('Ctrl Pts',(-19.8607156345021,-41.8648118905217,
0.));
#75878=CARTESIAN_POINT('Ctrl Pts',(-19.8607156345021,-41.8648118905217,
20.));
#75879=CARTESIAN_POINT('Ctrl Pts',(-19.889003062557,-41.8481020959867,0.));
#75880=CARTESIAN_POINT('Ctrl Pts',(-19.889003062557,-41.8481020959867,20.));
#75881=CARTESIAN_POINT('Ctrl Pts',(-19.9172777227157,-41.8313728982175,
0.));
#75882=CARTESIAN_POINT('Ctrl Pts',(-19.9172777227157,-41.8313728982175,
20.));
#75883=CARTESIAN_POINT('Ctrl Pts',(-19.945539601327,-41.8146243063151,0.));
#75884=CARTESIAN_POINT('Ctrl Pts',(-19.945539601327,-41.8146243063151,20.));
#75885=CARTESIAN_POINT('Ctrl Pts',(-19.9737886847462,-41.7978563293914,
0.));
#75886=CARTESIAN_POINT('Ctrl Pts',(-19.9737886847462,-41.7978563293914,
20.));
#75887=CARTESIAN_POINT('Ctrl Pts',(-20.0020249593348,-41.7810689765678,
0.));
#75888=CARTESIAN_POINT('Ctrl Pts',(-20.0020249593348,-41.7810689765678,
20.));
#75889=CARTESIAN_POINT('Ctrl Pts',(-20.0302484114611,-41.7642622569769,
0.));
#75890=CARTESIAN_POINT('Ctrl Pts',(-20.0302484114611,-41.7642622569769,
20.));
#75891=CARTESIAN_POINT('Ctrl Pts',(-20.0584590274992,-41.7474361797609,
0.));
#75892=CARTESIAN_POINT('Ctrl Pts',(-20.0584590274992,-41.7474361797609,
20.));
#75893=CARTESIAN_POINT('Ctrl Pts',(-20.0866567938288,-41.7305907540713,
0.));
#75894=CARTESIAN_POINT('Ctrl Pts',(-20.0866567938288,-41.7305907540713,
20.));
#75895=CARTESIAN_POINT('Ctrl Pts',(-20.1148416968357,-41.7137259890696,
0.));
#75896=CARTESIAN_POINT('Ctrl Pts',(-20.1148416968357,-41.7137259890696,
20.));
#75897=CARTESIAN_POINT('Ctrl Pts',(-20.1430137229118,-41.6968418939263,
0.));
#75898=CARTESIAN_POINT('Ctrl Pts',(-20.1430137229118,-41.6968418939263,
20.));
#75899=CARTESIAN_POINT('Ctrl Pts',(-20.1711728584549,-41.6799384778218,
0.));
#75900=CARTESIAN_POINT('Ctrl Pts',(-20.1711728584549,-41.6799384778218,
20.));
#75901=CARTESIAN_POINT('Ctrl Pts',(-20.199319089869,-41.6630157499462,0.));
#75902=CARTESIAN_POINT('Ctrl Pts',(-20.199319089869,-41.6630157499462,20.));
#75903=CARTESIAN_POINT('Ctrl Pts',(-20.2274524035648,-41.6460737195007,
0.));
#75904=CARTESIAN_POINT('Ctrl Pts',(-20.2274524035648,-41.6460737195007,
20.));
#75905=CARTESIAN_POINT('Ctrl Pts',(-20.2555727859589,-41.6291123956959,
0.));
#75906=CARTESIAN_POINT('Ctrl Pts',(-20.2555727859589,-41.6291123956959,
20.));
#75907=CARTESIAN_POINT('Ctrl Pts',(-20.2836802234745,-41.6121317877528,
0.));
#75908=CARTESIAN_POINT('Ctrl Pts',(-20.2836802234745,-41.6121317877528,
20.));
#75909=CARTESIAN_POINT('Ctrl Pts',(-20.3117747025404,-41.5951319049016,
0.));
#75910=CARTESIAN_POINT('Ctrl Pts',(-20.3117747025404,-41.5951319049016,
20.));
#75911=CARTESIAN_POINT('Ctrl Pts',(-20.3398562095917,-41.5781127563818,
0.));
#75912=CARTESIAN_POINT('Ctrl Pts',(-20.3398562095917,-41.5781127563818,
20.));
#75913=CARTESIAN_POINT('Ctrl Pts',(-20.3679247310694,-41.561074351443,0.));
#75914=CARTESIAN_POINT('Ctrl Pts',(-20.3679247310694,-41.561074351443,20.));
#75915=CARTESIAN_POINT('Ctrl Pts',(-20.3959802534211,-41.5440166993445,
0.));
#75916=CARTESIAN_POINT('Ctrl Pts',(-20.3959802534211,-41.5440166993445,
20.));
#75917=CARTESIAN_POINT('Ctrl Pts',(-20.4240227631002,-41.5269398093561,
0.));
#75918=CARTESIAN_POINT('Ctrl Pts',(-20.4240227631002,-41.5269398093561,
20.));
#75919=CARTESIAN_POINT('Ctrl Pts',(-20.4520522465668,-41.5098436907568,
0.));
#75920=CARTESIAN_POINT('Ctrl Pts',(-20.4520522465668,-41.5098436907568,
20.));
#75921=CARTESIAN_POINT('Ctrl Pts',(-20.4800686902869,-41.4927283528358,
0.));
#75922=CARTESIAN_POINT('Ctrl Pts',(-20.4800686902869,-41.4927283528358,
20.));
#75923=CARTESIAN_POINT('Ctrl Pts',(-20.5080720807336,-41.4755938048931,
0.));
#75924=CARTESIAN_POINT('Ctrl Pts',(-20.5080720807336,-41.4755938048931,
20.));
#75925=CARTESIAN_POINT('Ctrl Pts',(-20.5360624043854,-41.4584400562379,
0.));
#75926=CARTESIAN_POINT('Ctrl Pts',(-20.5360624043854,-41.4584400562379,
20.));
#75927=CARTESIAN_POINT('Ctrl Pts',(-20.564039647727,-41.4412671161883,0.));
#75928=CARTESIAN_POINT('Ctrl Pts',(-20.564039647727,-41.4412671161883,20.));
#75929=CARTESIAN_POINT('Ctrl Pts',(-20.592003797249,-41.4240749940721,0.));
#75930=CARTESIAN_POINT('Ctrl Pts',(-20.592003797249,-41.4240749940721,20.));
#75931=CARTESIAN_POINT('Ctrl Pts',(-20.6199548394484,-41.4068636992265,
0.));
#75932=CARTESIAN_POINT('Ctrl Pts',(-20.6199548394484,-41.4068636992265,
20.));
#75933=CARTESIAN_POINT('Ctrl Pts',(-20.6478927608288,-41.3896332409988,
0.));
#75934=CARTESIAN_POINT('Ctrl Pts',(-20.6478927608288,-41.3896332409988,
20.));
#75935=CARTESIAN_POINT('Ctrl Pts',(-20.6758175479,-41.372383628747,0.));
#75936=CARTESIAN_POINT('Ctrl Pts',(-20.6758175479,-41.372383628747,20.));
#75937=CARTESIAN_POINT('Ctrl Pts',(-20.7037291871782,-41.3551148718389,
0.));
#75938=CARTESIAN_POINT('Ctrl Pts',(-20.7037291871782,-41.3551148718389,
20.));
#75939=CARTESIAN_POINT('Ctrl Pts',(-20.731627665186,-41.3378269796522,0.));
#75940=CARTESIAN_POINT('Ctrl Pts',(-20.731627665186,-41.3378269796522,20.));
#75941=CARTESIAN_POINT('Ctrl Pts',(-20.7595129684521,-41.3205199615745,
0.));
#75942=CARTESIAN_POINT('Ctrl Pts',(-20.7595129684521,-41.3205199615745,
20.));
#75943=CARTESIAN_POINT('Ctrl Pts',(-20.7873850835117,-41.303193827003,0.));
#75944=CARTESIAN_POINT('Ctrl Pts',(-20.7873850835117,-41.303193827003,20.));
#75945=CARTESIAN_POINT('Ctrl Pts',(-20.8152439969059,-41.285848585344,0.));
#75946=CARTESIAN_POINT('Ctrl Pts',(-20.8152439969059,-41.285848585344,20.));
#75947=CARTESIAN_POINT('Ctrl Pts',(-20.8430896951822,-41.268484246013,0.));
#75948=CARTESIAN_POINT('Ctrl Pts',(-20.8430896951822,-41.268484246013,20.));
#75949=CARTESIAN_POINT('Ctrl Pts',(-20.8709221648944,-41.2511008184358,
0.));
#75950=CARTESIAN_POINT('Ctrl Pts',(-20.8709221648944,-41.2511008184358,
20.));
#75951=CARTESIAN_POINT('Ctrl Pts',(-20.8987413926025,-41.2336983120481,
0.));
#75952=CARTESIAN_POINT('Ctrl Pts',(-20.8987413926025,-41.2336983120481,
20.));
#75953=CARTESIAN_POINT('Ctrl Pts',(-20.9265473648728,-41.2162767362953,
0.));
#75954=CARTESIAN_POINT('Ctrl Pts',(-20.9265473648728,-41.2162767362953,
20.));
#75955=CARTESIAN_POINT('Ctrl Pts',(-20.9543400682781,-41.1988361006333,
0.));
#75956=CARTESIAN_POINT('Ctrl Pts',(-20.9543400682781,-41.1988361006333,
20.));
#75957=CARTESIAN_POINT('Ctrl Pts',(-20.9821194893979,-41.1813764145274,
0.));
#75958=CARTESIAN_POINT('Ctrl Pts',(-20.9821194893979,-41.1813764145274,
20.));
#75959=CARTESIAN_POINT('Ctrl Pts',(-21.009885614818,-41.1638976874526,0.));
#75960=CARTESIAN_POINT('Ctrl Pts',(-21.009885614818,-41.1638976874526,20.));
#75961=CARTESIAN_POINT('Ctrl Pts',(-21.0376384311301,-41.1463999288927,
0.));
#75962=CARTESIAN_POINT('Ctrl Pts',(-21.0376384311301,-41.1463999288927,
20.));
#75963=CARTESIAN_POINT('Ctrl Pts',(-21.0653779249329,-41.128883148342,0.));
#75964=CARTESIAN_POINT('Ctrl Pts',(-21.0653779249329,-41.128883148342,20.));
#75965=CARTESIAN_POINT('Ctrl Pts',(-21.0931040828311,-41.1113473553046,
0.));
#75966=CARTESIAN_POINT('Ctrl Pts',(-21.0931040828311,-41.1113473553046,
20.));
#75967=CARTESIAN_POINT('Ctrl Pts',(-21.1208168914355,-41.0937925592943,
0.));
#75968=CARTESIAN_POINT('Ctrl Pts',(-21.1208168914355,-41.0937925592943,
20.));
#75969=CARTESIAN_POINT('Ctrl Pts',(-21.1485163373635,-41.076218769835,0.));
#75970=CARTESIAN_POINT('Ctrl Pts',(-21.1485163373635,-41.076218769835,20.));
#75971=CARTESIAN_POINT('Ctrl Pts',(-21.1762024072388,-41.0586259964597,
0.));
#75972=CARTESIAN_POINT('Ctrl Pts',(-21.1762024072388,-41.0586259964597,
20.));
#75973=CARTESIAN_POINT('Ctrl Pts',(-21.2038750876913,-41.0410142487106,
0.));
#75974=CARTESIAN_POINT('Ctrl Pts',(-21.2038750876913,-41.0410142487106,
20.));
#75975=CARTESIAN_POINT('Ctrl Pts',(-21.2315343653574,-41.0233835361399,
0.));
#75976=CARTESIAN_POINT('Ctrl Pts',(-21.2315343653574,-41.0233835361399,
20.));
#75977=CARTESIAN_POINT('Ctrl Pts',(-21.25918022688,-41.0057338683097,0.));
#75978=CARTESIAN_POINT('Ctrl Pts',(-21.25918022688,-41.0057338683097,20.));
#75979=CARTESIAN_POINT('Ctrl Pts',(-21.286812658909,-40.9880652547927,0.));
#75980=CARTESIAN_POINT('Ctrl Pts',(-21.286812658909,-40.9880652547927,20.));
#75981=CARTESIAN_POINT('Ctrl Pts',(-21.3144316481012,-40.9703777051716,
0.));
#75982=CARTESIAN_POINT('Ctrl Pts',(-21.3144316481012,-40.9703777051716,
20.));
#75983=CARTESIAN_POINT('Ctrl Pts',(-21.342037181119,-40.9526712290373,0.));
#75984=CARTESIAN_POINT('Ctrl Pts',(-21.342037181119,-40.9526712290373,20.));
#75985=CARTESIAN_POINT('Ctrl Pts',(-21.3696292446317,-40.9349458359905,
0.));
#75986=CARTESIAN_POINT('Ctrl Pts',(-21.3696292446317,-40.9349458359905,
20.));
#75987=CARTESIAN_POINT('Ctrl Pts',(-21.3972078253142,-40.9172015356414,
0.));
#75988=CARTESIAN_POINT('Ctrl Pts',(-21.3972078253142,-40.9172015356414,
20.));
#75989=CARTESIAN_POINT('Ctrl Pts',(-21.424772909848,-40.8994383376102,0.));
#75990=CARTESIAN_POINT('Ctrl Pts',(-21.424772909848,-40.8994383376102,20.));
#75991=CARTESIAN_POINT('Ctrl Pts',(-21.45232448492,-40.8816562515268,0.));
#75992=CARTESIAN_POINT('Ctrl Pts',(-21.45232448492,-40.8816562515268,20.));
#75993=CARTESIAN_POINT('Ctrl Pts',(-21.4798625372243,-40.8638552870319,
0.));
#75994=CARTESIAN_POINT('Ctrl Pts',(-21.4798625372243,-40.8638552870319,
20.));
#75995=CARTESIAN_POINT('Ctrl Pts',(-21.5073870534614,-40.8460354537749,
0.));
#75996=CARTESIAN_POINT('Ctrl Pts',(-21.5073870534614,-40.8460354537749,
20.));
#75997=CARTESIAN_POINT('Ctrl Pts',(-21.5348980203391,-40.8281967614155,
0.));
#75998=CARTESIAN_POINT('Ctrl Pts',(-21.5348980203391,-40.8281967614155,
20.));
#75999=CARTESIAN_POINT('Ctrl Pts',(-21.5623954245725,-40.8103392196221,
0.));
#76000=CARTESIAN_POINT('Ctrl Pts',(-21.5623954245725,-40.8103392196221,
20.));
#76001=CARTESIAN_POINT('Ctrl Pts',(-21.5898792528837,-40.7924628380726,
0.));
#76002=CARTESIAN_POINT('Ctrl Pts',(-21.5898792528837,-40.7924628380726,
20.));
#76003=CARTESIAN_POINT('Ctrl Pts',(-21.6173494920019,-40.7745676264537,
0.));
#76004=CARTESIAN_POINT('Ctrl Pts',(-21.6173494920019,-40.7745676264537,
20.));
#76005=CARTESIAN_POINT('Ctrl Pts',(-21.6448061286619,-40.7566535944621,
0.));
#76006=CARTESIAN_POINT('Ctrl Pts',(-21.6448061286619,-40.7566535944621,
20.));
#76007=CARTESIAN_POINT('Ctrl Pts',(-21.6722491496038,-40.7387207518043,
0.));
#76008=CARTESIAN_POINT('Ctrl Pts',(-21.6722491496038,-40.7387207518043,
20.));
#76009=CARTESIAN_POINT('Ctrl Pts',(-21.6996785415723,-40.7207691081984,
0.));
#76010=CARTESIAN_POINT('Ctrl Pts',(-21.6996785415723,-40.7207691081984,
20.));
#76011=CARTESIAN_POINT('Ctrl Pts',(-21.7270942913167,-40.7027986733736,
0.));
#76012=CARTESIAN_POINT('Ctrl Pts',(-21.7270942913167,-40.7027986733736,
20.));
#76013=CARTESIAN_POINT('Ctrl Pts',(-21.7544963855931,-40.6848094570694,
0.));
#76014=CARTESIAN_POINT('Ctrl Pts',(-21.7544963855931,-40.6848094570694,
20.));
#76015=CARTESIAN_POINT('Ctrl Pts',(-21.781884811165,-40.6668014690334,0.));
#76016=CARTESIAN_POINT('Ctrl Pts',(-21.781884811165,-40.6668014690334,20.));
#76017=CARTESIAN_POINT('Ctrl Pts',(-21.8092595548052,-40.6487747190214,
0.));
#76018=CARTESIAN_POINT('Ctrl Pts',(-21.8092595548052,-40.6487747190214,
20.));
#76019=CARTESIAN_POINT('Ctrl Pts',(-21.8366206032979,-40.6307292167951,
0.));
#76020=CARTESIAN_POINT('Ctrl Pts',(-21.8366206032979,-40.6307292167951,
20.));
#76021=CARTESIAN_POINT('Ctrl Pts',(-21.8639679434382,-40.6126649721233,
0.));
#76022=CARTESIAN_POINT('Ctrl Pts',(-21.8639679434382,-40.6126649721233,
20.));
#76023=CARTESIAN_POINT('Ctrl Pts',(-21.8913015620281,-40.594581994783,0.));
#76024=CARTESIAN_POINT('Ctrl Pts',(-21.8913015620281,-40.594581994783,20.));
#76025=CARTESIAN_POINT('Ctrl Pts',(-21.9186214458728,-40.5764802945639,
0.));
#76026=CARTESIAN_POINT('Ctrl Pts',(-21.9186214458728,-40.5764802945639,
20.));
#76027=CARTESIAN_POINT('Ctrl Pts',(-21.9459275817778,-40.5583598812699,
0.));
#76028=CARTESIAN_POINT('Ctrl Pts',(-21.9459275817778,-40.5583598812699,
20.));
#76029=CARTESIAN_POINT('Ctrl Pts',(-21.9732199565439,-40.5402207647219,
0.));
#76030=CARTESIAN_POINT('Ctrl Pts',(-21.9732199565439,-40.5402207647219,
20.));
#76031=CARTESIAN_POINT('Ctrl Pts',(-22.0004985569689,-40.5220629547578,
0.));
#76032=CARTESIAN_POINT('Ctrl Pts',(-22.0004985569689,-40.5220629547578,
20.));
#76033=CARTESIAN_POINT('Ctrl Pts',(-22.0277633698572,-40.5038864612252,
0.));
#76034=CARTESIAN_POINT('Ctrl Pts',(-22.0277633698572,-40.5038864612252,
20.));
#76035=CARTESIAN_POINT('Ctrl Pts',(-22.0550143820281,-40.485691293976,0.));
#76036=CARTESIAN_POINT('Ctrl Pts',(-22.0550143820281,-40.485691293976,20.));
#76037=CARTESIAN_POINT('Ctrl Pts',(-22.0822515803231,-40.4674774628609,
0.));
#76038=CARTESIAN_POINT('Ctrl Pts',(-22.0822515803231,-40.4674774628609,
20.));
#76039=CARTESIAN_POINT('Ctrl Pts',(-22.1094749516164,-40.4492449777204,
0.));
#76040=CARTESIAN_POINT('Ctrl Pts',(-22.1094749516164,-40.4492449777204,
20.));
#76041=CARTESIAN_POINT('Ctrl Pts',(-22.1366844828092,-40.4309938483881,
0.));
#76042=CARTESIAN_POINT('Ctrl Pts',(-22.1366844828092,-40.4309938483881,
20.));
#76043=CARTESIAN_POINT('Ctrl Pts',(-22.1638801608087,-40.4127240847076,
0.));
#76044=CARTESIAN_POINT('Ctrl Pts',(-22.1638801608087,-40.4127240847076,
20.));
#76045=CARTESIAN_POINT('Ctrl Pts',(-22.1910619725087,-40.3944356965472,
0.));
#76046=CARTESIAN_POINT('Ctrl Pts',(-22.1910619725087,-40.3944356965472,
20.));
#76047=CARTESIAN_POINT('Ctrl Pts',(-22.2182299047735,-40.3761286938114,
0.));
#76048=CARTESIAN_POINT('Ctrl Pts',(-22.2182299047735,-40.3761286938114,
20.));
#76049=CARTESIAN_POINT('Ctrl Pts',(-22.2453839444114,-40.357803086462,0.));
#76050=CARTESIAN_POINT('Ctrl Pts',(-22.2453839444114,-40.357803086462,20.));
#76051=CARTESIAN_POINT('Ctrl Pts',(-22.2725240781926,-40.3394588845042,
0.));
#76052=CARTESIAN_POINT('Ctrl Pts',(-22.2725240781926,-40.3394588845042,
20.));
#76053=CARTESIAN_POINT('Ctrl Pts',(-22.2996502928986,-40.3210960979489,
0.));
#76054=CARTESIAN_POINT('Ctrl Pts',(-22.2996502928986,-40.3210960979489,
20.));
#76055=CARTESIAN_POINT('Ctrl Pts',(-22.3267625753671,-40.3027147367803,
0.));
#76056=CARTESIAN_POINT('Ctrl Pts',(-22.3267625753671,-40.3027147367803,
20.));
#76057=CARTESIAN_POINT('Ctrl Pts',(-22.3538609125294,-40.2843148109267,
0.));
#76058=CARTESIAN_POINT('Ctrl Pts',(-22.3538609125294,-40.2843148109267,
20.));
#76059=CARTESIAN_POINT('Ctrl Pts',(-22.3809452914735,-40.2658963302133,
0.));
#76060=CARTESIAN_POINT('Ctrl Pts',(-22.3809452914735,-40.2658963302133,
20.));
#76061=CARTESIAN_POINT('Ctrl Pts',(-22.4080156993888,-40.2474593044019,
0.));
#76062=CARTESIAN_POINT('Ctrl Pts',(-22.4080156993888,-40.2474593044019,
20.));
#76063=CARTESIAN_POINT('Ctrl Pts',(-22.4350721234534,-40.229003743277,0.));
#76064=CARTESIAN_POINT('Ctrl Pts',(-22.4350721234534,-40.229003743277,20.));
#76065=CARTESIAN_POINT('Ctrl Pts',(-22.4621145507305,-40.2105296567239,
0.));
#76066=CARTESIAN_POINT('Ctrl Pts',(-22.4621145507305,-40.2105296567239,
20.));
#76067=CARTESIAN_POINT('Ctrl Pts',(-22.4891429680799,-40.1920370547964,
0.));
#76068=CARTESIAN_POINT('Ctrl Pts',(-22.4891429680799,-40.1920370547964,
20.));
#76069=CARTESIAN_POINT('Ctrl Pts',(-22.5161573620162,-40.1735259478254,
0.));
#76070=CARTESIAN_POINT('Ctrl Pts',(-22.5161573620162,-40.1735259478254,
20.));
#76071=CARTESIAN_POINT('Ctrl Pts',(-22.5431577188606,-40.1549963463026,
0.));
#76072=CARTESIAN_POINT('Ctrl Pts',(-22.5431577188606,-40.1549963463026,
20.));
#76073=CARTESIAN_POINT('Ctrl Pts',(-22.5701440249982,-40.1364482606861,
0.));
#76074=CARTESIAN_POINT('Ctrl Pts',(-22.5701440249982,-40.1364482606861,
20.));
#76075=CARTESIAN_POINT('Ctrl Pts',(-22.5971162671187,-40.1178817012184,
0.));
#76076=CARTESIAN_POINT('Ctrl Pts',(-22.5971162671187,-40.1178817012184,
20.));
#76077=CARTESIAN_POINT('Ctrl Pts',(-22.6240744324259,-40.0992966777668,
0.));
#76078=CARTESIAN_POINT('Ctrl Pts',(-22.6240744324259,-40.0992966777668,
20.));
#76079=CARTESIAN_POINT('Ctrl Pts',(-22.6510185089549,-40.0806931995834,
0.));
#76080=CARTESIAN_POINT('Ctrl Pts',(-22.6510185089549,-40.0806931995834,
20.));
#76081=CARTESIAN_POINT('Ctrl Pts',(-22.6779484851672,-40.0620712756149,
0.));
#76082=CARTESIAN_POINT('Ctrl Pts',(-22.6779484851672,-40.0620712756149,
20.));
#76083=CARTESIAN_POINT('Ctrl Pts',(-22.7048643493645,-40.0434309149416,
0.));
#76084=CARTESIAN_POINT('Ctrl Pts',(-22.7048643493645,-40.0434309149416,
20.));
#76085=CARTESIAN_POINT('Ctrl Pts',(-22.73176608914,-40.0247721271957,0.));
#76086=CARTESIAN_POINT('Ctrl Pts',(-22.73176608914,-40.0247721271957,20.));
#76087=CARTESIAN_POINT('Ctrl Pts',(-22.7586536908732,-40.0060949229408,
0.));
#76088=CARTESIAN_POINT('Ctrl Pts',(-22.7586536908732,-40.0060949229408,
20.));
#76089=CARTESIAN_POINT('Ctrl Pts',(-22.7855271390494,-39.987399314188,0.));
#76090=CARTESIAN_POINT('Ctrl Pts',(-22.7855271390494,-39.987399314188,20.));
#76091=CARTESIAN_POINT('Ctrl Pts',(-22.8123864172494,-39.9686853136472,
0.));
#76092=CARTESIAN_POINT('Ctrl Pts',(-22.8123864172494,-39.9686853136472,
20.));
#76093=CARTESIAN_POINT('Ctrl Pts',(-22.839231509399,-39.9499529337848,0.));
#76094=CARTESIAN_POINT('Ctrl Pts',(-22.839231509399,-39.9499529337848,20.));
#76095=CARTESIAN_POINT('Ctrl Pts',(-22.8660624009432,-39.9312021859374,
0.));
#76096=CARTESIAN_POINT('Ctrl Pts',(-22.8660624009432,-39.9312021859374,
20.));
#76097=CARTESIAN_POINT('Ctrl Pts',(-22.8928790800155,-39.91243307943,0.));
#76098=CARTESIAN_POINT('Ctrl Pts',(-22.8928790800155,-39.91243307943,20.));
#76099=CARTESIAN_POINT('Ctrl Pts',(-22.9196815387084,-39.8936456206159,
0.));
#76100=CARTESIAN_POINT('Ctrl Pts',(-22.9196815387084,-39.8936456206159,
20.));
#76101=CARTESIAN_POINT('Ctrl Pts',(-22.9464697723601,-39.8748398133807,
0.));
#76102=CARTESIAN_POINT('Ctrl Pts',(-22.9464697723601,-39.8748398133807,
20.));
#76103=CARTESIAN_POINT('Ctrl Pts',(-22.9678889774251,-39.8597804904793,
0.));
#76104=CARTESIAN_POINT('Ctrl Pts',(-22.9678889774251,-39.8597804904793,
20.));
#76105=CARTESIAN_POINT('Ctrl Pts',(-22.9839469786126,-39.8484777427633,
0.));
#76106=CARTESIAN_POINT('Ctrl Pts',(-22.9839469786126,-39.8484777427633,
20.));
#76107=CARTESIAN_POINT('Ctrl Pts',(-22.9946494671375,-39.8409389084975,
0.));
#76108=CARTESIAN_POINT('Ctrl Pts',(-22.9946494671375,-39.8409389084975,
20.));
#76109=CARTESIAN_POINT('Ctrl Pts',(-23.,-39.8371685740842,0.));
#76110=CARTESIAN_POINT('Ctrl Pts',(-23.,-39.8371685740842,20.));
#76111=CARTESIAN_POINT('',(-23.,-39.8371685740842,2.));
#76112=CARTESIAN_POINT('',(-23.,-39.8371685740842,0.));
#76113=CARTESIAN_POINT('Ctrl Pts',(-23.,-39.8371685740842,2.));
#76114=CARTESIAN_POINT('Ctrl Pts',(-20.9761380116544,-41.2633137261046,
2.));
#76115=CARTESIAN_POINT('Ctrl Pts',(-18.8450107958689,-42.5215950809686,
2.));
#76116=CARTESIAN_POINT('Ctrl Pts',(-16.6286143535706,-43.6047734830004,
2.));
#76117=CARTESIAN_POINT('Ctrl Pts',(-37.5361777128299,-31.4965928746404,
0.));
#76118=CARTESIAN_POINT('Ctrl Pts',(-37.5361777128299,-31.4965928746404,
20.));
#76119=CARTESIAN_POINT('Ctrl Pts',(-37.5400435810124,-31.4910366171629,
0.));
#76120=CARTESIAN_POINT('Ctrl Pts',(-37.5400435810124,-31.4910366171629,
20.));
#76121=CARTESIAN_POINT('Ctrl Pts',(-37.5477733397939,-31.4799228688318,
0.));
#76122=CARTESIAN_POINT('Ctrl Pts',(-37.5477733397939,-31.4799228688318,
20.));
#76123=CARTESIAN_POINT('Ctrl Pts',(-37.5593620452151,-31.4632485462068,
0.));
#76124=CARTESIAN_POINT('Ctrl Pts',(-37.5593620452151,-31.4632485462068,
20.));
#76125=CARTESIAN_POINT('Ctrl Pts',(-37.574801786924,-31.4410087157717,0.));
#76126=CARTESIAN_POINT('Ctrl Pts',(-37.574801786924,-31.4410087157717,20.));
#76127=CARTESIAN_POINT('Ctrl Pts',(-37.5940816876034,-31.4131965946731,
0.));
#76128=CARTESIAN_POINT('Ctrl Pts',(-37.5940816876034,-31.4131965946731,
20.));
#76129=CARTESIAN_POINT('Ctrl Pts',(-37.6133418102375,-31.3853721428083,
0.));
#76130=CARTESIAN_POINT('Ctrl Pts',(-37.6133418102375,-31.3853721428083,
20.));
#76131=CARTESIAN_POINT('Ctrl Pts',(-37.6325821517747,-31.3575353648538,
0.));
#76132=CARTESIAN_POINT('Ctrl Pts',(-37.6325821517747,-31.3575353648538,
20.));
#76133=CARTESIAN_POINT('Ctrl Pts',(-37.6518027072643,-31.3296862686536,
0.));
#76134=CARTESIAN_POINT('Ctrl Pts',(-37.6518027072643,-31.3296862686536,
20.));
#76135=CARTESIAN_POINT('Ctrl Pts',(-37.6710034693473,-31.3018248661211,
0.));
#76136=CARTESIAN_POINT('Ctrl Pts',(-37.6710034693473,-31.3018248661211,
20.));
#76137=CARTESIAN_POINT('Ctrl Pts',(-37.6901844288974,-31.2739511721649,
0.));
#76138=CARTESIAN_POINT('Ctrl Pts',(-37.6901844288974,-31.2739511721649,
20.));
#76139=CARTESIAN_POINT('Ctrl Pts',(-37.7093455757381,-31.2460652034827,
0.));
#76140=CARTESIAN_POINT('Ctrl Pts',(-37.7093455757381,-31.2460652034827,
20.));
#76141=CARTESIAN_POINT('Ctrl Pts',(-37.7284868993471,-31.2181669773772,
0.));
#76142=CARTESIAN_POINT('Ctrl Pts',(-37.7284868993471,-31.2181669773772,
20.));
#76143=CARTESIAN_POINT('Ctrl Pts',(-37.7476083895316,-31.1902565106222,
0.));
#76144=CARTESIAN_POINT('Ctrl Pts',(-37.7476083895316,-31.1902565106222,
20.));
#76145=CARTESIAN_POINT('Ctrl Pts',(-37.7667100372089,-31.1623338181506,
0.));
#76146=CARTESIAN_POINT('Ctrl Pts',(-37.7667100372089,-31.1623338181506,
20.));
#76147=CARTESIAN_POINT('Ctrl Pts',(-37.7857918342009,-31.1343989133989,
0.));
#76148=CARTESIAN_POINT('Ctrl Pts',(-37.7857918342009,-31.1343989133989,
20.));
#76149=CARTESIAN_POINT('Ctrl Pts',(-37.8048537728749,-31.1064518089103,
0.));
#76150=CARTESIAN_POINT('Ctrl Pts',(-37.8048537728749,-31.1064518089103,
20.));
#76151=CARTESIAN_POINT('Ctrl Pts',(-37.8238958458276,-31.0784925168637,
0.));
#76152=CARTESIAN_POINT('Ctrl Pts',(-37.8238958458276,-31.0784925168637,
20.));
#76153=CARTESIAN_POINT('Ctrl Pts',(-37.8429180455734,-31.0505210495984,
0.));
#76154=CARTESIAN_POINT('Ctrl Pts',(-37.8429180455734,-31.0505210495984,
20.));
#76155=CARTESIAN_POINT('Ctrl Pts',(-37.861920364175,-31.0225374202321,0.));
#76156=CARTESIAN_POINT('Ctrl Pts',(-37.861920364175,-31.0225374202321,20.));
#76157=CARTESIAN_POINT('Ctrl Pts',(-37.8809027932971,-30.9945416425721,
0.));
#76158=CARTESIAN_POINT('Ctrl Pts',(-37.8809027932971,-30.9945416425721,
20.));
#76159=CARTESIAN_POINT('Ctrl Pts',(-37.8998653243731,-30.9665337308352,
0.));
#76160=CARTESIAN_POINT('Ctrl Pts',(-37.8998653243731,-30.9665337308352,
20.));
#76161=CARTESIAN_POINT('Ctrl Pts',(-37.9188079487378,-30.938513699426,0.));
#76162=CARTESIAN_POINT('Ctrl Pts',(-37.9188079487378,-30.938513699426,20.));
#76163=CARTESIAN_POINT('Ctrl Pts',(-37.9377306577632,-30.9104815627079,
0.));
#76164=CARTESIAN_POINT('Ctrl Pts',(-37.9377306577632,-30.9104815627079,
20.));
#76165=CARTESIAN_POINT('Ctrl Pts',(-37.9566334430211,-30.882437334731,0.));
#76166=CARTESIAN_POINT('Ctrl Pts',(-37.9566334430211,-30.882437334731,20.));
#76167=CARTESIAN_POINT('Ctrl Pts',(-37.9755162962752,-30.8543810292446,
0.));
#76168=CARTESIAN_POINT('Ctrl Pts',(-37.9755162962752,-30.8543810292446,
20.));
#76169=CARTESIAN_POINT('Ctrl Pts',(-37.9943792094053,-30.8263126598247,
0.));
#76170=CARTESIAN_POINT('Ctrl Pts',(-37.9943792094053,-30.8263126598247,
20.));
#76171=CARTESIAN_POINT('Ctrl Pts',(-38.0132221743517,-30.7982322399668,
0.));
#76172=CARTESIAN_POINT('Ctrl Pts',(-38.0132221743517,-30.7982322399668,
20.));
#76173=CARTESIAN_POINT('Ctrl Pts',(-38.0320451830565,-30.7701397831859,
0.));
#76174=CARTESIAN_POINT('Ctrl Pts',(-38.0320451830565,-30.7701397831859,
20.));
#76175=CARTESIAN_POINT('Ctrl Pts',(-38.0508482273931,-30.7420353031339,
0.));
#76176=CARTESIAN_POINT('Ctrl Pts',(-38.0508482273931,-30.7420353031339,
20.));
#76177=CARTESIAN_POINT('Ctrl Pts',(-38.0696312991626,-30.7139188136053,
0.));
#76178=CARTESIAN_POINT('Ctrl Pts',(-38.0696312991626,-30.7139188136053,
20.));
#76179=CARTESIAN_POINT('Ctrl Pts',(-38.088394390128,-30.6857903284809,0.));
#76180=CARTESIAN_POINT('Ctrl Pts',(-38.088394390128,-30.6857903284809,20.));
#76181=CARTESIAN_POINT('Ctrl Pts',(-38.1071374920373,-30.6576498616875,
0.));
#76182=CARTESIAN_POINT('Ctrl Pts',(-38.1071374920373,-30.6576498616875,
20.));
#76183=CARTESIAN_POINT('Ctrl Pts',(-38.125860596649,-30.6294974271553,0.));
#76184=CARTESIAN_POINT('Ctrl Pts',(-38.125860596649,-30.6294974271553,20.));
#76185=CARTESIAN_POINT('Ctrl Pts',(-38.1445636957629,-30.6013330387674,
0.));
#76186=CARTESIAN_POINT('Ctrl Pts',(-38.1445636957629,-30.6013330387674,
20.));
#76187=CARTESIAN_POINT('Ctrl Pts',(-38.1632467812242,-30.5731567103519,
0.));
#76188=CARTESIAN_POINT('Ctrl Pts',(-38.1632467812242,-30.5731567103519,
20.));
#76189=CARTESIAN_POINT('Ctrl Pts',(-38.1819098449085,-30.5449684557073,
0.));
#76190=CARTESIAN_POINT('Ctrl Pts',(-38.1819098449085,-30.5449684557073,
20.));
#76191=CARTESIAN_POINT('Ctrl Pts',(-38.2005528787125,-30.5167682886194,
0.));
#76192=CARTESIAN_POINT('Ctrl Pts',(-38.2005528787125,-30.5167682886194,
20.));
#76193=CARTESIAN_POINT('Ctrl Pts',(-38.2191758745422,-30.4885562228796,
0.));
#76194=CARTESIAN_POINT('Ctrl Pts',(-38.2191758745422,-30.4885562228796,
20.));
#76195=CARTESIAN_POINT('Ctrl Pts',(-38.2377788243005,-30.460332272307,0.));
#76196=CARTESIAN_POINT('Ctrl Pts',(-38.2377788243005,-30.460332272307,20.));
#76197=CARTESIAN_POINT('Ctrl Pts',(-38.2563617198829,-30.4320964507535,
0.));
#76198=CARTESIAN_POINT('Ctrl Pts',(-38.2563617198829,-30.4320964507535,
20.));
#76199=CARTESIAN_POINT('Ctrl Pts',(-38.2749245531853,-30.4038487720928,
0.));
#76200=CARTESIAN_POINT('Ctrl Pts',(-38.2749245531853,-30.4038487720928,
20.));
#76201=CARTESIAN_POINT('Ctrl Pts',(-38.2934673161074,-30.3755892502132,
0.));
#76202=CARTESIAN_POINT('Ctrl Pts',(-38.2934673161074,-30.3755892502132,
20.));
#76203=CARTESIAN_POINT('Ctrl Pts',(-38.3119900005578,-30.3473178990095,
0.));
#76204=CARTESIAN_POINT('Ctrl Pts',(-38.3119900005578,-30.3473178990095,
20.));
#76205=CARTESIAN_POINT('Ctrl Pts',(-38.3304925984593,-30.3190347323738,
0.));
#76206=CARTESIAN_POINT('Ctrl Pts',(-38.3304925984593,-30.3190347323738,
20.));
#76207=CARTESIAN_POINT('Ctrl Pts',(-38.3489751017513,-30.2907397641919,
0.));
#76208=CARTESIAN_POINT('Ctrl Pts',(-38.3489751017513,-30.2907397641919,
20.));
#76209=CARTESIAN_POINT('Ctrl Pts',(-38.3674375023871,-30.2624330083488,
0.));
#76210=CARTESIAN_POINT('Ctrl Pts',(-38.3674375023871,-30.2624330083488,
20.));
#76211=CARTESIAN_POINT('Ctrl Pts',(-38.3858797923318,-30.2341144787313,
0.));
#76212=CARTESIAN_POINT('Ctrl Pts',(-38.3858797923318,-30.2341144787313,
20.));
#76213=CARTESIAN_POINT('Ctrl Pts',(-38.4043019635603,-30.2057841892317,
0.));
#76214=CARTESIAN_POINT('Ctrl Pts',(-38.4043019635603,-30.2057841892317,
20.));
#76215=CARTESIAN_POINT('Ctrl Pts',(-38.4227040080549,-30.1774421537519,
0.));
#76216=CARTESIAN_POINT('Ctrl Pts',(-38.4227040080549,-30.1774421537519,
20.));
#76217=CARTESIAN_POINT('Ctrl Pts',(-38.4410859178039,-30.1490883862047,
0.));
#76218=CARTESIAN_POINT('Ctrl Pts',(-38.4410859178039,-30.1490883862047,
20.));
#76219=CARTESIAN_POINT('Ctrl Pts',(-38.4594476848032,-30.1207229005118,
0.));
#76220=CARTESIAN_POINT('Ctrl Pts',(-38.4594476848032,-30.1207229005118,
20.));
#76221=CARTESIAN_POINT('Ctrl Pts',(-38.4777893010568,-30.0923457106026,
0.));
#76222=CARTESIAN_POINT('Ctrl Pts',(-38.4777893010568,-30.0923457106026,
20.));
#76223=CARTESIAN_POINT('Ctrl Pts',(-38.4961107585777,-30.0639568304126,
0.));
#76224=CARTESIAN_POINT('Ctrl Pts',(-38.4961107585777,-30.0639568304126,
20.));
#76225=CARTESIAN_POINT('Ctrl Pts',(-38.5144120493894,-30.0355562738816,
0.));
#76226=CARTESIAN_POINT('Ctrl Pts',(-38.5144120493894,-30.0355562738816,
20.));
#76227=CARTESIAN_POINT('Ctrl Pts',(-38.532693165526,-30.0071440549534,0.));
#76228=CARTESIAN_POINT('Ctrl Pts',(-38.532693165526,-30.0071440549534,20.));
#76229=CARTESIAN_POINT('Ctrl Pts',(-38.5509540990321,-29.978720187576,0.));
#76230=CARTESIAN_POINT('Ctrl Pts',(-38.5509540990321,-29.978720187576,20.));
#76231=CARTESIAN_POINT('Ctrl Pts',(-38.5691948419622,-29.9502846857025,
0.));
#76232=CARTESIAN_POINT('Ctrl Pts',(-38.5691948419622,-29.9502846857025,
20.));
#76233=CARTESIAN_POINT('Ctrl Pts',(-38.5874153863803,-29.9218375632917,
0.));
#76234=CARTESIAN_POINT('Ctrl Pts',(-38.5874153863803,-29.9218375632917,
20.));
#76235=CARTESIAN_POINT('Ctrl Pts',(-38.6056157243597,-29.8933788343089,
0.));
#76236=CARTESIAN_POINT('Ctrl Pts',(-38.6056157243597,-29.8933788343089,
20.));
#76237=CARTESIAN_POINT('Ctrl Pts',(-38.6237958479822,-29.864908512726,0.));
#76238=CARTESIAN_POINT('Ctrl Pts',(-38.6237958479822,-29.864908512726,20.));
#76239=CARTESIAN_POINT('Ctrl Pts',(-38.6419557493389,-29.8364266125215,
0.));
#76240=CARTESIAN_POINT('Ctrl Pts',(-38.6419557493389,-29.8364266125215,
20.));
#76241=CARTESIAN_POINT('Ctrl Pts',(-38.66009542053,-29.8079331476799,0.));
#76242=CARTESIAN_POINT('Ctrl Pts',(-38.66009542053,-29.8079331476799,20.));
#76243=CARTESIAN_POINT('Ctrl Pts',(-38.6782148536649,-29.7794281321916,
0.));
#76244=CARTESIAN_POINT('Ctrl Pts',(-38.6782148536649,-29.7794281321916,
20.));
#76245=CARTESIAN_POINT('Ctrl Pts',(-38.6963140408627,-29.7509115800524,
0.));
#76246=CARTESIAN_POINT('Ctrl Pts',(-38.6963140408627,-29.7509115800524,
20.));
#76247=CARTESIAN_POINT('Ctrl Pts',(-38.7143929742521,-29.7223835052637,
0.));
#76248=CARTESIAN_POINT('Ctrl Pts',(-38.7143929742521,-29.7223835052637,
20.));
#76249=CARTESIAN_POINT('Ctrl Pts',(-38.7324516459718,-29.6938439218325,
0.));
#76250=CARTESIAN_POINT('Ctrl Pts',(-38.7324516459718,-29.6938439218325,
20.));
#76251=CARTESIAN_POINT('Ctrl Pts',(-38.7504900481697,-29.6652928437714,
0.));
#76252=CARTESIAN_POINT('Ctrl Pts',(-38.7504900481697,-29.6652928437714,
20.));
#76253=CARTESIAN_POINT('Ctrl Pts',(-38.7685081730036,-29.6367302850988,
0.));
#76254=CARTESIAN_POINT('Ctrl Pts',(-38.7685081730036,-29.6367302850988,
20.));
#76255=CARTESIAN_POINT('Ctrl Pts',(-38.7865060126402,-29.6081562598384,
0.));
#76256=CARTESIAN_POINT('Ctrl Pts',(-38.7865060126402,-29.6081562598384,
20.));
#76257=CARTESIAN_POINT('Ctrl Pts',(-38.8044835592559,-29.5795707820205,
0.));
#76258=CARTESIAN_POINT('Ctrl Pts',(-38.8044835592559,-29.5795707820205,
20.));
#76259=CARTESIAN_POINT('Ctrl Pts',(-38.8224408050366,-29.5509738656807,
0.));
#76260=CARTESIAN_POINT('Ctrl Pts',(-38.8224408050366,-29.5509738656807,
20.));
#76261=CARTESIAN_POINT('Ctrl Pts',(-38.8403777421773,-29.5223655248609,
0.));
#76262=CARTESIAN_POINT('Ctrl Pts',(-38.8403777421773,-29.5223655248609,
20.));
#76263=CARTESIAN_POINT('Ctrl Pts',(-38.8582943628826,-29.4937457736083,
0.));
#76264=CARTESIAN_POINT('Ctrl Pts',(-38.8582943628826,-29.4937457736083,
20.));
#76265=CARTESIAN_POINT('Ctrl Pts',(-38.8761906593666,-29.4651146259764,
0.));
#76266=CARTESIAN_POINT('Ctrl Pts',(-38.8761906593666,-29.4651146259764,
20.));
#76267=CARTESIAN_POINT('Ctrl Pts',(-38.8940666238533,-29.4364720960241,
0.));
#76268=CARTESIAN_POINT('Ctrl Pts',(-38.8940666238533,-29.4364720960241,
20.));
#76269=CARTESIAN_POINT('Ctrl Pts',(-38.9119222485755,-29.4078181978158,
0.));
#76270=CARTESIAN_POINT('Ctrl Pts',(-38.9119222485755,-29.4078181978158,
20.));
#76271=CARTESIAN_POINT('Ctrl Pts',(-38.9297575257761,-29.3791529454216,
0.));
#76272=CARTESIAN_POINT('Ctrl Pts',(-38.9297575257761,-29.3791529454216,
20.));
#76273=CARTESIAN_POINT('Ctrl Pts',(-38.9475724477072,-29.3504763529173,
0.));
#76274=CARTESIAN_POINT('Ctrl Pts',(-38.9475724477072,-29.3504763529173,
20.));
#76275=CARTESIAN_POINT('Ctrl Pts',(-38.9653670066308,-29.3217884343845,
0.));
#76276=CARTESIAN_POINT('Ctrl Pts',(-38.9653670066308,-29.3217884343845,
20.));
#76277=CARTESIAN_POINT('Ctrl Pts',(-38.9831411948183,-29.2930892039104,
0.));
#76278=CARTESIAN_POINT('Ctrl Pts',(-38.9831411948183,-29.2930892039104,
20.));
#76279=CARTESIAN_POINT('Ctrl Pts',(-39.0008950045503,-29.2643786755883,
0.));
#76280=CARTESIAN_POINT('Ctrl Pts',(-39.0008950045503,-29.2643786755883,
20.));
#76281=CARTESIAN_POINT('Ctrl Pts',(-39.0186284281173,-29.2356568635168,
0.));
#76282=CARTESIAN_POINT('Ctrl Pts',(-39.0186284281173,-29.2356568635168,
20.));
#76283=CARTESIAN_POINT('Ctrl Pts',(-39.0363414578191,-29.2069237818005,
0.));
#76284=CARTESIAN_POINT('Ctrl Pts',(-39.0363414578191,-29.2069237818005,
20.));
#76285=CARTESIAN_POINT('Ctrl Pts',(-39.054034085965,-29.1781794445493,0.));
#76286=CARTESIAN_POINT('Ctrl Pts',(-39.054034085965,-29.1781794445493,20.));
#76287=CARTESIAN_POINT('Ctrl Pts',(-39.0717063048737,-29.1494238658788,
0.));
#76288=CARTESIAN_POINT('Ctrl Pts',(-39.0717063048737,-29.1494238658788,
20.));
#76289=CARTESIAN_POINT('Ctrl Pts',(-39.0893581068737,-29.1206570599103,
0.));
#76290=CARTESIAN_POINT('Ctrl Pts',(-39.0893581068737,-29.1206570599103,
20.));
#76291=CARTESIAN_POINT('Ctrl Pts',(-39.106989484303,-29.0918790407708,0.));
#76292=CARTESIAN_POINT('Ctrl Pts',(-39.106989484303,-29.0918790407708,20.));
#76293=CARTESIAN_POINT('Ctrl Pts',(-39.1246004295092,-29.0630898225929,
0.));
#76294=CARTESIAN_POINT('Ctrl Pts',(-39.1246004295092,-29.0630898225929,
20.));
#76295=CARTESIAN_POINT('Ctrl Pts',(-39.1421909348497,-29.034289419515,0.));
#76296=CARTESIAN_POINT('Ctrl Pts',(-39.1421909348497,-29.034289419515,20.));
#76297=CARTESIAN_POINT('Ctrl Pts',(-39.1597609926911,-29.0054778456813,
0.));
#76298=CARTESIAN_POINT('Ctrl Pts',(-39.1597609926911,-29.0054778456813,
20.));
#76299=CARTESIAN_POINT('Ctrl Pts',(-39.1773105954099,-28.9766551152413,
0.));
#76300=CARTESIAN_POINT('Ctrl Pts',(-39.1773105954099,-28.9766551152413,
20.));
#76301=CARTESIAN_POINT('Ctrl Pts',(-39.1948397353917,-28.9478212423503,
0.));
#76302=CARTESIAN_POINT('Ctrl Pts',(-39.1948397353917,-28.9478212423503,
20.));
#76303=CARTESIAN_POINT('Ctrl Pts',(-39.2123484050317,-28.9189762411689,
0.));
#76304=CARTESIAN_POINT('Ctrl Pts',(-39.2123484050317,-28.9189762411689,
20.));
#76305=CARTESIAN_POINT('Ctrl Pts',(-39.2298365967351,-28.8901201258634,
0.));
#76306=CARTESIAN_POINT('Ctrl Pts',(-39.2298365967351,-28.8901201258634,
20.));
#76307=CARTESIAN_POINT('Ctrl Pts',(-39.2473043029163,-28.8612529106058,
0.));
#76308=CARTESIAN_POINT('Ctrl Pts',(-39.2473043029163,-28.8612529106058,
20.));
#76309=CARTESIAN_POINT('Ctrl Pts',(-39.2647515159997,-28.8323746095736,
0.));
#76310=CARTESIAN_POINT('Ctrl Pts',(-39.2647515159997,-28.8323746095736,
20.));
#76311=CARTESIAN_POINT('Ctrl Pts',(-39.2821782284193,-28.80348523695,0.));
#76312=CARTESIAN_POINT('Ctrl Pts',(-39.2821782284193,-28.80348523695,20.));
#76313=CARTESIAN_POINT('Ctrl Pts',(-39.2995844326181,-28.7745848069238,
0.));
#76314=CARTESIAN_POINT('Ctrl Pts',(-39.2995844326181,-28.7745848069238,
20.));
#76315=CARTESIAN_POINT('Ctrl Pts',(-39.316970121049,-28.7456733336894,0.));
#76316=CARTESIAN_POINT('Ctrl Pts',(-39.316970121049,-28.7456733336894,20.));
#76317=CARTESIAN_POINT('Ctrl Pts',(-39.3343352861746,-28.7167508314468,
0.));
#76318=CARTESIAN_POINT('Ctrl Pts',(-39.3343352861746,-28.7167508314468,
20.));
#76319=CARTESIAN_POINT('Ctrl Pts',(-39.3516799204672,-28.6878173144015,
0.));
#76320=CARTESIAN_POINT('Ctrl Pts',(-39.3516799204672,-28.6878173144015,
20.));
#76321=CARTESIAN_POINT('Ctrl Pts',(-39.3690040164086,-28.6588727967647,
0.));
#76322=CARTESIAN_POINT('Ctrl Pts',(-39.3690040164086,-28.6588727967647,
20.));
#76323=CARTESIAN_POINT('Ctrl Pts',(-39.3863075664906,-28.6299172927529,
0.));
#76324=CARTESIAN_POINT('Ctrl Pts',(-39.3863075664906,-28.6299172927529,
20.));
#76325=CARTESIAN_POINT('Ctrl Pts',(-39.4035905632141,-28.600950816588,0.));
#76326=CARTESIAN_POINT('Ctrl Pts',(-39.4035905632141,-28.600950816588,20.));
#76327=CARTESIAN_POINT('Ctrl Pts',(-39.4208529990894,-28.5719733824975,
0.));
#76328=CARTESIAN_POINT('Ctrl Pts',(-39.4208529990894,-28.5719733824975,
20.));
#76329=CARTESIAN_POINT('Ctrl Pts',(-39.4380948666368,-28.5429850047148,
0.));
#76330=CARTESIAN_POINT('Ctrl Pts',(-39.4380948666368,-28.5429850047148,
20.));
#76331=CARTESIAN_POINT('Ctrl Pts',(-39.4553161583861,-28.5139856974786,
0.));
#76332=CARTESIAN_POINT('Ctrl Pts',(-39.4553161583861,-28.5139856974786,
20.));
#76333=CARTESIAN_POINT('Ctrl Pts',(-39.4725168668771,-28.4849754750331,
0.));
#76334=CARTESIAN_POINT('Ctrl Pts',(-39.4725168668771,-28.4849754750331,
20.));
#76335=CARTESIAN_POINT('Ctrl Pts',(-39.4896969846589,-28.455954351628,0.));
#76336=CARTESIAN_POINT('Ctrl Pts',(-39.4896969846589,-28.455954351628,20.));
#76337=CARTESIAN_POINT('Ctrl Pts',(-39.5068565042907,-28.4269223415187,
0.));
#76338=CARTESIAN_POINT('Ctrl Pts',(-39.5068565042907,-28.4269223415187,
20.));
#76339=CARTESIAN_POINT('Ctrl Pts',(-39.5239954183412,-28.3978794589661,
0.));
#76340=CARTESIAN_POINT('Ctrl Pts',(-39.5239954183412,-28.3978794589661,
20.));
#76341=CARTESIAN_POINT('Ctrl Pts',(-39.5411137193887,-28.3688257182364,
0.));
#76342=CARTESIAN_POINT('Ctrl Pts',(-39.5411137193887,-28.3688257182364,
20.));
#76343=CARTESIAN_POINT('Ctrl Pts',(-39.5582114000212,-28.3397611336014,
0.));
#76344=CARTESIAN_POINT('Ctrl Pts',(-39.5582114000212,-28.3397611336014,
20.));
#76345=CARTESIAN_POINT('Ctrl Pts',(-39.5752884528361,-28.3106857193381,
0.));
#76346=CARTESIAN_POINT('Ctrl Pts',(-39.5752884528361,-28.3106857193381,
20.));
#76347=CARTESIAN_POINT('Ctrl Pts',(-39.5923448704403,-28.2815994897291,
0.));
#76348=CARTESIAN_POINT('Ctrl Pts',(-39.5923448704403,-28.2815994897291,
20.));
#76349=CARTESIAN_POINT('Ctrl Pts',(-39.6093806454502,-28.2525024590626,
0.));
#76350=CARTESIAN_POINT('Ctrl Pts',(-39.6093806454502,-28.2525024590626,
20.));
#76351=CARTESIAN_POINT('Ctrl Pts',(-39.6263957704923,-28.2233946416323,
0.));
#76352=CARTESIAN_POINT('Ctrl Pts',(-39.6263957704923,-28.2233946416323,
20.));
#76353=CARTESIAN_POINT('Ctrl Pts',(-39.6433902382029,-28.1942760517371,
0.));
#76354=CARTESIAN_POINT('Ctrl Pts',(-39.6433902382029,-28.1942760517371,
20.));
#76355=CARTESIAN_POINT('Ctrl Pts',(-39.6603640412281,-28.1651467036817,
0.));
#76356=CARTESIAN_POINT('Ctrl Pts',(-39.6603640412281,-28.1651467036817,
20.));
#76357=CARTESIAN_POINT('Ctrl Pts',(-39.6773171722241,-28.136006611776,0.));
#76358=CARTESIAN_POINT('Ctrl Pts',(-39.6773171722241,-28.136006611776,20.));
#76359=CARTESIAN_POINT('Ctrl Pts',(-39.6942496238565,-28.1068557903356,
0.));
#76360=CARTESIAN_POINT('Ctrl Pts',(-39.6942496238565,-28.1068557903356,
20.));
#76361=CARTESIAN_POINT('Ctrl Pts',(-39.7111613888006,-28.0776942536814,
0.));
#76362=CARTESIAN_POINT('Ctrl Pts',(-39.7111613888006,-28.0776942536814,
20.));
#76363=CARTESIAN_POINT('Ctrl Pts',(-39.728052459741,-28.0485220161395,0.));
#76364=CARTESIAN_POINT('Ctrl Pts',(-39.728052459741,-28.0485220161395,20.));
#76365=CARTESIAN_POINT('Ctrl Pts',(-39.7449228293718,-28.0193390920415,
0.));
#76366=CARTESIAN_POINT('Ctrl Pts',(-39.7449228293718,-28.0193390920415,
20.));
#76367=CARTESIAN_POINT('Ctrl Pts',(-39.7617724903968,-27.9901454957246,
0.));
#76368=CARTESIAN_POINT('Ctrl Pts',(-39.7617724903968,-27.9901454957246,
20.));
#76369=CARTESIAN_POINT('Ctrl Pts',(-39.7786014355293,-27.960941241531,0.));
#76370=CARTESIAN_POINT('Ctrl Pts',(-39.7786014355293,-27.960941241531,20.));
#76371=CARTESIAN_POINT('Ctrl Pts',(-39.795409657493,-27.9317263438086,0.));
#76372=CARTESIAN_POINT('Ctrl Pts',(-39.795409657493,-27.9317263438086,20.));
#76373=CARTESIAN_POINT('Ctrl Pts',(-39.8121971490214,-27.9025008169107,
0.));
#76374=CARTESIAN_POINT('Ctrl Pts',(-39.8121971490214,-27.9025008169107,
20.));
#76375=CARTESIAN_POINT('Ctrl Pts',(-39.828963902858,-27.8732646751959,0.));
#76376=CARTESIAN_POINT('Ctrl Pts',(-39.828963902858,-27.8732646751959,20.));
#76377=CARTESIAN_POINT('Ctrl Pts',(-39.845709911756,-27.8440179330284,0.));
#76378=CARTESIAN_POINT('Ctrl Pts',(-39.845709911756,-27.8440179330284,20.));
#76379=CARTESIAN_POINT('Ctrl Pts',(-39.8624351684781,-27.8147606047778,
0.));
#76380=CARTESIAN_POINT('Ctrl Pts',(-39.8624351684781,-27.8147606047778,
20.));
#76381=CARTESIAN_POINT('Ctrl Pts',(-39.8791396657966,-27.785492704819,0.));
#76382=CARTESIAN_POINT('Ctrl Pts',(-39.8791396657966,-27.785492704819,20.));
#76383=CARTESIAN_POINT('Ctrl Pts',(-39.8958233964934,-27.7562142475319,
0.));
#76384=CARTESIAN_POINT('Ctrl Pts',(-39.8958233964934,-27.7562142475319,
20.));
#76385=CARTESIAN_POINT('Ctrl Pts',(-39.9124863533599,-27.726925247302,0.));
#76386=CARTESIAN_POINT('Ctrl Pts',(-39.9124863533599,-27.726925247302,20.));
#76387=CARTESIAN_POINT('Ctrl Pts',(-39.9291285291975,-27.6976257185198,
0.));
#76388=CARTESIAN_POINT('Ctrl Pts',(-39.9291285291975,-27.6976257185198,
20.));
#76389=CARTESIAN_POINT('Ctrl Pts',(-39.9457499168175,-27.6683156755815,
0.));
#76390=CARTESIAN_POINT('Ctrl Pts',(-39.9457499168175,-27.6683156755815,
20.));
#76391=CARTESIAN_POINT('Ctrl Pts',(-39.9623505090412,-27.6389951328887,
0.));
#76392=CARTESIAN_POINT('Ctrl Pts',(-39.9623505090412,-27.6389951328887,
20.));
#76393=CARTESIAN_POINT('Ctrl Pts',(-39.9789302986995,-27.6096641048483,
0.));
#76394=CARTESIAN_POINT('Ctrl Pts',(-39.9789302986995,-27.6096641048483,
20.));
#76395=CARTESIAN_POINT('Ctrl Pts',(-39.9954892786331,-27.5803226058724,
0.));
#76396=CARTESIAN_POINT('Ctrl Pts',(-39.9954892786331,-27.5803226058724,
20.));
#76397=CARTESIAN_POINT('Ctrl Pts',(-40.0120274416924,-27.5509706503786,
0.));
#76398=CARTESIAN_POINT('Ctrl Pts',(-40.0120274416924,-27.5509706503786,
20.));
#76399=CARTESIAN_POINT('Ctrl Pts',(-40.0285447807378,-27.5216082527897,
0.));
#76400=CARTESIAN_POINT('Ctrl Pts',(-40.0285447807378,-27.5216082527897,
20.));
#76401=CARTESIAN_POINT('Ctrl Pts',(-40.045041288639,-27.4922354275335,0.));
#76402=CARTESIAN_POINT('Ctrl Pts',(-40.045041288639,-27.4922354275335,20.));
#76403=CARTESIAN_POINT('Ctrl Pts',(-40.0615169582759,-27.4628521890436,
0.));
#76404=CARTESIAN_POINT('Ctrl Pts',(-40.0615169582759,-27.4628521890436,
20.));
#76405=CARTESIAN_POINT('Ctrl Pts',(-40.077971782538,-27.4334585517582,0.));
#76406=CARTESIAN_POINT('Ctrl Pts',(-40.077971782538,-27.4334585517582,20.));
#76407=CARTESIAN_POINT('Ctrl Pts',(-40.0944057543248,-27.4040545301216,
0.));
#76408=CARTESIAN_POINT('Ctrl Pts',(-40.0944057543248,-27.4040545301216,
20.));
#76409=CARTESIAN_POINT('Ctrl Pts',(-40.1108188665452,-27.374640138583,0.));
#76410=CARTESIAN_POINT('Ctrl Pts',(-40.1108188665452,-27.374640138583,20.));
#76411=CARTESIAN_POINT('Ctrl Pts',(-40.1272111121183,-27.3452153915969,
0.));
#76412=CARTESIAN_POINT('Ctrl Pts',(-40.1272111121183,-27.3452153915969,
20.));
#76413=CARTESIAN_POINT('Ctrl Pts',(-40.1435824839731,-27.3157803036231,
0.));
#76414=CARTESIAN_POINT('Ctrl Pts',(-40.1435824839731,-27.3157803036231,
20.));
#76415=CARTESIAN_POINT('Ctrl Pts',(-40.1599329750483,-27.2863348891265,
0.));
#76416=CARTESIAN_POINT('Ctrl Pts',(-40.1599329750483,-27.2863348891265,
20.));
#76417=CARTESIAN_POINT('Ctrl Pts',(-40.1762625782924,-27.2568791625774,
0.));
#76418=CARTESIAN_POINT('Ctrl Pts',(-40.1762625782924,-27.2568791625774,
20.));
#76419=CARTESIAN_POINT('Ctrl Pts',(-40.1925712866631,-27.2274131384508,
0.));
#76420=CARTESIAN_POINT('Ctrl Pts',(-40.1925712866631,-27.2274131384508,
20.));
#76421=CARTESIAN_POINT('Ctrl Pts',(-40.2088590931287,-27.1979368312277,
0.));
#76422=CARTESIAN_POINT('Ctrl Pts',(-40.2088590931287,-27.1979368312277,
20.));
#76423=CARTESIAN_POINT('Ctrl Pts',(-40.225125990667,-27.1684502553939,0.));
#76424=CARTESIAN_POINT('Ctrl Pts',(-40.225125990667,-27.1684502553939,20.));
#76425=CARTESIAN_POINT('Ctrl Pts',(-40.2413719722657,-27.1389534254409,
0.));
#76426=CARTESIAN_POINT('Ctrl Pts',(-40.2413719722657,-27.1389534254409,
20.));
#76427=CARTESIAN_POINT('Ctrl Pts',(-40.2575970309226,-27.1094463558649,
0.));
#76428=CARTESIAN_POINT('Ctrl Pts',(-40.2575970309226,-27.1094463558649,
20.));
#76429=CARTESIAN_POINT('Ctrl Pts',(-40.2738011596454,-27.0799290611676,
0.));
#76430=CARTESIAN_POINT('Ctrl Pts',(-40.2738011596454,-27.0799290611676,
20.));
#76431=CARTESIAN_POINT('Ctrl Pts',(-40.2899843514517,-27.0504015558557,
0.));
#76432=CARTESIAN_POINT('Ctrl Pts',(-40.2899843514517,-27.0504015558557,
20.));
#76433=CARTESIAN_POINT('Ctrl Pts',(-40.3061465993685,-27.0208638544413,
0.));
#76434=CARTESIAN_POINT('Ctrl Pts',(-40.3061465993685,-27.0208638544413,
20.));
#76435=CARTESIAN_POINT('Ctrl Pts',(-40.3222878964329,-26.9913159714415,
0.));
#76436=CARTESIAN_POINT('Ctrl Pts',(-40.3222878964329,-26.9913159714415,
20.));
#76437=CARTESIAN_POINT('Ctrl Pts',(-40.3384082356913,-26.9617579213786,
0.));
#76438=CARTESIAN_POINT('Ctrl Pts',(-40.3384082356913,-26.9617579213786,
20.));
#76439=CARTESIAN_POINT('Ctrl Pts',(-40.3545076102003,-26.9321897187802,
0.));
#76440=CARTESIAN_POINT('Ctrl Pts',(-40.3545076102003,-26.9321897187802,
20.));
#76441=CARTESIAN_POINT('Ctrl Pts',(-40.3705860130263,-26.9026113781788,
0.));
#76442=CARTESIAN_POINT('Ctrl Pts',(-40.3705860130263,-26.9026113781788,
20.));
#76443=CARTESIAN_POINT('Ctrl Pts',(-40.386643437246,-26.8730229141124,0.));
#76444=CARTESIAN_POINT('Ctrl Pts',(-40.386643437246,-26.8730229141124,20.));
#76445=CARTESIAN_POINT('Ctrl Pts',(-40.4026798759458,-26.8434243411241,
0.));
#76446=CARTESIAN_POINT('Ctrl Pts',(-40.4026798759458,-26.8434243411241,
20.));
#76447=CARTESIAN_POINT('Ctrl Pts',(-40.4186953222224,-26.8138156737619,
0.));
#76448=CARTESIAN_POINT('Ctrl Pts',(-40.4186953222224,-26.8138156737619,
20.));
#76449=CARTESIAN_POINT('Ctrl Pts',(-40.4346897691821,-26.7841969265794,
0.));
#76450=CARTESIAN_POINT('Ctrl Pts',(-40.4346897691821,-26.7841969265794,
20.));
#76451=CARTESIAN_POINT('Ctrl Pts',(-40.4506632099408,-26.754568114135,0.));
#76452=CARTESIAN_POINT('Ctrl Pts',(-40.4506632099408,-26.754568114135,20.));
#76453=CARTESIAN_POINT('Ctrl Pts',(-40.4666156376241,-26.7249292509923,
0.));
#76454=CARTESIAN_POINT('Ctrl Pts',(-40.4666156376241,-26.7249292509923,
20.));
#76455=CARTESIAN_POINT('Ctrl Pts',(-40.4825470453679,-26.6952803517197,
0.));
#76456=CARTESIAN_POINT('Ctrl Pts',(-40.4825470453679,-26.6952803517197,
20.));
#76457=CARTESIAN_POINT('Ctrl Pts',(-40.4984574263178,-26.6656214308914,
0.));
#76458=CARTESIAN_POINT('Ctrl Pts',(-40.4984574263178,-26.6656214308914,
20.));
#76459=CARTESIAN_POINT('Ctrl Pts',(-40.5143467736295,-26.6359525030862,
0.));
#76460=CARTESIAN_POINT('Ctrl Pts',(-40.5143467736295,-26.6359525030862,
20.));
#76461=CARTESIAN_POINT('Ctrl Pts',(-40.5302150804687,-26.606273582888,0.));
#76462=CARTESIAN_POINT('Ctrl Pts',(-40.5302150804687,-26.606273582888,20.));
#76463=CARTESIAN_POINT('Ctrl Pts',(-40.546062340011,-26.5765846848862,0.));
#76464=CARTESIAN_POINT('Ctrl Pts',(-40.546062340011,-26.5765846848862,20.));
#76465=CARTESIAN_POINT('Ctrl Pts',(-40.5618885454414,-26.5468858236748,
0.));
#76466=CARTESIAN_POINT('Ctrl Pts',(-40.5618885454414,-26.5468858236748,
20.));
#76467=CARTESIAN_POINT('Ctrl Pts',(-40.5776936899555,-26.5171770138532,
0.));
#76468=CARTESIAN_POINT('Ctrl Pts',(-40.5776936899555,-26.5171770138532,
20.));
#76469=CARTESIAN_POINT('Ctrl Pts',(-40.5934777667583,-26.4874582700259,
0.));
#76470=CARTESIAN_POINT('Ctrl Pts',(-40.5934777667583,-26.4874582700259,
20.));
#76471=CARTESIAN_POINT('Ctrl Pts',(-40.6092407690651,-26.4577296068023,
0.));
#76472=CARTESIAN_POINT('Ctrl Pts',(-40.6092407690651,-26.4577296068023,
20.));
#76473=CARTESIAN_POINT('Ctrl Pts',(-40.6249826901011,-26.427991038797,0.));
#76474=CARTESIAN_POINT('Ctrl Pts',(-40.6249826901011,-26.427991038797,20.));
#76475=CARTESIAN_POINT('Ctrl Pts',(-40.6407035231015,-26.3982425806297,
0.));
#76476=CARTESIAN_POINT('Ctrl Pts',(-40.6407035231015,-26.3982425806297,
20.));
#76477=CARTESIAN_POINT('Ctrl Pts',(-40.6564032613109,-26.3684842469248,
0.));
#76478=CARTESIAN_POINT('Ctrl Pts',(-40.6564032613109,-26.3684842469248,
20.));
#76479=CARTESIAN_POINT('Ctrl Pts',(-40.6720818979844,-26.338716052312,0.));
#76480=CARTESIAN_POINT('Ctrl Pts',(-40.6720818979844,-26.338716052312,20.));
#76481=CARTESIAN_POINT('Ctrl Pts',(-40.6877394263869,-26.308938011426,0.));
#76482=CARTESIAN_POINT('Ctrl Pts',(-40.6877394263869,-26.308938011426,20.));
#76483=CARTESIAN_POINT('Ctrl Pts',(-40.7033758397932,-26.2791501389067,
0.));
#76484=CARTESIAN_POINT('Ctrl Pts',(-40.7033758397932,-26.2791501389067,
20.));
#76485=CARTESIAN_POINT('Ctrl Pts',(-40.7189911314882,-26.2493524493989,
0.));
#76486=CARTESIAN_POINT('Ctrl Pts',(-40.7189911314882,-26.2493524493989,
20.));
#76487=CARTESIAN_POINT('Ctrl Pts',(-40.7345852947664,-26.2195449575524,
0.));
#76488=CARTESIAN_POINT('Ctrl Pts',(-40.7345852947664,-26.2195449575524,
20.));
#76489=CARTESIAN_POINT('Ctrl Pts',(-40.7501583229328,-26.1897276780219,
0.));
#76490=CARTESIAN_POINT('Ctrl Pts',(-40.7501583229328,-26.1897276780219,
20.));
#76491=CARTESIAN_POINT('Ctrl Pts',(-40.7657102093021,-26.1599006254674,
0.));
#76492=CARTESIAN_POINT('Ctrl Pts',(-40.7657102093021,-26.1599006254674,
20.));
#76493=CARTESIAN_POINT('Ctrl Pts',(-40.7812409471992,-26.1300638145535,
0.));
#76494=CARTESIAN_POINT('Ctrl Pts',(-40.7812409471992,-26.1300638145535,
20.));
#76495=CARTESIAN_POINT('Ctrl Pts',(-40.7967505299588,-26.1002172599501,
0.));
#76496=CARTESIAN_POINT('Ctrl Pts',(-40.7967505299588,-26.1002172599501,
20.));
#76497=CARTESIAN_POINT('Ctrl Pts',(-40.8122389509256,-26.0703609763318,
0.));
#76498=CARTESIAN_POINT('Ctrl Pts',(-40.8122389509256,-26.0703609763318,
20.));
#76499=CARTESIAN_POINT('Ctrl Pts',(-40.8277062034539,-26.0404949783787,
0.));
#76500=CARTESIAN_POINT('Ctrl Pts',(-40.8277062034539,-26.0404949783787,
20.));
#76501=CARTESIAN_POINT('Ctrl Pts',(-40.843152280908,-26.0106192807756,0.));
#76502=CARTESIAN_POINT('Ctrl Pts',(-40.843152280908,-26.0106192807756,20.));
#76503=CARTESIAN_POINT('Ctrl Pts',(-40.8585771766627,-25.9807338982121,
0.));
#76504=CARTESIAN_POINT('Ctrl Pts',(-40.8585771766627,-25.9807338982121,
20.));
#76505=CARTESIAN_POINT('Ctrl Pts',(-40.8739808841024,-25.950838845383,0.));
#76506=CARTESIAN_POINT('Ctrl Pts',(-40.8739808841024,-25.950838845383,20.));
#76507=CARTESIAN_POINT('Ctrl Pts',(-40.8893633966224,-25.9209341369879,
0.));
#76508=CARTESIAN_POINT('Ctrl Pts',(-40.8893633966224,-25.9209341369879,
20.));
#76509=CARTESIAN_POINT('Ctrl Pts',(-40.9047247076274,-25.891019787731,0.));
#76510=CARTESIAN_POINT('Ctrl Pts',(-40.9047247076274,-25.891019787731,20.));
#76511=CARTESIAN_POINT('Ctrl Pts',(-40.9200648105322,-25.861095812322,0.));
#76512=CARTESIAN_POINT('Ctrl Pts',(-40.9200648105322,-25.861095812322,20.));
#76513=CARTESIAN_POINT('Ctrl Pts',(-40.9353836987613,-25.8311622254754,
0.));
#76514=CARTESIAN_POINT('Ctrl Pts',(-40.9353836987613,-25.8311622254754,
20.));
#76515=CARTESIAN_POINT('Ctrl Pts',(-40.9506813657491,-25.8012190419102,
0.));
#76516=CARTESIAN_POINT('Ctrl Pts',(-40.9506813657491,-25.8012190419102,
20.));
#76517=CARTESIAN_POINT('Ctrl Pts',(-40.9659578049399,-25.7712662763511,
0.));
#76518=CARTESIAN_POINT('Ctrl Pts',(-40.9659578049399,-25.7712662763511,
20.));
#76519=CARTESIAN_POINT('Ctrl Pts',(-40.981213009789,-25.7413039435271,0.));
#76520=CARTESIAN_POINT('Ctrl Pts',(-40.981213009789,-25.7413039435271,20.));
#76521=CARTESIAN_POINT('Ctrl Pts',(-40.9964469737613,-25.7113320581728,
0.));
#76522=CARTESIAN_POINT('Ctrl Pts',(-40.9964469737613,-25.7113320581728,
20.));
#76523=CARTESIAN_POINT('Ctrl Pts',(-41.0116596903317,-25.6813506350271,
0.));
#76524=CARTESIAN_POINT('Ctrl Pts',(-41.0116596903317,-25.6813506350271,
20.));
#76525=CARTESIAN_POINT('Ctrl Pts',(-41.0268511529852,-25.6513596888338,
0.));
#76526=CARTESIAN_POINT('Ctrl Pts',(-41.0268511529852,-25.6513596888338,
20.));
#76527=CARTESIAN_POINT('Ctrl Pts',(-41.0420213552163,-25.6213592343415,
0.));
#76528=CARTESIAN_POINT('Ctrl Pts',(-41.0420213552163,-25.6213592343415,
20.));
#76529=CARTESIAN_POINT('Ctrl Pts',(-41.05717029053,-25.5913492863038,0.));
#76530=CARTESIAN_POINT('Ctrl Pts',(-41.05717029053,-25.5913492863038,20.));
#76531=CARTESIAN_POINT('Ctrl Pts',(-41.072297952441,-25.5613298594791,0.));
#76532=CARTESIAN_POINT('Ctrl Pts',(-41.072297952441,-25.5613298594791,20.));
#76533=CARTESIAN_POINT('Ctrl Pts',(-41.0874043344745,-25.5313009686309,
0.));
#76534=CARTESIAN_POINT('Ctrl Pts',(-41.0874043344745,-25.5313009686309,
20.));
#76535=CARTESIAN_POINT('Ctrl Pts',(-41.1024894301655,-25.5012626285275,
0.));
#76536=CARTESIAN_POINT('Ctrl Pts',(-41.1024894301655,-25.5012626285275,
20.));
#76537=CARTESIAN_POINT('Ctrl Pts',(-41.1175532330596,-25.4712148539422,
0.));
#76538=CARTESIAN_POINT('Ctrl Pts',(-41.1175532330596,-25.4712148539422,
20.));
#76539=CARTESIAN_POINT('Ctrl Pts',(-41.132595736712,-25.4411576596529,0.));
#76540=CARTESIAN_POINT('Ctrl Pts',(-41.132595736712,-25.4411576596529,20.));
#76541=CARTESIAN_POINT('Ctrl Pts',(-41.1476169346881,-25.4110910604425,
0.));
#76542=CARTESIAN_POINT('Ctrl Pts',(-41.1476169346881,-25.4110910604425,
20.));
#76543=CARTESIAN_POINT('Ctrl Pts',(-41.1626168205634,-25.3810150710984,
0.));
#76544=CARTESIAN_POINT('Ctrl Pts',(-41.1626168205634,-25.3810150710984,
20.));
#76545=CARTESIAN_POINT('Ctrl Pts',(-41.1775953879232,-25.3509297064131,
0.));
#76546=CARTESIAN_POINT('Ctrl Pts',(-41.1775953879232,-25.3509297064131,
20.));
#76547=CARTESIAN_POINT('Ctrl Pts',(-41.1925526303629,-25.3208349811839,
0.));
#76548=CARTESIAN_POINT('Ctrl Pts',(-41.1925526303629,-25.3208349811839,
20.));
#76549=CARTESIAN_POINT('Ctrl Pts',(-41.2074885414881,-25.2907309102128,
0.));
#76550=CARTESIAN_POINT('Ctrl Pts',(-41.2074885414881,-25.2907309102128,
20.));
#76551=CARTESIAN_POINT('Ctrl Pts',(-41.2224031149147,-25.2606175083067,
0.));
#76552=CARTESIAN_POINT('Ctrl Pts',(-41.2224031149147,-25.2606175083067,
20.));
#76553=CARTESIAN_POINT('Ctrl Pts',(-41.2372963442684,-25.2304947902774,
0.));
#76554=CARTESIAN_POINT('Ctrl Pts',(-41.2372963442684,-25.2304947902774,
20.));
#76555=CARTESIAN_POINT('Ctrl Pts',(-41.2521682231854,-25.2003627709414,
0.));
#76556=CARTESIAN_POINT('Ctrl Pts',(-41.2521682231854,-25.2003627709414,
20.));
#76557=CARTESIAN_POINT('Ctrl Pts',(-41.2670187453114,-25.1702214651198,
0.));
#76558=CARTESIAN_POINT('Ctrl Pts',(-41.2670187453114,-25.1702214651198,
20.));
#76559=CARTESIAN_POINT('Ctrl Pts',(-41.2818479043026,-25.1400708876386,
0.));
#76560=CARTESIAN_POINT('Ctrl Pts',(-41.2818479043026,-25.1400708876386,
20.));
#76561=CARTESIAN_POINT('Ctrl Pts',(-41.2966556938255,-25.1099110533288,
0.));
#76562=CARTESIAN_POINT('Ctrl Pts',(-41.2966556938255,-25.1099110533288,
20.));
#76563=CARTESIAN_POINT('Ctrl Pts',(-41.3114421075567,-25.0797419770258,
0.));
#76564=CARTESIAN_POINT('Ctrl Pts',(-41.3114421075567,-25.0797419770258,
20.));
#76565=CARTESIAN_POINT('Ctrl Pts',(-41.3262071391823,-25.0495636735701,
0.));
#76566=CARTESIAN_POINT('Ctrl Pts',(-41.3262071391823,-25.0495636735701,
20.));
#76567=CARTESIAN_POINT('Ctrl Pts',(-41.3409507823989,-25.0193761578067,
0.));
#76568=CARTESIAN_POINT('Ctrl Pts',(-41.3409507823989,-25.0193761578067,
20.));
#76569=CARTESIAN_POINT('Ctrl Pts',(-41.3556730309131,-24.9891794445855,
0.));
#76570=CARTESIAN_POINT('Ctrl Pts',(-41.3556730309131,-24.9891794445855,
20.));
#76571=CARTESIAN_POINT('Ctrl Pts',(-41.3703738784418,-24.9589735487609,
0.));
#76572=CARTESIAN_POINT('Ctrl Pts',(-41.3703738784418,-24.9589735487609,
20.));
#76573=CARTESIAN_POINT('Ctrl Pts',(-41.3850533187123,-24.9287584851923,
0.));
#76574=CARTESIAN_POINT('Ctrl Pts',(-41.3850533187123,-24.9287584851923,
20.));
#76575=CARTESIAN_POINT('Ctrl Pts',(-41.3997113454618,-24.8985342687436,
0.));
#76576=CARTESIAN_POINT('Ctrl Pts',(-41.3997113454618,-24.8985342687436,
20.));
#76577=CARTESIAN_POINT('Ctrl Pts',(-41.4143479524375,-24.8683009142837,
0.));
#76578=CARTESIAN_POINT('Ctrl Pts',(-41.4143479524375,-24.8683009142837,
20.));
#76579=CARTESIAN_POINT('Ctrl Pts',(-41.4289631333969,-24.8380584366858,
0.));
#76580=CARTESIAN_POINT('Ctrl Pts',(-41.4289631333969,-24.8380584366858,
20.));
#76581=CARTESIAN_POINT('Ctrl Pts',(-41.4435568821071,-24.8078068508284,
0.));
#76582=CARTESIAN_POINT('Ctrl Pts',(-41.4435568821071,-24.8078068508284,
20.));
#76583=CARTESIAN_POINT('Ctrl Pts',(-41.4581291923457,-24.7775461715943,
0.));
#76584=CARTESIAN_POINT('Ctrl Pts',(-41.4581291923457,-24.7775461715943,
20.));
#76585=CARTESIAN_POINT('Ctrl Pts',(-41.4726800579006,-24.7472764138709,
0.));
#76586=CARTESIAN_POINT('Ctrl Pts',(-41.4726800579006,-24.7472764138709,
20.));
#76587=CARTESIAN_POINT('Ctrl Pts',(-41.4872094725702,-24.7169975925505,
0.));
#76588=CARTESIAN_POINT('Ctrl Pts',(-41.4872094725702,-24.7169975925505,
20.));
#76589=CARTESIAN_POINT('Ctrl Pts',(-41.5017174301628,-24.68670972253,0.));
#76590=CARTESIAN_POINT('Ctrl Pts',(-41.5017174301628,-24.68670972253,20.));
#76591=CARTESIAN_POINT('Ctrl Pts',(-41.516203924497,-24.6564128187107,0.));
#76592=CARTESIAN_POINT('Ctrl Pts',(-41.516203924497,-24.6564128187107,20.));
#76593=CARTESIAN_POINT('Ctrl Pts',(-41.5306689494012,-24.626106895999,0.));
#76594=CARTESIAN_POINT('Ctrl Pts',(-41.5306689494012,-24.626106895999,20.));
#76595=CARTESIAN_POINT('Ctrl Pts',(-41.545112498714,-24.5957919693057,0.));
#76596=CARTESIAN_POINT('Ctrl Pts',(-41.545112498714,-24.5957919693057,20.));
#76597=CARTESIAN_POINT('Ctrl Pts',(-41.5595345662842,-24.5654680535465,
0.));
#76598=CARTESIAN_POINT('Ctrl Pts',(-41.5595345662842,-24.5654680535465,
20.));
#76599=CARTESIAN_POINT('Ctrl Pts',(-41.5739351459709,-24.5351351636416,
0.));
#76600=CARTESIAN_POINT('Ctrl Pts',(-41.5739351459709,-24.5351351636416,
20.));
#76601=CARTESIAN_POINT('Ctrl Pts',(-41.5883142316433,-24.5047933145158,
0.));
#76602=CARTESIAN_POINT('Ctrl Pts',(-41.5883142316433,-24.5047933145158,
20.));
#76603=CARTESIAN_POINT('Ctrl Pts',(-41.6026718171809,-24.4744425210985,
0.));
#76604=CARTESIAN_POINT('Ctrl Pts',(-41.6026718171809,-24.4744425210985,
20.));
#76605=CARTESIAN_POINT('Ctrl Pts',(-41.6170078964732,-24.4440827983238,
0.));
#76606=CARTESIAN_POINT('Ctrl Pts',(-41.6170078964732,-24.4440827983238,
20.));
#76607=CARTESIAN_POINT('Ctrl Pts',(-41.6313224634201,-24.4137141611302,
0.));
#76608=CARTESIAN_POINT('Ctrl Pts',(-41.6313224634201,-24.4137141611302,
20.));
#76609=CARTESIAN_POINT('Ctrl Pts',(-41.6456155119319,-24.3833366244611,
0.));
#76610=CARTESIAN_POINT('Ctrl Pts',(-41.6456155119319,-24.3833366244611,
20.));
#76611=CARTESIAN_POINT('Ctrl Pts',(-41.6598870359289,-24.3529502032644,
0.));
#76612=CARTESIAN_POINT('Ctrl Pts',(-41.6598870359289,-24.3529502032644,
20.));
#76613=CARTESIAN_POINT('Ctrl Pts',(-41.6741370293416,-24.3225549124927,
0.));
#76614=CARTESIAN_POINT('Ctrl Pts',(-41.6741370293416,-24.3225549124927,
20.));
#76615=CARTESIAN_POINT('Ctrl Pts',(-41.6883654861106,-24.2921507671029,
0.));
#76616=CARTESIAN_POINT('Ctrl Pts',(-41.6883654861106,-24.2921507671029,
20.));
#76617=CARTESIAN_POINT('Ctrl Pts',(-41.7025724001866,-24.2617377820568,
0.));
#76618=CARTESIAN_POINT('Ctrl Pts',(-41.7025724001866,-24.2617377820568,
20.));
#76619=CARTESIAN_POINT('Ctrl Pts',(-41.7167577655309,-24.2313159723205,
0.));
#76620=CARTESIAN_POINT('Ctrl Pts',(-41.7167577655309,-24.2313159723205,
20.));
#76621=CARTESIAN_POINT('Ctrl Pts',(-41.7309215761147,-24.2008853528648,
0.));
#76622=CARTESIAN_POINT('Ctrl Pts',(-41.7309215761147,-24.2008853528648,
20.));
#76623=CARTESIAN_POINT('Ctrl Pts',(-41.7450638259196,-24.1704459386651,
0.));
#76624=CARTESIAN_POINT('Ctrl Pts',(-41.7450638259196,-24.1704459386651,
20.));
#76625=CARTESIAN_POINT('Ctrl Pts',(-41.7591845089374,-24.1399977447013,
0.));
#76626=CARTESIAN_POINT('Ctrl Pts',(-41.7591845089374,-24.1399977447013,
20.));
#76627=CARTESIAN_POINT('Ctrl Pts',(-41.7732836191701,-24.1095407859578,
0.));
#76628=CARTESIAN_POINT('Ctrl Pts',(-41.7732836191701,-24.1095407859578,
20.));
#76629=CARTESIAN_POINT('Ctrl Pts',(-41.78736115063,-24.0790750774236,0.));
#76630=CARTESIAN_POINT('Ctrl Pts',(-41.78736115063,-24.0790750774236,20.));
#76631=CARTESIAN_POINT('Ctrl Pts',(-41.8014170973399,-24.0486006340924,
0.));
#76632=CARTESIAN_POINT('Ctrl Pts',(-41.8014170973399,-24.0486006340924,
20.));
#76633=CARTESIAN_POINT('Ctrl Pts',(-41.8154514533324,-24.0181174709622,
0.));
#76634=CARTESIAN_POINT('Ctrl Pts',(-41.8154514533324,-24.0181174709622,
20.));
#76635=CARTESIAN_POINT('Ctrl Pts',(-41.8294642126506,-23.9876256030355,
0.));
#76636=CARTESIAN_POINT('Ctrl Pts',(-41.8294642126506,-23.9876256030355,
20.));
#76637=CARTESIAN_POINT('Ctrl Pts',(-41.8434553693478,-23.9571250453194,
0.));
#76638=CARTESIAN_POINT('Ctrl Pts',(-41.8434553693478,-23.9571250453194,
20.));
#76639=CARTESIAN_POINT('Ctrl Pts',(-41.8574249174873,-23.9266158128252,
0.));
#76640=CARTESIAN_POINT('Ctrl Pts',(-41.8574249174873,-23.9266158128252,
20.));
#76641=CARTESIAN_POINT('Ctrl Pts',(-41.8713728511429,-23.8960979205694,
0.));
#76642=CARTESIAN_POINT('Ctrl Pts',(-41.8713728511429,-23.8960979205694,
20.));
#76643=CARTESIAN_POINT('Ctrl Pts',(-41.8852991643986,-23.8655713835725,
0.));
#76644=CARTESIAN_POINT('Ctrl Pts',(-41.8852991643986,-23.8655713835725,
20.));
#76645=CARTESIAN_POINT('Ctrl Pts',(-41.8992038513488,-23.8350362168598,
0.));
#76646=CARTESIAN_POINT('Ctrl Pts',(-41.8992038513488,-23.8350362168598,
20.));
#76647=CARTESIAN_POINT('Ctrl Pts',(-41.9130869060982,-23.8044924354607,
0.));
#76648=CARTESIAN_POINT('Ctrl Pts',(-41.9130869060982,-23.8044924354607,
20.));
#76649=CARTESIAN_POINT('Ctrl Pts',(-41.9269483227618,-23.7739400544092,
0.));
#76650=CARTESIAN_POINT('Ctrl Pts',(-41.9269483227618,-23.7739400544092,
20.));
#76651=CARTESIAN_POINT('Ctrl Pts',(-41.9407880954647,-23.7433790887435,
0.));
#76652=CARTESIAN_POINT('Ctrl Pts',(-41.9407880954647,-23.7433790887435,
20.));
#76653=CARTESIAN_POINT('Ctrl Pts',(-41.9546062183422,-23.7128095535066,
0.));
#76654=CARTESIAN_POINT('Ctrl Pts',(-41.9546062183422,-23.7128095535066,
20.));
#76655=CARTESIAN_POINT('Ctrl Pts',(-41.9684026855399,-23.6822314637457,
0.));
#76656=CARTESIAN_POINT('Ctrl Pts',(-41.9684026855399,-23.6822314637457,
20.));
#76657=CARTESIAN_POINT('Ctrl Pts',(-41.9821774912142,-23.651644834513,0.));
#76658=CARTESIAN_POINT('Ctrl Pts',(-41.9821774912142,-23.651644834513,20.));
#76659=CARTESIAN_POINT('Ctrl Pts',(-41.9959306295311,-23.6210496808648,
0.));
#76660=CARTESIAN_POINT('Ctrl Pts',(-41.9959306295311,-23.6210496808648,
20.));
#76661=CARTESIAN_POINT('Ctrl Pts',(-42.0096620946675,-23.5904460178619,
0.));
#76662=CARTESIAN_POINT('Ctrl Pts',(-42.0096620946675,-23.5904460178619,
20.));
#76663=CARTESIAN_POINT('Ctrl Pts',(-42.02337188081,-23.5598338605694,0.));
#76664=CARTESIAN_POINT('Ctrl Pts',(-42.02337188081,-23.5598338605694,20.));
#76665=CARTESIAN_POINT('Ctrl Pts',(-42.0370599821558,-23.5292132240566,
0.));
#76666=CARTESIAN_POINT('Ctrl Pts',(-42.0370599821558,-23.5292132240566,
20.));
#76667=CARTESIAN_POINT('Ctrl Pts',(-42.0507263929126,-23.4985841233977,
0.));
#76668=CARTESIAN_POINT('Ctrl Pts',(-42.0507263929126,-23.4985841233977,
20.));
#76669=CARTESIAN_POINT('Ctrl Pts',(-42.0643711072981,-23.4679465736707,
0.));
#76670=CARTESIAN_POINT('Ctrl Pts',(-42.0643711072981,-23.4679465736707,
20.));
#76671=CARTESIAN_POINT('Ctrl Pts',(-42.0779941195407,-23.4373005899585,
0.));
#76672=CARTESIAN_POINT('Ctrl Pts',(-42.0779941195407,-23.4373005899585,
20.));
#76673=CARTESIAN_POINT('Ctrl Pts',(-42.0915954238788,-23.4066461873484,
0.));
#76674=CARTESIAN_POINT('Ctrl Pts',(-42.0915954238788,-23.4066461873484,
20.));
#76675=CARTESIAN_POINT('Ctrl Pts',(-42.1051750145614,-23.3759833809318,
0.));
#76676=CARTESIAN_POINT('Ctrl Pts',(-42.1051750145614,-23.3759833809318,
20.));
#76677=CARTESIAN_POINT('Ctrl Pts',(-42.1187328858474,-23.3453121858047,
0.));
#76678=CARTESIAN_POINT('Ctrl Pts',(-42.1187328858474,-23.3453121858047,
20.));
#76679=CARTESIAN_POINT('Ctrl Pts',(-42.1322690320059,-23.3146326170671,
0.));
#76680=CARTESIAN_POINT('Ctrl Pts',(-42.1322690320059,-23.3146326170671,
20.));
#76681=CARTESIAN_POINT('Ctrl Pts',(-42.145783447317,-23.2839446898238,0.));
#76682=CARTESIAN_POINT('Ctrl Pts',(-42.145783447317,-23.2839446898238,20.));
#76683=CARTESIAN_POINT('Ctrl Pts',(-42.1592761260708,-23.2532484191837,
0.));
#76684=CARTESIAN_POINT('Ctrl Pts',(-42.1592761260708,-23.2532484191837,
20.));
#76685=CARTESIAN_POINT('Ctrl Pts',(-42.1727470625681,-23.2225438202604,
0.));
#76686=CARTESIAN_POINT('Ctrl Pts',(-42.1727470625681,-23.2225438202604,
20.));
#76687=CARTESIAN_POINT('Ctrl Pts',(-42.1861962511195,-23.1918309081713,
0.));
#76688=CARTESIAN_POINT('Ctrl Pts',(-42.1861962511195,-23.1918309081713,
20.));
#76689=CARTESIAN_POINT('Ctrl Pts',(-42.1996236860461,-23.1611096980384,
0.));
#76690=CARTESIAN_POINT('Ctrl Pts',(-42.1996236860461,-23.1611096980384,
20.));
#76691=CARTESIAN_POINT('Ctrl Pts',(-42.2130293616794,-23.1303802049881,
0.));
#76692=CARTESIAN_POINT('Ctrl Pts',(-42.2130293616794,-23.1303802049881,
20.));
#76693=CARTESIAN_POINT('Ctrl Pts',(-42.2264132723612,-23.0996424441509,
0.));
#76694=CARTESIAN_POINT('Ctrl Pts',(-42.2264132723612,-23.0996424441509,
20.));
#76695=CARTESIAN_POINT('Ctrl Pts',(-42.2397754124437,-23.0688964306618,
0.));
#76696=CARTESIAN_POINT('Ctrl Pts',(-42.2397754124437,-23.0688964306618,
20.));
#76697=CARTESIAN_POINT('Ctrl Pts',(-42.2531157762897,-23.0381421796601,
0.));
#76698=CARTESIAN_POINT('Ctrl Pts',(-42.2531157762897,-23.0381421796601,
20.));
#76699=CARTESIAN_POINT('Ctrl Pts',(-42.2664343582719,-23.0073797062893,
0.));
#76700=CARTESIAN_POINT('Ctrl Pts',(-42.2664343582719,-23.0073797062893,
20.));
#76701=CARTESIAN_POINT('Ctrl Pts',(-42.2797311527738,-22.9766090256973,
0.));
#76702=CARTESIAN_POINT('Ctrl Pts',(-42.2797311527738,-22.9766090256973,
20.));
#76703=CARTESIAN_POINT('Ctrl Pts',(-42.2930061541893,-22.9458301530364,
0.));
#76704=CARTESIAN_POINT('Ctrl Pts',(-42.2930061541893,-22.9458301530364,
20.));
#76705=CARTESIAN_POINT('Ctrl Pts',(-42.3062593569226,-22.9150431034629,
0.));
#76706=CARTESIAN_POINT('Ctrl Pts',(-42.3062593569226,-22.9150431034629,
20.));
#76707=CARTESIAN_POINT('Ctrl Pts',(-42.3194907553882,-22.8842478921374,
0.));
#76708=CARTESIAN_POINT('Ctrl Pts',(-42.3194907553882,-22.8842478921374,
20.));
#76709=CARTESIAN_POINT('Ctrl Pts',(-42.3327003440109,-22.8534445342249,
0.));
#76710=CARTESIAN_POINT('Ctrl Pts',(-42.3327003440109,-22.8534445342249,
20.));
#76711=CARTESIAN_POINT('Ctrl Pts',(-42.3458881172255,-22.8226330448945,
0.));
#76712=CARTESIAN_POINT('Ctrl Pts',(-42.3458881172255,-22.8226330448945,
20.));
#76713=CARTESIAN_POINT('Ctrl Pts',(-42.3590540694774,-22.7918134393197,
0.));
#76714=CARTESIAN_POINT('Ctrl Pts',(-42.3590540694774,-22.7918134393197,
20.));
#76715=CARTESIAN_POINT('Ctrl Pts',(-42.3721981952224,-22.7609857326781,
0.));
#76716=CARTESIAN_POINT('Ctrl Pts',(-42.3721981952224,-22.7609857326781,
20.));
#76717=CARTESIAN_POINT('Ctrl Pts',(-42.3853204889273,-22.7301499401517,
0.));
#76718=CARTESIAN_POINT('Ctrl Pts',(-42.3853204889273,-22.7301499401517,
20.));
#76719=CARTESIAN_POINT('Ctrl Pts',(-42.398420945069,-22.6993060769268,0.));
#76720=CARTESIAN_POINT('Ctrl Pts',(-42.398420945069,-22.6993060769268,20.));
#76721=CARTESIAN_POINT('Ctrl Pts',(-42.411499558135,-22.6684541581936,0.));
#76722=CARTESIAN_POINT('Ctrl Pts',(-42.411499558135,-22.6684541581936,20.));
#76723=CARTESIAN_POINT('Ctrl Pts',(-42.4245563226236,-22.6375941991468,
0.));
#76724=CARTESIAN_POINT('Ctrl Pts',(-42.4245563226236,-22.6375941991468,
20.));
#76725=CARTESIAN_POINT('Ctrl Pts',(-42.4375912330427,-22.6067262149851,
0.));
#76726=CARTESIAN_POINT('Ctrl Pts',(-42.4375912330427,-22.6067262149851,
20.));
#76727=CARTESIAN_POINT('Ctrl Pts',(-42.4506042839107,-22.5758502209116,
0.));
#76728=CARTESIAN_POINT('Ctrl Pts',(-42.4506042839107,-22.5758502209116,
20.));
#76729=CARTESIAN_POINT('Ctrl Pts',(-42.4635954697559,-22.5449662321334,
0.));
#76730=CARTESIAN_POINT('Ctrl Pts',(-42.4635954697559,-22.5449662321334,
20.));
#76731=CARTESIAN_POINT('Ctrl Pts',(-42.4765647851171,-22.5140742638619,
0.));
#76732=CARTESIAN_POINT('Ctrl Pts',(-42.4765647851171,-22.5140742638619,
20.));
#76733=CARTESIAN_POINT('Ctrl Pts',(-42.4895122245441,-22.4831743313126,
0.));
#76734=CARTESIAN_POINT('Ctrl Pts',(-42.4895122245441,-22.4831743313126,
20.));
#76735=CARTESIAN_POINT('Ctrl Pts',(-42.502437782597,-22.4522664497054,0.));
#76736=CARTESIAN_POINT('Ctrl Pts',(-42.502437782597,-22.4522664497054,20.));
#76737=CARTESIAN_POINT('Ctrl Pts',(-42.5153414538467,-22.4213506342639,
0.));
#76738=CARTESIAN_POINT('Ctrl Pts',(-42.5153414538467,-22.4213506342639,
20.));
#76739=CARTESIAN_POINT('Ctrl Pts',(-42.5282232328748,-22.3904269002165,
0.));
#76740=CARTESIAN_POINT('Ctrl Pts',(-42.5282232328748,-22.3904269002165,
20.));
#76741=CARTESIAN_POINT('Ctrl Pts',(-42.5410831142727,-22.3594952627952,
0.));
#76742=CARTESIAN_POINT('Ctrl Pts',(-42.5410831142727,-22.3594952627952,
20.));
#76743=CARTESIAN_POINT('Ctrl Pts',(-42.5539210926424,-22.3285557372364,
0.));
#76744=CARTESIAN_POINT('Ctrl Pts',(-42.5539210926424,-22.3285557372364,
20.));
#76745=CARTESIAN_POINT('Ctrl Pts',(-42.5667371625962,-22.2976083387805,
0.));
#76746=CARTESIAN_POINT('Ctrl Pts',(-42.5667371625962,-22.2976083387805,
20.));
#76747=CARTESIAN_POINT('Ctrl Pts',(-42.5795313187569,-22.2666530826722,
0.));
#76748=CARTESIAN_POINT('Ctrl Pts',(-42.5795313187569,-22.2666530826722,
20.));
#76749=CARTESIAN_POINT('Ctrl Pts',(-42.5923035557573,-22.2356899841602,
0.));
#76750=CARTESIAN_POINT('Ctrl Pts',(-42.5923035557573,-22.2356899841602,
20.));
#76751=CARTESIAN_POINT('Ctrl Pts',(-42.6050538682411,-22.2047190584974,
0.));
#76752=CARTESIAN_POINT('Ctrl Pts',(-42.6050538682411,-22.2047190584974,
20.));
#76753=CARTESIAN_POINT('Ctrl Pts',(-42.6177822508627,-22.1737403209406,
0.));
#76754=CARTESIAN_POINT('Ctrl Pts',(-42.6177822508627,-22.1737403209406,
20.));
#76755=CARTESIAN_POINT('Ctrl Pts',(-42.6304886982869,-22.1427537867512,
0.));
#76756=CARTESIAN_POINT('Ctrl Pts',(-42.6304886982869,-22.1427537867512,
20.));
#76757=CARTESIAN_POINT('Ctrl Pts',(-42.6431732051887,-22.1117594711942,
0.));
#76758=CARTESIAN_POINT('Ctrl Pts',(-42.6431732051887,-22.1117594711942,
20.));
#76759=CARTESIAN_POINT('Ctrl Pts',(-42.6558357662536,-22.0807573895388,
0.));
#76760=CARTESIAN_POINT('Ctrl Pts',(-42.6558357662536,-22.0807573895388,
20.));
#76761=CARTESIAN_POINT('Ctrl Pts',(-42.6684763761777,-22.0497475570584,
0.));
#76762=CARTESIAN_POINT('Ctrl Pts',(-42.6684763761777,-22.0497475570584,
20.));
#76763=CARTESIAN_POINT('Ctrl Pts',(-42.6810950296678,-22.0187299890302,
0.));
#76764=CARTESIAN_POINT('Ctrl Pts',(-42.6810950296678,-22.0187299890302,
20.));
#76765=CARTESIAN_POINT('Ctrl Pts',(-42.6936917214411,-21.9877047007357,
0.));
#76766=CARTESIAN_POINT('Ctrl Pts',(-42.6936917214411,-21.9877047007357,
20.));
#76767=CARTESIAN_POINT('Ctrl Pts',(-42.7062664462249,-21.9566717074606,
0.));
#76768=CARTESIAN_POINT('Ctrl Pts',(-42.7062664462249,-21.9566717074606,
20.));
#76769=CARTESIAN_POINT('Ctrl Pts',(-42.7188191987573,-21.9256310244944,
0.));
#76770=CARTESIAN_POINT('Ctrl Pts',(-42.7188191987573,-21.9256310244944,
20.));
#76771=CARTESIAN_POINT('Ctrl Pts',(-42.7313499737866,-21.8945826671308,
0.));
#76772=CARTESIAN_POINT('Ctrl Pts',(-42.7313499737866,-21.8945826671308,
20.));
#76773=CARTESIAN_POINT('Ctrl Pts',(-42.7438587660714,-21.8635266506674,
0.));
#76774=CARTESIAN_POINT('Ctrl Pts',(-42.7438587660714,-21.8635266506674,
20.));
#76775=CARTESIAN_POINT('Ctrl Pts',(-42.7563455703812,-21.832462990406,0.));
#76776=CARTESIAN_POINT('Ctrl Pts',(-42.7563455703812,-21.832462990406,20.));
#76777=CARTESIAN_POINT('Ctrl Pts',(-42.7688103814962,-21.8013917016521,
0.));
#76778=CARTESIAN_POINT('Ctrl Pts',(-42.7688103814962,-21.8013917016521,
20.));
#76779=CARTESIAN_POINT('Ctrl Pts',(-42.7812531942069,-21.7703127997157,
0.));
#76780=CARTESIAN_POINT('Ctrl Pts',(-42.7812531942069,-21.7703127997157,
20.));
#76781=CARTESIAN_POINT('Ctrl Pts',(-42.7936740033148,-21.7392262999104,
0.));
#76782=CARTESIAN_POINT('Ctrl Pts',(-42.7936740033148,-21.7392262999104,
20.));
#76783=CARTESIAN_POINT('Ctrl Pts',(-42.8060728036314,-21.7081322175539,
0.));
#76784=CARTESIAN_POINT('Ctrl Pts',(-42.8060728036314,-21.7081322175539,
20.));
#76785=CARTESIAN_POINT('Ctrl Pts',(-42.8184495899785,-21.677030567968,0.));
#76786=CARTESIAN_POINT('Ctrl Pts',(-42.8184495899785,-21.677030567968,20.));
#76787=CARTESIAN_POINT('Ctrl Pts',(-42.8308043571887,-21.6459213664784,
0.));
#76788=CARTESIAN_POINT('Ctrl Pts',(-42.8308043571887,-21.6459213664784,
20.));
#76789=CARTESIAN_POINT('Ctrl Pts',(-42.8431371001047,-21.6148046284149,
0.));
#76790=CARTESIAN_POINT('Ctrl Pts',(-42.8431371001047,-21.6148046284149,
20.));
#76791=CARTESIAN_POINT('Ctrl Pts',(-42.8554478135801,-21.5836803691112,
0.));
#76792=CARTESIAN_POINT('Ctrl Pts',(-42.8554478135801,-21.5836803691112,
20.));
#76793=CARTESIAN_POINT('Ctrl Pts',(-42.8677364924794,-21.5525486039049,
0.));
#76794=CARTESIAN_POINT('Ctrl Pts',(-42.8677364924794,-21.5525486039049,
20.));
#76795=CARTESIAN_POINT('Ctrl Pts',(-42.8800031316769,-21.5214093481377,
0.));
#76796=CARTESIAN_POINT('Ctrl Pts',(-42.8800031316769,-21.5214093481377,
20.));
#76797=CARTESIAN_POINT('Ctrl Pts',(-42.8922477260581,-21.490262617155,0.));
#76798=CARTESIAN_POINT('Ctrl Pts',(-42.8922477260581,-21.490262617155,20.));
#76799=CARTESIAN_POINT('Ctrl Pts',(-42.9044702705183,-21.4591084263065,
0.));
#76800=CARTESIAN_POINT('Ctrl Pts',(-42.9044702705183,-21.4591084263065,
20.));
#76801=CARTESIAN_POINT('Ctrl Pts',(-42.916670759964,-21.4279467909454,0.));
#76802=CARTESIAN_POINT('Ctrl Pts',(-42.916670759964,-21.4279467909454,20.));
#76803=CARTESIAN_POINT('Ctrl Pts',(-42.9288491893122,-21.3967777264294,
0.));
#76804=CARTESIAN_POINT('Ctrl Pts',(-42.9288491893122,-21.3967777264294,
20.));
#76805=CARTESIAN_POINT('Ctrl Pts',(-42.9410055534907,-21.3656012481198,
0.));
#76806=CARTESIAN_POINT('Ctrl Pts',(-42.9410055534907,-21.3656012481198,
20.));
#76807=CARTESIAN_POINT('Ctrl Pts',(-42.9531398474371,-21.3344173713818,
0.));
#76808=CARTESIAN_POINT('Ctrl Pts',(-42.9531398474371,-21.3344173713818,
20.));
#76809=CARTESIAN_POINT('Ctrl Pts',(-42.9652520660998,-21.3032261115844,
0.));
#76810=CARTESIAN_POINT('Ctrl Pts',(-42.9652520660998,-21.3032261115844,
20.));
#76811=CARTESIAN_POINT('Ctrl Pts',(-42.9773422044374,-21.2720274841006,
0.));
#76812=CARTESIAN_POINT('Ctrl Pts',(-42.9773422044374,-21.2720274841006,
20.));
#76813=CARTESIAN_POINT('Ctrl Pts',(-42.9894102574195,-21.2408215043074,
0.));
#76814=CARTESIAN_POINT('Ctrl Pts',(-42.9894102574195,-21.2408215043074,
20.));
#76815=CARTESIAN_POINT('Ctrl Pts',(-43.0014562200264,-21.2096081875857,
0.));
#76816=CARTESIAN_POINT('Ctrl Pts',(-43.0014562200264,-21.2096081875857,
20.));
#76817=CARTESIAN_POINT('Ctrl Pts',(-43.0134800872489,-21.1783875493204,
0.));
#76818=CARTESIAN_POINT('Ctrl Pts',(-43.0134800872489,-21.1783875493204,
20.));
#76819=CARTESIAN_POINT('Ctrl Pts',(-43.0254818540885,-21.1471596049,0.));
#76820=CARTESIAN_POINT('Ctrl Pts',(-43.0254818540885,-21.1471596049,20.));
#76821=CARTESIAN_POINT('Ctrl Pts',(-43.037461515557,-21.1159243697169,0.));
#76822=CARTESIAN_POINT('Ctrl Pts',(-43.037461515557,-21.1159243697169,20.));
#76823=CARTESIAN_POINT('Ctrl Pts',(-43.0494190666771,-21.0846818591673,
0.));
#76824=CARTESIAN_POINT('Ctrl Pts',(-43.0494190666771,-21.0846818591673,
20.));
#76825=CARTESIAN_POINT('Ctrl Pts',(-43.0613545024815,-21.0534320886512,
0.));
#76826=CARTESIAN_POINT('Ctrl Pts',(-43.0613545024815,-21.0534320886512,
20.));
#76827=CARTESIAN_POINT('Ctrl Pts',(-43.0732678180139,-21.0221750735727,
0.));
#76828=CARTESIAN_POINT('Ctrl Pts',(-43.0732678180139,-21.0221750735727,
20.));
#76829=CARTESIAN_POINT('Ctrl Pts',(-43.0851590083283,-20.9909108293397,
0.));
#76830=CARTESIAN_POINT('Ctrl Pts',(-43.0851590083283,-20.9909108293397,
20.));
#76831=CARTESIAN_POINT('Ctrl Pts',(-43.0970280684896,-20.959639371364,0.));
#76832=CARTESIAN_POINT('Ctrl Pts',(-43.0970280684896,-20.959639371364,20.));
#76833=CARTESIAN_POINT('Ctrl Pts',(-43.1088749935734,-20.9283607150615,
0.));
#76834=CARTESIAN_POINT('Ctrl Pts',(-43.1088749935734,-20.9283607150615,
20.));
#76835=CARTESIAN_POINT('Ctrl Pts',(-43.1206997786657,-20.8970748758512,
0.));
#76836=CARTESIAN_POINT('Ctrl Pts',(-43.1206997786657,-20.8970748758512,
20.));
#76837=CARTESIAN_POINT('Ctrl Pts',(-43.132502418863,-20.8657818691565,0.));
#76838=CARTESIAN_POINT('Ctrl Pts',(-43.132502418863,-20.8657818691565,20.));
#76839=CARTESIAN_POINT('Ctrl Pts',(-43.1442829092724,-20.8344817104039,
0.));
#76840=CARTESIAN_POINT('Ctrl Pts',(-43.1442829092724,-20.8344817104039,
20.));
#76841=CARTESIAN_POINT('Ctrl Pts',(-43.1560412450117,-20.8031744150242,
0.));
#76842=CARTESIAN_POINT('Ctrl Pts',(-43.1560412450117,-20.8031744150242,
20.));
#76843=CARTESIAN_POINT('Ctrl Pts',(-43.1677774212093,-20.7718599984518,
0.));
#76844=CARTESIAN_POINT('Ctrl Pts',(-43.1677774212093,-20.7718599984518,
20.));
#76845=CARTESIAN_POINT('Ctrl Pts',(-43.1794914330045,-20.7405384761252,
0.));
#76846=CARTESIAN_POINT('Ctrl Pts',(-43.1794914330045,-20.7405384761252,
20.));
#76847=CARTESIAN_POINT('Ctrl Pts',(-43.1911832755467,-20.7092098634864,
0.));
#76848=CARTESIAN_POINT('Ctrl Pts',(-43.1911832755467,-20.7092098634864,
20.));
#76849=CARTESIAN_POINT('Ctrl Pts',(-43.202852943996,-20.6778741759814,0.));
#76850=CARTESIAN_POINT('Ctrl Pts',(-43.202852943996,-20.6778741759814,20.));
#76851=CARTESIAN_POINT('Ctrl Pts',(-43.2145004335236,-20.6465314290598,
0.));
#76852=CARTESIAN_POINT('Ctrl Pts',(-43.2145004335236,-20.6465314290598,
20.));
#76853=CARTESIAN_POINT('Ctrl Pts',(-43.2261257393109,-20.615181638175,0.));
#76854=CARTESIAN_POINT('Ctrl Pts',(-43.2261257393109,-20.615181638175,20.));
#76855=CARTESIAN_POINT('Ctrl Pts',(-43.2377288565503,-20.5838248187841,
0.));
#76856=CARTESIAN_POINT('Ctrl Pts',(-43.2377288565503,-20.5838248187841,
20.));
#76857=CARTESIAN_POINT('Ctrl Pts',(-43.2493097804445,-20.5524609863481,
0.));
#76858=CARTESIAN_POINT('Ctrl Pts',(-43.2493097804445,-20.5524609863481,
20.));
#76859=CARTESIAN_POINT('Ctrl Pts',(-43.2608685062069,-20.5210901563314,
0.));
#76860=CARTESIAN_POINT('Ctrl Pts',(-43.2608685062069,-20.5210901563314,
20.));
#76861=CARTESIAN_POINT('Ctrl Pts',(-43.2724050290617,-20.4897123442023,
0.));
#76862=CARTESIAN_POINT('Ctrl Pts',(-43.2724050290617,-20.4897123442023,
20.));
#76863=CARTESIAN_POINT('Ctrl Pts',(-43.283919344243,-20.4583275654327,0.));
#76864=CARTESIAN_POINT('Ctrl Pts',(-43.283919344243,-20.4583275654327,20.));
#76865=CARTESIAN_POINT('Ctrl Pts',(-43.2954114469964,-20.4269358354984,
0.));
#76866=CARTESIAN_POINT('Ctrl Pts',(-43.2954114469964,-20.4269358354984,
20.));
#76867=CARTESIAN_POINT('Ctrl Pts',(-43.3068813325774,-20.3955371698787,
0.));
#76868=CARTESIAN_POINT('Ctrl Pts',(-43.3068813325774,-20.3955371698787,
20.));
#76869=CARTESIAN_POINT('Ctrl Pts',(-43.3183289962528,-20.3641315840566,
0.));
#76870=CARTESIAN_POINT('Ctrl Pts',(-43.3183289962528,-20.3641315840566,
20.));
#76871=CARTESIAN_POINT('Ctrl Pts',(-43.3297544333003,-20.3327190935193,
0.));
#76872=CARTESIAN_POINT('Ctrl Pts',(-43.3297544333003,-20.3327190935193,
20.));
#76873=CARTESIAN_POINT('Ctrl Pts',(-43.3411576390085,-20.3012997137575,
0.));
#76874=CARTESIAN_POINT('Ctrl Pts',(-43.3411576390085,-20.3012997137575,
20.));
#76875=CARTESIAN_POINT('Ctrl Pts',(-43.3525386086763,-20.2698734602656,
0.));
#76876=CARTESIAN_POINT('Ctrl Pts',(-43.3525386086763,-20.2698734602656,
20.));
#76877=CARTESIAN_POINT('Ctrl Pts',(-43.3638973376125,-20.2384403485411,
0.));
#76878=CARTESIAN_POINT('Ctrl Pts',(-43.3638973376125,-20.2384403485411,
20.));
#76879=CARTESIAN_POINT('Ctrl Pts',(-43.3752338211368,-20.2070003940853,
0.));
#76880=CARTESIAN_POINT('Ctrl Pts',(-43.3752338211368,-20.2070003940853,
20.));
#76881=CARTESIAN_POINT('Ctrl Pts',(-43.3865480545792,-20.1755536124033,
0.));
#76882=CARTESIAN_POINT('Ctrl Pts',(-43.3865480545792,-20.1755536124033,
20.));
#76883=CARTESIAN_POINT('Ctrl Pts',(-43.3978400332808,-20.1441000190037,
0.));
#76884=CARTESIAN_POINT('Ctrl Pts',(-43.3978400332808,-20.1441000190037,
20.));
#76885=CARTESIAN_POINT('Ctrl Pts',(-43.409109752594,-20.1126396293992,0.));
#76886=CARTESIAN_POINT('Ctrl Pts',(-43.409109752594,-20.1126396293992,20.));
#76887=CARTESIAN_POINT('Ctrl Pts',(-43.4203572078819,-20.0811724591058,
0.));
#76888=CARTESIAN_POINT('Ctrl Pts',(-43.4203572078819,-20.0811724591058,
20.));
#76889=CARTESIAN_POINT('Ctrl Pts',(-43.4315823945181,-20.0496985236436,
0.));
#76890=CARTESIAN_POINT('Ctrl Pts',(-43.4315823945181,-20.0496985236436,
20.));
#76891=CARTESIAN_POINT('Ctrl Pts',(-43.4427853078868,-20.0182178385356,
0.));
#76892=CARTESIAN_POINT('Ctrl Pts',(-43.4427853078868,-20.0182178385356,
20.));
#76893=CARTESIAN_POINT('Ctrl Pts',(-43.4539659433821,-19.9867304193089,
0.));
#76894=CARTESIAN_POINT('Ctrl Pts',(-43.4539659433821,-19.9867304193089,
20.));
#76895=CARTESIAN_POINT('Ctrl Pts',(-43.4651242964088,-19.9552362814936,
0.));
#76896=CARTESIAN_POINT('Ctrl Pts',(-43.4651242964088,-19.9552362814936,
20.));
#76897=CARTESIAN_POINT('Ctrl Pts',(-43.4762603623832,-19.923735440624,0.));
#76898=CARTESIAN_POINT('Ctrl Pts',(-43.4762603623832,-19.923735440624,20.));
#76899=CARTESIAN_POINT('Ctrl Pts',(-43.4873741367321,-19.8922279122378,
0.));
#76900=CARTESIAN_POINT('Ctrl Pts',(-43.4873741367321,-19.8922279122378,
20.));
#76901=CARTESIAN_POINT('Ctrl Pts',(-43.4984656148936,-19.8607137118763,
0.));
#76902=CARTESIAN_POINT('Ctrl Pts',(-43.4984656148936,-19.8607137118763,
20.));
#76903=CARTESIAN_POINT('Ctrl Pts',(-43.5095347923164,-19.8291928550844,
0.));
#76904=CARTESIAN_POINT('Ctrl Pts',(-43.5095347923164,-19.8291928550844,
20.));
#76905=CARTESIAN_POINT('Ctrl Pts',(-43.5205816644596,-19.7976653574108,
0.));
#76906=CARTESIAN_POINT('Ctrl Pts',(-43.5205816644596,-19.7976653574108,
20.));
#76907=CARTESIAN_POINT('Ctrl Pts',(-43.5316062267925,-19.7661312344072,
0.));
#76908=CARTESIAN_POINT('Ctrl Pts',(-43.5316062267925,-19.7661312344072,
20.));
#76909=CARTESIAN_POINT('Ctrl Pts',(-43.542608474795,-19.734590501629,0.));
#76910=CARTESIAN_POINT('Ctrl Pts',(-43.542608474795,-19.734590501629,20.));
#76911=CARTESIAN_POINT('Ctrl Pts',(-43.5535884039576,-19.7030431746352,
0.));
#76912=CARTESIAN_POINT('Ctrl Pts',(-43.5535884039576,-19.7030431746352,
20.));
#76913=CARTESIAN_POINT('Ctrl Pts',(-43.5645460097823,-19.6714892689885,
0.));
#76914=CARTESIAN_POINT('Ctrl Pts',(-43.5645460097823,-19.6714892689885,
20.));
#76915=CARTESIAN_POINT('Ctrl Pts',(-43.5754812877819,-19.639928800255,0.));
#76916=CARTESIAN_POINT('Ctrl Pts',(-43.5754812877819,-19.639928800255,20.));
#76917=CARTESIAN_POINT('Ctrl Pts',(-43.5863942334797,-19.6083617840046,
0.));
#76918=CARTESIAN_POINT('Ctrl Pts',(-43.5863942334797,-19.6083617840046,
20.));
#76919=CARTESIAN_POINT('Ctrl Pts',(-43.5972848424097,-19.5767882358104,
0.));
#76920=CARTESIAN_POINT('Ctrl Pts',(-43.5972848424097,-19.5767882358104,
20.));
#76921=CARTESIAN_POINT('Ctrl Pts',(-43.6081531101168,-19.545208171249,0.));
#76922=CARTESIAN_POINT('Ctrl Pts',(-43.6081531101168,-19.545208171249,20.));
#76923=CARTESIAN_POINT('Ctrl Pts',(-43.6189990321561,-19.5136216059004,
0.));
#76924=CARTESIAN_POINT('Ctrl Pts',(-43.6189990321561,-19.5136216059004,
20.));
#76925=CARTESIAN_POINT('Ctrl Pts',(-43.629822604094,-19.4820285553483,0.));
#76926=CARTESIAN_POINT('Ctrl Pts',(-43.629822604094,-19.4820285553483,20.));
#76927=CARTESIAN_POINT('Ctrl Pts',(-43.6406238215078,-19.4504290351799,
0.));
#76928=CARTESIAN_POINT('Ctrl Pts',(-43.6406238215078,-19.4504290351799,
20.));
#76929=CARTESIAN_POINT('Ctrl Pts',(-43.6514026799849,-19.4188230609858,
0.));
#76930=CARTESIAN_POINT('Ctrl Pts',(-43.6514026799849,-19.4188230609858,
20.));
#76931=CARTESIAN_POINT('Ctrl Pts',(-43.6621591751234,-19.3872106483603,
0.));
#76932=CARTESIAN_POINT('Ctrl Pts',(-43.6621591751234,-19.3872106483603,
20.));
#76933=CARTESIAN_POINT('Ctrl Pts',(-43.6728933025325,-19.3555918129009,
0.));
#76934=CARTESIAN_POINT('Ctrl Pts',(-43.6728933025325,-19.3555918129009,
20.));
#76935=CARTESIAN_POINT('Ctrl Pts',(-43.6836050578319,-19.3239665702086,
0.));
#76936=CARTESIAN_POINT('Ctrl Pts',(-43.6836050578319,-19.3239665702086,
20.));
#76937=CARTESIAN_POINT('Ctrl Pts',(-43.6942944366523,-19.2923349358879,
0.));
#76938=CARTESIAN_POINT('Ctrl Pts',(-43.6942944366523,-19.2923349358879,
20.));
#76939=CARTESIAN_POINT('Ctrl Pts',(-43.7049614346349,-19.2606969255464,
0.));
#76940=CARTESIAN_POINT('Ctrl Pts',(-43.7049614346349,-19.2606969255464,
20.));
#76941=CARTESIAN_POINT('Ctrl Pts',(-43.7156060474324,-19.2290525547956,
0.));
#76942=CARTESIAN_POINT('Ctrl Pts',(-43.7156060474324,-19.2290525547956,
20.));
#76943=CARTESIAN_POINT('Ctrl Pts',(-43.7262282707082,-19.1974018392505,
0.));
#76944=CARTESIAN_POINT('Ctrl Pts',(-43.7262282707082,-19.1974018392505,
20.));
#76945=CARTESIAN_POINT('Ctrl Pts',(-43.7368281001363,-19.1657447945291,
0.));
#76946=CARTESIAN_POINT('Ctrl Pts',(-43.7368281001363,-19.1657447945291,
20.));
#76947=CARTESIAN_POINT('Ctrl Pts',(-43.747405531401,-19.1340814362531,0.));
#76948=CARTESIAN_POINT('Ctrl Pts',(-43.747405531401,-19.1340814362531,20.));
#76949=CARTESIAN_POINT('Ctrl Pts',(-43.7579605601976,-19.1024117800474,
0.));
#76950=CARTESIAN_POINT('Ctrl Pts',(-43.7579605601976,-19.1024117800474,
20.));
#76951=CARTESIAN_POINT('Ctrl Pts',(-43.7684931822314,-19.0707358415405,
0.));
#76952=CARTESIAN_POINT('Ctrl Pts',(-43.7684931822314,-19.0707358415405,
20.));
#76953=CARTESIAN_POINT('Ctrl Pts',(-43.779003393219,-19.039053636364,0.));
#76954=CARTESIAN_POINT('Ctrl Pts',(-43.779003393219,-19.039053636364,20.));
#76955=CARTESIAN_POINT('Ctrl Pts',(-43.7894911888877,-19.0073651801531,
0.));
#76956=CARTESIAN_POINT('Ctrl Pts',(-43.7894911888877,-19.0073651801531,
20.));
#76957=CARTESIAN_POINT('Ctrl Pts',(-43.7999565649762,-18.9756704885464,
0.));
#76958=CARTESIAN_POINT('Ctrl Pts',(-43.7999565649762,-18.9756704885464,
20.));
#76959=CARTESIAN_POINT('Ctrl Pts',(-43.8103995172341,-18.9439695771858,
0.));
#76960=CARTESIAN_POINT('Ctrl Pts',(-43.8103995172341,-18.9439695771858,
20.));
#76961=CARTESIAN_POINT('Ctrl Pts',(-43.8208200414219,-18.9122624617166,
0.));
#76962=CARTESIAN_POINT('Ctrl Pts',(-43.8208200414219,-18.9122624617166,
20.));
#76963=CARTESIAN_POINT('Ctrl Pts',(-43.8312181333106,-18.8805491577876,
0.));
#76964=CARTESIAN_POINT('Ctrl Pts',(-43.8312181333106,-18.8805491577876,
20.));
#76965=CARTESIAN_POINT('Ctrl Pts',(-43.8415937886817,-18.8488296810507,
0.));
#76966=CARTESIAN_POINT('Ctrl Pts',(-43.8415937886817,-18.8488296810507,
20.));
#76967=CARTESIAN_POINT('Ctrl Pts',(-43.8519470033272,-18.8171040471611,
0.));
#76968=CARTESIAN_POINT('Ctrl Pts',(-43.8519470033272,-18.8171040471611,
20.));
#76969=CARTESIAN_POINT('Ctrl Pts',(-43.8622777730502,-18.7853722717774,
0.));
#76970=CARTESIAN_POINT('Ctrl Pts',(-43.8622777730502,-18.7853722717774,
20.));
#76971=CARTESIAN_POINT('Ctrl Pts',(-43.8725860936644,-18.7536343705616,
0.));
#76972=CARTESIAN_POINT('Ctrl Pts',(-43.8725860936644,-18.7536343705616,
20.));
#76973=CARTESIAN_POINT('Ctrl Pts',(-43.8828719609947,-18.721890359179,0.));
#76974=CARTESIAN_POINT('Ctrl Pts',(-43.8828719609947,-18.721890359179,20.));
#76975=CARTESIAN_POINT('Ctrl Pts',(-43.8931353708767,-18.6901402532984,
0.));
#76976=CARTESIAN_POINT('Ctrl Pts',(-43.8931353708767,-18.6901402532984,
20.));
#76977=CARTESIAN_POINT('Ctrl Pts',(-43.903376319157,-18.6583840685915,0.));
#76978=CARTESIAN_POINT('Ctrl Pts',(-43.903376319157,-18.6583840685915,20.));
#76979=CARTESIAN_POINT('Ctrl Pts',(-43.913594801693,-18.6266218207337,0.));
#76980=CARTESIAN_POINT('Ctrl Pts',(-43.913594801693,-18.6266218207337,20.));
#76981=CARTESIAN_POINT('Ctrl Pts',(-43.9237908143526,-18.5948535254034,
0.));
#76982=CARTESIAN_POINT('Ctrl Pts',(-43.9237908143526,-18.5948535254034,
20.));
#76983=CARTESIAN_POINT('Ctrl Pts',(-43.9339643530151,-18.5630791982821,
0.));
#76984=CARTESIAN_POINT('Ctrl Pts',(-43.9339643530151,-18.5630791982821,
20.));
#76985=CARTESIAN_POINT('Ctrl Pts',(-43.94411541357,-18.5312988550549,0.));
#76986=CARTESIAN_POINT('Ctrl Pts',(-43.94411541357,-18.5312988550549,20.));
#76987=CARTESIAN_POINT('Ctrl Pts',(-43.9542439919177,-18.4995125114099,
0.));
#76988=CARTESIAN_POINT('Ctrl Pts',(-43.9542439919177,-18.4995125114099,
20.));
#76989=CARTESIAN_POINT('Ctrl Pts',(-43.9643500839697,-18.4677201830388,
0.));
#76990=CARTESIAN_POINT('Ctrl Pts',(-43.9643500839697,-18.4677201830388,
20.));
#76991=CARTESIAN_POINT('Ctrl Pts',(-43.9744336856481,-18.4359218856365,
0.));
#76992=CARTESIAN_POINT('Ctrl Pts',(-43.9744336856481,-18.4359218856365,
20.));
#76993=CARTESIAN_POINT('Ctrl Pts',(-43.9844947928861,-18.4041176349014,
0.));
#76994=CARTESIAN_POINT('Ctrl Pts',(-43.9844947928861,-18.4041176349014,
20.));
#76995=CARTESIAN_POINT('Ctrl Pts',(-43.9945334016277,-18.3723074465347,
0.));
#76996=CARTESIAN_POINT('Ctrl Pts',(-43.9945334016277,-18.3723074465347,
20.));
#76997=CARTESIAN_POINT('Ctrl Pts',(-44.0045495078276,-18.3404913362408,
0.));
#76998=CARTESIAN_POINT('Ctrl Pts',(-44.0045495078276,-18.3404913362408,
20.));
#76999=CARTESIAN_POINT('Ctrl Pts',(-44.0145431074514,-18.3086693197275,
0.));
#77000=CARTESIAN_POINT('Ctrl Pts',(-44.0145431074514,-18.3086693197275,
20.));
#77001=CARTESIAN_POINT('Ctrl Pts',(-44.0245141964756,-18.2768414127056,
0.));
#77002=CARTESIAN_POINT('Ctrl Pts',(-44.0245141964756,-18.2768414127056,
20.));
#77003=CARTESIAN_POINT('Ctrl Pts',(-44.0344627708874,-18.2450076308889,
0.));
#77004=CARTESIAN_POINT('Ctrl Pts',(-44.0344627708874,-18.2450076308889,
20.));
#77005=CARTESIAN_POINT('Ctrl Pts',(-44.044388826685,-18.2131679899948,0.));
#77006=CARTESIAN_POINT('Ctrl Pts',(-44.044388826685,-18.2131679899948,20.));
#77007=CARTESIAN_POINT('Ctrl Pts',(-44.0542923598773,-18.1813225057438,
0.));
#77008=CARTESIAN_POINT('Ctrl Pts',(-44.0542923598773,-18.1813225057438,
20.));
#77009=CARTESIAN_POINT('Ctrl Pts',(-44.0641733664839,-18.1494711938598,
0.));
#77010=CARTESIAN_POINT('Ctrl Pts',(-44.0641733664839,-18.1494711938598,
20.));
#77011=CARTESIAN_POINT('Ctrl Pts',(-44.0740318425361,-18.1176140700699,
0.));
#77012=CARTESIAN_POINT('Ctrl Pts',(-44.0740318425361,-18.1176140700699,
20.));
#77013=CARTESIAN_POINT('Ctrl Pts',(-44.0838677840754,-18.0857511501043,
0.));
#77014=CARTESIAN_POINT('Ctrl Pts',(-44.0838677840754,-18.0857511501043,
20.));
#77015=CARTESIAN_POINT('Ctrl Pts',(-44.0936811871546,-18.0538824496962,
0.));
#77016=CARTESIAN_POINT('Ctrl Pts',(-44.0936811871546,-18.0538824496962,
20.));
#77017=CARTESIAN_POINT('Ctrl Pts',(-44.1034720478372,-18.0220079845822,
0.));
#77018=CARTESIAN_POINT('Ctrl Pts',(-44.1034720478372,-18.0220079845822,
20.));
#77019=CARTESIAN_POINT('Ctrl Pts',(-44.1132403621971,-17.9901277705015,
0.));
#77020=CARTESIAN_POINT('Ctrl Pts',(-44.1132403621971,-17.9901277705015,
20.));
#77021=CARTESIAN_POINT('Ctrl Pts',(-44.1229861263191,-17.9582418231966,
0.));
#77022=CARTESIAN_POINT('Ctrl Pts',(-44.1229861263191,-17.9582418231966,
20.));
#77023=CARTESIAN_POINT('Ctrl Pts',(-44.1327093362991,-17.9263501584131,
0.));
#77024=CARTESIAN_POINT('Ctrl Pts',(-44.1327093362991,-17.9263501584131,
20.));
#77025=CARTESIAN_POINT('Ctrl Pts',(-44.142409988244,-17.8944527919,0.));
#77026=CARTESIAN_POINT('Ctrl Pts',(-44.142409988244,-17.8944527919,20.));
#77027=CARTESIAN_POINT('Ctrl Pts',(-44.1520880782717,-17.8625497394092,
0.));
#77028=CARTESIAN_POINT('Ctrl Pts',(-44.1520880782717,-17.8625497394092,
20.));
#77029=CARTESIAN_POINT('Ctrl Pts',(-44.1617436025112,-17.8306410166963,
0.));
#77030=CARTESIAN_POINT('Ctrl Pts',(-44.1617436025112,-17.8306410166963,
20.));
#77031=CARTESIAN_POINT('Ctrl Pts',(-44.1713765571021,-17.7987266395196,
0.));
#77032=CARTESIAN_POINT('Ctrl Pts',(-44.1713765571021,-17.7987266395196,
20.));
#77033=CARTESIAN_POINT('Ctrl Pts',(-44.1809869381949,-17.7668066236405,
0.));
#77034=CARTESIAN_POINT('Ctrl Pts',(-44.1809869381949,-17.7668066236405,
20.));
#77035=CARTESIAN_POINT('Ctrl Pts',(-44.1905747419505,-17.7348809848234,
0.));
#77036=CARTESIAN_POINT('Ctrl Pts',(-44.1905747419505,-17.7348809848234,
20.));
#77037=CARTESIAN_POINT('Ctrl Pts',(-44.2001399645408,-17.7029497388358,
0.));
#77038=CARTESIAN_POINT('Ctrl Pts',(-44.2001399645408,-17.7029497388358,
20.));
#77039=CARTESIAN_POINT('Ctrl Pts',(-44.2096826021493,-17.6710129014481,
0.));
#77040=CARTESIAN_POINT('Ctrl Pts',(-44.2096826021493,-17.6710129014481,
20.));
#77041=CARTESIAN_POINT('Ctrl Pts',(-44.2192026509705,-17.6390704884341,
0.));
#77042=CARTESIAN_POINT('Ctrl Pts',(-44.2192026509705,-17.6390704884341,
20.));
#77043=CARTESIAN_POINT('Ctrl Pts',(-44.2287001072093,-17.6071225155702,
0.));
#77044=CARTESIAN_POINT('Ctrl Pts',(-44.2287001072093,-17.6071225155702,
20.));
#77045=CARTESIAN_POINT('Ctrl Pts',(-44.2381749670816,-17.5751689986363,
0.));
#77046=CARTESIAN_POINT('Ctrl Pts',(-44.2381749670816,-17.5751689986363,
20.));
#77047=CARTESIAN_POINT('Ctrl Pts',(-44.2476272268138,-17.5432099534151,
0.));
#77048=CARTESIAN_POINT('Ctrl Pts',(-44.2476272268138,-17.5432099534151,
20.));
#77049=CARTESIAN_POINT('Ctrl Pts',(-44.2570568826434,-17.5112453956925,
0.));
#77050=CARTESIAN_POINT('Ctrl Pts',(-44.2570568826434,-17.5112453956925,
20.));
#77051=CARTESIAN_POINT('Ctrl Pts',(-44.2664639308192,-17.4792753412574,
0.));
#77052=CARTESIAN_POINT('Ctrl Pts',(-44.2664639308192,-17.4792753412574,
20.));
#77053=CARTESIAN_POINT('Ctrl Pts',(-44.2758483676008,-17.447299805902,0.));
#77054=CARTESIAN_POINT('Ctrl Pts',(-44.2758483676008,-17.447299805902,20.));
#77055=CARTESIAN_POINT('Ctrl Pts',(-44.2852101892593,-17.4153188054211,
0.));
#77056=CARTESIAN_POINT('Ctrl Pts',(-44.2852101892593,-17.4153188054211,
20.));
#77057=CARTESIAN_POINT('Ctrl Pts',(-44.2945493920761,-17.3833323556128,
0.));
#77058=CARTESIAN_POINT('Ctrl Pts',(-44.2945493920761,-17.3833323556128,
20.));
#77059=CARTESIAN_POINT('Ctrl Pts',(-44.3038659723435,-17.3513404722779,
0.));
#77060=CARTESIAN_POINT('Ctrl Pts',(-44.3038659723435,-17.3513404722779,
20.));
#77061=CARTESIAN_POINT('Ctrl Pts',(-44.3131599263643,-17.3193431712198,
0.));
#77062=CARTESIAN_POINT('Ctrl Pts',(-44.3131599263643,-17.3193431712198,
20.));
#77063=CARTESIAN_POINT('Ctrl Pts',(-44.3224312504523,-17.2873404682456,
0.));
#77064=CARTESIAN_POINT('Ctrl Pts',(-44.3224312504523,-17.2873404682456,
20.));
#77065=CARTESIAN_POINT('Ctrl Pts',(-44.3316799409325,-17.2553323791649,
0.));
#77066=CARTESIAN_POINT('Ctrl Pts',(-44.3316799409325,-17.2553323791649,
20.));
#77067=CARTESIAN_POINT('Ctrl Pts',(-44.340905994141,-17.2233189197905,0.));
#77068=CARTESIAN_POINT('Ctrl Pts',(-44.340905994141,-17.2233189197905,20.));
#77069=CARTESIAN_POINT('Ctrl Pts',(-44.3501094064252,-17.1913001059384,
0.));
#77070=CARTESIAN_POINT('Ctrl Pts',(-44.3501094064252,-17.1913001059384,
20.));
#77071=CARTESIAN_POINT('Ctrl Pts',(-44.3592901741436,-17.1592759534275,
0.));
#77072=CARTESIAN_POINT('Ctrl Pts',(-44.3592901741436,-17.1592759534275,
20.));
#77073=CARTESIAN_POINT('Ctrl Pts',(-44.3684482936655,-17.1272464780797,
0.));
#77074=CARTESIAN_POINT('Ctrl Pts',(-44.3684482936655,-17.1272464780797,
20.));
#77075=CARTESIAN_POINT('Ctrl Pts',(-44.3775837613707,-17.0952116957196,
0.));
#77076=CARTESIAN_POINT('Ctrl Pts',(-44.3775837613707,-17.0952116957196,
20.));
#77077=CARTESIAN_POINT('Ctrl Pts',(-44.3866965736492,-17.0631716221745,
0.));
#77078=CARTESIAN_POINT('Ctrl Pts',(-44.3866965736492,-17.0631716221745,
20.));
#77079=CARTESIAN_POINT('Ctrl Pts',(-44.3957867269024,-17.0311262732746,
0.));
#77080=CARTESIAN_POINT('Ctrl Pts',(-44.3957867269024,-17.0311262732746,
20.));
#77081=CARTESIAN_POINT('Ctrl Pts',(-44.404854217543,-16.9990756648532,0.));
#77082=CARTESIAN_POINT('Ctrl Pts',(-44.404854217543,-16.9990756648532,20.));
#77083=CARTESIAN_POINT('Ctrl Pts',(-44.4138990419958,-16.967019812747,0.));
#77084=CARTESIAN_POINT('Ctrl Pts',(-44.4138990419958,-16.967019812747,20.));
#77085=CARTESIAN_POINT('Ctrl Pts',(-44.4229211966955,-16.9349587327952,
0.));
#77086=CARTESIAN_POINT('Ctrl Pts',(-44.4229211966955,-16.9349587327952,
20.));
#77087=CARTESIAN_POINT('Ctrl Pts',(-44.431920678088,-16.9028924408399,0.));
#77088=CARTESIAN_POINT('Ctrl Pts',(-44.431920678088,-16.9028924408399,20.));
#77089=CARTESIAN_POINT('Ctrl Pts',(-44.4408974826294,-16.870820952726,0.));
#77090=CARTESIAN_POINT('Ctrl Pts',(-44.4408974826294,-16.870820952726,20.));
#77091=CARTESIAN_POINT('Ctrl Pts',(-44.4498516067869,-16.8387442843012,
0.));
#77092=CARTESIAN_POINT('Ctrl Pts',(-44.4498516067869,-16.8387442843012,
20.));
#77093=CARTESIAN_POINT('Ctrl Pts',(-44.4587830470388,-16.8066624514163,
0.));
#77094=CARTESIAN_POINT('Ctrl Pts',(-44.4587830470388,-16.8066624514163,
20.));
#77095=CARTESIAN_POINT('Ctrl Pts',(-44.4676917998748,-16.7745754699247,
0.));
#77096=CARTESIAN_POINT('Ctrl Pts',(-44.4676917998748,-16.7745754699247,
20.));
#77097=CARTESIAN_POINT('Ctrl Pts',(-44.4765778617956,-16.742483355683,0.));
#77098=CARTESIAN_POINT('Ctrl Pts',(-44.4765778617956,-16.742483355683,20.));
#77099=CARTESIAN_POINT('Ctrl Pts',(-44.4854412293128,-16.7103861245505,
0.));
#77100=CARTESIAN_POINT('Ctrl Pts',(-44.4854412293128,-16.7103861245505,
20.));
#77101=CARTESIAN_POINT('Ctrl Pts',(-44.4942818989491,-16.6782837923892,
0.));
#77102=CARTESIAN_POINT('Ctrl Pts',(-44.4942818989491,-16.6782837923892,
20.));
#77103=CARTESIAN_POINT('Ctrl Pts',(-44.5030998672381,-16.6461763750644,
0.));
#77104=CARTESIAN_POINT('Ctrl Pts',(-44.5030998672381,-16.6461763750644,
20.));
#77105=CARTESIAN_POINT('Ctrl Pts',(-44.5118951307243,-16.6140638884438,
0.));
#77106=CARTESIAN_POINT('Ctrl Pts',(-44.5118951307243,-16.6140638884438,
20.));
#77107=CARTESIAN_POINT('Ctrl Pts',(-44.5206676859633,-16.581946348398,0.));
#77108=CARTESIAN_POINT('Ctrl Pts',(-44.5206676859633,-16.581946348398,20.));
#77109=CARTESIAN_POINT('Ctrl Pts',(-44.5294175295214,-16.5498237708003,
0.));
#77110=CARTESIAN_POINT('Ctrl Pts',(-44.5294175295214,-16.5498237708003,
20.));
#77111=CARTESIAN_POINT('Ctrl Pts',(-44.5381446579761,-16.5176961715269,
0.));
#77112=CARTESIAN_POINT('Ctrl Pts',(-44.5381446579761,-16.5176961715269,
20.));
#77113=CARTESIAN_POINT('Ctrl Pts',(-44.5468490679154,-16.4855635664567,
0.));
#77114=CARTESIAN_POINT('Ctrl Pts',(-44.5468490679154,-16.4855635664567,
20.));
#77115=CARTESIAN_POINT('Ctrl Pts',(-44.5555307559385,-16.4534259714715,
0.));
#77116=CARTESIAN_POINT('Ctrl Pts',(-44.5555307559385,-16.4534259714715,
20.));
#77117=CARTESIAN_POINT('Ctrl Pts',(-44.5641897186557,-16.4212834024559,
0.));
#77118=CARTESIAN_POINT('Ctrl Pts',(-44.5641897186557,-16.4212834024559,
20.));
#77119=CARTESIAN_POINT('Ctrl Pts',(-44.5728259526889,-16.3891358752972,
0.));
#77120=CARTESIAN_POINT('Ctrl Pts',(-44.5728259526889,-16.3891358752972,
20.));
#77121=CARTESIAN_POINT('Ctrl Pts',(-44.581439454671,-16.3569834058857,0.));
#77122=CARTESIAN_POINT('Ctrl Pts',(-44.581439454671,-16.3569834058857,20.));
#77123=CARTESIAN_POINT('Ctrl Pts',(-44.5900302212458,-16.3248260101143,
0.));
#77124=CARTESIAN_POINT('Ctrl Pts',(-44.5900302212458,-16.3248260101143,
20.));
#77125=CARTESIAN_POINT('Ctrl Pts',(-44.5985982490682,-16.2926637038787,
0.));
#77126=CARTESIAN_POINT('Ctrl Pts',(-44.5985982490682,-16.2926637038787,
20.));
#77127=CARTESIAN_POINT('Ctrl Pts',(-44.6071435348036,-16.2604965030773,
0.));
#77128=CARTESIAN_POINT('Ctrl Pts',(-44.6071435348036,-16.2604965030773,
20.));
#77129=CARTESIAN_POINT('Ctrl Pts',(-44.6156660751288,-16.2283244236112,
0.));
#77130=CARTESIAN_POINT('Ctrl Pts',(-44.6156660751288,-16.2283244236112,
20.));
#77131=CARTESIAN_POINT('Ctrl Pts',(-44.6241658667307,-16.196147481384,0.));
#77132=CARTESIAN_POINT('Ctrl Pts',(-44.6241658667307,-16.196147481384,20.));
#77133=CARTESIAN_POINT('Ctrl Pts',(-44.6326429063072,-16.1639656923022,
0.));
#77134=CARTESIAN_POINT('Ctrl Pts',(-44.6326429063072,-16.1639656923022,
20.));
#77135=CARTESIAN_POINT('Ctrl Pts',(-44.6410971905673,-16.131779072275,0.));
#77136=CARTESIAN_POINT('Ctrl Pts',(-44.6410971905673,-16.131779072275,20.));
#77137=CARTESIAN_POINT('Ctrl Pts',(-44.649528716232,-16.0995876372141,0.));
#77138=CARTESIAN_POINT('Ctrl Pts',(-44.649528716232,-16.0995876372141,20.));
#77139=CARTESIAN_POINT('Ctrl Pts',(-44.6579374800339,-16.0673914030343,
0.));
#77140=CARTESIAN_POINT('Ctrl Pts',(-44.6579374800339,-16.0673914030343,
20.));
#77141=CARTESIAN_POINT('Ctrl Pts',(-44.6663234787169,-16.0351903856534,
0.));
#77142=CARTESIAN_POINT('Ctrl Pts',(-44.6663234787169,-16.0351903856534,
20.));
#77143=CARTESIAN_POINT('Ctrl Pts',(-44.6746867090345,-16.0029846009915,
0.));
#77144=CARTESIAN_POINT('Ctrl Pts',(-44.6746867090345,-16.0029846009915,
20.));
#77145=CARTESIAN_POINT('Ctrl Pts',(-44.6830271677516,-15.9707740649715,
0.));
#77146=CARTESIAN_POINT('Ctrl Pts',(-44.6830271677516,-15.9707740649715,
20.));
#77147=CARTESIAN_POINT('Ctrl Pts',(-44.691344851643,-15.9385587935186,0.));
#77148=CARTESIAN_POINT('Ctrl Pts',(-44.691344851643,-15.9385587935186,20.));
#77149=CARTESIAN_POINT('Ctrl Pts',(-44.6996397574952,-15.9063388025603,
0.));
#77150=CARTESIAN_POINT('Ctrl Pts',(-44.6996397574952,-15.9063388025603,
20.));
#77151=CARTESIAN_POINT('Ctrl Pts',(-44.7079118821065,-15.8741141080271,
0.));
#77152=CARTESIAN_POINT('Ctrl Pts',(-44.7079118821065,-15.8741141080271,
20.));
#77153=CARTESIAN_POINT('Ctrl Pts',(-44.7161612222865,-15.8418847258528,
0.));
#77154=CARTESIAN_POINT('Ctrl Pts',(-44.7161612222865,-15.8418847258528,
20.));
#77155=CARTESIAN_POINT('Ctrl Pts',(-44.7243877748558,-15.8096506719735,
0.));
#77156=CARTESIAN_POINT('Ctrl Pts',(-44.7243877748558,-15.8096506719735,
20.));
#77157=CARTESIAN_POINT('Ctrl Pts',(-44.7325915366458,-15.7774119623278,
0.));
#77158=CARTESIAN_POINT('Ctrl Pts',(-44.7325915366458,-15.7774119623278,
20.));
#77159=CARTESIAN_POINT('Ctrl Pts',(-44.7407725044985,-15.745168612857,0.));
#77160=CARTESIAN_POINT('Ctrl Pts',(-44.7407725044985,-15.745168612857,20.));
#77161=CARTESIAN_POINT('Ctrl Pts',(-44.7489306752664,-15.7129206395047,
0.));
#77162=CARTESIAN_POINT('Ctrl Pts',(-44.7489306752664,-15.7129206395047,
20.));
#77163=CARTESIAN_POINT('Ctrl Pts',(-44.7570660458133,-15.6806680582172,
0.));
#77164=CARTESIAN_POINT('Ctrl Pts',(-44.7570660458133,-15.6806680582172,
20.));
#77165=CARTESIAN_POINT('Ctrl Pts',(-44.7651786130144,-15.6484108849434,
0.));
#77166=CARTESIAN_POINT('Ctrl Pts',(-44.7651786130144,-15.6484108849434,
20.));
#77167=CARTESIAN_POINT('Ctrl Pts',(-44.7732683737566,-15.6161491356348,
0.));
#77168=CARTESIAN_POINT('Ctrl Pts',(-44.7732683737566,-15.6161491356348,
20.));
#77169=CARTESIAN_POINT('Ctrl Pts',(-44.7813353249379,-15.583882826246,0.));
#77170=CARTESIAN_POINT('Ctrl Pts',(-44.7813353249379,-15.583882826246,20.));
#77171=CARTESIAN_POINT('Ctrl Pts',(-44.7893794634672,-15.5516119727338,
0.));
#77172=CARTESIAN_POINT('Ctrl Pts',(-44.7893794634672,-15.5516119727338,
20.));
#77173=CARTESIAN_POINT('Ctrl Pts',(-44.7974007862643,-15.5193365910578,
0.));
#77174=CARTESIAN_POINT('Ctrl Pts',(-44.7974007862643,-15.5193365910578,
20.));
#77175=CARTESIAN_POINT('Ctrl Pts',(-44.8053992902599,-15.4870566971798,
0.));
#77176=CARTESIAN_POINT('Ctrl Pts',(-44.8053992902599,-15.4870566971798,
20.));
#77177=CARTESIAN_POINT('Ctrl Pts',(-44.8133749723964,-15.4547723070643,
0.));
#77178=CARTESIAN_POINT('Ctrl Pts',(-44.8133749723964,-15.4547723070643,
20.));
#77179=CARTESIAN_POINT('Ctrl Pts',(-44.8213278296263,-15.4224834366782,
0.));
#77180=CARTESIAN_POINT('Ctrl Pts',(-44.8213278296263,-15.4224834366782,
20.));
#77181=CARTESIAN_POINT('Ctrl Pts',(-44.8292578589132,-15.3901901019906,
0.));
#77182=CARTESIAN_POINT('Ctrl Pts',(-44.8292578589132,-15.3901901019906,
20.));
#77183=CARTESIAN_POINT('Ctrl Pts',(-44.8371650572316,-15.3578923189739,
0.));
#77184=CARTESIAN_POINT('Ctrl Pts',(-44.8371650572316,-15.3578923189739,
20.));
#77185=CARTESIAN_POINT('Ctrl Pts',(-44.8450494215678,-15.3255901036026,
0.));
#77186=CARTESIAN_POINT('Ctrl Pts',(-44.8450494215678,-15.3255901036026,
20.));
#77187=CARTESIAN_POINT('Ctrl Pts',(-44.8529109489191,-15.2932834718541,
0.));
#77188=CARTESIAN_POINT('Ctrl Pts',(-44.8529109489191,-15.2932834718541,
20.));
#77189=CARTESIAN_POINT('Ctrl Pts',(-44.8607496362943,-15.2609724397079,
0.));
#77190=CARTESIAN_POINT('Ctrl Pts',(-44.8607496362943,-15.2609724397079,
20.));
#77191=CARTESIAN_POINT('Ctrl Pts',(-44.8685654807131,-15.2286570231461,
0.));
#77192=CARTESIAN_POINT('Ctrl Pts',(-44.8685654807131,-15.2286570231461,
20.));
#77193=CARTESIAN_POINT('Ctrl Pts',(-44.8763584792064,-15.1963372381533,
0.));
#77194=CARTESIAN_POINT('Ctrl Pts',(-44.8763584792064,-15.1963372381533,
20.));
#77195=CARTESIAN_POINT('Ctrl Pts',(-44.8841286288163,-15.1640131007166,
0.));
#77196=CARTESIAN_POINT('Ctrl Pts',(-44.8841286288163,-15.1640131007166,
20.));
#77197=CARTESIAN_POINT('Ctrl Pts',(-44.8918759265956,-15.1316846268256,
0.));
#77198=CARTESIAN_POINT('Ctrl Pts',(-44.8918759265956,-15.1316846268256,
20.));
#77199=CARTESIAN_POINT('Ctrl Pts',(-44.8996003696078,-15.0993518324721,
0.));
#77200=CARTESIAN_POINT('Ctrl Pts',(-44.8996003696078,-15.0993518324721,
20.));
#77201=CARTESIAN_POINT('Ctrl Pts',(-44.9073019549277,-15.0670147336509,
0.));
#77202=CARTESIAN_POINT('Ctrl Pts',(-44.9073019549277,-15.0670147336509,
20.));
#77203=CARTESIAN_POINT('Ctrl Pts',(-44.9149806796409,-15.034673346359,0.));
#77204=CARTESIAN_POINT('Ctrl Pts',(-44.9149806796409,-15.034673346359,20.));
#77205=CARTESIAN_POINT('Ctrl Pts',(-44.9226365408441,-15.0023276865958,
0.));
#77206=CARTESIAN_POINT('Ctrl Pts',(-44.9226365408441,-15.0023276865958,
20.));
#77207=CARTESIAN_POINT('Ctrl Pts',(-44.9302695356455,-14.969977770363,0.));
#77208=CARTESIAN_POINT('Ctrl Pts',(-44.9302695356455,-14.969977770363,20.));
#77209=CARTESIAN_POINT('Ctrl Pts',(-44.9378796611651,-14.9376236136649,
0.));
#77210=CARTESIAN_POINT('Ctrl Pts',(-44.9378796611651,-14.9376236136649,
20.));
#77211=CARTESIAN_POINT('Ctrl Pts',(-44.9454669145344,-14.9052652325081,
0.));
#77212=CARTESIAN_POINT('Ctrl Pts',(-44.9454669145344,-14.9052652325081,
20.));
#77213=CARTESIAN_POINT('Ctrl Pts',(-44.9530312928958,-14.8729026429019,
0.));
#77214=CARTESIAN_POINT('Ctrl Pts',(-44.9530312928958,-14.8729026429019,
20.));
#77215=CARTESIAN_POINT('Ctrl Pts',(-44.9605727934022,-14.8405358608577,
0.));
#77216=CARTESIAN_POINT('Ctrl Pts',(-44.9605727934022,-14.8405358608577,
20.));
#77217=CARTESIAN_POINT('Ctrl Pts',(-44.9680914132176,-14.8081649023895,
0.));
#77218=CARTESIAN_POINT('Ctrl Pts',(-44.9680914132176,-14.8081649023895,
20.));
#77219=CARTESIAN_POINT('Ctrl Pts',(-44.9755871495162,-14.7757897835134,
0.));
#77220=CARTESIAN_POINT('Ctrl Pts',(-44.9755871495162,-14.7757897835134,
20.));
#77221=CARTESIAN_POINT('Ctrl Pts',(-44.9830599994838,-14.7434105202483,
0.));
#77222=CARTESIAN_POINT('Ctrl Pts',(-44.9830599994838,-14.7434105202483,
20.));
#77223=CARTESIAN_POINT('Ctrl Pts',(-44.9905099603172,-14.7110271286153,
0.));
#77224=CARTESIAN_POINT('Ctrl Pts',(-44.9905099603172,-14.7110271286153,
20.));
#77225=CARTESIAN_POINT('Ctrl Pts',(-44.9979370292253,-14.6786396246378,
0.));
#77226=CARTESIAN_POINT('Ctrl Pts',(-44.9979370292253,-14.6786396246378,
20.));
#77227=CARTESIAN_POINT('Ctrl Pts',(-45.0053412034276,-14.6462480243418,
0.));
#77228=CARTESIAN_POINT('Ctrl Pts',(-45.0053412034276,-14.6462480243418,
20.));
#77229=CARTESIAN_POINT('Ctrl Pts',(-45.0127224801553,-14.6138523437553,
0.));
#77230=CARTESIAN_POINT('Ctrl Pts',(-45.0127224801553,-14.6138523437553,
20.));
#77231=CARTESIAN_POINT('Ctrl Pts',(-45.020080856651,-14.5814525989087,0.));
#77232=CARTESIAN_POINT('Ctrl Pts',(-45.020080856651,-14.5814525989087,20.));
#77233=CARTESIAN_POINT('Ctrl Pts',(-45.0274163301681,-14.5490488058349,
0.));
#77234=CARTESIAN_POINT('Ctrl Pts',(-45.0274163301681,-14.5490488058349,
20.));
#77235=CARTESIAN_POINT('Ctrl Pts',(-45.0347288979708,-14.516640980569,0.));
#77236=CARTESIAN_POINT('Ctrl Pts',(-45.0347288979708,-14.516640980569,20.));
#77237=CARTESIAN_POINT('Ctrl Pts',(-45.0420185573342,-14.4842291391484,
0.));
#77238=CARTESIAN_POINT('Ctrl Pts',(-45.0420185573342,-14.4842291391484,
20.));
#77239=CARTESIAN_POINT('Ctrl Pts',(-45.0492853055441,-14.451813297613,0.));
#77240=CARTESIAN_POINT('Ctrl Pts',(-45.0492853055441,-14.451813297613,20.));
#77241=CARTESIAN_POINT('Ctrl Pts',(-45.0565291398984,-14.4193934720051,
0.));
#77242=CARTESIAN_POINT('Ctrl Pts',(-45.0565291398984,-14.4193934720051,
20.));
#77243=CARTESIAN_POINT('Ctrl Pts',(-45.0637500577056,-14.3869696783692,
0.));
#77244=CARTESIAN_POINT('Ctrl Pts',(-45.0637500577056,-14.3869696783692,
20.));
#77245=CARTESIAN_POINT('Ctrl Pts',(-45.0709480562863,-14.354541932752,0.));
#77246=CARTESIAN_POINT('Ctrl Pts',(-45.0709480562863,-14.354541932752,20.));
#77247=CARTESIAN_POINT('Ctrl Pts',(-45.078123132972,-14.3221102512025,0.));
#77248=CARTESIAN_POINT('Ctrl Pts',(-45.078123132972,-14.3221102512025,20.));
#77249=CARTESIAN_POINT('Ctrl Pts',(-45.0852752851048,-14.2896746497719,
0.));
#77250=CARTESIAN_POINT('Ctrl Pts',(-45.0852752851048,-14.2896746497719,
20.));
#77251=CARTESIAN_POINT('Ctrl Pts',(-45.0924045100383,-14.2572351445137,
0.));
#77252=CARTESIAN_POINT('Ctrl Pts',(-45.0924045100383,-14.2572351445137,
20.));
#77253=CARTESIAN_POINT('Ctrl Pts',(-45.0995108051367,-14.2247917514836,
0.));
#77254=CARTESIAN_POINT('Ctrl Pts',(-45.0995108051367,-14.2247917514836,
20.));
#77255=CARTESIAN_POINT('Ctrl Pts',(-45.1065941677758,-14.1923444867396,
0.));
#77256=CARTESIAN_POINT('Ctrl Pts',(-45.1065941677758,-14.1923444867396,
20.));
#77257=CARTESIAN_POINT('Ctrl Pts',(-45.1136545953429,-14.1598933663422,
0.));
#77258=CARTESIAN_POINT('Ctrl Pts',(-45.1136545953429,-14.1598933663422,
20.));
#77259=CARTESIAN_POINT('Ctrl Pts',(-45.1206920852361,-14.127438406354,0.));
#77260=CARTESIAN_POINT('Ctrl Pts',(-45.1206920852361,-14.127438406354,20.));
#77261=CARTESIAN_POINT('Ctrl Pts',(-45.127706634865,-14.0949796228398,0.));
#77262=CARTESIAN_POINT('Ctrl Pts',(-45.127706634865,-14.0949796228398,20.));
#77263=CARTESIAN_POINT('Ctrl Pts',(-45.1346982416501,-14.0625170318664,
0.));
#77264=CARTESIAN_POINT('Ctrl Pts',(-45.1346982416501,-14.0625170318664,
20.));
#77265=CARTESIAN_POINT('Ctrl Pts',(-45.1416669030232,-14.0300506495033,
0.));
#77266=CARTESIAN_POINT('Ctrl Pts',(-45.1416669030232,-14.0300506495033,
20.));
#77267=CARTESIAN_POINT('Ctrl Pts',(-45.1486126164275,-13.997580491822,0.));
#77268=CARTESIAN_POINT('Ctrl Pts',(-45.1486126164275,-13.997580491822,20.));
#77269=CARTESIAN_POINT('Ctrl Pts',(-45.1555353793172,-13.9651065748961,
0.));
#77270=CARTESIAN_POINT('Ctrl Pts',(-45.1555353793172,-13.9651065748961,
20.));
#77271=CARTESIAN_POINT('Ctrl Pts',(-45.1624351891574,-13.9326289148012,
0.));
#77272=CARTESIAN_POINT('Ctrl Pts',(-45.1624351891574,-13.9326289148012,
20.));
#77273=CARTESIAN_POINT('Ctrl Pts',(-45.1693120434241,-13.9001475276153,
0.));
#77274=CARTESIAN_POINT('Ctrl Pts',(-45.1693120434241,-13.9001475276153,
20.));
#77275=CARTESIAN_POINT('Ctrl Pts',(-45.1761659396043,-13.8676624294184,
0.));
#77276=CARTESIAN_POINT('Ctrl Pts',(-45.1761659396043,-13.8676624294184,
20.));
#77277=CARTESIAN_POINT('Ctrl Pts',(-45.1829968751969,-13.8351736362929,
0.));
#77278=CARTESIAN_POINT('Ctrl Pts',(-45.1829968751969,-13.8351736362929,
20.));
#77279=CARTESIAN_POINT('Ctrl Pts',(-45.1898048477123,-13.8026811643234,
0.));
#77280=CARTESIAN_POINT('Ctrl Pts',(-45.1898048477123,-13.8026811643234,
20.));
#77281=CARTESIAN_POINT('Ctrl Pts',(-45.1965898546723,-13.7701850295967,
0.));
#77282=CARTESIAN_POINT('Ctrl Pts',(-45.1965898546723,-13.7701850295967,
20.));
#77283=CARTESIAN_POINT('Ctrl Pts',(-45.2033518936101,-13.7376852482019,
0.));
#77284=CARTESIAN_POINT('Ctrl Pts',(-45.2033518936101,-13.7376852482019,
20.));
#77285=CARTESIAN_POINT('Ctrl Pts',(-45.2100909620697,-13.7051818362299,
0.));
#77286=CARTESIAN_POINT('Ctrl Pts',(-45.2100909620697,-13.7051818362299,
20.));
#77287=CARTESIAN_POINT('Ctrl Pts',(-45.2168070576061,-13.6726748097738,
0.));
#77288=CARTESIAN_POINT('Ctrl Pts',(-45.2168070576061,-13.6726748097738,
20.));
#77289=CARTESIAN_POINT('Ctrl Pts',(-45.2235001777847,-13.6401641849286,
0.));
#77290=CARTESIAN_POINT('Ctrl Pts',(-45.2235001777847,-13.6401641849286,
20.));
#77291=CARTESIAN_POINT('Ctrl Pts',(-45.2301703201819,-13.6076499777914,
0.));
#77292=CARTESIAN_POINT('Ctrl Pts',(-45.2301703201819,-13.6076499777914,
20.));
#77293=CARTESIAN_POINT('Ctrl Pts',(-45.2368174823856,-13.5751322044618,
0.));
#77294=CARTESIAN_POINT('Ctrl Pts',(-45.2368174823856,-13.5751322044618,
20.));
#77295=CARTESIAN_POINT('Ctrl Pts',(-45.2434416619952,-13.542610881041,0.));
#77296=CARTESIAN_POINT('Ctrl Pts',(-45.2434416619952,-13.542610881041,20.));
#77297=CARTESIAN_POINT('Ctrl Pts',(-45.2500428566225,-13.5100860236329,
0.));
#77298=CARTESIAN_POINT('Ctrl Pts',(-45.2500428566225,-13.5100860236329,
20.));
#77299=CARTESIAN_POINT('Ctrl Pts',(-45.2566210638904,-13.4775576483433,
0.));
#77300=CARTESIAN_POINT('Ctrl Pts',(-45.2566210638904,-13.4775576483433,
20.));
#77301=CARTESIAN_POINT('Ctrl Pts',(-45.2631762814325,-13.44502577128,0.));
#77302=CARTESIAN_POINT('Ctrl Pts',(-45.2631762814325,-13.44502577128,20.));
#77303=CARTESIAN_POINT('Ctrl Pts',(-45.2697085068935,-13.4124904085531,
0.));
#77304=CARTESIAN_POINT('Ctrl Pts',(-45.2697085068935,-13.4124904085531,
20.));
#77305=CARTESIAN_POINT('Ctrl Pts',(-45.276217737929,-13.3799515762744,0.));
#77306=CARTESIAN_POINT('Ctrl Pts',(-45.276217737929,-13.3799515762744,20.));
#77307=CARTESIAN_POINT('Ctrl Pts',(-45.2827039722059,-13.3474092905576,
0.));
#77308=CARTESIAN_POINT('Ctrl Pts',(-45.2827039722059,-13.3474092905576,
20.));
#77309=CARTESIAN_POINT('Ctrl Pts',(-45.2891672074022,-13.3148635675188,
0.));
#77310=CARTESIAN_POINT('Ctrl Pts',(-45.2891672074022,-13.3148635675188,
20.));
#77311=CARTESIAN_POINT('Ctrl Pts',(-45.2956074412073,-13.282314423276,0.));
#77312=CARTESIAN_POINT('Ctrl Pts',(-45.2956074412073,-13.282314423276,20.));
#77313=CARTESIAN_POINT('Ctrl Pts',(-45.3020246713218,-13.2497618739494,
0.));
#77314=CARTESIAN_POINT('Ctrl Pts',(-45.3020246713218,-13.2497618739494,
20.));
#77315=CARTESIAN_POINT('Ctrl Pts',(-45.3084188954577,-13.217205935661,0.));
#77316=CARTESIAN_POINT('Ctrl Pts',(-45.3084188954577,-13.217205935661,20.));
#77317=CARTESIAN_POINT('Ctrl Pts',(-45.3147901113387,-13.1846466245352,
0.));
#77318=CARTESIAN_POINT('Ctrl Pts',(-45.3147901113387,-13.1846466245352,
20.));
#77319=CARTESIAN_POINT('Ctrl Pts',(-45.321138316699,-13.1520839566979,0.));
#77320=CARTESIAN_POINT('Ctrl Pts',(-45.321138316699,-13.1520839566979,20.));
#77321=CARTESIAN_POINT('Ctrl Pts',(-45.3274635092846,-13.1195179482773,
0.));
#77322=CARTESIAN_POINT('Ctrl Pts',(-45.3274635092846,-13.1195179482773,
20.));
#77323=CARTESIAN_POINT('Ctrl Pts',(-45.3337656868523,-13.0869486154035,
0.));
#77324=CARTESIAN_POINT('Ctrl Pts',(-45.3337656868523,-13.0869486154035,
20.));
#77325=CARTESIAN_POINT('Ctrl Pts',(-45.3400448471699,-13.0543759742083,
0.));
#77326=CARTESIAN_POINT('Ctrl Pts',(-45.3400448471699,-13.0543759742083,
20.));
#77327=CARTESIAN_POINT('Ctrl Pts',(-45.3463009880171,-13.021800040826,0.));
#77328=CARTESIAN_POINT('Ctrl Pts',(-45.3463009880171,-13.021800040826,20.));
#77329=CARTESIAN_POINT('Ctrl Pts',(-45.3525341071849,-12.9892208313927,
0.));
#77330=CARTESIAN_POINT('Ctrl Pts',(-45.3525341071849,-12.9892208313927,
20.));
#77331=CARTESIAN_POINT('Ctrl Pts',(-45.3587442024753,-12.9566383620464,
0.));
#77332=CARTESIAN_POINT('Ctrl Pts',(-45.3587442024753,-12.9566383620464,
20.));
#77333=CARTESIAN_POINT('Ctrl Pts',(-45.3649312717011,-12.9240526489272,
0.));
#77334=CARTESIAN_POINT('Ctrl Pts',(-45.3649312717011,-12.9240526489272,
20.));
#77335=CARTESIAN_POINT('Ctrl Pts',(-45.371095312686,-12.8914637081769,0.));
#77336=CARTESIAN_POINT('Ctrl Pts',(-45.371095312686,-12.8914637081769,20.));
#77337=CARTESIAN_POINT('Ctrl Pts',(-45.3772363232658,-12.8588715559393,
0.));
#77338=CARTESIAN_POINT('Ctrl Pts',(-45.3772363232658,-12.8588715559393,
20.));
#77339=CARTESIAN_POINT('Ctrl Pts',(-45.3833543012877,-12.82627620836,0.));
#77340=CARTESIAN_POINT('Ctrl Pts',(-45.3833543012877,-12.82627620836,20.));
#77341=CARTESIAN_POINT('Ctrl Pts',(-45.3894492446102,-12.7936776815868,
0.));
#77342=CARTESIAN_POINT('Ctrl Pts',(-45.3894492446102,-12.7936776815868,
20.));
#77343=CARTESIAN_POINT('Ctrl Pts',(-45.3955211511034,-12.7610759917694,
0.));
#77344=CARTESIAN_POINT('Ctrl Pts',(-45.3955211511034,-12.7610759917694,
20.));
#77345=CARTESIAN_POINT('Ctrl Pts',(-45.4015700186485,-12.7284711550592,
0.));
#77346=CARTESIAN_POINT('Ctrl Pts',(-45.4015700186485,-12.7284711550592,
20.));
#77347=CARTESIAN_POINT('Ctrl Pts',(-45.407595845137,-12.6958631876099,0.));
#77348=CARTESIAN_POINT('Ctrl Pts',(-45.407595845137,-12.6958631876099,20.));
#77349=CARTESIAN_POINT('Ctrl Pts',(-45.4135986284717,-12.6632521055766,
0.));
#77350=CARTESIAN_POINT('Ctrl Pts',(-45.4135986284717,-12.6632521055766,
20.));
#77351=CARTESIAN_POINT('Ctrl Pts',(-45.4195783665665,-12.6306379251164,
0.));
#77352=CARTESIAN_POINT('Ctrl Pts',(-45.4195783665665,-12.6306379251164,
20.));
#77353=CARTESIAN_POINT('Ctrl Pts',(-45.4255350573473,-12.5980206623884,
0.));
#77354=CARTESIAN_POINT('Ctrl Pts',(-45.4255350573473,-12.5980206623884,
20.));
#77355=CARTESIAN_POINT('Ctrl Pts',(-45.4314686987515,-12.5654003335532,
0.));
#77356=CARTESIAN_POINT('Ctrl Pts',(-45.4314686987515,-12.5654003335532,
20.));
#77357=CARTESIAN_POINT('Ctrl Pts',(-45.4373792887274,-12.5327769547739,
0.));
#77358=CARTESIAN_POINT('Ctrl Pts',(-45.4373792887274,-12.5327769547739,
20.));
#77359=CARTESIAN_POINT('Ctrl Pts',(-45.4432668252347,-12.500150542215,0.));
#77360=CARTESIAN_POINT('Ctrl Pts',(-45.4432668252347,-12.500150542215,20.));
#77361=CARTESIAN_POINT('Ctrl Pts',(-45.4491313062444,-12.4675211120431,
0.));
#77362=CARTESIAN_POINT('Ctrl Pts',(-45.4491313062444,-12.4675211120431,
20.));
#77363=CARTESIAN_POINT('Ctrl Pts',(-45.4549727297392,-12.4348886804266,
0.));
#77364=CARTESIAN_POINT('Ctrl Pts',(-45.4549727297392,-12.4348886804266,
20.));
#77365=CARTESIAN_POINT('Ctrl Pts',(-45.4607910937128,-12.4022532635357,
0.));
#77366=CARTESIAN_POINT('Ctrl Pts',(-45.4607910937128,-12.4022532635357,
20.));
#77367=CARTESIAN_POINT('Ctrl Pts',(-45.4665863961701,-12.3696148775423,
0.));
#77368=CARTESIAN_POINT('Ctrl Pts',(-45.4665863961701,-12.3696148775423,
20.));
#77369=CARTESIAN_POINT('Ctrl Pts',(-45.4723586351267,-12.3369735386201,
0.));
#77370=CARTESIAN_POINT('Ctrl Pts',(-45.4723586351267,-12.3369735386201,
20.));
#77371=CARTESIAN_POINT('Ctrl Pts',(-45.4781078086095,-12.3043292629445,
0.));
#77372=CARTESIAN_POINT('Ctrl Pts',(-45.4781078086095,-12.3043292629445,
20.));
#77373=CARTESIAN_POINT('Ctrl Pts',(-45.483833914657,-12.2716820666929,0.));
#77374=CARTESIAN_POINT('Ctrl Pts',(-45.483833914657,-12.2716820666929,20.));
#77375=CARTESIAN_POINT('Ctrl Pts',(-45.4895369513189,-12.2390319660445,
0.));
#77376=CARTESIAN_POINT('Ctrl Pts',(-45.4895369513189,-12.2390319660445,
20.));
#77377=CARTESIAN_POINT('Ctrl Pts',(-45.4952169166561,-12.2063789771801,
0.));
#77378=CARTESIAN_POINT('Ctrl Pts',(-45.4952169166561,-12.2063789771801,
20.));
#77379=CARTESIAN_POINT('Ctrl Pts',(-45.5008738087416,-12.1737231162825,
0.));
#77380=CARTESIAN_POINT('Ctrl Pts',(-45.5008738087416,-12.1737231162825,
20.));
#77381=CARTESIAN_POINT('Ctrl Pts',(-45.5065076256599,-12.1410643995363,
0.));
#77382=CARTESIAN_POINT('Ctrl Pts',(-45.5065076256599,-12.1410643995363,
20.));
#77383=CARTESIAN_POINT('Ctrl Pts',(-45.5121183655068,-12.1084028431278,
0.));
#77384=CARTESIAN_POINT('Ctrl Pts',(-45.5121183655068,-12.1084028431278,
20.));
#77385=CARTESIAN_POINT('Ctrl Pts',(-45.5177060263888,-12.0757384632451,
0.));
#77386=CARTESIAN_POINT('Ctrl Pts',(-45.5177060263888,-12.0757384632451,
20.));
#77387=CARTESIAN_POINT('Ctrl Pts',(-45.5232706064237,-12.0430712760778,
0.));
#77388=CARTESIAN_POINT('Ctrl Pts',(-45.5232706064237,-12.0430712760778,
20.));
#77389=CARTESIAN_POINT('Ctrl Pts',(-45.5288121037395,-12.0104012978174,
0.));
#77390=CARTESIAN_POINT('Ctrl Pts',(-45.5288121037395,-12.0104012978174,
20.));
#77391=CARTESIAN_POINT('Ctrl Pts',(-45.5343305164759,-11.9777285446569,
0.));
#77392=CARTESIAN_POINT('Ctrl Pts',(-45.5343305164759,-11.9777285446569,
20.));
#77393=CARTESIAN_POINT('Ctrl Pts',(-45.5398258427845,-11.945053032791,0.));
#77394=CARTESIAN_POINT('Ctrl Pts',(-45.5398258427845,-11.945053032791,20.));
#77395=CARTESIAN_POINT('Ctrl Pts',(-45.5452980808284,-11.9123747784165,
0.));
#77396=CARTESIAN_POINT('Ctrl Pts',(-45.5452980808284,-11.9123747784165,
20.));
#77397=CARTESIAN_POINT('Ctrl Pts',(-45.5507472287824,-11.8796937977314,
0.));
#77398=CARTESIAN_POINT('Ctrl Pts',(-45.5507472287824,-11.8796937977314,
20.));
#77399=CARTESIAN_POINT('Ctrl Pts',(-45.5561732848327,-11.8470101069358,
0.));
#77400=CARTESIAN_POINT('Ctrl Pts',(-45.5561732848327,-11.8470101069358,
20.));
#77401=CARTESIAN_POINT('Ctrl Pts',(-45.5615762471761,-11.8143237222317,
0.));
#77402=CARTESIAN_POINT('Ctrl Pts',(-45.5615762471761,-11.8143237222317,
20.));
#77403=CARTESIAN_POINT('Ctrl Pts',(-45.5669561140206,-11.7816346598227,
0.));
#77404=CARTESIAN_POINT('Ctrl Pts',(-45.5669561140206,-11.7816346598227,
20.));
#77405=CARTESIAN_POINT('Ctrl Pts',(-45.5723128835857,-11.748942935914,0.));
#77406=CARTESIAN_POINT('Ctrl Pts',(-45.5723128835857,-11.748942935914,20.));
#77407=CARTESIAN_POINT('Ctrl Pts',(-45.5776465541021,-11.7162485667124,
0.));
#77408=CARTESIAN_POINT('Ctrl Pts',(-45.5776465541021,-11.7162485667124,
20.));
#77409=CARTESIAN_POINT('Ctrl Pts',(-45.5829571238122,-11.6835515684258,
0.));
#77410=CARTESIAN_POINT('Ctrl Pts',(-45.5829571238122,-11.6835515684258,
20.));
#77411=CARTESIAN_POINT('Ctrl Pts',(-45.5882445909695,-11.6508519572639,
0.));
#77412=CARTESIAN_POINT('Ctrl Pts',(-45.5882445909695,-11.6508519572639,
20.));
#77413=CARTESIAN_POINT('Ctrl Pts',(-45.5935089538387,-11.6181497494381,
0.));
#77414=CARTESIAN_POINT('Ctrl Pts',(-45.5935089538387,-11.6181497494381,
20.));
#77415=CARTESIAN_POINT('Ctrl Pts',(-45.598750210696,-11.5854449611619,0.));
#77416=CARTESIAN_POINT('Ctrl Pts',(-45.598750210696,-11.5854449611619,20.));
#77417=CARTESIAN_POINT('Ctrl Pts',(-45.6039683598295,-11.5527376086502,
0.));
#77418=CARTESIAN_POINT('Ctrl Pts',(-45.6039683598295,-11.5527376086502,
20.));
#77419=CARTESIAN_POINT('Ctrl Pts',(-45.6091633995383,-11.5200277081201,
0.));
#77420=CARTESIAN_POINT('Ctrl Pts',(-45.6091633995383,-11.5200277081201,
20.));
#77421=CARTESIAN_POINT('Ctrl Pts',(-45.6143353281323,-11.4873152757897,
0.));
#77422=CARTESIAN_POINT('Ctrl Pts',(-45.6143353281323,-11.4873152757897,
20.));
#77423=CARTESIAN_POINT('Ctrl Pts',(-45.6194841439321,-11.4546003278786,
0.));
#77424=CARTESIAN_POINT('Ctrl Pts',(-45.6194841439321,-11.4546003278786,
20.));
#77425=CARTESIAN_POINT('Ctrl Pts',(-45.6246098452703,-11.421882880608,0.));
#77426=CARTESIAN_POINT('Ctrl Pts',(-45.6246098452703,-11.421882880608,20.));
#77427=CARTESIAN_POINT('Ctrl Pts',(-45.6297124304911,-11.3891629502006,
0.));
#77428=CARTESIAN_POINT('Ctrl Pts',(-45.6297124304911,-11.3891629502006,
20.));
#77429=CARTESIAN_POINT('Ctrl Pts',(-45.6347918979506,-11.3564405528809,
0.));
#77430=CARTESIAN_POINT('Ctrl Pts',(-45.6347918979506,-11.3564405528809,
20.));
#77431=CARTESIAN_POINT('Ctrl Pts',(-45.6398482460165,-11.3237157048751,
0.));
#77432=CARTESIAN_POINT('Ctrl Pts',(-45.6398482460165,-11.3237157048751,
20.));
#77433=CARTESIAN_POINT('Ctrl Pts',(-45.6448814730677,-11.290988422411,0.));
#77434=CARTESIAN_POINT('Ctrl Pts',(-45.6448814730677,-11.290988422411,20.));
#77435=CARTESIAN_POINT('Ctrl Pts',(-45.6498915774933,-11.2582587217178,
0.));
#77436=CARTESIAN_POINT('Ctrl Pts',(-45.6498915774933,-11.2582587217178,
20.));
#77437=CARTESIAN_POINT('Ctrl Pts',(-45.6548785576938,-11.2255266190259,
0.));
#77438=CARTESIAN_POINT('Ctrl Pts',(-45.6548785576938,-11.2255266190259,
20.));
#77439=CARTESIAN_POINT('Ctrl Pts',(-45.6598424120808,-11.1927921305675,
0.));
#77440=CARTESIAN_POINT('Ctrl Pts',(-45.6598424120808,-11.1927921305675,
20.));
#77441=CARTESIAN_POINT('Ctrl Pts',(-45.6647831390778,-11.1600552725764,
0.));
#77442=CARTESIAN_POINT('Ctrl Pts',(-45.6647831390778,-11.1600552725764,
20.));
#77443=CARTESIAN_POINT('Ctrl Pts',(-45.6697007371202,-11.1273160612881,
0.));
#77444=CARTESIAN_POINT('Ctrl Pts',(-45.6697007371202,-11.1273160612881,
20.));
#77445=CARTESIAN_POINT('Ctrl Pts',(-45.6745952046549,-11.0945745129393,
0.));
#77446=CARTESIAN_POINT('Ctrl Pts',(-45.6745952046549,-11.0945745129393,
20.));
#77447=CARTESIAN_POINT('Ctrl Pts',(-45.6794665401395,-11.0618306437685,
0.));
#77448=CARTESIAN_POINT('Ctrl Pts',(-45.6794665401395,-11.0618306437685,
20.));
#77449=CARTESIAN_POINT('Ctrl Pts',(-45.684314742043,-11.0290844700154,0.));
#77450=CARTESIAN_POINT('Ctrl Pts',(-45.684314742043,-11.0290844700154,20.));
#77451=CARTESIAN_POINT('Ctrl Pts',(-45.6891398088456,-10.9963360079212,
0.));
#77452=CARTESIAN_POINT('Ctrl Pts',(-45.6891398088456,-10.9963360079212,
20.));
#77453=CARTESIAN_POINT('Ctrl Pts',(-45.6939417390393,-10.9635852737287,
0.));
#77454=CARTESIAN_POINT('Ctrl Pts',(-45.6939417390393,-10.9635852737287,
20.));
#77455=CARTESIAN_POINT('Ctrl Pts',(-45.698720531127,-10.930832283682,0.));
#77456=CARTESIAN_POINT('Ctrl Pts',(-45.698720531127,-10.930832283682,20.));
#77457=CARTESIAN_POINT('Ctrl Pts',(-45.7034761836229,-10.8980770540269,
0.));
#77458=CARTESIAN_POINT('Ctrl Pts',(-45.7034761836229,-10.8980770540269,
20.));
#77459=CARTESIAN_POINT('Ctrl Pts',(-45.7082086950532,-10.8653196010107,
0.));
#77460=CARTESIAN_POINT('Ctrl Pts',(-45.7082086950532,-10.8653196010107,
20.));
#77461=CARTESIAN_POINT('Ctrl Pts',(-45.7129180639559,-10.832559940882,0.));
#77462=CARTESIAN_POINT('Ctrl Pts',(-45.7129180639559,-10.832559940882,20.));
#77463=CARTESIAN_POINT('Ctrl Pts',(-45.7176042888794,-10.7997980898913,
0.));
#77464=CARTESIAN_POINT('Ctrl Pts',(-45.7176042888794,-10.7997980898913,
20.));
#77465=CARTESIAN_POINT('Ctrl Pts',(-45.7222673683833,-10.7670340642896,
0.));
#77466=CARTESIAN_POINT('Ctrl Pts',(-45.7222673683833,-10.7670340642896,
20.));
#77467=CARTESIAN_POINT('Ctrl Pts',(-45.7269073010391,-10.73426788033,0.));
#77468=CARTESIAN_POINT('Ctrl Pts',(-45.7269073010391,-10.73426788033,20.));
#77469=CARTESIAN_POINT('Ctrl Pts',(-45.7315240854293,-10.7014995542666,
0.));
#77470=CARTESIAN_POINT('Ctrl Pts',(-45.7315240854293,-10.7014995542666,
20.));
#77471=CARTESIAN_POINT('Ctrl Pts',(-45.7361177201484,-10.6687291023553,
0.));
#77472=CARTESIAN_POINT('Ctrl Pts',(-45.7361177201484,-10.6687291023553,
20.));
#77473=CARTESIAN_POINT('Ctrl Pts',(-45.7406882038015,-10.6359565408533,
0.));
#77474=CARTESIAN_POINT('Ctrl Pts',(-45.7406882038015,-10.6359565408533,
20.));
#77475=CARTESIAN_POINT('Ctrl Pts',(-45.745235535006,-10.6031818860194,0.));
#77476=CARTESIAN_POINT('Ctrl Pts',(-45.745235535006,-10.6031818860194,20.));
#77477=CARTESIAN_POINT('Ctrl Pts',(-45.7497597123901,-10.5704051541135,
0.));
#77478=CARTESIAN_POINT('Ctrl Pts',(-45.7497597123901,-10.5704051541135,
20.));
#77479=CARTESIAN_POINT('Ctrl Pts',(-45.7542607345937,-10.5376263613968,
0.));
#77480=CARTESIAN_POINT('Ctrl Pts',(-45.7542607345937,-10.5376263613968,
20.));
#77481=CARTESIAN_POINT('Ctrl Pts',(-45.7587386002674,-10.504845524132,0.));
#77482=CARTESIAN_POINT('Ctrl Pts',(-45.7587386002674,-10.504845524132,20.));
#77483=CARTESIAN_POINT('Ctrl Pts',(-45.7631933080735,-10.4720626585828,
0.));
#77484=CARTESIAN_POINT('Ctrl Pts',(-45.7631933080735,-10.4720626585828,
20.));
#77485=CARTESIAN_POINT('Ctrl Pts',(-45.7676248566855,-10.4392777810149,
0.));
#77486=CARTESIAN_POINT('Ctrl Pts',(-45.7676248566855,-10.4392777810149,
20.));
#77487=CARTESIAN_POINT('Ctrl Pts',(-45.772033244789,-10.406490907695,0.));
#77488=CARTESIAN_POINT('Ctrl Pts',(-45.772033244789,-10.406490907695,20.));
#77489=CARTESIAN_POINT('Ctrl Pts',(-45.7764184710811,-10.3737020548914,
0.));
#77490=CARTESIAN_POINT('Ctrl Pts',(-45.7764184710811,-10.3737020548914,
20.));
#77491=CARTESIAN_POINT('Ctrl Pts',(-45.7807805342697,-10.3409112388736,
0.));
#77492=CARTESIAN_POINT('Ctrl Pts',(-45.7807805342697,-10.3409112388736,
20.));
#77493=CARTESIAN_POINT('Ctrl Pts',(-45.7851194330743,-10.3081184759123,
0.));
#77494=CARTESIAN_POINT('Ctrl Pts',(-45.7851194330743,-10.3081184759123,
20.));
#77495=CARTESIAN_POINT('Ctrl Pts',(-45.7894351662253,-10.2753237822795,
0.));
#77496=CARTESIAN_POINT('Ctrl Pts',(-45.7894351662253,-10.2753237822795,
20.));
#77497=CARTESIAN_POINT('Ctrl Pts',(-45.7937277324643,-10.2425271742485,
0.));
#77498=CARTESIAN_POINT('Ctrl Pts',(-45.7937277324643,-10.2425271742485,
20.));
#77499=CARTESIAN_POINT('Ctrl Pts',(-45.7979971305449,-10.2097286680937,
0.));
#77500=CARTESIAN_POINT('Ctrl Pts',(-45.7979971305449,-10.2097286680937,
20.));
#77501=CARTESIAN_POINT('Ctrl Pts',(-45.8022433592327,-10.1769282800914,
0.));
#77502=CARTESIAN_POINT('Ctrl Pts',(-45.8022433592327,-10.1769282800914,
20.));
#77503=CARTESIAN_POINT('Ctrl Pts',(-45.8064664173048,-10.1441260265191,
0.));
#77504=CARTESIAN_POINT('Ctrl Pts',(-45.8064664173048,-10.1441260265191,
20.));
#77505=CARTESIAN_POINT('Ctrl Pts',(-45.8106663035491,-10.1113219236554,
0.));
#77506=CARTESIAN_POINT('Ctrl Pts',(-45.8106663035491,-10.1113219236554,
20.));
#77507=CARTESIAN_POINT('Ctrl Pts',(-45.8148430167647,-10.0785159877801,
0.));
#77508=CARTESIAN_POINT('Ctrl Pts',(-45.8148430167647,-10.0785159877801,
20.));
#77509=CARTESIAN_POINT('Ctrl Pts',(-45.8189965557614,-10.0457082351741,
0.));
#77510=CARTESIAN_POINT('Ctrl Pts',(-45.8189965557614,-10.0457082351741,
20.));
#77511=CARTESIAN_POINT('Ctrl Pts',(-45.8231269193611,-10.0128986821194,
0.));
#77512=CARTESIAN_POINT('Ctrl Pts',(-45.8231269193611,-10.0128986821194,
20.));
#77513=CARTESIAN_POINT('Ctrl Pts',(-45.8272341063969,-9.98008734489947,
0.));
#77514=CARTESIAN_POINT('Ctrl Pts',(-45.8272341063969,-9.98008734489947,
20.));
#77515=CARTESIAN_POINT('Ctrl Pts',(-45.8313181157134,-9.94727423979905,
0.));
#77516=CARTESIAN_POINT('Ctrl Pts',(-45.8313181157134,-9.94727423979905,
20.));
#77517=CARTESIAN_POINT('Ctrl Pts',(-45.8353789461673,-9.91445938310424,
0.));
#77518=CARTESIAN_POINT('Ctrl Pts',(-45.8353789461673,-9.91445938310424,
20.));
#77519=CARTESIAN_POINT('Ctrl Pts',(-45.8394165966264,-9.88164279110241,
0.));
#77520=CARTESIAN_POINT('Ctrl Pts',(-45.8394165966264,-9.88164279110241,
20.));
#77521=CARTESIAN_POINT('Ctrl Pts',(-45.84343106597,-9.84882448008225,0.));
#77522=CARTESIAN_POINT('Ctrl Pts',(-45.84343106597,-9.84882448008225,20.));
#77523=CARTESIAN_POINT('Ctrl Pts',(-45.8474223530896,-9.81600446633367,
0.));
#77524=CARTESIAN_POINT('Ctrl Pts',(-45.8474223530896,-9.81600446633367,
20.));
#77525=CARTESIAN_POINT('Ctrl Pts',(-45.8513904568872,-9.78318276614761,
0.));
#77526=CARTESIAN_POINT('Ctrl Pts',(-45.8513904568872,-9.78318276614761,
20.));
#77527=CARTESIAN_POINT('Ctrl Pts',(-45.8553353762765,-9.75035939581618,
0.));
#77528=CARTESIAN_POINT('Ctrl Pts',(-45.8553353762765,-9.75035939581618,
20.));
#77529=CARTESIAN_POINT('Ctrl Pts',(-45.8592571101813,-9.7175343716322,0.));
#77530=CARTESIAN_POINT('Ctrl Pts',(-45.8592571101813,-9.7175343716322,20.));
#77531=CARTESIAN_POINT('Ctrl Pts',(-45.8631556575366,-9.68470770988975,
0.));
#77532=CARTESIAN_POINT('Ctrl Pts',(-45.8631556575366,-9.68470770988975,
20.));
#77533=CARTESIAN_POINT('Ctrl Pts',(-45.8670310172895,-9.65187942688401,
0.));
#77534=CARTESIAN_POINT('Ctrl Pts',(-45.8670310172895,-9.65187942688401,
20.));
#77535=CARTESIAN_POINT('Ctrl Pts',(-45.870883188399,-9.61904953891159,0.));
#77536=CARTESIAN_POINT('Ctrl Pts',(-45.870883188399,-9.61904953891159,20.));
#77537=CARTESIAN_POINT('Ctrl Pts',(-45.8747121698355,-9.58621806227057,
0.));
#77538=CARTESIAN_POINT('Ctrl Pts',(-45.8747121698355,-9.58621806227057,
20.));
#77539=CARTESIAN_POINT('Ctrl Pts',(-45.8785179605829,-9.55338501326047,
0.));
#77540=CARTESIAN_POINT('Ctrl Pts',(-45.8785179605829,-9.55338501326047,
20.));
#77541=CARTESIAN_POINT('Ctrl Pts',(-45.882300559635,-9.52055040818184,0.));
#77542=CARTESIAN_POINT('Ctrl Pts',(-45.882300559635,-9.52055040818184,20.));
#77543=CARTESIAN_POINT('Ctrl Pts',(-45.8860599659967,-9.48771426333609,
0.));
#77544=CARTESIAN_POINT('Ctrl Pts',(-45.8860599659967,-9.48771426333609,
20.));
#77545=CARTESIAN_POINT('Ctrl Pts',(-45.8897961786838,-9.45487659502548,
0.));
#77546=CARTESIAN_POINT('Ctrl Pts',(-45.8897961786838,-9.45487659502548,
20.));
#77547=CARTESIAN_POINT('Ctrl Pts',(-45.8935091967241,-9.42203741955324,
0.));
#77548=CARTESIAN_POINT('Ctrl Pts',(-45.8935091967241,-9.42203741955324,
20.));
#77549=CARTESIAN_POINT('Ctrl Pts',(-45.8971990191563,-9.3891967532238,0.));
#77550=CARTESIAN_POINT('Ctrl Pts',(-45.8971990191563,-9.3891967532238,20.));
#77551=CARTESIAN_POINT('Ctrl Pts',(-45.90086564503,-9.35635461234246,0.));
#77552=CARTESIAN_POINT('Ctrl Pts',(-45.90086564503,-9.35635461234246,20.));
#77553=CARTESIAN_POINT('Ctrl Pts',(-45.9045090734063,-9.32351101321579,
0.));
#77554=CARTESIAN_POINT('Ctrl Pts',(-45.9045090734063,-9.32351101321579,
20.));
#77555=CARTESIAN_POINT('Ctrl Pts',(-45.9081293033577,-9.29066597215162,
0.));
#77556=CARTESIAN_POINT('Ctrl Pts',(-45.9081293033577,-9.29066597215162,
20.));
#77557=CARTESIAN_POINT('Ctrl Pts',(-45.9117263339694,-9.25781950545901,
0.));
#77558=CARTESIAN_POINT('Ctrl Pts',(-45.9117263339694,-9.25781950545901,
20.));
#77559=CARTESIAN_POINT('Ctrl Pts',(-45.9153001643391,-9.22497162944821,
0.));
#77560=CARTESIAN_POINT('Ctrl Pts',(-45.9153001643391,-9.22497162944821,
20.));
#77561=CARTESIAN_POINT('Ctrl Pts',(-45.9188507935764,-9.19212236043073,
0.));
#77562=CARTESIAN_POINT('Ctrl Pts',(-45.9188507935764,-9.19212236043073,
20.));
#77563=CARTESIAN_POINT('Ctrl Pts',(-45.9223782208015,-9.15927171471891,
0.));
#77564=CARTESIAN_POINT('Ctrl Pts',(-45.9223782208015,-9.15927171471891,
20.));
#77565=CARTESIAN_POINT('Ctrl Pts',(-45.9258824451441,-9.12641970862566,
0.));
#77566=CARTESIAN_POINT('Ctrl Pts',(-45.9258824451441,-9.12641970862566,
20.));
#77567=CARTESIAN_POINT('Ctrl Pts',(-45.9293634657451,-9.09356635846485,
0.));
#77568=CARTESIAN_POINT('Ctrl Pts',(-45.9293634657451,-9.09356635846485,
20.));
#77569=CARTESIAN_POINT('Ctrl Pts',(-45.9328212817567,-9.06071168055121,
0.));
#77570=CARTESIAN_POINT('Ctrl Pts',(-45.9328212817567,-9.06071168055121,
20.));
#77571=CARTESIAN_POINT('Ctrl Pts',(-45.9362558923428,-9.02785569120061,
0.));
#77572=CARTESIAN_POINT('Ctrl Pts',(-45.9362558923428,-9.02785569120061,
20.));
#77573=CARTESIAN_POINT('Ctrl Pts',(-45.939667296681,-8.99499840673046,0.));
#77574=CARTESIAN_POINT('Ctrl Pts',(-45.939667296681,-8.99499840673046,20.));
#77575=CARTESIAN_POINT('Ctrl Pts',(-45.9430554939595,-8.96213984345905,
0.));
#77576=CARTESIAN_POINT('Ctrl Pts',(-45.9430554939595,-8.96213984345905,
20.));
#77577=CARTESIAN_POINT('Ctrl Pts',(-45.9464204833787,-8.92928001770575,
0.));
#77578=CARTESIAN_POINT('Ctrl Pts',(-45.9464204833787,-8.92928001770575,
20.));
#77579=CARTESIAN_POINT('Ctrl Pts',(-45.9497622641496,-8.89641894579082,
0.));
#77580=CARTESIAN_POINT('Ctrl Pts',(-45.9497622641496,-8.89641894579082,
20.));
#77581=CARTESIAN_POINT('Ctrl Pts',(-45.9530808354938,-8.86355664403534,
0.));
#77582=CARTESIAN_POINT('Ctrl Pts',(-45.9530808354938,-8.86355664403534,
20.));
#77583=CARTESIAN_POINT('Ctrl Pts',(-45.9563761966444,-8.83069312876127,
0.));
#77584=CARTESIAN_POINT('Ctrl Pts',(-45.9563761966444,-8.83069312876127,
20.));
#77585=CARTESIAN_POINT('Ctrl Pts',(-45.9596483468462,-8.79782841629147,
0.));
#77586=CARTESIAN_POINT('Ctrl Pts',(-45.9596483468462,-8.79782841629147,
20.));
#77587=CARTESIAN_POINT('Ctrl Pts',(-45.9628972853566,-8.76496252295001,
0.));
#77588=CARTESIAN_POINT('Ctrl Pts',(-45.9628972853566,-8.76496252295001,
20.));
#77589=CARTESIAN_POINT('Ctrl Pts',(-45.9661230114446,-8.73209546506199,
0.));
#77590=CARTESIAN_POINT('Ctrl Pts',(-45.9661230114446,-8.73209546506199,
20.));
#77591=CARTESIAN_POINT('Ctrl Pts',(-45.9693255243897,-8.69922725895329,
0.));
#77592=CARTESIAN_POINT('Ctrl Pts',(-45.9693255243897,-8.69922725895329,
20.));
#77593=CARTESIAN_POINT('Ctrl Pts',(-45.9725048234817,-8.66635792095043,
0.));
#77594=CARTESIAN_POINT('Ctrl Pts',(-45.9725048234817,-8.66635792095043,
20.));
#77595=CARTESIAN_POINT('Ctrl Pts',(-45.9756609080225,-8.63348746738099,
0.));
#77596=CARTESIAN_POINT('Ctrl Pts',(-45.9756609080225,-8.63348746738099,
20.));
#77597=CARTESIAN_POINT('Ctrl Pts',(-45.9787937773254,-8.60061591457339,
0.));
#77598=CARTESIAN_POINT('Ctrl Pts',(-45.9787937773254,-8.60061591457339,
20.));
#77599=CARTESIAN_POINT('Ctrl Pts',(-45.9819034307166,-8.56774327885725,
0.));
#77600=CARTESIAN_POINT('Ctrl Pts',(-45.9819034307166,-8.56774327885725,
20.));
#77601=CARTESIAN_POINT('Ctrl Pts',(-45.9849898675351,-8.53486957656347,
0.));
#77602=CARTESIAN_POINT('Ctrl Pts',(-45.9849898675351,-8.53486957656347,
20.));
#77603=CARTESIAN_POINT('Ctrl Pts',(-45.9880530871298,-8.50199482402354,
0.));
#77604=CARTESIAN_POINT('Ctrl Pts',(-45.9880530871298,-8.50199482402354,
20.));
#77605=CARTESIAN_POINT('Ctrl Pts',(-45.991093088861,-8.46911903756973,0.));
#77606=CARTESIAN_POINT('Ctrl Pts',(-45.991093088861,-8.46911903756973,20.));
#77607=CARTESIAN_POINT('Ctrl Pts',(-45.9941098720982,-8.43624223353471,
0.));
#77608=CARTESIAN_POINT('Ctrl Pts',(-45.9941098720982,-8.43624223353471,
20.));
#77609=CARTESIAN_POINT('Ctrl Pts',(-45.9971034362229,-8.40336442825199,
0.));
#77610=CARTESIAN_POINT('Ctrl Pts',(-45.9971034362229,-8.40336442825199,
20.));
#77611=CARTESIAN_POINT('Ctrl Pts',(-46.000073780629,-8.37048563805605,0.));
#77612=CARTESIAN_POINT('Ctrl Pts',(-46.000073780629,-8.37048563805605,20.));
#77613=CARTESIAN_POINT('Ctrl Pts',(-46.0030209047226,-8.33760587928253,
0.));
#77614=CARTESIAN_POINT('Ctrl Pts',(-46.0030209047226,-8.33760587928253,
20.));
#77615=CARTESIAN_POINT('Ctrl Pts',(-46.0059448079215,-8.30472516826797,
0.));
#77616=CARTESIAN_POINT('Ctrl Pts',(-46.0059448079215,-8.30472516826797,
20.));
#77617=CARTESIAN_POINT('Ctrl Pts',(-46.0088454896554,-8.27184352134994,
0.));
#77618=CARTESIAN_POINT('Ctrl Pts',(-46.0088454896554,-8.27184352134994,
20.));
#77619=CARTESIAN_POINT('Ctrl Pts',(-46.0117229493647,-8.23896095486669,
0.));
#77620=CARTESIAN_POINT('Ctrl Pts',(-46.0117229493647,-8.23896095486669,
20.));
#77621=CARTESIAN_POINT('Ctrl Pts',(-46.0145771865005,-8.20607748515696,
0.));
#77622=CARTESIAN_POINT('Ctrl Pts',(-46.0145771865005,-8.20607748515696,
20.));
#77623=CARTESIAN_POINT('Ctrl Pts',(-46.0174082005262,-8.17319312856042,
0.));
#77624=CARTESIAN_POINT('Ctrl Pts',(-46.0174082005262,-8.17319312856042,
20.));
#77625=CARTESIAN_POINT('Ctrl Pts',(-46.0202159909161,-8.14030790141739,
0.));
#77626=CARTESIAN_POINT('Ctrl Pts',(-46.0202159909161,-8.14030790141739,
20.));
#77627=CARTESIAN_POINT('Ctrl Pts',(-46.0230005571558,-8.107421820069,0.));
#77628=CARTESIAN_POINT('Ctrl Pts',(-46.0230005571558,-8.107421820069,20.));
#77629=CARTESIAN_POINT('Ctrl Pts',(-46.025761898743,-8.07453490085736,0.));
#77630=CARTESIAN_POINT('Ctrl Pts',(-46.025761898743,-8.07453490085736,20.));
#77631=CARTESIAN_POINT('Ctrl Pts',(-46.0285000151874,-8.04164716012545,
0.));
#77632=CARTESIAN_POINT('Ctrl Pts',(-46.0285000151874,-8.04164716012545,
20.));
#77633=CARTESIAN_POINT('Ctrl Pts',(-46.0312149060105,-8.00875861421695,
0.));
#77634=CARTESIAN_POINT('Ctrl Pts',(-46.0312149060105,-8.00875861421695,
20.));
#77635=CARTESIAN_POINT('Ctrl Pts',(-46.0339065707442,-7.9758692794762,0.));
#77636=CARTESIAN_POINT('Ctrl Pts',(-46.0339065707442,-7.9758692794762,20.));
#77637=CARTESIAN_POINT('Ctrl Pts',(-46.0365750089318,-7.94297917224815,
0.));
#77638=CARTESIAN_POINT('Ctrl Pts',(-46.0365750089318,-7.94297917224815,
20.));
#77639=CARTESIAN_POINT('Ctrl Pts',(-46.0392202201279,-7.91008830887855,
0.));
#77640=CARTESIAN_POINT('Ctrl Pts',(-46.0392202201279,-7.91008830887855,
20.));
#77641=CARTESIAN_POINT('Ctrl Pts',(-46.0418422038989,-7.877196705714,0.));
#77642=CARTESIAN_POINT('Ctrl Pts',(-46.0418422038989,-7.877196705714,20.));
#77643=CARTESIAN_POINT('Ctrl Pts',(-46.0444409598224,-7.84430437910167,
0.));
#77644=CARTESIAN_POINT('Ctrl Pts',(-46.0444409598224,-7.84430437910167,
20.));
#77645=CARTESIAN_POINT('Ctrl Pts',(-46.0470164874882,-7.81141134538954,
0.));
#77646=CARTESIAN_POINT('Ctrl Pts',(-46.0470164874882,-7.81141134538954,
20.));
#77647=CARTESIAN_POINT('Ctrl Pts',(-46.0495687864972,-7.77851762092636,
0.));
#77648=CARTESIAN_POINT('Ctrl Pts',(-46.0495687864972,-7.77851762092636,
20.));
#77649=CARTESIAN_POINT('Ctrl Pts',(-46.052097856463,-7.74562322206167,0.));
#77650=CARTESIAN_POINT('Ctrl Pts',(-46.052097856463,-7.74562322206167,20.));
#77651=CARTESIAN_POINT('Ctrl Pts',(-46.0546036970108,-7.71272816514571,
0.));
#77652=CARTESIAN_POINT('Ctrl Pts',(-46.0546036970108,-7.71272816514571,
20.));
#77653=CARTESIAN_POINT('Ctrl Pts',(-46.0570863077758,-7.67983246652917,
0.));
#77654=CARTESIAN_POINT('Ctrl Pts',(-46.0570863077758,-7.67983246652917,
20.));
#77655=CARTESIAN_POINT('Ctrl Pts',(-46.0595456884042,-7.64693614256335,
0.));
#77656=CARTESIAN_POINT('Ctrl Pts',(-46.0595456884042,-7.64693614256335,
20.));
#77657=CARTESIAN_POINT('Ctrl Pts',(-46.0619818385541,-7.61403920960035,
0.));
#77658=CARTESIAN_POINT('Ctrl Pts',(-46.0619818385541,-7.61403920960035,
20.));
#77659=CARTESIAN_POINT('Ctrl Pts',(-46.0643947578955,-7.58114168399302,
0.));
#77660=CARTESIAN_POINT('Ctrl Pts',(-46.0643947578955,-7.58114168399302,
20.));
#77661=CARTESIAN_POINT('Ctrl Pts',(-46.0667844461104,-7.54824358209484,
0.));
#77662=CARTESIAN_POINT('Ctrl Pts',(-46.0667844461104,-7.54824358209484,
20.));
#77663=CARTESIAN_POINT('Ctrl Pts',(-46.0691509028928,-7.51534492025983,
0.));
#77664=CARTESIAN_POINT('Ctrl Pts',(-46.0691509028928,-7.51534492025983,
20.));
#77665=CARTESIAN_POINT('Ctrl Pts',(-46.0714941279471,-7.4824457148425,0.));
#77666=CARTESIAN_POINT('Ctrl Pts',(-46.0714941279471,-7.4824457148425,20.));
#77667=CARTESIAN_POINT('Ctrl Pts',(-46.0738141209885,-7.44954598219809,
0.));
#77668=CARTESIAN_POINT('Ctrl Pts',(-46.0738141209885,-7.44954598219809,
20.));
#77669=CARTESIAN_POINT('Ctrl Pts',(-46.0761108817447,-7.4166457386826,0.));
#77670=CARTESIAN_POINT('Ctrl Pts',(-46.0761108817447,-7.4166457386826,20.));
#77671=CARTESIAN_POINT('Ctrl Pts',(-46.0783844099553,-7.38374500065294,
0.));
#77672=CARTESIAN_POINT('Ctrl Pts',(-46.0783844099553,-7.38374500065294,
20.));
#77673=CARTESIAN_POINT('Ctrl Pts',(-46.0806347053718,-7.35084378446661,
0.));
#77674=CARTESIAN_POINT('Ctrl Pts',(-46.0806347053718,-7.35084378446661,
20.));
#77675=CARTESIAN_POINT('Ctrl Pts',(-46.0828617677561,-7.31794210648139,
0.));
#77676=CARTESIAN_POINT('Ctrl Pts',(-46.0828617677561,-7.31794210648139,
20.));
#77677=CARTESIAN_POINT('Ctrl Pts',(-46.0850655968817,-7.2850399830555,0.));
#77678=CARTESIAN_POINT('Ctrl Pts',(-46.0850655968817,-7.2850399830555,20.));
#77679=CARTESIAN_POINT('Ctrl Pts',(-46.0872461925336,-7.25213743054749,
0.));
#77680=CARTESIAN_POINT('Ctrl Pts',(-46.0872461925336,-7.25213743054749,
20.));
#77681=CARTESIAN_POINT('Ctrl Pts',(-46.0894035545083,-7.2192344653164,0.));
#77682=CARTESIAN_POINT('Ctrl Pts',(-46.0894035545083,-7.2192344653164,20.));
#77683=CARTESIAN_POINT('Ctrl Pts',(-46.0915376826137,-7.18633110372211,
0.));
#77684=CARTESIAN_POINT('Ctrl Pts',(-46.0915376826137,-7.18633110372211,
20.));
#77685=CARTESIAN_POINT('Ctrl Pts',(-46.0936485766695,-7.15342736212529,
0.));
#77686=CARTESIAN_POINT('Ctrl Pts',(-46.0936485766695,-7.15342736212529,
20.));
#77687=CARTESIAN_POINT('Ctrl Pts',(-46.0957362365075,-7.12052325688752,
0.));
#77688=CARTESIAN_POINT('Ctrl Pts',(-46.0957362365075,-7.12052325688752,
20.));
#77689=CARTESIAN_POINT('Ctrl Pts',(-46.097800661971,-7.08761880437093,0.));
#77690=CARTESIAN_POINT('Ctrl Pts',(-46.097800661971,-7.08761880437093,20.));
#77691=CARTESIAN_POINT('Ctrl Pts',(-46.0998418529147,-7.05471402093801,
0.));
#77692=CARTESIAN_POINT('Ctrl Pts',(-46.0998418529147,-7.05471402093801,
20.));
#77693=CARTESIAN_POINT('Ctrl Pts',(-46.1018598092046,-7.02180892295147,
0.));
#77694=CARTESIAN_POINT('Ctrl Pts',(-46.1018598092046,-7.02180892295147,
20.));
#77695=CARTESIAN_POINT('Ctrl Pts',(-46.103854530718,-6.98890352677438,0.));
#77696=CARTESIAN_POINT('Ctrl Pts',(-46.103854530718,-6.98890352677438,20.));
#77697=CARTESIAN_POINT('Ctrl Pts',(-46.1058260173429,-6.95599784877019,
0.));
#77698=CARTESIAN_POINT('Ctrl Pts',(-46.1058260173429,-6.95599784877019,
20.));
#77699=CARTESIAN_POINT('Ctrl Pts',(-46.1077742689797,-6.92309190530285,
0.));
#77700=CARTESIAN_POINT('Ctrl Pts',(-46.1077742689797,-6.92309190530285,
20.));
#77701=CARTESIAN_POINT('Ctrl Pts',(-46.1096992855399,-6.89018571273689,
0.));
#77702=CARTESIAN_POINT('Ctrl Pts',(-46.1096992855399,-6.89018571273689,
20.));
#77703=CARTESIAN_POINT('Ctrl Pts',(-46.111601066948,-6.85727928743787,0.));
#77704=CARTESIAN_POINT('Ctrl Pts',(-46.111601066948,-6.85727928743787,20.));
#77705=CARTESIAN_POINT('Ctrl Pts',(-46.1134796131392,-6.82437264577169,
0.));
#77706=CARTESIAN_POINT('Ctrl Pts',(-46.1134796131392,-6.82437264577169,
20.));
#77707=CARTESIAN_POINT('Ctrl Pts',(-46.1153349240611,-6.7914658041047,0.));
#77708=CARTESIAN_POINT('Ctrl Pts',(-46.1153349240611,-6.7914658041047,20.));
#77709=CARTESIAN_POINT('Ctrl Pts',(-46.1171669996709,-6.75855877880356,
0.));
#77710=CARTESIAN_POINT('Ctrl Pts',(-46.1171669996709,-6.75855877880356,
20.));
#77711=CARTESIAN_POINT('Ctrl Pts',(-46.1189758399374,-6.7256515862352,0.));
#77712=CARTESIAN_POINT('Ctrl Pts',(-46.1189758399374,-6.7256515862352,20.));
#77713=CARTESIAN_POINT('Ctrl Pts',(-46.1207614448407,-6.69274424276687,
0.));
#77714=CARTESIAN_POINT('Ctrl Pts',(-46.1207614448407,-6.69274424276687,
20.));
#77715=CARTESIAN_POINT('Ctrl Pts',(-46.122523814374,-6.65983676476652,0.));
#77716=CARTESIAN_POINT('Ctrl Pts',(-46.122523814374,-6.65983676476652,20.));
#77717=CARTESIAN_POINT('Ctrl Pts',(-46.124262948542,-6.62692916860257,0.));
#77718=CARTESIAN_POINT('Ctrl Pts',(-46.124262948542,-6.62692916860257,20.));
#77719=CARTESIAN_POINT('Ctrl Pts',(-46.1259788473615,-6.59402147064399,
0.));
#77720=CARTESIAN_POINT('Ctrl Pts',(-46.1259788473615,-6.59402147064399,
20.));
#77721=CARTESIAN_POINT('Ctrl Pts',(-46.1276715108604,-6.56111368726009,
0.));
#77722=CARTESIAN_POINT('Ctrl Pts',(-46.1276715108604,-6.56111368726009,
20.));
#77723=CARTESIAN_POINT('Ctrl Pts',(-46.1293409390781,-6.52820583482049,
0.));
#77724=CARTESIAN_POINT('Ctrl Pts',(-46.1293409390781,-6.52820583482049,
20.));
#77725=CARTESIAN_POINT('Ctrl Pts',(-46.1309871320644,-6.49529792969508,
0.));
#77726=CARTESIAN_POINT('Ctrl Pts',(-46.1309871320644,-6.49529792969508,
20.));
#77727=CARTESIAN_POINT('Ctrl Pts',(-46.1326100898806,-6.46238998825407,
0.));
#77728=CARTESIAN_POINT('Ctrl Pts',(-46.1326100898806,-6.46238998825407,
20.));
#77729=CARTESIAN_POINT('Ctrl Pts',(-46.1342098125991,-6.42948202686813,
0.));
#77730=CARTESIAN_POINT('Ctrl Pts',(-46.1342098125991,-6.42948202686813,
20.));
#77731=CARTESIAN_POINT('Ctrl Pts',(-46.1357863003044,-6.39657406190844,
0.));
#77732=CARTESIAN_POINT('Ctrl Pts',(-46.1357863003044,-6.39657406190844,
20.));
#77733=CARTESIAN_POINT('Ctrl Pts',(-46.1373395530931,-6.36366610974647,
0.));
#77734=CARTESIAN_POINT('Ctrl Pts',(-46.1373395530931,-6.36366610974647,
20.));
#77735=CARTESIAN_POINT('Ctrl Pts',(-46.138869571074,-6.33075818675419,0.));
#77736=CARTESIAN_POINT('Ctrl Pts',(-46.138869571074,-6.33075818675419,20.));
#77737=CARTESIAN_POINT('Ctrl Pts',(-46.1403763543673,-6.29785030930381,
0.));
#77738=CARTESIAN_POINT('Ctrl Pts',(-46.1403763543673,-6.29785030930381,
20.));
#77739=CARTESIAN_POINT('Ctrl Pts',(-46.141859903105,-6.26494249376777,0.));
#77740=CARTESIAN_POINT('Ctrl Pts',(-46.141859903105,-6.26494249376777,20.));
#77741=CARTESIAN_POINT('Ctrl Pts',(-46.1433202174297,-6.23203475651882,
0.));
#77742=CARTESIAN_POINT('Ctrl Pts',(-46.1433202174297,-6.23203475651882,
20.));
#77743=CARTESIAN_POINT('Ctrl Pts',(-46.1447572974959,-6.19912711393004,
0.));
#77744=CARTESIAN_POINT('Ctrl Pts',(-46.1447572974959,-6.19912711393004,
20.));
#77745=CARTESIAN_POINT('Ctrl Pts',(-46.1461711434687,-6.16621958237487,
0.));
#77746=CARTESIAN_POINT('Ctrl Pts',(-46.1461711434687,-6.16621958237487,
20.));
#77747=CARTESIAN_POINT('Ctrl Pts',(-46.1475617555249,-6.1333121782271,0.));
#77748=CARTESIAN_POINT('Ctrl Pts',(-46.1475617555249,-6.1333121782271,20.));
#77749=CARTESIAN_POINT('Ctrl Pts',(-46.1489291338532,-6.10040491786085,
0.));
#77750=CARTESIAN_POINT('Ctrl Pts',(-46.1489291338532,-6.10040491786085,
20.));
#77751=CARTESIAN_POINT('Ctrl Pts',(-46.1502732786543,-6.06749781765058,
0.));
#77752=CARTESIAN_POINT('Ctrl Pts',(-46.1502732786543,-6.06749781765058,
20.));
#77753=CARTESIAN_POINT('Ctrl Pts',(-46.151594190141,-6.03459089397104,0.));
#77754=CARTESIAN_POINT('Ctrl Pts',(-46.151594190141,-6.03459089397104,20.));
#77755=CARTESIAN_POINT('Ctrl Pts',(-46.1528918685373,-6.0016841631972,0.));
#77756=CARTESIAN_POINT('Ctrl Pts',(-46.1528918685373,-6.0016841631972,20.));
#77757=CARTESIAN_POINT('Ctrl Pts',(-46.1541663140783,-5.96877764170411,
0.));
#77758=CARTESIAN_POINT('Ctrl Pts',(-46.1541663140783,-5.96877764170411,
20.));
#77759=CARTESIAN_POINT('Ctrl Pts',(-46.1554175270101,-5.93587134586689,
0.));
#77760=CARTESIAN_POINT('Ctrl Pts',(-46.1554175270101,-5.93587134586689,
20.));
#77761=CARTESIAN_POINT('Ctrl Pts',(-46.1566455075904,-5.90296529206097,
0.));
#77762=CARTESIAN_POINT('Ctrl Pts',(-46.1566455075904,-5.90296529206097,
20.));
#77763=CARTESIAN_POINT('Ctrl Pts',(-46.1578502560886,-5.87005949666211,
0.));
#77764=CARTESIAN_POINT('Ctrl Pts',(-46.1578502560886,-5.87005949666211,
20.));
#77765=CARTESIAN_POINT('Ctrl Pts',(-46.1590317727861,-5.83715397604653,
0.));
#77766=CARTESIAN_POINT('Ctrl Pts',(-46.1590317727861,-5.83715397604653,
20.));
#77767=CARTESIAN_POINT('Ctrl Pts',(-46.160190057976,-5.80424874659071,0.));
#77768=CARTESIAN_POINT('Ctrl Pts',(-46.160190057976,-5.80424874659071,20.));
#77769=CARTESIAN_POINT('Ctrl Pts',(-46.1613251119636,-5.77134382467172,
0.));
#77770=CARTESIAN_POINT('Ctrl Pts',(-46.1613251119636,-5.77134382467172,
20.));
#77771=CARTESIAN_POINT('Ctrl Pts',(-46.1624369350662,-5.73843922666647,
0.));
#77772=CARTESIAN_POINT('Ctrl Pts',(-46.1624369350662,-5.73843922666647,
20.));
#77773=CARTESIAN_POINT('Ctrl Pts',(-46.1635255276116,-5.70553496895184,
0.));
#77774=CARTESIAN_POINT('Ctrl Pts',(-46.1635255276116,-5.70553496895184,
20.));
#77775=CARTESIAN_POINT('Ctrl Pts',(-46.1645908899393,-5.67263106790478,
0.));
#77776=CARTESIAN_POINT('Ctrl Pts',(-46.1645908899393,-5.67263106790478,
20.));
#77777=CARTESIAN_POINT('Ctrl Pts',(-46.1656330223979,-5.63972753990235,
0.));
#77778=CARTESIAN_POINT('Ctrl Pts',(-46.1656330223979,-5.63972753990235,
20.));
#77779=CARTESIAN_POINT('Ctrl Pts',(-46.166651925349,-5.60682440132181,0.));
#77780=CARTESIAN_POINT('Ctrl Pts',(-46.166651925349,-5.60682440132181,20.));
#77781=CARTESIAN_POINT('Ctrl Pts',(-46.1676475991657,-5.57392166854074,
0.));
#77782=CARTESIAN_POINT('Ctrl Pts',(-46.1676475991657,-5.57392166854074,
20.));
#77783=CARTESIAN_POINT('Ctrl Pts',(-46.1686200442337,-5.54101935793709,
0.));
#77784=CARTESIAN_POINT('Ctrl Pts',(-46.1686200442337,-5.54101935793709,
20.));
#77785=CARTESIAN_POINT('Ctrl Pts',(-46.1695692609505,-5.50811748588893,
0.));
#77786=CARTESIAN_POINT('Ctrl Pts',(-46.1695692609505,-5.50811748588893,
20.));
#77787=CARTESIAN_POINT('Ctrl Pts',(-46.170495249726,-5.47521606877459,0.));
#77788=CARTESIAN_POINT('Ctrl Pts',(-46.170495249726,-5.47521606877459,20.));
#77789=CARTESIAN_POINT('Ctrl Pts',(-46.1713980109807,-5.44231512297238,
0.));
#77790=CARTESIAN_POINT('Ctrl Pts',(-46.1713980109807,-5.44231512297238,
20.));
#77791=CARTESIAN_POINT('Ctrl Pts',(-46.1722775451467,-5.40941466486069,
0.));
#77792=CARTESIAN_POINT('Ctrl Pts',(-46.1722775451467,-5.40941466486069,
20.));
#77793=CARTESIAN_POINT('Ctrl Pts',(-46.1731338526667,-5.37651471081787,
0.));
#77794=CARTESIAN_POINT('Ctrl Pts',(-46.1731338526667,-5.37651471081787,
20.));
#77795=CARTESIAN_POINT('Ctrl Pts',(-46.1739669339953,-5.34361527722239,
0.));
#77796=CARTESIAN_POINT('Ctrl Pts',(-46.1739669339953,-5.34361527722239,
20.));
#77797=CARTESIAN_POINT('Ctrl Pts',(-46.1747767895978,-5.31071638045279,
0.));
#77798=CARTESIAN_POINT('Ctrl Pts',(-46.1747767895978,-5.31071638045279,
20.));
#77799=CARTESIAN_POINT('Ctrl Pts',(-46.1755634199519,-5.2778180368879,0.));
#77800=CARTESIAN_POINT('Ctrl Pts',(-46.1755634199519,-5.2778180368879,20.));
#77801=CARTESIAN_POINT('Ctrl Pts',(-46.1763268255471,-5.24492026290662,
0.));
#77802=CARTESIAN_POINT('Ctrl Pts',(-46.1763268255471,-5.24492026290662,
20.));
#77803=CARTESIAN_POINT('Ctrl Pts',(-46.1770670068854,-5.21202307488801,
0.));
#77804=CARTESIAN_POINT('Ctrl Pts',(-46.1770670068854,-5.21202307488801,
20.));
#77805=CARTESIAN_POINT('Ctrl Pts',(-46.1777839644797,-5.17912648921101,
0.));
#77806=CARTESIAN_POINT('Ctrl Pts',(-46.1777839644797,-5.17912648921101,
20.));
#77807=CARTESIAN_POINT('Ctrl Pts',(-46.1784776988548,-5.14623052225471,
0.));
#77808=CARTESIAN_POINT('Ctrl Pts',(-46.1784776988548,-5.14623052225471,
20.));
#77809=CARTESIAN_POINT('Ctrl Pts',(-46.1791482105459,-5.11333519039808,
0.));
#77810=CARTESIAN_POINT('Ctrl Pts',(-46.1791482105459,-5.11333519039808,
20.));
#77811=CARTESIAN_POINT('Ctrl Pts',(-46.1797955000997,-5.08044051002025,
0.));
#77812=CARTESIAN_POINT('Ctrl Pts',(-46.1797955000997,-5.08044051002025,
20.));
#77813=CARTESIAN_POINT('Ctrl Pts',(-46.1804195680748,-5.0475464975003,0.));
#77814=CARTESIAN_POINT('Ctrl Pts',(-46.1804195680748,-5.0475464975003,20.));
#77815=CARTESIAN_POINT('Ctrl Pts',(-46.1810204150412,-5.01465316921748,
0.));
#77816=CARTESIAN_POINT('Ctrl Pts',(-46.1810204150412,-5.01465316921748,
20.));
#77817=CARTESIAN_POINT('Ctrl Pts',(-46.1815980415817,-4.981760541551,0.));
#77818=CARTESIAN_POINT('Ctrl Pts',(-46.1815980415817,-4.981760541551,20.));
#77819=CARTESIAN_POINT('Ctrl Pts',(-46.182152448291,-4.94886863088032,0.));
#77820=CARTESIAN_POINT('Ctrl Pts',(-46.182152448291,-4.94886863088032,20.));
#77821=CARTESIAN_POINT('Ctrl Pts',(-46.1826836357763,-4.91597745358481,
0.));
#77822=CARTESIAN_POINT('Ctrl Pts',(-46.1826836357763,-4.91597745358481,
20.));
#77823=CARTESIAN_POINT('Ctrl Pts',(-46.1831916046531,-4.88308702604349,
0.));
#77824=CARTESIAN_POINT('Ctrl Pts',(-46.1831916046531,-4.88308702604349,
20.));
#77825=CARTESIAN_POINT('Ctrl Pts',(-46.1836763555496,-4.85019736463543,
0.));
#77826=CARTESIAN_POINT('Ctrl Pts',(-46.1836763555496,-4.85019736463543,
20.));
#77827=CARTESIAN_POINT('Ctrl Pts',(-46.1841378891039,-4.81730848573953,
0.));
#77828=CARTESIAN_POINT('Ctrl Pts',(-46.1841378891039,-4.81730848573953,
20.));
#77829=CARTESIAN_POINT('Ctrl Pts',(-46.1845762059678,-4.78442040573514,
0.));
#77830=CARTESIAN_POINT('Ctrl Pts',(-46.1845762059678,-4.78442040573514,
20.));
#77831=CARTESIAN_POINT('Ctrl Pts',(-46.1849913068043,-4.7515331410016,0.));
#77832=CARTESIAN_POINT('Ctrl Pts',(-46.1849913068043,-4.7515331410016,20.));
#77833=CARTESIAN_POINT('Ctrl Pts',(-46.1853831922891,-4.71864670791826,
0.));
#77834=CARTESIAN_POINT('Ctrl Pts',(-46.1853831922891,-4.71864670791826,
20.));
#77835=CARTESIAN_POINT('Ctrl Pts',(-46.1857518631086,-4.68576112286394,
0.));
#77836=CARTESIAN_POINT('Ctrl Pts',(-46.1857518631086,-4.68576112286394,
20.));
#77837=CARTESIAN_POINT('Ctrl Pts',(-46.1860973199616,-4.65287640221747,
0.));
#77838=CARTESIAN_POINT('Ctrl Pts',(-46.1860973199616,-4.65287640221747,
20.));
#77839=CARTESIAN_POINT('Ctrl Pts',(-46.1864195635571,-4.6199925623574,0.));
#77840=CARTESIAN_POINT('Ctrl Pts',(-46.1864195635571,-4.6199925623574,20.));
#77841=CARTESIAN_POINT('Ctrl Pts',(-46.1867185946155,-4.58710961966232,
0.));
#77842=CARTESIAN_POINT('Ctrl Pts',(-46.1867185946155,-4.58710961966232,
20.));
#77843=CARTESIAN_POINT('Ctrl Pts',(-46.1869944138693,-4.55422759051101,
0.));
#77844=CARTESIAN_POINT('Ctrl Pts',(-46.1869944138693,-4.55422759051101,
20.));
#77845=CARTESIAN_POINT('Ctrl Pts',(-46.1872470220627,-4.52134649128217,
0.));
#77846=CARTESIAN_POINT('Ctrl Pts',(-46.1872470220627,-4.52134649128217,
20.));
#77847=CARTESIAN_POINT('Ctrl Pts',(-46.1874764199521,-4.48846633835459,
0.));
#77848=CARTESIAN_POINT('Ctrl Pts',(-46.1874764199521,-4.48846633835459,
20.));
#77849=CARTESIAN_POINT('Ctrl Pts',(-46.1876826083051,-4.4555871481068,0.));
#77850=CARTESIAN_POINT('Ctrl Pts',(-46.1876826083051,-4.4555871481068,20.));
#77851=CARTESIAN_POINT('Ctrl Pts',(-46.1878655879008,-4.42270893691723,
0.));
#77852=CARTESIAN_POINT('Ctrl Pts',(-46.1878655879008,-4.42270893691723,
20.));
#77853=CARTESIAN_POINT('Ctrl Pts',(-46.1880253595297,-4.38983172116389,
0.));
#77854=CARTESIAN_POINT('Ctrl Pts',(-46.1880253595297,-4.38983172116389,
20.));
#77855=CARTESIAN_POINT('Ctrl Pts',(-46.1881619239926,-4.35695551722447,
0.));
#77856=CARTESIAN_POINT('Ctrl Pts',(-46.1881619239926,-4.35695551722447,
20.));
#77857=CARTESIAN_POINT('Ctrl Pts',(-46.1882752821036,-4.32408034147654,
0.));
#77858=CARTESIAN_POINT('Ctrl Pts',(-46.1882752821036,-4.32408034147654,
20.));
#77859=CARTESIAN_POINT('Ctrl Pts',(-46.1883654346888,-4.29120621029776,
0.));
#77860=CARTESIAN_POINT('Ctrl Pts',(-46.1883654346888,-4.29120621029776,
20.));
#77861=CARTESIAN_POINT('Ctrl Pts',(-46.1884323825857,-4.25833314006578,
0.));
#77862=CARTESIAN_POINT('Ctrl Pts',(-46.1884323825857,-4.25833314006578,
20.));
#77863=CARTESIAN_POINT('Ctrl Pts',(-46.1884761266433,-4.22546114715825,
0.));
#77864=CARTESIAN_POINT('Ctrl Pts',(-46.1884761266433,-4.22546114715825,
20.));
#77865=CARTESIAN_POINT('Ctrl Pts',(-46.1884966677209,-4.19259024795238,
0.));
#77866=CARTESIAN_POINT('Ctrl Pts',(-46.1884966677209,-4.19259024795238,
20.));
#77867=CARTESIAN_POINT('Ctrl Pts',(-46.1884940066895,-4.15972045882508,
0.));
#77868=CARTESIAN_POINT('Ctrl Pts',(-46.1884940066895,-4.15972045882508,
20.));
#77869=CARTESIAN_POINT('Ctrl Pts',(-46.1884681444317,-4.12685179615294,
0.));
#77870=CARTESIAN_POINT('Ctrl Pts',(-46.1884681444317,-4.12685179615294,
20.));
#77871=CARTESIAN_POINT('Ctrl Pts',(-46.188419081843,-4.09398427631254,0.));
#77872=CARTESIAN_POINT('Ctrl Pts',(-46.188419081843,-4.09398427631254,20.));
#77873=CARTESIAN_POINT('Ctrl Pts',(-46.18834681983,-4.06111791568023,0.));
#77874=CARTESIAN_POINT('Ctrl Pts',(-46.18834681983,-4.06111791568023,20.));
#77875=CARTESIAN_POINT('Ctrl Pts',(-46.1882513593113,-4.02825273063217,
0.));
#77876=CARTESIAN_POINT('Ctrl Pts',(-46.1882513593113,-4.02825273063217,
20.));
#77877=CARTESIAN_POINT('Ctrl Pts',(-46.1881327012171,-3.99538873754442,
0.));
#77878=CARTESIAN_POINT('Ctrl Pts',(-46.1881327012171,-3.99538873754442,
20.));
#77879=CARTESIAN_POINT('Ctrl Pts',(-46.1879908464881,-3.96252595279274,
0.));
#77880=CARTESIAN_POINT('Ctrl Pts',(-46.1879908464881,-3.96252595279274,
20.));
#77881=CARTESIAN_POINT('Ctrl Pts',(-46.1878257960766,-3.92966439275257,
0.));
#77882=CARTESIAN_POINT('Ctrl Pts',(-46.1878257960766,-3.92966439275257,
20.));
#77883=CARTESIAN_POINT('Ctrl Pts',(-46.1876375509469,-3.89680407379914,
0.));
#77884=CARTESIAN_POINT('Ctrl Pts',(-46.1876375509469,-3.89680407379914,
20.));
#77885=CARTESIAN_POINT('Ctrl Pts',(-46.1874261120751,-3.86394501230744,
0.));
#77886=CARTESIAN_POINT('Ctrl Pts',(-46.1874261120751,-3.86394501230744,
20.));
#77887=CARTESIAN_POINT('Ctrl Pts',(-46.1871914804492,-3.83108722465198,
0.));
#77888=CARTESIAN_POINT('Ctrl Pts',(-46.1871914804492,-3.83108722465198,
20.));
#77889=CARTESIAN_POINT('Ctrl Pts',(-46.1869336570686,-3.79823072720685,
0.));
#77890=CARTESIAN_POINT('Ctrl Pts',(-46.1869336570686,-3.79823072720685,
20.));
#77891=CARTESIAN_POINT('Ctrl Pts',(-46.1866526429445,-3.76537553634595,
0.));
#77892=CARTESIAN_POINT('Ctrl Pts',(-46.1866526429445,-3.76537553634595,
20.));
#77893=CARTESIAN_POINT('Ctrl Pts',(-46.1863484390996,-3.73252166844327,
0.));
#77894=CARTESIAN_POINT('Ctrl Pts',(-46.1863484390996,-3.73252166844327,
20.));
#77895=CARTESIAN_POINT('Ctrl Pts',(-46.1860210465678,-3.69966913987252,
0.));
#77896=CARTESIAN_POINT('Ctrl Pts',(-46.1860210465678,-3.69966913987252,
20.));
#77897=CARTESIAN_POINT('Ctrl Pts',(-46.185670466394,-3.66681796700709,0.));
#77898=CARTESIAN_POINT('Ctrl Pts',(-46.185670466394,-3.66681796700709,20.));
#77899=CARTESIAN_POINT('Ctrl Pts',(-46.1852966996347,-3.63396816621989,
0.));
#77900=CARTESIAN_POINT('Ctrl Pts',(-46.1852966996347,-3.63396816621989,
20.));
#77901=CARTESIAN_POINT('Ctrl Pts',(-46.1848997473582,-3.60111975388338,
0.));
#77902=CARTESIAN_POINT('Ctrl Pts',(-46.1848997473582,-3.60111975388338,
20.));
#77903=CARTESIAN_POINT('Ctrl Pts',(-46.1844796106451,-3.56827274636958,
0.));
#77904=CARTESIAN_POINT('Ctrl Pts',(-46.1844796106451,-3.56827274636958,
20.));
#77905=CARTESIAN_POINT('Ctrl Pts',(-46.1840362905882,-3.53542716005024,
0.));
#77906=CARTESIAN_POINT('Ctrl Pts',(-46.1840362905882,-3.53542716005024,
20.));
#77907=CARTESIAN_POINT('Ctrl Pts',(-46.1835697882921,-3.50258301129688,
0.));
#77908=CARTESIAN_POINT('Ctrl Pts',(-46.1835697882921,-3.50258301129688,
20.));
#77909=CARTESIAN_POINT('Ctrl Pts',(-46.1830801048722,-3.4697403164807,0.));
#77910=CARTESIAN_POINT('Ctrl Pts',(-46.1830801048722,-3.4697403164807,20.));
#77911=CARTESIAN_POINT('Ctrl Pts',(-46.1825672414553,-3.43689909197262,
0.));
#77912=CARTESIAN_POINT('Ctrl Pts',(-46.1825672414553,-3.43689909197262,
20.));
#77913=CARTESIAN_POINT('Ctrl Pts',(-46.1820311991793,-3.40405935414302,
0.));
#77914=CARTESIAN_POINT('Ctrl Pts',(-46.1820311991793,-3.40405935414302,
20.));
#77915=CARTESIAN_POINT('Ctrl Pts',(-46.1814719791936,-3.37122111936182,
0.));
#77916=CARTESIAN_POINT('Ctrl Pts',(-46.1814719791936,-3.37122111936182,
20.));
#77917=CARTESIAN_POINT('Ctrl Pts',(-46.1808895826591,-3.33838440399861,
0.));
#77918=CARTESIAN_POINT('Ctrl Pts',(-46.1808895826591,-3.33838440399861,
20.));
#77919=CARTESIAN_POINT('Ctrl Pts',(-46.1802840107495,-3.30554922442265,
0.));
#77920=CARTESIAN_POINT('Ctrl Pts',(-46.1802840107495,-3.30554922442265,
20.));
#77921=CARTESIAN_POINT('Ctrl Pts',(-46.1796552646498,-3.27271559700278,
0.));
#77922=CARTESIAN_POINT('Ctrl Pts',(-46.1796552646498,-3.27271559700278,
20.));
#77923=CARTESIAN_POINT('Ctrl Pts',(-46.1790033455572,-3.23988353810748,
0.));
#77924=CARTESIAN_POINT('Ctrl Pts',(-46.1790033455572,-3.23988353810748,
20.));
#77925=CARTESIAN_POINT('Ctrl Pts',(-46.1783282546796,-3.2070530641047,0.));
#77926=CARTESIAN_POINT('Ctrl Pts',(-46.1783282546796,-3.2070530641047,20.));
#77927=CARTESIAN_POINT('Ctrl Pts',(-46.1776299932363,-3.17422419136187,
0.));
#77928=CARTESIAN_POINT('Ctrl Pts',(-46.1776299932363,-3.17422419136187,
20.));
#77929=CARTESIAN_POINT('Ctrl Pts',(-46.1769085624582,-3.14139693624604,
0.));
#77930=CARTESIAN_POINT('Ctrl Pts',(-46.1769085624582,-3.14139693624604,
20.));
#77931=CARTESIAN_POINT('Ctrl Pts',(-46.1761639635878,-3.10857131512384,
0.));
#77932=CARTESIAN_POINT('Ctrl Pts',(-46.1761639635878,-3.10857131512384,
20.));
#77933=CARTESIAN_POINT('Ctrl Pts',(-46.1753961978798,-3.07574734436159,
0.));
#77934=CARTESIAN_POINT('Ctrl Pts',(-46.1753961978798,-3.07574734436159,
20.));
#77935=CARTESIAN_POINT('Ctrl Pts',(-46.1746052665999,-3.04292504032496,
0.));
#77936=CARTESIAN_POINT('Ctrl Pts',(-46.1746052665999,-3.04292504032496,
20.));
#77937=CARTESIAN_POINT('Ctrl Pts',(-46.1737911710261,-3.01010441937912,
0.));
#77938=CARTESIAN_POINT('Ctrl Pts',(-46.1737911710261,-3.01010441937912,
20.));
#77939=CARTESIAN_POINT('Ctrl Pts',(-46.1729539124487,-2.97728549788889,
0.));
#77940=CARTESIAN_POINT('Ctrl Pts',(-46.1729539124487,-2.97728549788889,
20.));
#77941=CARTESIAN_POINT('Ctrl Pts',(-46.172093492169,-2.94446829221864,0.));
#77942=CARTESIAN_POINT('Ctrl Pts',(-46.172093492169,-2.94446829221864,20.));
#77943=CARTESIAN_POINT('Ctrl Pts',(-46.1712099114993,-2.91165281873224,
0.));
#77944=CARTESIAN_POINT('Ctrl Pts',(-46.1712099114993,-2.91165281873224,
20.));
#77945=CARTESIAN_POINT('Ctrl Pts',(-46.1703031717627,-2.87883909379286,
0.));
#77946=CARTESIAN_POINT('Ctrl Pts',(-46.1703031717627,-2.87883909379286,
20.));
#77947=CARTESIAN_POINT('Ctrl Pts',(-46.169373274294,-2.84602713376308,0.));
#77948=CARTESIAN_POINT('Ctrl Pts',(-46.169373274294,-2.84602713376308,20.));
#77949=CARTESIAN_POINT('Ctrl Pts',(-46.1684202204402,-2.81321695500491,
0.));
#77950=CARTESIAN_POINT('Ctrl Pts',(-46.1684202204402,-2.81321695500491,
20.));
#77951=CARTESIAN_POINT('Ctrl Pts',(-46.1674440115603,-2.78040857388008,
0.));
#77952=CARTESIAN_POINT('Ctrl Pts',(-46.1674440115603,-2.78040857388008,
20.));
#77953=CARTESIAN_POINT('Ctrl Pts',(-46.1664446490252,-2.74760200674979,
0.));
#77954=CARTESIAN_POINT('Ctrl Pts',(-46.1664446490252,-2.74760200674979,
20.));
#77955=CARTESIAN_POINT('Ctrl Pts',(-46.1654221342175,-2.71479726997479,
0.));
#77956=CARTESIAN_POINT('Ctrl Pts',(-46.1654221342175,-2.71479726997479,
20.));
#77957=CARTESIAN_POINT('Ctrl Pts',(-46.1643764685316,-2.68199437991523,
0.));
#77958=CARTESIAN_POINT('Ctrl Pts',(-46.1643764685316,-2.68199437991523,
20.));
#77959=CARTESIAN_POINT('Ctrl Pts',(-46.163307653373,-2.64919335293067,0.));
#77960=CARTESIAN_POINT('Ctrl Pts',(-46.163307653373,-2.64919335293067,20.));
#77961=CARTESIAN_POINT('Ctrl Pts',(-46.1622156901587,-2.61639420537994,
0.));
#77962=CARTESIAN_POINT('Ctrl Pts',(-46.1622156901587,-2.61639420537994,
20.));
#77963=CARTESIAN_POINT('Ctrl Pts',(-46.1611005803162,-2.58359695362107,
0.));
#77964=CARTESIAN_POINT('Ctrl Pts',(-46.1611005803162,-2.58359695362107,
20.));
#77965=CARTESIAN_POINT('Ctrl Pts',(-46.1599623252856,-2.55080161401166,
0.));
#77966=CARTESIAN_POINT('Ctrl Pts',(-46.1599623252856,-2.55080161401166,
20.));
#77967=CARTESIAN_POINT('Ctrl Pts',(-46.1588009265184,-2.51800820290891,
0.));
#77968=CARTESIAN_POINT('Ctrl Pts',(-46.1588009265184,-2.51800820290891,
20.));
#77969=CARTESIAN_POINT('Ctrl Pts',(-46.1576163854777,-2.48521673666957,
0.));
#77970=CARTESIAN_POINT('Ctrl Pts',(-46.1576163854777,-2.48521673666957,
20.));
#77971=CARTESIAN_POINT('Ctrl Pts',(-46.1564087036389,-2.4524272316497,0.));
#77972=CARTESIAN_POINT('Ctrl Pts',(-46.1564087036389,-2.4524272316497,20.));
#77973=CARTESIAN_POINT('Ctrl Pts',(-46.155177882489,-2.41963970420457,0.));
#77974=CARTESIAN_POINT('Ctrl Pts',(-46.155177882489,-2.41963970420457,20.));
#77975=CARTESIAN_POINT('Ctrl Pts',(-46.1539239235264,-2.3868541706887,0.));
#77976=CARTESIAN_POINT('Ctrl Pts',(-46.1539239235264,-2.3868541706887,20.));
#77977=CARTESIAN_POINT('Ctrl Pts',(-46.1526468282604,-2.35407064745589,
0.));
#77978=CARTESIAN_POINT('Ctrl Pts',(-46.1526468282604,-2.35407064745589,
20.));
#77979=CARTESIAN_POINT('Ctrl Pts',(-46.1513465982124,-2.32128915085919,
0.));
#77980=CARTESIAN_POINT('Ctrl Pts',(-46.1513465982124,-2.32128915085919,
20.));
#77981=CARTESIAN_POINT('Ctrl Pts',(-46.1500232349155,-2.28850969725138,
0.));
#77982=CARTESIAN_POINT('Ctrl Pts',(-46.1500232349155,-2.28850969725138,
20.));
#77983=CARTESIAN_POINT('Ctrl Pts',(-46.1486767399146,-2.25573230298458,
0.));
#77984=CARTESIAN_POINT('Ctrl Pts',(-46.1486767399146,-2.25573230298458,
20.));
#77985=CARTESIAN_POINT('Ctrl Pts',(-46.147307114766,-2.22295698441049,0.));
#77986=CARTESIAN_POINT('Ctrl Pts',(-46.147307114766,-2.22295698441049,20.));
#77987=CARTESIAN_POINT('Ctrl Pts',(-46.1459143610377,-2.19018375787986,
0.));
#77988=CARTESIAN_POINT('Ctrl Pts',(-46.1459143610377,-2.19018375787986,
20.));
#77989=CARTESIAN_POINT('Ctrl Pts',(-46.1444984803082,-2.15741263974262,
0.));
#77990=CARTESIAN_POINT('Ctrl Pts',(-46.1444984803082,-2.15741263974262,
20.));
#77991=CARTESIAN_POINT('Ctrl Pts',(-46.1430594741682,-2.12464364634812,
0.));
#77992=CARTESIAN_POINT('Ctrl Pts',(-46.1430594741682,-2.12464364634812,
20.));
#77993=CARTESIAN_POINT('Ctrl Pts',(-46.1415973442202,-2.09187679404497,
0.));
#77994=CARTESIAN_POINT('Ctrl Pts',(-46.1415973442202,-2.09187679404497,
20.));
#77995=CARTESIAN_POINT('Ctrl Pts',(-46.1401120920793,-2.05911209918101,
0.));
#77996=CARTESIAN_POINT('Ctrl Pts',(-46.1401120920793,-2.05911209918101,
20.));
#77997=CARTESIAN_POINT('Ctrl Pts',(-46.1386037193727,-2.02634957810317,
0.));
#77998=CARTESIAN_POINT('Ctrl Pts',(-46.1386037193727,-2.02634957810317,
20.));
#77999=CARTESIAN_POINT('Ctrl Pts',(-46.1370722277379,-1.99358924715753,
0.));
#78000=CARTESIAN_POINT('Ctrl Pts',(-46.1370722277379,-1.99358924715753,
20.));
#78001=CARTESIAN_POINT('Ctrl Pts',(-46.1355176188236,-1.9608311226893,0.));
#78002=CARTESIAN_POINT('Ctrl Pts',(-46.1355176188236,-1.9608311226893,20.));
#78003=CARTESIAN_POINT('Ctrl Pts',(-46.1339398942902,-1.92807522104339,
0.));
#78004=CARTESIAN_POINT('Ctrl Pts',(-46.1339398942902,-1.92807522104339,
20.));
#78005=CARTESIAN_POINT('Ctrl Pts',(-46.1323390558096,-1.89532155856414,
0.));
#78006=CARTESIAN_POINT('Ctrl Pts',(-46.1323390558096,-1.89532155856414,
20.));
#78007=CARTESIAN_POINT('Ctrl Pts',(-46.1307151050651,-1.86257015159582,
0.));
#78008=CARTESIAN_POINT('Ctrl Pts',(-46.1307151050651,-1.86257015159582,
20.));
#78009=CARTESIAN_POINT('Ctrl Pts',(-46.1290680437528,-1.82982101648206,
0.));
#78010=CARTESIAN_POINT('Ctrl Pts',(-46.1290680437528,-1.82982101648206,
20.));
#78011=CARTESIAN_POINT('Ctrl Pts',(-46.1273978735796,-1.79707416956534,
0.));
#78012=CARTESIAN_POINT('Ctrl Pts',(-46.1273978735796,-1.79707416956534,
20.));
#78013=CARTESIAN_POINT('Ctrl Pts',(-46.1257045962649,-1.76432962718685,
0.));
#78014=CARTESIAN_POINT('Ctrl Pts',(-46.1257045962649,-1.76432962718685,
20.));
#78015=CARTESIAN_POINT('Ctrl Pts',(-46.1239882135394,-1.73158740568597,
0.));
#78016=CARTESIAN_POINT('Ctrl Pts',(-46.1239882135394,-1.73158740568597,
20.));
#78017=CARTESIAN_POINT('Ctrl Pts',(-46.1222487271454,-1.69884752140039,
0.));
#78018=CARTESIAN_POINT('Ctrl Pts',(-46.1222487271454,-1.69884752140039,
20.));
#78019=CARTESIAN_POINT('Ctrl Pts',(-46.1204861388364,-1.66610999066655,
0.));
#78020=CARTESIAN_POINT('Ctrl Pts',(-46.1204861388364,-1.66610999066655,
20.));
#78021=CARTESIAN_POINT('Ctrl Pts',(-46.1187004503775,-1.6333748298207,0.));
#78022=CARTESIAN_POINT('Ctrl Pts',(-46.1187004503775,-1.6333748298207,20.));
#78023=CARTESIAN_POINT('Ctrl Pts',(-46.1168916635447,-1.60064205519958,
0.));
#78024=CARTESIAN_POINT('Ctrl Pts',(-46.1168916635447,-1.60064205519958,
20.));
#78025=CARTESIAN_POINT('Ctrl Pts',(-46.1150597801266,-1.56791168314158,
0.));
#78026=CARTESIAN_POINT('Ctrl Pts',(-46.1150597801266,-1.56791168314158,
20.));
#78027=CARTESIAN_POINT('Ctrl Pts',(-46.1132048019234,-1.53518372998667,
0.));
#78028=CARTESIAN_POINT('Ctrl Pts',(-46.1132048019234,-1.53518372998667,
20.));
#78029=CARTESIAN_POINT('Ctrl Pts',(-46.111326730748,-1.5024582120743,0.));
#78030=CARTESIAN_POINT('Ctrl Pts',(-46.111326730748,-1.5024582120743,20.));
#78031=CARTESIAN_POINT('Ctrl Pts',(-46.1094255684237,-1.46973514574143,
0.));
#78032=CARTESIAN_POINT('Ctrl Pts',(-46.1094255684237,-1.46973514574143,
20.));
#78033=CARTESIAN_POINT('Ctrl Pts',(-46.1075013167858,-1.4370145473209,0.));
#78034=CARTESIAN_POINT('Ctrl Pts',(-46.1075013167858,-1.4370145473209,20.));
#78035=CARTESIAN_POINT('Ctrl Pts',(-46.1055539776802,-1.40429643313893,
0.));
#78036=CARTESIAN_POINT('Ctrl Pts',(-46.1055539776802,-1.40429643313893,
20.));
#78037=CARTESIAN_POINT('Ctrl Pts',(-46.1035835529643,-1.37158081951551,
0.));
#78038=CARTESIAN_POINT('Ctrl Pts',(-46.1035835529643,-1.37158081951551,
20.));
#78039=CARTESIAN_POINT('Ctrl Pts',(-46.1015900445065,-1.33886772276919,
0.));
#78040=CARTESIAN_POINT('Ctrl Pts',(-46.1015900445065,-1.33886772276919,
20.));
#78041=CARTESIAN_POINT('Ctrl Pts',(-46.0995734541875,-1.30615715922172,
0.));
#78042=CARTESIAN_POINT('Ctrl Pts',(-46.0995734541875,-1.30615715922172,
20.));
#78043=CARTESIAN_POINT('Ctrl Pts',(-46.0975337839002,-1.27344914520175,
0.));
#78044=CARTESIAN_POINT('Ctrl Pts',(-46.0975337839002,-1.27344914520175,
20.));
#78045=CARTESIAN_POINT('Ctrl Pts',(-46.0954710355506,-1.24074369705072,
0.));
#78046=CARTESIAN_POINT('Ctrl Pts',(-46.0954710355506,-1.24074369705072,
20.));
#78047=CARTESIAN_POINT('Ctrl Pts',(-46.0933852110571,-1.20804083112097,
0.));
#78048=CARTESIAN_POINT('Ctrl Pts',(-46.0933852110571,-1.20804083112097,
20.));
#78049=CARTESIAN_POINT('Ctrl Pts',(-46.0912763123502,-1.17534056376402,
0.));
#78050=CARTESIAN_POINT('Ctrl Pts',(-46.0912763123502,-1.17534056376402,
20.));
#78051=CARTESIAN_POINT('Ctrl Pts',(-46.0891443413718,-1.14264291132052,
0.));
#78052=CARTESIAN_POINT('Ctrl Pts',(-46.0891443413718,-1.14264291132052,
20.));
#78053=CARTESIAN_POINT('Ctrl Pts',(-46.0869893000734,-1.10994789011162,
0.));
#78054=CARTESIAN_POINT('Ctrl Pts',(-46.0869893000734,-1.10994789011162,
20.));
#78055=CARTESIAN_POINT('Ctrl Pts',(-46.0848111904142,-1.07725551642471,
0.));
#78056=CARTESIAN_POINT('Ctrl Pts',(-46.0848111904142,-1.07725551642471,
20.));
#78057=CARTESIAN_POINT('Ctrl Pts',(-46.0826100143611,-1.04456580652047,
0.));
#78058=CARTESIAN_POINT('Ctrl Pts',(-46.0826100143611,-1.04456580652047,
20.));
#78059=CARTESIAN_POINT('Ctrl Pts',(-46.0803857738924,-1.01187877665954,
0.));
#78060=CARTESIAN_POINT('Ctrl Pts',(-46.0803857738924,-1.01187877665954,
20.));
#78061=CARTESIAN_POINT('Ctrl Pts',(-46.0781384710012,-0.979194443126286,
0.));
#78062=CARTESIAN_POINT('Ctrl Pts',(-46.0781384710012,-0.979194443126286,
20.));
#78063=CARTESIAN_POINT('Ctrl Pts',(-46.0758681076973,-0.946512822248744,
0.));
#78064=CARTESIAN_POINT('Ctrl Pts',(-46.0758681076973,-0.946512822248744,
20.));
#78065=CARTESIAN_POINT('Ctrl Pts',(-46.0735746860119,-0.913833930432268,
0.));
#78066=CARTESIAN_POINT('Ctrl Pts',(-46.0735746860119,-0.913833930432268,
20.));
#78067=CARTESIAN_POINT('Ctrl Pts',(-46.0712582079948,-0.881157784136737,
0.));
#78068=CARTESIAN_POINT('Ctrl Pts',(-46.0712582079948,-0.881157784136737,
20.));
#78069=CARTESIAN_POINT('Ctrl Pts',(-46.0689186757066,-0.848484399815181,
0.));
#78070=CARTESIAN_POINT('Ctrl Pts',(-46.0689186757066,-0.848484399815181,
20.));
#78071=CARTESIAN_POINT('Ctrl Pts',(-46.0665560912128,-0.815813793858633,
0.));
#78072=CARTESIAN_POINT('Ctrl Pts',(-46.0665560912128,-0.815813793858633,
20.));
#78073=CARTESIAN_POINT('Ctrl Pts',(-46.064170456577,-0.78314598254893,0.));
#78074=CARTESIAN_POINT('Ctrl Pts',(-46.064170456577,-0.78314598254893,20.));
#78075=CARTESIAN_POINT('Ctrl Pts',(-46.0617617738521,-0.750480981980923,
0.));
#78076=CARTESIAN_POINT('Ctrl Pts',(-46.0617617738521,-0.750480981980923,
20.));
#78077=CARTESIAN_POINT('Ctrl Pts',(-46.0593300450868,-0.717818808129722,
0.));
#78078=CARTESIAN_POINT('Ctrl Pts',(-46.0593300450868,-0.717818808129722,
20.));
#78079=CARTESIAN_POINT('Ctrl Pts',(-46.0568752723439,-0.685159476991759,
0.));
#78080=CARTESIAN_POINT('Ctrl Pts',(-46.0568752723439,-0.685159476991759,
20.));
#78081=CARTESIAN_POINT('Ctrl Pts',(-46.0543974577158,-0.652503004713259,
0.));
#78082=CARTESIAN_POINT('Ctrl Pts',(-46.0543974577158,-0.652503004713259,
20.));
#78083=CARTESIAN_POINT('Ctrl Pts',(-46.0518966033391,-0.619849407700859,
0.));
#78084=CARTESIAN_POINT('Ctrl Pts',(-46.0518966033391,-0.619849407700859,
20.));
#78085=CARTESIAN_POINT('Ctrl Pts',(-46.0493727114182,-0.587198702798619,
0.));
#78086=CARTESIAN_POINT('Ctrl Pts',(-46.0493727114182,-0.587198702798619,
20.));
#78087=CARTESIAN_POINT('Ctrl Pts',(-46.0468257841997,-0.554550907098827,
0.));
#78088=CARTESIAN_POINT('Ctrl Pts',(-46.0468257841997,-0.554550907098827,
20.));
#78089=CARTESIAN_POINT('Ctrl Pts',(-46.044255823933,-0.521906037621043,
0.));
#78090=CARTESIAN_POINT('Ctrl Pts',(-46.044255823933,-0.521906037621043,
20.));
#78091=CARTESIAN_POINT('Ctrl Pts',(-46.0416628328334,-0.489264111013836,
0.));
#78092=CARTESIAN_POINT('Ctrl Pts',(-46.0416628328334,-0.489264111013836,
20.));
#78093=CARTESIAN_POINT('Ctrl Pts',(-46.0390468130479,-0.456625143292611,
0.));
#78094=CARTESIAN_POINT('Ctrl Pts',(-46.0390468130479,-0.456625143292611,
20.));
#78095=CARTESIAN_POINT('Ctrl Pts',(-46.0364077666069,-0.423989149445243,
0.));
#78096=CARTESIAN_POINT('Ctrl Pts',(-46.0364077666069,-0.423989149445243,
20.));
#78097=CARTESIAN_POINT('Ctrl Pts',(-46.0337456954889,-0.391356143937831,
0.));
#78098=CARTESIAN_POINT('Ctrl Pts',(-46.0337456954889,-0.391356143937831,
20.));
#78099=CARTESIAN_POINT('Ctrl Pts',(-46.0310606017089,-0.358726141441568,
0.));
#78100=CARTESIAN_POINT('Ctrl Pts',(-46.0310606017089,-0.358726141441568,
20.));
#78101=CARTESIAN_POINT('Ctrl Pts',(-46.0283524874048,-0.32609915751695,
0.));
#78102=CARTESIAN_POINT('Ctrl Pts',(-46.0283524874048,-0.32609915751695,
20.));
#78103=CARTESIAN_POINT('Ctrl Pts',(-46.025621354915,-0.293475209241787,
0.));
#78104=CARTESIAN_POINT('Ctrl Pts',(-46.025621354915,-0.293475209241787,
20.));
#78105=CARTESIAN_POINT('Ctrl Pts',(-46.022867206884,-0.260854316057531,
0.));
#78106=CARTESIAN_POINT('Ctrl Pts',(-46.022867206884,-0.260854316057531,
20.));
#78107=CARTESIAN_POINT('Ctrl Pts',(-46.0200900461091,-0.228236498538561,
0.));
#78108=CARTESIAN_POINT('Ctrl Pts',(-46.0200900461091,-0.228236498538561,
20.));
#78109=CARTESIAN_POINT('Ctrl Pts',(-46.0172898753497,-0.195621776838879,
0.));
#78110=CARTESIAN_POINT('Ctrl Pts',(-46.0172898753497,-0.195621776838879,
20.));
#78111=CARTESIAN_POINT('Ctrl Pts',(-46.0144666971462,-0.163010169231703,
0.));
#78112=CARTESIAN_POINT('Ctrl Pts',(-46.0144666971462,-0.163010169231703,
20.));
#78113=CARTESIAN_POINT('Ctrl Pts',(-46.0116205136405,-0.130401690656317,
0.));
#78114=CARTESIAN_POINT('Ctrl Pts',(-46.0116205136405,-0.130401690656317,
20.));
#78115=CARTESIAN_POINT('Ctrl Pts',(-46.0087513263814,-0.0977963511372804,
0.));
#78116=CARTESIAN_POINT('Ctrl Pts',(-46.0087513263814,-0.0977963511372804,
20.));
#78117=CARTESIAN_POINT('Ctrl Pts',(-46.0058591364029,-0.0651941566547531,
0.));
#78118=CARTESIAN_POINT('Ctrl Pts',(-46.0058591364029,-0.0651941566547531,
20.));
#78119=CARTESIAN_POINT('Ctrl Pts',(-46.0035269827389,-0.0391149194889384,
0.));
#78120=CARTESIAN_POINT('Ctrl Pts',(-46.0035269827389,-0.0391149194889384,
20.));
#78121=CARTESIAN_POINT('Ctrl Pts',(-46.0017675166781,-0.019556908668581,
0.));
#78122=CARTESIAN_POINT('Ctrl Pts',(-46.0017675166781,-0.019556908668581,
20.));
#78123=CARTESIAN_POINT('Ctrl Pts',(-46.0005899389515,-0.00651886458936213,
0.));
#78124=CARTESIAN_POINT('Ctrl Pts',(-46.0005899389515,-0.00651886458936213,
20.));
#78125=CARTESIAN_POINT('Ctrl Pts',(-46.,6.66133814775094E-15,0.));
#78126=CARTESIAN_POINT('Ctrl Pts',(-46.,6.66133814775094E-15,20.));
#78127=CARTESIAN_POINT('',(-37.5361777128299,-31.4965928746404,2.));
#78128=CARTESIAN_POINT('Ctrl Pts',(-45.2025619355895,-13.7414592977624,
2.));
#78129=CARTESIAN_POINT('Ctrl Pts',(-45.039110381915,-14.5281012519506,2.));
#78130=CARTESIAN_POINT('Ctrl Pts',(-44.8554703046336,-15.3115504167957,
2.));
#78131=CARTESIAN_POINT('Ctrl Pts',(-44.6518239974238,-16.0907854020754,
2.));
#78132=CARTESIAN_POINT('Ctrl Pts',(-44.4484766164816,-16.8688765718406,
2.));
#78133=CARTESIAN_POINT('Ctrl Pts',(-44.2251817634589,-17.6427657588129,
2.));
#78134=CARTESIAN_POINT('Ctrl Pts',(-43.9821717973476,-18.4114484455697,
2.));
#78135=CARTESIAN_POINT('Ctrl Pts',(-43.7389516037332,-19.1807961183945,
2.));
#78136=CARTESIAN_POINT('Ctrl Pts',(-43.4759822277029,-19.9449281117179,
2.));
#78137=CARTESIAN_POINT('Ctrl Pts',(-43.1935467196845,-20.7028522155842,
2.));
#78138=CARTESIAN_POINT('Ctrl Pts',(-42.910867002848,-21.4614316610926,2.));
#78139=CARTESIAN_POINT('Ctrl Pts',(-42.6086875412903,-22.2137923134146,
2.));
#78140=CARTESIAN_POINT('Ctrl Pts',(-42.2873413628421,-22.9589568069778,
2.));
#78141=CARTESIAN_POINT('Ctrl Pts',(-41.9655415151298,-23.7051733069134,
2.));
#78142=CARTESIAN_POINT('Ctrl Pts',(-41.6245208625705,-24.4441731529251,
2.));
#78143=CARTESIAN_POINT('Ctrl Pts',(-41.264662211266,-25.1749947461293,2.));
#78144=CARTESIAN_POINT('Ctrl Pts',(-40.9045440154532,-25.9063434372103,
2.));
#78145=CARTESIAN_POINT('Ctrl Pts',(-40.5255607195679,-26.6295019186582,
2.));
#78146=CARTESIAN_POINT('Ctrl Pts',(-40.1281432215925,-27.3435288185695,
2.));
#78147=CARTESIAN_POINT('Ctrl Pts',(-39.7321221742634,-28.0550467617012,
2.));
#78148=CARTESIAN_POINT('Ctrl Pts',(-39.3177963661132,-28.7574970523859,
2.));
#78149=CARTESIAN_POINT('Ctrl Pts',(-38.8856375198795,-29.4499724760943,
2.));
#78150=CARTESIAN_POINT('Ctrl Pts',(-38.6009983664357,-29.9060677755493,
2.));
#78151=CARTESIAN_POINT('Ctrl Pts',(-38.3086239303204,-30.3578363585341,
2.));
#78152=CARTESIAN_POINT('Ctrl Pts',(-38.0086594336355,-30.8050251768588,
2.));
#78153=CARTESIAN_POINT('Ctrl Pts',(-37.8531970881941,-31.0367893466863,
2.));
#78154=CARTESIAN_POINT('Ctrl Pts',(-37.6956964623238,-31.2673229660863,
2.));
#78155=CARTESIAN_POINT('Ctrl Pts',(-37.5361777128299,-31.4965928746404,
2.));
#78156=CARTESIAN_POINT('',(-37.5361777128299,-31.4965928746404,0.));
#78157=CARTESIAN_POINT('Ctrl Pts',(-37.5361777128299,-31.4965928746404,
0.));
#78158=CARTESIAN_POINT('Ctrl Pts',(-37.5361777128299,-31.4965928746404,
20.));
#78159=CARTESIAN_POINT('Ctrl Pts',(-37.5400435810124,-31.4910366171629,
0.));
#78160=CARTESIAN_POINT('Ctrl Pts',(-37.5400435810124,-31.4910366171629,
20.));
#78161=CARTESIAN_POINT('Ctrl Pts',(-37.5477733397939,-31.4799228688318,
0.));
#78162=CARTESIAN_POINT('Ctrl Pts',(-37.5477733397939,-31.4799228688318,
20.));
#78163=CARTESIAN_POINT('Ctrl Pts',(-37.5593620452151,-31.4632485462068,
0.));
#78164=CARTESIAN_POINT('Ctrl Pts',(-37.5593620452151,-31.4632485462068,
20.));
#78165=CARTESIAN_POINT('Ctrl Pts',(-37.574801786924,-31.4410087157717,0.));
#78166=CARTESIAN_POINT('Ctrl Pts',(-37.574801786924,-31.4410087157717,20.));
#78167=CARTESIAN_POINT('Ctrl Pts',(-37.5940816876034,-31.4131965946731,
0.));
#78168=CARTESIAN_POINT('Ctrl Pts',(-37.5940816876034,-31.4131965946731,
20.));
#78169=CARTESIAN_POINT('Ctrl Pts',(-37.6133418102375,-31.3853721428083,
0.));
#78170=CARTESIAN_POINT('Ctrl Pts',(-37.6133418102375,-31.3853721428083,
20.));
#78171=CARTESIAN_POINT('Ctrl Pts',(-37.6325821517747,-31.3575353648538,
0.));
#78172=CARTESIAN_POINT('Ctrl Pts',(-37.6325821517747,-31.3575353648538,
20.));
#78173=CARTESIAN_POINT('Ctrl Pts',(-37.6518027072643,-31.3296862686536,
0.));
#78174=CARTESIAN_POINT('Ctrl Pts',(-37.6518027072643,-31.3296862686536,
20.));
#78175=CARTESIAN_POINT('Ctrl Pts',(-37.6710034693473,-31.3018248661211,
0.));
#78176=CARTESIAN_POINT('Ctrl Pts',(-37.6710034693473,-31.3018248661211,
20.));
#78177=CARTESIAN_POINT('Ctrl Pts',(-37.6901844288974,-31.2739511721649,
0.));
#78178=CARTESIAN_POINT('Ctrl Pts',(-37.6901844288974,-31.2739511721649,
20.));
#78179=CARTESIAN_POINT('Ctrl Pts',(-37.7093455757381,-31.2460652034827,
0.));
#78180=CARTESIAN_POINT('Ctrl Pts',(-37.7093455757381,-31.2460652034827,
20.));
#78181=CARTESIAN_POINT('Ctrl Pts',(-37.7284868993471,-31.2181669773772,
0.));
#78182=CARTESIAN_POINT('Ctrl Pts',(-37.7284868993471,-31.2181669773772,
20.));
#78183=CARTESIAN_POINT('Ctrl Pts',(-37.7476083895316,-31.1902565106222,
0.));
#78184=CARTESIAN_POINT('Ctrl Pts',(-37.7476083895316,-31.1902565106222,
20.));
#78185=CARTESIAN_POINT('Ctrl Pts',(-37.7667100372089,-31.1623338181506,
0.));
#78186=CARTESIAN_POINT('Ctrl Pts',(-37.7667100372089,-31.1623338181506,
20.));
#78187=CARTESIAN_POINT('Ctrl Pts',(-37.7857918342009,-31.1343989133989,
0.));
#78188=CARTESIAN_POINT('Ctrl Pts',(-37.7857918342009,-31.1343989133989,
20.));
#78189=CARTESIAN_POINT('Ctrl Pts',(-37.8048537728749,-31.1064518089103,
0.));
#78190=CARTESIAN_POINT('Ctrl Pts',(-37.8048537728749,-31.1064518089103,
20.));
#78191=CARTESIAN_POINT('Ctrl Pts',(-37.8238958458276,-31.0784925168637,
0.));
#78192=CARTESIAN_POINT('Ctrl Pts',(-37.8238958458276,-31.0784925168637,
20.));
#78193=CARTESIAN_POINT('Ctrl Pts',(-37.8429180455734,-31.0505210495984,
0.));
#78194=CARTESIAN_POINT('Ctrl Pts',(-37.8429180455734,-31.0505210495984,
20.));
#78195=CARTESIAN_POINT('Ctrl Pts',(-37.861920364175,-31.0225374202321,0.));
#78196=CARTESIAN_POINT('Ctrl Pts',(-37.861920364175,-31.0225374202321,20.));
#78197=CARTESIAN_POINT('Ctrl Pts',(-37.8809027932971,-30.9945416425721,
0.));
#78198=CARTESIAN_POINT('Ctrl Pts',(-37.8809027932971,-30.9945416425721,
20.));
#78199=CARTESIAN_POINT('Ctrl Pts',(-37.8998653243731,-30.9665337308352,
0.));
#78200=CARTESIAN_POINT('Ctrl Pts',(-37.8998653243731,-30.9665337308352,
20.));
#78201=CARTESIAN_POINT('Ctrl Pts',(-37.9188079487378,-30.938513699426,0.));
#78202=CARTESIAN_POINT('Ctrl Pts',(-37.9188079487378,-30.938513699426,20.));
#78203=CARTESIAN_POINT('Ctrl Pts',(-37.9377306577632,-30.9104815627079,
0.));
#78204=CARTESIAN_POINT('Ctrl Pts',(-37.9377306577632,-30.9104815627079,
20.));
#78205=CARTESIAN_POINT('Ctrl Pts',(-37.9566334430211,-30.882437334731,0.));
#78206=CARTESIAN_POINT('Ctrl Pts',(-37.9566334430211,-30.882437334731,20.));
#78207=CARTESIAN_POINT('Ctrl Pts',(-37.9755162962752,-30.8543810292446,
0.));
#78208=CARTESIAN_POINT('Ctrl Pts',(-37.9755162962752,-30.8543810292446,
20.));
#78209=CARTESIAN_POINT('Ctrl Pts',(-37.9943792094053,-30.8263126598247,
0.));
#78210=CARTESIAN_POINT('Ctrl Pts',(-37.9943792094053,-30.8263126598247,
20.));
#78211=CARTESIAN_POINT('Ctrl Pts',(-38.0132221743517,-30.7982322399668,
0.));
#78212=CARTESIAN_POINT('Ctrl Pts',(-38.0132221743517,-30.7982322399668,
20.));
#78213=CARTESIAN_POINT('Ctrl Pts',(-38.0320451830565,-30.7701397831859,
0.));
#78214=CARTESIAN_POINT('Ctrl Pts',(-38.0320451830565,-30.7701397831859,
20.));
#78215=CARTESIAN_POINT('Ctrl Pts',(-38.0508482273931,-30.7420353031339,
0.));
#78216=CARTESIAN_POINT('Ctrl Pts',(-38.0508482273931,-30.7420353031339,
20.));
#78217=CARTESIAN_POINT('Ctrl Pts',(-38.0696312991626,-30.7139188136053,
0.));
#78218=CARTESIAN_POINT('Ctrl Pts',(-38.0696312991626,-30.7139188136053,
20.));
#78219=CARTESIAN_POINT('Ctrl Pts',(-38.088394390128,-30.6857903284809,0.));
#78220=CARTESIAN_POINT('Ctrl Pts',(-38.088394390128,-30.6857903284809,20.));
#78221=CARTESIAN_POINT('Ctrl Pts',(-38.1071374920373,-30.6576498616875,
0.));
#78222=CARTESIAN_POINT('Ctrl Pts',(-38.1071374920373,-30.6576498616875,
20.));
#78223=CARTESIAN_POINT('Ctrl Pts',(-38.125860596649,-30.6294974271553,0.));
#78224=CARTESIAN_POINT('Ctrl Pts',(-38.125860596649,-30.6294974271553,20.));
#78225=CARTESIAN_POINT('Ctrl Pts',(-38.1445636957629,-30.6013330387674,
0.));
#78226=CARTESIAN_POINT('Ctrl Pts',(-38.1445636957629,-30.6013330387674,
20.));
#78227=CARTESIAN_POINT('Ctrl Pts',(-38.1632467812242,-30.5731567103519,
0.));
#78228=CARTESIAN_POINT('Ctrl Pts',(-38.1632467812242,-30.5731567103519,
20.));
#78229=CARTESIAN_POINT('Ctrl Pts',(-38.1819098449085,-30.5449684557073,
0.));
#78230=CARTESIAN_POINT('Ctrl Pts',(-38.1819098449085,-30.5449684557073,
20.));
#78231=CARTESIAN_POINT('Ctrl Pts',(-38.2005528787125,-30.5167682886194,
0.));
#78232=CARTESIAN_POINT('Ctrl Pts',(-38.2005528787125,-30.5167682886194,
20.));
#78233=CARTESIAN_POINT('Ctrl Pts',(-38.2191758745422,-30.4885562228796,
0.));
#78234=CARTESIAN_POINT('Ctrl Pts',(-38.2191758745422,-30.4885562228796,
20.));
#78235=CARTESIAN_POINT('Ctrl Pts',(-38.2377788243005,-30.460332272307,0.));
#78236=CARTESIAN_POINT('Ctrl Pts',(-38.2377788243005,-30.460332272307,20.));
#78237=CARTESIAN_POINT('Ctrl Pts',(-38.2563617198829,-30.4320964507535,
0.));
#78238=CARTESIAN_POINT('Ctrl Pts',(-38.2563617198829,-30.4320964507535,
20.));
#78239=CARTESIAN_POINT('Ctrl Pts',(-38.2749245531853,-30.4038487720928,
0.));
#78240=CARTESIAN_POINT('Ctrl Pts',(-38.2749245531853,-30.4038487720928,
20.));
#78241=CARTESIAN_POINT('Ctrl Pts',(-38.2934673161074,-30.3755892502132,
0.));
#78242=CARTESIAN_POINT('Ctrl Pts',(-38.2934673161074,-30.3755892502132,
20.));
#78243=CARTESIAN_POINT('Ctrl Pts',(-38.3119900005578,-30.3473178990095,
0.));
#78244=CARTESIAN_POINT('Ctrl Pts',(-38.3119900005578,-30.3473178990095,
20.));
#78245=CARTESIAN_POINT('Ctrl Pts',(-38.3304925984593,-30.3190347323738,
0.));
#78246=CARTESIAN_POINT('Ctrl Pts',(-38.3304925984593,-30.3190347323738,
20.));
#78247=CARTESIAN_POINT('Ctrl Pts',(-38.3489751017513,-30.2907397641919,
0.));
#78248=CARTESIAN_POINT('Ctrl Pts',(-38.3489751017513,-30.2907397641919,
20.));
#78249=CARTESIAN_POINT('Ctrl Pts',(-38.3674375023871,-30.2624330083488,
0.));
#78250=CARTESIAN_POINT('Ctrl Pts',(-38.3674375023871,-30.2624330083488,
20.));
#78251=CARTESIAN_POINT('Ctrl Pts',(-38.3858797923318,-30.2341144787313,
0.));
#78252=CARTESIAN_POINT('Ctrl Pts',(-38.3858797923318,-30.2341144787313,
20.));
#78253=CARTESIAN_POINT('Ctrl Pts',(-38.4043019635603,-30.2057841892317,
0.));
#78254=CARTESIAN_POINT('Ctrl Pts',(-38.4043019635603,-30.2057841892317,
20.));
#78255=CARTESIAN_POINT('Ctrl Pts',(-38.4227040080549,-30.1774421537519,
0.));
#78256=CARTESIAN_POINT('Ctrl Pts',(-38.4227040080549,-30.1774421537519,
20.));
#78257=CARTESIAN_POINT('Ctrl Pts',(-38.4410859178039,-30.1490883862047,
0.));
#78258=CARTESIAN_POINT('Ctrl Pts',(-38.4410859178039,-30.1490883862047,
20.));
#78259=CARTESIAN_POINT('Ctrl Pts',(-38.4594476848032,-30.1207229005118,
0.));
#78260=CARTESIAN_POINT('Ctrl Pts',(-38.4594476848032,-30.1207229005118,
20.));
#78261=CARTESIAN_POINT('Ctrl Pts',(-38.4777893010568,-30.0923457106026,
0.));
#78262=CARTESIAN_POINT('Ctrl Pts',(-38.4777893010568,-30.0923457106026,
20.));
#78263=CARTESIAN_POINT('Ctrl Pts',(-38.4961107585777,-30.0639568304126,
0.));
#78264=CARTESIAN_POINT('Ctrl Pts',(-38.4961107585777,-30.0639568304126,
20.));
#78265=CARTESIAN_POINT('Ctrl Pts',(-38.5144120493894,-30.0355562738816,
0.));
#78266=CARTESIAN_POINT('Ctrl Pts',(-38.5144120493894,-30.0355562738816,
20.));
#78267=CARTESIAN_POINT('Ctrl Pts',(-38.532693165526,-30.0071440549534,0.));
#78268=CARTESIAN_POINT('Ctrl Pts',(-38.532693165526,-30.0071440549534,20.));
#78269=CARTESIAN_POINT('Ctrl Pts',(-38.5509540990321,-29.978720187576,0.));
#78270=CARTESIAN_POINT('Ctrl Pts',(-38.5509540990321,-29.978720187576,20.));
#78271=CARTESIAN_POINT('Ctrl Pts',(-38.5691948419622,-29.9502846857025,
0.));
#78272=CARTESIAN_POINT('Ctrl Pts',(-38.5691948419622,-29.9502846857025,
20.));
#78273=CARTESIAN_POINT('Ctrl Pts',(-38.5874153863803,-29.9218375632917,
0.));
#78274=CARTESIAN_POINT('Ctrl Pts',(-38.5874153863803,-29.9218375632917,
20.));
#78275=CARTESIAN_POINT('Ctrl Pts',(-38.6056157243597,-29.8933788343089,
0.));
#78276=CARTESIAN_POINT('Ctrl Pts',(-38.6056157243597,-29.8933788343089,
20.));
#78277=CARTESIAN_POINT('Ctrl Pts',(-38.6237958479822,-29.864908512726,0.));
#78278=CARTESIAN_POINT('Ctrl Pts',(-38.6237958479822,-29.864908512726,20.));
#78279=CARTESIAN_POINT('Ctrl Pts',(-38.6419557493389,-29.8364266125215,
0.));
#78280=CARTESIAN_POINT('Ctrl Pts',(-38.6419557493389,-29.8364266125215,
20.));
#78281=CARTESIAN_POINT('Ctrl Pts',(-38.66009542053,-29.8079331476799,0.));
#78282=CARTESIAN_POINT('Ctrl Pts',(-38.66009542053,-29.8079331476799,20.));
#78283=CARTESIAN_POINT('Ctrl Pts',(-38.6782148536649,-29.7794281321916,
0.));
#78284=CARTESIAN_POINT('Ctrl Pts',(-38.6782148536649,-29.7794281321916,
20.));
#78285=CARTESIAN_POINT('Ctrl Pts',(-38.6963140408627,-29.7509115800524,
0.));
#78286=CARTESIAN_POINT('Ctrl Pts',(-38.6963140408627,-29.7509115800524,
20.));
#78287=CARTESIAN_POINT('Ctrl Pts',(-38.7143929742521,-29.7223835052637,
0.));
#78288=CARTESIAN_POINT('Ctrl Pts',(-38.7143929742521,-29.7223835052637,
20.));
#78289=CARTESIAN_POINT('Ctrl Pts',(-38.7324516459718,-29.6938439218325,
0.));
#78290=CARTESIAN_POINT('Ctrl Pts',(-38.7324516459718,-29.6938439218325,
20.));
#78291=CARTESIAN_POINT('Ctrl Pts',(-38.7504900481697,-29.6652928437714,
0.));
#78292=CARTESIAN_POINT('Ctrl Pts',(-38.7504900481697,-29.6652928437714,
20.));
#78293=CARTESIAN_POINT('Ctrl Pts',(-38.7685081730036,-29.6367302850988,
0.));
#78294=CARTESIAN_POINT('Ctrl Pts',(-38.7685081730036,-29.6367302850988,
20.));
#78295=CARTESIAN_POINT('Ctrl Pts',(-38.7865060126402,-29.6081562598384,
0.));
#78296=CARTESIAN_POINT('Ctrl Pts',(-38.7865060126402,-29.6081562598384,
20.));
#78297=CARTESIAN_POINT('Ctrl Pts',(-38.8044835592559,-29.5795707820205,
0.));
#78298=CARTESIAN_POINT('Ctrl Pts',(-38.8044835592559,-29.5795707820205,
20.));
#78299=CARTESIAN_POINT('Ctrl Pts',(-38.8224408050366,-29.5509738656807,
0.));
#78300=CARTESIAN_POINT('Ctrl Pts',(-38.8224408050366,-29.5509738656807,
20.));
#78301=CARTESIAN_POINT('Ctrl Pts',(-38.8403777421773,-29.5223655248609,
0.));
#78302=CARTESIAN_POINT('Ctrl Pts',(-38.8403777421773,-29.5223655248609,
20.));
#78303=CARTESIAN_POINT('Ctrl Pts',(-38.8582943628826,-29.4937457736083,
0.));
#78304=CARTESIAN_POINT('Ctrl Pts',(-38.8582943628826,-29.4937457736083,
20.));
#78305=CARTESIAN_POINT('Ctrl Pts',(-38.8761906593666,-29.4651146259764,
0.));
#78306=CARTESIAN_POINT('Ctrl Pts',(-38.8761906593666,-29.4651146259764,
20.));
#78307=CARTESIAN_POINT('Ctrl Pts',(-38.8940666238533,-29.4364720960241,
0.));
#78308=CARTESIAN_POINT('Ctrl Pts',(-38.8940666238533,-29.4364720960241,
20.));
#78309=CARTESIAN_POINT('Ctrl Pts',(-38.9119222485755,-29.4078181978158,
0.));
#78310=CARTESIAN_POINT('Ctrl Pts',(-38.9119222485755,-29.4078181978158,
20.));
#78311=CARTESIAN_POINT('Ctrl Pts',(-38.9297575257761,-29.3791529454216,
0.));
#78312=CARTESIAN_POINT('Ctrl Pts',(-38.9297575257761,-29.3791529454216,
20.));
#78313=CARTESIAN_POINT('Ctrl Pts',(-38.9475724477072,-29.3504763529173,
0.));
#78314=CARTESIAN_POINT('Ctrl Pts',(-38.9475724477072,-29.3504763529173,
20.));
#78315=CARTESIAN_POINT('Ctrl Pts',(-38.9653670066308,-29.3217884343845,
0.));
#78316=CARTESIAN_POINT('Ctrl Pts',(-38.9653670066308,-29.3217884343845,
20.));
#78317=CARTESIAN_POINT('Ctrl Pts',(-38.9831411948183,-29.2930892039104,
0.));
#78318=CARTESIAN_POINT('Ctrl Pts',(-38.9831411948183,-29.2930892039104,
20.));
#78319=CARTESIAN_POINT('Ctrl Pts',(-39.0008950045503,-29.2643786755883,
0.));
#78320=CARTESIAN_POINT('Ctrl Pts',(-39.0008950045503,-29.2643786755883,
20.));
#78321=CARTESIAN_POINT('Ctrl Pts',(-39.0186284281173,-29.2356568635168,
0.));
#78322=CARTESIAN_POINT('Ctrl Pts',(-39.0186284281173,-29.2356568635168,
20.));
#78323=CARTESIAN_POINT('Ctrl Pts',(-39.0363414578191,-29.2069237818005,
0.));
#78324=CARTESIAN_POINT('Ctrl Pts',(-39.0363414578191,-29.2069237818005,
20.));
#78325=CARTESIAN_POINT('Ctrl Pts',(-39.054034085965,-29.1781794445493,0.));
#78326=CARTESIAN_POINT('Ctrl Pts',(-39.054034085965,-29.1781794445493,20.));
#78327=CARTESIAN_POINT('Ctrl Pts',(-39.0717063048737,-29.1494238658788,
0.));
#78328=CARTESIAN_POINT('Ctrl Pts',(-39.0717063048737,-29.1494238658788,
20.));
#78329=CARTESIAN_POINT('Ctrl Pts',(-39.0893581068737,-29.1206570599103,
0.));
#78330=CARTESIAN_POINT('Ctrl Pts',(-39.0893581068737,-29.1206570599103,
20.));
#78331=CARTESIAN_POINT('Ctrl Pts',(-39.106989484303,-29.0918790407708,0.));
#78332=CARTESIAN_POINT('Ctrl Pts',(-39.106989484303,-29.0918790407708,20.));
#78333=CARTESIAN_POINT('Ctrl Pts',(-39.1246004295092,-29.0630898225929,
0.));
#78334=CARTESIAN_POINT('Ctrl Pts',(-39.1246004295092,-29.0630898225929,
20.));
#78335=CARTESIAN_POINT('Ctrl Pts',(-39.1421909348497,-29.034289419515,0.));
#78336=CARTESIAN_POINT('Ctrl Pts',(-39.1421909348497,-29.034289419515,20.));
#78337=CARTESIAN_POINT('Ctrl Pts',(-39.1597609926911,-29.0054778456813,
0.));
#78338=CARTESIAN_POINT('Ctrl Pts',(-39.1597609926911,-29.0054778456813,
20.));
#78339=CARTESIAN_POINT('Ctrl Pts',(-39.1773105954099,-28.9766551152413,
0.));
#78340=CARTESIAN_POINT('Ctrl Pts',(-39.1773105954099,-28.9766551152413,
20.));
#78341=CARTESIAN_POINT('Ctrl Pts',(-39.1948397353917,-28.9478212423503,
0.));
#78342=CARTESIAN_POINT('Ctrl Pts',(-39.1948397353917,-28.9478212423503,
20.));
#78343=CARTESIAN_POINT('Ctrl Pts',(-39.2123484050317,-28.9189762411689,
0.));
#78344=CARTESIAN_POINT('Ctrl Pts',(-39.2123484050317,-28.9189762411689,
20.));
#78345=CARTESIAN_POINT('Ctrl Pts',(-39.2298365967351,-28.8901201258634,
0.));
#78346=CARTESIAN_POINT('Ctrl Pts',(-39.2298365967351,-28.8901201258634,
20.));
#78347=CARTESIAN_POINT('Ctrl Pts',(-39.2473043029163,-28.8612529106058,
0.));
#78348=CARTESIAN_POINT('Ctrl Pts',(-39.2473043029163,-28.8612529106058,
20.));
#78349=CARTESIAN_POINT('Ctrl Pts',(-39.2647515159997,-28.8323746095736,
0.));
#78350=CARTESIAN_POINT('Ctrl Pts',(-39.2647515159997,-28.8323746095736,
20.));
#78351=CARTESIAN_POINT('Ctrl Pts',(-39.2821782284193,-28.80348523695,0.));
#78352=CARTESIAN_POINT('Ctrl Pts',(-39.2821782284193,-28.80348523695,20.));
#78353=CARTESIAN_POINT('Ctrl Pts',(-39.2995844326181,-28.7745848069238,
0.));
#78354=CARTESIAN_POINT('Ctrl Pts',(-39.2995844326181,-28.7745848069238,
20.));
#78355=CARTESIAN_POINT('Ctrl Pts',(-39.316970121049,-28.7456733336894,0.));
#78356=CARTESIAN_POINT('Ctrl Pts',(-39.316970121049,-28.7456733336894,20.));
#78357=CARTESIAN_POINT('Ctrl Pts',(-39.3343352861746,-28.7167508314468,
0.));
#78358=CARTESIAN_POINT('Ctrl Pts',(-39.3343352861746,-28.7167508314468,
20.));
#78359=CARTESIAN_POINT('Ctrl Pts',(-39.3516799204672,-28.6878173144015,
0.));
#78360=CARTESIAN_POINT('Ctrl Pts',(-39.3516799204672,-28.6878173144015,
20.));
#78361=CARTESIAN_POINT('Ctrl Pts',(-39.3690040164086,-28.6588727967647,
0.));
#78362=CARTESIAN_POINT('Ctrl Pts',(-39.3690040164086,-28.6588727967647,
20.));
#78363=CARTESIAN_POINT('Ctrl Pts',(-39.3863075664906,-28.6299172927529,
0.));
#78364=CARTESIAN_POINT('Ctrl Pts',(-39.3863075664906,-28.6299172927529,
20.));
#78365=CARTESIAN_POINT('Ctrl Pts',(-39.4035905632141,-28.600950816588,0.));
#78366=CARTESIAN_POINT('Ctrl Pts',(-39.4035905632141,-28.600950816588,20.));
#78367=CARTESIAN_POINT('Ctrl Pts',(-39.4208529990894,-28.5719733824975,
0.));
#78368=CARTESIAN_POINT('Ctrl Pts',(-39.4208529990894,-28.5719733824975,
20.));
#78369=CARTESIAN_POINT('Ctrl Pts',(-39.4380948666368,-28.5429850047148,
0.));
#78370=CARTESIAN_POINT('Ctrl Pts',(-39.4380948666368,-28.5429850047148,
20.));
#78371=CARTESIAN_POINT('Ctrl Pts',(-39.4553161583861,-28.5139856974786,
0.));
#78372=CARTESIAN_POINT('Ctrl Pts',(-39.4553161583861,-28.5139856974786,
20.));
#78373=CARTESIAN_POINT('Ctrl Pts',(-39.4725168668771,-28.4849754750331,
0.));
#78374=CARTESIAN_POINT('Ctrl Pts',(-39.4725168668771,-28.4849754750331,
20.));
#78375=CARTESIAN_POINT('Ctrl Pts',(-39.4896969846589,-28.455954351628,0.));
#78376=CARTESIAN_POINT('Ctrl Pts',(-39.4896969846589,-28.455954351628,20.));
#78377=CARTESIAN_POINT('Ctrl Pts',(-39.5068565042907,-28.4269223415187,
0.));
#78378=CARTESIAN_POINT('Ctrl Pts',(-39.5068565042907,-28.4269223415187,
20.));
#78379=CARTESIAN_POINT('Ctrl Pts',(-39.5239954183412,-28.3978794589661,
0.));
#78380=CARTESIAN_POINT('Ctrl Pts',(-39.5239954183412,-28.3978794589661,
20.));
#78381=CARTESIAN_POINT('Ctrl Pts',(-39.5411137193887,-28.3688257182364,
0.));
#78382=CARTESIAN_POINT('Ctrl Pts',(-39.5411137193887,-28.3688257182364,
20.));
#78383=CARTESIAN_POINT('Ctrl Pts',(-39.5582114000212,-28.3397611336014,
0.));
#78384=CARTESIAN_POINT('Ctrl Pts',(-39.5582114000212,-28.3397611336014,
20.));
#78385=CARTESIAN_POINT('Ctrl Pts',(-39.5752884528361,-28.3106857193381,
0.));
#78386=CARTESIAN_POINT('Ctrl Pts',(-39.5752884528361,-28.3106857193381,
20.));
#78387=CARTESIAN_POINT('Ctrl Pts',(-39.5923448704403,-28.2815994897291,
0.));
#78388=CARTESIAN_POINT('Ctrl Pts',(-39.5923448704403,-28.2815994897291,
20.));
#78389=CARTESIAN_POINT('Ctrl Pts',(-39.6093806454502,-28.2525024590626,
0.));
#78390=CARTESIAN_POINT('Ctrl Pts',(-39.6093806454502,-28.2525024590626,
20.));
#78391=CARTESIAN_POINT('Ctrl Pts',(-39.6263957704923,-28.2233946416323,
0.));
#78392=CARTESIAN_POINT('Ctrl Pts',(-39.6263957704923,-28.2233946416323,
20.));
#78393=CARTESIAN_POINT('Ctrl Pts',(-39.6433902382029,-28.1942760517371,
0.));
#78394=CARTESIAN_POINT('Ctrl Pts',(-39.6433902382029,-28.1942760517371,
20.));
#78395=CARTESIAN_POINT('Ctrl Pts',(-39.6603640412281,-28.1651467036817,
0.));
#78396=CARTESIAN_POINT('Ctrl Pts',(-39.6603640412281,-28.1651467036817,
20.));
#78397=CARTESIAN_POINT('Ctrl Pts',(-39.6773171722241,-28.136006611776,0.));
#78398=CARTESIAN_POINT('Ctrl Pts',(-39.6773171722241,-28.136006611776,20.));
#78399=CARTESIAN_POINT('Ctrl Pts',(-39.6942496238565,-28.1068557903356,
0.));
#78400=CARTESIAN_POINT('Ctrl Pts',(-39.6942496238565,-28.1068557903356,
20.));
#78401=CARTESIAN_POINT('Ctrl Pts',(-39.7111613888006,-28.0776942536814,
0.));
#78402=CARTESIAN_POINT('Ctrl Pts',(-39.7111613888006,-28.0776942536814,
20.));
#78403=CARTESIAN_POINT('Ctrl Pts',(-39.728052459741,-28.0485220161395,0.));
#78404=CARTESIAN_POINT('Ctrl Pts',(-39.728052459741,-28.0485220161395,20.));
#78405=CARTESIAN_POINT('Ctrl Pts',(-39.7449228293718,-28.0193390920415,
0.));
#78406=CARTESIAN_POINT('Ctrl Pts',(-39.7449228293718,-28.0193390920415,
20.));
#78407=CARTESIAN_POINT('Ctrl Pts',(-39.7617724903968,-27.9901454957246,
0.));
#78408=CARTESIAN_POINT('Ctrl Pts',(-39.7617724903968,-27.9901454957246,
20.));
#78409=CARTESIAN_POINT('Ctrl Pts',(-39.7786014355293,-27.960941241531,0.));
#78410=CARTESIAN_POINT('Ctrl Pts',(-39.7786014355293,-27.960941241531,20.));
#78411=CARTESIAN_POINT('Ctrl Pts',(-39.795409657493,-27.9317263438086,0.));
#78412=CARTESIAN_POINT('Ctrl Pts',(-39.795409657493,-27.9317263438086,20.));
#78413=CARTESIAN_POINT('Ctrl Pts',(-39.8121971490214,-27.9025008169107,
0.));
#78414=CARTESIAN_POINT('Ctrl Pts',(-39.8121971490214,-27.9025008169107,
20.));
#78415=CARTESIAN_POINT('Ctrl Pts',(-39.828963902858,-27.8732646751959,0.));
#78416=CARTESIAN_POINT('Ctrl Pts',(-39.828963902858,-27.8732646751959,20.));
#78417=CARTESIAN_POINT('Ctrl Pts',(-39.845709911756,-27.8440179330284,0.));
#78418=CARTESIAN_POINT('Ctrl Pts',(-39.845709911756,-27.8440179330284,20.));
#78419=CARTESIAN_POINT('Ctrl Pts',(-39.8624351684781,-27.8147606047778,
0.));
#78420=CARTESIAN_POINT('Ctrl Pts',(-39.8624351684781,-27.8147606047778,
20.));
#78421=CARTESIAN_POINT('Ctrl Pts',(-39.8791396657966,-27.785492704819,0.));
#78422=CARTESIAN_POINT('Ctrl Pts',(-39.8791396657966,-27.785492704819,20.));
#78423=CARTESIAN_POINT('Ctrl Pts',(-39.8958233964934,-27.7562142475319,
0.));
#78424=CARTESIAN_POINT('Ctrl Pts',(-39.8958233964934,-27.7562142475319,
20.));
#78425=CARTESIAN_POINT('Ctrl Pts',(-39.9124863533599,-27.726925247302,0.));
#78426=CARTESIAN_POINT('Ctrl Pts',(-39.9124863533599,-27.726925247302,20.));
#78427=CARTESIAN_POINT('Ctrl Pts',(-39.9291285291975,-27.6976257185198,
0.));
#78428=CARTESIAN_POINT('Ctrl Pts',(-39.9291285291975,-27.6976257185198,
20.));
#78429=CARTESIAN_POINT('Ctrl Pts',(-39.9457499168175,-27.6683156755815,
0.));
#78430=CARTESIAN_POINT('Ctrl Pts',(-39.9457499168175,-27.6683156755815,
20.));
#78431=CARTESIAN_POINT('Ctrl Pts',(-39.9623505090412,-27.6389951328887,
0.));
#78432=CARTESIAN_POINT('Ctrl Pts',(-39.9623505090412,-27.6389951328887,
20.));
#78433=CARTESIAN_POINT('Ctrl Pts',(-39.9789302986995,-27.6096641048483,
0.));
#78434=CARTESIAN_POINT('Ctrl Pts',(-39.9789302986995,-27.6096641048483,
20.));
#78435=CARTESIAN_POINT('Ctrl Pts',(-39.9954892786331,-27.5803226058724,
0.));
#78436=CARTESIAN_POINT('Ctrl Pts',(-39.9954892786331,-27.5803226058724,
20.));
#78437=CARTESIAN_POINT('Ctrl Pts',(-40.0120274416924,-27.5509706503786,
0.));
#78438=CARTESIAN_POINT('Ctrl Pts',(-40.0120274416924,-27.5509706503786,
20.));
#78439=CARTESIAN_POINT('Ctrl Pts',(-40.0285447807378,-27.5216082527897,
0.));
#78440=CARTESIAN_POINT('Ctrl Pts',(-40.0285447807378,-27.5216082527897,
20.));
#78441=CARTESIAN_POINT('Ctrl Pts',(-40.045041288639,-27.4922354275335,0.));
#78442=CARTESIAN_POINT('Ctrl Pts',(-40.045041288639,-27.4922354275335,20.));
#78443=CARTESIAN_POINT('Ctrl Pts',(-40.0615169582759,-27.4628521890436,
0.));
#78444=CARTESIAN_POINT('Ctrl Pts',(-40.0615169582759,-27.4628521890436,
20.));
#78445=CARTESIAN_POINT('Ctrl Pts',(-40.077971782538,-27.4334585517582,0.));
#78446=CARTESIAN_POINT('Ctrl Pts',(-40.077971782538,-27.4334585517582,20.));
#78447=CARTESIAN_POINT('Ctrl Pts',(-40.0944057543248,-27.4040545301216,
0.));
#78448=CARTESIAN_POINT('Ctrl Pts',(-40.0944057543248,-27.4040545301216,
20.));
#78449=CARTESIAN_POINT('Ctrl Pts',(-40.1108188665452,-27.374640138583,0.));
#78450=CARTESIAN_POINT('Ctrl Pts',(-40.1108188665452,-27.374640138583,20.));
#78451=CARTESIAN_POINT('Ctrl Pts',(-40.1272111121183,-27.3452153915969,
0.));
#78452=CARTESIAN_POINT('Ctrl Pts',(-40.1272111121183,-27.3452153915969,
20.));
#78453=CARTESIAN_POINT('Ctrl Pts',(-40.1435824839731,-27.3157803036231,
0.));
#78454=CARTESIAN_POINT('Ctrl Pts',(-40.1435824839731,-27.3157803036231,
20.));
#78455=CARTESIAN_POINT('Ctrl Pts',(-40.1599329750483,-27.2863348891265,
0.));
#78456=CARTESIAN_POINT('Ctrl Pts',(-40.1599329750483,-27.2863348891265,
20.));
#78457=CARTESIAN_POINT('Ctrl Pts',(-40.1762625782924,-27.2568791625774,
0.));
#78458=CARTESIAN_POINT('Ctrl Pts',(-40.1762625782924,-27.2568791625774,
20.));
#78459=CARTESIAN_POINT('Ctrl Pts',(-40.1925712866631,-27.2274131384508,
0.));
#78460=CARTESIAN_POINT('Ctrl Pts',(-40.1925712866631,-27.2274131384508,
20.));
#78461=CARTESIAN_POINT('Ctrl Pts',(-40.2088590931287,-27.1979368312277,
0.));
#78462=CARTESIAN_POINT('Ctrl Pts',(-40.2088590931287,-27.1979368312277,
20.));
#78463=CARTESIAN_POINT('Ctrl Pts',(-40.225125990667,-27.1684502553939,0.));
#78464=CARTESIAN_POINT('Ctrl Pts',(-40.225125990667,-27.1684502553939,20.));
#78465=CARTESIAN_POINT('Ctrl Pts',(-40.2413719722657,-27.1389534254409,
0.));
#78466=CARTESIAN_POINT('Ctrl Pts',(-40.2413719722657,-27.1389534254409,
20.));
#78467=CARTESIAN_POINT('Ctrl Pts',(-40.2575970309226,-27.1094463558649,
0.));
#78468=CARTESIAN_POINT('Ctrl Pts',(-40.2575970309226,-27.1094463558649,
20.));
#78469=CARTESIAN_POINT('Ctrl Pts',(-40.2738011596454,-27.0799290611676,
0.));
#78470=CARTESIAN_POINT('Ctrl Pts',(-40.2738011596454,-27.0799290611676,
20.));
#78471=CARTESIAN_POINT('Ctrl Pts',(-40.2899843514517,-27.0504015558557,
0.));
#78472=CARTESIAN_POINT('Ctrl Pts',(-40.2899843514517,-27.0504015558557,
20.));
#78473=CARTESIAN_POINT('Ctrl Pts',(-40.3061465993685,-27.0208638544413,
0.));
#78474=CARTESIAN_POINT('Ctrl Pts',(-40.3061465993685,-27.0208638544413,
20.));
#78475=CARTESIAN_POINT('Ctrl Pts',(-40.3222878964329,-26.9913159714415,
0.));
#78476=CARTESIAN_POINT('Ctrl Pts',(-40.3222878964329,-26.9913159714415,
20.));
#78477=CARTESIAN_POINT('Ctrl Pts',(-40.3384082356913,-26.9617579213786,
0.));
#78478=CARTESIAN_POINT('Ctrl Pts',(-40.3384082356913,-26.9617579213786,
20.));
#78479=CARTESIAN_POINT('Ctrl Pts',(-40.3545076102003,-26.9321897187802,
0.));
#78480=CARTESIAN_POINT('Ctrl Pts',(-40.3545076102003,-26.9321897187802,
20.));
#78481=CARTESIAN_POINT('Ctrl Pts',(-40.3705860130263,-26.9026113781788,
0.));
#78482=CARTESIAN_POINT('Ctrl Pts',(-40.3705860130263,-26.9026113781788,
20.));
#78483=CARTESIAN_POINT('Ctrl Pts',(-40.386643437246,-26.8730229141124,0.));
#78484=CARTESIAN_POINT('Ctrl Pts',(-40.386643437246,-26.8730229141124,20.));
#78485=CARTESIAN_POINT('Ctrl Pts',(-40.4026798759458,-26.8434243411241,
0.));
#78486=CARTESIAN_POINT('Ctrl Pts',(-40.4026798759458,-26.8434243411241,
20.));
#78487=CARTESIAN_POINT('Ctrl Pts',(-40.4186953222224,-26.8138156737619,
0.));
#78488=CARTESIAN_POINT('Ctrl Pts',(-40.4186953222224,-26.8138156737619,
20.));
#78489=CARTESIAN_POINT('Ctrl Pts',(-40.4346897691821,-26.7841969265794,
0.));
#78490=CARTESIAN_POINT('Ctrl Pts',(-40.4346897691821,-26.7841969265794,
20.));
#78491=CARTESIAN_POINT('Ctrl Pts',(-40.4506632099408,-26.754568114135,0.));
#78492=CARTESIAN_POINT('Ctrl Pts',(-40.4506632099408,-26.754568114135,20.));
#78493=CARTESIAN_POINT('Ctrl Pts',(-40.4666156376241,-26.7249292509923,
0.));
#78494=CARTESIAN_POINT('Ctrl Pts',(-40.4666156376241,-26.7249292509923,
20.));
#78495=CARTESIAN_POINT('Ctrl Pts',(-40.4825470453679,-26.6952803517197,
0.));
#78496=CARTESIAN_POINT('Ctrl Pts',(-40.4825470453679,-26.6952803517197,
20.));
#78497=CARTESIAN_POINT('Ctrl Pts',(-40.4984574263178,-26.6656214308914,
0.));
#78498=CARTESIAN_POINT('Ctrl Pts',(-40.4984574263178,-26.6656214308914,
20.));
#78499=CARTESIAN_POINT('Ctrl Pts',(-40.5143467736295,-26.6359525030862,
0.));
#78500=CARTESIAN_POINT('Ctrl Pts',(-40.5143467736295,-26.6359525030862,
20.));
#78501=CARTESIAN_POINT('Ctrl Pts',(-40.5302150804687,-26.606273582888,0.));
#78502=CARTESIAN_POINT('Ctrl Pts',(-40.5302150804687,-26.606273582888,20.));
#78503=CARTESIAN_POINT('Ctrl Pts',(-40.546062340011,-26.5765846848862,0.));
#78504=CARTESIAN_POINT('Ctrl Pts',(-40.546062340011,-26.5765846848862,20.));
#78505=CARTESIAN_POINT('Ctrl Pts',(-40.5618885454414,-26.5468858236748,
0.));
#78506=CARTESIAN_POINT('Ctrl Pts',(-40.5618885454414,-26.5468858236748,
20.));
#78507=CARTESIAN_POINT('Ctrl Pts',(-40.5776936899555,-26.5171770138532,
0.));
#78508=CARTESIAN_POINT('Ctrl Pts',(-40.5776936899555,-26.5171770138532,
20.));
#78509=CARTESIAN_POINT('Ctrl Pts',(-40.5934777667583,-26.4874582700259,
0.));
#78510=CARTESIAN_POINT('Ctrl Pts',(-40.5934777667583,-26.4874582700259,
20.));
#78511=CARTESIAN_POINT('Ctrl Pts',(-40.6092407690651,-26.4577296068023,
0.));
#78512=CARTESIAN_POINT('Ctrl Pts',(-40.6092407690651,-26.4577296068023,
20.));
#78513=CARTESIAN_POINT('Ctrl Pts',(-40.6249826901011,-26.427991038797,0.));
#78514=CARTESIAN_POINT('Ctrl Pts',(-40.6249826901011,-26.427991038797,20.));
#78515=CARTESIAN_POINT('Ctrl Pts',(-40.6407035231015,-26.3982425806297,
0.));
#78516=CARTESIAN_POINT('Ctrl Pts',(-40.6407035231015,-26.3982425806297,
20.));
#78517=CARTESIAN_POINT('Ctrl Pts',(-40.6564032613109,-26.3684842469248,
0.));
#78518=CARTESIAN_POINT('Ctrl Pts',(-40.6564032613109,-26.3684842469248,
20.));
#78519=CARTESIAN_POINT('Ctrl Pts',(-40.6720818979844,-26.338716052312,0.));
#78520=CARTESIAN_POINT('Ctrl Pts',(-40.6720818979844,-26.338716052312,20.));
#78521=CARTESIAN_POINT('Ctrl Pts',(-40.6877394263869,-26.308938011426,0.));
#78522=CARTESIAN_POINT('Ctrl Pts',(-40.6877394263869,-26.308938011426,20.));
#78523=CARTESIAN_POINT('Ctrl Pts',(-40.7033758397932,-26.2791501389067,
0.));
#78524=CARTESIAN_POINT('Ctrl Pts',(-40.7033758397932,-26.2791501389067,
20.));
#78525=CARTESIAN_POINT('Ctrl Pts',(-40.7189911314882,-26.2493524493989,
0.));
#78526=CARTESIAN_POINT('Ctrl Pts',(-40.7189911314882,-26.2493524493989,
20.));
#78527=CARTESIAN_POINT('Ctrl Pts',(-40.7345852947664,-26.2195449575524,
0.));
#78528=CARTESIAN_POINT('Ctrl Pts',(-40.7345852947664,-26.2195449575524,
20.));
#78529=CARTESIAN_POINT('Ctrl Pts',(-40.7501583229328,-26.1897276780219,
0.));
#78530=CARTESIAN_POINT('Ctrl Pts',(-40.7501583229328,-26.1897276780219,
20.));
#78531=CARTESIAN_POINT('Ctrl Pts',(-40.7657102093021,-26.1599006254674,
0.));
#78532=CARTESIAN_POINT('Ctrl Pts',(-40.7657102093021,-26.1599006254674,
20.));
#78533=CARTESIAN_POINT('Ctrl Pts',(-40.7812409471992,-26.1300638145535,
0.));
#78534=CARTESIAN_POINT('Ctrl Pts',(-40.7812409471992,-26.1300638145535,
20.));
#78535=CARTESIAN_POINT('Ctrl Pts',(-40.7967505299588,-26.1002172599501,
0.));
#78536=CARTESIAN_POINT('Ctrl Pts',(-40.7967505299588,-26.1002172599501,
20.));
#78537=CARTESIAN_POINT('Ctrl Pts',(-40.8122389509256,-26.0703609763318,
0.));
#78538=CARTESIAN_POINT('Ctrl Pts',(-40.8122389509256,-26.0703609763318,
20.));
#78539=CARTESIAN_POINT('Ctrl Pts',(-40.8277062034539,-26.0404949783787,
0.));
#78540=CARTESIAN_POINT('Ctrl Pts',(-40.8277062034539,-26.0404949783787,
20.));
#78541=CARTESIAN_POINT('Ctrl Pts',(-40.843152280908,-26.0106192807756,0.));
#78542=CARTESIAN_POINT('Ctrl Pts',(-40.843152280908,-26.0106192807756,20.));
#78543=CARTESIAN_POINT('Ctrl Pts',(-40.8585771766627,-25.9807338982121,
0.));
#78544=CARTESIAN_POINT('Ctrl Pts',(-40.8585771766627,-25.9807338982121,
20.));
#78545=CARTESIAN_POINT('Ctrl Pts',(-40.8739808841024,-25.950838845383,0.));
#78546=CARTESIAN_POINT('Ctrl Pts',(-40.8739808841024,-25.950838845383,20.));
#78547=CARTESIAN_POINT('Ctrl Pts',(-40.8893633966224,-25.9209341369879,
0.));
#78548=CARTESIAN_POINT('Ctrl Pts',(-40.8893633966224,-25.9209341369879,
20.));
#78549=CARTESIAN_POINT('Ctrl Pts',(-40.9047247076274,-25.891019787731,0.));
#78550=CARTESIAN_POINT('Ctrl Pts',(-40.9047247076274,-25.891019787731,20.));
#78551=CARTESIAN_POINT('Ctrl Pts',(-40.9200648105322,-25.861095812322,0.));
#78552=CARTESIAN_POINT('Ctrl Pts',(-40.9200648105322,-25.861095812322,20.));
#78553=CARTESIAN_POINT('Ctrl Pts',(-40.9353836987613,-25.8311622254754,
0.));
#78554=CARTESIAN_POINT('Ctrl Pts',(-40.9353836987613,-25.8311622254754,
20.));
#78555=CARTESIAN_POINT('Ctrl Pts',(-40.9506813657491,-25.8012190419102,
0.));
#78556=CARTESIAN_POINT('Ctrl Pts',(-40.9506813657491,-25.8012190419102,
20.));
#78557=CARTESIAN_POINT('Ctrl Pts',(-40.9659578049399,-25.7712662763511,
0.));
#78558=CARTESIAN_POINT('Ctrl Pts',(-40.9659578049399,-25.7712662763511,
20.));
#78559=CARTESIAN_POINT('Ctrl Pts',(-40.981213009789,-25.7413039435271,0.));
#78560=CARTESIAN_POINT('Ctrl Pts',(-40.981213009789,-25.7413039435271,20.));
#78561=CARTESIAN_POINT('Ctrl Pts',(-40.9964469737613,-25.7113320581728,
0.));
#78562=CARTESIAN_POINT('Ctrl Pts',(-40.9964469737613,-25.7113320581728,
20.));
#78563=CARTESIAN_POINT('Ctrl Pts',(-41.0116596903317,-25.6813506350271,
0.));
#78564=CARTESIAN_POINT('Ctrl Pts',(-41.0116596903317,-25.6813506350271,
20.));
#78565=CARTESIAN_POINT('Ctrl Pts',(-41.0268511529852,-25.6513596888338,
0.));
#78566=CARTESIAN_POINT('Ctrl Pts',(-41.0268511529852,-25.6513596888338,
20.));
#78567=CARTESIAN_POINT('Ctrl Pts',(-41.0420213552163,-25.6213592343415,
0.));
#78568=CARTESIAN_POINT('Ctrl Pts',(-41.0420213552163,-25.6213592343415,
20.));
#78569=CARTESIAN_POINT('Ctrl Pts',(-41.05717029053,-25.5913492863038,0.));
#78570=CARTESIAN_POINT('Ctrl Pts',(-41.05717029053,-25.5913492863038,20.));
#78571=CARTESIAN_POINT('Ctrl Pts',(-41.072297952441,-25.5613298594791,0.));
#78572=CARTESIAN_POINT('Ctrl Pts',(-41.072297952441,-25.5613298594791,20.));
#78573=CARTESIAN_POINT('Ctrl Pts',(-41.0874043344745,-25.5313009686309,
0.));
#78574=CARTESIAN_POINT('Ctrl Pts',(-41.0874043344745,-25.5313009686309,
20.));
#78575=CARTESIAN_POINT('Ctrl Pts',(-41.1024894301655,-25.5012626285275,
0.));
#78576=CARTESIAN_POINT('Ctrl Pts',(-41.1024894301655,-25.5012626285275,
20.));
#78577=CARTESIAN_POINT('Ctrl Pts',(-41.1175532330596,-25.4712148539422,
0.));
#78578=CARTESIAN_POINT('Ctrl Pts',(-41.1175532330596,-25.4712148539422,
20.));
#78579=CARTESIAN_POINT('Ctrl Pts',(-41.132595736712,-25.4411576596529,0.));
#78580=CARTESIAN_POINT('Ctrl Pts',(-41.132595736712,-25.4411576596529,20.));
#78581=CARTESIAN_POINT('Ctrl Pts',(-41.1476169346881,-25.4110910604425,
0.));
#78582=CARTESIAN_POINT('Ctrl Pts',(-41.1476169346881,-25.4110910604425,
20.));
#78583=CARTESIAN_POINT('Ctrl Pts',(-41.1626168205634,-25.3810150710984,
0.));
#78584=CARTESIAN_POINT('Ctrl Pts',(-41.1626168205634,-25.3810150710984,
20.));
#78585=CARTESIAN_POINT('Ctrl Pts',(-41.1775953879232,-25.3509297064131,
0.));
#78586=CARTESIAN_POINT('Ctrl Pts',(-41.1775953879232,-25.3509297064131,
20.));
#78587=CARTESIAN_POINT('Ctrl Pts',(-41.1925526303629,-25.3208349811839,
0.));
#78588=CARTESIAN_POINT('Ctrl Pts',(-41.1925526303629,-25.3208349811839,
20.));
#78589=CARTESIAN_POINT('Ctrl Pts',(-41.2074885414881,-25.2907309102128,
0.));
#78590=CARTESIAN_POINT('Ctrl Pts',(-41.2074885414881,-25.2907309102128,
20.));
#78591=CARTESIAN_POINT('Ctrl Pts',(-41.2224031149147,-25.2606175083067,
0.));
#78592=CARTESIAN_POINT('Ctrl Pts',(-41.2224031149147,-25.2606175083067,
20.));
#78593=CARTESIAN_POINT('Ctrl Pts',(-41.2372963442684,-25.2304947902774,
0.));
#78594=CARTESIAN_POINT('Ctrl Pts',(-41.2372963442684,-25.2304947902774,
20.));
#78595=CARTESIAN_POINT('Ctrl Pts',(-41.2521682231854,-25.2003627709414,
0.));
#78596=CARTESIAN_POINT('Ctrl Pts',(-41.2521682231854,-25.2003627709414,
20.));
#78597=CARTESIAN_POINT('Ctrl Pts',(-41.2670187453114,-25.1702214651198,
0.));
#78598=CARTESIAN_POINT('Ctrl Pts',(-41.2670187453114,-25.1702214651198,
20.));
#78599=CARTESIAN_POINT('Ctrl Pts',(-41.2818479043026,-25.1400708876386,
0.));
#78600=CARTESIAN_POINT('Ctrl Pts',(-41.2818479043026,-25.1400708876386,
20.));
#78601=CARTESIAN_POINT('Ctrl Pts',(-41.2966556938255,-25.1099110533288,
0.));
#78602=CARTESIAN_POINT('Ctrl Pts',(-41.2966556938255,-25.1099110533288,
20.));
#78603=CARTESIAN_POINT('Ctrl Pts',(-41.3114421075567,-25.0797419770258,
0.));
#78604=CARTESIAN_POINT('Ctrl Pts',(-41.3114421075567,-25.0797419770258,
20.));
#78605=CARTESIAN_POINT('Ctrl Pts',(-41.3262071391823,-25.0495636735701,
0.));
#78606=CARTESIAN_POINT('Ctrl Pts',(-41.3262071391823,-25.0495636735701,
20.));
#78607=CARTESIAN_POINT('Ctrl Pts',(-41.3409507823989,-25.0193761578067,
0.));
#78608=CARTESIAN_POINT('Ctrl Pts',(-41.3409507823989,-25.0193761578067,
20.));
#78609=CARTESIAN_POINT('Ctrl Pts',(-41.3556730309131,-24.9891794445855,
0.));
#78610=CARTESIAN_POINT('Ctrl Pts',(-41.3556730309131,-24.9891794445855,
20.));
#78611=CARTESIAN_POINT('Ctrl Pts',(-41.3703738784418,-24.9589735487609,
0.));
#78612=CARTESIAN_POINT('Ctrl Pts',(-41.3703738784418,-24.9589735487609,
20.));
#78613=CARTESIAN_POINT('Ctrl Pts',(-41.3850533187123,-24.9287584851923,
0.));
#78614=CARTESIAN_POINT('Ctrl Pts',(-41.3850533187123,-24.9287584851923,
20.));
#78615=CARTESIAN_POINT('Ctrl Pts',(-41.3997113454618,-24.8985342687436,
0.));
#78616=CARTESIAN_POINT('Ctrl Pts',(-41.3997113454618,-24.8985342687436,
20.));
#78617=CARTESIAN_POINT('Ctrl Pts',(-41.4143479524375,-24.8683009142837,
0.));
#78618=CARTESIAN_POINT('Ctrl Pts',(-41.4143479524375,-24.8683009142837,
20.));
#78619=CARTESIAN_POINT('Ctrl Pts',(-41.4289631333969,-24.8380584366858,
0.));
#78620=CARTESIAN_POINT('Ctrl Pts',(-41.4289631333969,-24.8380584366858,
20.));
#78621=CARTESIAN_POINT('Ctrl Pts',(-41.4435568821071,-24.8078068508284,
0.));
#78622=CARTESIAN_POINT('Ctrl Pts',(-41.4435568821071,-24.8078068508284,
20.));
#78623=CARTESIAN_POINT('Ctrl Pts',(-41.4581291923457,-24.7775461715943,
0.));
#78624=CARTESIAN_POINT('Ctrl Pts',(-41.4581291923457,-24.7775461715943,
20.));
#78625=CARTESIAN_POINT('Ctrl Pts',(-41.4726800579006,-24.7472764138709,
0.));
#78626=CARTESIAN_POINT('Ctrl Pts',(-41.4726800579006,-24.7472764138709,
20.));
#78627=CARTESIAN_POINT('Ctrl Pts',(-41.4872094725702,-24.7169975925505,
0.));
#78628=CARTESIAN_POINT('Ctrl Pts',(-41.4872094725702,-24.7169975925505,
20.));
#78629=CARTESIAN_POINT('Ctrl Pts',(-41.5017174301628,-24.68670972253,0.));
#78630=CARTESIAN_POINT('Ctrl Pts',(-41.5017174301628,-24.68670972253,20.));
#78631=CARTESIAN_POINT('Ctrl Pts',(-41.516203924497,-24.6564128187107,0.));
#78632=CARTESIAN_POINT('Ctrl Pts',(-41.516203924497,-24.6564128187107,20.));
#78633=CARTESIAN_POINT('Ctrl Pts',(-41.5306689494012,-24.626106895999,0.));
#78634=CARTESIAN_POINT('Ctrl Pts',(-41.5306689494012,-24.626106895999,20.));
#78635=CARTESIAN_POINT('Ctrl Pts',(-41.545112498714,-24.5957919693057,0.));
#78636=CARTESIAN_POINT('Ctrl Pts',(-41.545112498714,-24.5957919693057,20.));
#78637=CARTESIAN_POINT('Ctrl Pts',(-41.5595345662842,-24.5654680535465,
0.));
#78638=CARTESIAN_POINT('Ctrl Pts',(-41.5595345662842,-24.5654680535465,
20.));
#78639=CARTESIAN_POINT('Ctrl Pts',(-41.5739351459709,-24.5351351636416,
0.));
#78640=CARTESIAN_POINT('Ctrl Pts',(-41.5739351459709,-24.5351351636416,
20.));
#78641=CARTESIAN_POINT('Ctrl Pts',(-41.5883142316433,-24.5047933145158,
0.));
#78642=CARTESIAN_POINT('Ctrl Pts',(-41.5883142316433,-24.5047933145158,
20.));
#78643=CARTESIAN_POINT('Ctrl Pts',(-41.6026718171809,-24.4744425210985,
0.));
#78644=CARTESIAN_POINT('Ctrl Pts',(-41.6026718171809,-24.4744425210985,
20.));
#78645=CARTESIAN_POINT('Ctrl Pts',(-41.6170078964732,-24.4440827983238,
0.));
#78646=CARTESIAN_POINT('Ctrl Pts',(-41.6170078964732,-24.4440827983238,
20.));
#78647=CARTESIAN_POINT('Ctrl Pts',(-41.6313224634201,-24.4137141611302,
0.));
#78648=CARTESIAN_POINT('Ctrl Pts',(-41.6313224634201,-24.4137141611302,
20.));
#78649=CARTESIAN_POINT('Ctrl Pts',(-41.6456155119319,-24.3833366244611,
0.));
#78650=CARTESIAN_POINT('Ctrl Pts',(-41.6456155119319,-24.3833366244611,
20.));
#78651=CARTESIAN_POINT('Ctrl Pts',(-41.6598870359289,-24.3529502032644,
0.));
#78652=CARTESIAN_POINT('Ctrl Pts',(-41.6598870359289,-24.3529502032644,
20.));
#78653=CARTESIAN_POINT('Ctrl Pts',(-41.6741370293416,-24.3225549124927,
0.));
#78654=CARTESIAN_POINT('Ctrl Pts',(-41.6741370293416,-24.3225549124927,
20.));
#78655=CARTESIAN_POINT('Ctrl Pts',(-41.6883654861106,-24.2921507671029,
0.));
#78656=CARTESIAN_POINT('Ctrl Pts',(-41.6883654861106,-24.2921507671029,
20.));
#78657=CARTESIAN_POINT('Ctrl Pts',(-41.7025724001866,-24.2617377820568,
0.));
#78658=CARTESIAN_POINT('Ctrl Pts',(-41.7025724001866,-24.2617377820568,
20.));
#78659=CARTESIAN_POINT('Ctrl Pts',(-41.7167577655309,-24.2313159723205,
0.));
#78660=CARTESIAN_POINT('Ctrl Pts',(-41.7167577655309,-24.2313159723205,
20.));
#78661=CARTESIAN_POINT('Ctrl Pts',(-41.7309215761147,-24.2008853528648,
0.));
#78662=CARTESIAN_POINT('Ctrl Pts',(-41.7309215761147,-24.2008853528648,
20.));
#78663=CARTESIAN_POINT('Ctrl Pts',(-41.7450638259196,-24.1704459386651,
0.));
#78664=CARTESIAN_POINT('Ctrl Pts',(-41.7450638259196,-24.1704459386651,
20.));
#78665=CARTESIAN_POINT('Ctrl Pts',(-41.7591845089374,-24.1399977447013,
0.));
#78666=CARTESIAN_POINT('Ctrl Pts',(-41.7591845089374,-24.1399977447013,
20.));
#78667=CARTESIAN_POINT('Ctrl Pts',(-41.7732836191701,-24.1095407859578,
0.));
#78668=CARTESIAN_POINT('Ctrl Pts',(-41.7732836191701,-24.1095407859578,
20.));
#78669=CARTESIAN_POINT('Ctrl Pts',(-41.78736115063,-24.0790750774236,0.));
#78670=CARTESIAN_POINT('Ctrl Pts',(-41.78736115063,-24.0790750774236,20.));
#78671=CARTESIAN_POINT('Ctrl Pts',(-41.8014170973399,-24.0486006340924,
0.));
#78672=CARTESIAN_POINT('Ctrl Pts',(-41.8014170973399,-24.0486006340924,
20.));
#78673=CARTESIAN_POINT('Ctrl Pts',(-41.8154514533324,-24.0181174709622,
0.));
#78674=CARTESIAN_POINT('Ctrl Pts',(-41.8154514533324,-24.0181174709622,
20.));
#78675=CARTESIAN_POINT('Ctrl Pts',(-41.8294642126506,-23.9876256030355,
0.));
#78676=CARTESIAN_POINT('Ctrl Pts',(-41.8294642126506,-23.9876256030355,
20.));
#78677=CARTESIAN_POINT('Ctrl Pts',(-41.8434553693478,-23.9571250453194,
0.));
#78678=CARTESIAN_POINT('Ctrl Pts',(-41.8434553693478,-23.9571250453194,
20.));
#78679=CARTESIAN_POINT('Ctrl Pts',(-41.8574249174873,-23.9266158128252,
0.));
#78680=CARTESIAN_POINT('Ctrl Pts',(-41.8574249174873,-23.9266158128252,
20.));
#78681=CARTESIAN_POINT('Ctrl Pts',(-41.8713728511429,-23.8960979205694,
0.));
#78682=CARTESIAN_POINT('Ctrl Pts',(-41.8713728511429,-23.8960979205694,
20.));
#78683=CARTESIAN_POINT('Ctrl Pts',(-41.8852991643986,-23.8655713835725,
0.));
#78684=CARTESIAN_POINT('Ctrl Pts',(-41.8852991643986,-23.8655713835725,
20.));
#78685=CARTESIAN_POINT('Ctrl Pts',(-41.8992038513488,-23.8350362168598,
0.));
#78686=CARTESIAN_POINT('Ctrl Pts',(-41.8992038513488,-23.8350362168598,
20.));
#78687=CARTESIAN_POINT('Ctrl Pts',(-41.9130869060982,-23.8044924354607,
0.));
#78688=CARTESIAN_POINT('Ctrl Pts',(-41.9130869060982,-23.8044924354607,
20.));
#78689=CARTESIAN_POINT('Ctrl Pts',(-41.9269483227618,-23.7739400544092,
0.));
#78690=CARTESIAN_POINT('Ctrl Pts',(-41.9269483227618,-23.7739400544092,
20.));
#78691=CARTESIAN_POINT('Ctrl Pts',(-41.9407880954647,-23.7433790887435,
0.));
#78692=CARTESIAN_POINT('Ctrl Pts',(-41.9407880954647,-23.7433790887435,
20.));
#78693=CARTESIAN_POINT('Ctrl Pts',(-41.9546062183422,-23.7128095535066,
0.));
#78694=CARTESIAN_POINT('Ctrl Pts',(-41.9546062183422,-23.7128095535066,
20.));
#78695=CARTESIAN_POINT('Ctrl Pts',(-41.9684026855399,-23.6822314637457,
0.));
#78696=CARTESIAN_POINT('Ctrl Pts',(-41.9684026855399,-23.6822314637457,
20.));
#78697=CARTESIAN_POINT('Ctrl Pts',(-41.9821774912142,-23.651644834513,0.));
#78698=CARTESIAN_POINT('Ctrl Pts',(-41.9821774912142,-23.651644834513,20.));
#78699=CARTESIAN_POINT('Ctrl Pts',(-41.9959306295311,-23.6210496808648,
0.));
#78700=CARTESIAN_POINT('Ctrl Pts',(-41.9959306295311,-23.6210496808648,
20.));
#78701=CARTESIAN_POINT('Ctrl Pts',(-42.0096620946675,-23.5904460178619,
0.));
#78702=CARTESIAN_POINT('Ctrl Pts',(-42.0096620946675,-23.5904460178619,
20.));
#78703=CARTESIAN_POINT('Ctrl Pts',(-42.02337188081,-23.5598338605694,0.));
#78704=CARTESIAN_POINT('Ctrl Pts',(-42.02337188081,-23.5598338605694,20.));
#78705=CARTESIAN_POINT('Ctrl Pts',(-42.0370599821558,-23.5292132240566,
0.));
#78706=CARTESIAN_POINT('Ctrl Pts',(-42.0370599821558,-23.5292132240566,
20.));
#78707=CARTESIAN_POINT('Ctrl Pts',(-42.0507263929126,-23.4985841233977,
0.));
#78708=CARTESIAN_POINT('Ctrl Pts',(-42.0507263929126,-23.4985841233977,
20.));
#78709=CARTESIAN_POINT('Ctrl Pts',(-42.0643711072981,-23.4679465736707,
0.));
#78710=CARTESIAN_POINT('Ctrl Pts',(-42.0643711072981,-23.4679465736707,
20.));
#78711=CARTESIAN_POINT('Ctrl Pts',(-42.0779941195407,-23.4373005899585,
0.));
#78712=CARTESIAN_POINT('Ctrl Pts',(-42.0779941195407,-23.4373005899585,
20.));
#78713=CARTESIAN_POINT('Ctrl Pts',(-42.0915954238788,-23.4066461873484,
0.));
#78714=CARTESIAN_POINT('Ctrl Pts',(-42.0915954238788,-23.4066461873484,
20.));
#78715=CARTESIAN_POINT('Ctrl Pts',(-42.1051750145614,-23.3759833809318,
0.));
#78716=CARTESIAN_POINT('Ctrl Pts',(-42.1051750145614,-23.3759833809318,
20.));
#78717=CARTESIAN_POINT('Ctrl Pts',(-42.1187328858474,-23.3453121858047,
0.));
#78718=CARTESIAN_POINT('Ctrl Pts',(-42.1187328858474,-23.3453121858047,
20.));
#78719=CARTESIAN_POINT('Ctrl Pts',(-42.1322690320059,-23.3146326170671,
0.));
#78720=CARTESIAN_POINT('Ctrl Pts',(-42.1322690320059,-23.3146326170671,
20.));
#78721=CARTESIAN_POINT('Ctrl Pts',(-42.145783447317,-23.2839446898238,0.));
#78722=CARTESIAN_POINT('Ctrl Pts',(-42.145783447317,-23.2839446898238,20.));
#78723=CARTESIAN_POINT('Ctrl Pts',(-42.1592761260708,-23.2532484191837,
0.));
#78724=CARTESIAN_POINT('Ctrl Pts',(-42.1592761260708,-23.2532484191837,
20.));
#78725=CARTESIAN_POINT('Ctrl Pts',(-42.1727470625681,-23.2225438202604,
0.));
#78726=CARTESIAN_POINT('Ctrl Pts',(-42.1727470625681,-23.2225438202604,
20.));
#78727=CARTESIAN_POINT('Ctrl Pts',(-42.1861962511195,-23.1918309081713,
0.));
#78728=CARTESIAN_POINT('Ctrl Pts',(-42.1861962511195,-23.1918309081713,
20.));
#78729=CARTESIAN_POINT('Ctrl Pts',(-42.1996236860461,-23.1611096980384,
0.));
#78730=CARTESIAN_POINT('Ctrl Pts',(-42.1996236860461,-23.1611096980384,
20.));
#78731=CARTESIAN_POINT('Ctrl Pts',(-42.2130293616794,-23.1303802049881,
0.));
#78732=CARTESIAN_POINT('Ctrl Pts',(-42.2130293616794,-23.1303802049881,
20.));
#78733=CARTESIAN_POINT('Ctrl Pts',(-42.2264132723612,-23.0996424441509,
0.));
#78734=CARTESIAN_POINT('Ctrl Pts',(-42.2264132723612,-23.0996424441509,
20.));
#78735=CARTESIAN_POINT('Ctrl Pts',(-42.2397754124437,-23.0688964306618,
0.));
#78736=CARTESIAN_POINT('Ctrl Pts',(-42.2397754124437,-23.0688964306618,
20.));
#78737=CARTESIAN_POINT('Ctrl Pts',(-42.2531157762897,-23.0381421796601,
0.));
#78738=CARTESIAN_POINT('Ctrl Pts',(-42.2531157762897,-23.0381421796601,
20.));
#78739=CARTESIAN_POINT('Ctrl Pts',(-42.2664343582719,-23.0073797062893,
0.));
#78740=CARTESIAN_POINT('Ctrl Pts',(-42.2664343582719,-23.0073797062893,
20.));
#78741=CARTESIAN_POINT('Ctrl Pts',(-42.2797311527738,-22.9766090256973,
0.));
#78742=CARTESIAN_POINT('Ctrl Pts',(-42.2797311527738,-22.9766090256973,
20.));
#78743=CARTESIAN_POINT('Ctrl Pts',(-42.2930061541893,-22.9458301530364,
0.));
#78744=CARTESIAN_POINT('Ctrl Pts',(-42.2930061541893,-22.9458301530364,
20.));
#78745=CARTESIAN_POINT('Ctrl Pts',(-42.3062593569226,-22.9150431034629,
0.));
#78746=CARTESIAN_POINT('Ctrl Pts',(-42.3062593569226,-22.9150431034629,
20.));
#78747=CARTESIAN_POINT('Ctrl Pts',(-42.3194907553882,-22.8842478921374,
0.));
#78748=CARTESIAN_POINT('Ctrl Pts',(-42.3194907553882,-22.8842478921374,
20.));
#78749=CARTESIAN_POINT('Ctrl Pts',(-42.3327003440109,-22.8534445342249,
0.));
#78750=CARTESIAN_POINT('Ctrl Pts',(-42.3327003440109,-22.8534445342249,
20.));
#78751=CARTESIAN_POINT('Ctrl Pts',(-42.3458881172255,-22.8226330448945,
0.));
#78752=CARTESIAN_POINT('Ctrl Pts',(-42.3458881172255,-22.8226330448945,
20.));
#78753=CARTESIAN_POINT('Ctrl Pts',(-42.3590540694774,-22.7918134393197,
0.));
#78754=CARTESIAN_POINT('Ctrl Pts',(-42.3590540694774,-22.7918134393197,
20.));
#78755=CARTESIAN_POINT('Ctrl Pts',(-42.3721981952224,-22.7609857326781,
0.));
#78756=CARTESIAN_POINT('Ctrl Pts',(-42.3721981952224,-22.7609857326781,
20.));
#78757=CARTESIAN_POINT('Ctrl Pts',(-42.3853204889273,-22.7301499401517,
0.));
#78758=CARTESIAN_POINT('Ctrl Pts',(-42.3853204889273,-22.7301499401517,
20.));
#78759=CARTESIAN_POINT('Ctrl Pts',(-42.398420945069,-22.6993060769268,0.));
#78760=CARTESIAN_POINT('Ctrl Pts',(-42.398420945069,-22.6993060769268,20.));
#78761=CARTESIAN_POINT('Ctrl Pts',(-42.411499558135,-22.6684541581936,0.));
#78762=CARTESIAN_POINT('Ctrl Pts',(-42.411499558135,-22.6684541581936,20.));
#78763=CARTESIAN_POINT('Ctrl Pts',(-42.4245563226236,-22.6375941991468,
0.));
#78764=CARTESIAN_POINT('Ctrl Pts',(-42.4245563226236,-22.6375941991468,
20.));
#78765=CARTESIAN_POINT('Ctrl Pts',(-42.4375912330427,-22.6067262149851,
0.));
#78766=CARTESIAN_POINT('Ctrl Pts',(-42.4375912330427,-22.6067262149851,
20.));
#78767=CARTESIAN_POINT('Ctrl Pts',(-42.4506042839107,-22.5758502209116,
0.));
#78768=CARTESIAN_POINT('Ctrl Pts',(-42.4506042839107,-22.5758502209116,
20.));
#78769=CARTESIAN_POINT('Ctrl Pts',(-42.4635954697559,-22.5449662321334,
0.));
#78770=CARTESIAN_POINT('Ctrl Pts',(-42.4635954697559,-22.5449662321334,
20.));
#78771=CARTESIAN_POINT('Ctrl Pts',(-42.4765647851171,-22.5140742638619,
0.));
#78772=CARTESIAN_POINT('Ctrl Pts',(-42.4765647851171,-22.5140742638619,
20.));
#78773=CARTESIAN_POINT('Ctrl Pts',(-42.4895122245441,-22.4831743313126,
0.));
#78774=CARTESIAN_POINT('Ctrl Pts',(-42.4895122245441,-22.4831743313126,
20.));
#78775=CARTESIAN_POINT('Ctrl Pts',(-42.502437782597,-22.4522664497054,0.));
#78776=CARTESIAN_POINT('Ctrl Pts',(-42.502437782597,-22.4522664497054,20.));
#78777=CARTESIAN_POINT('Ctrl Pts',(-42.5153414538467,-22.4213506342639,
0.));
#78778=CARTESIAN_POINT('Ctrl Pts',(-42.5153414538467,-22.4213506342639,
20.));
#78779=CARTESIAN_POINT('Ctrl Pts',(-42.5282232328748,-22.3904269002165,
0.));
#78780=CARTESIAN_POINT('Ctrl Pts',(-42.5282232328748,-22.3904269002165,
20.));
#78781=CARTESIAN_POINT('Ctrl Pts',(-42.5410831142727,-22.3594952627952,
0.));
#78782=CARTESIAN_POINT('Ctrl Pts',(-42.5410831142727,-22.3594952627952,
20.));
#78783=CARTESIAN_POINT('Ctrl Pts',(-42.5539210926424,-22.3285557372364,
0.));
#78784=CARTESIAN_POINT('Ctrl Pts',(-42.5539210926424,-22.3285557372364,
20.));
#78785=CARTESIAN_POINT('Ctrl Pts',(-42.5667371625962,-22.2976083387805,
0.));
#78786=CARTESIAN_POINT('Ctrl Pts',(-42.5667371625962,-22.2976083387805,
20.));
#78787=CARTESIAN_POINT('Ctrl Pts',(-42.5795313187569,-22.2666530826722,
0.));
#78788=CARTESIAN_POINT('Ctrl Pts',(-42.5795313187569,-22.2666530826722,
20.));
#78789=CARTESIAN_POINT('Ctrl Pts',(-42.5923035557573,-22.2356899841602,
0.));
#78790=CARTESIAN_POINT('Ctrl Pts',(-42.5923035557573,-22.2356899841602,
20.));
#78791=CARTESIAN_POINT('Ctrl Pts',(-42.6050538682411,-22.2047190584974,
0.));
#78792=CARTESIAN_POINT('Ctrl Pts',(-42.6050538682411,-22.2047190584974,
20.));
#78793=CARTESIAN_POINT('Ctrl Pts',(-42.6177822508627,-22.1737403209406,
0.));
#78794=CARTESIAN_POINT('Ctrl Pts',(-42.6177822508627,-22.1737403209406,
20.));
#78795=CARTESIAN_POINT('Ctrl Pts',(-42.6304886982869,-22.1427537867512,
0.));
#78796=CARTESIAN_POINT('Ctrl Pts',(-42.6304886982869,-22.1427537867512,
20.));
#78797=CARTESIAN_POINT('Ctrl Pts',(-42.6431732051887,-22.1117594711942,
0.));
#78798=CARTESIAN_POINT('Ctrl Pts',(-42.6431732051887,-22.1117594711942,
20.));
#78799=CARTESIAN_POINT('Ctrl Pts',(-42.6558357662536,-22.0807573895388,
0.));
#78800=CARTESIAN_POINT('Ctrl Pts',(-42.6558357662536,-22.0807573895388,
20.));
#78801=CARTESIAN_POINT('Ctrl Pts',(-42.6684763761777,-22.0497475570584,
0.));
#78802=CARTESIAN_POINT('Ctrl Pts',(-42.6684763761777,-22.0497475570584,
20.));
#78803=CARTESIAN_POINT('Ctrl Pts',(-42.6810950296678,-22.0187299890302,
0.));
#78804=CARTESIAN_POINT('Ctrl Pts',(-42.6810950296678,-22.0187299890302,
20.));
#78805=CARTESIAN_POINT('Ctrl Pts',(-42.6936917214411,-21.9877047007357,
0.));
#78806=CARTESIAN_POINT('Ctrl Pts',(-42.6936917214411,-21.9877047007357,
20.));
#78807=CARTESIAN_POINT('Ctrl Pts',(-42.7062664462249,-21.9566717074606,
0.));
#78808=CARTESIAN_POINT('Ctrl Pts',(-42.7062664462249,-21.9566717074606,
20.));
#78809=CARTESIAN_POINT('Ctrl Pts',(-42.7188191987573,-21.9256310244944,
0.));
#78810=CARTESIAN_POINT('Ctrl Pts',(-42.7188191987573,-21.9256310244944,
20.));
#78811=CARTESIAN_POINT('Ctrl Pts',(-42.7313499737866,-21.8945826671308,
0.));
#78812=CARTESIAN_POINT('Ctrl Pts',(-42.7313499737866,-21.8945826671308,
20.));
#78813=CARTESIAN_POINT('Ctrl Pts',(-42.7438587660714,-21.8635266506674,
0.));
#78814=CARTESIAN_POINT('Ctrl Pts',(-42.7438587660714,-21.8635266506674,
20.));
#78815=CARTESIAN_POINT('Ctrl Pts',(-42.7563455703812,-21.832462990406,0.));
#78816=CARTESIAN_POINT('Ctrl Pts',(-42.7563455703812,-21.832462990406,20.));
#78817=CARTESIAN_POINT('Ctrl Pts',(-42.7688103814962,-21.8013917016521,
0.));
#78818=CARTESIAN_POINT('Ctrl Pts',(-42.7688103814962,-21.8013917016521,
20.));
#78819=CARTESIAN_POINT('Ctrl Pts',(-42.7812531942069,-21.7703127997157,
0.));
#78820=CARTESIAN_POINT('Ctrl Pts',(-42.7812531942069,-21.7703127997157,
20.));
#78821=CARTESIAN_POINT('Ctrl Pts',(-42.7936740033148,-21.7392262999104,
0.));
#78822=CARTESIAN_POINT('Ctrl Pts',(-42.7936740033148,-21.7392262999104,
20.));
#78823=CARTESIAN_POINT('Ctrl Pts',(-42.8060728036314,-21.7081322175539,
0.));
#78824=CARTESIAN_POINT('Ctrl Pts',(-42.8060728036314,-21.7081322175539,
20.));
#78825=CARTESIAN_POINT('Ctrl Pts',(-42.8184495899785,-21.677030567968,0.));
#78826=CARTESIAN_POINT('Ctrl Pts',(-42.8184495899785,-21.677030567968,20.));
#78827=CARTESIAN_POINT('Ctrl Pts',(-42.8308043571887,-21.6459213664784,
0.));
#78828=CARTESIAN_POINT('Ctrl Pts',(-42.8308043571887,-21.6459213664784,
20.));
#78829=CARTESIAN_POINT('Ctrl Pts',(-42.8431371001047,-21.6148046284149,
0.));
#78830=CARTESIAN_POINT('Ctrl Pts',(-42.8431371001047,-21.6148046284149,
20.));
#78831=CARTESIAN_POINT('Ctrl Pts',(-42.8554478135801,-21.5836803691112,
0.));
#78832=CARTESIAN_POINT('Ctrl Pts',(-42.8554478135801,-21.5836803691112,
20.));
#78833=CARTESIAN_POINT('Ctrl Pts',(-42.8677364924794,-21.5525486039049,
0.));
#78834=CARTESIAN_POINT('Ctrl Pts',(-42.8677364924794,-21.5525486039049,
20.));
#78835=CARTESIAN_POINT('Ctrl Pts',(-42.8800031316769,-21.5214093481377,
0.));
#78836=CARTESIAN_POINT('Ctrl Pts',(-42.8800031316769,-21.5214093481377,
20.));
#78837=CARTESIAN_POINT('Ctrl Pts',(-42.8922477260581,-21.490262617155,0.));
#78838=CARTESIAN_POINT('Ctrl Pts',(-42.8922477260581,-21.490262617155,20.));
#78839=CARTESIAN_POINT('Ctrl Pts',(-42.9044702705183,-21.4591084263065,
0.));
#78840=CARTESIAN_POINT('Ctrl Pts',(-42.9044702705183,-21.4591084263065,
20.));
#78841=CARTESIAN_POINT('Ctrl Pts',(-42.916670759964,-21.4279467909454,0.));
#78842=CARTESIAN_POINT('Ctrl Pts',(-42.916670759964,-21.4279467909454,20.));
#78843=CARTESIAN_POINT('Ctrl Pts',(-42.9288491893122,-21.3967777264294,
0.));
#78844=CARTESIAN_POINT('Ctrl Pts',(-42.9288491893122,-21.3967777264294,
20.));
#78845=CARTESIAN_POINT('Ctrl Pts',(-42.9410055534907,-21.3656012481198,
0.));
#78846=CARTESIAN_POINT('Ctrl Pts',(-42.9410055534907,-21.3656012481198,
20.));
#78847=CARTESIAN_POINT('Ctrl Pts',(-42.9531398474371,-21.3344173713818,
0.));
#78848=CARTESIAN_POINT('Ctrl Pts',(-42.9531398474371,-21.3344173713818,
20.));
#78849=CARTESIAN_POINT('Ctrl Pts',(-42.9652520660998,-21.3032261115844,
0.));
#78850=CARTESIAN_POINT('Ctrl Pts',(-42.9652520660998,-21.3032261115844,
20.));
#78851=CARTESIAN_POINT('Ctrl Pts',(-42.9773422044374,-21.2720274841006,
0.));
#78852=CARTESIAN_POINT('Ctrl Pts',(-42.9773422044374,-21.2720274841006,
20.));
#78853=CARTESIAN_POINT('Ctrl Pts',(-42.9894102574195,-21.2408215043074,
0.));
#78854=CARTESIAN_POINT('Ctrl Pts',(-42.9894102574195,-21.2408215043074,
20.));
#78855=CARTESIAN_POINT('Ctrl Pts',(-43.0014562200264,-21.2096081875857,
0.));
#78856=CARTESIAN_POINT('Ctrl Pts',(-43.0014562200264,-21.2096081875857,
20.));
#78857=CARTESIAN_POINT('Ctrl Pts',(-43.0134800872489,-21.1783875493204,
0.));
#78858=CARTESIAN_POINT('Ctrl Pts',(-43.0134800872489,-21.1783875493204,
20.));
#78859=CARTESIAN_POINT('Ctrl Pts',(-43.0254818540885,-21.1471596049,0.));
#78860=CARTESIAN_POINT('Ctrl Pts',(-43.0254818540885,-21.1471596049,20.));
#78861=CARTESIAN_POINT('Ctrl Pts',(-43.037461515557,-21.1159243697169,0.));
#78862=CARTESIAN_POINT('Ctrl Pts',(-43.037461515557,-21.1159243697169,20.));
#78863=CARTESIAN_POINT('Ctrl Pts',(-43.0494190666771,-21.0846818591673,
0.));
#78864=CARTESIAN_POINT('Ctrl Pts',(-43.0494190666771,-21.0846818591673,
20.));
#78865=CARTESIAN_POINT('Ctrl Pts',(-43.0613545024815,-21.0534320886512,
0.));
#78866=CARTESIAN_POINT('Ctrl Pts',(-43.0613545024815,-21.0534320886512,
20.));
#78867=CARTESIAN_POINT('Ctrl Pts',(-43.0732678180139,-21.0221750735727,
0.));
#78868=CARTESIAN_POINT('Ctrl Pts',(-43.0732678180139,-21.0221750735727,
20.));
#78869=CARTESIAN_POINT('Ctrl Pts',(-43.0851590083283,-20.9909108293397,
0.));
#78870=CARTESIAN_POINT('Ctrl Pts',(-43.0851590083283,-20.9909108293397,
20.));
#78871=CARTESIAN_POINT('Ctrl Pts',(-43.0970280684896,-20.959639371364,0.));
#78872=CARTESIAN_POINT('Ctrl Pts',(-43.0970280684896,-20.959639371364,20.));
#78873=CARTESIAN_POINT('Ctrl Pts',(-43.1088749935734,-20.9283607150615,
0.));
#78874=CARTESIAN_POINT('Ctrl Pts',(-43.1088749935734,-20.9283607150615,
20.));
#78875=CARTESIAN_POINT('Ctrl Pts',(-43.1206997786657,-20.8970748758512,
0.));
#78876=CARTESIAN_POINT('Ctrl Pts',(-43.1206997786657,-20.8970748758512,
20.));
#78877=CARTESIAN_POINT('Ctrl Pts',(-43.132502418863,-20.8657818691565,0.));
#78878=CARTESIAN_POINT('Ctrl Pts',(-43.132502418863,-20.8657818691565,20.));
#78879=CARTESIAN_POINT('Ctrl Pts',(-43.1442829092724,-20.8344817104039,
0.));
#78880=CARTESIAN_POINT('Ctrl Pts',(-43.1442829092724,-20.8344817104039,
20.));
#78881=CARTESIAN_POINT('Ctrl Pts',(-43.1560412450117,-20.8031744150242,
0.));
#78882=CARTESIAN_POINT('Ctrl Pts',(-43.1560412450117,-20.8031744150242,
20.));
#78883=CARTESIAN_POINT('Ctrl Pts',(-43.1677774212093,-20.7718599984518,
0.));
#78884=CARTESIAN_POINT('Ctrl Pts',(-43.1677774212093,-20.7718599984518,
20.));
#78885=CARTESIAN_POINT('Ctrl Pts',(-43.1794914330045,-20.7405384761252,
0.));
#78886=CARTESIAN_POINT('Ctrl Pts',(-43.1794914330045,-20.7405384761252,
20.));
#78887=CARTESIAN_POINT('Ctrl Pts',(-43.1911832755467,-20.7092098634864,
0.));
#78888=CARTESIAN_POINT('Ctrl Pts',(-43.1911832755467,-20.7092098634864,
20.));
#78889=CARTESIAN_POINT('Ctrl Pts',(-43.202852943996,-20.6778741759814,0.));
#78890=CARTESIAN_POINT('Ctrl Pts',(-43.202852943996,-20.6778741759814,20.));
#78891=CARTESIAN_POINT('Ctrl Pts',(-43.2145004335236,-20.6465314290598,
0.));
#78892=CARTESIAN_POINT('Ctrl Pts',(-43.2145004335236,-20.6465314290598,
20.));
#78893=CARTESIAN_POINT('Ctrl Pts',(-43.2261257393109,-20.615181638175,0.));
#78894=CARTESIAN_POINT('Ctrl Pts',(-43.2261257393109,-20.615181638175,20.));
#78895=CARTESIAN_POINT('Ctrl Pts',(-43.2377288565503,-20.5838248187841,
0.));
#78896=CARTESIAN_POINT('Ctrl Pts',(-43.2377288565503,-20.5838248187841,
20.));
#78897=CARTESIAN_POINT('Ctrl Pts',(-43.2493097804445,-20.5524609863481,
0.));
#78898=CARTESIAN_POINT('Ctrl Pts',(-43.2493097804445,-20.5524609863481,
20.));
#78899=CARTESIAN_POINT('Ctrl Pts',(-43.2608685062069,-20.5210901563314,
0.));
#78900=CARTESIAN_POINT('Ctrl Pts',(-43.2608685062069,-20.5210901563314,
20.));
#78901=CARTESIAN_POINT('Ctrl Pts',(-43.2724050290617,-20.4897123442023,
0.));
#78902=CARTESIAN_POINT('Ctrl Pts',(-43.2724050290617,-20.4897123442023,
20.));
#78903=CARTESIAN_POINT('Ctrl Pts',(-43.283919344243,-20.4583275654327,0.));
#78904=CARTESIAN_POINT('Ctrl Pts',(-43.283919344243,-20.4583275654327,20.));
#78905=CARTESIAN_POINT('Ctrl Pts',(-43.2954114469964,-20.4269358354984,
0.));
#78906=CARTESIAN_POINT('Ctrl Pts',(-43.2954114469964,-20.4269358354984,
20.));
#78907=CARTESIAN_POINT('Ctrl Pts',(-43.3068813325774,-20.3955371698787,
0.));
#78908=CARTESIAN_POINT('Ctrl Pts',(-43.3068813325774,-20.3955371698787,
20.));
#78909=CARTESIAN_POINT('Ctrl Pts',(-43.3183289962528,-20.3641315840566,
0.));
#78910=CARTESIAN_POINT('Ctrl Pts',(-43.3183289962528,-20.3641315840566,
20.));
#78911=CARTESIAN_POINT('Ctrl Pts',(-43.3297544333003,-20.3327190935193,
0.));
#78912=CARTESIAN_POINT('Ctrl Pts',(-43.3297544333003,-20.3327190935193,
20.));
#78913=CARTESIAN_POINT('Ctrl Pts',(-43.3411576390085,-20.3012997137575,
0.));
#78914=CARTESIAN_POINT('Ctrl Pts',(-43.3411576390085,-20.3012997137575,
20.));
#78915=CARTESIAN_POINT('Ctrl Pts',(-43.3525386086763,-20.2698734602656,
0.));
#78916=CARTESIAN_POINT('Ctrl Pts',(-43.3525386086763,-20.2698734602656,
20.));
#78917=CARTESIAN_POINT('Ctrl Pts',(-43.3638973376125,-20.2384403485411,
0.));
#78918=CARTESIAN_POINT('Ctrl Pts',(-43.3638973376125,-20.2384403485411,
20.));
#78919=CARTESIAN_POINT('Ctrl Pts',(-43.3752338211368,-20.2070003940853,
0.));
#78920=CARTESIAN_POINT('Ctrl Pts',(-43.3752338211368,-20.2070003940853,
20.));
#78921=CARTESIAN_POINT('Ctrl Pts',(-43.3865480545792,-20.1755536124033,
0.));
#78922=CARTESIAN_POINT('Ctrl Pts',(-43.3865480545792,-20.1755536124033,
20.));
#78923=CARTESIAN_POINT('Ctrl Pts',(-43.3978400332808,-20.1441000190037,
0.));
#78924=CARTESIAN_POINT('Ctrl Pts',(-43.3978400332808,-20.1441000190037,
20.));
#78925=CARTESIAN_POINT('Ctrl Pts',(-43.409109752594,-20.1126396293992,0.));
#78926=CARTESIAN_POINT('Ctrl Pts',(-43.409109752594,-20.1126396293992,20.));
#78927=CARTESIAN_POINT('Ctrl Pts',(-43.4203572078819,-20.0811724591058,
0.));
#78928=CARTESIAN_POINT('Ctrl Pts',(-43.4203572078819,-20.0811724591058,
20.));
#78929=CARTESIAN_POINT('Ctrl Pts',(-43.4315823945181,-20.0496985236436,
0.));
#78930=CARTESIAN_POINT('Ctrl Pts',(-43.4315823945181,-20.0496985236436,
20.));
#78931=CARTESIAN_POINT('Ctrl Pts',(-43.4427853078868,-20.0182178385356,
0.));
#78932=CARTESIAN_POINT('Ctrl Pts',(-43.4427853078868,-20.0182178385356,
20.));
#78933=CARTESIAN_POINT('Ctrl Pts',(-43.4539659433821,-19.9867304193089,
0.));
#78934=CARTESIAN_POINT('Ctrl Pts',(-43.4539659433821,-19.9867304193089,
20.));
#78935=CARTESIAN_POINT('Ctrl Pts',(-43.4651242964088,-19.9552362814936,
0.));
#78936=CARTESIAN_POINT('Ctrl Pts',(-43.4651242964088,-19.9552362814936,
20.));
#78937=CARTESIAN_POINT('Ctrl Pts',(-43.4762603623832,-19.923735440624,0.));
#78938=CARTESIAN_POINT('Ctrl Pts',(-43.4762603623832,-19.923735440624,20.));
#78939=CARTESIAN_POINT('Ctrl Pts',(-43.4873741367321,-19.8922279122378,
0.));
#78940=CARTESIAN_POINT('Ctrl Pts',(-43.4873741367321,-19.8922279122378,
20.));
#78941=CARTESIAN_POINT('Ctrl Pts',(-43.4984656148936,-19.8607137118763,
0.));
#78942=CARTESIAN_POINT('Ctrl Pts',(-43.4984656148936,-19.8607137118763,
20.));
#78943=CARTESIAN_POINT('Ctrl Pts',(-43.5095347923164,-19.8291928550844,
0.));
#78944=CARTESIAN_POINT('Ctrl Pts',(-43.5095347923164,-19.8291928550844,
20.));
#78945=CARTESIAN_POINT('Ctrl Pts',(-43.5205816644596,-19.7976653574108,
0.));
#78946=CARTESIAN_POINT('Ctrl Pts',(-43.5205816644596,-19.7976653574108,
20.));
#78947=CARTESIAN_POINT('Ctrl Pts',(-43.5316062267925,-19.7661312344072,
0.));
#78948=CARTESIAN_POINT('Ctrl Pts',(-43.5316062267925,-19.7661312344072,
20.));
#78949=CARTESIAN_POINT('Ctrl Pts',(-43.542608474795,-19.734590501629,0.));
#78950=CARTESIAN_POINT('Ctrl Pts',(-43.542608474795,-19.734590501629,20.));
#78951=CARTESIAN_POINT('Ctrl Pts',(-43.5535884039576,-19.7030431746352,
0.));
#78952=CARTESIAN_POINT('Ctrl Pts',(-43.5535884039576,-19.7030431746352,
20.));
#78953=CARTESIAN_POINT('Ctrl Pts',(-43.5645460097823,-19.6714892689885,
0.));
#78954=CARTESIAN_POINT('Ctrl Pts',(-43.5645460097823,-19.6714892689885,
20.));
#78955=CARTESIAN_POINT('Ctrl Pts',(-43.5754812877819,-19.639928800255,0.));
#78956=CARTESIAN_POINT('Ctrl Pts',(-43.5754812877819,-19.639928800255,20.));
#78957=CARTESIAN_POINT('Ctrl Pts',(-43.5863942334797,-19.6083617840046,
0.));
#78958=CARTESIAN_POINT('Ctrl Pts',(-43.5863942334797,-19.6083617840046,
20.));
#78959=CARTESIAN_POINT('Ctrl Pts',(-43.5972848424097,-19.5767882358104,
0.));
#78960=CARTESIAN_POINT('Ctrl Pts',(-43.5972848424097,-19.5767882358104,
20.));
#78961=CARTESIAN_POINT('Ctrl Pts',(-43.6081531101168,-19.545208171249,0.));
#78962=CARTESIAN_POINT('Ctrl Pts',(-43.6081531101168,-19.545208171249,20.));
#78963=CARTESIAN_POINT('Ctrl Pts',(-43.6189990321561,-19.5136216059004,
0.));
#78964=CARTESIAN_POINT('Ctrl Pts',(-43.6189990321561,-19.5136216059004,
20.));
#78965=CARTESIAN_POINT('Ctrl Pts',(-43.629822604094,-19.4820285553483,0.));
#78966=CARTESIAN_POINT('Ctrl Pts',(-43.629822604094,-19.4820285553483,20.));
#78967=CARTESIAN_POINT('Ctrl Pts',(-43.6406238215078,-19.4504290351799,
0.));
#78968=CARTESIAN_POINT('Ctrl Pts',(-43.6406238215078,-19.4504290351799,
20.));
#78969=CARTESIAN_POINT('Ctrl Pts',(-43.6514026799849,-19.4188230609858,
0.));
#78970=CARTESIAN_POINT('Ctrl Pts',(-43.6514026799849,-19.4188230609858,
20.));
#78971=CARTESIAN_POINT('Ctrl Pts',(-43.6621591751234,-19.3872106483603,
0.));
#78972=CARTESIAN_POINT('Ctrl Pts',(-43.6621591751234,-19.3872106483603,
20.));
#78973=CARTESIAN_POINT('Ctrl Pts',(-43.6728933025325,-19.3555918129009,
0.));
#78974=CARTESIAN_POINT('Ctrl Pts',(-43.6728933025325,-19.3555918129009,
20.));
#78975=CARTESIAN_POINT('Ctrl Pts',(-43.6836050578319,-19.3239665702086,
0.));
#78976=CARTESIAN_POINT('Ctrl Pts',(-43.6836050578319,-19.3239665702086,
20.));
#78977=CARTESIAN_POINT('Ctrl Pts',(-43.6942944366523,-19.2923349358879,
0.));
#78978=CARTESIAN_POINT('Ctrl Pts',(-43.6942944366523,-19.2923349358879,
20.));
#78979=CARTESIAN_POINT('Ctrl Pts',(-43.7049614346349,-19.2606969255464,
0.));
#78980=CARTESIAN_POINT('Ctrl Pts',(-43.7049614346349,-19.2606969255464,
20.));
#78981=CARTESIAN_POINT('Ctrl Pts',(-43.7156060474324,-19.2290525547956,
0.));
#78982=CARTESIAN_POINT('Ctrl Pts',(-43.7156060474324,-19.2290525547956,
20.));
#78983=CARTESIAN_POINT('Ctrl Pts',(-43.7262282707082,-19.1974018392505,
0.));
#78984=CARTESIAN_POINT('Ctrl Pts',(-43.7262282707082,-19.1974018392505,
20.));
#78985=CARTESIAN_POINT('Ctrl Pts',(-43.7368281001363,-19.1657447945291,
0.));
#78986=CARTESIAN_POINT('Ctrl Pts',(-43.7368281001363,-19.1657447945291,
20.));
#78987=CARTESIAN_POINT('Ctrl Pts',(-43.747405531401,-19.1340814362531,0.));
#78988=CARTESIAN_POINT('Ctrl Pts',(-43.747405531401,-19.1340814362531,20.));
#78989=CARTESIAN_POINT('Ctrl Pts',(-43.7579605601976,-19.1024117800474,
0.));
#78990=CARTESIAN_POINT('Ctrl Pts',(-43.7579605601976,-19.1024117800474,
20.));
#78991=CARTESIAN_POINT('Ctrl Pts',(-43.7684931822314,-19.0707358415405,
0.));
#78992=CARTESIAN_POINT('Ctrl Pts',(-43.7684931822314,-19.0707358415405,
20.));
#78993=CARTESIAN_POINT('Ctrl Pts',(-43.779003393219,-19.039053636364,0.));
#78994=CARTESIAN_POINT('Ctrl Pts',(-43.779003393219,-19.039053636364,20.));
#78995=CARTESIAN_POINT('Ctrl Pts',(-43.7894911888877,-19.0073651801531,
0.));
#78996=CARTESIAN_POINT('Ctrl Pts',(-43.7894911888877,-19.0073651801531,
20.));
#78997=CARTESIAN_POINT('Ctrl Pts',(-43.7999565649762,-18.9756704885464,
0.));
#78998=CARTESIAN_POINT('Ctrl Pts',(-43.7999565649762,-18.9756704885464,
20.));
#78999=CARTESIAN_POINT('Ctrl Pts',(-43.8103995172341,-18.9439695771858,
0.));
#79000=CARTESIAN_POINT('Ctrl Pts',(-43.8103995172341,-18.9439695771858,
20.));
#79001=CARTESIAN_POINT('Ctrl Pts',(-43.8208200414219,-18.9122624617166,
0.));
#79002=CARTESIAN_POINT('Ctrl Pts',(-43.8208200414219,-18.9122624617166,
20.));
#79003=CARTESIAN_POINT('Ctrl Pts',(-43.8312181333106,-18.8805491577876,
0.));
#79004=CARTESIAN_POINT('Ctrl Pts',(-43.8312181333106,-18.8805491577876,
20.));
#79005=CARTESIAN_POINT('Ctrl Pts',(-43.8415937886817,-18.8488296810507,
0.));
#79006=CARTESIAN_POINT('Ctrl Pts',(-43.8415937886817,-18.8488296810507,
20.));
#79007=CARTESIAN_POINT('Ctrl Pts',(-43.8519470033272,-18.8171040471611,
0.));
#79008=CARTESIAN_POINT('Ctrl Pts',(-43.8519470033272,-18.8171040471611,
20.));
#79009=CARTESIAN_POINT('Ctrl Pts',(-43.8622777730502,-18.7853722717774,
0.));
#79010=CARTESIAN_POINT('Ctrl Pts',(-43.8622777730502,-18.7853722717774,
20.));
#79011=CARTESIAN_POINT('Ctrl Pts',(-43.8725860936644,-18.7536343705616,
0.));
#79012=CARTESIAN_POINT('Ctrl Pts',(-43.8725860936644,-18.7536343705616,
20.));
#79013=CARTESIAN_POINT('Ctrl Pts',(-43.8828719609947,-18.721890359179,0.));
#79014=CARTESIAN_POINT('Ctrl Pts',(-43.8828719609947,-18.721890359179,20.));
#79015=CARTESIAN_POINT('Ctrl Pts',(-43.8931353708767,-18.6901402532984,
0.));
#79016=CARTESIAN_POINT('Ctrl Pts',(-43.8931353708767,-18.6901402532984,
20.));
#79017=CARTESIAN_POINT('Ctrl Pts',(-43.903376319157,-18.6583840685915,0.));
#79018=CARTESIAN_POINT('Ctrl Pts',(-43.903376319157,-18.6583840685915,20.));
#79019=CARTESIAN_POINT('Ctrl Pts',(-43.913594801693,-18.6266218207337,0.));
#79020=CARTESIAN_POINT('Ctrl Pts',(-43.913594801693,-18.6266218207337,20.));
#79021=CARTESIAN_POINT('Ctrl Pts',(-43.9237908143526,-18.5948535254034,
0.));
#79022=CARTESIAN_POINT('Ctrl Pts',(-43.9237908143526,-18.5948535254034,
20.));
#79023=CARTESIAN_POINT('Ctrl Pts',(-43.9339643530151,-18.5630791982821,
0.));
#79024=CARTESIAN_POINT('Ctrl Pts',(-43.9339643530151,-18.5630791982821,
20.));
#79025=CARTESIAN_POINT('Ctrl Pts',(-43.94411541357,-18.5312988550549,0.));
#79026=CARTESIAN_POINT('Ctrl Pts',(-43.94411541357,-18.5312988550549,20.));
#79027=CARTESIAN_POINT('Ctrl Pts',(-43.9542439919177,-18.4995125114099,
0.));
#79028=CARTESIAN_POINT('Ctrl Pts',(-43.9542439919177,-18.4995125114099,
20.));
#79029=CARTESIAN_POINT('Ctrl Pts',(-43.9643500839697,-18.4677201830388,
0.));
#79030=CARTESIAN_POINT('Ctrl Pts',(-43.9643500839697,-18.4677201830388,
20.));
#79031=CARTESIAN_POINT('Ctrl Pts',(-43.9744336856481,-18.4359218856365,
0.));
#79032=CARTESIAN_POINT('Ctrl Pts',(-43.9744336856481,-18.4359218856365,
20.));
#79033=CARTESIAN_POINT('Ctrl Pts',(-43.9844947928861,-18.4041176349014,
0.));
#79034=CARTESIAN_POINT('Ctrl Pts',(-43.9844947928861,-18.4041176349014,
20.));
#79035=CARTESIAN_POINT('Ctrl Pts',(-43.9945334016277,-18.3723074465347,
0.));
#79036=CARTESIAN_POINT('Ctrl Pts',(-43.9945334016277,-18.3723074465347,
20.));
#79037=CARTESIAN_POINT('Ctrl Pts',(-44.0045495078276,-18.3404913362408,
0.));
#79038=CARTESIAN_POINT('Ctrl Pts',(-44.0045495078276,-18.3404913362408,
20.));
#79039=CARTESIAN_POINT('Ctrl Pts',(-44.0145431074514,-18.3086693197275,
0.));
#79040=CARTESIAN_POINT('Ctrl Pts',(-44.0145431074514,-18.3086693197275,
20.));
#79041=CARTESIAN_POINT('Ctrl Pts',(-44.0245141964756,-18.2768414127056,
0.));
#79042=CARTESIAN_POINT('Ctrl Pts',(-44.0245141964756,-18.2768414127056,
20.));
#79043=CARTESIAN_POINT('Ctrl Pts',(-44.0344627708874,-18.2450076308889,
0.));
#79044=CARTESIAN_POINT('Ctrl Pts',(-44.0344627708874,-18.2450076308889,
20.));
#79045=CARTESIAN_POINT('Ctrl Pts',(-44.044388826685,-18.2131679899948,0.));
#79046=CARTESIAN_POINT('Ctrl Pts',(-44.044388826685,-18.2131679899948,20.));
#79047=CARTESIAN_POINT('Ctrl Pts',(-44.0542923598773,-18.1813225057438,
0.));
#79048=CARTESIAN_POINT('Ctrl Pts',(-44.0542923598773,-18.1813225057438,
20.));
#79049=CARTESIAN_POINT('Ctrl Pts',(-44.0641733664839,-18.1494711938598,
0.));
#79050=CARTESIAN_POINT('Ctrl Pts',(-44.0641733664839,-18.1494711938598,
20.));
#79051=CARTESIAN_POINT('Ctrl Pts',(-44.0740318425361,-18.1176140700699,
0.));
#79052=CARTESIAN_POINT('Ctrl Pts',(-44.0740318425361,-18.1176140700699,
20.));
#79053=CARTESIAN_POINT('Ctrl Pts',(-44.0838677840754,-18.0857511501043,
0.));
#79054=CARTESIAN_POINT('Ctrl Pts',(-44.0838677840754,-18.0857511501043,
20.));
#79055=CARTESIAN_POINT('Ctrl Pts',(-44.0936811871546,-18.0538824496962,
0.));
#79056=CARTESIAN_POINT('Ctrl Pts',(-44.0936811871546,-18.0538824496962,
20.));
#79057=CARTESIAN_POINT('Ctrl Pts',(-44.1034720478372,-18.0220079845822,
0.));
#79058=CARTESIAN_POINT('Ctrl Pts',(-44.1034720478372,-18.0220079845822,
20.));
#79059=CARTESIAN_POINT('Ctrl Pts',(-44.1132403621971,-17.9901277705015,
0.));
#79060=CARTESIAN_POINT('Ctrl Pts',(-44.1132403621971,-17.9901277705015,
20.));
#79061=CARTESIAN_POINT('Ctrl Pts',(-44.1229861263191,-17.9582418231966,
0.));
#79062=CARTESIAN_POINT('Ctrl Pts',(-44.1229861263191,-17.9582418231966,
20.));
#79063=CARTESIAN_POINT('Ctrl Pts',(-44.1327093362991,-17.9263501584131,
0.));
#79064=CARTESIAN_POINT('Ctrl Pts',(-44.1327093362991,-17.9263501584131,
20.));
#79065=CARTESIAN_POINT('Ctrl Pts',(-44.142409988244,-17.8944527919,0.));
#79066=CARTESIAN_POINT('Ctrl Pts',(-44.142409988244,-17.8944527919,20.));
#79067=CARTESIAN_POINT('Ctrl Pts',(-44.1520880782717,-17.8625497394092,
0.));
#79068=CARTESIAN_POINT('Ctrl Pts',(-44.1520880782717,-17.8625497394092,
20.));
#79069=CARTESIAN_POINT('Ctrl Pts',(-44.1617436025112,-17.8306410166963,
0.));
#79070=CARTESIAN_POINT('Ctrl Pts',(-44.1617436025112,-17.8306410166963,
20.));
#79071=CARTESIAN_POINT('Ctrl Pts',(-44.1713765571021,-17.7987266395196,
0.));
#79072=CARTESIAN_POINT('Ctrl Pts',(-44.1713765571021,-17.7987266395196,
20.));
#79073=CARTESIAN_POINT('Ctrl Pts',(-44.1809869381949,-17.7668066236405,
0.));
#79074=CARTESIAN_POINT('Ctrl Pts',(-44.1809869381949,-17.7668066236405,
20.));
#79075=CARTESIAN_POINT('Ctrl Pts',(-44.1905747419505,-17.7348809848234,
0.));
#79076=CARTESIAN_POINT('Ctrl Pts',(-44.1905747419505,-17.7348809848234,
20.));
#79077=CARTESIAN_POINT('Ctrl Pts',(-44.2001399645408,-17.7029497388358,
0.));
#79078=CARTESIAN_POINT('Ctrl Pts',(-44.2001399645408,-17.7029497388358,
20.));
#79079=CARTESIAN_POINT('Ctrl Pts',(-44.2096826021493,-17.6710129014481,
0.));
#79080=CARTESIAN_POINT('Ctrl Pts',(-44.2096826021493,-17.6710129014481,
20.));
#79081=CARTESIAN_POINT('Ctrl Pts',(-44.2192026509705,-17.6390704884341,
0.));
#79082=CARTESIAN_POINT('Ctrl Pts',(-44.2192026509705,-17.6390704884341,
20.));
#79083=CARTESIAN_POINT('Ctrl Pts',(-44.2287001072093,-17.6071225155702,
0.));
#79084=CARTESIAN_POINT('Ctrl Pts',(-44.2287001072093,-17.6071225155702,
20.));
#79085=CARTESIAN_POINT('Ctrl Pts',(-44.2381749670816,-17.5751689986363,
0.));
#79086=CARTESIAN_POINT('Ctrl Pts',(-44.2381749670816,-17.5751689986363,
20.));
#79087=CARTESIAN_POINT('Ctrl Pts',(-44.2476272268138,-17.5432099534151,
0.));
#79088=CARTESIAN_POINT('Ctrl Pts',(-44.2476272268138,-17.5432099534151,
20.));
#79089=CARTESIAN_POINT('Ctrl Pts',(-44.2570568826434,-17.5112453956925,
0.));
#79090=CARTESIAN_POINT('Ctrl Pts',(-44.2570568826434,-17.5112453956925,
20.));
#79091=CARTESIAN_POINT('Ctrl Pts',(-44.2664639308192,-17.4792753412574,
0.));
#79092=CARTESIAN_POINT('Ctrl Pts',(-44.2664639308192,-17.4792753412574,
20.));
#79093=CARTESIAN_POINT('Ctrl Pts',(-44.2758483676008,-17.447299805902,0.));
#79094=CARTESIAN_POINT('Ctrl Pts',(-44.2758483676008,-17.447299805902,20.));
#79095=CARTESIAN_POINT('Ctrl Pts',(-44.2852101892593,-17.4153188054211,
0.));
#79096=CARTESIAN_POINT('Ctrl Pts',(-44.2852101892593,-17.4153188054211,
20.));
#79097=CARTESIAN_POINT('Ctrl Pts',(-44.2945493920761,-17.3833323556128,
0.));
#79098=CARTESIAN_POINT('Ctrl Pts',(-44.2945493920761,-17.3833323556128,
20.));
#79099=CARTESIAN_POINT('Ctrl Pts',(-44.3038659723435,-17.3513404722779,
0.));
#79100=CARTESIAN_POINT('Ctrl Pts',(-44.3038659723435,-17.3513404722779,
20.));
#79101=CARTESIAN_POINT('Ctrl Pts',(-44.3131599263643,-17.3193431712198,
0.));
#79102=CARTESIAN_POINT('Ctrl Pts',(-44.3131599263643,-17.3193431712198,
20.));
#79103=CARTESIAN_POINT('Ctrl Pts',(-44.3224312504523,-17.2873404682456,
0.));
#79104=CARTESIAN_POINT('Ctrl Pts',(-44.3224312504523,-17.2873404682456,
20.));
#79105=CARTESIAN_POINT('Ctrl Pts',(-44.3316799409325,-17.2553323791649,
0.));
#79106=CARTESIAN_POINT('Ctrl Pts',(-44.3316799409325,-17.2553323791649,
20.));
#79107=CARTESIAN_POINT('Ctrl Pts',(-44.340905994141,-17.2233189197905,0.));
#79108=CARTESIAN_POINT('Ctrl Pts',(-44.340905994141,-17.2233189197905,20.));
#79109=CARTESIAN_POINT('Ctrl Pts',(-44.3501094064252,-17.1913001059384,
0.));
#79110=CARTESIAN_POINT('Ctrl Pts',(-44.3501094064252,-17.1913001059384,
20.));
#79111=CARTESIAN_POINT('Ctrl Pts',(-44.3592901741436,-17.1592759534275,
0.));
#79112=CARTESIAN_POINT('Ctrl Pts',(-44.3592901741436,-17.1592759534275,
20.));
#79113=CARTESIAN_POINT('Ctrl Pts',(-44.3684482936655,-17.1272464780797,
0.));
#79114=CARTESIAN_POINT('Ctrl Pts',(-44.3684482936655,-17.1272464780797,
20.));
#79115=CARTESIAN_POINT('Ctrl Pts',(-44.3775837613707,-17.0952116957196,
0.));
#79116=CARTESIAN_POINT('Ctrl Pts',(-44.3775837613707,-17.0952116957196,
20.));
#79117=CARTESIAN_POINT('Ctrl Pts',(-44.3866965736492,-17.0631716221745,
0.));
#79118=CARTESIAN_POINT('Ctrl Pts',(-44.3866965736492,-17.0631716221745,
20.));
#79119=CARTESIAN_POINT('Ctrl Pts',(-44.3957867269024,-17.0311262732746,
0.));
#79120=CARTESIAN_POINT('Ctrl Pts',(-44.3957867269024,-17.0311262732746,
20.));
#79121=CARTESIAN_POINT('Ctrl Pts',(-44.404854217543,-16.9990756648532,0.));
#79122=CARTESIAN_POINT('Ctrl Pts',(-44.404854217543,-16.9990756648532,20.));
#79123=CARTESIAN_POINT('Ctrl Pts',(-44.4138990419958,-16.967019812747,0.));
#79124=CARTESIAN_POINT('Ctrl Pts',(-44.4138990419958,-16.967019812747,20.));
#79125=CARTESIAN_POINT('Ctrl Pts',(-44.4229211966955,-16.9349587327952,
0.));
#79126=CARTESIAN_POINT('Ctrl Pts',(-44.4229211966955,-16.9349587327952,
20.));
#79127=CARTESIAN_POINT('Ctrl Pts',(-44.431920678088,-16.9028924408399,0.));
#79128=CARTESIAN_POINT('Ctrl Pts',(-44.431920678088,-16.9028924408399,20.));
#79129=CARTESIAN_POINT('Ctrl Pts',(-44.4408974826294,-16.870820952726,0.));
#79130=CARTESIAN_POINT('Ctrl Pts',(-44.4408974826294,-16.870820952726,20.));
#79131=CARTESIAN_POINT('Ctrl Pts',(-44.4498516067869,-16.8387442843012,
0.));
#79132=CARTESIAN_POINT('Ctrl Pts',(-44.4498516067869,-16.8387442843012,
20.));
#79133=CARTESIAN_POINT('Ctrl Pts',(-44.4587830470388,-16.8066624514163,
0.));
#79134=CARTESIAN_POINT('Ctrl Pts',(-44.4587830470388,-16.8066624514163,
20.));
#79135=CARTESIAN_POINT('Ctrl Pts',(-44.4676917998748,-16.7745754699247,
0.));
#79136=CARTESIAN_POINT('Ctrl Pts',(-44.4676917998748,-16.7745754699247,
20.));
#79137=CARTESIAN_POINT('Ctrl Pts',(-44.4765778617956,-16.742483355683,0.));
#79138=CARTESIAN_POINT('Ctrl Pts',(-44.4765778617956,-16.742483355683,20.));
#79139=CARTESIAN_POINT('Ctrl Pts',(-44.4854412293128,-16.7103861245505,
0.));
#79140=CARTESIAN_POINT('Ctrl Pts',(-44.4854412293128,-16.7103861245505,
20.));
#79141=CARTESIAN_POINT('Ctrl Pts',(-44.4942818989491,-16.6782837923892,
0.));
#79142=CARTESIAN_POINT('Ctrl Pts',(-44.4942818989491,-16.6782837923892,
20.));
#79143=CARTESIAN_POINT('Ctrl Pts',(-44.5030998672381,-16.6461763750644,
0.));
#79144=CARTESIAN_POINT('Ctrl Pts',(-44.5030998672381,-16.6461763750644,
20.));
#79145=CARTESIAN_POINT('Ctrl Pts',(-44.5118951307243,-16.6140638884438,
0.));
#79146=CARTESIAN_POINT('Ctrl Pts',(-44.5118951307243,-16.6140638884438,
20.));
#79147=CARTESIAN_POINT('Ctrl Pts',(-44.5206676859633,-16.581946348398,0.));
#79148=CARTESIAN_POINT('Ctrl Pts',(-44.5206676859633,-16.581946348398,20.));
#79149=CARTESIAN_POINT('Ctrl Pts',(-44.5294175295214,-16.5498237708003,
0.));
#79150=CARTESIAN_POINT('Ctrl Pts',(-44.5294175295214,-16.5498237708003,
20.));
#79151=CARTESIAN_POINT('Ctrl Pts',(-44.5381446579761,-16.5176961715269,
0.));
#79152=CARTESIAN_POINT('Ctrl Pts',(-44.5381446579761,-16.5176961715269,
20.));
#79153=CARTESIAN_POINT('Ctrl Pts',(-44.5468490679154,-16.4855635664567,
0.));
#79154=CARTESIAN_POINT('Ctrl Pts',(-44.5468490679154,-16.4855635664567,
20.));
#79155=CARTESIAN_POINT('Ctrl Pts',(-44.5555307559385,-16.4534259714715,
0.));
#79156=CARTESIAN_POINT('Ctrl Pts',(-44.5555307559385,-16.4534259714715,
20.));
#79157=CARTESIAN_POINT('Ctrl Pts',(-44.5641897186557,-16.4212834024559,
0.));
#79158=CARTESIAN_POINT('Ctrl Pts',(-44.5641897186557,-16.4212834024559,
20.));
#79159=CARTESIAN_POINT('Ctrl Pts',(-44.5728259526889,-16.3891358752972,
0.));
#79160=CARTESIAN_POINT('Ctrl Pts',(-44.5728259526889,-16.3891358752972,
20.));
#79161=CARTESIAN_POINT('Ctrl Pts',(-44.581439454671,-16.3569834058857,0.));
#79162=CARTESIAN_POINT('Ctrl Pts',(-44.581439454671,-16.3569834058857,20.));
#79163=CARTESIAN_POINT('Ctrl Pts',(-44.5900302212458,-16.3248260101143,
0.));
#79164=CARTESIAN_POINT('Ctrl Pts',(-44.5900302212458,-16.3248260101143,
20.));
#79165=CARTESIAN_POINT('Ctrl Pts',(-44.5985982490682,-16.2926637038787,
0.));
#79166=CARTESIAN_POINT('Ctrl Pts',(-44.5985982490682,-16.2926637038787,
20.));
#79167=CARTESIAN_POINT('Ctrl Pts',(-44.6071435348036,-16.2604965030773,
0.));
#79168=CARTESIAN_POINT('Ctrl Pts',(-44.6071435348036,-16.2604965030773,
20.));
#79169=CARTESIAN_POINT('Ctrl Pts',(-44.6156660751288,-16.2283244236112,
0.));
#79170=CARTESIAN_POINT('Ctrl Pts',(-44.6156660751288,-16.2283244236112,
20.));
#79171=CARTESIAN_POINT('Ctrl Pts',(-44.6241658667307,-16.196147481384,0.));
#79172=CARTESIAN_POINT('Ctrl Pts',(-44.6241658667307,-16.196147481384,20.));
#79173=CARTESIAN_POINT('Ctrl Pts',(-44.6326429063072,-16.1639656923022,
0.));
#79174=CARTESIAN_POINT('Ctrl Pts',(-44.6326429063072,-16.1639656923022,
20.));
#79175=CARTESIAN_POINT('Ctrl Pts',(-44.6410971905673,-16.131779072275,0.));
#79176=CARTESIAN_POINT('Ctrl Pts',(-44.6410971905673,-16.131779072275,20.));
#79177=CARTESIAN_POINT('Ctrl Pts',(-44.649528716232,-16.0995876372141,0.));
#79178=CARTESIAN_POINT('Ctrl Pts',(-44.649528716232,-16.0995876372141,20.));
#79179=CARTESIAN_POINT('Ctrl Pts',(-44.6579374800339,-16.0673914030343,
0.));
#79180=CARTESIAN_POINT('Ctrl Pts',(-44.6579374800339,-16.0673914030343,
20.));
#79181=CARTESIAN_POINT('Ctrl Pts',(-44.6663234787169,-16.0351903856534,
0.));
#79182=CARTESIAN_POINT('Ctrl Pts',(-44.6663234787169,-16.0351903856534,
20.));
#79183=CARTESIAN_POINT('Ctrl Pts',(-44.6746867090345,-16.0029846009915,
0.));
#79184=CARTESIAN_POINT('Ctrl Pts',(-44.6746867090345,-16.0029846009915,
20.));
#79185=CARTESIAN_POINT('Ctrl Pts',(-44.6830271677516,-15.9707740649715,
0.));
#79186=CARTESIAN_POINT('Ctrl Pts',(-44.6830271677516,-15.9707740649715,
20.));
#79187=CARTESIAN_POINT('Ctrl Pts',(-44.691344851643,-15.9385587935186,0.));
#79188=CARTESIAN_POINT('Ctrl Pts',(-44.691344851643,-15.9385587935186,20.));
#79189=CARTESIAN_POINT('Ctrl Pts',(-44.6996397574952,-15.9063388025603,
0.));
#79190=CARTESIAN_POINT('Ctrl Pts',(-44.6996397574952,-15.9063388025603,
20.));
#79191=CARTESIAN_POINT('Ctrl Pts',(-44.7079118821065,-15.8741141080271,
0.));
#79192=CARTESIAN_POINT('Ctrl Pts',(-44.7079118821065,-15.8741141080271,
20.));
#79193=CARTESIAN_POINT('Ctrl Pts',(-44.7161612222865,-15.8418847258528,
0.));
#79194=CARTESIAN_POINT('Ctrl Pts',(-44.7161612222865,-15.8418847258528,
20.));
#79195=CARTESIAN_POINT('Ctrl Pts',(-44.7243877748558,-15.8096506719735,
0.));
#79196=CARTESIAN_POINT('Ctrl Pts',(-44.7243877748558,-15.8096506719735,
20.));
#79197=CARTESIAN_POINT('Ctrl Pts',(-44.7325915366458,-15.7774119623278,
0.));
#79198=CARTESIAN_POINT('Ctrl Pts',(-44.7325915366458,-15.7774119623278,
20.));
#79199=CARTESIAN_POINT('Ctrl Pts',(-44.7407725044985,-15.745168612857,0.));
#79200=CARTESIAN_POINT('Ctrl Pts',(-44.7407725044985,-15.745168612857,20.));
#79201=CARTESIAN_POINT('Ctrl Pts',(-44.7489306752664,-15.7129206395047,
0.));
#79202=CARTESIAN_POINT('Ctrl Pts',(-44.7489306752664,-15.7129206395047,
20.));
#79203=CARTESIAN_POINT('Ctrl Pts',(-44.7570660458133,-15.6806680582172,
0.));
#79204=CARTESIAN_POINT('Ctrl Pts',(-44.7570660458133,-15.6806680582172,
20.));
#79205=CARTESIAN_POINT('Ctrl Pts',(-44.7651786130144,-15.6484108849434,
0.));
#79206=CARTESIAN_POINT('Ctrl Pts',(-44.7651786130144,-15.6484108849434,
20.));
#79207=CARTESIAN_POINT('Ctrl Pts',(-44.7732683737566,-15.6161491356348,
0.));
#79208=CARTESIAN_POINT('Ctrl Pts',(-44.7732683737566,-15.6161491356348,
20.));
#79209=CARTESIAN_POINT('Ctrl Pts',(-44.7813353249379,-15.583882826246,0.));
#79210=CARTESIAN_POINT('Ctrl Pts',(-44.7813353249379,-15.583882826246,20.));
#79211=CARTESIAN_POINT('Ctrl Pts',(-44.7893794634672,-15.5516119727338,
0.));
#79212=CARTESIAN_POINT('Ctrl Pts',(-44.7893794634672,-15.5516119727338,
20.));
#79213=CARTESIAN_POINT('Ctrl Pts',(-44.7974007862643,-15.5193365910578,
0.));
#79214=CARTESIAN_POINT('Ctrl Pts',(-44.7974007862643,-15.5193365910578,
20.));
#79215=CARTESIAN_POINT('Ctrl Pts',(-44.8053992902599,-15.4870566971798,
0.));
#79216=CARTESIAN_POINT('Ctrl Pts',(-44.8053992902599,-15.4870566971798,
20.));
#79217=CARTESIAN_POINT('Ctrl Pts',(-44.8133749723964,-15.4547723070643,
0.));
#79218=CARTESIAN_POINT('Ctrl Pts',(-44.8133749723964,-15.4547723070643,
20.));
#79219=CARTESIAN_POINT('Ctrl Pts',(-44.8213278296263,-15.4224834366782,
0.));
#79220=CARTESIAN_POINT('Ctrl Pts',(-44.8213278296263,-15.4224834366782,
20.));
#79221=CARTESIAN_POINT('Ctrl Pts',(-44.8292578589132,-15.3901901019906,
0.));
#79222=CARTESIAN_POINT('Ctrl Pts',(-44.8292578589132,-15.3901901019906,
20.));
#79223=CARTESIAN_POINT('Ctrl Pts',(-44.8371650572316,-15.3578923189739,
0.));
#79224=CARTESIAN_POINT('Ctrl Pts',(-44.8371650572316,-15.3578923189739,
20.));
#79225=CARTESIAN_POINT('Ctrl Pts',(-44.8450494215678,-15.3255901036026,
0.));
#79226=CARTESIAN_POINT('Ctrl Pts',(-44.8450494215678,-15.3255901036026,
20.));
#79227=CARTESIAN_POINT('Ctrl Pts',(-44.8529109489191,-15.2932834718541,
0.));
#79228=CARTESIAN_POINT('Ctrl Pts',(-44.8529109489191,-15.2932834718541,
20.));
#79229=CARTESIAN_POINT('Ctrl Pts',(-44.8607496362943,-15.2609724397079,
0.));
#79230=CARTESIAN_POINT('Ctrl Pts',(-44.8607496362943,-15.2609724397079,
20.));
#79231=CARTESIAN_POINT('Ctrl Pts',(-44.8685654807131,-15.2286570231461,
0.));
#79232=CARTESIAN_POINT('Ctrl Pts',(-44.8685654807131,-15.2286570231461,
20.));
#79233=CARTESIAN_POINT('Ctrl Pts',(-44.8763584792064,-15.1963372381533,
0.));
#79234=CARTESIAN_POINT('Ctrl Pts',(-44.8763584792064,-15.1963372381533,
20.));
#79235=CARTESIAN_POINT('Ctrl Pts',(-44.8841286288163,-15.1640131007166,
0.));
#79236=CARTESIAN_POINT('Ctrl Pts',(-44.8841286288163,-15.1640131007166,
20.));
#79237=CARTESIAN_POINT('Ctrl Pts',(-44.8918759265956,-15.1316846268256,
0.));
#79238=CARTESIAN_POINT('Ctrl Pts',(-44.8918759265956,-15.1316846268256,
20.));
#79239=CARTESIAN_POINT('Ctrl Pts',(-44.8996003696078,-15.0993518324721,
0.));
#79240=CARTESIAN_POINT('Ctrl Pts',(-44.8996003696078,-15.0993518324721,
20.));
#79241=CARTESIAN_POINT('Ctrl Pts',(-44.9073019549277,-15.0670147336509,
0.));
#79242=CARTESIAN_POINT('Ctrl Pts',(-44.9073019549277,-15.0670147336509,
20.));
#79243=CARTESIAN_POINT('Ctrl Pts',(-44.9149806796409,-15.034673346359,0.));
#79244=CARTESIAN_POINT('Ctrl Pts',(-44.9149806796409,-15.034673346359,20.));
#79245=CARTESIAN_POINT('Ctrl Pts',(-44.9226365408441,-15.0023276865958,
0.));
#79246=CARTESIAN_POINT('Ctrl Pts',(-44.9226365408441,-15.0023276865958,
20.));
#79247=CARTESIAN_POINT('Ctrl Pts',(-44.9302695356455,-14.969977770363,0.));
#79248=CARTESIAN_POINT('Ctrl Pts',(-44.9302695356455,-14.969977770363,20.));
#79249=CARTESIAN_POINT('Ctrl Pts',(-44.9378796611651,-14.9376236136649,
0.));
#79250=CARTESIAN_POINT('Ctrl Pts',(-44.9378796611651,-14.9376236136649,
20.));
#79251=CARTESIAN_POINT('Ctrl Pts',(-44.9454669145344,-14.9052652325081,
0.));
#79252=CARTESIAN_POINT('Ctrl Pts',(-44.9454669145344,-14.9052652325081,
20.));
#79253=CARTESIAN_POINT('Ctrl Pts',(-44.9530312928958,-14.8729026429019,
0.));
#79254=CARTESIAN_POINT('Ctrl Pts',(-44.9530312928958,-14.8729026429019,
20.));
#79255=CARTESIAN_POINT('Ctrl Pts',(-44.9605727934022,-14.8405358608577,
0.));
#79256=CARTESIAN_POINT('Ctrl Pts',(-44.9605727934022,-14.8405358608577,
20.));
#79257=CARTESIAN_POINT('Ctrl Pts',(-44.9680914132176,-14.8081649023895,
0.));
#79258=CARTESIAN_POINT('Ctrl Pts',(-44.9680914132176,-14.8081649023895,
20.));
#79259=CARTESIAN_POINT('Ctrl Pts',(-44.9755871495162,-14.7757897835134,
0.));
#79260=CARTESIAN_POINT('Ctrl Pts',(-44.9755871495162,-14.7757897835134,
20.));
#79261=CARTESIAN_POINT('Ctrl Pts',(-44.9830599994838,-14.7434105202483,
0.));
#79262=CARTESIAN_POINT('Ctrl Pts',(-44.9830599994838,-14.7434105202483,
20.));
#79263=CARTESIAN_POINT('Ctrl Pts',(-44.9905099603172,-14.7110271286153,
0.));
#79264=CARTESIAN_POINT('Ctrl Pts',(-44.9905099603172,-14.7110271286153,
20.));
#79265=CARTESIAN_POINT('Ctrl Pts',(-44.9979370292253,-14.6786396246378,
0.));
#79266=CARTESIAN_POINT('Ctrl Pts',(-44.9979370292253,-14.6786396246378,
20.));
#79267=CARTESIAN_POINT('Ctrl Pts',(-45.0053412034276,-14.6462480243418,
0.));
#79268=CARTESIAN_POINT('Ctrl Pts',(-45.0053412034276,-14.6462480243418,
20.));
#79269=CARTESIAN_POINT('Ctrl Pts',(-45.0127224801553,-14.6138523437553,
0.));
#79270=CARTESIAN_POINT('Ctrl Pts',(-45.0127224801553,-14.6138523437553,
20.));
#79271=CARTESIAN_POINT('Ctrl Pts',(-45.020080856651,-14.5814525989087,0.));
#79272=CARTESIAN_POINT('Ctrl Pts',(-45.020080856651,-14.5814525989087,20.));
#79273=CARTESIAN_POINT('Ctrl Pts',(-45.0274163301681,-14.5490488058349,
0.));
#79274=CARTESIAN_POINT('Ctrl Pts',(-45.0274163301681,-14.5490488058349,
20.));
#79275=CARTESIAN_POINT('Ctrl Pts',(-45.0347288979708,-14.516640980569,0.));
#79276=CARTESIAN_POINT('Ctrl Pts',(-45.0347288979708,-14.516640980569,20.));
#79277=CARTESIAN_POINT('Ctrl Pts',(-45.0420185573342,-14.4842291391484,
0.));
#79278=CARTESIAN_POINT('Ctrl Pts',(-45.0420185573342,-14.4842291391484,
20.));
#79279=CARTESIAN_POINT('Ctrl Pts',(-45.0492853055441,-14.451813297613,0.));
#79280=CARTESIAN_POINT('Ctrl Pts',(-45.0492853055441,-14.451813297613,20.));
#79281=CARTESIAN_POINT('Ctrl Pts',(-45.0565291398984,-14.4193934720051,
0.));
#79282=CARTESIAN_POINT('Ctrl Pts',(-45.0565291398984,-14.4193934720051,
20.));
#79283=CARTESIAN_POINT('Ctrl Pts',(-45.0637500577056,-14.3869696783692,
0.));
#79284=CARTESIAN_POINT('Ctrl Pts',(-45.0637500577056,-14.3869696783692,
20.));
#79285=CARTESIAN_POINT('Ctrl Pts',(-45.0709480562863,-14.354541932752,0.));
#79286=CARTESIAN_POINT('Ctrl Pts',(-45.0709480562863,-14.354541932752,20.));
#79287=CARTESIAN_POINT('Ctrl Pts',(-45.078123132972,-14.3221102512025,0.));
#79288=CARTESIAN_POINT('Ctrl Pts',(-45.078123132972,-14.3221102512025,20.));
#79289=CARTESIAN_POINT('Ctrl Pts',(-45.0852752851048,-14.2896746497719,
0.));
#79290=CARTESIAN_POINT('Ctrl Pts',(-45.0852752851048,-14.2896746497719,
20.));
#79291=CARTESIAN_POINT('Ctrl Pts',(-45.0924045100383,-14.2572351445137,
0.));
#79292=CARTESIAN_POINT('Ctrl Pts',(-45.0924045100383,-14.2572351445137,
20.));
#79293=CARTESIAN_POINT('Ctrl Pts',(-45.0995108051367,-14.2247917514836,
0.));
#79294=CARTESIAN_POINT('Ctrl Pts',(-45.0995108051367,-14.2247917514836,
20.));
#79295=CARTESIAN_POINT('Ctrl Pts',(-45.1065941677758,-14.1923444867396,
0.));
#79296=CARTESIAN_POINT('Ctrl Pts',(-45.1065941677758,-14.1923444867396,
20.));
#79297=CARTESIAN_POINT('Ctrl Pts',(-45.1136545953429,-14.1598933663422,
0.));
#79298=CARTESIAN_POINT('Ctrl Pts',(-45.1136545953429,-14.1598933663422,
20.));
#79299=CARTESIAN_POINT('Ctrl Pts',(-45.1206920852361,-14.127438406354,0.));
#79300=CARTESIAN_POINT('Ctrl Pts',(-45.1206920852361,-14.127438406354,20.));
#79301=CARTESIAN_POINT('Ctrl Pts',(-45.127706634865,-14.0949796228398,0.));
#79302=CARTESIAN_POINT('Ctrl Pts',(-45.127706634865,-14.0949796228398,20.));
#79303=CARTESIAN_POINT('Ctrl Pts',(-45.1346982416501,-14.0625170318664,
0.));
#79304=CARTESIAN_POINT('Ctrl Pts',(-45.1346982416501,-14.0625170318664,
20.));
#79305=CARTESIAN_POINT('Ctrl Pts',(-45.1416669030232,-14.0300506495033,
0.));
#79306=CARTESIAN_POINT('Ctrl Pts',(-45.1416669030232,-14.0300506495033,
20.));
#79307=CARTESIAN_POINT('Ctrl Pts',(-45.1486126164275,-13.997580491822,0.));
#79308=CARTESIAN_POINT('Ctrl Pts',(-45.1486126164275,-13.997580491822,20.));
#79309=CARTESIAN_POINT('Ctrl Pts',(-45.1555353793172,-13.9651065748961,
0.));
#79310=CARTESIAN_POINT('Ctrl Pts',(-45.1555353793172,-13.9651065748961,
20.));
#79311=CARTESIAN_POINT('Ctrl Pts',(-45.1624351891574,-13.9326289148012,
0.));
#79312=CARTESIAN_POINT('Ctrl Pts',(-45.1624351891574,-13.9326289148012,
20.));
#79313=CARTESIAN_POINT('Ctrl Pts',(-45.1693120434241,-13.9001475276153,
0.));
#79314=CARTESIAN_POINT('Ctrl Pts',(-45.1693120434241,-13.9001475276153,
20.));
#79315=CARTESIAN_POINT('Ctrl Pts',(-45.1761659396043,-13.8676624294184,
0.));
#79316=CARTESIAN_POINT('Ctrl Pts',(-45.1761659396043,-13.8676624294184,
20.));
#79317=CARTESIAN_POINT('Ctrl Pts',(-45.1829968751969,-13.8351736362929,
0.));
#79318=CARTESIAN_POINT('Ctrl Pts',(-45.1829968751969,-13.8351736362929,
20.));
#79319=CARTESIAN_POINT('Ctrl Pts',(-45.1898048477123,-13.8026811643234,
0.));
#79320=CARTESIAN_POINT('Ctrl Pts',(-45.1898048477123,-13.8026811643234,
20.));
#79321=CARTESIAN_POINT('Ctrl Pts',(-45.1965898546723,-13.7701850295967,
0.));
#79322=CARTESIAN_POINT('Ctrl Pts',(-45.1965898546723,-13.7701850295967,
20.));
#79323=CARTESIAN_POINT('Ctrl Pts',(-45.2033518936101,-13.7376852482019,
0.));
#79324=CARTESIAN_POINT('Ctrl Pts',(-45.2033518936101,-13.7376852482019,
20.));
#79325=CARTESIAN_POINT('Ctrl Pts',(-45.2100909620697,-13.7051818362299,
0.));
#79326=CARTESIAN_POINT('Ctrl Pts',(-45.2100909620697,-13.7051818362299,
20.));
#79327=CARTESIAN_POINT('Ctrl Pts',(-45.2168070576061,-13.6726748097738,
0.));
#79328=CARTESIAN_POINT('Ctrl Pts',(-45.2168070576061,-13.6726748097738,
20.));
#79329=CARTESIAN_POINT('Ctrl Pts',(-45.2235001777847,-13.6401641849286,
0.));
#79330=CARTESIAN_POINT('Ctrl Pts',(-45.2235001777847,-13.6401641849286,
20.));
#79331=CARTESIAN_POINT('Ctrl Pts',(-45.2301703201819,-13.6076499777914,
0.));
#79332=CARTESIAN_POINT('Ctrl Pts',(-45.2301703201819,-13.6076499777914,
20.));
#79333=CARTESIAN_POINT('Ctrl Pts',(-45.2368174823856,-13.5751322044618,
0.));
#79334=CARTESIAN_POINT('Ctrl Pts',(-45.2368174823856,-13.5751322044618,
20.));
#79335=CARTESIAN_POINT('Ctrl Pts',(-45.2434416619952,-13.542610881041,0.));
#79336=CARTESIAN_POINT('Ctrl Pts',(-45.2434416619952,-13.542610881041,20.));
#79337=CARTESIAN_POINT('Ctrl Pts',(-45.2500428566225,-13.5100860236329,
0.));
#79338=CARTESIAN_POINT('Ctrl Pts',(-45.2500428566225,-13.5100860236329,
20.));
#79339=CARTESIAN_POINT('Ctrl Pts',(-45.2566210638904,-13.4775576483433,
0.));
#79340=CARTESIAN_POINT('Ctrl Pts',(-45.2566210638904,-13.4775576483433,
20.));
#79341=CARTESIAN_POINT('Ctrl Pts',(-45.2631762814325,-13.44502577128,0.));
#79342=CARTESIAN_POINT('Ctrl Pts',(-45.2631762814325,-13.44502577128,20.));
#79343=CARTESIAN_POINT('Ctrl Pts',(-45.2697085068935,-13.4124904085531,
0.));
#79344=CARTESIAN_POINT('Ctrl Pts',(-45.2697085068935,-13.4124904085531,
20.));
#79345=CARTESIAN_POINT('Ctrl Pts',(-45.276217737929,-13.3799515762744,0.));
#79346=CARTESIAN_POINT('Ctrl Pts',(-45.276217737929,-13.3799515762744,20.));
#79347=CARTESIAN_POINT('Ctrl Pts',(-45.2827039722059,-13.3474092905576,
0.));
#79348=CARTESIAN_POINT('Ctrl Pts',(-45.2827039722059,-13.3474092905576,
20.));
#79349=CARTESIAN_POINT('Ctrl Pts',(-45.2891672074022,-13.3148635675188,
0.));
#79350=CARTESIAN_POINT('Ctrl Pts',(-45.2891672074022,-13.3148635675188,
20.));
#79351=CARTESIAN_POINT('Ctrl Pts',(-45.2956074412073,-13.282314423276,0.));
#79352=CARTESIAN_POINT('Ctrl Pts',(-45.2956074412073,-13.282314423276,20.));
#79353=CARTESIAN_POINT('Ctrl Pts',(-45.3020246713218,-13.2497618739494,
0.));
#79354=CARTESIAN_POINT('Ctrl Pts',(-45.3020246713218,-13.2497618739494,
20.));
#79355=CARTESIAN_POINT('Ctrl Pts',(-45.3084188954577,-13.217205935661,0.));
#79356=CARTESIAN_POINT('Ctrl Pts',(-45.3084188954577,-13.217205935661,20.));
#79357=CARTESIAN_POINT('Ctrl Pts',(-45.3147901113387,-13.1846466245352,
0.));
#79358=CARTESIAN_POINT('Ctrl Pts',(-45.3147901113387,-13.1846466245352,
20.));
#79359=CARTESIAN_POINT('Ctrl Pts',(-45.321138316699,-13.1520839566979,0.));
#79360=CARTESIAN_POINT('Ctrl Pts',(-45.321138316699,-13.1520839566979,20.));
#79361=CARTESIAN_POINT('Ctrl Pts',(-45.3274635092846,-13.1195179482773,
0.));
#79362=CARTESIAN_POINT('Ctrl Pts',(-45.3274635092846,-13.1195179482773,
20.));
#79363=CARTESIAN_POINT('Ctrl Pts',(-45.3337656868523,-13.0869486154035,
0.));
#79364=CARTESIAN_POINT('Ctrl Pts',(-45.3337656868523,-13.0869486154035,
20.));
#79365=CARTESIAN_POINT('Ctrl Pts',(-45.3400448471699,-13.0543759742083,
0.));
#79366=CARTESIAN_POINT('Ctrl Pts',(-45.3400448471699,-13.0543759742083,
20.));
#79367=CARTESIAN_POINT('Ctrl Pts',(-45.3463009880171,-13.021800040826,0.));
#79368=CARTESIAN_POINT('Ctrl Pts',(-45.3463009880171,-13.021800040826,20.));
#79369=CARTESIAN_POINT('Ctrl Pts',(-45.3525341071849,-12.9892208313927,
0.));
#79370=CARTESIAN_POINT('Ctrl Pts',(-45.3525341071849,-12.9892208313927,
20.));
#79371=CARTESIAN_POINT('Ctrl Pts',(-45.3587442024753,-12.9566383620464,
0.));
#79372=CARTESIAN_POINT('Ctrl Pts',(-45.3587442024753,-12.9566383620464,
20.));
#79373=CARTESIAN_POINT('Ctrl Pts',(-45.3649312717011,-12.9240526489272,
0.));
#79374=CARTESIAN_POINT('Ctrl Pts',(-45.3649312717011,-12.9240526489272,
20.));
#79375=CARTESIAN_POINT('Ctrl Pts',(-45.371095312686,-12.8914637081769,0.));
#79376=CARTESIAN_POINT('Ctrl Pts',(-45.371095312686,-12.8914637081769,20.));
#79377=CARTESIAN_POINT('Ctrl Pts',(-45.3772363232658,-12.8588715559393,
0.));
#79378=CARTESIAN_POINT('Ctrl Pts',(-45.3772363232658,-12.8588715559393,
20.));
#79379=CARTESIAN_POINT('Ctrl Pts',(-45.3833543012877,-12.82627620836,0.));
#79380=CARTESIAN_POINT('Ctrl Pts',(-45.3833543012877,-12.82627620836,20.));
#79381=CARTESIAN_POINT('Ctrl Pts',(-45.3894492446102,-12.7936776815868,
0.));
#79382=CARTESIAN_POINT('Ctrl Pts',(-45.3894492446102,-12.7936776815868,
20.));
#79383=CARTESIAN_POINT('Ctrl Pts',(-45.3955211511034,-12.7610759917694,
0.));
#79384=CARTESIAN_POINT('Ctrl Pts',(-45.3955211511034,-12.7610759917694,
20.));
#79385=CARTESIAN_POINT('Ctrl Pts',(-45.4015700186485,-12.7284711550592,
0.));
#79386=CARTESIAN_POINT('Ctrl Pts',(-45.4015700186485,-12.7284711550592,
20.));
#79387=CARTESIAN_POINT('Ctrl Pts',(-45.407595845137,-12.6958631876099,0.));
#79388=CARTESIAN_POINT('Ctrl Pts',(-45.407595845137,-12.6958631876099,20.));
#79389=CARTESIAN_POINT('Ctrl Pts',(-45.4135986284717,-12.6632521055766,
0.));
#79390=CARTESIAN_POINT('Ctrl Pts',(-45.4135986284717,-12.6632521055766,
20.));
#79391=CARTESIAN_POINT('Ctrl Pts',(-45.4195783665665,-12.6306379251164,
0.));
#79392=CARTESIAN_POINT('Ctrl Pts',(-45.4195783665665,-12.6306379251164,
20.));
#79393=CARTESIAN_POINT('Ctrl Pts',(-45.4255350573473,-12.5980206623884,
0.));
#79394=CARTESIAN_POINT('Ctrl Pts',(-45.4255350573473,-12.5980206623884,
20.));
#79395=CARTESIAN_POINT('Ctrl Pts',(-45.4314686987515,-12.5654003335532,
0.));
#79396=CARTESIAN_POINT('Ctrl Pts',(-45.4314686987515,-12.5654003335532,
20.));
#79397=CARTESIAN_POINT('Ctrl Pts',(-45.4373792887274,-12.5327769547739,
0.));
#79398=CARTESIAN_POINT('Ctrl Pts',(-45.4373792887274,-12.5327769547739,
20.));
#79399=CARTESIAN_POINT('Ctrl Pts',(-45.4432668252347,-12.500150542215,0.));
#79400=CARTESIAN_POINT('Ctrl Pts',(-45.4432668252347,-12.500150542215,20.));
#79401=CARTESIAN_POINT('Ctrl Pts',(-45.4491313062444,-12.4675211120431,
0.));
#79402=CARTESIAN_POINT('Ctrl Pts',(-45.4491313062444,-12.4675211120431,
20.));
#79403=CARTESIAN_POINT('Ctrl Pts',(-45.4549727297392,-12.4348886804266,
0.));
#79404=CARTESIAN_POINT('Ctrl Pts',(-45.4549727297392,-12.4348886804266,
20.));
#79405=CARTESIAN_POINT('Ctrl Pts',(-45.4607910937128,-12.4022532635357,
0.));
#79406=CARTESIAN_POINT('Ctrl Pts',(-45.4607910937128,-12.4022532635357,
20.));
#79407=CARTESIAN_POINT('Ctrl Pts',(-45.4665863961701,-12.3696148775423,
0.));
#79408=CARTESIAN_POINT('Ctrl Pts',(-45.4665863961701,-12.3696148775423,
20.));
#79409=CARTESIAN_POINT('Ctrl Pts',(-45.4723586351267,-12.3369735386201,
0.));
#79410=CARTESIAN_POINT('Ctrl Pts',(-45.4723586351267,-12.3369735386201,
20.));
#79411=CARTESIAN_POINT('Ctrl Pts',(-45.4781078086095,-12.3043292629445,
0.));
#79412=CARTESIAN_POINT('Ctrl Pts',(-45.4781078086095,-12.3043292629445,
20.));
#79413=CARTESIAN_POINT('Ctrl Pts',(-45.483833914657,-12.2716820666929,0.));
#79414=CARTESIAN_POINT('Ctrl Pts',(-45.483833914657,-12.2716820666929,20.));
#79415=CARTESIAN_POINT('Ctrl Pts',(-45.4895369513189,-12.2390319660445,
0.));
#79416=CARTESIAN_POINT('Ctrl Pts',(-45.4895369513189,-12.2390319660445,
20.));
#79417=CARTESIAN_POINT('Ctrl Pts',(-45.4952169166561,-12.2063789771801,
0.));
#79418=CARTESIAN_POINT('Ctrl Pts',(-45.4952169166561,-12.2063789771801,
20.));
#79419=CARTESIAN_POINT('Ctrl Pts',(-45.5008738087416,-12.1737231162825,
0.));
#79420=CARTESIAN_POINT('Ctrl Pts',(-45.5008738087416,-12.1737231162825,
20.));
#79421=CARTESIAN_POINT('Ctrl Pts',(-45.5065076256599,-12.1410643995363,
0.));
#79422=CARTESIAN_POINT('Ctrl Pts',(-45.5065076256599,-12.1410643995363,
20.));
#79423=CARTESIAN_POINT('Ctrl Pts',(-45.5121183655068,-12.1084028431278,
0.));
#79424=CARTESIAN_POINT('Ctrl Pts',(-45.5121183655068,-12.1084028431278,
20.));
#79425=CARTESIAN_POINT('Ctrl Pts',(-45.5177060263888,-12.0757384632451,
0.));
#79426=CARTESIAN_POINT('Ctrl Pts',(-45.5177060263888,-12.0757384632451,
20.));
#79427=CARTESIAN_POINT('Ctrl Pts',(-45.5232706064237,-12.0430712760778,
0.));
#79428=CARTESIAN_POINT('Ctrl Pts',(-45.5232706064237,-12.0430712760778,
20.));
#79429=CARTESIAN_POINT('Ctrl Pts',(-45.5288121037395,-12.0104012978174,
0.));
#79430=CARTESIAN_POINT('Ctrl Pts',(-45.5288121037395,-12.0104012978174,
20.));
#79431=CARTESIAN_POINT('Ctrl Pts',(-45.5343305164759,-11.9777285446569,
0.));
#79432=CARTESIAN_POINT('Ctrl Pts',(-45.5343305164759,-11.9777285446569,
20.));
#79433=CARTESIAN_POINT('Ctrl Pts',(-45.5398258427845,-11.945053032791,0.));
#79434=CARTESIAN_POINT('Ctrl Pts',(-45.5398258427845,-11.945053032791,20.));
#79435=CARTESIAN_POINT('Ctrl Pts',(-45.5452980808284,-11.9123747784165,
0.));
#79436=CARTESIAN_POINT('Ctrl Pts',(-45.5452980808284,-11.9123747784165,
20.));
#79437=CARTESIAN_POINT('Ctrl Pts',(-45.5507472287824,-11.8796937977314,
0.));
#79438=CARTESIAN_POINT('Ctrl Pts',(-45.5507472287824,-11.8796937977314,
20.));
#79439=CARTESIAN_POINT('Ctrl Pts',(-45.5561732848327,-11.8470101069358,
0.));
#79440=CARTESIAN_POINT('Ctrl Pts',(-45.5561732848327,-11.8470101069358,
20.));
#79441=CARTESIAN_POINT('Ctrl Pts',(-45.5615762471761,-11.8143237222317,
0.));
#79442=CARTESIAN_POINT('Ctrl Pts',(-45.5615762471761,-11.8143237222317,
20.));
#79443=CARTESIAN_POINT('Ctrl Pts',(-45.5669561140206,-11.7816346598227,
0.));
#79444=CARTESIAN_POINT('Ctrl Pts',(-45.5669561140206,-11.7816346598227,
20.));
#79445=CARTESIAN_POINT('Ctrl Pts',(-45.5723128835857,-11.748942935914,0.));
#79446=CARTESIAN_POINT('Ctrl Pts',(-45.5723128835857,-11.748942935914,20.));
#79447=CARTESIAN_POINT('Ctrl Pts',(-45.5776465541021,-11.7162485667124,
0.));
#79448=CARTESIAN_POINT('Ctrl Pts',(-45.5776465541021,-11.7162485667124,
20.));
#79449=CARTESIAN_POINT('Ctrl Pts',(-45.5829571238122,-11.6835515684258,
0.));
#79450=CARTESIAN_POINT('Ctrl Pts',(-45.5829571238122,-11.6835515684258,
20.));
#79451=CARTESIAN_POINT('Ctrl Pts',(-45.5882445909695,-11.6508519572639,
0.));
#79452=CARTESIAN_POINT('Ctrl Pts',(-45.5882445909695,-11.6508519572639,
20.));
#79453=CARTESIAN_POINT('Ctrl Pts',(-45.5935089538387,-11.6181497494381,
0.));
#79454=CARTESIAN_POINT('Ctrl Pts',(-45.5935089538387,-11.6181497494381,
20.));
#79455=CARTESIAN_POINT('Ctrl Pts',(-45.598750210696,-11.5854449611619,0.));
#79456=CARTESIAN_POINT('Ctrl Pts',(-45.598750210696,-11.5854449611619,20.));
#79457=CARTESIAN_POINT('Ctrl Pts',(-45.6039683598295,-11.5527376086502,
0.));
#79458=CARTESIAN_POINT('Ctrl Pts',(-45.6039683598295,-11.5527376086502,
20.));
#79459=CARTESIAN_POINT('Ctrl Pts',(-45.6091633995383,-11.5200277081201,
0.));
#79460=CARTESIAN_POINT('Ctrl Pts',(-45.6091633995383,-11.5200277081201,
20.));
#79461=CARTESIAN_POINT('Ctrl Pts',(-45.6143353281323,-11.4873152757897,
0.));
#79462=CARTESIAN_POINT('Ctrl Pts',(-45.6143353281323,-11.4873152757897,
20.));
#79463=CARTESIAN_POINT('Ctrl Pts',(-45.6194841439321,-11.4546003278786,
0.));
#79464=CARTESIAN_POINT('Ctrl Pts',(-45.6194841439321,-11.4546003278786,
20.));
#79465=CARTESIAN_POINT('Ctrl Pts',(-45.6246098452703,-11.421882880608,0.));
#79466=CARTESIAN_POINT('Ctrl Pts',(-45.6246098452703,-11.421882880608,20.));
#79467=CARTESIAN_POINT('Ctrl Pts',(-45.6297124304911,-11.3891629502006,
0.));
#79468=CARTESIAN_POINT('Ctrl Pts',(-45.6297124304911,-11.3891629502006,
20.));
#79469=CARTESIAN_POINT('Ctrl Pts',(-45.6347918979506,-11.3564405528809,
0.));
#79470=CARTESIAN_POINT('Ctrl Pts',(-45.6347918979506,-11.3564405528809,
20.));
#79471=CARTESIAN_POINT('Ctrl Pts',(-45.6398482460165,-11.3237157048751,
0.));
#79472=CARTESIAN_POINT('Ctrl Pts',(-45.6398482460165,-11.3237157048751,
20.));
#79473=CARTESIAN_POINT('Ctrl Pts',(-45.6448814730677,-11.290988422411,0.));
#79474=CARTESIAN_POINT('Ctrl Pts',(-45.6448814730677,-11.290988422411,20.));
#79475=CARTESIAN_POINT('Ctrl Pts',(-45.6498915774933,-11.2582587217178,
0.));
#79476=CARTESIAN_POINT('Ctrl Pts',(-45.6498915774933,-11.2582587217178,
20.));
#79477=CARTESIAN_POINT('Ctrl Pts',(-45.6548785576938,-11.2255266190259,
0.));
#79478=CARTESIAN_POINT('Ctrl Pts',(-45.6548785576938,-11.2255266190259,
20.));
#79479=CARTESIAN_POINT('Ctrl Pts',(-45.6598424120808,-11.1927921305675,
0.));
#79480=CARTESIAN_POINT('Ctrl Pts',(-45.6598424120808,-11.1927921305675,
20.));
#79481=CARTESIAN_POINT('Ctrl Pts',(-45.6647831390778,-11.1600552725764,
0.));
#79482=CARTESIAN_POINT('Ctrl Pts',(-45.6647831390778,-11.1600552725764,
20.));
#79483=CARTESIAN_POINT('Ctrl Pts',(-45.6697007371202,-11.1273160612881,
0.));
#79484=CARTESIAN_POINT('Ctrl Pts',(-45.6697007371202,-11.1273160612881,
20.));
#79485=CARTESIAN_POINT('Ctrl Pts',(-45.6745952046549,-11.0945745129393,
0.));
#79486=CARTESIAN_POINT('Ctrl Pts',(-45.6745952046549,-11.0945745129393,
20.));
#79487=CARTESIAN_POINT('Ctrl Pts',(-45.6794665401395,-11.0618306437685,
0.));
#79488=CARTESIAN_POINT('Ctrl Pts',(-45.6794665401395,-11.0618306437685,
20.));
#79489=CARTESIAN_POINT('Ctrl Pts',(-45.684314742043,-11.0290844700154,0.));
#79490=CARTESIAN_POINT('Ctrl Pts',(-45.684314742043,-11.0290844700154,20.));
#79491=CARTESIAN_POINT('Ctrl Pts',(-45.6891398088456,-10.9963360079212,
0.));
#79492=CARTESIAN_POINT('Ctrl Pts',(-45.6891398088456,-10.9963360079212,
20.));
#79493=CARTESIAN_POINT('Ctrl Pts',(-45.6939417390393,-10.9635852737287,
0.));
#79494=CARTESIAN_POINT('Ctrl Pts',(-45.6939417390393,-10.9635852737287,
20.));
#79495=CARTESIAN_POINT('Ctrl Pts',(-45.698720531127,-10.930832283682,0.));
#79496=CARTESIAN_POINT('Ctrl Pts',(-45.698720531127,-10.930832283682,20.));
#79497=CARTESIAN_POINT('Ctrl Pts',(-45.7034761836229,-10.8980770540269,
0.));
#79498=CARTESIAN_POINT('Ctrl Pts',(-45.7034761836229,-10.8980770540269,
20.));
#79499=CARTESIAN_POINT('Ctrl Pts',(-45.7082086950532,-10.8653196010107,
0.));
#79500=CARTESIAN_POINT('Ctrl Pts',(-45.7082086950532,-10.8653196010107,
20.));
#79501=CARTESIAN_POINT('Ctrl Pts',(-45.7129180639559,-10.832559940882,0.));
#79502=CARTESIAN_POINT('Ctrl Pts',(-45.7129180639559,-10.832559940882,20.));
#79503=CARTESIAN_POINT('Ctrl Pts',(-45.7176042888794,-10.7997980898913,
0.));
#79504=CARTESIAN_POINT('Ctrl Pts',(-45.7176042888794,-10.7997980898913,
20.));
#79505=CARTESIAN_POINT('Ctrl Pts',(-45.7222673683833,-10.7670340642896,
0.));
#79506=CARTESIAN_POINT('Ctrl Pts',(-45.7222673683833,-10.7670340642896,
20.));
#79507=CARTESIAN_POINT('Ctrl Pts',(-45.7269073010391,-10.73426788033,0.));
#79508=CARTESIAN_POINT('Ctrl Pts',(-45.7269073010391,-10.73426788033,20.));
#79509=CARTESIAN_POINT('Ctrl Pts',(-45.7315240854293,-10.7014995542666,
0.));
#79510=CARTESIAN_POINT('Ctrl Pts',(-45.7315240854293,-10.7014995542666,
20.));
#79511=CARTESIAN_POINT('Ctrl Pts',(-45.7361177201484,-10.6687291023553,
0.));
#79512=CARTESIAN_POINT('Ctrl Pts',(-45.7361177201484,-10.6687291023553,
20.));
#79513=CARTESIAN_POINT('Ctrl Pts',(-45.7406882038015,-10.6359565408533,
0.));
#79514=CARTESIAN_POINT('Ctrl Pts',(-45.7406882038015,-10.6359565408533,
20.));
#79515=CARTESIAN_POINT('Ctrl Pts',(-45.745235535006,-10.6031818860194,0.));
#79516=CARTESIAN_POINT('Ctrl Pts',(-45.745235535006,-10.6031818860194,20.));
#79517=CARTESIAN_POINT('Ctrl Pts',(-45.7497597123901,-10.5704051541135,
0.));
#79518=CARTESIAN_POINT('Ctrl Pts',(-45.7497597123901,-10.5704051541135,
20.));
#79519=CARTESIAN_POINT('Ctrl Pts',(-45.7542607345937,-10.5376263613968,
0.));
#79520=CARTESIAN_POINT('Ctrl Pts',(-45.7542607345937,-10.5376263613968,
20.));
#79521=CARTESIAN_POINT('Ctrl Pts',(-45.7587386002674,-10.504845524132,0.));
#79522=CARTESIAN_POINT('Ctrl Pts',(-45.7587386002674,-10.504845524132,20.));
#79523=CARTESIAN_POINT('Ctrl Pts',(-45.7631933080735,-10.4720626585828,
0.));
#79524=CARTESIAN_POINT('Ctrl Pts',(-45.7631933080735,-10.4720626585828,
20.));
#79525=CARTESIAN_POINT('Ctrl Pts',(-45.7676248566855,-10.4392777810149,
0.));
#79526=CARTESIAN_POINT('Ctrl Pts',(-45.7676248566855,-10.4392777810149,
20.));
#79527=CARTESIAN_POINT('Ctrl Pts',(-45.772033244789,-10.406490907695,0.));
#79528=CARTESIAN_POINT('Ctrl Pts',(-45.772033244789,-10.406490907695,20.));
#79529=CARTESIAN_POINT('Ctrl Pts',(-45.7764184710811,-10.3737020548914,
0.));
#79530=CARTESIAN_POINT('Ctrl Pts',(-45.7764184710811,-10.3737020548914,
20.));
#79531=CARTESIAN_POINT('Ctrl Pts',(-45.7807805342697,-10.3409112388736,
0.));
#79532=CARTESIAN_POINT('Ctrl Pts',(-45.7807805342697,-10.3409112388736,
20.));
#79533=CARTESIAN_POINT('Ctrl Pts',(-45.7851194330743,-10.3081184759123,
0.));
#79534=CARTESIAN_POINT('Ctrl Pts',(-45.7851194330743,-10.3081184759123,
20.));
#79535=CARTESIAN_POINT('Ctrl Pts',(-45.7894351662253,-10.2753237822795,
0.));
#79536=CARTESIAN_POINT('Ctrl Pts',(-45.7894351662253,-10.2753237822795,
20.));
#79537=CARTESIAN_POINT('Ctrl Pts',(-45.7937277324643,-10.2425271742485,
0.));
#79538=CARTESIAN_POINT('Ctrl Pts',(-45.7937277324643,-10.2425271742485,
20.));
#79539=CARTESIAN_POINT('Ctrl Pts',(-45.7979971305449,-10.2097286680937,
0.));
#79540=CARTESIAN_POINT('Ctrl Pts',(-45.7979971305449,-10.2097286680937,
20.));
#79541=CARTESIAN_POINT('Ctrl Pts',(-45.8022433592327,-10.1769282800914,
0.));
#79542=CARTESIAN_POINT('Ctrl Pts',(-45.8022433592327,-10.1769282800914,
20.));
#79543=CARTESIAN_POINT('Ctrl Pts',(-45.8064664173048,-10.1441260265191,
0.));
#79544=CARTESIAN_POINT('Ctrl Pts',(-45.8064664173048,-10.1441260265191,
20.));
#79545=CARTESIAN_POINT('Ctrl Pts',(-45.8106663035491,-10.1113219236554,
0.));
#79546=CARTESIAN_POINT('Ctrl Pts',(-45.8106663035491,-10.1113219236554,
20.));
#79547=CARTESIAN_POINT('Ctrl Pts',(-45.8148430167647,-10.0785159877801,
0.));
#79548=CARTESIAN_POINT('Ctrl Pts',(-45.8148430167647,-10.0785159877801,
20.));
#79549=CARTESIAN_POINT('Ctrl Pts',(-45.8189965557614,-10.0457082351741,
0.));
#79550=CARTESIAN_POINT('Ctrl Pts',(-45.8189965557614,-10.0457082351741,
20.));
#79551=CARTESIAN_POINT('Ctrl Pts',(-45.8231269193611,-10.0128986821194,
0.));
#79552=CARTESIAN_POINT('Ctrl Pts',(-45.8231269193611,-10.0128986821194,
20.));
#79553=CARTESIAN_POINT('Ctrl Pts',(-45.8272341063969,-9.98008734489947,
0.));
#79554=CARTESIAN_POINT('Ctrl Pts',(-45.8272341063969,-9.98008734489947,
20.));
#79555=CARTESIAN_POINT('Ctrl Pts',(-45.8313181157134,-9.94727423979905,
0.));
#79556=CARTESIAN_POINT('Ctrl Pts',(-45.8313181157134,-9.94727423979905,
20.));
#79557=CARTESIAN_POINT('Ctrl Pts',(-45.8353789461673,-9.91445938310424,
0.));
#79558=CARTESIAN_POINT('Ctrl Pts',(-45.8353789461673,-9.91445938310424,
20.));
#79559=CARTESIAN_POINT('Ctrl Pts',(-45.8394165966264,-9.88164279110241,
0.));
#79560=CARTESIAN_POINT('Ctrl Pts',(-45.8394165966264,-9.88164279110241,
20.));
#79561=CARTESIAN_POINT('Ctrl Pts',(-45.84343106597,-9.84882448008225,0.));
#79562=CARTESIAN_POINT('Ctrl Pts',(-45.84343106597,-9.84882448008225,20.));
#79563=CARTESIAN_POINT('Ctrl Pts',(-45.8474223530896,-9.81600446633367,
0.));
#79564=CARTESIAN_POINT('Ctrl Pts',(-45.8474223530896,-9.81600446633367,
20.));
#79565=CARTESIAN_POINT('Ctrl Pts',(-45.8513904568872,-9.78318276614761,
0.));
#79566=CARTESIAN_POINT('Ctrl Pts',(-45.8513904568872,-9.78318276614761,
20.));
#79567=CARTESIAN_POINT('Ctrl Pts',(-45.8553353762765,-9.75035939581618,
0.));
#79568=CARTESIAN_POINT('Ctrl Pts',(-45.8553353762765,-9.75035939581618,
20.));
#79569=CARTESIAN_POINT('Ctrl Pts',(-45.8592571101813,-9.7175343716322,0.));
#79570=CARTESIAN_POINT('Ctrl Pts',(-45.8592571101813,-9.7175343716322,20.));
#79571=CARTESIAN_POINT('Ctrl Pts',(-45.8631556575366,-9.68470770988975,
0.));
#79572=CARTESIAN_POINT('Ctrl Pts',(-45.8631556575366,-9.68470770988975,
20.));
#79573=CARTESIAN_POINT('Ctrl Pts',(-45.8670310172895,-9.65187942688401,
0.));
#79574=CARTESIAN_POINT('Ctrl Pts',(-45.8670310172895,-9.65187942688401,
20.));
#79575=CARTESIAN_POINT('Ctrl Pts',(-45.870883188399,-9.61904953891159,0.));
#79576=CARTESIAN_POINT('Ctrl Pts',(-45.870883188399,-9.61904953891159,20.));
#79577=CARTESIAN_POINT('Ctrl Pts',(-45.8747121698355,-9.58621806227057,
0.));
#79578=CARTESIAN_POINT('Ctrl Pts',(-45.8747121698355,-9.58621806227057,
20.));
#79579=CARTESIAN_POINT('Ctrl Pts',(-45.8785179605829,-9.55338501326047,
0.));
#79580=CARTESIAN_POINT('Ctrl Pts',(-45.8785179605829,-9.55338501326047,
20.));
#79581=CARTESIAN_POINT('Ctrl Pts',(-45.882300559635,-9.52055040818184,0.));
#79582=CARTESIAN_POINT('Ctrl Pts',(-45.882300559635,-9.52055040818184,20.));
#79583=CARTESIAN_POINT('Ctrl Pts',(-45.8860599659967,-9.48771426333609,
0.));
#79584=CARTESIAN_POINT('Ctrl Pts',(-45.8860599659967,-9.48771426333609,
20.));
#79585=CARTESIAN_POINT('Ctrl Pts',(-45.8897961786838,-9.45487659502548,
0.));
#79586=CARTESIAN_POINT('Ctrl Pts',(-45.8897961786838,-9.45487659502548,
20.));
#79587=CARTESIAN_POINT('Ctrl Pts',(-45.8935091967241,-9.42203741955324,
0.));
#79588=CARTESIAN_POINT('Ctrl Pts',(-45.8935091967241,-9.42203741955324,
20.));
#79589=CARTESIAN_POINT('Ctrl Pts',(-45.8971990191563,-9.3891967532238,0.));
#79590=CARTESIAN_POINT('Ctrl Pts',(-45.8971990191563,-9.3891967532238,20.));
#79591=CARTESIAN_POINT('Ctrl Pts',(-45.90086564503,-9.35635461234246,0.));
#79592=CARTESIAN_POINT('Ctrl Pts',(-45.90086564503,-9.35635461234246,20.));
#79593=CARTESIAN_POINT('Ctrl Pts',(-45.9045090734063,-9.32351101321579,
0.));
#79594=CARTESIAN_POINT('Ctrl Pts',(-45.9045090734063,-9.32351101321579,
20.));
#79595=CARTESIAN_POINT('Ctrl Pts',(-45.9081293033577,-9.29066597215162,
0.));
#79596=CARTESIAN_POINT('Ctrl Pts',(-45.9081293033577,-9.29066597215162,
20.));
#79597=CARTESIAN_POINT('Ctrl Pts',(-45.9117263339694,-9.25781950545901,
0.));
#79598=CARTESIAN_POINT('Ctrl Pts',(-45.9117263339694,-9.25781950545901,
20.));
#79599=CARTESIAN_POINT('Ctrl Pts',(-45.9153001643391,-9.22497162944821,
0.));
#79600=CARTESIAN_POINT('Ctrl Pts',(-45.9153001643391,-9.22497162944821,
20.));
#79601=CARTESIAN_POINT('Ctrl Pts',(-45.9188507935764,-9.19212236043073,
0.));
#79602=CARTESIAN_POINT('Ctrl Pts',(-45.9188507935764,-9.19212236043073,
20.));
#79603=CARTESIAN_POINT('Ctrl Pts',(-45.9223782208015,-9.15927171471891,
0.));
#79604=CARTESIAN_POINT('Ctrl Pts',(-45.9223782208015,-9.15927171471891,
20.));
#79605=CARTESIAN_POINT('Ctrl Pts',(-45.9258824451441,-9.12641970862566,
0.));
#79606=CARTESIAN_POINT('Ctrl Pts',(-45.9258824451441,-9.12641970862566,
20.));
#79607=CARTESIAN_POINT('Ctrl Pts',(-45.9293634657451,-9.09356635846485,
0.));
#79608=CARTESIAN_POINT('Ctrl Pts',(-45.9293634657451,-9.09356635846485,
20.));
#79609=CARTESIAN_POINT('Ctrl Pts',(-45.9328212817567,-9.06071168055121,
0.));
#79610=CARTESIAN_POINT('Ctrl Pts',(-45.9328212817567,-9.06071168055121,
20.));
#79611=CARTESIAN_POINT('Ctrl Pts',(-45.9362558923428,-9.02785569120061,
0.));
#79612=CARTESIAN_POINT('Ctrl Pts',(-45.9362558923428,-9.02785569120061,
20.));
#79613=CARTESIAN_POINT('Ctrl Pts',(-45.939667296681,-8.99499840673046,0.));
#79614=CARTESIAN_POINT('Ctrl Pts',(-45.939667296681,-8.99499840673046,20.));
#79615=CARTESIAN_POINT('Ctrl Pts',(-45.9430554939595,-8.96213984345905,
0.));
#79616=CARTESIAN_POINT('Ctrl Pts',(-45.9430554939595,-8.96213984345905,
20.));
#79617=CARTESIAN_POINT('Ctrl Pts',(-45.9464204833787,-8.92928001770575,
0.));
#79618=CARTESIAN_POINT('Ctrl Pts',(-45.9464204833787,-8.92928001770575,
20.));
#79619=CARTESIAN_POINT('Ctrl Pts',(-45.9497622641496,-8.89641894579082,
0.));
#79620=CARTESIAN_POINT('Ctrl Pts',(-45.9497622641496,-8.89641894579082,
20.));
#79621=CARTESIAN_POINT('Ctrl Pts',(-45.9530808354938,-8.86355664403534,
0.));
#79622=CARTESIAN_POINT('Ctrl Pts',(-45.9530808354938,-8.86355664403534,
20.));
#79623=CARTESIAN_POINT('Ctrl Pts',(-45.9563761966444,-8.83069312876127,
0.));
#79624=CARTESIAN_POINT('Ctrl Pts',(-45.9563761966444,-8.83069312876127,
20.));
#79625=CARTESIAN_POINT('Ctrl Pts',(-45.9596483468462,-8.79782841629147,
0.));
#79626=CARTESIAN_POINT('Ctrl Pts',(-45.9596483468462,-8.79782841629147,
20.));
#79627=CARTESIAN_POINT('Ctrl Pts',(-45.9628972853566,-8.76496252295001,
0.));
#79628=CARTESIAN_POINT('Ctrl Pts',(-45.9628972853566,-8.76496252295001,
20.));
#79629=CARTESIAN_POINT('Ctrl Pts',(-45.9661230114446,-8.73209546506199,
0.));
#79630=CARTESIAN_POINT('Ctrl Pts',(-45.9661230114446,-8.73209546506199,
20.));
#79631=CARTESIAN_POINT('Ctrl Pts',(-45.9693255243897,-8.69922725895329,
0.));
#79632=CARTESIAN_POINT('Ctrl Pts',(-45.9693255243897,-8.69922725895329,
20.));
#79633=CARTESIAN_POINT('Ctrl Pts',(-45.9725048234817,-8.66635792095043,
0.));
#79634=CARTESIAN_POINT('Ctrl Pts',(-45.9725048234817,-8.66635792095043,
20.));
#79635=CARTESIAN_POINT('Ctrl Pts',(-45.9756609080225,-8.63348746738099,
0.));
#79636=CARTESIAN_POINT('Ctrl Pts',(-45.9756609080225,-8.63348746738099,
20.));
#79637=CARTESIAN_POINT('Ctrl Pts',(-45.9787937773254,-8.60061591457339,
0.));
#79638=CARTESIAN_POINT('Ctrl Pts',(-45.9787937773254,-8.60061591457339,
20.));
#79639=CARTESIAN_POINT('Ctrl Pts',(-45.9819034307166,-8.56774327885725,
0.));
#79640=CARTESIAN_POINT('Ctrl Pts',(-45.9819034307166,-8.56774327885725,
20.));
#79641=CARTESIAN_POINT('Ctrl Pts',(-45.9849898675351,-8.53486957656347,
0.));
#79642=CARTESIAN_POINT('Ctrl Pts',(-45.9849898675351,-8.53486957656347,
20.));
#79643=CARTESIAN_POINT('Ctrl Pts',(-45.9880530871298,-8.50199482402354,
0.));
#79644=CARTESIAN_POINT('Ctrl Pts',(-45.9880530871298,-8.50199482402354,
20.));
#79645=CARTESIAN_POINT('Ctrl Pts',(-45.991093088861,-8.46911903756973,0.));
#79646=CARTESIAN_POINT('Ctrl Pts',(-45.991093088861,-8.46911903756973,20.));
#79647=CARTESIAN_POINT('Ctrl Pts',(-45.9941098720982,-8.43624223353471,
0.));
#79648=CARTESIAN_POINT('Ctrl Pts',(-45.9941098720982,-8.43624223353471,
20.));
#79649=CARTESIAN_POINT('Ctrl Pts',(-45.9971034362229,-8.40336442825199,
0.));
#79650=CARTESIAN_POINT('Ctrl Pts',(-45.9971034362229,-8.40336442825199,
20.));
#79651=CARTESIAN_POINT('Ctrl Pts',(-46.000073780629,-8.37048563805605,0.));
#79652=CARTESIAN_POINT('Ctrl Pts',(-46.000073780629,-8.37048563805605,20.));
#79653=CARTESIAN_POINT('Ctrl Pts',(-46.0030209047226,-8.33760587928253,
0.));
#79654=CARTESIAN_POINT('Ctrl Pts',(-46.0030209047226,-8.33760587928253,
20.));
#79655=CARTESIAN_POINT('Ctrl Pts',(-46.0059448079215,-8.30472516826797,
0.));
#79656=CARTESIAN_POINT('Ctrl Pts',(-46.0059448079215,-8.30472516826797,
20.));
#79657=CARTESIAN_POINT('Ctrl Pts',(-46.0088454896554,-8.27184352134994,
0.));
#79658=CARTESIAN_POINT('Ctrl Pts',(-46.0088454896554,-8.27184352134994,
20.));
#79659=CARTESIAN_POINT('Ctrl Pts',(-46.0117229493647,-8.23896095486669,
0.));
#79660=CARTESIAN_POINT('Ctrl Pts',(-46.0117229493647,-8.23896095486669,
20.));
#79661=CARTESIAN_POINT('Ctrl Pts',(-46.0145771865005,-8.20607748515696,
0.));
#79662=CARTESIAN_POINT('Ctrl Pts',(-46.0145771865005,-8.20607748515696,
20.));
#79663=CARTESIAN_POINT('Ctrl Pts',(-46.0174082005262,-8.17319312856042,
0.));
#79664=CARTESIAN_POINT('Ctrl Pts',(-46.0174082005262,-8.17319312856042,
20.));
#79665=CARTESIAN_POINT('Ctrl Pts',(-46.0202159909161,-8.14030790141739,
0.));
#79666=CARTESIAN_POINT('Ctrl Pts',(-46.0202159909161,-8.14030790141739,
20.));
#79667=CARTESIAN_POINT('Ctrl Pts',(-46.0230005571558,-8.107421820069,0.));
#79668=CARTESIAN_POINT('Ctrl Pts',(-46.0230005571558,-8.107421820069,20.));
#79669=CARTESIAN_POINT('Ctrl Pts',(-46.025761898743,-8.07453490085736,0.));
#79670=CARTESIAN_POINT('Ctrl Pts',(-46.025761898743,-8.07453490085736,20.));
#79671=CARTESIAN_POINT('Ctrl Pts',(-46.0285000151874,-8.04164716012545,
0.));
#79672=CARTESIAN_POINT('Ctrl Pts',(-46.0285000151874,-8.04164716012545,
20.));
#79673=CARTESIAN_POINT('Ctrl Pts',(-46.0312149060105,-8.00875861421695,
0.));
#79674=CARTESIAN_POINT('Ctrl Pts',(-46.0312149060105,-8.00875861421695,
20.));
#79675=CARTESIAN_POINT('Ctrl Pts',(-46.0339065707442,-7.9758692794762,0.));
#79676=CARTESIAN_POINT('Ctrl Pts',(-46.0339065707442,-7.9758692794762,20.));
#79677=CARTESIAN_POINT('Ctrl Pts',(-46.0365750089318,-7.94297917224815,
0.));
#79678=CARTESIAN_POINT('Ctrl Pts',(-46.0365750089318,-7.94297917224815,
20.));
#79679=CARTESIAN_POINT('Ctrl Pts',(-46.0392202201279,-7.91008830887855,
0.));
#79680=CARTESIAN_POINT('Ctrl Pts',(-46.0392202201279,-7.91008830887855,
20.));
#79681=CARTESIAN_POINT('Ctrl Pts',(-46.0418422038989,-7.877196705714,0.));
#79682=CARTESIAN_POINT('Ctrl Pts',(-46.0418422038989,-7.877196705714,20.));
#79683=CARTESIAN_POINT('Ctrl Pts',(-46.0444409598224,-7.84430437910167,
0.));
#79684=CARTESIAN_POINT('Ctrl Pts',(-46.0444409598224,-7.84430437910167,
20.));
#79685=CARTESIAN_POINT('Ctrl Pts',(-46.0470164874882,-7.81141134538954,
0.));
#79686=CARTESIAN_POINT('Ctrl Pts',(-46.0470164874882,-7.81141134538954,
20.));
#79687=CARTESIAN_POINT('Ctrl Pts',(-46.0495687864972,-7.77851762092636,
0.));
#79688=CARTESIAN_POINT('Ctrl Pts',(-46.0495687864972,-7.77851762092636,
20.));
#79689=CARTESIAN_POINT('Ctrl Pts',(-46.052097856463,-7.74562322206167,0.));
#79690=CARTESIAN_POINT('Ctrl Pts',(-46.052097856463,-7.74562322206167,20.));
#79691=CARTESIAN_POINT('Ctrl Pts',(-46.0546036970108,-7.71272816514571,
0.));
#79692=CARTESIAN_POINT('Ctrl Pts',(-46.0546036970108,-7.71272816514571,
20.));
#79693=CARTESIAN_POINT('Ctrl Pts',(-46.0570863077758,-7.67983246652917,
0.));
#79694=CARTESIAN_POINT('Ctrl Pts',(-46.0570863077758,-7.67983246652917,
20.));
#79695=CARTESIAN_POINT('Ctrl Pts',(-46.0595456884042,-7.64693614256335,
0.));
#79696=CARTESIAN_POINT('Ctrl Pts',(-46.0595456884042,-7.64693614256335,
20.));
#79697=CARTESIAN_POINT('Ctrl Pts',(-46.0619818385541,-7.61403920960035,
0.));
#79698=CARTESIAN_POINT('Ctrl Pts',(-46.0619818385541,-7.61403920960035,
20.));
#79699=CARTESIAN_POINT('Ctrl Pts',(-46.0643947578955,-7.58114168399302,
0.));
#79700=CARTESIAN_POINT('Ctrl Pts',(-46.0643947578955,-7.58114168399302,
20.));
#79701=CARTESIAN_POINT('Ctrl Pts',(-46.0667844461104,-7.54824358209484,
0.));
#79702=CARTESIAN_POINT('Ctrl Pts',(-46.0667844461104,-7.54824358209484,
20.));
#79703=CARTESIAN_POINT('Ctrl Pts',(-46.0691509028928,-7.51534492025983,
0.));
#79704=CARTESIAN_POINT('Ctrl Pts',(-46.0691509028928,-7.51534492025983,
20.));
#79705=CARTESIAN_POINT('Ctrl Pts',(-46.0714941279471,-7.4824457148425,0.));
#79706=CARTESIAN_POINT('Ctrl Pts',(-46.0714941279471,-7.4824457148425,20.));
#79707=CARTESIAN_POINT('Ctrl Pts',(-46.0738141209885,-7.44954598219809,
0.));
#79708=CARTESIAN_POINT('Ctrl Pts',(-46.0738141209885,-7.44954598219809,
20.));
#79709=CARTESIAN_POINT('Ctrl Pts',(-46.0761108817447,-7.4166457386826,0.));
#79710=CARTESIAN_POINT('Ctrl Pts',(-46.0761108817447,-7.4166457386826,20.));
#79711=CARTESIAN_POINT('Ctrl Pts',(-46.0783844099553,-7.38374500065294,
0.));
#79712=CARTESIAN_POINT('Ctrl Pts',(-46.0783844099553,-7.38374500065294,
20.));
#79713=CARTESIAN_POINT('Ctrl Pts',(-46.0806347053718,-7.35084378446661,
0.));
#79714=CARTESIAN_POINT('Ctrl Pts',(-46.0806347053718,-7.35084378446661,
20.));
#79715=CARTESIAN_POINT('Ctrl Pts',(-46.0828617677561,-7.31794210648139,
0.));
#79716=CARTESIAN_POINT('Ctrl Pts',(-46.0828617677561,-7.31794210648139,
20.));
#79717=CARTESIAN_POINT('Ctrl Pts',(-46.0850655968817,-7.2850399830555,0.));
#79718=CARTESIAN_POINT('Ctrl Pts',(-46.0850655968817,-7.2850399830555,20.));
#79719=CARTESIAN_POINT('Ctrl Pts',(-46.0872461925336,-7.25213743054749,
0.));
#79720=CARTESIAN_POINT('Ctrl Pts',(-46.0872461925336,-7.25213743054749,
20.));
#79721=CARTESIAN_POINT('Ctrl Pts',(-46.0894035545083,-7.2192344653164,0.));
#79722=CARTESIAN_POINT('Ctrl Pts',(-46.0894035545083,-7.2192344653164,20.));
#79723=CARTESIAN_POINT('Ctrl Pts',(-46.0915376826137,-7.18633110372211,
0.));
#79724=CARTESIAN_POINT('Ctrl Pts',(-46.0915376826137,-7.18633110372211,
20.));
#79725=CARTESIAN_POINT('Ctrl Pts',(-46.0936485766695,-7.15342736212529,
0.));
#79726=CARTESIAN_POINT('Ctrl Pts',(-46.0936485766695,-7.15342736212529,
20.));
#79727=CARTESIAN_POINT('Ctrl Pts',(-46.0957362365075,-7.12052325688752,
0.));
#79728=CARTESIAN_POINT('Ctrl Pts',(-46.0957362365075,-7.12052325688752,
20.));
#79729=CARTESIAN_POINT('Ctrl Pts',(-46.097800661971,-7.08761880437093,0.));
#79730=CARTESIAN_POINT('Ctrl Pts',(-46.097800661971,-7.08761880437093,20.));
#79731=CARTESIAN_POINT('Ctrl Pts',(-46.0998418529147,-7.05471402093801,
0.));
#79732=CARTESIAN_POINT('Ctrl Pts',(-46.0998418529147,-7.05471402093801,
20.));
#79733=CARTESIAN_POINT('Ctrl Pts',(-46.1018598092046,-7.02180892295147,
0.));
#79734=CARTESIAN_POINT('Ctrl Pts',(-46.1018598092046,-7.02180892295147,
20.));
#79735=CARTESIAN_POINT('Ctrl Pts',(-46.103854530718,-6.98890352677438,0.));
#79736=CARTESIAN_POINT('Ctrl Pts',(-46.103854530718,-6.98890352677438,20.));
#79737=CARTESIAN_POINT('Ctrl Pts',(-46.1058260173429,-6.95599784877019,
0.));
#79738=CARTESIAN_POINT('Ctrl Pts',(-46.1058260173429,-6.95599784877019,
20.));
#79739=CARTESIAN_POINT('Ctrl Pts',(-46.1077742689797,-6.92309190530285,
0.));
#79740=CARTESIAN_POINT('Ctrl Pts',(-46.1077742689797,-6.92309190530285,
20.));
#79741=CARTESIAN_POINT('Ctrl Pts',(-46.1096992855399,-6.89018571273689,
0.));
#79742=CARTESIAN_POINT('Ctrl Pts',(-46.1096992855399,-6.89018571273689,
20.));
#79743=CARTESIAN_POINT('Ctrl Pts',(-46.111601066948,-6.85727928743787,0.));
#79744=CARTESIAN_POINT('Ctrl Pts',(-46.111601066948,-6.85727928743787,20.));
#79745=CARTESIAN_POINT('Ctrl Pts',(-46.1134796131392,-6.82437264577169,
0.));
#79746=CARTESIAN_POINT('Ctrl Pts',(-46.1134796131392,-6.82437264577169,
20.));
#79747=CARTESIAN_POINT('Ctrl Pts',(-46.1153349240611,-6.7914658041047,0.));
#79748=CARTESIAN_POINT('Ctrl Pts',(-46.1153349240611,-6.7914658041047,20.));
#79749=CARTESIAN_POINT('Ctrl Pts',(-46.1171669996709,-6.75855877880356,
0.));
#79750=CARTESIAN_POINT('Ctrl Pts',(-46.1171669996709,-6.75855877880356,
20.));
#79751=CARTESIAN_POINT('Ctrl Pts',(-46.1189758399374,-6.7256515862352,0.));
#79752=CARTESIAN_POINT('Ctrl Pts',(-46.1189758399374,-6.7256515862352,20.));
#79753=CARTESIAN_POINT('Ctrl Pts',(-46.1207614448407,-6.69274424276687,
0.));
#79754=CARTESIAN_POINT('Ctrl Pts',(-46.1207614448407,-6.69274424276687,
20.));
#79755=CARTESIAN_POINT('Ctrl Pts',(-46.122523814374,-6.65983676476652,0.));
#79756=CARTESIAN_POINT('Ctrl Pts',(-46.122523814374,-6.65983676476652,20.));
#79757=CARTESIAN_POINT('Ctrl Pts',(-46.124262948542,-6.62692916860257,0.));
#79758=CARTESIAN_POINT('Ctrl Pts',(-46.124262948542,-6.62692916860257,20.));
#79759=CARTESIAN_POINT('Ctrl Pts',(-46.1259788473615,-6.59402147064399,
0.));
#79760=CARTESIAN_POINT('Ctrl Pts',(-46.1259788473615,-6.59402147064399,
20.));
#79761=CARTESIAN_POINT('Ctrl Pts',(-46.1276715108604,-6.56111368726009,
0.));
#79762=CARTESIAN_POINT('Ctrl Pts',(-46.1276715108604,-6.56111368726009,
20.));
#79763=CARTESIAN_POINT('Ctrl Pts',(-46.1293409390781,-6.52820583482049,
0.));
#79764=CARTESIAN_POINT('Ctrl Pts',(-46.1293409390781,-6.52820583482049,
20.));
#79765=CARTESIAN_POINT('Ctrl Pts',(-46.1309871320644,-6.49529792969508,
0.));
#79766=CARTESIAN_POINT('Ctrl Pts',(-46.1309871320644,-6.49529792969508,
20.));
#79767=CARTESIAN_POINT('Ctrl Pts',(-46.1326100898806,-6.46238998825407,
0.));
#79768=CARTESIAN_POINT('Ctrl Pts',(-46.1326100898806,-6.46238998825407,
20.));
#79769=CARTESIAN_POINT('Ctrl Pts',(-46.1342098125991,-6.42948202686813,
0.));
#79770=CARTESIAN_POINT('Ctrl Pts',(-46.1342098125991,-6.42948202686813,
20.));
#79771=CARTESIAN_POINT('Ctrl Pts',(-46.1357863003044,-6.39657406190844,
0.));
#79772=CARTESIAN_POINT('Ctrl Pts',(-46.1357863003044,-6.39657406190844,
20.));
#79773=CARTESIAN_POINT('Ctrl Pts',(-46.1373395530931,-6.36366610974647,
0.));
#79774=CARTESIAN_POINT('Ctrl Pts',(-46.1373395530931,-6.36366610974647,
20.));
#79775=CARTESIAN_POINT('Ctrl Pts',(-46.138869571074,-6.33075818675419,0.));
#79776=CARTESIAN_POINT('Ctrl Pts',(-46.138869571074,-6.33075818675419,20.));
#79777=CARTESIAN_POINT('Ctrl Pts',(-46.1403763543673,-6.29785030930381,
0.));
#79778=CARTESIAN_POINT('Ctrl Pts',(-46.1403763543673,-6.29785030930381,
20.));
#79779=CARTESIAN_POINT('Ctrl Pts',(-46.141859903105,-6.26494249376777,0.));
#79780=CARTESIAN_POINT('Ctrl Pts',(-46.141859903105,-6.26494249376777,20.));
#79781=CARTESIAN_POINT('Ctrl Pts',(-46.1433202174297,-6.23203475651882,
0.));
#79782=CARTESIAN_POINT('Ctrl Pts',(-46.1433202174297,-6.23203475651882,
20.));
#79783=CARTESIAN_POINT('Ctrl Pts',(-46.1447572974959,-6.19912711393004,
0.));
#79784=CARTESIAN_POINT('Ctrl Pts',(-46.1447572974959,-6.19912711393004,
20.));
#79785=CARTESIAN_POINT('Ctrl Pts',(-46.1461711434687,-6.16621958237487,
0.));
#79786=CARTESIAN_POINT('Ctrl Pts',(-46.1461711434687,-6.16621958237487,
20.));
#79787=CARTESIAN_POINT('Ctrl Pts',(-46.1475617555249,-6.1333121782271,0.));
#79788=CARTESIAN_POINT('Ctrl Pts',(-46.1475617555249,-6.1333121782271,20.));
#79789=CARTESIAN_POINT('Ctrl Pts',(-46.1489291338532,-6.10040491786085,
0.));
#79790=CARTESIAN_POINT('Ctrl Pts',(-46.1489291338532,-6.10040491786085,
20.));
#79791=CARTESIAN_POINT('Ctrl Pts',(-46.1502732786543,-6.06749781765058,
0.));
#79792=CARTESIAN_POINT('Ctrl Pts',(-46.1502732786543,-6.06749781765058,
20.));
#79793=CARTESIAN_POINT('Ctrl Pts',(-46.151594190141,-6.03459089397104,0.));
#79794=CARTESIAN_POINT('Ctrl Pts',(-46.151594190141,-6.03459089397104,20.));
#79795=CARTESIAN_POINT('Ctrl Pts',(-46.1528918685373,-6.0016841631972,0.));
#79796=CARTESIAN_POINT('Ctrl Pts',(-46.1528918685373,-6.0016841631972,20.));
#79797=CARTESIAN_POINT('Ctrl Pts',(-46.1541663140783,-5.96877764170411,
0.));
#79798=CARTESIAN_POINT('Ctrl Pts',(-46.1541663140783,-5.96877764170411,
20.));
#79799=CARTESIAN_POINT('Ctrl Pts',(-46.1554175270101,-5.93587134586689,
0.));
#79800=CARTESIAN_POINT('Ctrl Pts',(-46.1554175270101,-5.93587134586689,
20.));
#79801=CARTESIAN_POINT('Ctrl Pts',(-46.1566455075904,-5.90296529206097,
0.));
#79802=CARTESIAN_POINT('Ctrl Pts',(-46.1566455075904,-5.90296529206097,
20.));
#79803=CARTESIAN_POINT('Ctrl Pts',(-46.1578502560886,-5.87005949666211,
0.));
#79804=CARTESIAN_POINT('Ctrl Pts',(-46.1578502560886,-5.87005949666211,
20.));
#79805=CARTESIAN_POINT('Ctrl Pts',(-46.1590317727861,-5.83715397604653,
0.));
#79806=CARTESIAN_POINT('Ctrl Pts',(-46.1590317727861,-5.83715397604653,
20.));
#79807=CARTESIAN_POINT('Ctrl Pts',(-46.160190057976,-5.80424874659071,0.));
#79808=CARTESIAN_POINT('Ctrl Pts',(-46.160190057976,-5.80424874659071,20.));
#79809=CARTESIAN_POINT('Ctrl Pts',(-46.1613251119636,-5.77134382467172,
0.));
#79810=CARTESIAN_POINT('Ctrl Pts',(-46.1613251119636,-5.77134382467172,
20.));
#79811=CARTESIAN_POINT('Ctrl Pts',(-46.1624369350662,-5.73843922666647,
0.));
#79812=CARTESIAN_POINT('Ctrl Pts',(-46.1624369350662,-5.73843922666647,
20.));
#79813=CARTESIAN_POINT('Ctrl Pts',(-46.1635255276116,-5.70553496895184,
0.));
#79814=CARTESIAN_POINT('Ctrl Pts',(-46.1635255276116,-5.70553496895184,
20.));
#79815=CARTESIAN_POINT('Ctrl Pts',(-46.1645908899393,-5.67263106790478,
0.));
#79816=CARTESIAN_POINT('Ctrl Pts',(-46.1645908899393,-5.67263106790478,
20.));
#79817=CARTESIAN_POINT('Ctrl Pts',(-46.1656330223979,-5.63972753990235,
0.));
#79818=CARTESIAN_POINT('Ctrl Pts',(-46.1656330223979,-5.63972753990235,
20.));
#79819=CARTESIAN_POINT('Ctrl Pts',(-46.166651925349,-5.60682440132181,0.));
#79820=CARTESIAN_POINT('Ctrl Pts',(-46.166651925349,-5.60682440132181,20.));
#79821=CARTESIAN_POINT('Ctrl Pts',(-46.1676475991657,-5.57392166854074,
0.));
#79822=CARTESIAN_POINT('Ctrl Pts',(-46.1676475991657,-5.57392166854074,
20.));
#79823=CARTESIAN_POINT('Ctrl Pts',(-46.1686200442337,-5.54101935793709,
0.));
#79824=CARTESIAN_POINT('Ctrl Pts',(-46.1686200442337,-5.54101935793709,
20.));
#79825=CARTESIAN_POINT('Ctrl Pts',(-46.1695692609505,-5.50811748588893,
0.));
#79826=CARTESIAN_POINT('Ctrl Pts',(-46.1695692609505,-5.50811748588893,
20.));
#79827=CARTESIAN_POINT('Ctrl Pts',(-46.170495249726,-5.47521606877459,0.));
#79828=CARTESIAN_POINT('Ctrl Pts',(-46.170495249726,-5.47521606877459,20.));
#79829=CARTESIAN_POINT('Ctrl Pts',(-46.1713980109807,-5.44231512297238,
0.));
#79830=CARTESIAN_POINT('Ctrl Pts',(-46.1713980109807,-5.44231512297238,
20.));
#79831=CARTESIAN_POINT('Ctrl Pts',(-46.1722775451467,-5.40941466486069,
0.));
#79832=CARTESIAN_POINT('Ctrl Pts',(-46.1722775451467,-5.40941466486069,
20.));
#79833=CARTESIAN_POINT('Ctrl Pts',(-46.1731338526667,-5.37651471081787,
0.));
#79834=CARTESIAN_POINT('Ctrl Pts',(-46.1731338526667,-5.37651471081787,
20.));
#79835=CARTESIAN_POINT('Ctrl Pts',(-46.1739669339953,-5.34361527722239,
0.));
#79836=CARTESIAN_POINT('Ctrl Pts',(-46.1739669339953,-5.34361527722239,
20.));
#79837=CARTESIAN_POINT('Ctrl Pts',(-46.1747767895978,-5.31071638045279,
0.));
#79838=CARTESIAN_POINT('Ctrl Pts',(-46.1747767895978,-5.31071638045279,
20.));
#79839=CARTESIAN_POINT('Ctrl Pts',(-46.1755634199519,-5.2778180368879,0.));
#79840=CARTESIAN_POINT('Ctrl Pts',(-46.1755634199519,-5.2778180368879,20.));
#79841=CARTESIAN_POINT('Ctrl Pts',(-46.1763268255471,-5.24492026290662,
0.));
#79842=CARTESIAN_POINT('Ctrl Pts',(-46.1763268255471,-5.24492026290662,
20.));
#79843=CARTESIAN_POINT('Ctrl Pts',(-46.1770670068854,-5.21202307488801,
0.));
#79844=CARTESIAN_POINT('Ctrl Pts',(-46.1770670068854,-5.21202307488801,
20.));
#79845=CARTESIAN_POINT('Ctrl Pts',(-46.1777839644797,-5.17912648921101,
0.));
#79846=CARTESIAN_POINT('Ctrl Pts',(-46.1777839644797,-5.17912648921101,
20.));
#79847=CARTESIAN_POINT('Ctrl Pts',(-46.1784776988548,-5.14623052225471,
0.));
#79848=CARTESIAN_POINT('Ctrl Pts',(-46.1784776988548,-5.14623052225471,
20.));
#79849=CARTESIAN_POINT('Ctrl Pts',(-46.1791482105459,-5.11333519039808,
0.));
#79850=CARTESIAN_POINT('Ctrl Pts',(-46.1791482105459,-5.11333519039808,
20.));
#79851=CARTESIAN_POINT('Ctrl Pts',(-46.1797955000997,-5.08044051002025,
0.));
#79852=CARTESIAN_POINT('Ctrl Pts',(-46.1797955000997,-5.08044051002025,
20.));
#79853=CARTESIAN_POINT('Ctrl Pts',(-46.1804195680748,-5.0475464975003,0.));
#79854=CARTESIAN_POINT('Ctrl Pts',(-46.1804195680748,-5.0475464975003,20.));
#79855=CARTESIAN_POINT('Ctrl Pts',(-46.1810204150412,-5.01465316921748,
0.));
#79856=CARTESIAN_POINT('Ctrl Pts',(-46.1810204150412,-5.01465316921748,
20.));
#79857=CARTESIAN_POINT('Ctrl Pts',(-46.1815980415817,-4.981760541551,0.));
#79858=CARTESIAN_POINT('Ctrl Pts',(-46.1815980415817,-4.981760541551,20.));
#79859=CARTESIAN_POINT('Ctrl Pts',(-46.182152448291,-4.94886863088032,0.));
#79860=CARTESIAN_POINT('Ctrl Pts',(-46.182152448291,-4.94886863088032,20.));
#79861=CARTESIAN_POINT('Ctrl Pts',(-46.1826836357763,-4.91597745358481,
0.));
#79862=CARTESIAN_POINT('Ctrl Pts',(-46.1826836357763,-4.91597745358481,
20.));
#79863=CARTESIAN_POINT('Ctrl Pts',(-46.1831916046531,-4.88308702604349,
0.));
#79864=CARTESIAN_POINT('Ctrl Pts',(-46.1831916046531,-4.88308702604349,
20.));
#79865=CARTESIAN_POINT('Ctrl Pts',(-46.1836763555496,-4.85019736463543,
0.));
#79866=CARTESIAN_POINT('Ctrl Pts',(-46.1836763555496,-4.85019736463543,
20.));
#79867=CARTESIAN_POINT('Ctrl Pts',(-46.1841378891039,-4.81730848573953,
0.));
#79868=CARTESIAN_POINT('Ctrl Pts',(-46.1841378891039,-4.81730848573953,
20.));
#79869=CARTESIAN_POINT('Ctrl Pts',(-46.1845762059678,-4.78442040573514,
0.));
#79870=CARTESIAN_POINT('Ctrl Pts',(-46.1845762059678,-4.78442040573514,
20.));
#79871=CARTESIAN_POINT('Ctrl Pts',(-46.1849913068043,-4.7515331410016,0.));
#79872=CARTESIAN_POINT('Ctrl Pts',(-46.1849913068043,-4.7515331410016,20.));
#79873=CARTESIAN_POINT('Ctrl Pts',(-46.1853831922891,-4.71864670791826,
0.));
#79874=CARTESIAN_POINT('Ctrl Pts',(-46.1853831922891,-4.71864670791826,
20.));
#79875=CARTESIAN_POINT('Ctrl Pts',(-46.1857518631086,-4.68576112286394,
0.));
#79876=CARTESIAN_POINT('Ctrl Pts',(-46.1857518631086,-4.68576112286394,
20.));
#79877=CARTESIAN_POINT('Ctrl Pts',(-46.1860973199616,-4.65287640221747,
0.));
#79878=CARTESIAN_POINT('Ctrl Pts',(-46.1860973199616,-4.65287640221747,
20.));
#79879=CARTESIAN_POINT('Ctrl Pts',(-46.1864195635571,-4.6199925623574,0.));
#79880=CARTESIAN_POINT('Ctrl Pts',(-46.1864195635571,-4.6199925623574,20.));
#79881=CARTESIAN_POINT('Ctrl Pts',(-46.1867185946155,-4.58710961966232,
0.));
#79882=CARTESIAN_POINT('Ctrl Pts',(-46.1867185946155,-4.58710961966232,
20.));
#79883=CARTESIAN_POINT('Ctrl Pts',(-46.1869944138693,-4.55422759051101,
0.));
#79884=CARTESIAN_POINT('Ctrl Pts',(-46.1869944138693,-4.55422759051101,
20.));
#79885=CARTESIAN_POINT('Ctrl Pts',(-46.1872470220627,-4.52134649128217,
0.));
#79886=CARTESIAN_POINT('Ctrl Pts',(-46.1872470220627,-4.52134649128217,
20.));
#79887=CARTESIAN_POINT('Ctrl Pts',(-46.1874764199521,-4.48846633835459,
0.));
#79888=CARTESIAN_POINT('Ctrl Pts',(-46.1874764199521,-4.48846633835459,
20.));
#79889=CARTESIAN_POINT('Ctrl Pts',(-46.1876826083051,-4.4555871481068,0.));
#79890=CARTESIAN_POINT('Ctrl Pts',(-46.1876826083051,-4.4555871481068,20.));
#79891=CARTESIAN_POINT('Ctrl Pts',(-46.1878655879008,-4.42270893691723,
0.));
#79892=CARTESIAN_POINT('Ctrl Pts',(-46.1878655879008,-4.42270893691723,
20.));
#79893=CARTESIAN_POINT('Ctrl Pts',(-46.1880253595297,-4.38983172116389,
0.));
#79894=CARTESIAN_POINT('Ctrl Pts',(-46.1880253595297,-4.38983172116389,
20.));
#79895=CARTESIAN_POINT('Ctrl Pts',(-46.1881619239926,-4.35695551722447,
0.));
#79896=CARTESIAN_POINT('Ctrl Pts',(-46.1881619239926,-4.35695551722447,
20.));
#79897=CARTESIAN_POINT('Ctrl Pts',(-46.1882752821036,-4.32408034147654,
0.));
#79898=CARTESIAN_POINT('Ctrl Pts',(-46.1882752821036,-4.32408034147654,
20.));
#79899=CARTESIAN_POINT('Ctrl Pts',(-46.1883654346888,-4.29120621029776,
0.));
#79900=CARTESIAN_POINT('Ctrl Pts',(-46.1883654346888,-4.29120621029776,
20.));
#79901=CARTESIAN_POINT('Ctrl Pts',(-46.1884323825857,-4.25833314006578,
0.));
#79902=CARTESIAN_POINT('Ctrl Pts',(-46.1884323825857,-4.25833314006578,
20.));
#79903=CARTESIAN_POINT('Ctrl Pts',(-46.1884761266433,-4.22546114715825,
0.));
#79904=CARTESIAN_POINT('Ctrl Pts',(-46.1884761266433,-4.22546114715825,
20.));
#79905=CARTESIAN_POINT('Ctrl Pts',(-46.1884966677209,-4.19259024795238,
0.));
#79906=CARTESIAN_POINT('Ctrl Pts',(-46.1884966677209,-4.19259024795238,
20.));
#79907=CARTESIAN_POINT('Ctrl Pts',(-46.1884940066895,-4.15972045882508,
0.));
#79908=CARTESIAN_POINT('Ctrl Pts',(-46.1884940066895,-4.15972045882508,
20.));
#79909=CARTESIAN_POINT('Ctrl Pts',(-46.1884681444317,-4.12685179615294,
0.));
#79910=CARTESIAN_POINT('Ctrl Pts',(-46.1884681444317,-4.12685179615294,
20.));
#79911=CARTESIAN_POINT('Ctrl Pts',(-46.188419081843,-4.09398427631254,0.));
#79912=CARTESIAN_POINT('Ctrl Pts',(-46.188419081843,-4.09398427631254,20.));
#79913=CARTESIAN_POINT('Ctrl Pts',(-46.18834681983,-4.06111791568023,0.));
#79914=CARTESIAN_POINT('Ctrl Pts',(-46.18834681983,-4.06111791568023,20.));
#79915=CARTESIAN_POINT('Ctrl Pts',(-46.1882513593113,-4.02825273063217,
0.));
#79916=CARTESIAN_POINT('Ctrl Pts',(-46.1882513593113,-4.02825273063217,
20.));
#79917=CARTESIAN_POINT('Ctrl Pts',(-46.1881327012171,-3.99538873754442,
0.));
#79918=CARTESIAN_POINT('Ctrl Pts',(-46.1881327012171,-3.99538873754442,
20.));
#79919=CARTESIAN_POINT('Ctrl Pts',(-46.1879908464881,-3.96252595279274,
0.));
#79920=CARTESIAN_POINT('Ctrl Pts',(-46.1879908464881,-3.96252595279274,
20.));
#79921=CARTESIAN_POINT('Ctrl Pts',(-46.1878257960766,-3.92966439275257,
0.));
#79922=CARTESIAN_POINT('Ctrl Pts',(-46.1878257960766,-3.92966439275257,
20.));
#79923=CARTESIAN_POINT('Ctrl Pts',(-46.1876375509469,-3.89680407379914,
0.));
#79924=CARTESIAN_POINT('Ctrl Pts',(-46.1876375509469,-3.89680407379914,
20.));
#79925=CARTESIAN_POINT('Ctrl Pts',(-46.1874261120751,-3.86394501230744,
0.));
#79926=CARTESIAN_POINT('Ctrl Pts',(-46.1874261120751,-3.86394501230744,
20.));
#79927=CARTESIAN_POINT('Ctrl Pts',(-46.1871914804492,-3.83108722465198,
0.));
#79928=CARTESIAN_POINT('Ctrl Pts',(-46.1871914804492,-3.83108722465198,
20.));
#79929=CARTESIAN_POINT('Ctrl Pts',(-46.1869336570686,-3.79823072720685,
0.));
#79930=CARTESIAN_POINT('Ctrl Pts',(-46.1869336570686,-3.79823072720685,
20.));
#79931=CARTESIAN_POINT('Ctrl Pts',(-46.1866526429445,-3.76537553634595,
0.));
#79932=CARTESIAN_POINT('Ctrl Pts',(-46.1866526429445,-3.76537553634595,
20.));
#79933=CARTESIAN_POINT('Ctrl Pts',(-46.1863484390996,-3.73252166844327,
0.));
#79934=CARTESIAN_POINT('Ctrl Pts',(-46.1863484390996,-3.73252166844327,
20.));
#79935=CARTESIAN_POINT('Ctrl Pts',(-46.1860210465678,-3.69966913987252,
0.));
#79936=CARTESIAN_POINT('Ctrl Pts',(-46.1860210465678,-3.69966913987252,
20.));
#79937=CARTESIAN_POINT('Ctrl Pts',(-46.185670466394,-3.66681796700709,0.));
#79938=CARTESIAN_POINT('Ctrl Pts',(-46.185670466394,-3.66681796700709,20.));
#79939=CARTESIAN_POINT('Ctrl Pts',(-46.1852966996347,-3.63396816621989,
0.));
#79940=CARTESIAN_POINT('Ctrl Pts',(-46.1852966996347,-3.63396816621989,
20.));
#79941=CARTESIAN_POINT('Ctrl Pts',(-46.1848997473582,-3.60111975388338,
0.));
#79942=CARTESIAN_POINT('Ctrl Pts',(-46.1848997473582,-3.60111975388338,
20.));
#79943=CARTESIAN_POINT('Ctrl Pts',(-46.1844796106451,-3.56827274636958,
0.));
#79944=CARTESIAN_POINT('Ctrl Pts',(-46.1844796106451,-3.56827274636958,
20.));
#79945=CARTESIAN_POINT('Ctrl Pts',(-46.1840362905882,-3.53542716005024,
0.));
#79946=CARTESIAN_POINT('Ctrl Pts',(-46.1840362905882,-3.53542716005024,
20.));
#79947=CARTESIAN_POINT('Ctrl Pts',(-46.1835697882921,-3.50258301129688,
0.));
#79948=CARTESIAN_POINT('Ctrl Pts',(-46.1835697882921,-3.50258301129688,
20.));
#79949=CARTESIAN_POINT('Ctrl Pts',(-46.1830801048722,-3.4697403164807,0.));
#79950=CARTESIAN_POINT('Ctrl Pts',(-46.1830801048722,-3.4697403164807,20.));
#79951=CARTESIAN_POINT('Ctrl Pts',(-46.1825672414553,-3.43689909197262,
0.));
#79952=CARTESIAN_POINT('Ctrl Pts',(-46.1825672414553,-3.43689909197262,
20.));
#79953=CARTESIAN_POINT('Ctrl Pts',(-46.1820311991793,-3.40405935414302,
0.));
#79954=CARTESIAN_POINT('Ctrl Pts',(-46.1820311991793,-3.40405935414302,
20.));
#79955=CARTESIAN_POINT('Ctrl Pts',(-46.1814719791936,-3.37122111936182,
0.));
#79956=CARTESIAN_POINT('Ctrl Pts',(-46.1814719791936,-3.37122111936182,
20.));
#79957=CARTESIAN_POINT('Ctrl Pts',(-46.1808895826591,-3.33838440399861,
0.));
#79958=CARTESIAN_POINT('Ctrl Pts',(-46.1808895826591,-3.33838440399861,
20.));
#79959=CARTESIAN_POINT('Ctrl Pts',(-46.1802840107495,-3.30554922442265,
0.));
#79960=CARTESIAN_POINT('Ctrl Pts',(-46.1802840107495,-3.30554922442265,
20.));
#79961=CARTESIAN_POINT('Ctrl Pts',(-46.1796552646498,-3.27271559700278,
0.));
#79962=CARTESIAN_POINT('Ctrl Pts',(-46.1796552646498,-3.27271559700278,
20.));
#79963=CARTESIAN_POINT('Ctrl Pts',(-46.1790033455572,-3.23988353810748,
0.));
#79964=CARTESIAN_POINT('Ctrl Pts',(-46.1790033455572,-3.23988353810748,
20.));
#79965=CARTESIAN_POINT('Ctrl Pts',(-46.1783282546796,-3.2070530641047,0.));
#79966=CARTESIAN_POINT('Ctrl Pts',(-46.1783282546796,-3.2070530641047,20.));
#79967=CARTESIAN_POINT('Ctrl Pts',(-46.1776299932363,-3.17422419136187,
0.));
#79968=CARTESIAN_POINT('Ctrl Pts',(-46.1776299932363,-3.17422419136187,
20.));
#79969=CARTESIAN_POINT('Ctrl Pts',(-46.1769085624582,-3.14139693624604,
0.));
#79970=CARTESIAN_POINT('Ctrl Pts',(-46.1769085624582,-3.14139693624604,
20.));
#79971=CARTESIAN_POINT('Ctrl Pts',(-46.1761639635878,-3.10857131512384,
0.));
#79972=CARTESIAN_POINT('Ctrl Pts',(-46.1761639635878,-3.10857131512384,
20.));
#79973=CARTESIAN_POINT('Ctrl Pts',(-46.1753961978798,-3.07574734436159,
0.));
#79974=CARTESIAN_POINT('Ctrl Pts',(-46.1753961978798,-3.07574734436159,
20.));
#79975=CARTESIAN_POINT('Ctrl Pts',(-46.1746052665999,-3.04292504032496,
0.));
#79976=CARTESIAN_POINT('Ctrl Pts',(-46.1746052665999,-3.04292504032496,
20.));
#79977=CARTESIAN_POINT('Ctrl Pts',(-46.1737911710261,-3.01010441937912,
0.));
#79978=CARTESIAN_POINT('Ctrl Pts',(-46.1737911710261,-3.01010441937912,
20.));
#79979=CARTESIAN_POINT('Ctrl Pts',(-46.1729539124487,-2.97728549788889,
0.));
#79980=CARTESIAN_POINT('Ctrl Pts',(-46.1729539124487,-2.97728549788889,
20.));
#79981=CARTESIAN_POINT('Ctrl Pts',(-46.172093492169,-2.94446829221864,0.));
#79982=CARTESIAN_POINT('Ctrl Pts',(-46.172093492169,-2.94446829221864,20.));
#79983=CARTESIAN_POINT('Ctrl Pts',(-46.1712099114993,-2.91165281873224,
0.));
#79984=CARTESIAN_POINT('Ctrl Pts',(-46.1712099114993,-2.91165281873224,
20.));
#79985=CARTESIAN_POINT('Ctrl Pts',(-46.1703031717627,-2.87883909379286,
0.));
#79986=CARTESIAN_POINT('Ctrl Pts',(-46.1703031717627,-2.87883909379286,
20.));
#79987=CARTESIAN_POINT('Ctrl Pts',(-46.169373274294,-2.84602713376308,0.));
#79988=CARTESIAN_POINT('Ctrl Pts',(-46.169373274294,-2.84602713376308,20.));
#79989=CARTESIAN_POINT('Ctrl Pts',(-46.1684202204402,-2.81321695500491,
0.));
#79990=CARTESIAN_POINT('Ctrl Pts',(-46.1684202204402,-2.81321695500491,
20.));
#79991=CARTESIAN_POINT('Ctrl Pts',(-46.1674440115603,-2.78040857388008,
0.));
#79992=CARTESIAN_POINT('Ctrl Pts',(-46.1674440115603,-2.78040857388008,
20.));
#79993=CARTESIAN_POINT('Ctrl Pts',(-46.1664446490252,-2.74760200674979,
0.));
#79994=CARTESIAN_POINT('Ctrl Pts',(-46.1664446490252,-2.74760200674979,
20.));
#79995=CARTESIAN_POINT('Ctrl Pts',(-46.1654221342175,-2.71479726997479,
0.));
#79996=CARTESIAN_POINT('Ctrl Pts',(-46.1654221342175,-2.71479726997479,
20.));
#79997=CARTESIAN_POINT('Ctrl Pts',(-46.1643764685316,-2.68199437991523,
0.));
#79998=CARTESIAN_POINT('Ctrl Pts',(-46.1643764685316,-2.68199437991523,
20.));
#79999=CARTESIAN_POINT('Ctrl Pts',(-46.163307653373,-2.64919335293067,0.));
#80000=CARTESIAN_POINT('Ctrl Pts',(-46.163307653373,-2.64919335293067,20.));
#80001=CARTESIAN_POINT('Ctrl Pts',(-46.1622156901587,-2.61639420537994,
0.));
#80002=CARTESIAN_POINT('Ctrl Pts',(-46.1622156901587,-2.61639420537994,
20.));
#80003=CARTESIAN_POINT('Ctrl Pts',(-46.1611005803162,-2.58359695362107,
0.));
#80004=CARTESIAN_POINT('Ctrl Pts',(-46.1611005803162,-2.58359695362107,
20.));
#80005=CARTESIAN_POINT('Ctrl Pts',(-46.1599623252856,-2.55080161401166,
0.));
#80006=CARTESIAN_POINT('Ctrl Pts',(-46.1599623252856,-2.55080161401166,
20.));
#80007=CARTESIAN_POINT('Ctrl Pts',(-46.1588009265184,-2.51800820290891,
0.));
#80008=CARTESIAN_POINT('Ctrl Pts',(-46.1588009265184,-2.51800820290891,
20.));
#80009=CARTESIAN_POINT('Ctrl Pts',(-46.1576163854777,-2.48521673666957,
0.));
#80010=CARTESIAN_POINT('Ctrl Pts',(-46.1576163854777,-2.48521673666957,
20.));
#80011=CARTESIAN_POINT('Ctrl Pts',(-46.1564087036389,-2.4524272316497,0.));
#80012=CARTESIAN_POINT('Ctrl Pts',(-46.1564087036389,-2.4524272316497,20.));
#80013=CARTESIAN_POINT('Ctrl Pts',(-46.155177882489,-2.41963970420457,0.));
#80014=CARTESIAN_POINT('Ctrl Pts',(-46.155177882489,-2.41963970420457,20.));
#80015=CARTESIAN_POINT('Ctrl Pts',(-46.1539239235264,-2.3868541706887,0.));
#80016=CARTESIAN_POINT('Ctrl Pts',(-46.1539239235264,-2.3868541706887,20.));
#80017=CARTESIAN_POINT('Ctrl Pts',(-46.1526468282604,-2.35407064745589,
0.));
#80018=CARTESIAN_POINT('Ctrl Pts',(-46.1526468282604,-2.35407064745589,
20.));
#80019=CARTESIAN_POINT('Ctrl Pts',(-46.1513465982124,-2.32128915085919,
0.));
#80020=CARTESIAN_POINT('Ctrl Pts',(-46.1513465982124,-2.32128915085919,
20.));
#80021=CARTESIAN_POINT('Ctrl Pts',(-46.1500232349155,-2.28850969725138,
0.));
#80022=CARTESIAN_POINT('Ctrl Pts',(-46.1500232349155,-2.28850969725138,
20.));
#80023=CARTESIAN_POINT('Ctrl Pts',(-46.1486767399146,-2.25573230298458,
0.));
#80024=CARTESIAN_POINT('Ctrl Pts',(-46.1486767399146,-2.25573230298458,
20.));
#80025=CARTESIAN_POINT('Ctrl Pts',(-46.147307114766,-2.22295698441049,0.));
#80026=CARTESIAN_POINT('Ctrl Pts',(-46.147307114766,-2.22295698441049,20.));
#80027=CARTESIAN_POINT('Ctrl Pts',(-46.1459143610377,-2.19018375787986,
0.));
#80028=CARTESIAN_POINT('Ctrl Pts',(-46.1459143610377,-2.19018375787986,
20.));
#80029=CARTESIAN_POINT('Ctrl Pts',(-46.1444984803082,-2.15741263974262,
0.));
#80030=CARTESIAN_POINT('Ctrl Pts',(-46.1444984803082,-2.15741263974262,
20.));
#80031=CARTESIAN_POINT('Ctrl Pts',(-46.1430594741682,-2.12464364634812,
0.));
#80032=CARTESIAN_POINT('Ctrl Pts',(-46.1430594741682,-2.12464364634812,
20.));
#80033=CARTESIAN_POINT('Ctrl Pts',(-46.1415973442202,-2.09187679404497,
0.));
#80034=CARTESIAN_POINT('Ctrl Pts',(-46.1415973442202,-2.09187679404497,
20.));
#80035=CARTESIAN_POINT('Ctrl Pts',(-46.1401120920793,-2.05911209918101,
0.));
#80036=CARTESIAN_POINT('Ctrl Pts',(-46.1401120920793,-2.05911209918101,
20.));
#80037=CARTESIAN_POINT('Ctrl Pts',(-46.1386037193727,-2.02634957810317,
0.));
#80038=CARTESIAN_POINT('Ctrl Pts',(-46.1386037193727,-2.02634957810317,
20.));
#80039=CARTESIAN_POINT('Ctrl Pts',(-46.1370722277379,-1.99358924715753,
0.));
#80040=CARTESIAN_POINT('Ctrl Pts',(-46.1370722277379,-1.99358924715753,
20.));
#80041=CARTESIAN_POINT('Ctrl Pts',(-46.1355176188236,-1.9608311226893,0.));
#80042=CARTESIAN_POINT('Ctrl Pts',(-46.1355176188236,-1.9608311226893,20.));
#80043=CARTESIAN_POINT('Ctrl Pts',(-46.1339398942902,-1.92807522104339,
0.));
#80044=CARTESIAN_POINT('Ctrl Pts',(-46.1339398942902,-1.92807522104339,
20.));
#80045=CARTESIAN_POINT('Ctrl Pts',(-46.1323390558096,-1.89532155856414,
0.));
#80046=CARTESIAN_POINT('Ctrl Pts',(-46.1323390558096,-1.89532155856414,
20.));
#80047=CARTESIAN_POINT('Ctrl Pts',(-46.1307151050651,-1.86257015159582,
0.));
#80048=CARTESIAN_POINT('Ctrl Pts',(-46.1307151050651,-1.86257015159582,
20.));
#80049=CARTESIAN_POINT('Ctrl Pts',(-46.1290680437528,-1.82982101648206,
0.));
#80050=CARTESIAN_POINT('Ctrl Pts',(-46.1290680437528,-1.82982101648206,
20.));
#80051=CARTESIAN_POINT('Ctrl Pts',(-46.1273978735796,-1.79707416956534,
0.));
#80052=CARTESIAN_POINT('Ctrl Pts',(-46.1273978735796,-1.79707416956534,
20.));
#80053=CARTESIAN_POINT('Ctrl Pts',(-46.1257045962649,-1.76432962718685,
0.));
#80054=CARTESIAN_POINT('Ctrl Pts',(-46.1257045962649,-1.76432962718685,
20.));
#80055=CARTESIAN_POINT('Ctrl Pts',(-46.1239882135394,-1.73158740568597,
0.));
#80056=CARTESIAN_POINT('Ctrl Pts',(-46.1239882135394,-1.73158740568597,
20.));
#80057=CARTESIAN_POINT('Ctrl Pts',(-46.1222487271454,-1.69884752140039,
0.));
#80058=CARTESIAN_POINT('Ctrl Pts',(-46.1222487271454,-1.69884752140039,
20.));
#80059=CARTESIAN_POINT('Ctrl Pts',(-46.1204861388364,-1.66610999066655,
0.));
#80060=CARTESIAN_POINT('Ctrl Pts',(-46.1204861388364,-1.66610999066655,
20.));
#80061=CARTESIAN_POINT('Ctrl Pts',(-46.1187004503775,-1.6333748298207,0.));
#80062=CARTESIAN_POINT('Ctrl Pts',(-46.1187004503775,-1.6333748298207,20.));
#80063=CARTESIAN_POINT('Ctrl Pts',(-46.1168916635447,-1.60064205519958,
0.));
#80064=CARTESIAN_POINT('Ctrl Pts',(-46.1168916635447,-1.60064205519958,
20.));
#80065=CARTESIAN_POINT('Ctrl Pts',(-46.1150597801266,-1.56791168314158,
0.));
#80066=CARTESIAN_POINT('Ctrl Pts',(-46.1150597801266,-1.56791168314158,
20.));
#80067=CARTESIAN_POINT('Ctrl Pts',(-46.1132048019234,-1.53518372998667,
0.));
#80068=CARTESIAN_POINT('Ctrl Pts',(-46.1132048019234,-1.53518372998667,
20.));
#80069=CARTESIAN_POINT('Ctrl Pts',(-46.111326730748,-1.5024582120743,0.));
#80070=CARTESIAN_POINT('Ctrl Pts',(-46.111326730748,-1.5024582120743,20.));
#80071=CARTESIAN_POINT('Ctrl Pts',(-46.1094255684237,-1.46973514574143,
0.));
#80072=CARTESIAN_POINT('Ctrl Pts',(-46.1094255684237,-1.46973514574143,
20.));
#80073=CARTESIAN_POINT('Ctrl Pts',(-46.1075013167858,-1.4370145473209,0.));
#80074=CARTESIAN_POINT('Ctrl Pts',(-46.1075013167858,-1.4370145473209,20.));
#80075=CARTESIAN_POINT('Ctrl Pts',(-46.1055539776802,-1.40429643313893,
0.));
#80076=CARTESIAN_POINT('Ctrl Pts',(-46.1055539776802,-1.40429643313893,
20.));
#80077=CARTESIAN_POINT('Ctrl Pts',(-46.1035835529643,-1.37158081951551,
0.));
#80078=CARTESIAN_POINT('Ctrl Pts',(-46.1035835529643,-1.37158081951551,
20.));
#80079=CARTESIAN_POINT('Ctrl Pts',(-46.1015900445065,-1.33886772276919,
0.));
#80080=CARTESIAN_POINT('Ctrl Pts',(-46.1015900445065,-1.33886772276919,
20.));
#80081=CARTESIAN_POINT('Ctrl Pts',(-46.0995734541875,-1.30615715922172,
0.));
#80082=CARTESIAN_POINT('Ctrl Pts',(-46.0995734541875,-1.30615715922172,
20.));
#80083=CARTESIAN_POINT('Ctrl Pts',(-46.0975337839002,-1.27344914520175,
0.));
#80084=CARTESIAN_POINT('Ctrl Pts',(-46.0975337839002,-1.27344914520175,
20.));
#80085=CARTESIAN_POINT('Ctrl Pts',(-46.0954710355506,-1.24074369705072,
0.));
#80086=CARTESIAN_POINT('Ctrl Pts',(-46.0954710355506,-1.24074369705072,
20.));
#80087=CARTESIAN_POINT('Ctrl Pts',(-46.0933852110571,-1.20804083112097,
0.));
#80088=CARTESIAN_POINT('Ctrl Pts',(-46.0933852110571,-1.20804083112097,
20.));
#80089=CARTESIAN_POINT('Ctrl Pts',(-46.0912763123502,-1.17534056376402,
0.));
#80090=CARTESIAN_POINT('Ctrl Pts',(-46.0912763123502,-1.17534056376402,
20.));
#80091=CARTESIAN_POINT('Ctrl Pts',(-46.0891443413718,-1.14264291132052,
0.));
#80092=CARTESIAN_POINT('Ctrl Pts',(-46.0891443413718,-1.14264291132052,
20.));
#80093=CARTESIAN_POINT('Ctrl Pts',(-46.0869893000734,-1.10994789011162,
0.));
#80094=CARTESIAN_POINT('Ctrl Pts',(-46.0869893000734,-1.10994789011162,
20.));
#80095=CARTESIAN_POINT('Ctrl Pts',(-46.0848111904142,-1.07725551642471,
0.));
#80096=CARTESIAN_POINT('Ctrl Pts',(-46.0848111904142,-1.07725551642471,
20.));
#80097=CARTESIAN_POINT('Ctrl Pts',(-46.0826100143611,-1.04456580652047,
0.));
#80098=CARTESIAN_POINT('Ctrl Pts',(-46.0826100143611,-1.04456580652047,
20.));
#80099=CARTESIAN_POINT('Ctrl Pts',(-46.0803857738924,-1.01187877665954,
0.));
#80100=CARTESIAN_POINT('Ctrl Pts',(-46.0803857738924,-1.01187877665954,
20.));
#80101=CARTESIAN_POINT('Ctrl Pts',(-46.0781384710012,-0.979194443126286,
0.));
#80102=CARTESIAN_POINT('Ctrl Pts',(-46.0781384710012,-0.979194443126286,
20.));
#80103=CARTESIAN_POINT('Ctrl Pts',(-46.0758681076973,-0.946512822248744,
0.));
#80104=CARTESIAN_POINT('Ctrl Pts',(-46.0758681076973,-0.946512822248744,
20.));
#80105=CARTESIAN_POINT('Ctrl Pts',(-46.0735746860119,-0.913833930432268,
0.));
#80106=CARTESIAN_POINT('Ctrl Pts',(-46.0735746860119,-0.913833930432268,
20.));
#80107=CARTESIAN_POINT('Ctrl Pts',(-46.0712582079948,-0.881157784136737,
0.));
#80108=CARTESIAN_POINT('Ctrl Pts',(-46.0712582079948,-0.881157784136737,
20.));
#80109=CARTESIAN_POINT('Ctrl Pts',(-46.0689186757066,-0.848484399815181,
0.));
#80110=CARTESIAN_POINT('Ctrl Pts',(-46.0689186757066,-0.848484399815181,
20.));
#80111=CARTESIAN_POINT('Ctrl Pts',(-46.0665560912128,-0.815813793858633,
0.));
#80112=CARTESIAN_POINT('Ctrl Pts',(-46.0665560912128,-0.815813793858633,
20.));
#80113=CARTESIAN_POINT('Ctrl Pts',(-46.064170456577,-0.78314598254893,0.));
#80114=CARTESIAN_POINT('Ctrl Pts',(-46.064170456577,-0.78314598254893,20.));
#80115=CARTESIAN_POINT('Ctrl Pts',(-46.0617617738521,-0.750480981980923,
0.));
#80116=CARTESIAN_POINT('Ctrl Pts',(-46.0617617738521,-0.750480981980923,
20.));
#80117=CARTESIAN_POINT('Ctrl Pts',(-46.0593300450868,-0.717818808129722,
0.));
#80118=CARTESIAN_POINT('Ctrl Pts',(-46.0593300450868,-0.717818808129722,
20.));
#80119=CARTESIAN_POINT('Ctrl Pts',(-46.0568752723439,-0.685159476991759,
0.));
#80120=CARTESIAN_POINT('Ctrl Pts',(-46.0568752723439,-0.685159476991759,
20.));
#80121=CARTESIAN_POINT('Ctrl Pts',(-46.0543974577158,-0.652503004713259,
0.));
#80122=CARTESIAN_POINT('Ctrl Pts',(-46.0543974577158,-0.652503004713259,
20.));
#80123=CARTESIAN_POINT('Ctrl Pts',(-46.0518966033391,-0.619849407700859,
0.));
#80124=CARTESIAN_POINT('Ctrl Pts',(-46.0518966033391,-0.619849407700859,
20.));
#80125=CARTESIAN_POINT('Ctrl Pts',(-46.0493727114182,-0.587198702798619,
0.));
#80126=CARTESIAN_POINT('Ctrl Pts',(-46.0493727114182,-0.587198702798619,
20.));
#80127=CARTESIAN_POINT('Ctrl Pts',(-46.0468257841997,-0.554550907098827,
0.));
#80128=CARTESIAN_POINT('Ctrl Pts',(-46.0468257841997,-0.554550907098827,
20.));
#80129=CARTESIAN_POINT('Ctrl Pts',(-46.044255823933,-0.521906037621043,
0.));
#80130=CARTESIAN_POINT('Ctrl Pts',(-46.044255823933,-0.521906037621043,
20.));
#80131=CARTESIAN_POINT('Ctrl Pts',(-46.0416628328334,-0.489264111013836,
0.));
#80132=CARTESIAN_POINT('Ctrl Pts',(-46.0416628328334,-0.489264111013836,
20.));
#80133=CARTESIAN_POINT('Ctrl Pts',(-46.0390468130479,-0.456625143292611,
0.));
#80134=CARTESIAN_POINT('Ctrl Pts',(-46.0390468130479,-0.456625143292611,
20.));
#80135=CARTESIAN_POINT('Ctrl Pts',(-46.0364077666069,-0.423989149445243,
0.));
#80136=CARTESIAN_POINT('Ctrl Pts',(-46.0364077666069,-0.423989149445243,
20.));
#80137=CARTESIAN_POINT('Ctrl Pts',(-46.0337456954889,-0.391356143937831,
0.));
#80138=CARTESIAN_POINT('Ctrl Pts',(-46.0337456954889,-0.391356143937831,
20.));
#80139=CARTESIAN_POINT('Ctrl Pts',(-46.0310606017089,-0.358726141441568,
0.));
#80140=CARTESIAN_POINT('Ctrl Pts',(-46.0310606017089,-0.358726141441568,
20.));
#80141=CARTESIAN_POINT('Ctrl Pts',(-46.0283524874048,-0.32609915751695,
0.));
#80142=CARTESIAN_POINT('Ctrl Pts',(-46.0283524874048,-0.32609915751695,
20.));
#80143=CARTESIAN_POINT('Ctrl Pts',(-46.025621354915,-0.293475209241787,
0.));
#80144=CARTESIAN_POINT('Ctrl Pts',(-46.025621354915,-0.293475209241787,
20.));
#80145=CARTESIAN_POINT('Ctrl Pts',(-46.022867206884,-0.260854316057531,
0.));
#80146=CARTESIAN_POINT('Ctrl Pts',(-46.022867206884,-0.260854316057531,
20.));
#80147=CARTESIAN_POINT('Ctrl Pts',(-46.0200900461091,-0.228236498538561,
0.));
#80148=CARTESIAN_POINT('Ctrl Pts',(-46.0200900461091,-0.228236498538561,
20.));
#80149=CARTESIAN_POINT('Ctrl Pts',(-46.0172898753497,-0.195621776838879,
0.));
#80150=CARTESIAN_POINT('Ctrl Pts',(-46.0172898753497,-0.195621776838879,
20.));
#80151=CARTESIAN_POINT('Ctrl Pts',(-46.0144666971462,-0.163010169231703,
0.));
#80152=CARTESIAN_POINT('Ctrl Pts',(-46.0144666971462,-0.163010169231703,
20.));
#80153=CARTESIAN_POINT('Ctrl Pts',(-46.0116205136405,-0.130401690656317,
0.));
#80154=CARTESIAN_POINT('Ctrl Pts',(-46.0116205136405,-0.130401690656317,
20.));
#80155=CARTESIAN_POINT('Ctrl Pts',(-46.0087513263814,-0.0977963511372804,
0.));
#80156=CARTESIAN_POINT('Ctrl Pts',(-46.0087513263814,-0.0977963511372804,
20.));
#80157=CARTESIAN_POINT('Ctrl Pts',(-46.0058591364029,-0.0651941566547531,
0.));
#80158=CARTESIAN_POINT('Ctrl Pts',(-46.0058591364029,-0.0651941566547531,
20.));
#80159=CARTESIAN_POINT('Ctrl Pts',(-46.0035269827389,-0.0391149194889384,
0.));
#80160=CARTESIAN_POINT('Ctrl Pts',(-46.0035269827389,-0.0391149194889384,
20.));
#80161=CARTESIAN_POINT('Ctrl Pts',(-46.0017675166781,-0.019556908668581,
0.));
#80162=CARTESIAN_POINT('Ctrl Pts',(-46.0017675166781,-0.019556908668581,
20.));
#80163=CARTESIAN_POINT('Ctrl Pts',(-46.0005899389515,-0.00651886458936213,
0.));
#80164=CARTESIAN_POINT('Ctrl Pts',(-46.0005899389515,-0.00651886458936213,
20.));
#80165=CARTESIAN_POINT('Ctrl Pts',(-46.,6.66133814775094E-15,0.));
#80166=CARTESIAN_POINT('Ctrl Pts',(-46.,6.66133814775094E-15,20.));
#80167=CARTESIAN_POINT('',(-46.,1.33226762955019E-14,2.));
#80168=CARTESIAN_POINT('',(-46.,1.33226762955019E-14,0.));
#80169=CARTESIAN_POINT('Ctrl Pts',(-46.,6.66133814775094E-15,2.));
#80170=CARTESIAN_POINT('Ctrl Pts',(-46.2231469371097,-2.46578847330934,
2.));
#80171=CARTESIAN_POINT('Ctrl Pts',(-46.2472869474438,-4.94053945739677,
2.));
#80172=CARTESIAN_POINT('Ctrl Pts',(-46.0771487393297,-7.40158428157358,
2.));
#80173=CARTESIAN_POINT('Ctrl Pts',(-46.0449384185095,16.7589870229578,0.));
#80174=CARTESIAN_POINT('Ctrl Pts',(-46.0449384185095,16.7589870229578,20.));
#80175=CARTESIAN_POINT('Ctrl Pts',(-46.0420594924752,16.7651130917503,0.));
#80176=CARTESIAN_POINT('Ctrl Pts',(-46.0420594924752,16.7651130917503,20.));
#80177=CARTESIAN_POINT('Ctrl Pts',(-46.0362995834799,16.7773641333857,0.));
#80178=CARTESIAN_POINT('Ctrl Pts',(-46.0362995834799,16.7773641333857,20.));
#80179=CARTESIAN_POINT('Ctrl Pts',(-46.0276535492065,16.7957374079899,0.));
#80180=CARTESIAN_POINT('Ctrl Pts',(-46.0276535492065,16.7957374079899,20.));
#80181=CARTESIAN_POINT('Ctrl Pts',(-46.0161131619282,16.8202285317553,0.));
#80182=CARTESIAN_POINT('Ctrl Pts',(-46.0161131619282,16.8202285317553,20.));
#80183=CARTESIAN_POINT('Ctrl Pts',(-46.0016671088634,16.8508314760754,0.));
#80184=CARTESIAN_POINT('Ctrl Pts',(-46.0016671088634,16.8508314760754,20.));
#80185=CARTESIAN_POINT('Ctrl Pts',(-45.9872004880192,16.8814234574888,0.));
#80186=CARTESIAN_POINT('Ctrl Pts',(-45.9872004880192,16.8814234574888,20.));
#80187=CARTESIAN_POINT('Ctrl Pts',(-45.9727133019197,16.9120044710149,0.));
#80188=CARTESIAN_POINT('Ctrl Pts',(-45.9727133019197,16.9120044710149,20.));
#80189=CARTESIAN_POINT('Ctrl Pts',(-45.9582055548827,16.9425745084438,0.));
#80190=CARTESIAN_POINT('Ctrl Pts',(-45.9582055548827,16.9425745084438,20.));
#80191=CARTESIAN_POINT('Ctrl Pts',(-45.9436772535459,16.9731335574459,0.));
#80192=CARTESIAN_POINT('Ctrl Pts',(-45.9436772535459,16.9731335574459,20.));
#80193=CARTESIAN_POINT('Ctrl Pts',(-45.9291284062576,17.0036816026634,0.));
#80194=CARTESIAN_POINT('Ctrl Pts',(-45.9291284062576,17.0036816026634,20.));
#80195=CARTESIAN_POINT('Ctrl Pts',(-45.91455902239,17.0342186269341,0.));
#80196=CARTESIAN_POINT('Ctrl Pts',(-45.91455902239,17.0342186269341,20.));
#80197=CARTESIAN_POINT('Ctrl Pts',(-45.8999691116667,17.0647446124944,0.));
#80198=CARTESIAN_POINT('Ctrl Pts',(-45.8999691116667,17.0647446124944,20.));
#80199=CARTESIAN_POINT('Ctrl Pts',(-45.8853586835176,17.0952595421299,0.));
#80200=CARTESIAN_POINT('Ctrl Pts',(-45.8853586835176,17.0952595421299,20.));
#80201=CARTESIAN_POINT('Ctrl Pts',(-45.8707277463338,17.1257634005083,0.));
#80202=CARTESIAN_POINT('Ctrl Pts',(-45.8707277463338,17.1257634005083,20.));
#80203=CARTESIAN_POINT('Ctrl Pts',(-45.8560763076625,17.1562561738292,0.));
#80204=CARTESIAN_POINT('Ctrl Pts',(-45.8560763076625,17.1562561738292,20.));
#80205=CARTESIAN_POINT('Ctrl Pts',(-45.8414043745501,17.1867378492105,0.));
#80206=CARTESIAN_POINT('Ctrl Pts',(-45.8414043745501,17.1867378492105,20.));
#80207=CARTESIAN_POINT('Ctrl Pts',(-45.8267119538424,17.2172084141516,0.));
#80208=CARTESIAN_POINT('Ctrl Pts',(-45.8267119538424,17.2172084141516,20.));
#80209=CARTESIAN_POINT('Ctrl Pts',(-45.8119990524824,17.247667856,0.));
#80210=CARTESIAN_POINT('Ctrl Pts',(-45.8119990524824,17.247667856,20.));
#80211=CARTESIAN_POINT('Ctrl Pts',(-45.7972656778619,17.2781161613228,0.));
#80212=CARTESIAN_POINT('Ctrl Pts',(-45.7972656778619,17.2781161613228,20.));
#80213=CARTESIAN_POINT('Ctrl Pts',(-45.7825118377706,17.3085533159981,0.));
#80214=CARTESIAN_POINT('Ctrl Pts',(-45.7825118377706,17.3085533159981,20.));
#80215=CARTESIAN_POINT('Ctrl Pts',(-45.7677375402376,17.3389793054984,0.));
#80216=CARTESIAN_POINT('Ctrl Pts',(-45.7677375402376,17.3389793054984,20.));
#80217=CARTESIAN_POINT('Ctrl Pts',(-45.7529427934047,17.3693941151172,0.));
#80218=CARTESIAN_POINT('Ctrl Pts',(-45.7529427934047,17.3693941151172,20.));
#80219=CARTESIAN_POINT('Ctrl Pts',(-45.7381276053972,17.3997977302007,0.));
#80220=CARTESIAN_POINT('Ctrl Pts',(-45.7381276053972,17.3997977302007,20.));
#80221=CARTESIAN_POINT('Ctrl Pts',(-45.7232919841685,17.4301901364248,0.));
#80222=CARTESIAN_POINT('Ctrl Pts',(-45.7232919841685,17.4301901364248,20.));
#80223=CARTESIAN_POINT('Ctrl Pts',(-45.7084359375081,17.460571319782,0.));
#80224=CARTESIAN_POINT('Ctrl Pts',(-45.7084359375081,17.460571319782,20.));
#80225=CARTESIAN_POINT('Ctrl Pts',(-45.6935594731126,17.4909412664519,0.));
#80226=CARTESIAN_POINT('Ctrl Pts',(-45.6935594731126,17.4909412664519,20.));
#80227=CARTESIAN_POINT('Ctrl Pts',(-45.6786625986401,17.5212999627071,0.));
#80228=CARTESIAN_POINT('Ctrl Pts',(-45.6786625986401,17.5212999627071,20.));
#80229=CARTESIAN_POINT('Ctrl Pts',(-45.6637453217655,17.5516473948116,0.));
#80230=CARTESIAN_POINT('Ctrl Pts',(-45.6637453217655,17.5516473948116,20.));
#80231=CARTESIAN_POINT('Ctrl Pts',(-45.6488076502485,17.5819835489016,0.));
#80232=CARTESIAN_POINT('Ctrl Pts',(-45.6488076502485,17.5819835489016,20.));
#80233=CARTESIAN_POINT('Ctrl Pts',(-45.6338495919363,17.6123084109793,0.));
#80234=CARTESIAN_POINT('Ctrl Pts',(-45.6338495919363,17.6123084109793,20.));
#80235=CARTESIAN_POINT('Ctrl Pts',(-45.6188711547313,17.6426219669711,0.));
#80236=CARTESIAN_POINT('Ctrl Pts',(-45.6188711547313,17.6426219669711,20.));
#80237=CARTESIAN_POINT('Ctrl Pts',(-45.6038723465685,17.672924202767,0.));
#80238=CARTESIAN_POINT('Ctrl Pts',(-45.6038723465685,17.672924202767,20.));
#80239=CARTESIAN_POINT('Ctrl Pts',(-45.5888531753912,17.7032151042645,0.));
#80240=CARTESIAN_POINT('Ctrl Pts',(-45.5888531753912,17.7032151042645,20.));
#80241=CARTESIAN_POINT('Ctrl Pts',(-45.5738136491221,17.7334946574206,0.));
#80242=CARTESIAN_POINT('Ctrl Pts',(-45.5738136491221,17.7334946574206,20.));
#80243=CARTESIAN_POINT('Ctrl Pts',(-45.5587537756595,17.7637628482589,0.));
#80244=CARTESIAN_POINT('Ctrl Pts',(-45.5587537756595,17.7637628482589,20.));
#80245=CARTESIAN_POINT('Ctrl Pts',(-45.5436735628911,17.7940196628442,0.));
#80246=CARTESIAN_POINT('Ctrl Pts',(-45.5436735628911,17.7940196628442,20.));
#80247=CARTESIAN_POINT('Ctrl Pts',(-45.528573018704,17.8242650872661,0.));
#80248=CARTESIAN_POINT('Ctrl Pts',(-45.528573018704,17.8242650872661,20.));
#80249=CARTESIAN_POINT('Ctrl Pts',(-45.5134521509949,17.8544991076191,0.));
#80250=CARTESIAN_POINT('Ctrl Pts',(-45.5134521509949,17.8544991076191,20.));
#80251=CARTESIAN_POINT('Ctrl Pts',(-45.498310967683,17.8847217099814,0.));
#80252=CARTESIAN_POINT('Ctrl Pts',(-45.498310967683,17.8847217099814,20.));
#80253=CARTESIAN_POINT('Ctrl Pts',(-45.4831494767122,17.9149328804084,0.));
#80254=CARTESIAN_POINT('Ctrl Pts',(-45.4831494767122,17.9149328804084,20.));
#80255=CARTESIAN_POINT('Ctrl Pts',(-45.4679676860453,17.9451326049449,0.));
#80256=CARTESIAN_POINT('Ctrl Pts',(-45.4679676860453,17.9451326049449,20.));
#80257=CARTESIAN_POINT('Ctrl Pts',(-45.4527656036598,17.9753208696315,0.));
#80258=CARTESIAN_POINT('Ctrl Pts',(-45.4527656036598,17.9753208696315,20.));
#80259=CARTESIAN_POINT('Ctrl Pts',(-45.4375432375433,18.0054976605137,0.));
#80260=CARTESIAN_POINT('Ctrl Pts',(-45.4375432375433,18.0054976605137,20.));
#80261=CARTESIAN_POINT('Ctrl Pts',(-45.4223005956881,18.0356629636502,0.));
#80262=CARTESIAN_POINT('Ctrl Pts',(-45.4223005956881,18.0356629636502,20.));
#80263=CARTESIAN_POINT('Ctrl Pts',(-45.4070376860893,18.0658167651176,0.));
#80264=CARTESIAN_POINT('Ctrl Pts',(-45.4070376860893,18.0658167651176,20.));
#80265=CARTESIAN_POINT('Ctrl Pts',(-45.3917545167484,18.0959590510046,0.));
#80266=CARTESIAN_POINT('Ctrl Pts',(-45.3917545167484,18.0959590510046,20.));
#80267=CARTESIAN_POINT('Ctrl Pts',(-45.3764510956741,18.1260898074095,0.));
#80268=CARTESIAN_POINT('Ctrl Pts',(-45.3764510956741,18.1260898074095,20.));
#80269=CARTESIAN_POINT('Ctrl Pts',(-45.3611274308852,18.156209020436,0.));
#80270=CARTESIAN_POINT('Ctrl Pts',(-45.3611274308852,18.156209020436,20.));
#80271=CARTESIAN_POINT('Ctrl Pts',(-45.345783530412,18.1863166761897,0.));
#80272=CARTESIAN_POINT('Ctrl Pts',(-45.345783530412,18.1863166761897,20.));
#80273=CARTESIAN_POINT('Ctrl Pts',(-45.3304194022976,18.216412760776,0.));
#80274=CARTESIAN_POINT('Ctrl Pts',(-45.3304194022976,18.216412760776,20.));
#80275=CARTESIAN_POINT('Ctrl Pts',(-45.3150350545965,18.2464972603023,0.));
#80276=CARTESIAN_POINT('Ctrl Pts',(-45.3150350545965,18.2464972603023,20.));
#80277=CARTESIAN_POINT('Ctrl Pts',(-45.299630495374,18.2765701608789,0.));
#80278=CARTESIAN_POINT('Ctrl Pts',(-45.299630495374,18.2765701608789,20.));
#80279=CARTESIAN_POINT('Ctrl Pts',(-45.2842057327049,18.3066314486214,0.));
#80280=CARTESIAN_POINT('Ctrl Pts',(-45.2842057327049,18.3066314486214,20.));
#80281=CARTESIAN_POINT('Ctrl Pts',(-45.2687607746732,18.3366811096519,0.));
#80282=CARTESIAN_POINT('Ctrl Pts',(-45.2687607746732,18.3366811096519,20.));
#80283=CARTESIAN_POINT('Ctrl Pts',(-45.2532956293718,18.3667191300999,0.));
#80284=CARTESIAN_POINT('Ctrl Pts',(-45.2532956293718,18.3667191300999,20.));
#80285=CARTESIAN_POINT('Ctrl Pts',(-45.2378103049023,18.3967454961016,0.));
#80286=CARTESIAN_POINT('Ctrl Pts',(-45.2378103049023,18.3967454961016,20.));
#80287=CARTESIAN_POINT('Ctrl Pts',(-45.2223048093755,18.4267601937997,0.));
#80288=CARTESIAN_POINT('Ctrl Pts',(-45.2223048093755,18.4267601937997,20.));
#80289=CARTESIAN_POINT('Ctrl Pts',(-45.2067791509123,18.456763209342,0.));
#80290=CARTESIAN_POINT('Ctrl Pts',(-45.2067791509123,18.456763209342,20.));
#80291=CARTESIAN_POINT('Ctrl Pts',(-45.1912333376434,18.4867545288811,0.));
#80292=CARTESIAN_POINT('Ctrl Pts',(-45.1912333376434,18.4867545288811,20.));
#80293=CARTESIAN_POINT('Ctrl Pts',(-45.1756673777099,18.5167341385735,0.));
#80294=CARTESIAN_POINT('Ctrl Pts',(-45.1756673777099,18.5167341385735,20.));
#80295=CARTESIAN_POINT('Ctrl Pts',(-45.1600812792631,18.5467020245809,0.));
#80296=CARTESIAN_POINT('Ctrl Pts',(-45.1600812792631,18.5467020245809,20.));
#80297=CARTESIAN_POINT('Ctrl Pts',(-45.144475050464,18.5766581730694,0.));
#80298=CARTESIAN_POINT('Ctrl Pts',(-45.144475050464,18.5766581730694,20.));
#80299=CARTESIAN_POINT('Ctrl Pts',(-45.1288486994834,18.6066025702106,0.));
#80300=CARTESIAN_POINT('Ctrl Pts',(-45.1288486994834,18.6066025702106,20.));
#80301=CARTESIAN_POINT('Ctrl Pts',(-45.1132022345013,18.6365352021813,0.));
#80302=CARTESIAN_POINT('Ctrl Pts',(-45.1132022345013,18.6365352021813,20.));
#80303=CARTESIAN_POINT('Ctrl Pts',(-45.097535663708,18.6664560551643,0.));
#80304=CARTESIAN_POINT('Ctrl Pts',(-45.097535663708,18.6664560551643,20.));
#80305=CARTESIAN_POINT('Ctrl Pts',(-45.081848995303,18.6963651153477,0.));
#80306=CARTESIAN_POINT('Ctrl Pts',(-45.081848995303,18.6963651153477,20.));
#80307=CARTESIAN_POINT('Ctrl Pts',(-45.0661422374956,18.7262623689254,0.));
#80308=CARTESIAN_POINT('Ctrl Pts',(-45.0661422374956,18.7262623689254,20.));
#80309=CARTESIAN_POINT('Ctrl Pts',(-45.050415398505,18.7561478020964,0.));
#80310=CARTESIAN_POINT('Ctrl Pts',(-45.050415398505,18.7561478020964,20.));
#80311=CARTESIAN_POINT('Ctrl Pts',(-45.0346684865594,18.7860214010651,0.));
#80312=CARTESIAN_POINT('Ctrl Pts',(-45.0346684865594,18.7860214010651,20.));
#80313=CARTESIAN_POINT('Ctrl Pts',(-45.0189015098976,18.815883152041,0.));
#80314=CARTESIAN_POINT('Ctrl Pts',(-45.0189015098976,18.815883152041,20.));
#80315=CARTESIAN_POINT('Ctrl Pts',(-45.0031144767678,18.8457330412389,0.));
#80316=CARTESIAN_POINT('Ctrl Pts',(-45.0031144767678,18.8457330412389,20.));
#80317=CARTESIAN_POINT('Ctrl Pts',(-44.9873073954281,18.8755710548787,0.));
#80318=CARTESIAN_POINT('Ctrl Pts',(-44.9873073954281,18.8755710548787,20.));
#80319=CARTESIAN_POINT('Ctrl Pts',(-44.971480274146,18.9053971791858,0.));
#80320=CARTESIAN_POINT('Ctrl Pts',(-44.971480274146,18.9053971791858,20.));
#80321=CARTESIAN_POINT('Ctrl Pts',(-44.9556331211993,18.9352114003906,0.));
#80322=CARTESIAN_POINT('Ctrl Pts',(-44.9556331211993,18.9352114003906,20.));
#80323=CARTESIAN_POINT('Ctrl Pts',(-44.9397659448753,18.9650137047293,0.));
#80324=CARTESIAN_POINT('Ctrl Pts',(-44.9397659448753,18.9650137047293,20.));
#80325=CARTESIAN_POINT('Ctrl Pts',(-44.9238787534705,18.9948040784434,0.));
#80326=CARTESIAN_POINT('Ctrl Pts',(-44.9238787534705,18.9948040784434,20.));
#80327=CARTESIAN_POINT('Ctrl Pts',(-44.9079715552916,19.0245825077797,0.));
#80328=CARTESIAN_POINT('Ctrl Pts',(-44.9079715552916,19.0245825077797,20.));
#80329=CARTESIAN_POINT('Ctrl Pts',(-44.8920443586544,19.0543489789907,0.));
#80330=CARTESIAN_POINT('Ctrl Pts',(-44.8920443586544,19.0543489789907,20.));
#80331=CARTESIAN_POINT('Ctrl Pts',(-44.8760971718851,19.0841034783341,0.));
#80332=CARTESIAN_POINT('Ctrl Pts',(-44.8760971718851,19.0841034783341,20.));
#80333=CARTESIAN_POINT('Ctrl Pts',(-44.8601300033192,19.1138459920731,0.));
#80334=CARTESIAN_POINT('Ctrl Pts',(-44.8601300033192,19.1138459920731,20.));
#80335=CARTESIAN_POINT('Ctrl Pts',(-44.8441428613021,19.143576506476,0.));
#80336=CARTESIAN_POINT('Ctrl Pts',(-44.8441428613021,19.143576506476,20.));
#80337=CARTESIAN_POINT('Ctrl Pts',(-44.8281357541891,19.1732950078168,0.));
#80338=CARTESIAN_POINT('Ctrl Pts',(-44.8281357541891,19.1732950078168,20.));
#80339=CARTESIAN_POINT('Ctrl Pts',(-44.8121086903447,19.2030014823748,0.));
#80340=CARTESIAN_POINT('Ctrl Pts',(-44.8121086903447,19.2030014823748,20.));
#80341=CARTESIAN_POINT('Ctrl Pts',(-44.7960616781431,19.2326959164344,0.));
#80342=CARTESIAN_POINT('Ctrl Pts',(-44.7960616781431,19.2326959164344,20.));
#80343=CARTESIAN_POINT('Ctrl Pts',(-44.7799947259683,19.2623782962858,0.));
#80344=CARTESIAN_POINT('Ctrl Pts',(-44.7799947259683,19.2623782962858,20.));
#80345=CARTESIAN_POINT('Ctrl Pts',(-44.7639078422139,19.2920486082247,0.));
#80346=CARTESIAN_POINT('Ctrl Pts',(-44.7639078422139,19.2920486082247,20.));
#80347=CARTESIAN_POINT('Ctrl Pts',(-44.7478010352831,19.3217068385519,0.));
#80348=CARTESIAN_POINT('Ctrl Pts',(-44.7478010352831,19.3217068385519,20.));
#80349=CARTESIAN_POINT('Ctrl Pts',(-44.731674313589,19.3513529735741,0.));
#80350=CARTESIAN_POINT('Ctrl Pts',(-44.731674313589,19.3513529735741,20.));
#80351=CARTESIAN_POINT('Ctrl Pts',(-44.7155276855546,19.3809869996033,0.));
#80352=CARTESIAN_POINT('Ctrl Pts',(-44.7155276855546,19.3809869996033,20.));
#80353=CARTESIAN_POINT('Ctrl Pts',(-44.6993611596123,19.4106089029568,0.));
#80354=CARTESIAN_POINT('Ctrl Pts',(-44.6993611596123,19.4106089029568,20.));
#80355=CARTESIAN_POINT('Ctrl Pts',(-44.6831747442042,19.4402186699576,0.));
#80356=CARTESIAN_POINT('Ctrl Pts',(-44.6831747442042,19.4402186699576,20.));
#80357=CARTESIAN_POINT('Ctrl Pts',(-44.666968447782,19.4698162869338,0.));
#80358=CARTESIAN_POINT('Ctrl Pts',(-44.666968447782,19.4698162869338,20.));
#80359=CARTESIAN_POINT('Ctrl Pts',(-44.6507422788067,19.4994017402193,0.));
#80360=CARTESIAN_POINT('Ctrl Pts',(-44.6507422788067,19.4994017402193,20.));
#80361=CARTESIAN_POINT('Ctrl Pts',(-44.6344962457493,19.5289750161533,0.));
#80362=CARTESIAN_POINT('Ctrl Pts',(-44.6344962457493,19.5289750161533,20.));
#80363=CARTESIAN_POINT('Ctrl Pts',(-44.6182303570903,19.5585361010809,0.));
#80364=CARTESIAN_POINT('Ctrl Pts',(-44.6182303570903,19.5585361010809,20.));
#80365=CARTESIAN_POINT('Ctrl Pts',(-44.60194462132,19.5880849813525,0.));
#80366=CARTESIAN_POINT('Ctrl Pts',(-44.60194462132,19.5880849813525,20.));
#80367=CARTESIAN_POINT('Ctrl Pts',(-44.5856390469384,19.6176216433241,0.));
#80368=CARTESIAN_POINT('Ctrl Pts',(-44.5856390469384,19.6176216433241,20.));
#80369=CARTESIAN_POINT('Ctrl Pts',(-44.5693136424549,19.6471460733568,0.));
#80370=CARTESIAN_POINT('Ctrl Pts',(-44.5693136424549,19.6471460733568,20.));
#80371=CARTESIAN_POINT('Ctrl Pts',(-44.5529684163885,19.6766582578175,0.));
#80372=CARTESIAN_POINT('Ctrl Pts',(-44.5529684163885,19.6766582578175,20.));
#80373=CARTESIAN_POINT('Ctrl Pts',(-44.5366033772682,19.7061581830785,0.));
#80374=CARTESIAN_POINT('Ctrl Pts',(-44.5366033772682,19.7061581830785,20.));
#80375=CARTESIAN_POINT('Ctrl Pts',(-44.5202185336324,19.7356458355178,0.));
#80376=CARTESIAN_POINT('Ctrl Pts',(-44.5202185336324,19.7356458355178,20.));
#80377=CARTESIAN_POINT('Ctrl Pts',(-44.5038138940293,19.7651212015191,0.));
#80378=CARTESIAN_POINT('Ctrl Pts',(-44.5038138940293,19.7651212015191,20.));
#80379=CARTESIAN_POINT('Ctrl Pts',(-44.4873894670167,19.7945842674717,0.));
#80380=CARTESIAN_POINT('Ctrl Pts',(-44.4873894670167,19.7945842674717,20.));
#80381=CARTESIAN_POINT('Ctrl Pts',(-44.4709452611615,19.8240350197702,0.));
#80382=CARTESIAN_POINT('Ctrl Pts',(-44.4709452611615,19.8240350197702,20.));
#80383=CARTESIAN_POINT('Ctrl Pts',(-44.4544812850403,19.8534734448146,0.));
#80384=CARTESIAN_POINT('Ctrl Pts',(-44.4544812850403,19.8534734448146,20.));
#80385=CARTESIAN_POINT('Ctrl Pts',(-44.4379975472397,19.8828995290107,0.));
#80386=CARTESIAN_POINT('Ctrl Pts',(-44.4379975472397,19.8828995290107,20.));
#80387=CARTESIAN_POINT('Ctrl Pts',(-44.4214940563557,19.9123132587697,0.));
#80388=CARTESIAN_POINT('Ctrl Pts',(-44.4214940563557,19.9123132587697,20.));
#80389=CARTESIAN_POINT('Ctrl Pts',(-44.4049708209939,19.9417146205087,0.));
#80390=CARTESIAN_POINT('Ctrl Pts',(-44.4049708209939,19.9417146205087,20.));
#80391=CARTESIAN_POINT('Ctrl Pts',(-44.3884278497697,19.9711036006503,0.));
#80392=CARTESIAN_POINT('Ctrl Pts',(-44.3884278497697,19.9711036006503,20.));
#80393=CARTESIAN_POINT('Ctrl Pts',(-44.371865151308,20.0004801856228,0.));
#80394=CARTESIAN_POINT('Ctrl Pts',(-44.371865151308,20.0004801856228,20.));
#80395=CARTESIAN_POINT('Ctrl Pts',(-44.3552827342435,20.0298443618602,0.));
#80396=CARTESIAN_POINT('Ctrl Pts',(-44.3552827342435,20.0298443618602,20.));
#80397=CARTESIAN_POINT('Ctrl Pts',(-44.3386806072204,20.0591961158018,0.));
#80398=CARTESIAN_POINT('Ctrl Pts',(-44.3386806072204,20.0591961158018,20.));
#80399=CARTESIAN_POINT('Ctrl Pts',(-44.3220587788923,20.0885354338929,0.));
#80400=CARTESIAN_POINT('Ctrl Pts',(-44.3220587788923,20.0885354338929,20.));
#80401=CARTESIAN_POINT('Ctrl Pts',(-44.3054172579222,20.117862302584,0.));
#80402=CARTESIAN_POINT('Ctrl Pts',(-44.3054172579222,20.117862302584,20.));
#80403=CARTESIAN_POINT('Ctrl Pts',(-44.2887560529826,20.1471767083313,0.));
#80404=CARTESIAN_POINT('Ctrl Pts',(-44.2887560529826,20.1471767083313,20.));
#80405=CARTESIAN_POINT('Ctrl Pts',(-44.2720751727557,20.1764786375963,0.));
#80406=CARTESIAN_POINT('Ctrl Pts',(-44.2720751727557,20.1764786375963,20.));
#80407=CARTESIAN_POINT('Ctrl Pts',(-44.2553746259333,20.2057680768465,0.));
#80408=CARTESIAN_POINT('Ctrl Pts',(-44.2553746259333,20.2057680768465,20.));
#80409=CARTESIAN_POINT('Ctrl Pts',(-44.238654421217,20.2350450125552,0.));
#80410=CARTESIAN_POINT('Ctrl Pts',(-44.238654421217,20.2350450125552,20.));
#80411=CARTESIAN_POINT('Ctrl Pts',(-44.221914567318,20.2643094312016,0.));
#80412=CARTESIAN_POINT('Ctrl Pts',(-44.221914567318,20.2643094312016,20.));
#80413=CARTESIAN_POINT('Ctrl Pts',(-44.205155072957,20.2935613192706,0.));
#80414=CARTESIAN_POINT('Ctrl Pts',(-44.205155072957,20.2935613192706,20.));
#80415=CARTESIAN_POINT('Ctrl Pts',(-44.1883759468646,20.3228006632528,0.));
#80416=CARTESIAN_POINT('Ctrl Pts',(-44.1883759468646,20.3228006632528,20.));
#80417=CARTESIAN_POINT('Ctrl Pts',(-44.1715771977807,20.3520274496443,0.));
#80418=CARTESIAN_POINT('Ctrl Pts',(-44.1715771977807,20.3520274496443,20.));
#80419=CARTESIAN_POINT('Ctrl Pts',(-44.1547588344544,20.3812416649468,0.));
#80420=CARTESIAN_POINT('Ctrl Pts',(-44.1547588344544,20.3812416649468,20.));
#80421=CARTESIAN_POINT('Ctrl Pts',(-44.1379208656442,20.4104432956673,0.));
#80422=CARTESIAN_POINT('Ctrl Pts',(-44.1379208656442,20.4104432956673,20.));
#80423=CARTESIAN_POINT('Ctrl Pts',(-44.1210633001184,20.4396323283186,0.));
#80424=CARTESIAN_POINT('Ctrl Pts',(-44.1210633001184,20.4396323283186,20.));
#80425=CARTESIAN_POINT('Ctrl Pts',(-44.1041861466545,20.468808749419,0.));
#80426=CARTESIAN_POINT('Ctrl Pts',(-44.1041861466545,20.468808749419,20.));
#80427=CARTESIAN_POINT('Ctrl Pts',(-44.0872894140398,20.4979725454932,0.));
#80428=CARTESIAN_POINT('Ctrl Pts',(-44.0872894140398,20.4979725454932,20.));
#80429=CARTESIAN_POINT('Ctrl Pts',(-44.0703731110714,20.5271237030716,0.));
#80430=CARTESIAN_POINT('Ctrl Pts',(-44.0703731110714,20.5271237030716,20.));
#80431=CARTESIAN_POINT('Ctrl Pts',(-44.053437246556,20.5562622086905,0.));
#80432=CARTESIAN_POINT('Ctrl Pts',(-44.053437246556,20.5562622086905,20.));
#80433=CARTESIAN_POINT('Ctrl Pts',(-44.03648182931,20.5853880488919,0.));
#80434=CARTESIAN_POINT('Ctrl Pts',(-44.03648182931,20.5853880488919,20.));
#80435=CARTESIAN_POINT('Ctrl Pts',(-44.0195068681592,20.6145012102233,0.));
#80436=CARTESIAN_POINT('Ctrl Pts',(-44.0195068681592,20.6145012102233,20.));
#80437=CARTESIAN_POINT('Ctrl Pts',(-44.0025123719387,20.6436016792381,0.));
#80438=CARTESIAN_POINT('Ctrl Pts',(-44.0025123719387,20.6436016792381,20.));
#80439=CARTESIAN_POINT('Ctrl Pts',(-43.9854983494929,20.6726894424949,0.));
#80440=CARTESIAN_POINT('Ctrl Pts',(-43.9854983494929,20.6726894424949,20.));
#80441=CARTESIAN_POINT('Ctrl Pts',(-43.9684648096756,20.7017644865584,0.));
#80442=CARTESIAN_POINT('Ctrl Pts',(-43.9684648096756,20.7017644865584,20.));
#80443=CARTESIAN_POINT('Ctrl Pts',(-43.9514117613501,20.7308267979991,0.));
#80444=CARTESIAN_POINT('Ctrl Pts',(-43.9514117613501,20.7308267979991,20.));
#80445=CARTESIAN_POINT('Ctrl Pts',(-43.9343392133895,20.7598763633934,0.));
#80446=CARTESIAN_POINT('Ctrl Pts',(-43.9343392133895,20.7598763633934,20.));
#80447=CARTESIAN_POINT('Ctrl Pts',(-43.9172471746767,20.7889131693233,0.));
#80448=CARTESIAN_POINT('Ctrl Pts',(-43.9172471746767,20.7889131693233,20.));
#80449=CARTESIAN_POINT('Ctrl Pts',(-43.9001356541037,20.817937202377,0.));
#80450=CARTESIAN_POINT('Ctrl Pts',(-43.9001356541037,20.817937202377,20.));
#80451=CARTESIAN_POINT('Ctrl Pts',(-43.8830046605723,20.8469484491482,0.));
#80452=CARTESIAN_POINT('Ctrl Pts',(-43.8830046605723,20.8469484491482,20.));
#80453=CARTESIAN_POINT('Ctrl Pts',(-43.8658542029936,20.8759468962364,0.));
#80454=CARTESIAN_POINT('Ctrl Pts',(-43.8658542029936,20.8759468962364,20.));
#80455=CARTESIAN_POINT('Ctrl Pts',(-43.8486842902882,20.9049325302471,0.));
#80456=CARTESIAN_POINT('Ctrl Pts',(-43.8486842902882,20.9049325302471,20.));
#80457=CARTESIAN_POINT('Ctrl Pts',(-43.8314949313861,20.9339053377913,0.));
#80458=CARTESIAN_POINT('Ctrl Pts',(-43.8314949313861,20.9339053377913,20.));
#80459=CARTESIAN_POINT('Ctrl Pts',(-43.8142861352268,20.9628653054863,0.));
#80460=CARTESIAN_POINT('Ctrl Pts',(-43.8142861352268,20.9628653054863,20.));
#80461=CARTESIAN_POINT('Ctrl Pts',(-43.7970579107591,20.9918124199547,0.));
#80462=CARTESIAN_POINT('Ctrl Pts',(-43.7970579107591,20.9918124199547,20.));
#80463=CARTESIAN_POINT('Ctrl Pts',(-43.7798102669417,21.0207466678254,0.));
#80464=CARTESIAN_POINT('Ctrl Pts',(-43.7798102669417,21.0207466678254,20.));
#80465=CARTESIAN_POINT('Ctrl Pts',(-43.7625432127426,21.0496680357328,0.));
#80466=CARTESIAN_POINT('Ctrl Pts',(-43.7625432127426,21.0496680357328,20.));
#80467=CARTESIAN_POINT('Ctrl Pts',(-43.7452567571393,21.0785765103172,0.));
#80468=CARTESIAN_POINT('Ctrl Pts',(-43.7452567571393,21.0785765103172,20.));
#80469=CARTESIAN_POINT('Ctrl Pts',(-43.7279509091188,21.1074720782252,0.));
#80470=CARTESIAN_POINT('Ctrl Pts',(-43.7279509091188,21.1074720782252,20.));
#80471=CARTESIAN_POINT('Ctrl Pts',(-43.7106256776774,21.1363547261089,0.));
#80472=CARTESIAN_POINT('Ctrl Pts',(-43.7106256776774,21.1363547261089,20.));
#80473=CARTESIAN_POINT('Ctrl Pts',(-43.6932810718209,21.1652244406266,0.));
#80474=CARTESIAN_POINT('Ctrl Pts',(-43.6932810718209,21.1652244406266,20.));
#80475=CARTESIAN_POINT('Ctrl Pts',(-43.6759171005642,21.1940812084419,0.));
#80476=CARTESIAN_POINT('Ctrl Pts',(-43.6759171005642,21.1940812084419,20.));
#80477=CARTESIAN_POINT('Ctrl Pts',(-43.658533772932,21.2229250162246,0.));
#80478=CARTESIAN_POINT('Ctrl Pts',(-43.658533772932,21.2229250162246,20.));
#80479=CARTESIAN_POINT('Ctrl Pts',(-43.6411310979585,21.2517558506503,0.));
#80480=CARTESIAN_POINT('Ctrl Pts',(-43.6411310979585,21.2517558506503,20.));
#80481=CARTESIAN_POINT('Ctrl Pts',(-43.6237090846874,21.2805736984007,0.));
#80482=CARTESIAN_POINT('Ctrl Pts',(-43.6237090846874,21.2805736984007,20.));
#80483=CARTESIAN_POINT('Ctrl Pts',(-43.6062677421718,21.3093785461635,0.));
#80484=CARTESIAN_POINT('Ctrl Pts',(-43.6062677421718,21.3093785461635,20.));
#80485=CARTESIAN_POINT('Ctrl Pts',(-43.5888070794743,21.3381703806323,0.));
#80486=CARTESIAN_POINT('Ctrl Pts',(-43.5888070794743,21.3381703806323,20.));
#80487=CARTESIAN_POINT('Ctrl Pts',(-43.571327105667,21.3669491885068,0.));
#80488=CARTESIAN_POINT('Ctrl Pts',(-43.571327105667,21.3669491885068,20.));
#80489=CARTESIAN_POINT('Ctrl Pts',(-43.5538278298311,21.3957149564922,0.));
#80490=CARTESIAN_POINT('Ctrl Pts',(-43.5538278298311,21.3957149564922,20.));
#80491=CARTESIAN_POINT('Ctrl Pts',(-43.5363092610574,21.4244676712999,0.));
#80492=CARTESIAN_POINT('Ctrl Pts',(-43.5363092610574,21.4244676712999,20.));
#80493=CARTESIAN_POINT('Ctrl Pts',(-43.5187714084458,21.4532073196468,0.));
#80494=CARTESIAN_POINT('Ctrl Pts',(-43.5187714084458,21.4532073196468,20.));
#80495=CARTESIAN_POINT('Ctrl Pts',(-43.5012142811058,21.4819338882558,0.));
#80496=CARTESIAN_POINT('Ctrl Pts',(-43.5012142811058,21.4819338882558,20.));
#80497=CARTESIAN_POINT('Ctrl Pts',(-43.4836378881563,21.5106473638561,0.));
#80498=CARTESIAN_POINT('Ctrl Pts',(-43.4836378881563,21.5106473638561,20.));
#80499=CARTESIAN_POINT('Ctrl Pts',(-43.4660422387257,21.5393477331829,0.));
#80500=CARTESIAN_POINT('Ctrl Pts',(-43.4660422387257,21.5393477331829,20.));
#80501=CARTESIAN_POINT('Ctrl Pts',(-43.4484273419519,21.5680349829773,0.));
#80502=CARTESIAN_POINT('Ctrl Pts',(-43.4484273419519,21.5680349829773,20.));
#80503=CARTESIAN_POINT('Ctrl Pts',(-43.4307932069824,21.5967090999869,0.));
#80504=CARTESIAN_POINT('Ctrl Pts',(-43.4307932069824,21.5967090999869,20.));
#80505=CARTESIAN_POINT('Ctrl Pts',(-43.4131398429739,21.6253700709647,0.));
#80506=CARTESIAN_POINT('Ctrl Pts',(-43.4131398429739,21.6253700709647,20.));
#80507=CARTESIAN_POINT('Ctrl Pts',(-43.3954672590924,21.6540178826698,0.));
#80508=CARTESIAN_POINT('Ctrl Pts',(-43.3954672590924,21.6540178826698,20.));
#80509=CARTESIAN_POINT('Ctrl Pts',(-43.3777754645132,21.682652521867,0.));
#80510=CARTESIAN_POINT('Ctrl Pts',(-43.3777754645132,21.682652521867,20.));
#80511=CARTESIAN_POINT('Ctrl Pts',(-43.3600644684208,21.7112739753274,0.));
#80512=CARTESIAN_POINT('Ctrl Pts',(-43.3600644684208,21.7112739753274,20.));
#80513=CARTESIAN_POINT('Ctrl Pts',(-43.3423342800096,21.7398822298281,0.));
#80514=CARTESIAN_POINT('Ctrl Pts',(-43.3423342800096,21.7398822298281,20.));
#80515=CARTESIAN_POINT('Ctrl Pts',(-43.3245849084831,21.7684772721522,0.));
#80516=CARTESIAN_POINT('Ctrl Pts',(-43.3245849084831,21.7684772721522,20.));
#80517=CARTESIAN_POINT('Ctrl Pts',(-43.3068163630542,21.7970590890891,0.));
#80518=CARTESIAN_POINT('Ctrl Pts',(-43.3068163630542,21.7970590890891,20.));
#80519=CARTESIAN_POINT('Ctrl Pts',(-43.2890286529453,21.8256276674339,0.));
#80520=CARTESIAN_POINT('Ctrl Pts',(-43.2890286529453,21.8256276674339,20.));
#80521=CARTESIAN_POINT('Ctrl Pts',(-43.271221787388,21.8541829939879,0.));
#80522=CARTESIAN_POINT('Ctrl Pts',(-43.271221787388,21.8541829939879,20.));
#80523=CARTESIAN_POINT('Ctrl Pts',(-43.2533957756234,21.8827250555583,0.));
#80524=CARTESIAN_POINT('Ctrl Pts',(-43.2533957756234,21.8827250555583,20.));
#80525=CARTESIAN_POINT('Ctrl Pts',(-43.2355506269018,21.9112538389585,0.));
#80526=CARTESIAN_POINT('Ctrl Pts',(-43.2355506269018,21.9112538389585,20.));
#80527=CARTESIAN_POINT('Ctrl Pts',(-43.217686350483,21.9397693310079,0.));
#80528=CARTESIAN_POINT('Ctrl Pts',(-43.217686350483,21.9397693310079,20.));
#80529=CARTESIAN_POINT('Ctrl Pts',(-43.1998029556363,21.9682715185322,0.));
#80530=CARTESIAN_POINT('Ctrl Pts',(-43.1998029556363,21.9682715185322,20.));
#80531=CARTESIAN_POINT('Ctrl Pts',(-43.1819004516401,21.9967603883628,0.));
#80532=CARTESIAN_POINT('Ctrl Pts',(-43.1819004516401,21.9967603883628,20.));
#80533=CARTESIAN_POINT('Ctrl Pts',(-43.1639788477821,22.0252359273373,0.));
#80534=CARTESIAN_POINT('Ctrl Pts',(-43.1639788477821,22.0252359273373,20.));
#80535=CARTESIAN_POINT('Ctrl Pts',(-43.1460381533594,22.0536981222997,0.));
#80536=CARTESIAN_POINT('Ctrl Pts',(-43.1460381533594,22.0536981222997,20.));
#80537=CARTESIAN_POINT('Ctrl Pts',(-43.1280783776785,22.0821469600997,0.));
#80538=CARTESIAN_POINT('Ctrl Pts',(-43.1280783776785,22.0821469600997,20.));
#80539=CARTESIAN_POINT('Ctrl Pts',(-43.1100995300552,22.1105824275933,0.));
#80540=CARTESIAN_POINT('Ctrl Pts',(-43.1100995300552,22.1105824275933,20.));
#80541=CARTESIAN_POINT('Ctrl Pts',(-43.0921016198148,22.1390045116426,0.));
#80542=CARTESIAN_POINT('Ctrl Pts',(-43.0921016198148,22.1390045116426,20.));
#80543=CARTESIAN_POINT('Ctrl Pts',(-43.0740846562917,22.1674131991155,0.));
#80544=CARTESIAN_POINT('Ctrl Pts',(-43.0740846562917,22.1674131991155,20.));
#80545=CARTESIAN_POINT('Ctrl Pts',(-43.0560486488298,22.1958084768867,0.));
#80546=CARTESIAN_POINT('Ctrl Pts',(-43.0560486488298,22.1958084768867,20.));
#80547=CARTESIAN_POINT('Ctrl Pts',(-43.0379936067822,22.2241903318366,0.));
#80548=CARTESIAN_POINT('Ctrl Pts',(-43.0379936067822,22.2241903318366,20.));
#80549=CARTESIAN_POINT('Ctrl Pts',(-43.0199195395115,22.252558750852,0.));
#80550=CARTESIAN_POINT('Ctrl Pts',(-43.0199195395115,22.252558750852,20.));
#80551=CARTESIAN_POINT('Ctrl Pts',(-43.0018264563892,22.2809137208256,0.));
#80552=CARTESIAN_POINT('Ctrl Pts',(-43.0018264563892,22.2809137208256,20.));
#80553=CARTESIAN_POINT('Ctrl Pts',(-42.9837143667966,22.3092552286564,0.));
#80554=CARTESIAN_POINT('Ctrl Pts',(-42.9837143667966,22.3092552286564,20.));
#80555=CARTESIAN_POINT('Ctrl Pts',(-42.965583280124,22.3375832612492,0.));
#80556=CARTESIAN_POINT('Ctrl Pts',(-42.965583280124,22.3375832612492,20.));
#80557=CARTESIAN_POINT('Ctrl Pts',(-42.947433205771,22.3658978055149,0.));
#80558=CARTESIAN_POINT('Ctrl Pts',(-42.947433205771,22.3658978055149,20.));
#80559=CARTESIAN_POINT('Ctrl Pts',(-42.9292641531465,22.3941988483709,0.));
#80560=CARTESIAN_POINT('Ctrl Pts',(-42.9292641531465,22.3941988483709,20.));
#80561=CARTESIAN_POINT('Ctrl Pts',(-42.9110761316689,22.4224863767407,0.));
#80562=CARTESIAN_POINT('Ctrl Pts',(-42.9110761316689,22.4224863767407,20.));
#80563=CARTESIAN_POINT('Ctrl Pts',(-42.8928691507659,22.4507603775546,0.));
#80564=CARTESIAN_POINT('Ctrl Pts',(-42.8928691507659,22.4507603775546,20.));
#80565=CARTESIAN_POINT('Ctrl Pts',(-42.8746432198744,22.4790208377488,0.));
#80566=CARTESIAN_POINT('Ctrl Pts',(-42.8746432198744,22.4790208377488,20.));
#80567=CARTESIAN_POINT('Ctrl Pts',(-42.8563983484404,22.5072677442656,0.));
#80568=CARTESIAN_POINT('Ctrl Pts',(-42.8563983484404,22.5072677442656,20.));
#80569=CARTESIAN_POINT('Ctrl Pts',(-42.8381345459193,22.535501084053,0.));
#80570=CARTESIAN_POINT('Ctrl Pts',(-42.8381345459193,22.535501084053,20.));
#80571=CARTESIAN_POINT('Ctrl Pts',(-42.8198518217756,22.5637208440656,0.));
#80572=CARTESIAN_POINT('Ctrl Pts',(-42.8198518217756,22.5637208440656,20.));
#80573=CARTESIAN_POINT('Ctrl Pts',(-42.8015501854832,22.5919270112639,0.));
#80574=CARTESIAN_POINT('Ctrl Pts',(-42.8015501854832,22.5919270112639,20.));
#80575=CARTESIAN_POINT('Ctrl Pts',(-42.7832296465255,22.620119572615,0.));
#80576=CARTESIAN_POINT('Ctrl Pts',(-42.7832296465255,22.620119572615,20.));
#80577=CARTESIAN_POINT('Ctrl Pts',(-42.7648902143955,22.6482985150925,0.));
#80578=CARTESIAN_POINT('Ctrl Pts',(-42.7648902143955,22.6482985150925,20.));
#80579=CARTESIAN_POINT('Ctrl Pts',(-42.7465318985949,22.6764638256759,0.));
#80580=CARTESIAN_POINT('Ctrl Pts',(-42.7465318985949,22.6764638256759,20.));
#80581=CARTESIAN_POINT('Ctrl Pts',(-42.7281547086347,22.7046154913511,0.));
#80582=CARTESIAN_POINT('Ctrl Pts',(-42.7281547086347,22.7046154913511,20.));
#80583=CARTESIAN_POINT('Ctrl Pts',(-42.7097586540349,22.73275349911,0.));
#80584=CARTESIAN_POINT('Ctrl Pts',(-42.7097586540349,22.73275349911,20.));
#80585=CARTESIAN_POINT('Ctrl Pts',(-42.6913437443248,22.7608778359508,0.));
#80586=CARTESIAN_POINT('Ctrl Pts',(-42.6913437443248,22.7608778359508,20.));
#80587=CARTESIAN_POINT('Ctrl Pts',(-42.6729099890431,22.788988488878,0.));
#80588=CARTESIAN_POINT('Ctrl Pts',(-42.6729099890431,22.788988488878,20.));
#80589=CARTESIAN_POINT('Ctrl Pts',(-42.6544573977378,22.8170854449023,0.));
#80590=CARTESIAN_POINT('Ctrl Pts',(-42.6544573977378,22.8170854449023,20.));
#80591=CARTESIAN_POINT('Ctrl Pts',(-42.6359859799663,22.845168691041,0.));
#80592=CARTESIAN_POINT('Ctrl Pts',(-42.6359859799663,22.845168691041,20.));
#80593=CARTESIAN_POINT('Ctrl Pts',(-42.6174957452953,22.8732382143174,0.));
#80594=CARTESIAN_POINT('Ctrl Pts',(-42.6174957452953,22.8732382143174,20.));
#80595=CARTESIAN_POINT('Ctrl Pts',(-42.5989867033005,22.9012940017616,0.));
#80596=CARTESIAN_POINT('Ctrl Pts',(-42.5989867033005,22.9012940017616,20.));
#80597=CARTESIAN_POINT('Ctrl Pts',(-42.5804588635669,22.9293360404094,0.));
#80598=CARTESIAN_POINT('Ctrl Pts',(-42.5804588635669,22.9293360404094,20.));
#80599=CARTESIAN_POINT('Ctrl Pts',(-42.5619122356886,22.9573643173033,0.));
#80600=CARTESIAN_POINT('Ctrl Pts',(-42.5619122356886,22.9573643173033,20.));
#80601=CARTESIAN_POINT('Ctrl Pts',(-42.5433468292689,22.9853788194919,0.));
#80602=CARTESIAN_POINT('Ctrl Pts',(-42.5433468292689,22.9853788194919,20.));
#80603=CARTESIAN_POINT('Ctrl Pts',(-42.5247626539203,23.0133795340298,0.));
#80604=CARTESIAN_POINT('Ctrl Pts',(-42.5247626539203,23.0133795340298,20.));
#80605=CARTESIAN_POINT('Ctrl Pts',(-42.5061597192647,23.0413664479785,0.));
#80606=CARTESIAN_POINT('Ctrl Pts',(-42.5061597192647,23.0413664479785,20.));
#80607=CARTESIAN_POINT('Ctrl Pts',(-42.4875380349329,23.0693395484056,0.));
#80608=CARTESIAN_POINT('Ctrl Pts',(-42.4875380349329,23.0693395484056,20.));
#80609=CARTESIAN_POINT('Ctrl Pts',(-42.4688976105654,23.0972988223849,0.));
#80610=CARTESIAN_POINT('Ctrl Pts',(-42.4688976105654,23.0972988223849,20.));
#80611=CARTESIAN_POINT('Ctrl Pts',(-42.4502384558115,23.125244256997,0.));
#80612=CARTESIAN_POINT('Ctrl Pts',(-42.4502384558115,23.125244256997,20.));
#80613=CARTESIAN_POINT('Ctrl Pts',(-42.4315605803298,23.1531758393284,0.));
#80614=CARTESIAN_POINT('Ctrl Pts',(-42.4315605803298,23.1531758393284,20.));
#80615=CARTESIAN_POINT('Ctrl Pts',(-42.4128639937879,23.1810935564721,0.));
#80616=CARTESIAN_POINT('Ctrl Pts',(-42.4128639937879,23.1810935564721,20.));
#80617=CARTESIAN_POINT('Ctrl Pts',(-42.3941487058631,23.2089973955278,0.));
#80618=CARTESIAN_POINT('Ctrl Pts',(-42.3941487058631,23.2089973955278,20.));
#80619=CARTESIAN_POINT('Ctrl Pts',(-42.3754147262417,23.2368873436013,0.));
#80620=CARTESIAN_POINT('Ctrl Pts',(-42.3754147262417,23.2368873436013,20.));
#80621=CARTESIAN_POINT('Ctrl Pts',(-42.3566620646188,23.2647633878047,0.));
#80622=CARTESIAN_POINT('Ctrl Pts',(-42.3566620646188,23.2647633878047,20.));
#80623=CARTESIAN_POINT('Ctrl Pts',(-42.3378907306988,23.2926255152563,0.));
#80624=CARTESIAN_POINT('Ctrl Pts',(-42.3378907306988,23.2926255152563,20.));
#80625=CARTESIAN_POINT('Ctrl Pts',(-42.3191007341954,23.320473713081,0.));
#80626=CARTESIAN_POINT('Ctrl Pts',(-42.3191007341954,23.320473713081,20.));
#80627=CARTESIAN_POINT('Ctrl Pts',(-42.3002920848317,23.3483079684103,0.));
#80628=CARTESIAN_POINT('Ctrl Pts',(-42.3002920848317,23.3483079684103,20.));
#80629=CARTESIAN_POINT('Ctrl Pts',(-42.2814647923395,23.3761282683822,0.));
#80630=CARTESIAN_POINT('Ctrl Pts',(-42.2814647923395,23.3761282683822,20.));
#80631=CARTESIAN_POINT('Ctrl Pts',(-42.2626188664603,23.4039346001409,0.));
#80632=CARTESIAN_POINT('Ctrl Pts',(-42.2626188664603,23.4039346001409,20.));
#80633=CARTESIAN_POINT('Ctrl Pts',(-42.2437543169442,23.4317269508371,0.));
#80634=CARTESIAN_POINT('Ctrl Pts',(-42.2437543169442,23.4317269508371,20.));
#80635=CARTESIAN_POINT('Ctrl Pts',(-42.2248711535508,23.4595053076277,0.));
#80636=CARTESIAN_POINT('Ctrl Pts',(-42.2248711535508,23.4595053076277,20.));
#80637=CARTESIAN_POINT('Ctrl Pts',(-42.2059693860486,23.4872696576759,0.));
#80638=CARTESIAN_POINT('Ctrl Pts',(-42.2059693860486,23.4872696576759,20.));
#80639=CARTESIAN_POINT('Ctrl Pts',(-42.1870490242153,23.5150199881514,0.));
#80640=CARTESIAN_POINT('Ctrl Pts',(-42.1870490242153,23.5150199881514,20.));
#80641=CARTESIAN_POINT('Ctrl Pts',(-42.1681100778379,23.5427562862307,0.));
#80642=CARTESIAN_POINT('Ctrl Pts',(-42.1681100778379,23.5427562862307,20.));
#80643=CARTESIAN_POINT('Ctrl Pts',(-42.1491525567126,23.5704785390969,0.));
#80644=CARTESIAN_POINT('Ctrl Pts',(-42.1491525567126,23.5704785390969,20.));
#80645=CARTESIAN_POINT('Ctrl Pts',(-42.1301764706447,23.5981867339394,0.));
#80646=CARTESIAN_POINT('Ctrl Pts',(-42.1301764706447,23.5981867339394,20.));
#80647=CARTESIAN_POINT('Ctrl Pts',(-42.1111818294483,23.6258808579542,0.));
#80648=CARTESIAN_POINT('Ctrl Pts',(-42.1111818294483,23.6258808579542,20.));
#80649=CARTESIAN_POINT('Ctrl Pts',(-42.0921686429469,23.6535608983435,0.));
#80650=CARTESIAN_POINT('Ctrl Pts',(-42.0921686429469,23.6535608983435,20.));
#80651=CARTESIAN_POINT('Ctrl Pts',(-42.0731369209731,23.6812268423159,0.));
#80652=CARTESIAN_POINT('Ctrl Pts',(-42.0731369209731,23.6812268423159,20.));
#80653=CARTESIAN_POINT('Ctrl Pts',(-42.0540866733685,23.7088786770864,0.));
#80654=CARTESIAN_POINT('Ctrl Pts',(-42.0540866733685,23.7088786770864,20.));
#80655=CARTESIAN_POINT('Ctrl Pts',(-42.0350179099839,23.7365163898767,0.));
#80656=CARTESIAN_POINT('Ctrl Pts',(-42.0350179099839,23.7365163898767,20.));
#80657=CARTESIAN_POINT('Ctrl Pts',(-42.0159306406794,23.7641399679152,0.));
#80658=CARTESIAN_POINT('Ctrl Pts',(-42.0159306406794,23.7641399679152,20.));
#80659=CARTESIAN_POINT('Ctrl Pts',(-41.9968248753238,23.7917493984363,0.));
#80660=CARTESIAN_POINT('Ctrl Pts',(-41.9968248753238,23.7917493984363,20.));
#80661=CARTESIAN_POINT('Ctrl Pts',(-41.9777006237952,23.8193446686815,0.));
#80662=CARTESIAN_POINT('Ctrl Pts',(-41.9777006237952,23.8193446686815,20.));
#80663=CARTESIAN_POINT('Ctrl Pts',(-41.9585578959807,23.8469257658985,0.));
#80664=CARTESIAN_POINT('Ctrl Pts',(-41.9585578959807,23.8469257658985,20.));
#80665=CARTESIAN_POINT('Ctrl Pts',(-41.9393967017767,23.8744926773418,0.));
#80666=CARTESIAN_POINT('Ctrl Pts',(-41.9393967017767,23.8744926773418,20.));
#80667=CARTESIAN_POINT('Ctrl Pts',(-41.9202170510888,23.9020453902722,0.));
#80668=CARTESIAN_POINT('Ctrl Pts',(-41.9202170510888,23.9020453902722,20.));
#80669=CARTESIAN_POINT('Ctrl Pts',(-41.9010189538314,23.9295838919572,0.));
#80670=CARTESIAN_POINT('Ctrl Pts',(-41.9010189538314,23.9295838919572,20.));
#80671=CARTESIAN_POINT('Ctrl Pts',(-41.8818024199281,23.9571081696707,0.));
#80672=CARTESIAN_POINT('Ctrl Pts',(-41.8818024199281,23.9571081696707,20.));
#80673=CARTESIAN_POINT('Ctrl Pts',(-41.8625674593112,23.984618210693,0.));
#80674=CARTESIAN_POINT('Ctrl Pts',(-41.8625674593112,23.984618210693,20.));
#80675=CARTESIAN_POINT('Ctrl Pts',(-41.8433140819226,24.0121140023113,0.));
#80676=CARTESIAN_POINT('Ctrl Pts',(-41.8433140819226,24.0121140023113,20.));
#80677=CARTESIAN_POINT('Ctrl Pts',(-41.824042297713,24.0395955318191,0.));
#80678=CARTESIAN_POINT('Ctrl Pts',(-41.824042297713,24.0395955318191,20.));
#80679=CARTESIAN_POINT('Ctrl Pts',(-41.8047521166422,24.0670627865166,0.));
#80680=CARTESIAN_POINT('Ctrl Pts',(-41.8047521166422,24.0670627865166,20.));
#80681=CARTESIAN_POINT('Ctrl Pts',(-41.785443548679,24.0945157537107,0.));
#80682=CARTESIAN_POINT('Ctrl Pts',(-41.785443548679,24.0945157537107,20.));
#80683=CARTESIAN_POINT('Ctrl Pts',(-41.7661166038015,24.1219544207148,0.));
#80684=CARTESIAN_POINT('Ctrl Pts',(-41.7661166038015,24.1219544207148,20.));
#80685=CARTESIAN_POINT('Ctrl Pts',(-41.7467712919966,24.1493787748488,0.));
#80686=CARTESIAN_POINT('Ctrl Pts',(-41.7467712919966,24.1493787748488,20.));
#80687=CARTESIAN_POINT('Ctrl Pts',(-41.7274076232605,24.1767888034393,0.));
#80688=CARTESIAN_POINT('Ctrl Pts',(-41.7274076232605,24.1767888034393,20.));
#80689=CARTESIAN_POINT('Ctrl Pts',(-41.7080256075983,24.2041844938197,0.));
#80690=CARTESIAN_POINT('Ctrl Pts',(-41.7080256075983,24.2041844938197,20.));
#80691=CARTESIAN_POINT('Ctrl Pts',(-41.688625255024,24.2315658333297,0.));
#80692=CARTESIAN_POINT('Ctrl Pts',(-41.688625255024,24.2315658333297,20.));
#80693=CARTESIAN_POINT('Ctrl Pts',(-41.6692065755608,24.2589328093159,0.));
#80694=CARTESIAN_POINT('Ctrl Pts',(-41.6692065755608,24.2589328093159,20.));
#80695=CARTESIAN_POINT('Ctrl Pts',(-41.6497695792407,24.2862854091312,0.));
#80696=CARTESIAN_POINT('Ctrl Pts',(-41.6497695792407,24.2862854091312,20.));
#80697=CARTESIAN_POINT('Ctrl Pts',(-41.630314276105,24.3136236201351,0.));
#80698=CARTESIAN_POINT('Ctrl Pts',(-41.630314276105,24.3136236201351,20.));
#80699=CARTESIAN_POINT('Ctrl Pts',(-41.610840676204,24.340947429694,0.));
#80700=CARTESIAN_POINT('Ctrl Pts',(-41.610840676204,24.340947429694,20.));
#80701=CARTESIAN_POINT('Ctrl Pts',(-41.5913487895971,24.368256825181,0.));
#80702=CARTESIAN_POINT('Ctrl Pts',(-41.5913487895971,24.368256825181,20.));
#80703=CARTESIAN_POINT('Ctrl Pts',(-41.5718386263526,24.3955517939756,0.));
#80704=CARTESIAN_POINT('Ctrl Pts',(-41.5718386263526,24.3955517939756,20.));
#80705=CARTESIAN_POINT('Ctrl Pts',(-41.5523101965477,24.4228323234645,0.));
#80706=CARTESIAN_POINT('Ctrl Pts',(-41.5523101965477,24.4228323234645,20.));
#80707=CARTESIAN_POINT('Ctrl Pts',(-41.5327635102685,24.4500984010406,0.));
#80708=CARTESIAN_POINT('Ctrl Pts',(-41.5327635102685,24.4500984010406,20.));
#80709=CARTESIAN_POINT('Ctrl Pts',(-41.5131985776101,24.4773500141036,0.));
#80710=CARTESIAN_POINT('Ctrl Pts',(-41.5131985776101,24.4773500141036,20.));
#80711=CARTESIAN_POINT('Ctrl Pts',(-41.4936154086768,24.5045871500598,0.));
#80712=CARTESIAN_POINT('Ctrl Pts',(-41.4936154086768,24.5045871500598,20.));
#80713=CARTESIAN_POINT('Ctrl Pts',(-41.4740140135823,24.5318097963222,0.));
#80714=CARTESIAN_POINT('Ctrl Pts',(-41.4740140135823,24.5318097963222,20.));
#80715=CARTESIAN_POINT('Ctrl Pts',(-41.4543944024488,24.5590179403106,0.));
#80716=CARTESIAN_POINT('Ctrl Pts',(-41.4543944024488,24.5590179403106,20.));
#80717=CARTESIAN_POINT('Ctrl Pts',(-41.4347565854076,24.5862115694513,0.));
#80718=CARTESIAN_POINT('Ctrl Pts',(-41.4347565854076,24.5862115694513,20.));
#80719=CARTESIAN_POINT('Ctrl Pts',(-41.4151005725989,24.6133906711774,0.));
#80720=CARTESIAN_POINT('Ctrl Pts',(-41.4151005725989,24.6133906711774,20.));
#80721=CARTESIAN_POINT('Ctrl Pts',(-41.3954263741717,24.6405552329288,0.));
#80722=CARTESIAN_POINT('Ctrl Pts',(-41.3954263741717,24.6405552329288,20.));
#80723=CARTESIAN_POINT('Ctrl Pts',(-41.3757340002844,24.6677052421523,0.));
#80724=CARTESIAN_POINT('Ctrl Pts',(-41.3757340002844,24.6677052421523,20.));
#80725=CARTESIAN_POINT('Ctrl Pts',(-41.3560234611038,24.694840686301,0.));
#80726=CARTESIAN_POINT('Ctrl Pts',(-41.3560234611038,24.694840686301,20.));
#80727=CARTESIAN_POINT('Ctrl Pts',(-41.3362947668064,24.7219615528352,0.));
#80728=CARTESIAN_POINT('Ctrl Pts',(-41.3362947668064,24.7219615528352,20.));
#80729=CARTESIAN_POINT('Ctrl Pts',(-41.3165479275773,24.7490678292217,0.));
#80730=CARTESIAN_POINT('Ctrl Pts',(-41.3165479275773,24.7490678292217,20.));
#80731=CARTESIAN_POINT('Ctrl Pts',(-41.2967829536105,24.776159502934,0.));
#80732=CARTESIAN_POINT('Ctrl Pts',(-41.2967829536105,24.776159502934,20.));
#80733=CARTESIAN_POINT('Ctrl Pts',(-41.276999855109,24.8032365614525,0.));
#80734=CARTESIAN_POINT('Ctrl Pts',(-41.276999855109,24.8032365614525,20.));
#80735=CARTESIAN_POINT('Ctrl Pts',(-41.2571986422843,24.8302989922639,0.));
#80736=CARTESIAN_POINT('Ctrl Pts',(-41.2571986422843,24.8302989922639,20.));
#80737=CARTESIAN_POINT('Ctrl Pts',(-41.2373793253577,24.8573467828623,0.));
#80738=CARTESIAN_POINT('Ctrl Pts',(-41.2373793253577,24.8573467828623,20.));
#80739=CARTESIAN_POINT('Ctrl Pts',(-41.2175419145589,24.8843799207482,0.));
#80740=CARTESIAN_POINT('Ctrl Pts',(-41.2175419145589,24.8843799207482,20.));
#80741=CARTESIAN_POINT('Ctrl Pts',(-41.1976864201268,24.9113983934293,0.));
#80742=CARTESIAN_POINT('Ctrl Pts',(-41.1976864201268,24.9113983934293,20.));
#80743=CARTESIAN_POINT('Ctrl Pts',(-41.1778128523092,24.9384021884197,0.));
#80744=CARTESIAN_POINT('Ctrl Pts',(-41.1778128523092,24.9384021884197,20.));
#80745=CARTESIAN_POINT('Ctrl Pts',(-41.1579212213625,24.9653912932402,0.));
#80746=CARTESIAN_POINT('Ctrl Pts',(-41.1579212213625,24.9653912932402,20.));
#80747=CARTESIAN_POINT('Ctrl Pts',(-41.1380115375521,24.9923656954187,0.));
#80748=CARTESIAN_POINT('Ctrl Pts',(-41.1380115375521,24.9923656954187,20.));
#80749=CARTESIAN_POINT('Ctrl Pts',(-41.1180838111525,25.0193253824897,0.));
#80750=CARTESIAN_POINT('Ctrl Pts',(-41.1180838111525,25.0193253824897,20.));
#80751=CARTESIAN_POINT('Ctrl Pts',(-41.0981380524472,25.0462703419947,0.));
#80752=CARTESIAN_POINT('Ctrl Pts',(-41.0981380524472,25.0462703419947,20.));
#80753=CARTESIAN_POINT('Ctrl Pts',(-41.0781742717283,25.0732005614819,0.));
#80754=CARTESIAN_POINT('Ctrl Pts',(-41.0781742717283,25.0732005614819,20.));
#80755=CARTESIAN_POINT('Ctrl Pts',(-41.058192479297,25.1001160285063,0.));
#80756=CARTESIAN_POINT('Ctrl Pts',(-41.058192479297,25.1001160285063,20.));
#80757=CARTESIAN_POINT('Ctrl Pts',(-41.0381926854636,25.1270167306298,0.));
#80758=CARTESIAN_POINT('Ctrl Pts',(-41.0381926854636,25.1270167306298,20.));
#80759=CARTESIAN_POINT('Ctrl Pts',(-41.0181749005471,25.1539026554213,0.));
#80760=CARTESIAN_POINT('Ctrl Pts',(-41.0181749005471,25.1539026554213,20.));
#80761=CARTESIAN_POINT('Ctrl Pts',(-40.9981391348755,25.1807737904566,0.));
#80762=CARTESIAN_POINT('Ctrl Pts',(-40.9981391348755,25.1807737904566,20.));
#80763=CARTESIAN_POINT('Ctrl Pts',(-40.9780853987856,25.2076301233182,0.));
#80764=CARTESIAN_POINT('Ctrl Pts',(-40.9780853987856,25.2076301233182,20.));
#80765=CARTESIAN_POINT('Ctrl Pts',(-40.9580137026228,25.2344716415952,0.));
#80766=CARTESIAN_POINT('Ctrl Pts',(-40.9580137026228,25.2344716415952,20.));
#80767=CARTESIAN_POINT('Ctrl Pts',(-40.9379240567416,25.2612983328836,0.));
#80768=CARTESIAN_POINT('Ctrl Pts',(-40.9379240567416,25.2612983328836,20.));
#80769=CARTESIAN_POINT('Ctrl Pts',(-40.9178164715051,25.2881101847861,0.));
#80770=CARTESIAN_POINT('Ctrl Pts',(-40.9178164715051,25.2881101847861,20.));
#80771=CARTESIAN_POINT('Ctrl Pts',(-40.8976909572856,25.3149071849127,0.));
#80772=CARTESIAN_POINT('Ctrl Pts',(-40.8976909572856,25.3149071849127,20.));
#80773=CARTESIAN_POINT('Ctrl Pts',(-40.8775475244644,25.3416893208802,0.));
#80774=CARTESIAN_POINT('Ctrl Pts',(-40.8775475244644,25.3416893208802,20.));
#80775=CARTESIAN_POINT('Ctrl Pts',(-40.8573861834316,25.3684565803126,0.));
#80776=CARTESIAN_POINT('Ctrl Pts',(-40.8573861834316,25.3684565803126,20.));
#80777=CARTESIAN_POINT('Ctrl Pts',(-40.8372069445862,25.3952089508407,0.));
#80778=CARTESIAN_POINT('Ctrl Pts',(-40.8372069445862,25.3952089508407,20.));
#80779=CARTESIAN_POINT('Ctrl Pts',(-40.8170098183362,25.4219464201024,0.));
#80780=CARTESIAN_POINT('Ctrl Pts',(-40.8170098183362,25.4219464201024,20.));
#80781=CARTESIAN_POINT('Ctrl Pts',(-40.7967948150981,25.4486689757422,0.));
#80782=CARTESIAN_POINT('Ctrl Pts',(-40.7967948150981,25.4486689757422,20.));
#80783=CARTESIAN_POINT('Ctrl Pts',(-40.7765619452973,25.4753766054114,0.));
#80784=CARTESIAN_POINT('Ctrl Pts',(-40.7765619452973,25.4753766054114,20.));
#80785=CARTESIAN_POINT('Ctrl Pts',(-40.7563112193678,25.5020692967677,0.));
#80786=CARTESIAN_POINT('Ctrl Pts',(-40.7563112193678,25.5020692967677,20.));
#80787=CARTESIAN_POINT('Ctrl Pts',(-40.7360426477524,25.528747037476,0.));
#80788=CARTESIAN_POINT('Ctrl Pts',(-40.7360426477524,25.528747037476,20.));
#80789=CARTESIAN_POINT('Ctrl Pts',(-40.715756240903,25.5554098152083,0.));
#80790=CARTESIAN_POINT('Ctrl Pts',(-40.715756240903,25.5554098152083,20.));
#80791=CARTESIAN_POINT('Ctrl Pts',(-40.6954520092804,25.5820576176439,0.));
#80792=CARTESIAN_POINT('Ctrl Pts',(-40.6954520092804,25.5820576176439,20.));
#80793=CARTESIAN_POINT('Ctrl Pts',(-40.6751299633543,25.6086904324689,0.));
#80794=CARTESIAN_POINT('Ctrl Pts',(-40.6751299633543,25.6086904324689,20.));
#80795=CARTESIAN_POINT('Ctrl Pts',(-40.6547901136033,25.6353082473768,0.));
#80796=CARTESIAN_POINT('Ctrl Pts',(-40.6547901136033,25.6353082473768,20.));
#80797=CARTESIAN_POINT('Ctrl Pts',(-40.6344324705148,25.6619110500677,0.));
#80798=CARTESIAN_POINT('Ctrl Pts',(-40.6344324705148,25.6619110500677,20.));
#80799=CARTESIAN_POINT('Ctrl Pts',(-40.6140570445847,25.6884988282486,0.));
#80800=CARTESIAN_POINT('Ctrl Pts',(-40.6140570445847,25.6884988282486,20.));
#80801=CARTESIAN_POINT('Ctrl Pts',(-40.5936638463177,25.7150715696332,0.));
#80802=CARTESIAN_POINT('Ctrl Pts',(-40.5936638463177,25.7150715696332,20.));
#80803=CARTESIAN_POINT('Ctrl Pts',(-40.5732528862276,25.7416292619425,0.));
#80804=CARTESIAN_POINT('Ctrl Pts',(-40.5732528862276,25.7416292619425,20.));
#80805=CARTESIAN_POINT('Ctrl Pts',(-40.5528241748366,25.768171892904,0.));
#80806=CARTESIAN_POINT('Ctrl Pts',(-40.5528241748366,25.768171892904,20.));
#80807=CARTESIAN_POINT('Ctrl Pts',(-40.5323777226758,25.7946994502526,0.));
#80808=CARTESIAN_POINT('Ctrl Pts',(-40.5323777226758,25.7946994502526,20.));
#80809=CARTESIAN_POINT('Ctrl Pts',(-40.5119135402853,25.8212119217304,0.));
#80810=CARTESIAN_POINT('Ctrl Pts',(-40.5119135402853,25.8212119217304,20.));
#80811=CARTESIAN_POINT('Ctrl Pts',(-40.4914316382141,25.8477092950863,0.));
#80812=CARTESIAN_POINT('Ctrl Pts',(-40.4914316382141,25.8477092950863,20.));
#80813=CARTESIAN_POINT('Ctrl Pts',(-40.4709320270197,25.8741915580762,0.));
#80814=CARTESIAN_POINT('Ctrl Pts',(-40.4709320270197,25.8741915580762,20.));
#80815=CARTESIAN_POINT('Ctrl Pts',(-40.4504147172684,25.900658698463,0.));
#80816=CARTESIAN_POINT('Ctrl Pts',(-40.4504147172684,25.900658698463,20.));
#80817=CARTESIAN_POINT('Ctrl Pts',(-40.4298797195353,25.9271107040168,0.));
#80818=CARTESIAN_POINT('Ctrl Pts',(-40.4298797195353,25.9271107040168,20.));
#80819=CARTESIAN_POINT('Ctrl Pts',(-40.4093270444043,25.953547562515,0.));
#80820=CARTESIAN_POINT('Ctrl Pts',(-40.4093270444043,25.953547562515,20.));
#80821=CARTESIAN_POINT('Ctrl Pts',(-40.3887567024682,25.9799692617416,0.));
#80822=CARTESIAN_POINT('Ctrl Pts',(-40.3887567024682,25.9799692617416,20.));
#80823=CARTESIAN_POINT('Ctrl Pts',(-40.3681687043284,26.0063757894875,0.));
#80824=CARTESIAN_POINT('Ctrl Pts',(-40.3681687043284,26.0063757894875,20.));
#80825=CARTESIAN_POINT('Ctrl Pts',(-40.347563060595,26.0327671335511,0.));
#80826=CARTESIAN_POINT('Ctrl Pts',(-40.347563060595,26.0327671335511,20.));
#80827=CARTESIAN_POINT('Ctrl Pts',(-40.326939781887,26.0591432817373,0.));
#80828=CARTESIAN_POINT('Ctrl Pts',(-40.326939781887,26.0591432817373,20.));
#80829=CARTESIAN_POINT('Ctrl Pts',(-40.3062988788318,26.0855042218583,0.));
#80830=CARTESIAN_POINT('Ctrl Pts',(-40.3062988788318,26.0855042218583,20.));
#80831=CARTESIAN_POINT('Ctrl Pts',(-40.2856403620657,26.1118499417334,0.));
#80832=CARTESIAN_POINT('Ctrl Pts',(-40.2856403620657,26.1118499417334,20.));
#80833=CARTESIAN_POINT('Ctrl Pts',(-40.2649642422341,26.1381804291892,0.));
#80834=CARTESIAN_POINT('Ctrl Pts',(-40.2649642422341,26.1381804291892,20.));
#80835=CARTESIAN_POINT('Ctrl Pts',(-40.2442705299908,26.1644956720595,0.));
#80836=CARTESIAN_POINT('Ctrl Pts',(-40.2442705299908,26.1644956720595,20.));
#80837=CARTESIAN_POINT('Ctrl Pts',(-40.2235592359986,26.1907956581851,0.));
#80838=CARTESIAN_POINT('Ctrl Pts',(-40.2235592359986,26.1907956581851,20.));
#80839=CARTESIAN_POINT('Ctrl Pts',(-40.2028303709288,26.217080375414,0.));
#80840=CARTESIAN_POINT('Ctrl Pts',(-40.2028303709288,26.217080375414,20.));
#80841=CARTESIAN_POINT('Ctrl Pts',(-40.1820839454613,26.2433498116008,0.));
#80842=CARTESIAN_POINT('Ctrl Pts',(-40.1820839454613,26.2433498116008,20.));
#80843=CARTESIAN_POINT('Ctrl Pts',(-40.161319970285,26.2696039546074,0.));
#80844=CARTESIAN_POINT('Ctrl Pts',(-40.161319970285,26.2696039546074,20.));
#80845=CARTESIAN_POINT('Ctrl Pts',(-40.1405384560971,26.2958427923028,0.));
#80846=CARTESIAN_POINT('Ctrl Pts',(-40.1405384560971,26.2958427923028,20.));
#80847=CARTESIAN_POINT('Ctrl Pts',(-40.1197394136039,26.3220663125631,0.));
#80848=CARTESIAN_POINT('Ctrl Pts',(-40.1197394136039,26.3220663125631,20.));
#80849=CARTESIAN_POINT('Ctrl Pts',(-40.0989228535202,26.3482745032719,0.));
#80850=CARTESIAN_POINT('Ctrl Pts',(-40.0989228535202,26.3482745032719,20.));
#80851=CARTESIAN_POINT('Ctrl Pts',(-40.0780887865696,26.3744673523197,0.));
#80852=CARTESIAN_POINT('Ctrl Pts',(-40.0780887865696,26.3744673523197,20.));
#80853=CARTESIAN_POINT('Ctrl Pts',(-40.0572372234844,26.4006448476041,0.));
#80854=CARTESIAN_POINT('Ctrl Pts',(-40.0572372234844,26.4006448476041,20.));
#80855=CARTESIAN_POINT('Ctrl Pts',(-40.0363681750053,26.4268069770299,0.));
#80856=CARTESIAN_POINT('Ctrl Pts',(-40.0363681750053,26.4268069770299,20.));
#80857=CARTESIAN_POINT('Ctrl Pts',(-40.015481651882,26.4529537285089,0.));
#80858=CARTESIAN_POINT('Ctrl Pts',(-40.015481651882,26.4529537285089,20.));
#80859=CARTESIAN_POINT('Ctrl Pts',(-39.9945776648731,26.4790850899607,0.));
#80860=CARTESIAN_POINT('Ctrl Pts',(-39.9945776648731,26.4790850899607,20.));
#80861=CARTESIAN_POINT('Ctrl Pts',(-39.9736562247456,26.5052010493117,0.));
#80862=CARTESIAN_POINT('Ctrl Pts',(-39.9736562247456,26.5052010493117,20.));
#80863=CARTESIAN_POINT('Ctrl Pts',(-39.9527173422752,26.5313015944953,0.));
#80864=CARTESIAN_POINT('Ctrl Pts',(-39.9527173422752,26.5313015944953,20.));
#80865=CARTESIAN_POINT('Ctrl Pts',(-39.9317610282459,26.5573867134521,0.));
#80866=CARTESIAN_POINT('Ctrl Pts',(-39.9317610282459,26.5573867134521,20.));
#80867=CARTESIAN_POINT('Ctrl Pts',(-39.9107872934506,26.5834563941296,0.));
#80868=CARTESIAN_POINT('Ctrl Pts',(-39.9107872934506,26.5834563941296,20.));
#80869=CARTESIAN_POINT('Ctrl Pts',(-39.8897961486907,26.6095106244829,0.));
#80870=CARTESIAN_POINT('Ctrl Pts',(-39.8897961486907,26.6095106244829,20.));
#80871=CARTESIAN_POINT('Ctrl Pts',(-39.8687876047769,26.6355493924743,0.));
#80872=CARTESIAN_POINT('Ctrl Pts',(-39.8687876047769,26.6355493924743,20.));
#80873=CARTESIAN_POINT('Ctrl Pts',(-39.847761672528,26.6615726860734,0.));
#80874=CARTESIAN_POINT('Ctrl Pts',(-39.847761672528,26.6615726860734,20.));
#80875=CARTESIAN_POINT('Ctrl Pts',(-39.8267183627717,26.687580493257,0.));
#80876=CARTESIAN_POINT('Ctrl Pts',(-39.8267183627717,26.687580493257,20.));
#80877=CARTESIAN_POINT('Ctrl Pts',(-39.8056576863443,26.713572802009,0.));
#80878=CARTESIAN_POINT('Ctrl Pts',(-39.8056576863443,26.713572802009,20.));
#80879=CARTESIAN_POINT('Ctrl Pts',(-39.7845796540903,26.7395496003209,0.));
#80880=CARTESIAN_POINT('Ctrl Pts',(-39.7845796540903,26.7395496003209,20.));
#80881=CARTESIAN_POINT('Ctrl Pts',(-39.7634842768632,26.7655108761908,0.));
#80882=CARTESIAN_POINT('Ctrl Pts',(-39.7634842768632,26.7655108761908,20.));
#80883=CARTESIAN_POINT('Ctrl Pts',(-39.7423715655248,26.7914566176244,0.));
#80884=CARTESIAN_POINT('Ctrl Pts',(-39.7423715655248,26.7914566176244,20.));
#80885=CARTESIAN_POINT('Ctrl Pts',(-39.7212415309462,26.8173868126344,0.));
#80886=CARTESIAN_POINT('Ctrl Pts',(-39.7212415309462,26.8173868126344,20.));
#80887=CARTESIAN_POINT('Ctrl Pts',(-39.7000941840066,26.843301449241,0.));
#80888=CARTESIAN_POINT('Ctrl Pts',(-39.7000941840066,26.843301449241,20.));
#80889=CARTESIAN_POINT('Ctrl Pts',(-39.6789295355942,26.8692005154716,0.));
#80890=CARTESIAN_POINT('Ctrl Pts',(-39.6789295355942,26.8692005154716,20.));
#80891=CARTESIAN_POINT('Ctrl Pts',(-39.6577475966055,26.8950839993609,0.));
#80892=CARTESIAN_POINT('Ctrl Pts',(-39.6577475966055,26.8950839993609,20.));
#80893=CARTESIAN_POINT('Ctrl Pts',(-39.6365483779458,26.9209518889509,0.));
#80894=CARTESIAN_POINT('Ctrl Pts',(-39.6365483779458,26.9209518889509,20.));
#80895=CARTESIAN_POINT('Ctrl Pts',(-39.6153318905283,26.9468041722907,0.));
#80896=CARTESIAN_POINT('Ctrl Pts',(-39.6153318905283,26.9468041722907,20.));
#80897=CARTESIAN_POINT('Ctrl Pts',(-39.5940981452753,26.972640837437,0.));
#80898=CARTESIAN_POINT('Ctrl Pts',(-39.5940981452753,26.972640837437,20.));
#80899=CARTESIAN_POINT('Ctrl Pts',(-39.5728471531178,26.9984618724537,0.));
#80900=CARTESIAN_POINT('Ctrl Pts',(-39.5728471531178,26.9984618724537,20.));
#80901=CARTESIAN_POINT('Ctrl Pts',(-39.5515789249953,27.0242672654118,0.));
#80902=CARTESIAN_POINT('Ctrl Pts',(-39.5515789249953,27.0242672654118,20.));
#80903=CARTESIAN_POINT('Ctrl Pts',(-39.5302934718558,27.0500570043898,0.));
#80904=CARTESIAN_POINT('Ctrl Pts',(-39.5302934718558,27.0500570043898,20.));
#80905=CARTESIAN_POINT('Ctrl Pts',(-39.5089908046561,27.0758310774732,0.));
#80906=CARTESIAN_POINT('Ctrl Pts',(-39.5089908046561,27.0758310774732,20.));
#80907=CARTESIAN_POINT('Ctrl Pts',(-39.4876709343614,27.1015894727552,0.));
#80908=CARTESIAN_POINT('Ctrl Pts',(-39.4876709343614,27.1015894727552,20.));
#80909=CARTESIAN_POINT('Ctrl Pts',(-39.4663338719455,27.1273321783362,0.));
#80910=CARTESIAN_POINT('Ctrl Pts',(-39.4663338719455,27.1273321783362,20.));
#80911=CARTESIAN_POINT('Ctrl Pts',(-39.4449796283908,27.153059182324,0.));
#80912=CARTESIAN_POINT('Ctrl Pts',(-39.4449796283908,27.153059182324,20.));
#80913=CARTESIAN_POINT('Ctrl Pts',(-39.4236082146882,27.1787704728336,0.));
#80914=CARTESIAN_POINT('Ctrl Pts',(-39.4236082146882,27.1787704728336,20.));
#80915=CARTESIAN_POINT('Ctrl Pts',(-39.4022196418372,27.2044660379877,0.));
#80916=CARTESIAN_POINT('Ctrl Pts',(-39.4022196418372,27.2044660379877,20.));
#80917=CARTESIAN_POINT('Ctrl Pts',(-39.3808139208456,27.2301458659157,0.));
#80918=CARTESIAN_POINT('Ctrl Pts',(-39.3808139208456,27.2301458659157,20.));
#80919=CARTESIAN_POINT('Ctrl Pts',(-39.3593910627297,27.2558099447548,0.));
#80920=CARTESIAN_POINT('Ctrl Pts',(-39.3593910627297,27.2558099447548,20.));
#80921=CARTESIAN_POINT('Ctrl Pts',(-39.3379510785145,27.2814582626492,0.));
#80922=CARTESIAN_POINT('Ctrl Pts',(-39.3379510785145,27.2814582626492,20.));
#80923=CARTESIAN_POINT('Ctrl Pts',(-39.3164939792334,27.3070908077508,0.));
#80924=CARTESIAN_POINT('Ctrl Pts',(-39.3164939792334,27.3070908077508,20.));
#80925=CARTESIAN_POINT('Ctrl Pts',(-39.2950197759285,27.3327075682187,0.));
#80926=CARTESIAN_POINT('Ctrl Pts',(-39.2950197759285,27.3327075682187,20.));
#80927=CARTESIAN_POINT('Ctrl Pts',(-39.2735284796508,27.3583085322198,0.));
#80928=CARTESIAN_POINT('Ctrl Pts',(-39.2735284796508,27.3583085322198,20.));
#80929=CARTESIAN_POINT('Ctrl Pts',(-39.25202010146,27.3838936879286,0.));
#80930=CARTESIAN_POINT('Ctrl Pts',(-39.25202010146,27.3838936879286,20.));
#80931=CARTESIAN_POINT('Ctrl Pts',(-39.2304946524241,27.4094630235265,0.));
#80932=CARTESIAN_POINT('Ctrl Pts',(-39.2304946524241,27.4094630235265,20.));
#80933=CARTESIAN_POINT('Ctrl Pts',(-39.2089521436188,27.4350165272023,0.));
#80934=CARTESIAN_POINT('Ctrl Pts',(-39.2089521436188,27.4350165272023,20.));
#80935=CARTESIAN_POINT('Ctrl Pts',(-39.1873925861285,27.4605541871518,0.));
#80936=CARTESIAN_POINT('Ctrl Pts',(-39.1873925861285,27.4605541871518,20.));
#80937=CARTESIAN_POINT('Ctrl Pts',(-39.1658159910458,27.4860759915783,0.));
#80938=CARTESIAN_POINT('Ctrl Pts',(-39.1658159910458,27.4860759915783,20.));
#80939=CARTESIAN_POINT('Ctrl Pts',(-39.1442223694722,27.5115819286926,0.));
#80940=CARTESIAN_POINT('Ctrl Pts',(-39.1442223694722,27.5115819286926,20.));
#80941=CARTESIAN_POINT('Ctrl Pts',(-39.1226117325183,27.5370719867136,0.));
#80942=CARTESIAN_POINT('Ctrl Pts',(-39.1226117325183,27.5370719867136,20.));
#80943=CARTESIAN_POINT('Ctrl Pts',(-39.100984091303,27.5625461538675,0.));
#80944=CARTESIAN_POINT('Ctrl Pts',(-39.100984091303,27.5625461538675,20.));
#80945=CARTESIAN_POINT('Ctrl Pts',(-39.0793394569537,27.5880044183879,0.));
#80946=CARTESIAN_POINT('Ctrl Pts',(-39.0793394569537,27.5880044183879,20.));
#80947=CARTESIAN_POINT('Ctrl Pts',(-39.057677840606,27.6134467685155,0.));
#80948=CARTESIAN_POINT('Ctrl Pts',(-39.057677840606,27.6134467685155,20.));
#80949=CARTESIAN_POINT('Ctrl Pts',(-39.0359992534037,27.6388731924983,0.));
#80950=CARTESIAN_POINT('Ctrl Pts',(-39.0359992534037,27.6388731924983,20.));
#80951=CARTESIAN_POINT('Ctrl Pts',(-39.0143037064988,27.6642836785915,0.));
#80952=CARTESIAN_POINT('Ctrl Pts',(-39.0143037064988,27.6642836785915,20.));
#80953=CARTESIAN_POINT('Ctrl Pts',(-38.9925912110523,27.6896782150583,0.));
#80954=CARTESIAN_POINT('Ctrl Pts',(-38.9925912110523,27.6896782150583,20.));
#80955=CARTESIAN_POINT('Ctrl Pts',(-38.9708617782339,27.7150567901695,0.));
#80956=CARTESIAN_POINT('Ctrl Pts',(-38.9708617782339,27.7150567901695,20.));
#80957=CARTESIAN_POINT('Ctrl Pts',(-38.9491154192216,27.7404193922036,0.));
#80958=CARTESIAN_POINT('Ctrl Pts',(-38.9491154192216,27.7404193922036,20.));
#80959=CARTESIAN_POINT('Ctrl Pts',(-38.9273521452022,27.7657660094466,0.));
#80960=CARTESIAN_POINT('Ctrl Pts',(-38.9273521452022,27.7657660094466,20.));
#80961=CARTESIAN_POINT('Ctrl Pts',(-38.9055719673706,27.7910966301919,0.));
#80962=CARTESIAN_POINT('Ctrl Pts',(-38.9055719673706,27.7910966301919,20.));
#80963=CARTESIAN_POINT('Ctrl Pts',(-38.8837748969299,27.8164112427396,0.));
#80964=CARTESIAN_POINT('Ctrl Pts',(-38.8837748969299,27.8164112427396,20.));
#80965=CARTESIAN_POINT('Ctrl Pts',(-38.8619609450913,27.8417098353975,0.));
#80966=CARTESIAN_POINT('Ctrl Pts',(-38.8619609450913,27.8417098353975,20.));
#80967=CARTESIAN_POINT('Ctrl Pts',(-38.8401301230745,27.866992396481,0.));
#80968=CARTESIAN_POINT('Ctrl Pts',(-38.8401301230745,27.866992396481,20.));
#80969=CARTESIAN_POINT('Ctrl Pts',(-38.8182824421082,27.8922589143132,0.));
#80970=CARTESIAN_POINT('Ctrl Pts',(-38.8182824421082,27.8922589143132,20.));
#80971=CARTESIAN_POINT('Ctrl Pts',(-38.7964179134294,27.917509377225,0.));
#80972=CARTESIAN_POINT('Ctrl Pts',(-38.7964179134294,27.917509377225,20.));
#80973=CARTESIAN_POINT('Ctrl Pts',(-38.7745365482838,27.9427437735546,0.));
#80974=CARTESIAN_POINT('Ctrl Pts',(-38.7745365482838,27.9427437735546,20.));
#80975=CARTESIAN_POINT('Ctrl Pts',(-38.752638357925,27.9679620916479,0.));
#80976=CARTESIAN_POINT('Ctrl Pts',(-38.752638357925,27.9679620916479,20.));
#80977=CARTESIAN_POINT('Ctrl Pts',(-38.7307233536152,27.993164319858,0.));
#80978=CARTESIAN_POINT('Ctrl Pts',(-38.7307233536152,27.993164319858,20.));
#80979=CARTESIAN_POINT('Ctrl Pts',(-38.7087915466247,28.0183504465458,0.));
#80980=CARTESIAN_POINT('Ctrl Pts',(-38.7087915466247,28.0183504465458,20.));
#80981=CARTESIAN_POINT('Ctrl Pts',(-38.6868429482325,28.0435204600798,0.));
#80982=CARTESIAN_POINT('Ctrl Pts',(-38.6868429482325,28.0435204600798,20.));
#80983=CARTESIAN_POINT('Ctrl Pts',(-38.6648775697261,28.0686743488361,0.));
#80984=CARTESIAN_POINT('Ctrl Pts',(-38.6648775697261,28.0686743488361,20.));
#80985=CARTESIAN_POINT('Ctrl Pts',(-38.6428954224012,28.0938121011982,0.));
#80986=CARTESIAN_POINT('Ctrl Pts',(-38.6428954224012,28.0938121011982,20.));
#80987=CARTESIAN_POINT('Ctrl Pts',(-38.6208965175619,28.1189337055566,0.));
#80988=CARTESIAN_POINT('Ctrl Pts',(-38.6208965175619,28.1189337055566,20.));
#80989=CARTESIAN_POINT('Ctrl Pts',(-38.5988808665205,28.14403915031,0.));
#80990=CARTESIAN_POINT('Ctrl Pts',(-38.5988808665205,28.14403915031,20.));
#80991=CARTESIAN_POINT('Ctrl Pts',(-38.5768484805979,28.1691284238645,0.));
#80992=CARTESIAN_POINT('Ctrl Pts',(-38.5768484805979,28.1691284238645,20.));
#80993=CARTESIAN_POINT('Ctrl Pts',(-38.5547993711231,28.194201514634,0.));
#80994=CARTESIAN_POINT('Ctrl Pts',(-38.5547993711231,28.194201514634,20.));
#80995=CARTESIAN_POINT('Ctrl Pts',(-38.5327335494335,28.2192584110398,0.));
#80996=CARTESIAN_POINT('Ctrl Pts',(-38.5327335494335,28.2192584110398,20.));
#80997=CARTESIAN_POINT('Ctrl Pts',(-38.5106510268752,28.2442991015113,0.));
#80998=CARTESIAN_POINT('Ctrl Pts',(-38.5106510268752,28.2442991015113,20.));
#80999=CARTESIAN_POINT('Ctrl Pts',(-38.4885518148031,28.2693235744854,0.));
#81000=CARTESIAN_POINT('Ctrl Pts',(-38.4885518148031,28.2693235744854,20.));
#81001=CARTESIAN_POINT('Ctrl Pts',(-38.4664359245797,28.2943318184065,0.));
#81002=CARTESIAN_POINT('Ctrl Pts',(-38.4664359245797,28.2943318184065,20.));
#81003=CARTESIAN_POINT('Ctrl Pts',(-38.444303367576,28.3193238217266,0.));
#81004=CARTESIAN_POINT('Ctrl Pts',(-38.444303367576,28.3193238217266,20.));
#81005=CARTESIAN_POINT('Ctrl Pts',(-38.422154155171,28.3442995729049,0.));
#81006=CARTESIAN_POINT('Ctrl Pts',(-38.422154155171,28.3442995729049,20.));
#81007=CARTESIAN_POINT('Ctrl Pts',(-38.3999882987522,28.3692590604082,0.));
#81008=CARTESIAN_POINT('Ctrl Pts',(-38.3999882987522,28.3692590604082,20.));
#81009=CARTESIAN_POINT('Ctrl Pts',(-38.3778058097152,28.3942022727108,0.));
#81010=CARTESIAN_POINT('Ctrl Pts',(-38.3778058097152,28.3942022727108,20.));
#81011=CARTESIAN_POINT('Ctrl Pts',(-38.3556066994642,28.419129198295,0.));
#81012=CARTESIAN_POINT('Ctrl Pts',(-38.3556066994642,28.419129198295,20.));
#81013=CARTESIAN_POINT('Ctrl Pts',(-38.333390979412,28.4440398256512,0.));
#81014=CARTESIAN_POINT('Ctrl Pts',(-38.333390979412,28.4440398256512,20.));
#81015=CARTESIAN_POINT('Ctrl Pts',(-38.3111586609795,28.4689341432774,0.));
#81016=CARTESIAN_POINT('Ctrl Pts',(-38.3111586609795,28.4689341432774,20.));
#81017=CARTESIAN_POINT('Ctrl Pts',(-38.2889097555964,28.4938121396793,0.));
#81018=CARTESIAN_POINT('Ctrl Pts',(-38.2889097555964,28.4938121396793,20.));
#81019=CARTESIAN_POINT('Ctrl Pts',(-38.2666442747002,28.5186738033703,0.));
#81020=CARTESIAN_POINT('Ctrl Pts',(-38.2666442747002,28.5186738033703,20.));
#81021=CARTESIAN_POINT('Ctrl Pts',(-38.2443622297368,28.543519122871,0.));
#81022=CARTESIAN_POINT('Ctrl Pts',(-38.2443622297368,28.543519122871,20.));
#81023=CARTESIAN_POINT('Ctrl Pts',(-38.2220636321601,28.5683480867097,0.));
#81024=CARTESIAN_POINT('Ctrl Pts',(-38.2220636321601,28.5683480867097,20.));
#81025=CARTESIAN_POINT('Ctrl Pts',(-38.1997484934321,28.5931606834223,0.));
#81026=CARTESIAN_POINT('Ctrl Pts',(-38.1997484934321,28.5931606834223,20.));
#81027=CARTESIAN_POINT('Ctrl Pts',(-38.1774168250235,28.6179569015525,0.));
#81028=CARTESIAN_POINT('Ctrl Pts',(-38.1774168250235,28.6179569015525,20.));
#81029=CARTESIAN_POINT('Ctrl Pts',(-38.1550686384134,28.6427367296518,0.));
#81030=CARTESIAN_POINT('Ctrl Pts',(-38.1550686384134,28.6427367296518,20.));
#81031=CARTESIAN_POINT('Ctrl Pts',(-38.1327039450889,28.6675001562794,0.));
#81032=CARTESIAN_POINT('Ctrl Pts',(-38.1327039450889,28.6675001562794,20.));
#81033=CARTESIAN_POINT('Ctrl Pts',(-38.1103227565456,28.6922471700024,0.));
#81034=CARTESIAN_POINT('Ctrl Pts',(-38.1103227565456,28.6922471700024,20.));
#81035=CARTESIAN_POINT('Ctrl Pts',(-38.0879250842874,28.7169777593955,0.));
#81036=CARTESIAN_POINT('Ctrl Pts',(-38.0879250842874,28.7169777593955,20.));
#81037=CARTESIAN_POINT('Ctrl Pts',(-38.0655109398262,28.7416919130413,0.));
#81038=CARTESIAN_POINT('Ctrl Pts',(-38.0655109398262,28.7416919130413,20.));
#81039=CARTESIAN_POINT('Ctrl Pts',(-38.0430803346823,28.76638961953,0.));
#81040=CARTESIAN_POINT('Ctrl Pts',(-38.0430803346823,28.76638961953,20.));
#81041=CARTESIAN_POINT('Ctrl Pts',(-38.020633280384,28.7910708674595,0.));
#81042=CARTESIAN_POINT('Ctrl Pts',(-38.020633280384,28.7910708674595,20.));
#81043=CARTESIAN_POINT('Ctrl Pts',(-37.9981697884679,28.8157356454354,0.));
#81044=CARTESIAN_POINT('Ctrl Pts',(-37.9981697884679,28.8157356454354,20.));
#81045=CARTESIAN_POINT('Ctrl Pts',(-37.975689870479,28.8403839420709,0.));
#81046=CARTESIAN_POINT('Ctrl Pts',(-37.975689870479,28.8403839420709,20.));
#81047=CARTESIAN_POINT('Ctrl Pts',(-37.9531935379708,28.8650157459871,0.));
#81048=CARTESIAN_POINT('Ctrl Pts',(-37.9531935379708,28.8650157459871,20.));
#81049=CARTESIAN_POINT('Ctrl Pts',(-37.9306808025049,28.8896310458131,0.));
#81050=CARTESIAN_POINT('Ctrl Pts',(-37.9306808025049,28.8896310458131,20.));
#81051=CARTESIAN_POINT('Ctrl Pts',(-37.9081516756509,28.9142298301853,0.));
#81052=CARTESIAN_POINT('Ctrl Pts',(-37.9081516756509,28.9142298301853,20.));
#81053=CARTESIAN_POINT('Ctrl Pts',(-37.8856061689868,28.9388120877483,0.));
#81054=CARTESIAN_POINT('Ctrl Pts',(-37.8856061689868,28.9388120877483,20.));
#81055=CARTESIAN_POINT('Ctrl Pts',(-37.8630442940985,28.9633778071544,0.));
#81056=CARTESIAN_POINT('Ctrl Pts',(-37.8630442940985,28.9633778071544,20.));
#81057=CARTESIAN_POINT('Ctrl Pts',(-37.8404660625803,28.9879269770637,0.));
#81058=CARTESIAN_POINT('Ctrl Pts',(-37.8404660625803,28.9879269770637,20.));
#81059=CARTESIAN_POINT('Ctrl Pts',(-37.8178714860345,29.0124595861441,0.));
#81060=CARTESIAN_POINT('Ctrl Pts',(-37.8178714860345,29.0124595861441,20.));
#81061=CARTESIAN_POINT('Ctrl Pts',(-37.7952605760716,29.0369756230713,0.));
#81062=CARTESIAN_POINT('Ctrl Pts',(-37.7952605760716,29.0369756230713,20.));
#81063=CARTESIAN_POINT('Ctrl Pts',(-37.7726333443105,29.0614750765285,0.));
#81064=CARTESIAN_POINT('Ctrl Pts',(-37.7726333443105,29.0614750765285,20.));
#81065=CARTESIAN_POINT('Ctrl Pts',(-37.7499898023785,29.0859579352069,0.));
#81066=CARTESIAN_POINT('Ctrl Pts',(-37.7499898023785,29.0859579352069,20.));
#81067=CARTESIAN_POINT('Ctrl Pts',(-37.7273299619109,29.1104241878056,0.));
#81068=CARTESIAN_POINT('Ctrl Pts',(-37.7273299619109,29.1104241878056,20.));
#81069=CARTESIAN_POINT('Ctrl Pts',(-37.7046538345516,29.1348738230316,0.));
#81070=CARTESIAN_POINT('Ctrl Pts',(-37.7046538345516,29.1348738230316,20.));
#81071=CARTESIAN_POINT('Ctrl Pts',(-37.6819614319523,29.1593068295997,0.));
#81072=CARTESIAN_POINT('Ctrl Pts',(-37.6819614319523,29.1593068295997,20.));
#81073=CARTESIAN_POINT('Ctrl Pts',(-37.6592527657727,29.1837231962328,0.));
#81074=CARTESIAN_POINT('Ctrl Pts',(-37.6592527657727,29.1837231962328,20.));
#81075=CARTESIAN_POINT('Ctrl Pts',(-37.6365278476807,29.208122911661,0.));
#81076=CARTESIAN_POINT('Ctrl Pts',(-37.6365278476807,29.208122911661,20.));
#81077=CARTESIAN_POINT('Ctrl Pts',(-37.613786689352,29.2325059646224,0.));
#81078=CARTESIAN_POINT('Ctrl Pts',(-37.613786689352,29.2325059646224,20.));
#81079=CARTESIAN_POINT('Ctrl Pts',(-37.5910293024705,29.2568723438631,0.));
#81080=CARTESIAN_POINT('Ctrl Pts',(-37.5910293024705,29.2568723438631,20.));
#81081=CARTESIAN_POINT('Ctrl Pts',(-37.5682556987287,29.2812220381372,0.));
#81082=CARTESIAN_POINT('Ctrl Pts',(-37.5682556987287,29.2812220381372,20.));
#81083=CARTESIAN_POINT('Ctrl Pts',(-37.5454658898274,29.3055550362067,0.));
#81084=CARTESIAN_POINT('Ctrl Pts',(-37.5454658898274,29.3055550362067,20.));
#81085=CARTESIAN_POINT('Ctrl Pts',(-37.5226598874754,29.3298713268414,0.));
#81086=CARTESIAN_POINT('Ctrl Pts',(-37.5226598874754,29.3298713268414,20.));
#81087=CARTESIAN_POINT('Ctrl Pts',(-37.4998377033899,29.3541708988191,0.));
#81088=CARTESIAN_POINT('Ctrl Pts',(-37.4998377033899,29.3541708988191,20.));
#81089=CARTESIAN_POINT('Ctrl Pts',(-37.4769993492958,29.378453740925,0.));
#81090=CARTESIAN_POINT('Ctrl Pts',(-37.4769993492958,29.378453740925,20.));
#81091=CARTESIAN_POINT('Ctrl Pts',(-37.4541448369259,29.4027198419524,0.));
#81092=CARTESIAN_POINT('Ctrl Pts',(-37.4541448369259,29.4027198419524,20.));
#81093=CARTESIAN_POINT('Ctrl Pts',(-37.4312741780213,29.4269691907023,0.));
#81094=CARTESIAN_POINT('Ctrl Pts',(-37.4312741780213,29.4269691907023,20.));
#81095=CARTESIAN_POINT('Ctrl Pts',(-37.4083873843313,29.4512017759842,0.));
#81096=CARTESIAN_POINT('Ctrl Pts',(-37.4083873843313,29.4512017759842,20.));
#81097=CARTESIAN_POINT('Ctrl Pts',(-37.3854844676135,29.4754175866156,0.));
#81098=CARTESIAN_POINT('Ctrl Pts',(-37.3854844676135,29.4754175866156,20.));
#81099=CARTESIAN_POINT('Ctrl Pts',(-37.3625654396335,29.4996166114217,0.));
#81100=CARTESIAN_POINT('Ctrl Pts',(-37.3625654396335,29.4996166114217,20.));
#81101=CARTESIAN_POINT('Ctrl Pts',(-37.3396303121646,29.5237988392353,0.));
#81102=CARTESIAN_POINT('Ctrl Pts',(-37.3396303121646,29.5237988392353,20.));
#81103=CARTESIAN_POINT('Ctrl Pts',(-37.3166790969884,29.5479642588972,0.));
#81104=CARTESIAN_POINT('Ctrl Pts',(-37.3166790969884,29.5479642588972,20.));
#81105=CARTESIAN_POINT('Ctrl Pts',(-37.2937118058947,29.5721128592559,0.));
#81106=CARTESIAN_POINT('Ctrl Pts',(-37.2937118058947,29.5721128592559,20.));
#81107=CARTESIAN_POINT('Ctrl Pts',(-37.2707284506814,29.5962446291682,0.));
#81108=CARTESIAN_POINT('Ctrl Pts',(-37.2707284506814,29.5962446291682,20.));
#81109=CARTESIAN_POINT('Ctrl Pts',(-37.2477290431548,29.6203595574991,0.));
#81110=CARTESIAN_POINT('Ctrl Pts',(-37.2477290431548,29.6203595574991,20.));
#81111=CARTESIAN_POINT('Ctrl Pts',(-37.2247135951292,29.6444576331214,0.));
#81112=CARTESIAN_POINT('Ctrl Pts',(-37.2247135951292,29.6444576331214,20.));
#81113=CARTESIAN_POINT('Ctrl Pts',(-37.2016821184267,29.668538844916,0.));
#81114=CARTESIAN_POINT('Ctrl Pts',(-37.2016821184267,29.668538844916,20.));
#81115=CARTESIAN_POINT('Ctrl Pts',(-37.1786346248774,29.6926031817715,0.));
#81116=CARTESIAN_POINT('Ctrl Pts',(-37.1786346248774,29.6926031817715,20.));
#81117=CARTESIAN_POINT('Ctrl Pts',(-37.155571126319,29.7166506325841,0.));
#81118=CARTESIAN_POINT('Ctrl Pts',(-37.155571126319,29.7166506325841,20.));
#81119=CARTESIAN_POINT('Ctrl Pts',(-37.1324916345976,29.7406811862582,0.));
#81120=CARTESIAN_POINT('Ctrl Pts',(-37.1324916345976,29.7406811862582,20.));
#81121=CARTESIAN_POINT('Ctrl Pts',(-37.1093961615672,29.7646948317061,0.));
#81122=CARTESIAN_POINT('Ctrl Pts',(-37.1093961615672,29.7646948317061,20.));
#81123=CARTESIAN_POINT('Ctrl Pts',(-37.0862847190902,29.7886915578485,0.));
#81124=CARTESIAN_POINT('Ctrl Pts',(-37.0862847190902,29.7886915578485,20.));
#81125=CARTESIAN_POINT('Ctrl Pts',(-37.0631573190374,29.8126713536142,0.));
#81126=CARTESIAN_POINT('Ctrl Pts',(-37.0631573190374,29.8126713536142,20.));
#81127=CARTESIAN_POINT('Ctrl Pts',(-37.0400139732874,29.83663420794,0.));
#81128=CARTESIAN_POINT('Ctrl Pts',(-37.0400139732874,29.83663420794,20.));
#81129=CARTESIAN_POINT('Ctrl Pts',(-37.0168546937273,29.8605801097708,0.));
#81130=CARTESIAN_POINT('Ctrl Pts',(-37.0168546937273,29.8605801097708,20.));
#81131=CARTESIAN_POINT('Ctrl Pts',(-36.9936794922513,29.884509048059,0.));
#81132=CARTESIAN_POINT('Ctrl Pts',(-36.9936794922513,29.884509048059,20.));
#81133=CARTESIAN_POINT('Ctrl Pts',(-36.9704883807614,29.9084210117647,0.));
#81134=CARTESIAN_POINT('Ctrl Pts',(-36.9704883807614,29.9084210117647,20.));
#81135=CARTESIAN_POINT('Ctrl Pts',(-36.9472813711676,29.9323159898562,0.));
#81136=CARTESIAN_POINT('Ctrl Pts',(-36.9472813711676,29.9323159898562,20.));
#81137=CARTESIAN_POINT('Ctrl Pts',(-36.9240584753883,29.9561939713102,0.));
#81138=CARTESIAN_POINT('Ctrl Pts',(-36.9240584753883,29.9561939713102,20.));
#81139=CARTESIAN_POINT('Ctrl Pts',(-36.9008197053507,29.9800549451122,0.));
#81140=CARTESIAN_POINT('Ctrl Pts',(-36.9008197053507,29.9800549451122,20.));
#81141=CARTESIAN_POINT('Ctrl Pts',(-36.8775650729895,30.0038989002549,0.));
#81142=CARTESIAN_POINT('Ctrl Pts',(-36.8775650729895,30.0038989002549,20.));
#81143=CARTESIAN_POINT('Ctrl Pts',(-36.8542945902473,30.0277258257393,0.));
#81144=CARTESIAN_POINT('Ctrl Pts',(-36.8542945902473,30.0277258257393,20.));
#81145=CARTESIAN_POINT('Ctrl Pts',(-36.8310082690741,30.0515357105739,0.));
#81146=CARTESIAN_POINT('Ctrl Pts',(-36.8310082690741,30.0515357105739,20.));
#81147=CARTESIAN_POINT('Ctrl Pts',(-36.8077061214283,30.0753285437754,0.));
#81148=CARTESIAN_POINT('Ctrl Pts',(-36.8077061214283,30.0753285437754,20.));
#81149=CARTESIAN_POINT('Ctrl Pts',(-36.784388159276,30.0991043143684,0.));
#81150=CARTESIAN_POINT('Ctrl Pts',(-36.784388159276,30.0991043143684,20.));
#81151=CARTESIAN_POINT('Ctrl Pts',(-36.7610543945915,30.1228630113862,0.));
#81152=CARTESIAN_POINT('Ctrl Pts',(-36.7610543945915,30.1228630113862,20.));
#81153=CARTESIAN_POINT('Ctrl Pts',(-36.7377048393574,30.14660462387,0.));
#81154=CARTESIAN_POINT('Ctrl Pts',(-36.7377048393574,30.14660462387,20.));
#81155=CARTESIAN_POINT('Ctrl Pts',(-36.7143395055641,30.1703291408693,0.));
#81156=CARTESIAN_POINT('Ctrl Pts',(-36.7143395055641,30.1703291408693,20.));
#81157=CARTESIAN_POINT('Ctrl Pts',(-36.6909584052099,30.1940365514414,0.));
#81158=CARTESIAN_POINT('Ctrl Pts',(-36.6909584052099,30.1940365514414,20.));
#81159=CARTESIAN_POINT('Ctrl Pts',(-36.6675615503012,30.2177268446518,0.));
#81160=CARTESIAN_POINT('Ctrl Pts',(-36.6675615503012,30.2177268446518,20.));
#81161=CARTESIAN_POINT('Ctrl Pts',(-36.6441489528521,30.2414000095742,0.));
#81162=CARTESIAN_POINT('Ctrl Pts',(-36.6441489528521,30.2414000095742,20.));
#81163=CARTESIAN_POINT('Ctrl Pts',(-36.6207206248849,30.2650560352902,0.));
#81164=CARTESIAN_POINT('Ctrl Pts',(-36.6207206248849,30.2650560352902,20.));
#81165=CARTESIAN_POINT('Ctrl Pts',(-36.5972765784293,30.2886949108895,0.));
#81166=CARTESIAN_POINT('Ctrl Pts',(-36.5972765784293,30.2886949108895,20.));
#81167=CARTESIAN_POINT('Ctrl Pts',(-36.5738168255233,30.3123166254701,0.));
#81168=CARTESIAN_POINT('Ctrl Pts',(-36.5738168255233,30.3123166254701,20.));
#81169=CARTESIAN_POINT('Ctrl Pts',(-36.5503413782123,30.3359211681375,0.));
#81170=CARTESIAN_POINT('Ctrl Pts',(-36.5503413782123,30.3359211681375,20.));
#81171=CARTESIAN_POINT('Ctrl Pts',(-36.5268502485502,30.3595085280058,0.));
#81172=CARTESIAN_POINT('Ctrl Pts',(-36.5268502485502,30.3595085280058,20.));
#81173=CARTESIAN_POINT('Ctrl Pts',(-36.5033434485984,30.3830786941972,0.));
#81174=CARTESIAN_POINT('Ctrl Pts',(-36.5033434485984,30.3830786941972,20.));
#81175=CARTESIAN_POINT('Ctrl Pts',(-36.4798209904267,30.4066316558423,0.));
#81176=CARTESIAN_POINT('Ctrl Pts',(-36.4798209904267,30.4066316558423,20.));
#81177=CARTESIAN_POINT('Ctrl Pts',(-36.456282886113,30.4301674020801,0.));
#81178=CARTESIAN_POINT('Ctrl Pts',(-36.456282886113,30.4301674020801,20.));
#81179=CARTESIAN_POINT('Ctrl Pts',(-36.4327291477429,30.4536859220576,0.));
#81180=CARTESIAN_POINT('Ctrl Pts',(-36.4327291477429,30.4536859220576,20.));
#81181=CARTESIAN_POINT('Ctrl Pts',(-36.4091597874097,30.4771872049298,0.));
#81182=CARTESIAN_POINT('Ctrl Pts',(-36.4091597874097,30.4771872049298,20.));
#81183=CARTESIAN_POINT('Ctrl Pts',(-36.3855748172148,30.5006712398601,0.));
#81184=CARTESIAN_POINT('Ctrl Pts',(-36.3855748172148,30.5006712398601,20.));
#81185=CARTESIAN_POINT('Ctrl Pts',(-36.3619742492671,30.5241380160195,0.));
#81186=CARTESIAN_POINT('Ctrl Pts',(-36.3619742492671,30.5241380160195,20.));
#81187=CARTESIAN_POINT('Ctrl Pts',(-36.3383580956833,30.5475875225872,0.));
#81188=CARTESIAN_POINT('Ctrl Pts',(-36.3383580956833,30.5475875225872,20.));
#81189=CARTESIAN_POINT('Ctrl Pts',(-36.3147263685875,30.5710197487502,0.));
#81190=CARTESIAN_POINT('Ctrl Pts',(-36.3147263685875,30.5710197487502,20.));
#81191=CARTESIAN_POINT('Ctrl Pts',(-36.2910790801119,30.5944346837039,0.));
#81192=CARTESIAN_POINT('Ctrl Pts',(-36.2910790801119,30.5944346837039,20.));
#81193=CARTESIAN_POINT('Ctrl Pts',(-36.2674162423973,30.6178323166527,0.));
#81194=CARTESIAN_POINT('Ctrl Pts',(-36.2674162423973,30.6178323166527,20.));
#81195=CARTESIAN_POINT('Ctrl Pts',(-36.2437378675924,30.6412126368094,0.));
#81196=CARTESIAN_POINT('Ctrl Pts',(-36.2437378675924,30.6412126368094,20.));
#81197=CARTESIAN_POINT('Ctrl Pts',(-36.2200439678543,30.6645756333954,0.));
#81198=CARTESIAN_POINT('Ctrl Pts',(-36.2200439678543,30.6645756333954,20.));
#81199=CARTESIAN_POINT('Ctrl Pts',(-36.1963345553471,30.6879212956391,0.));
#81200=CARTESIAN_POINT('Ctrl Pts',(-36.1963345553471,30.6879212956391,20.));
#81201=CARTESIAN_POINT('Ctrl Pts',(-36.1726096422428,30.7112496127774,0.));
#81202=CARTESIAN_POINT('Ctrl Pts',(-36.1726096422428,30.7112496127774,20.));
#81203=CARTESIAN_POINT('Ctrl Pts',(-36.1488692407204,30.7345605740544,0.));
#81204=CARTESIAN_POINT('Ctrl Pts',(-36.1488692407204,30.7345605740544,20.));
#81205=CARTESIAN_POINT('Ctrl Pts',(-36.125113362967,30.7578541687236,0.));
#81206=CARTESIAN_POINT('Ctrl Pts',(-36.125113362967,30.7578541687236,20.));
#81207=CARTESIAN_POINT('Ctrl Pts',(-36.1013420211777,30.7811303860468,0.));
#81208=CARTESIAN_POINT('Ctrl Pts',(-36.1013420211777,30.7811303860468,20.));
#81209=CARTESIAN_POINT('Ctrl Pts',(-36.0775552275565,30.8043892152943,0.));
#81210=CARTESIAN_POINT('Ctrl Pts',(-36.0775552275565,30.8043892152943,20.));
#81211=CARTESIAN_POINT('Ctrl Pts',(-36.0537529943146,30.8276306457446,0.));
#81212=CARTESIAN_POINT('Ctrl Pts',(-36.0537529943146,30.8276306457446,20.));
#81213=CARTESIAN_POINT('Ctrl Pts',(-36.0299353336712,30.8508546666841,0.));
#81214=CARTESIAN_POINT('Ctrl Pts',(-36.0299353336712,30.8508546666841,20.));
#81215=CARTESIAN_POINT('Ctrl Pts',(-36.0061022578528,30.8740612674075,0.));
#81216=CARTESIAN_POINT('Ctrl Pts',(-36.0061022578528,30.8740612674075,20.));
#81217=CARTESIAN_POINT('Ctrl Pts',(-35.9822537790931,30.8972504372171,0.));
#81218=CARTESIAN_POINT('Ctrl Pts',(-35.9822537790931,30.8972504372171,20.));
#81219=CARTESIAN_POINT('Ctrl Pts',(-35.9583899096339,30.9204221654236,0.));
#81220=CARTESIAN_POINT('Ctrl Pts',(-35.9583899096339,30.9204221654236,20.));
#81221=CARTESIAN_POINT('Ctrl Pts',(-35.9345106617251,30.9435764413467,0.));
#81222=CARTESIAN_POINT('Ctrl Pts',(-35.9345106617251,30.9435764413467,20.));
#81223=CARTESIAN_POINT('Ctrl Pts',(-35.9106160476245,30.9667132543142,0.));
#81224=CARTESIAN_POINT('Ctrl Pts',(-35.9106160476245,30.9667132543142,20.));
#81225=CARTESIAN_POINT('Ctrl Pts',(-35.886706079598,30.9898325936627,0.));
#81226=CARTESIAN_POINT('Ctrl Pts',(-35.886706079598,30.9898325936627,20.));
#81227=CARTESIAN_POINT('Ctrl Pts',(-35.8627807699193,31.0129344487367,0.));
#81228=CARTESIAN_POINT('Ctrl Pts',(-35.8627807699193,31.0129344487367,20.));
#81229=CARTESIAN_POINT('Ctrl Pts',(-35.8388401308696,31.036018808889,0.));
#81230=CARTESIAN_POINT('Ctrl Pts',(-35.8388401308696,31.036018808889,20.));
#81231=CARTESIAN_POINT('Ctrl Pts',(-35.8148841747376,31.0590856634804,0.));
#81232=CARTESIAN_POINT('Ctrl Pts',(-35.8148841747376,31.0590856634804,20.));
#81233=CARTESIAN_POINT('Ctrl Pts',(-35.7909129138202,31.0821350018809,0.));
#81234=CARTESIAN_POINT('Ctrl Pts',(-35.7909129138202,31.0821350018809,20.));
#81235=CARTESIAN_POINT('Ctrl Pts',(-35.7669263604212,31.1051668134678,0.));
#81236=CARTESIAN_POINT('Ctrl Pts',(-35.7669263604212,31.1051668134678,20.));
#81237=CARTESIAN_POINT('Ctrl Pts',(-35.7429245268523,31.1281810876267,0.));
#81238=CARTESIAN_POINT('Ctrl Pts',(-35.7429245268523,31.1281810876267,20.));
#81239=CARTESIAN_POINT('Ctrl Pts',(-35.7189074254331,31.1511778137516,0.));
#81240=CARTESIAN_POINT('Ctrl Pts',(-35.7189074254331,31.1511778137516,20.));
#81241=CARTESIAN_POINT('Ctrl Pts',(-35.6948750684911,31.1741569812451,0.));
#81242=CARTESIAN_POINT('Ctrl Pts',(-35.6948750684911,31.1741569812451,20.));
#81243=CARTESIAN_POINT('Ctrl Pts',(-35.6708274683619,31.1971185795181,0.));
#81244=CARTESIAN_POINT('Ctrl Pts',(-35.6708274683619,31.1971185795181,20.));
#81245=CARTESIAN_POINT('Ctrl Pts',(-35.6467646373884,31.2200625979904,0.));
#81246=CARTESIAN_POINT('Ctrl Pts',(-35.6467646373884,31.2200625979904,20.));
#81247=CARTESIAN_POINT('Ctrl Pts',(-35.6226865879214,31.24298902609,0.));
#81248=CARTESIAN_POINT('Ctrl Pts',(-35.6226865879214,31.24298902609,20.));
#81249=CARTESIAN_POINT('Ctrl Pts',(-35.5985933323195,31.2658978532533,0.));
#81250=CARTESIAN_POINT('Ctrl Pts',(-35.5985933323195,31.2658978532533,20.));
#81251=CARTESIAN_POINT('Ctrl Pts',(-35.5744848829488,31.288789068925,0.));
#81252=CARTESIAN_POINT('Ctrl Pts',(-35.5744848829488,31.288789068925,20.));
#81253=CARTESIAN_POINT('Ctrl Pts',(-35.5503612521832,31.3116626625581,0.));
#81254=CARTESIAN_POINT('Ctrl Pts',(-35.5503612521832,31.3116626625581,20.));
#81255=CARTESIAN_POINT('Ctrl Pts',(-35.5262224524039,31.3345186236135,0.));
#81256=CARTESIAN_POINT('Ctrl Pts',(-35.5262224524039,31.3345186236135,20.));
#81257=CARTESIAN_POINT('Ctrl Pts',(-35.502068496,31.3573569415605,0.));
#81258=CARTESIAN_POINT('Ctrl Pts',(-35.502068496,31.3573569415605,20.));
#81259=CARTESIAN_POINT('Ctrl Pts',(-35.4778993953681,31.3801776058767,0.));
#81260=CARTESIAN_POINT('Ctrl Pts',(-35.4778993953681,31.3801776058767,20.));
#81261=CARTESIAN_POINT('Ctrl Pts',(-35.4537151629127,31.4029806060482,0.));
#81262=CARTESIAN_POINT('Ctrl Pts',(-35.4537151629127,31.4029806060482,20.));
#81263=CARTESIAN_POINT('Ctrl Pts',(-35.4295158110455,31.4257659315696,0.));
#81264=CARTESIAN_POINT('Ctrl Pts',(-35.4295158110455,31.4257659315696,20.));
#81265=CARTESIAN_POINT('Ctrl Pts',(-35.4053013521866,31.4485335719446,0.));
#81266=CARTESIAN_POINT('Ctrl Pts',(-35.4053013521866,31.4485335719446,20.));
#81267=CARTESIAN_POINT('Ctrl Pts',(-35.3810717987641,31.4712835166857,0.));
#81268=CARTESIAN_POINT('Ctrl Pts',(-35.3810717987641,31.4712835166857,20.));
#81269=CARTESIAN_POINT('Ctrl Pts',(-35.3568271632136,31.4940157553136,0.));
#81270=CARTESIAN_POINT('Ctrl Pts',(-35.3568271632136,31.4940157553136,20.));
#81271=CARTESIAN_POINT('Ctrl Pts',(-35.3325674579779,31.5167302773569,0.));
#81272=CARTESIAN_POINT('Ctrl Pts',(-35.3325674579779,31.5167302773569,20.));
#81273=CARTESIAN_POINT('Ctrl Pts',(-35.3082926955072,31.5394270723526,0.));
#81274=CARTESIAN_POINT('Ctrl Pts',(-35.3082926955072,31.5394270723526,20.));
#81275=CARTESIAN_POINT('Ctrl Pts',(-35.2840028882593,31.5621061298453,0.));
#81276=CARTESIAN_POINT('Ctrl Pts',(-35.2840028882593,31.5621061298453,20.));
#81277=CARTESIAN_POINT('Ctrl Pts',(-35.2596980486997,31.5847674393884,0.));
#81278=CARTESIAN_POINT('Ctrl Pts',(-35.2596980486997,31.5847674393884,20.));
#81279=CARTESIAN_POINT('Ctrl Pts',(-35.2353781893015,31.6074109905439,0.));
#81280=CARTESIAN_POINT('Ctrl Pts',(-35.2353781893015,31.6074109905439,20.));
#81281=CARTESIAN_POINT('Ctrl Pts',(-35.2110433225459,31.6300367728826,0.));
#81282=CARTESIAN_POINT('Ctrl Pts',(-35.2110433225459,31.6300367728826,20.));
#81283=CARTESIAN_POINT('Ctrl Pts',(-35.1866934609214,31.6526447759839,0.));
#81284=CARTESIAN_POINT('Ctrl Pts',(-35.1866934609214,31.6526447759839,20.));
#81285=CARTESIAN_POINT('Ctrl Pts',(-35.1623286169245,31.6752349894358,0.));
#81286=CARTESIAN_POINT('Ctrl Pts',(-35.1623286169245,31.6752349894358,20.));
#81287=CARTESIAN_POINT('Ctrl Pts',(-35.1379488030591,31.6978074028349,0.));
#81288=CARTESIAN_POINT('Ctrl Pts',(-35.1379488030591,31.6978074028349,20.));
#81289=CARTESIAN_POINT('Ctrl Pts',(-35.1135540318367,31.7203620057864,0.));
#81290=CARTESIAN_POINT('Ctrl Pts',(-35.1135540318367,31.7203620057864,20.));
#81291=CARTESIAN_POINT('Ctrl Pts',(-35.0891443157764,31.7428987879034,0.));
#81292=CARTESIAN_POINT('Ctrl Pts',(-35.0891443157764,31.7428987879034,20.));
#81293=CARTESIAN_POINT('Ctrl Pts',(-35.0647196674044,31.7654177388073,0.));
#81294=CARTESIAN_POINT('Ctrl Pts',(-35.0647196674044,31.7654177388073,20.));
#81295=CARTESIAN_POINT('Ctrl Pts',(-35.0402800992547,31.7879188481277,0.));
#81296=CARTESIAN_POINT('Ctrl Pts',(-35.0402800992547,31.7879188481277,20.));
#81297=CARTESIAN_POINT('Ctrl Pts',(-35.0158256238691,31.8104021055032,0.));
#81298=CARTESIAN_POINT('Ctrl Pts',(-35.0158256238691,31.8104021055032,20.));
#81299=CARTESIAN_POINT('Ctrl Pts',(-34.991356253797,31.8328675005809,0.));
#81300=CARTESIAN_POINT('Ctrl Pts',(-34.991356253797,31.8328675005809,20.));
#81301=CARTESIAN_POINT('Ctrl Pts',(-34.9668720015954,31.8553150230168,0.));
#81302=CARTESIAN_POINT('Ctrl Pts',(-34.9668720015954,31.8553150230168,20.));
#81303=CARTESIAN_POINT('Ctrl Pts',(-34.9423728798289,31.8777446624754,0.));
#81304=CARTESIAN_POINT('Ctrl Pts',(-34.9423728798289,31.8777446624754,20.));
#81305=CARTESIAN_POINT('Ctrl Pts',(-34.9178589010694,31.9001564086295,0.));
#81306=CARTESIAN_POINT('Ctrl Pts',(-34.9178589010694,31.9001564086295,20.));
#81307=CARTESIAN_POINT('Ctrl Pts',(-34.8933300778963,31.9225502511603,0.));
#81308=CARTESIAN_POINT('Ctrl Pts',(-34.8933300778963,31.9225502511603,20.));
#81309=CARTESIAN_POINT('Ctrl Pts',(-34.8687864228965,31.9449261797574,0.));
#81310=CARTESIAN_POINT('Ctrl Pts',(-34.8687864228965,31.9449261797574,20.));
#81311=CARTESIAN_POINT('Ctrl Pts',(-34.8442279486644,31.967284184119,0.));
#81312=CARTESIAN_POINT('Ctrl Pts',(-34.8442279486644,31.967284184119,20.));
#81313=CARTESIAN_POINT('Ctrl Pts',(-34.8196546678026,31.9896242539524,0.));
#81314=CARTESIAN_POINT('Ctrl Pts',(-34.8196546678026,31.9896242539524,20.));
#81315=CARTESIAN_POINT('Ctrl Pts',(-34.7950665929206,32.0119463789729,0.));
#81316=CARTESIAN_POINT('Ctrl Pts',(-34.7950665929206,32.0119463789729,20.));
#81317=CARTESIAN_POINT('Ctrl Pts',(-34.7704637366357,32.0342505489048,0.));
#81318=CARTESIAN_POINT('Ctrl Pts',(-34.7704637366357,32.0342505489048,20.));
#81319=CARTESIAN_POINT('Ctrl Pts',(-34.7458461115727,32.0565367534806,0.));
#81320=CARTESIAN_POINT('Ctrl Pts',(-34.7458461115727,32.0565367534806,20.));
#81321=CARTESIAN_POINT('Ctrl Pts',(-34.7212137303638,32.0788049824416,0.));
#81322=CARTESIAN_POINT('Ctrl Pts',(-34.7212137303638,32.0788049824416,20.));
#81323=CARTESIAN_POINT('Ctrl Pts',(-34.6965666056491,32.1010552255378,0.));
#81324=CARTESIAN_POINT('Ctrl Pts',(-34.6965666056491,32.1010552255378,20.));
#81325=CARTESIAN_POINT('Ctrl Pts',(-34.6719047500757,32.1232874725276,0.));
#81326=CARTESIAN_POINT('Ctrl Pts',(-34.6719047500757,32.1232874725276,20.));
#81327=CARTESIAN_POINT('Ctrl Pts',(-34.6472281762982,32.145501713178,0.));
#81328=CARTESIAN_POINT('Ctrl Pts',(-34.6472281762982,32.145501713178,20.));
#81329=CARTESIAN_POINT('Ctrl Pts',(-34.6225368969784,32.167697937264,0.));
#81330=CARTESIAN_POINT('Ctrl Pts',(-34.6225368969784,32.167697937264,20.));
#81331=CARTESIAN_POINT('Ctrl Pts',(-34.5978309247855,32.1898761345694,0.));
#81332=CARTESIAN_POINT('Ctrl Pts',(-34.5978309247855,32.1898761345694,20.));
#81333=CARTESIAN_POINT('Ctrl Pts',(-34.5731102723969,32.212036294887,0.));
#81334=CARTESIAN_POINT('Ctrl Pts',(-34.5731102723969,32.212036294887,20.));
#81335=CARTESIAN_POINT('Ctrl Pts',(-34.5483749524972,32.2341784080183,0.));
#81336=CARTESIAN_POINT('Ctrl Pts',(-34.5483749524972,32.2341784080183,20.));
#81337=CARTESIAN_POINT('Ctrl Pts',(-34.5236249777791,32.2563024637739,0.));
#81338=CARTESIAN_POINT('Ctrl Pts',(-34.5236249777791,32.2563024637739,20.));
#81339=CARTESIAN_POINT('Ctrl Pts',(-34.4988603609427,32.2784084519728,0.));
#81340=CARTESIAN_POINT('Ctrl Pts',(-34.4988603609427,32.2784084519728,20.));
#81341=CARTESIAN_POINT('Ctrl Pts',(-34.474081114695,32.3004963624427,0.));
#81342=CARTESIAN_POINT('Ctrl Pts',(-34.474081114695,32.3004963624427,20.));
#81343=CARTESIAN_POINT('Ctrl Pts',(-34.4492872517507,32.3225661850195,0.));
#81344=CARTESIAN_POINT('Ctrl Pts',(-34.4492872517507,32.3225661850195,20.));
#81345=CARTESIAN_POINT('Ctrl Pts',(-34.4244787848311,32.3446179095473,0.));
#81346=CARTESIAN_POINT('Ctrl Pts',(-34.4244787848311,32.3446179095473,20.));
#81347=CARTESIAN_POINT('Ctrl Pts',(-34.3996557266651,32.3666515258787,0.));
#81348=CARTESIAN_POINT('Ctrl Pts',(-34.3996557266651,32.3666515258787,20.));
#81349=CARTESIAN_POINT('Ctrl Pts',(-34.3748180899889,32.388667023875,0.));
#81350=CARTESIAN_POINT('Ctrl Pts',(-34.3748180899889,32.388667023875,20.));
#81351=CARTESIAN_POINT('Ctrl Pts',(-34.3499658875467,32.4106643934066,0.));
#81352=CARTESIAN_POINT('Ctrl Pts',(-34.3499658875467,32.4106643934066,20.));
#81353=CARTESIAN_POINT('Ctrl Pts',(-34.3250991320905,32.4326436243532,0.));
#81354=CARTESIAN_POINT('Ctrl Pts',(-34.3250991320905,32.4326436243532,20.));
#81355=CARTESIAN_POINT('Ctrl Pts',(-34.3002178363797,32.4546047066033,0.));
#81356=CARTESIAN_POINT('Ctrl Pts',(-34.3002178363797,32.4546047066033,20.));
#81357=CARTESIAN_POINT('Ctrl Pts',(-34.2753220131812,32.4765476300538,0.));
#81358=CARTESIAN_POINT('Ctrl Pts',(-34.2753220131812,32.4765476300538,20.));
#81359=CARTESIAN_POINT('Ctrl Pts',(-34.2504116752689,32.4984723846097,0.));
#81360=CARTESIAN_POINT('Ctrl Pts',(-34.2504116752689,32.4984723846097,20.));
#81361=CARTESIAN_POINT('Ctrl Pts',(-34.2254868354237,32.5203789601849,0.));
#81362=CARTESIAN_POINT('Ctrl Pts',(-34.2254868354237,32.5203789601849,20.));
#81363=CARTESIAN_POINT('Ctrl Pts',(-34.2005475064343,32.542267346702,0.));
#81364=CARTESIAN_POINT('Ctrl Pts',(-34.2005475064343,32.542267346702,20.));
#81365=CARTESIAN_POINT('Ctrl Pts',(-34.1755937010963,32.564137534092,0.));
#81366=CARTESIAN_POINT('Ctrl Pts',(-34.1755937010963,32.564137534092,20.));
#81367=CARTESIAN_POINT('Ctrl Pts',(-34.1506254322131,32.585989512295,0.));
#81368=CARTESIAN_POINT('Ctrl Pts',(-34.1506254322131,32.585989512295,20.));
#81369=CARTESIAN_POINT('Ctrl Pts',(-34.1256427125956,32.6078232712594,0.));
#81370=CARTESIAN_POINT('Ctrl Pts',(-34.1256427125956,32.6078232712594,20.));
#81371=CARTESIAN_POINT('Ctrl Pts',(-34.1006455550618,32.6296388009428,0.));
#81372=CARTESIAN_POINT('Ctrl Pts',(-34.1006455550618,32.6296388009428,20.));
#81373=CARTESIAN_POINT('Ctrl Pts',(-34.0756339724376,32.6514360913116,0.));
#81374=CARTESIAN_POINT('Ctrl Pts',(-34.0756339724376,32.6514360913116,20.));
#81375=CARTESIAN_POINT('Ctrl Pts',(-34.0506079775557,32.6732151323407,0.));
#81376=CARTESIAN_POINT('Ctrl Pts',(-34.0506079775557,32.6732151323407,20.));
#81377=CARTESIAN_POINT('Ctrl Pts',(-34.0255675832564,32.694975914014,0.));
#81378=CARTESIAN_POINT('Ctrl Pts',(-34.0255675832564,32.694975914014,20.));
#81379=CARTESIAN_POINT('Ctrl Pts',(-34.0005128023872,32.7167184263237,0.));
#81380=CARTESIAN_POINT('Ctrl Pts',(-34.0005128023872,32.7167184263237,20.));
#81381=CARTESIAN_POINT('Ctrl Pts',(-33.9754436478026,32.7384426592708,0.));
#81382=CARTESIAN_POINT('Ctrl Pts',(-33.9754436478026,32.7384426592708,20.));
#81383=CARTESIAN_POINT('Ctrl Pts',(-33.9503601323651,32.7601486028652,0.));
#81384=CARTESIAN_POINT('Ctrl Pts',(-33.9503601323651,32.7601486028652,20.));
#81385=CARTESIAN_POINT('Ctrl Pts',(-33.9252622689445,32.781836247126,0.));
#81386=CARTESIAN_POINT('Ctrl Pts',(-33.9252622689445,32.781836247126,20.));
#81387=CARTESIAN_POINT('Ctrl Pts',(-33.9001500704179,32.8035055820805,0.));
#81388=CARTESIAN_POINT('Ctrl Pts',(-33.9001500704179,32.8035055820805,20.));
#81389=CARTESIAN_POINT('Ctrl Pts',(-33.8750235496691,32.8251565977646,0.));
#81390=CARTESIAN_POINT('Ctrl Pts',(-33.8750235496691,32.8251565977646,20.));
#81391=CARTESIAN_POINT('Ctrl Pts',(-33.8498827195893,32.8467892842227,0.));
#81392=CARTESIAN_POINT('Ctrl Pts',(-33.8498827195893,32.8467892842227,20.));
#81393=CARTESIAN_POINT('Ctrl Pts',(-33.8247275930774,32.8684036315085,0.));
#81394=CARTESIAN_POINT('Ctrl Pts',(-33.8247275930774,32.8684036315085,20.));
#81395=CARTESIAN_POINT('Ctrl Pts',(-33.7995581830395,32.8899996296849,0.));
#81396=CARTESIAN_POINT('Ctrl Pts',(-33.7995581830395,32.8899996296849,20.));
#81397=CARTESIAN_POINT('Ctrl Pts',(-33.7743745023893,32.9115772688235,0.));
#81398=CARTESIAN_POINT('Ctrl Pts',(-33.7743745023893,32.9115772688235,20.));
#81399=CARTESIAN_POINT('Ctrl Pts',(-33.7491765640476,32.9331365390046,0.));
#81400=CARTESIAN_POINT('Ctrl Pts',(-33.7491765640476,32.9331365390046,20.));
#81401=CARTESIAN_POINT('Ctrl Pts',(-33.723964380943,32.9546774303179,0.));
#81402=CARTESIAN_POINT('Ctrl Pts',(-33.723964380943,32.9546774303179,20.));
#81403=CARTESIAN_POINT('Ctrl Pts',(-33.6987379660104,32.9761999328604,0.));
#81404=CARTESIAN_POINT('Ctrl Pts',(-33.6987379660104,32.9761999328604,20.));
#81405=CARTESIAN_POINT('Ctrl Pts',(-33.673497332192,32.9977040367383,0.));
#81406=CARTESIAN_POINT('Ctrl Pts',(-33.673497332192,32.9977040367383,20.));
#81407=CARTESIAN_POINT('Ctrl Pts',(-33.6482424924373,33.0191897320665,0.));
#81408=CARTESIAN_POINT('Ctrl Pts',(-33.6482424924373,33.0191897320665,20.));
#81409=CARTESIAN_POINT('Ctrl Pts',(-33.6229734597032,33.0406570089692,0.));
#81410=CARTESIAN_POINT('Ctrl Pts',(-33.6229734597032,33.0406570089692,20.));
#81411=CARTESIAN_POINT('Ctrl Pts',(-33.5976902469543,33.0621058575797,0.));
#81412=CARTESIAN_POINT('Ctrl Pts',(-33.5976902469543,33.0621058575797,20.));
#81413=CARTESIAN_POINT('Ctrl Pts',(-33.572392867162,33.0835362680399,0.));
#81414=CARTESIAN_POINT('Ctrl Pts',(-33.572392867162,33.0835362680399,20.));
#81415=CARTESIAN_POINT('Ctrl Pts',(-33.5470813333053,33.1049482305003,0.));
#81416=CARTESIAN_POINT('Ctrl Pts',(-33.5470813333053,33.1049482305003,20.));
#81417=CARTESIAN_POINT('Ctrl Pts',(-33.5217556583704,33.1263417351207,0.));
#81418=CARTESIAN_POINT('Ctrl Pts',(-33.5217556583704,33.1263417351207,20.));
#81419=CARTESIAN_POINT('Ctrl Pts',(-33.4964158553506,33.1477167720697,0.));
#81420=CARTESIAN_POINT('Ctrl Pts',(-33.4964158553506,33.1477167720697,20.));
#81421=CARTESIAN_POINT('Ctrl Pts',(-33.4710619372468,33.1690733315248,0.));
#81422=CARTESIAN_POINT('Ctrl Pts',(-33.4710619372468,33.1690733315248,20.));
#81423=CARTESIAN_POINT('Ctrl Pts',(-33.4456939170666,33.1904114036721,0.));
#81424=CARTESIAN_POINT('Ctrl Pts',(-33.4456939170666,33.1904114036721,20.));
#81425=CARTESIAN_POINT('Ctrl Pts',(-33.4203118078248,33.2117309787063,0.));
#81426=CARTESIAN_POINT('Ctrl Pts',(-33.4203118078248,33.2117309787063,20.));
#81427=CARTESIAN_POINT('Ctrl Pts',(-33.3949156225429,33.233032046831,0.));
#81428=CARTESIAN_POINT('Ctrl Pts',(-33.3949156225429,33.233032046831,20.));
#81429=CARTESIAN_POINT('Ctrl Pts',(-33.3695053742505,33.2543145982587,0.));
#81430=CARTESIAN_POINT('Ctrl Pts',(-33.3695053742505,33.2543145982587,20.));
#81431=CARTESIAN_POINT('Ctrl Pts',(-33.3440810759838,33.2755786232108,0.));
#81432=CARTESIAN_POINT('Ctrl Pts',(-33.3440810759838,33.2755786232108,20.));
#81433=CARTESIAN_POINT('Ctrl Pts',(-33.3186427407863,33.2968241119176,0.));
#81434=CARTESIAN_POINT('Ctrl Pts',(-33.3186427407863,33.2968241119176,20.));
#81435=CARTESIAN_POINT('Ctrl Pts',(-33.2931903817093,33.318051054619,0.));
#81436=CARTESIAN_POINT('Ctrl Pts',(-33.2931903817093,33.318051054619,20.));
#81437=CARTESIAN_POINT('Ctrl Pts',(-33.2677240118112,33.3392594415636,0.));
#81438=CARTESIAN_POINT('Ctrl Pts',(-33.2677240118112,33.3392594415636,20.));
#81439=CARTESIAN_POINT('Ctrl Pts',(-33.2422436441578,33.3604492630093,0.));
#81440=CARTESIAN_POINT('Ctrl Pts',(-33.2422436441578,33.3604492630093,20.));
#81441=CARTESIAN_POINT('Ctrl Pts',(-33.2167492918215,33.3816205092222,0.));
#81442=CARTESIAN_POINT('Ctrl Pts',(-33.2167492918215,33.3816205092222,20.));
#81443=CARTESIAN_POINT('Ctrl Pts',(-33.1912409678819,33.4027731704774,0.));
#81444=CARTESIAN_POINT('Ctrl Pts',(-33.1912409678819,33.4027731704774,20.));
#81445=CARTESIAN_POINT('Ctrl Pts',(-33.1657186854252,33.4239072370581,0.));
#81446=CARTESIAN_POINT('Ctrl Pts',(-33.1657186854252,33.4239072370581,20.));
#81447=CARTESIAN_POINT('Ctrl Pts',(-33.1401824575448,33.4450226992567,0.));
#81448=CARTESIAN_POINT('Ctrl Pts',(-33.1401824575448,33.4450226992567,20.));
#81449=CARTESIAN_POINT('Ctrl Pts',(-33.1146322973416,33.4661195473749,0.));
#81450=CARTESIAN_POINT('Ctrl Pts',(-33.1146322973416,33.4661195473749,20.));
#81451=CARTESIAN_POINT('Ctrl Pts',(-33.0890682179239,33.4871977717238,0.));
#81452=CARTESIAN_POINT('Ctrl Pts',(-33.0890682179239,33.4871977717238,20.));
#81453=CARTESIAN_POINT('Ctrl Pts',(-33.063490232407,33.5082573626235,0.));
#81454=CARTESIAN_POINT('Ctrl Pts',(-33.063490232407,33.5082573626235,20.));
#81455=CARTESIAN_POINT('Ctrl Pts',(-33.0378983539138,33.5292983104032,0.));
#81456=CARTESIAN_POINT('Ctrl Pts',(-33.0378983539138,33.5292983104032,20.));
#81457=CARTESIAN_POINT('Ctrl Pts',(-33.0122925955739,33.5503206054003,0.));
#81458=CARTESIAN_POINT('Ctrl Pts',(-33.0122925955739,33.5503206054003,20.));
#81459=CARTESIAN_POINT('Ctrl Pts',(-32.986672970524,33.5713242379612,0.));
#81460=CARTESIAN_POINT('Ctrl Pts',(-32.986672970524,33.5713242379612,20.));
#81461=CARTESIAN_POINT('Ctrl Pts',(-32.9610394919081,33.5923091984411,0.));
#81462=CARTESIAN_POINT('Ctrl Pts',(-32.9610394919081,33.5923091984411,20.));
#81463=CARTESIAN_POINT('Ctrl Pts',(-32.935392172877,33.6132754772045,0.));
#81464=CARTESIAN_POINT('Ctrl Pts',(-32.935392172877,33.6132754772045,20.));
#81465=CARTESIAN_POINT('Ctrl Pts',(-32.9097310265884,33.6342230646254,0.));
#81466=CARTESIAN_POINT('Ctrl Pts',(-32.9097310265884,33.6342230646254,20.));
#81467=CARTESIAN_POINT('Ctrl Pts',(-32.8840560662069,33.6551519510862,0.));
#81468=CARTESIAN_POINT('Ctrl Pts',(-32.8840560662069,33.6551519510862,20.));
#81469=CARTESIAN_POINT('Ctrl Pts',(-32.8583673049046,33.6760621269785,0.));
#81470=CARTESIAN_POINT('Ctrl Pts',(-32.8583673049046,33.6760621269785,20.));
#81471=CARTESIAN_POINT('Ctrl Pts',(-32.8326647558606,33.6969535827028,0.));
#81472=CARTESIAN_POINT('Ctrl Pts',(-32.8326647558606,33.6969535827028,20.));
#81473=CARTESIAN_POINT('Ctrl Pts',(-32.8069484322617,33.717826308669,0.));
#81474=CARTESIAN_POINT('Ctrl Pts',(-32.8069484322617,33.717826308669,20.));
#81475=CARTESIAN_POINT('Ctrl Pts',(-32.7812183473018,33.7386802952956,0.));
#81476=CARTESIAN_POINT('Ctrl Pts',(-32.7812183473018,33.7386802952956,20.));
#81477=CARTESIAN_POINT('Ctrl Pts',(-32.7554745141811,33.7595155330097,0.));
#81478=CARTESIAN_POINT('Ctrl Pts',(-32.7554745141811,33.7595155330097,20.));
#81479=CARTESIAN_POINT('Ctrl Pts',(-32.7297169461065,33.7803320122473,0.));
#81480=CARTESIAN_POINT('Ctrl Pts',(-32.7297169461065,33.7803320122473,20.));
#81481=CARTESIAN_POINT('Ctrl Pts',(-32.7039456562922,33.8011297234537,0.));
#81482=CARTESIAN_POINT('Ctrl Pts',(-32.7039456562922,33.8011297234537,20.));
#81483=CARTESIAN_POINT('Ctrl Pts',(-32.6781606579598,33.8219086570836,0.));
#81484=CARTESIAN_POINT('Ctrl Pts',(-32.6781606579598,33.8219086570836,20.));
#81485=CARTESIAN_POINT('Ctrl Pts',(-32.652361964338,33.8426688036011,0.));
#81486=CARTESIAN_POINT('Ctrl Pts',(-32.652361964338,33.8426688036011,20.));
#81487=CARTESIAN_POINT('Ctrl Pts',(-32.6265495886629,33.8634101534794,0.));
#81488=CARTESIAN_POINT('Ctrl Pts',(-32.6265495886629,33.8634101534794,20.));
#81489=CARTESIAN_POINT('Ctrl Pts',(-32.6007235441777,33.8841326972007,0.));
#81490=CARTESIAN_POINT('Ctrl Pts',(-32.6007235441777,33.8841326972007,20.));
#81491=CARTESIAN_POINT('Ctrl Pts',(-32.5748838441319,33.9048364252556,0.));
#81492=CARTESIAN_POINT('Ctrl Pts',(-32.5748838441319,33.9048364252556,20.));
#81493=CARTESIAN_POINT('Ctrl Pts',(-32.5490305017817,33.9255213281433,0.));
#81494=CARTESIAN_POINT('Ctrl Pts',(-32.5490305017817,33.9255213281433,20.));
#81495=CARTESIAN_POINT('Ctrl Pts',(-32.5231635303904,33.9461873963724,0.));
#81496=CARTESIAN_POINT('Ctrl Pts',(-32.5231635303904,33.9461873963724,20.));
#81497=CARTESIAN_POINT('Ctrl Pts',(-32.4972829432285,33.9668346204604,0.));
#81498=CARTESIAN_POINT('Ctrl Pts',(-32.4972829432285,33.9668346204604,20.));
#81499=CARTESIAN_POINT('Ctrl Pts',(-32.4713887535742,33.987462990935,0.));
#81500=CARTESIAN_POINT('Ctrl Pts',(-32.4713887535742,33.987462990935,20.));
#81501=CARTESIAN_POINT('Ctrl Pts',(-32.4454809747123,34.0080724983324,0.));
#81502=CARTESIAN_POINT('Ctrl Pts',(-32.4454809747123,34.0080724983324,20.));
#81503=CARTESIAN_POINT('Ctrl Pts',(-32.4195596199345,34.0286631331978,0.));
#81504=CARTESIAN_POINT('Ctrl Pts',(-32.4195596199345,34.0286631331978,20.));
#81505=CARTESIAN_POINT('Ctrl Pts',(-32.3936247025393,34.0492348860854,0.));
#81506=CARTESIAN_POINT('Ctrl Pts',(-32.3936247025393,34.0492348860854,20.));
#81507=CARTESIAN_POINT('Ctrl Pts',(-32.3676762358321,34.0697877475586,0.));
#81508=CARTESIAN_POINT('Ctrl Pts',(-32.3676762358321,34.0697877475586,20.));
#81509=CARTESIAN_POINT('Ctrl Pts',(-32.3417142331257,34.0903217081898,0.));
#81510=CARTESIAN_POINT('Ctrl Pts',(-32.3417142331257,34.0903217081898,20.));
#81511=CARTESIAN_POINT('Ctrl Pts',(-32.3157387077392,34.1108367585604,0.));
#81512=CARTESIAN_POINT('Ctrl Pts',(-32.3157387077392,34.1108367585604,20.));
#81513=CARTESIAN_POINT('Ctrl Pts',(-32.2897496729991,34.131332889261,0.));
#81514=CARTESIAN_POINT('Ctrl Pts',(-32.2897496729991,34.131332889261,20.));
#81515=CARTESIAN_POINT('Ctrl Pts',(-32.2637471422389,34.1518100908915,0.));
#81516=CARTESIAN_POINT('Ctrl Pts',(-32.2637471422389,34.1518100908915,20.));
#81517=CARTESIAN_POINT('Ctrl Pts',(-32.2377311287994,34.1722683540613,0.));
#81518=CARTESIAN_POINT('Ctrl Pts',(-32.2377311287994,34.1722683540613,20.));
#81519=CARTESIAN_POINT('Ctrl Pts',(-32.2117016460282,34.1927076693883,0.));
#81520=CARTESIAN_POINT('Ctrl Pts',(-32.2117016460282,34.1927076693883,20.));
#81521=CARTESIAN_POINT('Ctrl Pts',(-32.1856587072789,34.2131280274994,0.));
#81522=CARTESIAN_POINT('Ctrl Pts',(-32.1856587072789,34.2131280274994,20.));
#81523=CARTESIAN_POINT('Ctrl Pts',(-32.1596023259127,34.233529419031,0.));
#81524=CARTESIAN_POINT('Ctrl Pts',(-32.1596023259127,34.233529419031,20.));
#81525=CARTESIAN_POINT('Ctrl Pts',(-32.1335325152974,34.2539118346284,0.));
#81526=CARTESIAN_POINT('Ctrl Pts',(-32.1335325152974,34.2539118346284,20.));
#81527=CARTESIAN_POINT('Ctrl Pts',(-32.1074492888083,34.2742752649465,0.));
#81528=CARTESIAN_POINT('Ctrl Pts',(-32.1074492888083,34.2742752649465,20.));
#81529=CARTESIAN_POINT('Ctrl Pts',(-32.081352659827,34.2946197006486,0.));
#81530=CARTESIAN_POINT('Ctrl Pts',(-32.081352659827,34.2946197006486,20.));
#81531=CARTESIAN_POINT('Ctrl Pts',(-32.0552426417428,34.3149451324081,0.));
#81532=CARTESIAN_POINT('Ctrl Pts',(-32.0552426417428,34.3149451324081,20.));
#81533=CARTESIAN_POINT('Ctrl Pts',(-32.0291192479513,34.335251550907,0.));
#81534=CARTESIAN_POINT('Ctrl Pts',(-32.0291192479513,34.335251550907,20.));
#81535=CARTESIAN_POINT('Ctrl Pts',(-32.0029824918551,34.3555389468366,0.));
#81536=CARTESIAN_POINT('Ctrl Pts',(-32.0029824918551,34.3555389468366,20.));
#81537=CARTESIAN_POINT('Ctrl Pts',(-31.9768323868632,34.3758073108972,0.));
#81538=CARTESIAN_POINT('Ctrl Pts',(-31.9768323868632,34.3758073108972,20.));
#81539=CARTESIAN_POINT('Ctrl Pts',(-31.9506689463919,34.3960566337982,0.));
#81540=CARTESIAN_POINT('Ctrl Pts',(-31.9506689463919,34.3960566337982,20.));
#81541=CARTESIAN_POINT('Ctrl Pts',(-31.9244921838641,34.4162869062583,0.));
#81542=CARTESIAN_POINT('Ctrl Pts',(-31.9244921838641,34.4162869062583,20.));
#81543=CARTESIAN_POINT('Ctrl Pts',(-31.8983021127102,34.4364981190057,0.));
#81544=CARTESIAN_POINT('Ctrl Pts',(-31.8983021127102,34.4364981190057,20.));
#81545=CARTESIAN_POINT('Ctrl Pts',(-31.8720987463673,34.4566902627777,0.));
#81546=CARTESIAN_POINT('Ctrl Pts',(-31.8720987463673,34.4566902627777,20.));
#81547=CARTESIAN_POINT('Ctrl Pts',(-31.8458820982794,34.4768633283209,0.));
#81548=CARTESIAN_POINT('Ctrl Pts',(-31.8458820982794,34.4768633283209,20.));
#81549=CARTESIAN_POINT('Ctrl Pts',(-31.819652181897,34.4970173063908,0.));
#81550=CARTESIAN_POINT('Ctrl Pts',(-31.819652181897,34.4970173063908,20.));
#81551=CARTESIAN_POINT('Ctrl Pts',(-31.7934090106771,34.5171521877518,0.));
#81552=CARTESIAN_POINT('Ctrl Pts',(-31.7934090106771,34.5171521877518,20.));
#81553=CARTESIAN_POINT('Ctrl Pts',(-31.7671525980838,34.5372679631777,0.));
#81554=CARTESIAN_POINT('Ctrl Pts',(-31.7671525980838,34.5372679631777,20.));
#81555=CARTESIAN_POINT('Ctrl Pts',(-31.7408829575879,34.5573646234518,0.));
#81556=CARTESIAN_POINT('Ctrl Pts',(-31.7408829575879,34.5573646234518,20.));
#81557=CARTESIAN_POINT('Ctrl Pts',(-31.7146001026678,34.5774421593669,0.));
#81558=CARTESIAN_POINT('Ctrl Pts',(-31.7146001026678,34.5774421593669,20.));
#81559=CARTESIAN_POINT('Ctrl Pts',(-31.6883040468088,34.5975005617252,0.));
#81560=CARTESIAN_POINT('Ctrl Pts',(-31.6883040468088,34.5975005617252,20.));
#81561=CARTESIAN_POINT('Ctrl Pts',(-31.6619948035027,34.6175398213376,0.));
#81562=CARTESIAN_POINT('Ctrl Pts',(-31.6619948035027,34.6175398213376,20.));
#81563=CARTESIAN_POINT('Ctrl Pts',(-31.6356723862475,34.6375599290242,0.));
#81564=CARTESIAN_POINT('Ctrl Pts',(-31.6356723862475,34.6375599290242,20.));
#81565=CARTESIAN_POINT('Ctrl Pts',(-31.609336808548,34.6575608756141,0.));
#81566=CARTESIAN_POINT('Ctrl Pts',(-31.609336808548,34.6575608756141,20.));
#81567=CARTESIAN_POINT('Ctrl Pts',(-31.5829880839157,34.6775426519456,0.));
#81568=CARTESIAN_POINT('Ctrl Pts',(-31.5829880839157,34.6775426519456,20.));
#81569=CARTESIAN_POINT('Ctrl Pts',(-31.556626225869,34.6975052488666,0.));
#81570=CARTESIAN_POINT('Ctrl Pts',(-31.556626225869,34.6975052488666,20.));
#81571=CARTESIAN_POINT('Ctrl Pts',(-31.5302512479332,34.7174486572342,0.));
#81572=CARTESIAN_POINT('Ctrl Pts',(-31.5302512479332,34.7174486572342,20.));
#81573=CARTESIAN_POINT('Ctrl Pts',(-31.5038631636409,34.7373728679152,0.));
#81574=CARTESIAN_POINT('Ctrl Pts',(-31.5038631636409,34.7373728679152,20.));
#81575=CARTESIAN_POINT('Ctrl Pts',(-31.4774619865312,34.7572778717852,0.));
#81576=CARTESIAN_POINT('Ctrl Pts',(-31.4774619865312,34.7572778717852,20.));
#81577=CARTESIAN_POINT('Ctrl Pts',(-31.4510477301503,34.7771636597296,0.));
#81578=CARTESIAN_POINT('Ctrl Pts',(-31.4510477301503,34.7771636597296,20.));
#81579=CARTESIAN_POINT('Ctrl Pts',(-31.4246204080513,34.7970302226433,0.));
#81580=CARTESIAN_POINT('Ctrl Pts',(-31.4246204080513,34.7970302226433,20.));
#81581=CARTESIAN_POINT('Ctrl Pts',(-31.3981800337935,34.8168775514299,0.));
#81582=CARTESIAN_POINT('Ctrl Pts',(-31.3981800337935,34.8168775514299,20.));
#81583=CARTESIAN_POINT('Ctrl Pts',(-31.3717266209434,34.8367056370026,0.));
#81584=CARTESIAN_POINT('Ctrl Pts',(-31.3717266209434,34.8367056370026,20.));
#81585=CARTESIAN_POINT('Ctrl Pts',(-31.3452601830726,34.856514470283,0.));
#81586=CARTESIAN_POINT('Ctrl Pts',(-31.3452601830726,34.856514470283,20.));
#81587=CARTESIAN_POINT('Ctrl Pts',(-31.3187807337598,34.8763040422018,0.));
#81588=CARTESIAN_POINT('Ctrl Pts',(-31.3187807337598,34.8763040422018,20.));
#81589=CARTESIAN_POINT('Ctrl Pts',(-31.2922882865907,34.8960743436995,0.));
#81590=CARTESIAN_POINT('Ctrl Pts',(-31.2922882865907,34.8960743436995,20.));
#81591=CARTESIAN_POINT('Ctrl Pts',(-31.2657828551579,34.9158253657262,0.));
#81592=CARTESIAN_POINT('Ctrl Pts',(-31.2657828551579,34.9158253657262,20.));
#81593=CARTESIAN_POINT('Ctrl Pts',(-31.2392644530613,34.9355570992414,0.));
#81594=CARTESIAN_POINT('Ctrl Pts',(-31.2392644530613,34.9355570992414,20.));
#81595=CARTESIAN_POINT('Ctrl Pts',(-31.2127330939086,34.9552695352152,0.));
#81596=CARTESIAN_POINT('Ctrl Pts',(-31.2127330939086,34.9552695352152,20.));
#81597=CARTESIAN_POINT('Ctrl Pts',(-31.1861887913133,34.9749626646259,0.));
#81598=CARTESIAN_POINT('Ctrl Pts',(-31.1861887913133,34.9749626646259,20.));
#81599=CARTESIAN_POINT('Ctrl Pts',(-31.1596315588953,34.9946364784612,0.));
#81600=CARTESIAN_POINT('Ctrl Pts',(-31.1596315588953,34.9946364784612,20.));
#81601=CARTESIAN_POINT('Ctrl Pts',(-31.1330614102809,35.0142909677175,0.));
#81602=CARTESIAN_POINT('Ctrl Pts',(-31.1330614102809,35.0142909677175,20.));
#81603=CARTESIAN_POINT('Ctrl Pts',(-31.1064783591027,35.0339261234012,0.));
#81604=CARTESIAN_POINT('Ctrl Pts',(-31.1064783591027,35.0339261234012,20.));
#81605=CARTESIAN_POINT('Ctrl Pts',(-31.0798824190004,35.0535419365277,0.));
#81606=CARTESIAN_POINT('Ctrl Pts',(-31.0798824190004,35.0535419365277,20.));
#81607=CARTESIAN_POINT('Ctrl Pts',(-31.0532736036193,35.0731383981212,0.));
#81608=CARTESIAN_POINT('Ctrl Pts',(-31.0532736036193,35.0731383981212,20.));
#81609=CARTESIAN_POINT('Ctrl Pts',(-31.026651926612,35.0927154992152,0.));
#81610=CARTESIAN_POINT('Ctrl Pts',(-31.026651926612,35.0927154992152,20.));
#81611=CARTESIAN_POINT('Ctrl Pts',(-31.0000174016378,35.1122732308527,0.));
#81612=CARTESIAN_POINT('Ctrl Pts',(-31.0000174016378,35.1122732308527,20.));
#81613=CARTESIAN_POINT('Ctrl Pts',(-30.9733700423633,35.131811584087,0.));
#81614=CARTESIAN_POINT('Ctrl Pts',(-30.9733700423633,35.131811584087,20.));
#81615=CARTESIAN_POINT('Ctrl Pts',(-30.9467098624624,35.1513305499814,0.));
#81616=CARTESIAN_POINT('Ctrl Pts',(-30.9467098624624,35.1513305499814,20.));
#81617=CARTESIAN_POINT('Ctrl Pts',(-30.9200368756162,35.170830119609,0.));
#81618=CARTESIAN_POINT('Ctrl Pts',(-30.9200368756162,35.170830119609,20.));
#81619=CARTESIAN_POINT('Ctrl Pts',(-30.8933510955116,35.1903102840518,0.));
#81620=CARTESIAN_POINT('Ctrl Pts',(-30.8933510955116,35.1903102840518,20.));
#81621=CARTESIAN_POINT('Ctrl Pts',(-30.8666525358408,35.2097710343997,0.));
#81622=CARTESIAN_POINT('Ctrl Pts',(-30.8666525358408,35.2097710343997,20.));
#81623=CARTESIAN_POINT('Ctrl Pts',(-30.8399412103027,35.2292123617517,0.));
#81624=CARTESIAN_POINT('Ctrl Pts',(-30.8399412103027,35.2292123617517,20.));
#81625=CARTESIAN_POINT('Ctrl Pts',(-30.8132171326021,35.2486342572162,0.));
#81626=CARTESIAN_POINT('Ctrl Pts',(-30.8132171326021,35.2486342572162,20.));
#81627=CARTESIAN_POINT('Ctrl Pts',(-30.7864803164511,35.2680367119112,0.));
#81628=CARTESIAN_POINT('Ctrl Pts',(-30.7864803164511,35.2680367119112,20.));
#81629=CARTESIAN_POINT('Ctrl Pts',(-30.7597307755696,35.2874197169657,0.));
#81630=CARTESIAN_POINT('Ctrl Pts',(-30.7597307755696,35.2874197169657,20.));
#81631=CARTESIAN_POINT('Ctrl Pts',(-30.732968523684,35.3067832635176,0.));
#81632=CARTESIAN_POINT('Ctrl Pts',(-30.732968523684,35.3067832635176,20.));
#81633=CARTESIAN_POINT('Ctrl Pts',(-30.7061935745273,35.3261273427148,0.));
#81634=CARTESIAN_POINT('Ctrl Pts',(-30.7061935745273,35.3261273427148,20.));
#81635=CARTESIAN_POINT('Ctrl Pts',(-30.6794059418388,35.3454519457137,0.));
#81636=CARTESIAN_POINT('Ctrl Pts',(-30.6794059418388,35.3454519457137,20.));
#81637=CARTESIAN_POINT('Ctrl Pts',(-30.6526056393639,35.3647570636798,0.));
#81638=CARTESIAN_POINT('Ctrl Pts',(-30.6526056393639,35.3647570636798,20.));
#81639=CARTESIAN_POINT('Ctrl Pts',(-30.6257926808542,35.3840426877879,0.));
#81640=CARTESIAN_POINT('Ctrl Pts',(-30.6257926808542,35.3840426877879,20.));
#81641=CARTESIAN_POINT('Ctrl Pts',(-30.5989670800681,35.4033088092225,0.));
#81642=CARTESIAN_POINT('Ctrl Pts',(-30.5989670800681,35.4033088092225,20.));
#81643=CARTESIAN_POINT('Ctrl Pts',(-30.5721288507715,35.4225554191786,0.));
#81644=CARTESIAN_POINT('Ctrl Pts',(-30.5721288507715,35.4225554191786,20.));
#81645=CARTESIAN_POINT('Ctrl Pts',(-30.5452780067369,35.4417825088605,0.));
#81646=CARTESIAN_POINT('Ctrl Pts',(-30.5452780067369,35.4417825088605,20.));
#81647=CARTESIAN_POINT('Ctrl Pts',(-30.5184145617425,35.4609900694812,0.));
#81648=CARTESIAN_POINT('Ctrl Pts',(-30.5184145617425,35.4609900694812,20.));
#81649=CARTESIAN_POINT('Ctrl Pts',(-30.4915385295724,35.4801780922625,0.));
#81650=CARTESIAN_POINT('Ctrl Pts',(-30.4915385295724,35.4801780922625,20.));
#81651=CARTESIAN_POINT('Ctrl Pts',(-30.4646499240178,35.4993465684361,0.));
#81652=CARTESIAN_POINT('Ctrl Pts',(-30.4646499240178,35.4993465684361,20.));
#81653=CARTESIAN_POINT('Ctrl Pts',(-30.437748758876,35.518495489243,0.));
#81654=CARTESIAN_POINT('Ctrl Pts',(-30.437748758876,35.518495489243,20.));
#81655=CARTESIAN_POINT('Ctrl Pts',(-30.4108350479521,35.5376248459348,0.));
#81656=CARTESIAN_POINT('Ctrl Pts',(-30.4108350479521,35.5376248459348,20.));
#81657=CARTESIAN_POINT('Ctrl Pts',(-30.3839088050584,35.5567346297736,0.));
#81658=CARTESIAN_POINT('Ctrl Pts',(-30.3839088050584,35.5567346297736,20.));
#81659=CARTESIAN_POINT('Ctrl Pts',(-30.3569700440131,35.5758248320301,0.));
#81660=CARTESIAN_POINT('Ctrl Pts',(-30.3569700440131,35.5758248320301,20.));
#81661=CARTESIAN_POINT('Ctrl Pts',(-30.3300187786403,35.5948954439837,0.));
#81662=CARTESIAN_POINT('Ctrl Pts',(-30.3300187786403,35.5948954439837,20.));
#81663=CARTESIAN_POINT('Ctrl Pts',(-30.3030550227693,35.6139464569223,0.));
#81664=CARTESIAN_POINT('Ctrl Pts',(-30.3030550227693,35.6139464569223,20.));
#81665=CARTESIAN_POINT('Ctrl Pts',(-30.2760787902362,35.6329778621436,0.));
#81666=CARTESIAN_POINT('Ctrl Pts',(-30.2760787902362,35.6329778621436,20.));
#81667=CARTESIAN_POINT('Ctrl Pts',(-30.2490900948838,35.6519896509552,0.));
#81668=CARTESIAN_POINT('Ctrl Pts',(-30.2490900948838,35.6519896509552,20.));
#81669=CARTESIAN_POINT('Ctrl Pts',(-30.2220889505625,35.6709818146751,0.));
#81670=CARTESIAN_POINT('Ctrl Pts',(-30.2220889505625,35.6709818146751,20.));
#81671=CARTESIAN_POINT('Ctrl Pts',(-30.1950753711288,35.6899543446308,0.));
#81672=CARTESIAN_POINT('Ctrl Pts',(-30.1950753711288,35.6899543446308,20.));
#81673=CARTESIAN_POINT('Ctrl Pts',(-30.1680493704465,35.7089072321597,0.));
#81674=CARTESIAN_POINT('Ctrl Pts',(-30.1680493704465,35.7089072321597,20.));
#81675=CARTESIAN_POINT('Ctrl Pts',(-30.141010962385,35.7278404686079,0.));
#81676=CARTESIAN_POINT('Ctrl Pts',(-30.141010962385,35.7278404686079,20.));
#81677=CARTESIAN_POINT('Ctrl Pts',(-30.1139601608197,35.7467540453308,0.));
#81678=CARTESIAN_POINT('Ctrl Pts',(-30.1139601608197,35.7467540453308,20.));
#81679=CARTESIAN_POINT('Ctrl Pts',(-30.0868969796328,35.7656479536938,0.));
#81680=CARTESIAN_POINT('Ctrl Pts',(-30.0868969796328,35.7656479536938,20.));
#81681=CARTESIAN_POINT('Ctrl Pts',(-30.0598214327127,35.7845221850715,0.));
#81682=CARTESIAN_POINT('Ctrl Pts',(-30.0598214327127,35.7845221850715,20.));
#81683=CARTESIAN_POINT('Ctrl Pts',(-30.0327335339539,35.8033767308478,0.));
#81684=CARTESIAN_POINT('Ctrl Pts',(-30.0327335339539,35.8033767308478,20.));
#81685=CARTESIAN_POINT('Ctrl Pts',(-30.005633297258,35.8222115824166,0.));
#81686=CARTESIAN_POINT('Ctrl Pts',(-30.005633297258,35.8222115824166,20.));
#81687=CARTESIAN_POINT('Ctrl Pts',(-29.9785207365333,35.841026731182,0.));
#81688=CARTESIAN_POINT('Ctrl Pts',(-29.9785207365333,35.841026731182,20.));
#81689=CARTESIAN_POINT('Ctrl Pts',(-29.9513958656946,35.8598221685576,0.));
#81690=CARTESIAN_POINT('Ctrl Pts',(-29.9513958656946,35.8598221685576,20.));
#81691=CARTESIAN_POINT('Ctrl Pts',(-29.9242586986624,35.8785978859658,0.));
#81692=CARTESIAN_POINT('Ctrl Pts',(-29.9242586986624,35.8785978859658,20.));
#81693=CARTESIAN_POINT('Ctrl Pts',(-29.8971092493635,35.8973538748387,0.));
#81694=CARTESIAN_POINT('Ctrl Pts',(-29.8971092493635,35.8973538748387,20.));
#81695=CARTESIAN_POINT('Ctrl Pts',(-29.869947531731,35.9160901266176,0.));
#81696=CARTESIAN_POINT('Ctrl Pts',(-29.869947531731,35.9160901266176,20.));
#81697=CARTESIAN_POINT('Ctrl Pts',(-29.8427735597049,35.9348066327539,0.));
#81698=CARTESIAN_POINT('Ctrl Pts',(-29.8427735597049,35.9348066327539,20.));
#81699=CARTESIAN_POINT('Ctrl Pts',(-29.8155873472308,35.9535033847081,0.));
#81700=CARTESIAN_POINT('Ctrl Pts',(-29.8155873472308,35.9535033847081,20.));
#81701=CARTESIAN_POINT('Ctrl Pts',(-29.7883889082614,35.9721803739509,0.));
#81702=CARTESIAN_POINT('Ctrl Pts',(-29.7883889082614,35.9721803739509,20.));
#81703=CARTESIAN_POINT('Ctrl Pts',(-29.7611782567557,35.9908375919623,0.));
#81704=CARTESIAN_POINT('Ctrl Pts',(-29.7611782567557,35.9908375919623,20.));
#81705=CARTESIAN_POINT('Ctrl Pts',(-29.7339554066796,36.009475030233,0.));
#81706=CARTESIAN_POINT('Ctrl Pts',(-29.7339554066796,36.009475030233,20.));
#81707=CARTESIAN_POINT('Ctrl Pts',(-29.7067203720053,36.0280926802632,0.));
#81708=CARTESIAN_POINT('Ctrl Pts',(-29.7067203720053,36.0280926802632,20.));
#81709=CARTESIAN_POINT('Ctrl Pts',(-29.6794731667107,36.0466905335617,0.));
#81710=CARTESIAN_POINT('Ctrl Pts',(-29.6794731667107,36.0466905335617,20.));
#81711=CARTESIAN_POINT('Ctrl Pts',(-29.6522138047794,36.0652685816464,0.));
#81712=CARTESIAN_POINT('Ctrl Pts',(-29.6522138047794,36.0652685816464,20.));
#81713=CARTESIAN_POINT('Ctrl Pts',(-29.6249423002017,36.0838268160451,0.));
#81714=CARTESIAN_POINT('Ctrl Pts',(-29.6249423002017,36.0838268160451,20.));
#81715=CARTESIAN_POINT('Ctrl Pts',(-29.5976586669748,36.1023652282957,0.));
#81716=CARTESIAN_POINT('Ctrl Pts',(-29.5976586669748,36.1023652282957,20.));
#81717=CARTESIAN_POINT('Ctrl Pts',(-29.5703629191022,36.120883809946,0.));
#81718=CARTESIAN_POINT('Ctrl Pts',(-29.5703629191022,36.120883809946,20.));
#81719=CARTESIAN_POINT('Ctrl Pts',(-29.5430550705938,36.1393825525541,0.));
#81720=CARTESIAN_POINT('Ctrl Pts',(-29.5430550705938,36.1393825525541,20.));
#81721=CARTESIAN_POINT('Ctrl Pts',(-29.5157351354652,36.1578614476865,0.));
#81722=CARTESIAN_POINT('Ctrl Pts',(-29.5157351354652,36.1578614476865,20.));
#81723=CARTESIAN_POINT('Ctrl Pts',(-29.4884031277381,36.1763204869192,0.));
#81724=CARTESIAN_POINT('Ctrl Pts',(-29.4884031277381,36.1763204869192,20.));
#81725=CARTESIAN_POINT('Ctrl Pts',(-29.4610590614411,36.1947596618382,0.));
#81726=CARTESIAN_POINT('Ctrl Pts',(-29.4610590614411,36.1947596618382,20.));
#81727=CARTESIAN_POINT('Ctrl Pts',(-29.4337029506094,36.2131789640396,0.));
#81728=CARTESIAN_POINT('Ctrl Pts',(-29.4337029506094,36.2131789640396,20.));
#81729=CARTESIAN_POINT('Ctrl Pts',(-29.4063348092849,36.2315783851295,0.));
#81730=CARTESIAN_POINT('Ctrl Pts',(-29.4063348092849,36.2315783851295,20.));
#81731=CARTESIAN_POINT('Ctrl Pts',(-29.3789546515147,36.2499579167227,0.));
#81732=CARTESIAN_POINT('Ctrl Pts',(-29.3789546515147,36.2499579167227,20.));
#81733=CARTESIAN_POINT('Ctrl Pts',(-29.3515624913523,36.2683175504441,0.));
#81734=CARTESIAN_POINT('Ctrl Pts',(-29.3515624913523,36.2683175504441,20.));
#81735=CARTESIAN_POINT('Ctrl Pts',(-29.3241583428569,36.286657277928,0.));
#81736=CARTESIAN_POINT('Ctrl Pts',(-29.3241583428569,36.286657277928,20.));
#81737=CARTESIAN_POINT('Ctrl Pts',(-29.2967422200943,36.3049770908188,0.));
#81738=CARTESIAN_POINT('Ctrl Pts',(-29.2967422200943,36.3049770908188,20.));
#81739=CARTESIAN_POINT('Ctrl Pts',(-29.2693141371364,36.3232769807701,0.));
#81740=CARTESIAN_POINT('Ctrl Pts',(-29.2693141371364,36.3232769807701,20.));
#81741=CARTESIAN_POINT('Ctrl Pts',(-29.241874108062,36.3415569394456,0.));
#81742=CARTESIAN_POINT('Ctrl Pts',(-29.241874108062,36.3415569394456,20.));
#81743=CARTESIAN_POINT('Ctrl Pts',(-29.2144221469563,36.3598169585186,0.));
#81744=CARTESIAN_POINT('Ctrl Pts',(-29.2144221469563,36.3598169585186,20.));
#81745=CARTESIAN_POINT('Ctrl Pts',(-29.186958267911,36.3780570296725,0.));
#81746=CARTESIAN_POINT('Ctrl Pts',(-29.186958267911,36.3780570296725,20.));
#81747=CARTESIAN_POINT('Ctrl Pts',(-29.1594824850239,36.3962771446002,0.));
#81748=CARTESIAN_POINT('Ctrl Pts',(-29.1594824850239,36.3962771446002,20.));
#81749=CARTESIAN_POINT('Ctrl Pts',(-29.1319948123985,36.4144772950043,0.));
#81750=CARTESIAN_POINT('Ctrl Pts',(-29.1319948123985,36.4144772950043,20.));
#81751=CARTESIAN_POINT('Ctrl Pts',(-29.1044952641443,36.4326574725969,0.));
#81752=CARTESIAN_POINT('Ctrl Pts',(-29.1044952641443,36.4326574725969,20.));
#81753=CARTESIAN_POINT('Ctrl Pts',(-29.0769838543763,36.4508176690994,0.));
#81754=CARTESIAN_POINT('Ctrl Pts',(-29.0769838543763,36.4508176690994,20.));
#81755=CARTESIAN_POINT('Ctrl Pts',(-29.0494605972165,36.4689578762435,0.));
#81756=CARTESIAN_POINT('Ctrl Pts',(-29.0494605972165,36.4689578762435,20.));
#81757=CARTESIAN_POINT('Ctrl Pts',(-29.0219255067927,36.4870780857703,0.));
#81758=CARTESIAN_POINT('Ctrl Pts',(-29.0219255067927,36.4870780857703,20.));
#81759=CARTESIAN_POINT('Ctrl Pts',(-28.99437859724,36.5051782894316,0.));
#81760=CARTESIAN_POINT('Ctrl Pts',(-28.99437859724,36.5051782894316,20.));
#81761=CARTESIAN_POINT('Ctrl Pts',(-28.9668198826995,36.5232584789885,0.));
#81762=CARTESIAN_POINT('Ctrl Pts',(-28.9668198826995,36.5232584789885,20.));
#81763=CARTESIAN_POINT('Ctrl Pts',(-28.9392493773185,36.5413186462123,0.));
#81764=CARTESIAN_POINT('Ctrl Pts',(-28.9392493773185,36.5413186462123,20.));
#81765=CARTESIAN_POINT('Ctrl Pts',(-28.9116670952497,36.5593587828826,0.));
#81766=CARTESIAN_POINT('Ctrl Pts',(-28.9116670952497,36.5593587828826,20.));
#81767=CARTESIAN_POINT('Ctrl Pts',(-28.8840730506515,36.577378880789,0.));
#81768=CARTESIAN_POINT('Ctrl Pts',(-28.8840730506515,36.577378880789,20.));
#81769=CARTESIAN_POINT('Ctrl Pts',(-28.8564672576885,36.5953789317305,0.));
#81770=CARTESIAN_POINT('Ctrl Pts',(-28.8564672576885,36.5953789317305,20.));
#81771=CARTESIAN_POINT('Ctrl Pts',(-28.8288497305324,36.6133589275174,0.));
#81772=CARTESIAN_POINT('Ctrl Pts',(-28.8288497305324,36.6133589275174,20.));
#81773=CARTESIAN_POINT('Ctrl Pts',(-28.8012204833609,36.6313188599694,0.));
#81774=CARTESIAN_POINT('Ctrl Pts',(-28.8012204833609,36.6313188599694,20.));
#81775=CARTESIAN_POINT('Ctrl Pts',(-28.7735795303585,36.6492587209167,0.));
#81776=CARTESIAN_POINT('Ctrl Pts',(-28.7735795303585,36.6492587209167,20.));
#81777=CARTESIAN_POINT('Ctrl Pts',(-28.7459268857152,36.6671785021988,0.));
#81778=CARTESIAN_POINT('Ctrl Pts',(-28.7459268857152,36.6671785021988,20.));
#81779=CARTESIAN_POINT('Ctrl Pts',(-28.7182625636274,36.6850781956649,0.));
#81780=CARTESIAN_POINT('Ctrl Pts',(-28.7182625636274,36.6850781956649,20.));
#81781=CARTESIAN_POINT('Ctrl Pts',(-28.6905865782966,36.7029577931733,0.));
#81782=CARTESIAN_POINT('Ctrl Pts',(-28.6905865782966,36.7029577931733,20.));
#81783=CARTESIAN_POINT('Ctrl Pts',(-28.6628989439305,36.7208172865919,0.));
#81784=CARTESIAN_POINT('Ctrl Pts',(-28.6628989439305,36.7208172865919,20.));
#81785=CARTESIAN_POINT('Ctrl Pts',(-28.6351996747428,36.738656667798,0.));
#81786=CARTESIAN_POINT('Ctrl Pts',(-28.6351996747428,36.738656667798,20.));
#81787=CARTESIAN_POINT('Ctrl Pts',(-28.6074887849535,36.7564759286795,0.));
#81788=CARTESIAN_POINT('Ctrl Pts',(-28.6074887849535,36.7564759286795,20.));
#81789=CARTESIAN_POINT('Ctrl Pts',(-28.5797662887891,36.774275061134,0.));
#81790=CARTESIAN_POINT('Ctrl Pts',(-28.5797662887891,36.774275061134,20.));
#81791=CARTESIAN_POINT('Ctrl Pts',(-28.5520322004825,36.7920540570698,0.));
#81792=CARTESIAN_POINT('Ctrl Pts',(-28.5520322004825,36.7920540570698,20.));
#81793=CARTESIAN_POINT('Ctrl Pts',(-28.5242865342725,36.809812908405,0.));
#81794=CARTESIAN_POINT('Ctrl Pts',(-28.5242865342725,36.809812908405,20.));
#81795=CARTESIAN_POINT('Ctrl Pts',(-28.496529304404,36.8275516070676,0.));
#81796=CARTESIAN_POINT('Ctrl Pts',(-28.496529304404,36.8275516070676,20.));
#81797=CARTESIAN_POINT('Ctrl Pts',(-28.4687605251277,36.8452701449948,0.));
#81798=CARTESIAN_POINT('Ctrl Pts',(-28.4687605251277,36.8452701449948,20.));
#81799=CARTESIAN_POINT('Ctrl Pts',(-28.4409802107003,36.8629685141338,0.));
#81800=CARTESIAN_POINT('Ctrl Pts',(-28.4409802107003,36.8629685141338,20.));
#81801=CARTESIAN_POINT('Ctrl Pts',(-28.4131883753841,36.8806467064409,0.));
#81802=CARTESIAN_POINT('Ctrl Pts',(-28.4131883753841,36.8806467064409,20.));
#81803=CARTESIAN_POINT('Ctrl Pts',(-28.3853850334476,36.8983047138822,0.));
#81804=CARTESIAN_POINT('Ctrl Pts',(-28.3853850334476,36.8983047138822,20.));
#81805=CARTESIAN_POINT('Ctrl Pts',(-28.3575701991656,36.9159425284342,0.));
#81806=CARTESIAN_POINT('Ctrl Pts',(-28.3575701991656,36.9159425284342,20.));
#81807=CARTESIAN_POINT('Ctrl Pts',(-28.3297438868192,36.9335601420835,0.));
#81808=CARTESIAN_POINT('Ctrl Pts',(-28.3297438868192,36.9335601420835,20.));
#81809=CARTESIAN_POINT('Ctrl Pts',(-28.3019061106957,36.9511575468269,0.));
#81810=CARTESIAN_POINT('Ctrl Pts',(-28.3019061106957,36.9511575468269,20.));
#81811=CARTESIAN_POINT('Ctrl Pts',(-28.2740568850882,36.9687347346709,0.));
#81812=CARTESIAN_POINT('Ctrl Pts',(-28.2740568850882,36.9687347346709,20.));
#81813=CARTESIAN_POINT('Ctrl Pts',(-28.2461962242955,36.9862916976318,0.));
#81814=CARTESIAN_POINT('Ctrl Pts',(-28.2461962242955,36.9862916976318,20.));
#81815=CARTESIAN_POINT('Ctrl Pts',(-28.2183241426219,37.0038284277349,0.));
#81816=CARTESIAN_POINT('Ctrl Pts',(-28.2183241426219,37.0038284277349,20.));
#81817=CARTESIAN_POINT('Ctrl Pts',(-28.1904406543778,37.0213449170157,0.));
#81818=CARTESIAN_POINT('Ctrl Pts',(-28.1904406543778,37.0213449170157,20.));
#81819=CARTESIAN_POINT('Ctrl Pts',(-28.1625457738798,37.0388411575197,0.));
#81820=CARTESIAN_POINT('Ctrl Pts',(-28.1625457738798,37.0388411575197,20.));
#81821=CARTESIAN_POINT('Ctrl Pts',(-28.1346395154507,37.0563171413025,0.));
#81822=CARTESIAN_POINT('Ctrl Pts',(-28.1346395154507,37.0563171413025,20.));
#81823=CARTESIAN_POINT('Ctrl Pts',(-28.1067218934195,37.0737728604297,0.));
#81824=CARTESIAN_POINT('Ctrl Pts',(-28.1067218934195,37.0737728604297,20.));
#81825=CARTESIAN_POINT('Ctrl Pts',(-28.0787929221219,37.0912083069771,0.));
#81826=CARTESIAN_POINT('Ctrl Pts',(-28.0787929221219,37.0912083069771,20.));
#81827=CARTESIAN_POINT('Ctrl Pts',(-28.0508526158994,37.1086234730311,0.));
#81828=CARTESIAN_POINT('Ctrl Pts',(-28.0508526158994,37.1086234730311,20.));
#81829=CARTESIAN_POINT('Ctrl Pts',(-28.0229009890986,37.1260183506872,0.));
#81830=CARTESIAN_POINT('Ctrl Pts',(-28.0229009890986,37.1260183506872,20.));
#81831=CARTESIAN_POINT('Ctrl Pts',(-27.994938056072,37.1433929320507,0.));
#81832=CARTESIAN_POINT('Ctrl Pts',(-27.994938056072,37.1433929320507,20.));
#81833=CARTESIAN_POINT('Ctrl Pts',(-27.9669638311771,37.1607472092352,0.));
#81834=CARTESIAN_POINT('Ctrl Pts',(-27.9669638311771,37.1607472092352,20.));
#81835=CARTESIAN_POINT('Ctrl Pts',(-27.9389783287777,37.1780811743651,0.));
#81836=CARTESIAN_POINT('Ctrl Pts',(-27.9389783287777,37.1780811743651,20.));
#81837=CARTESIAN_POINT('Ctrl Pts',(-27.9109815632437,37.1953948195748,0.));
#81838=CARTESIAN_POINT('Ctrl Pts',(-27.9109815632437,37.1953948195748,20.));
#81839=CARTESIAN_POINT('Ctrl Pts',(-27.8829735489517,37.2126881370093,0.));
#81840=CARTESIAN_POINT('Ctrl Pts',(-27.8829735489517,37.2126881370093,20.));
#81841=CARTESIAN_POINT('Ctrl Pts',(-27.8549543002843,37.2299611188238,0.));
#81842=CARTESIAN_POINT('Ctrl Pts',(-27.8549543002843,37.2299611188238,20.));
#81843=CARTESIAN_POINT('Ctrl Pts',(-27.8269238316305,37.2472137571841,0.));
#81844=CARTESIAN_POINT('Ctrl Pts',(-27.8269238316305,37.2472137571841,20.));
#81845=CARTESIAN_POINT('Ctrl Pts',(-27.7988821573847,37.2644460442654,0.));
#81846=CARTESIAN_POINT('Ctrl Pts',(-27.7988821573847,37.2644460442654,20.));
#81847=CARTESIAN_POINT('Ctrl Pts',(-27.7708292919468,37.2816579722525,0.));
#81848=CARTESIAN_POINT('Ctrl Pts',(-27.7708292919468,37.2816579722525,20.));
#81849=CARTESIAN_POINT('Ctrl Pts',(-27.7427652497224,37.2988495333397,0.));
#81850=CARTESIAN_POINT('Ctrl Pts',(-27.7427652497224,37.2988495333397,20.));
#81851=CARTESIAN_POINT('Ctrl Pts',(-27.7146900451229,37.3160207197314,0.));
#81852=CARTESIAN_POINT('Ctrl Pts',(-27.7146900451229,37.3160207197314,20.));
#81853=CARTESIAN_POINT('Ctrl Pts',(-27.6866036925651,37.3331715236413,0.));
#81854=CARTESIAN_POINT('Ctrl Pts',(-27.6866036925651,37.3331715236413,20.));
#81855=CARTESIAN_POINT('Ctrl Pts',(-27.6585062064726,37.3503019372939,0.));
#81856=CARTESIAN_POINT('Ctrl Pts',(-27.6585062064726,37.3503019372939,20.));
#81857=CARTESIAN_POINT('Ctrl Pts',(-27.6303976012745,37.3674119529233,0.));
#81858=CARTESIAN_POINT('Ctrl Pts',(-27.6303976012745,37.3674119529233,20.));
#81859=CARTESIAN_POINT('Ctrl Pts',(-27.6022778914064,37.384501562775,0.));
#81860=CARTESIAN_POINT('Ctrl Pts',(-27.6022778914064,37.384501562775,20.));
#81861=CARTESIAN_POINT('Ctrl Pts',(-27.5741470913095,37.4015707591036,0.));
#81862=CARTESIAN_POINT('Ctrl Pts',(-27.5741470913095,37.4015707591036,20.));
#81863=CARTESIAN_POINT('Ctrl Pts',(-27.5460052154308,37.418619534174,0.));
#81864=CARTESIAN_POINT('Ctrl Pts',(-27.5460052154308,37.418619534174,20.));
#81865=CARTESIAN_POINT('Ctrl Pts',(-27.5178522782226,37.4356478802604,0.));
#81866=CARTESIAN_POINT('Ctrl Pts',(-27.5178522782226,37.4356478802604,20.));
#81867=CARTESIAN_POINT('Ctrl Pts',(-27.489688294143,37.4526557896465,0.));
#81868=CARTESIAN_POINT('Ctrl Pts',(-27.489688294143,37.4526557896465,20.));
#81869=CARTESIAN_POINT('Ctrl Pts',(-27.4615132776558,37.4696432546266,0.));
#81870=CARTESIAN_POINT('Ctrl Pts',(-27.4615132776558,37.4696432546266,20.));
#81871=CARTESIAN_POINT('Ctrl Pts',(-27.4333272432311,37.4866102675047,0.));
#81872=CARTESIAN_POINT('Ctrl Pts',(-27.4333272432311,37.4866102675047,20.));
#81873=CARTESIAN_POINT('Ctrl Pts',(-27.4051302053449,37.5035568205959,0.));
#81874=CARTESIAN_POINT('Ctrl Pts',(-27.4051302053449,37.5035568205959,20.));
#81875=CARTESIAN_POINT('Ctrl Pts',(-27.3769221784798,37.5204829062256,0.));
#81876=CARTESIAN_POINT('Ctrl Pts',(-27.3769221784798,37.5204829062256,20.));
#81877=CARTESIAN_POINT('Ctrl Pts',(-27.3487031771241,37.5373885167297,0.));
#81878=CARTESIAN_POINT('Ctrl Pts',(-27.3487031771241,37.5373885167297,20.));
#81879=CARTESIAN_POINT('Ctrl Pts',(-27.3204732157704,37.5542736444521,0.));
#81880=CARTESIAN_POINT('Ctrl Pts',(-27.3204732157704,37.5542736444521,20.));
#81881=CARTESIAN_POINT('Ctrl Pts',(-27.2922323089174,37.571138281747,0.));
#81882=CARTESIAN_POINT('Ctrl Pts',(-27.2922323089174,37.571138281747,20.));
#81883=CARTESIAN_POINT('Ctrl Pts',(-27.2639804710687,37.5879824209777,0.));
#81884=CARTESIAN_POINT('Ctrl Pts',(-27.2639804710687,37.5879824209777,20.));
#81885=CARTESIAN_POINT('Ctrl Pts',(-27.2357177167352,37.6048060545188,0.));
#81886=CARTESIAN_POINT('Ctrl Pts',(-27.2357177167352,37.6048060545188,20.));
#81887=CARTESIAN_POINT('Ctrl Pts',(-27.2074440604332,37.6216091747552,0.));
#81888=CARTESIAN_POINT('Ctrl Pts',(-27.2074440604332,37.6216091747552,20.));
#81889=CARTESIAN_POINT('Ctrl Pts',(-27.1791595166856,37.6383917740821,0.));
#81890=CARTESIAN_POINT('Ctrl Pts',(-27.1791595166856,37.6383917740821,20.));
#81891=CARTESIAN_POINT('Ctrl Pts',(-27.15086410002,37.6551538449046,0.));
#81892=CARTESIAN_POINT('Ctrl Pts',(-27.15086410002,37.6551538449046,20.));
#81893=CARTESIAN_POINT('Ctrl Pts',(-27.1225578249703,37.6718953796384,0.));
#81894=CARTESIAN_POINT('Ctrl Pts',(-27.1225578249703,37.6718953796384,20.));
#81895=CARTESIAN_POINT('Ctrl Pts',(-27.0942407060752,37.6886163707084,0.));
#81896=CARTESIAN_POINT('Ctrl Pts',(-27.0942407060752,37.6886163707084,20.));
#81897=CARTESIAN_POINT('Ctrl Pts',(-27.0659127578793,37.705316810549,0.));
#81898=CARTESIAN_POINT('Ctrl Pts',(-27.0659127578793,37.705316810549,20.));
#81899=CARTESIAN_POINT('Ctrl Pts',(-27.0375739949332,37.7219966916053,0.));
#81900=CARTESIAN_POINT('Ctrl Pts',(-27.0375739949332,37.7219966916053,20.));
#81901=CARTESIAN_POINT('Ctrl Pts',(-27.0092244317934,37.7386560063324,0.));
#81902=CARTESIAN_POINT('Ctrl Pts',(-27.0092244317934,37.7386560063324,20.));
#81903=CARTESIAN_POINT('Ctrl Pts',(-26.9808640830224,37.755294747196,0.));
#81904=CARTESIAN_POINT('Ctrl Pts',(-26.9808640830224,37.755294747196,20.));
#81905=CARTESIAN_POINT('Ctrl Pts',(-26.9524929631885,37.7719129066715,0.));
#81906=CARTESIAN_POINT('Ctrl Pts',(-26.9524929631885,37.7719129066715,20.));
#81907=CARTESIAN_POINT('Ctrl Pts',(-26.9241110868652,37.7885104772446,0.));
#81908=CARTESIAN_POINT('Ctrl Pts',(-26.9241110868652,37.7885104772446,20.));
#81909=CARTESIAN_POINT('Ctrl Pts',(-26.8957184686315,37.8050874514106,0.));
#81910=CARTESIAN_POINT('Ctrl Pts',(-26.8957184686315,37.8050874514106,20.));
#81911=CARTESIAN_POINT('Ctrl Pts',(-26.8673151230714,37.8216438216745,0.));
#81912=CARTESIAN_POINT('Ctrl Pts',(-26.8673151230714,37.8216438216745,20.));
#81913=CARTESIAN_POINT('Ctrl Pts',(-26.8389010647754,37.8381795805523,0.));
#81914=CARTESIAN_POINT('Ctrl Pts',(-26.8389010647754,37.8381795805523,20.));
#81915=CARTESIAN_POINT('Ctrl Pts',(-26.8104763083398,37.8546947205707,0.));
#81916=CARTESIAN_POINT('Ctrl Pts',(-26.8104763083398,37.8546947205707,20.));
#81917=CARTESIAN_POINT('Ctrl Pts',(-26.782040868367,37.8711892342661,0.));
#81918=CARTESIAN_POINT('Ctrl Pts',(-26.782040868367,37.8711892342661,20.));
#81919=CARTESIAN_POINT('Ctrl Pts',(-26.7535947594648,37.887663114185,0.));
#81920=CARTESIAN_POINT('Ctrl Pts',(-26.7535947594648,37.887663114185,20.));
#81921=CARTESIAN_POINT('Ctrl Pts',(-26.7251379962461,37.904116352883,0.));
#81922=CARTESIAN_POINT('Ctrl Pts',(-26.7251379962461,37.904116352883,20.));
#81923=CARTESIAN_POINT('Ctrl Pts',(-26.6966705933291,37.9205489429259,0.));
#81924=CARTESIAN_POINT('Ctrl Pts',(-26.6966705933291,37.9205489429259,20.));
#81925=CARTESIAN_POINT('Ctrl Pts',(-26.6681925653377,37.9369608768896,0.));
#81926=CARTESIAN_POINT('Ctrl Pts',(-26.6681925653377,37.9369608768896,20.));
#81927=CARTESIAN_POINT('Ctrl Pts',(-26.6397039269022,37.9533521473617,0.));
#81928=CARTESIAN_POINT('Ctrl Pts',(-26.6397039269022,37.9533521473617,20.));
#81929=CARTESIAN_POINT('Ctrl Pts',(-26.6112046926582,37.9697227469388,0.));
#81930=CARTESIAN_POINT('Ctrl Pts',(-26.6112046926582,37.9697227469388,20.));
#81931=CARTESIAN_POINT('Ctrl Pts',(-26.5826948772472,37.9860726682286,0.));
#81932=CARTESIAN_POINT('Ctrl Pts',(-26.5826948772472,37.9860726682286,20.));
#81933=CARTESIAN_POINT('Ctrl Pts',(-26.5541744953163,38.0024019038486,0.));
#81934=CARTESIAN_POINT('Ctrl Pts',(-26.5541744953163,38.0024019038486,20.));
#81935=CARTESIAN_POINT('Ctrl Pts',(-26.5256435615177,38.0187104464255,0.));
#81936=CARTESIAN_POINT('Ctrl Pts',(-26.5256435615177,38.0187104464255,20.));
#81937=CARTESIAN_POINT('Ctrl Pts',(-26.4971020905092,38.0349982885963,0.));
#81938=CARTESIAN_POINT('Ctrl Pts',(-26.4971020905092,38.0349982885963,20.));
#81939=CARTESIAN_POINT('Ctrl Pts',(-26.4685500969542,38.0512654230085,0.));
#81940=CARTESIAN_POINT('Ctrl Pts',(-26.4685500969542,38.0512654230085,20.));
#81941=CARTESIAN_POINT('Ctrl Pts',(-26.439987595522,38.0675118423201,0.));
#81942=CARTESIAN_POINT('Ctrl Pts',(-26.439987595522,38.0675118423201,20.));
#81943=CARTESIAN_POINT('Ctrl Pts',(-26.4114146008872,38.0837375391992,0.));
#81944=CARTESIAN_POINT('Ctrl Pts',(-26.4114146008872,38.0837375391992,20.));
#81945=CARTESIAN_POINT('Ctrl Pts',(-26.3828311277301,38.0999425063245,0.));
#81946=CARTESIAN_POINT('Ctrl Pts',(-26.3828311277301,38.0999425063245,20.));
#81947=CARTESIAN_POINT('Ctrl Pts',(-26.3542371907363,38.1161267363846,0.));
#81948=CARTESIAN_POINT('Ctrl Pts',(-26.3542371907363,38.1161267363846,20.));
#81949=CARTESIAN_POINT('Ctrl Pts',(-26.3256328045976,38.1322902220784,0.));
#81950=CARTESIAN_POINT('Ctrl Pts',(-26.3256328045976,38.1322902220784,20.));
#81951=CARTESIAN_POINT('Ctrl Pts',(-26.2970179840108,38.1484329561142,0.));
#81952=CARTESIAN_POINT('Ctrl Pts',(-26.2970179840108,38.1484329561142,20.));
#81953=CARTESIAN_POINT('Ctrl Pts',(-26.2683927436784,38.1645549312104,0.));
#81954=CARTESIAN_POINT('Ctrl Pts',(-26.2683927436784,38.1645549312104,20.));
#81955=CARTESIAN_POINT('Ctrl Pts',(-26.2397570983077,38.1806561400953,0.));
#81956=CARTESIAN_POINT('Ctrl Pts',(-26.2397570983077,38.1806561400953,20.));
#81957=CARTESIAN_POINT('Ctrl Pts',(-26.2111110626121,38.196736575508,0.));
#81958=CARTESIAN_POINT('Ctrl Pts',(-26.2111110626121,38.196736575508,20.));
#81959=CARTESIAN_POINT('Ctrl Pts',(-26.1824546513102,38.2127962301983,0.));
#81960=CARTESIAN_POINT('Ctrl Pts',(-26.1824546513102,38.2127962301983,20.));
#81961=CARTESIAN_POINT('Ctrl Pts',(-26.1537878791271,38.2288350969267,0.));
#81962=CARTESIAN_POINT('Ctrl Pts',(-26.1537878791271,38.2288350969267,20.));
#81963=CARTESIAN_POINT('Ctrl Pts',(-26.1251107607929,38.244853168464,0.));
#81964=CARTESIAN_POINT('Ctrl Pts',(-26.1251107607929,38.244853168464,20.));
#81965=CARTESIAN_POINT('Ctrl Pts',(-26.0964233110434,38.2608504375906,0.));
#81966=CARTESIAN_POINT('Ctrl Pts',(-26.0964233110434,38.2608504375906,20.));
#81967=CARTESIAN_POINT('Ctrl Pts',(-26.0677255446196,38.276826897097,0.));
#81968=CARTESIAN_POINT('Ctrl Pts',(-26.0677255446196,38.276826897097,20.));
#81969=CARTESIAN_POINT('Ctrl Pts',(-26.0390174762676,38.2927825397833,0.));
#81970=CARTESIAN_POINT('Ctrl Pts',(-26.0390174762676,38.2927825397833,20.));
#81971=CARTESIAN_POINT('Ctrl Pts',(-26.0102991207387,38.3087173584599,0.));
#81972=CARTESIAN_POINT('Ctrl Pts',(-26.0102991207387,38.3087173584599,20.));
#81973=CARTESIAN_POINT('Ctrl Pts',(-25.9815704927901,38.3246313459476,0.));
#81974=CARTESIAN_POINT('Ctrl Pts',(-25.9815704927901,38.3246313459476,20.));
#81975=CARTESIAN_POINT('Ctrl Pts',(-25.9528316071847,38.3405244950781,0.));
#81976=CARTESIAN_POINT('Ctrl Pts',(-25.9528316071847,38.3405244950781,20.));
#81977=CARTESIAN_POINT('Ctrl Pts',(-25.9240824786909,38.3563967986931,0.));
#81978=CARTESIAN_POINT('Ctrl Pts',(-25.9240824786909,38.3563967986931,20.));
#81979=CARTESIAN_POINT('Ctrl Pts',(-25.8953231220827,38.3722482496454,0.));
#81980=CARTESIAN_POINT('Ctrl Pts',(-25.8953231220827,38.3722482496454,20.));
#81981=CARTESIAN_POINT('Ctrl Pts',(-25.8665535521392,38.3880788407969,0.));
#81982=CARTESIAN_POINT('Ctrl Pts',(-25.8665535521392,38.3880788407969,20.));
#81983=CARTESIAN_POINT('Ctrl Pts',(-25.8377737836446,38.4038885650199,0.));
#81984=CARTESIAN_POINT('Ctrl Pts',(-25.8377737836446,38.4038885650199,20.));
#81985=CARTESIAN_POINT('Ctrl Pts',(-25.8089838313888,38.4196774151969,0.));
#81986=CARTESIAN_POINT('Ctrl Pts',(-25.8089838313888,38.4196774151969,20.));
#81987=CARTESIAN_POINT('Ctrl Pts',(-25.7801837101667,38.4354453842206,0.));
#81988=CARTESIAN_POINT('Ctrl Pts',(-25.7801837101667,38.4354453842206,20.));
#81989=CARTESIAN_POINT('Ctrl Pts',(-25.7513734347795,38.4511924649945,0.));
#81990=CARTESIAN_POINT('Ctrl Pts',(-25.7513734347795,38.4511924649945,20.));
#81991=CARTESIAN_POINT('Ctrl Pts',(-25.7225530200332,38.4669186504318,0.));
#81992=CARTESIAN_POINT('Ctrl Pts',(-25.7225530200332,38.4669186504318,20.));
#81993=CARTESIAN_POINT('Ctrl Pts',(-25.6937224807392,38.4826239334567,0.));
#81994=CARTESIAN_POINT('Ctrl Pts',(-25.6937224807392,38.4826239334567,20.));
#81995=CARTESIAN_POINT('Ctrl Pts',(-25.6648818317151,38.4983083070042,0.));
#81996=CARTESIAN_POINT('Ctrl Pts',(-25.6648818317151,38.4983083070042,20.));
#81997=CARTESIAN_POINT('Ctrl Pts',(-25.6360310877836,38.5139717640192,0.));
#81998=CARTESIAN_POINT('Ctrl Pts',(-25.6360310877836,38.5139717640192,20.));
#81999=CARTESIAN_POINT('Ctrl Pts',(-25.6071702637723,38.5296142974561,0.));
#82000=CARTESIAN_POINT('Ctrl Pts',(-25.6071702637723,38.5296142974561,20.));
#82001=CARTESIAN_POINT('Ctrl Pts',(-25.5782993745137,38.5452359002793,0.));
#82002=CARTESIAN_POINT('Ctrl Pts',(-25.5782993745137,38.5452359002793,20.));
#82003=CARTESIAN_POINT('Ctrl Pts',(-25.5494184348457,38.5608365654634,0.));
#82004=CARTESIAN_POINT('Ctrl Pts',(-25.5494184348457,38.5608365654634,20.));
#82005=CARTESIAN_POINT('Ctrl Pts',(-25.5205274596115,38.5764162859939,0.));
#82006=CARTESIAN_POINT('Ctrl Pts',(-25.5205274596115,38.5764162859939,20.));
#82007=CARTESIAN_POINT('Ctrl Pts',(-25.4916264636604,38.591975054867,0.));
#82008=CARTESIAN_POINT('Ctrl Pts',(-25.4916264636604,38.591975054867,20.));
#82009=CARTESIAN_POINT('Ctrl Pts',(-25.462715461847,38.6075128650891,0.));
#82010=CARTESIAN_POINT('Ctrl Pts',(-25.462715461847,38.6075128650891,20.));
#82011=CARTESIAN_POINT('Ctrl Pts',(-25.4337944690316,38.6230297096774,0.));
#82012=CARTESIAN_POINT('Ctrl Pts',(-25.4337944690316,38.6230297096774,20.));
#82013=CARTESIAN_POINT('Ctrl Pts',(-25.4048635000795,38.6385255816593,0.));
#82014=CARTESIAN_POINT('Ctrl Pts',(-25.4048635000795,38.6385255816593,20.));
#82015=CARTESIAN_POINT('Ctrl Pts',(-25.3759225698613,38.6540004740723,0.));
#82016=CARTESIAN_POINT('Ctrl Pts',(-25.3759225698613,38.6540004740723,20.));
#82017=CARTESIAN_POINT('Ctrl Pts',(-25.3469716932528,38.6694543799641,0.));
#82018=CARTESIAN_POINT('Ctrl Pts',(-25.3469716932528,38.6694543799641,20.));
#82019=CARTESIAN_POINT('Ctrl Pts',(-25.3180108851341,38.6848872923919,0.));
#82020=CARTESIAN_POINT('Ctrl Pts',(-25.3180108851341,38.6848872923919,20.));
#82021=CARTESIAN_POINT('Ctrl Pts',(-25.2890401603913,38.7002992044241,0.));
#82022=CARTESIAN_POINT('Ctrl Pts',(-25.2890401603913,38.7002992044241,20.));
#82023=CARTESIAN_POINT('Ctrl Pts',(-25.2600595339159,38.7156901091392,0.));
#82024=CARTESIAN_POINT('Ctrl Pts',(-25.2600595339159,38.7156901091392,20.));
#82025=CARTESIAN_POINT('Ctrl Pts',(-25.231069020605,38.7310599996258,0.));
#82026=CARTESIAN_POINT('Ctrl Pts',(-25.231069020605,38.7310599996258,20.));
#82027=CARTESIAN_POINT('Ctrl Pts',(-25.2020686353608,38.7464088689836,0.));
#82028=CARTESIAN_POINT('Ctrl Pts',(-25.2020686353608,38.7464088689836,20.));
#82029=CARTESIAN_POINT('Ctrl Pts',(-25.1730583930911,38.7617367103228,0.));
#82030=CARTESIAN_POINT('Ctrl Pts',(-25.1730583930911,38.7617367103228,20.));
#82031=CARTESIAN_POINT('Ctrl Pts',(-25.1440383087085,38.7770435167639,0.));
#82032=CARTESIAN_POINT('Ctrl Pts',(-25.1440383087085,38.7770435167639,20.));
#82033=CARTESIAN_POINT('Ctrl Pts',(-25.1150083971302,38.7923292814368,0.));
#82034=CARTESIAN_POINT('Ctrl Pts',(-25.1150083971302,38.7923292814368,20.));
#82035=CARTESIAN_POINT('Ctrl Pts',(-25.0859686732795,38.8075939974829,0.));
#82036=CARTESIAN_POINT('Ctrl Pts',(-25.0859686732795,38.8075939974829,20.));
#82037=CARTESIAN_POINT('Ctrl Pts',(-25.0569191520845,38.8228376580533,0.));
#82038=CARTESIAN_POINT('Ctrl Pts',(-25.0569191520845,38.8228376580533,20.));
#82039=CARTESIAN_POINT('Ctrl Pts',(-25.0278598484791,38.8380602563098,0.));
#82040=CARTESIAN_POINT('Ctrl Pts',(-25.0278598484791,38.8380602563098,20.));
#82041=CARTESIAN_POINT('Ctrl Pts',(-24.9987907774025,38.8532617854245,0.));
#82042=CARTESIAN_POINT('Ctrl Pts',(-24.9987907774025,38.8532617854245,20.));
#82043=CARTESIAN_POINT('Ctrl Pts',(-24.9697119537989,38.8684422385799,0.));
#82044=CARTESIAN_POINT('Ctrl Pts',(-24.9697119537989,38.8684422385799,20.));
#82045=CARTESIAN_POINT('Ctrl Pts',(-24.9406233926168,38.883601608968,0.));
#82046=CARTESIAN_POINT('Ctrl Pts',(-24.9406233926168,38.883601608968,20.));
#82047=CARTESIAN_POINT('Ctrl Pts',(-24.9115251088108,38.8987398897918,0.));
#82048=CARTESIAN_POINT('Ctrl Pts',(-24.9115251088108,38.8987398897918,20.));
#82049=CARTESIAN_POINT('Ctrl Pts',(-24.8824171173402,38.9138570742648,0.));
#82050=CARTESIAN_POINT('Ctrl Pts',(-24.8824171173402,38.9138570742648,20.));
#82051=CARTESIAN_POINT('Ctrl Pts',(-24.8532994331703,38.9289531556117,0.));
#82052=CARTESIAN_POINT('Ctrl Pts',(-24.8532994331703,38.9289531556117,20.));
#82053=CARTESIAN_POINT('Ctrl Pts',(-24.8241720712716,38.9440281270684,0.));
#82054=CARTESIAN_POINT('Ctrl Pts',(-24.8241720712716,38.9440281270684,20.));
#82055=CARTESIAN_POINT('Ctrl Pts',(-24.7950350466188,38.9590819818797,0.));
#82056=CARTESIAN_POINT('Ctrl Pts',(-24.7950350466188,38.9590819818797,20.));
#82057=CARTESIAN_POINT('Ctrl Pts',(-24.7658883741919,38.9741147133012,0.));
#82058=CARTESIAN_POINT('Ctrl Pts',(-24.7658883741919,38.9741147133012,20.));
#82059=CARTESIAN_POINT('Ctrl Pts',(-24.736732068976,38.989126314598,0.));
#82060=CARTESIAN_POINT('Ctrl Pts',(-24.736732068976,38.989126314598,20.));
#82061=CARTESIAN_POINT('Ctrl Pts',(-24.7075661459617,39.0041167790461,0.));
#82062=CARTESIAN_POINT('Ctrl Pts',(-24.7075661459617,39.0041167790461,20.));
#82063=CARTESIAN_POINT('Ctrl Pts',(-24.6783906201452,39.019086099931,0.));
#82064=CARTESIAN_POINT('Ctrl Pts',(-24.6783906201452,39.019086099931,20.));
#82065=CARTESIAN_POINT('Ctrl Pts',(-24.6492055065285,39.0340342705498,0.));
#82066=CARTESIAN_POINT('Ctrl Pts',(-24.6492055065285,39.0340342705498,20.));
#82067=CARTESIAN_POINT('Ctrl Pts',(-24.6200108201182,39.0489612842095,0.));
#82068=CARTESIAN_POINT('Ctrl Pts',(-24.6200108201182,39.0489612842095,20.));
#82069=CARTESIAN_POINT('Ctrl Pts',(-24.5908065759258,39.0638671342286,0.));
#82070=CARTESIAN_POINT('Ctrl Pts',(-24.5908065759258,39.0638671342286,20.));
#82071=CARTESIAN_POINT('Ctrl Pts',(-24.5615927889669,39.0787518139362,0.));
#82072=CARTESIAN_POINT('Ctrl Pts',(-24.5615927889669,39.0787518139362,20.));
#82073=CARTESIAN_POINT('Ctrl Pts',(-24.5323694742617,39.0936153166722,0.));
#82074=CARTESIAN_POINT('Ctrl Pts',(-24.5323694742617,39.0936153166722,20.));
#82075=CARTESIAN_POINT('Ctrl Pts',(-24.5031366468345,39.1084576357871,0.));
#82076=CARTESIAN_POINT('Ctrl Pts',(-24.5031366468345,39.1084576357871,20.));
#82077=CARTESIAN_POINT('Ctrl Pts',(-24.4738943217155,39.1232787646414,0.));
#82078=CARTESIAN_POINT('Ctrl Pts',(-24.4738943217155,39.1232787646414,20.));
#82079=CARTESIAN_POINT('Ctrl Pts',(-24.4446425139409,39.1380786966047,0.));
#82080=CARTESIAN_POINT('Ctrl Pts',(-24.4446425139409,39.1380786966047,20.));
#82081=CARTESIAN_POINT('Ctrl Pts',(-24.4153812385543,39.1528574250568,0.));
#82082=CARTESIAN_POINT('Ctrl Pts',(-24.4153812385543,39.1528574250568,20.));
#82083=CARTESIAN_POINT('Ctrl Pts',(-24.3861105106067,39.1676149433869,0.));
#82084=CARTESIAN_POINT('Ctrl Pts',(-24.3861105106067,39.1676149433869,20.));
#82085=CARTESIAN_POINT('Ctrl Pts',(-24.3568303451549,39.1823512449951,0.));
#82086=CARTESIAN_POINT('Ctrl Pts',(-24.3568303451549,39.1823512449951,20.));
#82087=CARTESIAN_POINT('Ctrl Pts',(-24.3275407572588,39.197066323292,0.));
#82088=CARTESIAN_POINT('Ctrl Pts',(-24.3275407572588,39.197066323292,20.));
#82089=CARTESIAN_POINT('Ctrl Pts',(-24.2982417619806,39.2117601717005,0.));
#82090=CARTESIAN_POINT('Ctrl Pts',(-24.2982417619806,39.2117601717005,20.));
#82091=CARTESIAN_POINT('Ctrl Pts',(-24.2689333743823,39.2264327836562,0.));
#82092=CARTESIAN_POINT('Ctrl Pts',(-24.2689333743823,39.2264327836562,20.));
#82093=CARTESIAN_POINT('Ctrl Pts',(-24.2396156095261,39.2410841526077,0.));
#82094=CARTESIAN_POINT('Ctrl Pts',(-24.2396156095261,39.2410841526077,20.));
#82095=CARTESIAN_POINT('Ctrl Pts',(-24.2102884824784,39.2557142720138,0.));
#82096=CARTESIAN_POINT('Ctrl Pts',(-24.2102884824784,39.2557142720138,20.));
#82097=CARTESIAN_POINT('Ctrl Pts',(-24.1809520083147,39.2703231353422,0.));
#82098=CARTESIAN_POINT('Ctrl Pts',(-24.1809520083147,39.2703231353422,20.));
#82099=CARTESIAN_POINT('Ctrl Pts',(-24.1516062021224,39.2849107360681,0.));
#82100=CARTESIAN_POINT('Ctrl Pts',(-24.1516062021224,39.2849107360681,20.));
#82101=CARTESIAN_POINT('Ctrl Pts',(-24.1222510790066,39.2994770676712,0.));
#82102=CARTESIAN_POINT('Ctrl Pts',(-24.1222510790066,39.2994770676712,20.));
#82103=CARTESIAN_POINT('Ctrl Pts',(-24.0928866540882,39.3140221236369,0.));
#82104=CARTESIAN_POINT('Ctrl Pts',(-24.0928866540882,39.3140221236369,20.));
#82105=CARTESIAN_POINT('Ctrl Pts',(-24.0635129424931,39.3285458974612,0.));
#82106=CARTESIAN_POINT('Ctrl Pts',(-24.0635129424931,39.3285458974612,20.));
#82107=CARTESIAN_POINT('Ctrl Pts',(-24.0341299593437,39.3430483826555,0.));
#82108=CARTESIAN_POINT('Ctrl Pts',(-24.0341299593437,39.3430483826555,20.));
#82109=CARTESIAN_POINT('Ctrl Pts',(-24.0047377197503,39.3575295727493,0.));
#82110=CARTESIAN_POINT('Ctrl Pts',(-24.0047377197503,39.3575295727493,20.));
#82111=CARTESIAN_POINT('Ctrl Pts',(-23.9753362387978,39.3719894612957,0.));
#82112=CARTESIAN_POINT('Ctrl Pts',(-23.9753362387978,39.3719894612957,20.));
#82113=CARTESIAN_POINT('Ctrl Pts',(-23.9459255315518,39.3864280418676,0.));
#82114=CARTESIAN_POINT('Ctrl Pts',(-23.9459255315518,39.3864280418676,20.));
#82115=CARTESIAN_POINT('Ctrl Pts',(-23.9165056130837,39.4008453080481,0.));
#82116=CARTESIAN_POINT('Ctrl Pts',(-23.9165056130837,39.4008453080481,20.));
#82117=CARTESIAN_POINT('Ctrl Pts',(-23.8870764984925,39.4152412534209,0.));
#82118=CARTESIAN_POINT('Ctrl Pts',(-23.8870764984925,39.4152412534209,20.));
#82119=CARTESIAN_POINT('Ctrl Pts',(-23.8576382029238,39.4296158715627,0.));
#82120=CARTESIAN_POINT('Ctrl Pts',(-23.8576382029238,39.4296158715627,20.));
#82121=CARTESIAN_POINT('Ctrl Pts',(-23.8281907416005,39.4439691560298,0.));
#82122=CARTESIAN_POINT('Ctrl Pts',(-23.8281907416005,39.4439691560298,20.));
#82123=CARTESIAN_POINT('Ctrl Pts',(-23.7987341298022,39.4583011003674,0.));
#82124=CARTESIAN_POINT('Ctrl Pts',(-23.7987341298022,39.4583011003674,20.));
#82125=CARTESIAN_POINT('Ctrl Pts',(-23.7692683828081,39.4726116981337,0.));
#82126=CARTESIAN_POINT('Ctrl Pts',(-23.7692683828081,39.4726116981337,20.));
#82127=CARTESIAN_POINT('Ctrl Pts',(-23.7397935158457,39.4869009429217,0.));
#82128=CARTESIAN_POINT('Ctrl Pts',(-23.7397935158457,39.4869009429217,20.));
#82129=CARTESIAN_POINT('Ctrl Pts',(-23.7103095440476,39.5011688283778,0.));
#82130=CARTESIAN_POINT('Ctrl Pts',(-23.7103095440476,39.5011688283778,20.));
#82131=CARTESIAN_POINT('Ctrl Pts',(-23.6808164823786,39.5154153482324,0.));
#82132=CARTESIAN_POINT('Ctrl Pts',(-23.6808164823786,39.5154153482324,20.));
#82133=CARTESIAN_POINT('Ctrl Pts',(-23.651314345698,39.5296404962721,0.));
#82134=CARTESIAN_POINT('Ctrl Pts',(-23.651314345698,39.5296404962721,20.));
#82135=CARTESIAN_POINT('Ctrl Pts',(-23.6218031488905,39.5438442662853,0.));
#82136=CARTESIAN_POINT('Ctrl Pts',(-23.6218031488905,39.5438442662853,20.));
#82137=CARTESIAN_POINT('Ctrl Pts',(-23.5922829069852,39.5580266520107,0.));
#82138=CARTESIAN_POINT('Ctrl Pts',(-23.5922829069852,39.5580266520107,20.));
#82139=CARTESIAN_POINT('Ctrl Pts',(-23.5627536352592,39.5721876470956,0.));
#82140=CARTESIAN_POINT('Ctrl Pts',(-23.5627536352592,39.5721876470956,20.));
#82141=CARTESIAN_POINT('Ctrl Pts',(-23.533215349402,39.5863272450267,0.));
#82142=CARTESIAN_POINT('Ctrl Pts',(-23.533215349402,39.5863272450267,20.));
#82143=CARTESIAN_POINT('Ctrl Pts',(-23.5036680653391,39.6004454392038,0.));
#82144=CARTESIAN_POINT('Ctrl Pts',(-23.5036680653391,39.6004454392038,20.));
#82145=CARTESIAN_POINT('Ctrl Pts',(-23.4741117989348,39.6145422230651,0.));
#82146=CARTESIAN_POINT('Ctrl Pts',(-23.4741117989348,39.6145422230651,20.));
#82147=CARTESIAN_POINT('Ctrl Pts',(-23.4445465657147,39.6286175902046,0.));
#82148=CARTESIAN_POINT('Ctrl Pts',(-23.4445465657147,39.6286175902046,20.));
#82149=CARTESIAN_POINT('Ctrl Pts',(-23.4149723806221,39.6426715344742,0.));
#82150=CARTESIAN_POINT('Ctrl Pts',(-23.4149723806221,39.6426715344742,20.));
#82151=CARTESIAN_POINT('Ctrl Pts',(-23.385389257652,39.6567040501382,0.));
#82152=CARTESIAN_POINT('Ctrl Pts',(-23.385389257652,39.6567040501382,20.));
#82153=CARTESIAN_POINT('Ctrl Pts',(-23.3557972103217,39.670715131677,0.));
#82154=CARTESIAN_POINT('Ctrl Pts',(-23.3557972103217,39.670715131677,20.));
#82155=CARTESIAN_POINT('Ctrl Pts',(-23.3261962523444,39.6847047735001,0.));
#82156=CARTESIAN_POINT('Ctrl Pts',(-23.3261962523444,39.6847047735001,20.));
#82157=CARTESIAN_POINT('Ctrl Pts',(-23.2965863982648,39.6986729696788,0.));
#82158=CARTESIAN_POINT('Ctrl Pts',(-23.2965863982648,39.6986729696788,20.));
#82159=CARTESIAN_POINT('Ctrl Pts',(-23.2669676640418,39.712619713699,0.));
#82160=CARTESIAN_POINT('Ctrl Pts',(-23.2669676640418,39.712619713699,20.));
#82161=CARTESIAN_POINT('Ctrl Pts',(-23.2373400678346,39.7265449981305,0.));
#82162=CARTESIAN_POINT('Ctrl Pts',(-23.2373400678346,39.7265449981305,20.));
#82163=CARTESIAN_POINT('Ctrl Pts',(-23.2077036288598,39.7404488151086,0.));
#82164=CARTESIAN_POINT('Ctrl Pts',(-23.2077036288598,39.7404488151086,20.));
#82165=CARTESIAN_POINT('Ctrl Pts',(-23.1780583659508,39.7543311569459,0.));
#82166=CARTESIAN_POINT('Ctrl Pts',(-23.1780583659508,39.7543311569459,20.));
#82167=CARTESIAN_POINT('Ctrl Pts',(-23.1484042962029,39.7681920167058,0.));
#82168=CARTESIAN_POINT('Ctrl Pts',(-23.1484042962029,39.7681920167058,20.));
#82169=CARTESIAN_POINT('Ctrl Pts',(-23.1187414336251,39.7820313887737,0.));
#82170=CARTESIAN_POINT('Ctrl Pts',(-23.1187414336251,39.7820313887737,20.));
#82171=CARTESIAN_POINT('Ctrl Pts',(-23.089069787673,39.7958492694787,0.));
#82172=CARTESIAN_POINT('Ctrl Pts',(-23.089069787673,39.7958492694787,20.));
#82173=CARTESIAN_POINT('Ctrl Pts',(-23.0593893640427,39.8096456567259,0.));
#82174=CARTESIAN_POINT('Ctrl Pts',(-23.0593893640427,39.8096456567259,20.));
#82175=CARTESIAN_POINT('Ctrl Pts',(-23.0356380053139,39.8206655709903,0.));
#82176=CARTESIAN_POINT('Ctrl Pts',(-23.0356380053139,39.8206655709903,20.));
#82177=CARTESIAN_POINT('Ctrl Pts',(-23.0178205380655,39.8289208340947,0.));
#82178=CARTESIAN_POINT('Ctrl Pts',(-23.0178205380655,39.8289208340947,20.));
#82179=CARTESIAN_POINT('Ctrl Pts',(-23.005940471814,39.8344200439082,0.));
#82180=CARTESIAN_POINT('Ctrl Pts',(-23.005940471814,39.8344200439082,20.));
#82181=CARTESIAN_POINT('Ctrl Pts',(-23.,39.8371685740842,0.));
#82182=CARTESIAN_POINT('Ctrl Pts',(-23.,39.8371685740842,20.));
#82183=CARTESIAN_POINT('',(-46.0449384185095,16.7589870229578,2.));
#82184=CARTESIAN_POINT('Ctrl Pts',(-34.5017338047269,32.2758373034787,2.));
#82185=CARTESIAN_POINT('Ctrl Pts',(-35.1012599438994,31.7409631286146,2.));
#82186=CARTESIAN_POINT('Ctrl Pts',(-35.6879267845883,31.1902015741133,2.));
#82187=CARTESIAN_POINT('Ctrl Pts',(-36.260940923753,30.624221206043,2.));
#82188=CARTESIAN_POINT('Ctrl Pts',(-36.8331139940994,30.0590715826381,2.));
#82189=CARTESIAN_POINT('Ctrl Pts',(-37.3916743025935,29.4787479308737,2.));
#82190=CARTESIAN_POINT('Ctrl Pts',(-37.9358680909622,28.8839537384041,2.));
#82191=CARTESIAN_POINT('Ctrl Pts',(-38.4805318739963,28.288645850072,2.));
#82192=CARTESIAN_POINT('Ctrl Pts',(-39.0108041943122,27.6788425476408,2.));
#82193=CARTESIAN_POINT('Ctrl Pts',(-39.5259673010255,27.0552850618763,2.));
#82194=CARTESIAN_POINT('Ctrl Pts',(-40.0415776804199,26.4311861937323,2.));
#82195=CARTESIAN_POINT('Ctrl Pts',(-40.5420524892488,25.7933093866071,2.));
#82196=CARTESIAN_POINT('Ctrl Pts',(-41.0267118135419,25.1424317389406,2.));
#82197=CARTESIAN_POINT('Ctrl Pts',(-41.5120542721152,24.4906366698793,2.));
#82198=CARTESIAN_POINT('Ctrl Pts',(-41.9815365243414,23.8258042250936,2.));
#82199=CARTESIAN_POINT('Ctrl Pts',(-42.4345172043854,23.1487467236845,2.));
#82200=CARTESIAN_POINT('Ctrl Pts',(-42.8878253137778,22.4711998228236,2.));
#82201=CARTESIAN_POINT('Ctrl Pts',(-43.3246078927956,21.7814103343397,2.));
#82202=CARTESIAN_POINT('Ctrl Pts',(-43.7442651357813,21.0802221166732,2.));
#82203=CARTESIAN_POINT('Ctrl Pts',(-44.1624466566267,20.3814996231056,2.));
#82204=CARTESIAN_POINT('Ctrl Pts',(-44.5636230181975,19.6714585963912,2.));
#82205=CARTESIAN_POINT('Ctrl Pts',(-44.9472444130411,18.9509611646836,2.));
#82206=CARTESIAN_POINT('Ctrl Pts',(-45.1999149529739,18.4764087087029,2.));
#82207=CARTESIAN_POINT('Ctrl Pts',(-45.4449708032456,17.9973206591027,2.));
#82208=CARTESIAN_POINT('Ctrl Pts',(-45.6822654287125,17.5139493060988,2.));
#82209=CARTESIAN_POINT('Ctrl Pts',(-45.8052474513848,17.2634337852467,2.));
#82210=CARTESIAN_POINT('Ctrl Pts',(-45.926144661035,17.0117683454893,2.));
#82211=CARTESIAN_POINT('Ctrl Pts',(-46.0449384185095,16.7589870229578,2.));
#82212=CARTESIAN_POINT('',(-46.0449384185095,16.7589870229578,0.));
#82213=CARTESIAN_POINT('Ctrl Pts',(-46.0449384185095,16.7589870229578,0.));
#82214=CARTESIAN_POINT('Ctrl Pts',(-46.0449384185095,16.7589870229578,20.));
#82215=CARTESIAN_POINT('Ctrl Pts',(-46.0420594924752,16.7651130917503,0.));
#82216=CARTESIAN_POINT('Ctrl Pts',(-46.0420594924752,16.7651130917503,20.));
#82217=CARTESIAN_POINT('Ctrl Pts',(-46.0362995834799,16.7773641333857,0.));
#82218=CARTESIAN_POINT('Ctrl Pts',(-46.0362995834799,16.7773641333857,20.));
#82219=CARTESIAN_POINT('Ctrl Pts',(-46.0276535492065,16.7957374079899,0.));
#82220=CARTESIAN_POINT('Ctrl Pts',(-46.0276535492065,16.7957374079899,20.));
#82221=CARTESIAN_POINT('Ctrl Pts',(-46.0161131619282,16.8202285317553,0.));
#82222=CARTESIAN_POINT('Ctrl Pts',(-46.0161131619282,16.8202285317553,20.));
#82223=CARTESIAN_POINT('Ctrl Pts',(-46.0016671088634,16.8508314760754,0.));
#82224=CARTESIAN_POINT('Ctrl Pts',(-46.0016671088634,16.8508314760754,20.));
#82225=CARTESIAN_POINT('Ctrl Pts',(-45.9872004880192,16.8814234574888,0.));
#82226=CARTESIAN_POINT('Ctrl Pts',(-45.9872004880192,16.8814234574888,20.));
#82227=CARTESIAN_POINT('Ctrl Pts',(-45.9727133019197,16.9120044710149,0.));
#82228=CARTESIAN_POINT('Ctrl Pts',(-45.9727133019197,16.9120044710149,20.));
#82229=CARTESIAN_POINT('Ctrl Pts',(-45.9582055548827,16.9425745084438,0.));
#82230=CARTESIAN_POINT('Ctrl Pts',(-45.9582055548827,16.9425745084438,20.));
#82231=CARTESIAN_POINT('Ctrl Pts',(-45.9436772535459,16.9731335574459,0.));
#82232=CARTESIAN_POINT('Ctrl Pts',(-45.9436772535459,16.9731335574459,20.));
#82233=CARTESIAN_POINT('Ctrl Pts',(-45.9291284062576,17.0036816026634,0.));
#82234=CARTESIAN_POINT('Ctrl Pts',(-45.9291284062576,17.0036816026634,20.));
#82235=CARTESIAN_POINT('Ctrl Pts',(-45.91455902239,17.0342186269341,0.));
#82236=CARTESIAN_POINT('Ctrl Pts',(-45.91455902239,17.0342186269341,20.));
#82237=CARTESIAN_POINT('Ctrl Pts',(-45.8999691116667,17.0647446124944,0.));
#82238=CARTESIAN_POINT('Ctrl Pts',(-45.8999691116667,17.0647446124944,20.));
#82239=CARTESIAN_POINT('Ctrl Pts',(-45.8853586835176,17.0952595421299,0.));
#82240=CARTESIAN_POINT('Ctrl Pts',(-45.8853586835176,17.0952595421299,20.));
#82241=CARTESIAN_POINT('Ctrl Pts',(-45.8707277463338,17.1257634005083,0.));
#82242=CARTESIAN_POINT('Ctrl Pts',(-45.8707277463338,17.1257634005083,20.));
#82243=CARTESIAN_POINT('Ctrl Pts',(-45.8560763076625,17.1562561738292,0.));
#82244=CARTESIAN_POINT('Ctrl Pts',(-45.8560763076625,17.1562561738292,20.));
#82245=CARTESIAN_POINT('Ctrl Pts',(-45.8414043745501,17.1867378492105,0.));
#82246=CARTESIAN_POINT('Ctrl Pts',(-45.8414043745501,17.1867378492105,20.));
#82247=CARTESIAN_POINT('Ctrl Pts',(-45.8267119538424,17.2172084141516,0.));
#82248=CARTESIAN_POINT('Ctrl Pts',(-45.8267119538424,17.2172084141516,20.));
#82249=CARTESIAN_POINT('Ctrl Pts',(-45.8119990524824,17.247667856,0.));
#82250=CARTESIAN_POINT('Ctrl Pts',(-45.8119990524824,17.247667856,20.));
#82251=CARTESIAN_POINT('Ctrl Pts',(-45.7972656778619,17.2781161613228,0.));
#82252=CARTESIAN_POINT('Ctrl Pts',(-45.7972656778619,17.2781161613228,20.));
#82253=CARTESIAN_POINT('Ctrl Pts',(-45.7825118377706,17.3085533159981,0.));
#82254=CARTESIAN_POINT('Ctrl Pts',(-45.7825118377706,17.3085533159981,20.));
#82255=CARTESIAN_POINT('Ctrl Pts',(-45.7677375402376,17.3389793054984,0.));
#82256=CARTESIAN_POINT('Ctrl Pts',(-45.7677375402376,17.3389793054984,20.));
#82257=CARTESIAN_POINT('Ctrl Pts',(-45.7529427934047,17.3693941151172,0.));
#82258=CARTESIAN_POINT('Ctrl Pts',(-45.7529427934047,17.3693941151172,20.));
#82259=CARTESIAN_POINT('Ctrl Pts',(-45.7381276053972,17.3997977302007,0.));
#82260=CARTESIAN_POINT('Ctrl Pts',(-45.7381276053972,17.3997977302007,20.));
#82261=CARTESIAN_POINT('Ctrl Pts',(-45.7232919841685,17.4301901364248,0.));
#82262=CARTESIAN_POINT('Ctrl Pts',(-45.7232919841685,17.4301901364248,20.));
#82263=CARTESIAN_POINT('Ctrl Pts',(-45.7084359375081,17.460571319782,0.));
#82264=CARTESIAN_POINT('Ctrl Pts',(-45.7084359375081,17.460571319782,20.));
#82265=CARTESIAN_POINT('Ctrl Pts',(-45.6935594731126,17.4909412664519,0.));
#82266=CARTESIAN_POINT('Ctrl Pts',(-45.6935594731126,17.4909412664519,20.));
#82267=CARTESIAN_POINT('Ctrl Pts',(-45.6786625986401,17.5212999627071,0.));
#82268=CARTESIAN_POINT('Ctrl Pts',(-45.6786625986401,17.5212999627071,20.));
#82269=CARTESIAN_POINT('Ctrl Pts',(-45.6637453217655,17.5516473948116,0.));
#82270=CARTESIAN_POINT('Ctrl Pts',(-45.6637453217655,17.5516473948116,20.));
#82271=CARTESIAN_POINT('Ctrl Pts',(-45.6488076502485,17.5819835489016,0.));
#82272=CARTESIAN_POINT('Ctrl Pts',(-45.6488076502485,17.5819835489016,20.));
#82273=CARTESIAN_POINT('Ctrl Pts',(-45.6338495919363,17.6123084109793,0.));
#82274=CARTESIAN_POINT('Ctrl Pts',(-45.6338495919363,17.6123084109793,20.));
#82275=CARTESIAN_POINT('Ctrl Pts',(-45.6188711547313,17.6426219669711,0.));
#82276=CARTESIAN_POINT('Ctrl Pts',(-45.6188711547313,17.6426219669711,20.));
#82277=CARTESIAN_POINT('Ctrl Pts',(-45.6038723465685,17.672924202767,0.));
#82278=CARTESIAN_POINT('Ctrl Pts',(-45.6038723465685,17.672924202767,20.));
#82279=CARTESIAN_POINT('Ctrl Pts',(-45.5888531753912,17.7032151042645,0.));
#82280=CARTESIAN_POINT('Ctrl Pts',(-45.5888531753912,17.7032151042645,20.));
#82281=CARTESIAN_POINT('Ctrl Pts',(-45.5738136491221,17.7334946574206,0.));
#82282=CARTESIAN_POINT('Ctrl Pts',(-45.5738136491221,17.7334946574206,20.));
#82283=CARTESIAN_POINT('Ctrl Pts',(-45.5587537756595,17.7637628482589,0.));
#82284=CARTESIAN_POINT('Ctrl Pts',(-45.5587537756595,17.7637628482589,20.));
#82285=CARTESIAN_POINT('Ctrl Pts',(-45.5436735628911,17.7940196628442,0.));
#82286=CARTESIAN_POINT('Ctrl Pts',(-45.5436735628911,17.7940196628442,20.));
#82287=CARTESIAN_POINT('Ctrl Pts',(-45.528573018704,17.8242650872661,0.));
#82288=CARTESIAN_POINT('Ctrl Pts',(-45.528573018704,17.8242650872661,20.));
#82289=CARTESIAN_POINT('Ctrl Pts',(-45.5134521509949,17.8544991076191,0.));
#82290=CARTESIAN_POINT('Ctrl Pts',(-45.5134521509949,17.8544991076191,20.));
#82291=CARTESIAN_POINT('Ctrl Pts',(-45.498310967683,17.8847217099814,0.));
#82292=CARTESIAN_POINT('Ctrl Pts',(-45.498310967683,17.8847217099814,20.));
#82293=CARTESIAN_POINT('Ctrl Pts',(-45.4831494767122,17.9149328804084,0.));
#82294=CARTESIAN_POINT('Ctrl Pts',(-45.4831494767122,17.9149328804084,20.));
#82295=CARTESIAN_POINT('Ctrl Pts',(-45.4679676860453,17.9451326049449,0.));
#82296=CARTESIAN_POINT('Ctrl Pts',(-45.4679676860453,17.9451326049449,20.));
#82297=CARTESIAN_POINT('Ctrl Pts',(-45.4527656036598,17.9753208696315,0.));
#82298=CARTESIAN_POINT('Ctrl Pts',(-45.4527656036598,17.9753208696315,20.));
#82299=CARTESIAN_POINT('Ctrl Pts',(-45.4375432375433,18.0054976605137,0.));
#82300=CARTESIAN_POINT('Ctrl Pts',(-45.4375432375433,18.0054976605137,20.));
#82301=CARTESIAN_POINT('Ctrl Pts',(-45.4223005956881,18.0356629636502,0.));
#82302=CARTESIAN_POINT('Ctrl Pts',(-45.4223005956881,18.0356629636502,20.));
#82303=CARTESIAN_POINT('Ctrl Pts',(-45.4070376860893,18.0658167651176,0.));
#82304=CARTESIAN_POINT('Ctrl Pts',(-45.4070376860893,18.0658167651176,20.));
#82305=CARTESIAN_POINT('Ctrl Pts',(-45.3917545167484,18.0959590510046,0.));
#82306=CARTESIAN_POINT('Ctrl Pts',(-45.3917545167484,18.0959590510046,20.));
#82307=CARTESIAN_POINT('Ctrl Pts',(-45.3764510956741,18.1260898074095,0.));
#82308=CARTESIAN_POINT('Ctrl Pts',(-45.3764510956741,18.1260898074095,20.));
#82309=CARTESIAN_POINT('Ctrl Pts',(-45.3611274308852,18.156209020436,0.));
#82310=CARTESIAN_POINT('Ctrl Pts',(-45.3611274308852,18.156209020436,20.));
#82311=CARTESIAN_POINT('Ctrl Pts',(-45.345783530412,18.1863166761897,0.));
#82312=CARTESIAN_POINT('Ctrl Pts',(-45.345783530412,18.1863166761897,20.));
#82313=CARTESIAN_POINT('Ctrl Pts',(-45.3304194022976,18.216412760776,0.));
#82314=CARTESIAN_POINT('Ctrl Pts',(-45.3304194022976,18.216412760776,20.));
#82315=CARTESIAN_POINT('Ctrl Pts',(-45.3150350545965,18.2464972603023,0.));
#82316=CARTESIAN_POINT('Ctrl Pts',(-45.3150350545965,18.2464972603023,20.));
#82317=CARTESIAN_POINT('Ctrl Pts',(-45.299630495374,18.2765701608789,0.));
#82318=CARTESIAN_POINT('Ctrl Pts',(-45.299630495374,18.2765701608789,20.));
#82319=CARTESIAN_POINT('Ctrl Pts',(-45.2842057327049,18.3066314486214,0.));
#82320=CARTESIAN_POINT('Ctrl Pts',(-45.2842057327049,18.3066314486214,20.));
#82321=CARTESIAN_POINT('Ctrl Pts',(-45.2687607746732,18.3366811096519,0.));
#82322=CARTESIAN_POINT('Ctrl Pts',(-45.2687607746732,18.3366811096519,20.));
#82323=CARTESIAN_POINT('Ctrl Pts',(-45.2532956293718,18.3667191300999,0.));
#82324=CARTESIAN_POINT('Ctrl Pts',(-45.2532956293718,18.3667191300999,20.));
#82325=CARTESIAN_POINT('Ctrl Pts',(-45.2378103049023,18.3967454961016,0.));
#82326=CARTESIAN_POINT('Ctrl Pts',(-45.2378103049023,18.3967454961016,20.));
#82327=CARTESIAN_POINT('Ctrl Pts',(-45.2223048093755,18.4267601937997,0.));
#82328=CARTESIAN_POINT('Ctrl Pts',(-45.2223048093755,18.4267601937997,20.));
#82329=CARTESIAN_POINT('Ctrl Pts',(-45.2067791509123,18.456763209342,0.));
#82330=CARTESIAN_POINT('Ctrl Pts',(-45.2067791509123,18.456763209342,20.));
#82331=CARTESIAN_POINT('Ctrl Pts',(-45.1912333376434,18.4867545288811,0.));
#82332=CARTESIAN_POINT('Ctrl Pts',(-45.1912333376434,18.4867545288811,20.));
#82333=CARTESIAN_POINT('Ctrl Pts',(-45.1756673777099,18.5167341385735,0.));
#82334=CARTESIAN_POINT('Ctrl Pts',(-45.1756673777099,18.5167341385735,20.));
#82335=CARTESIAN_POINT('Ctrl Pts',(-45.1600812792631,18.5467020245809,0.));
#82336=CARTESIAN_POINT('Ctrl Pts',(-45.1600812792631,18.5467020245809,20.));
#82337=CARTESIAN_POINT('Ctrl Pts',(-45.144475050464,18.5766581730694,0.));
#82338=CARTESIAN_POINT('Ctrl Pts',(-45.144475050464,18.5766581730694,20.));
#82339=CARTESIAN_POINT('Ctrl Pts',(-45.1288486994834,18.6066025702106,0.));
#82340=CARTESIAN_POINT('Ctrl Pts',(-45.1288486994834,18.6066025702106,20.));
#82341=CARTESIAN_POINT('Ctrl Pts',(-45.1132022345013,18.6365352021813,0.));
#82342=CARTESIAN_POINT('Ctrl Pts',(-45.1132022345013,18.6365352021813,20.));
#82343=CARTESIAN_POINT('Ctrl Pts',(-45.097535663708,18.6664560551643,0.));
#82344=CARTESIAN_POINT('Ctrl Pts',(-45.097535663708,18.6664560551643,20.));
#82345=CARTESIAN_POINT('Ctrl Pts',(-45.081848995303,18.6963651153477,0.));
#82346=CARTESIAN_POINT('Ctrl Pts',(-45.081848995303,18.6963651153477,20.));
#82347=CARTESIAN_POINT('Ctrl Pts',(-45.0661422374956,18.7262623689254,0.));
#82348=CARTESIAN_POINT('Ctrl Pts',(-45.0661422374956,18.7262623689254,20.));
#82349=CARTESIAN_POINT('Ctrl Pts',(-45.050415398505,18.7561478020964,0.));
#82350=CARTESIAN_POINT('Ctrl Pts',(-45.050415398505,18.7561478020964,20.));
#82351=CARTESIAN_POINT('Ctrl Pts',(-45.0346684865594,18.7860214010651,0.));
#82352=CARTESIAN_POINT('Ctrl Pts',(-45.0346684865594,18.7860214010651,20.));
#82353=CARTESIAN_POINT('Ctrl Pts',(-45.0189015098976,18.815883152041,0.));
#82354=CARTESIAN_POINT('Ctrl Pts',(-45.0189015098976,18.815883152041,20.));
#82355=CARTESIAN_POINT('Ctrl Pts',(-45.0031144767678,18.8457330412389,0.));
#82356=CARTESIAN_POINT('Ctrl Pts',(-45.0031144767678,18.8457330412389,20.));
#82357=CARTESIAN_POINT('Ctrl Pts',(-44.9873073954281,18.8755710548787,0.));
#82358=CARTESIAN_POINT('Ctrl Pts',(-44.9873073954281,18.8755710548787,20.));
#82359=CARTESIAN_POINT('Ctrl Pts',(-44.971480274146,18.9053971791858,0.));
#82360=CARTESIAN_POINT('Ctrl Pts',(-44.971480274146,18.9053971791858,20.));
#82361=CARTESIAN_POINT('Ctrl Pts',(-44.9556331211993,18.9352114003906,0.));
#82362=CARTESIAN_POINT('Ctrl Pts',(-44.9556331211993,18.9352114003906,20.));
#82363=CARTESIAN_POINT('Ctrl Pts',(-44.9397659448753,18.9650137047293,0.));
#82364=CARTESIAN_POINT('Ctrl Pts',(-44.9397659448753,18.9650137047293,20.));
#82365=CARTESIAN_POINT('Ctrl Pts',(-44.9238787534705,18.9948040784434,0.));
#82366=CARTESIAN_POINT('Ctrl Pts',(-44.9238787534705,18.9948040784434,20.));
#82367=CARTESIAN_POINT('Ctrl Pts',(-44.9079715552916,19.0245825077797,0.));
#82368=CARTESIAN_POINT('Ctrl Pts',(-44.9079715552916,19.0245825077797,20.));
#82369=CARTESIAN_POINT('Ctrl Pts',(-44.8920443586544,19.0543489789907,0.));
#82370=CARTESIAN_POINT('Ctrl Pts',(-44.8920443586544,19.0543489789907,20.));
#82371=CARTESIAN_POINT('Ctrl Pts',(-44.8760971718851,19.0841034783341,0.));
#82372=CARTESIAN_POINT('Ctrl Pts',(-44.8760971718851,19.0841034783341,20.));
#82373=CARTESIAN_POINT('Ctrl Pts',(-44.8601300033192,19.1138459920731,0.));
#82374=CARTESIAN_POINT('Ctrl Pts',(-44.8601300033192,19.1138459920731,20.));
#82375=CARTESIAN_POINT('Ctrl Pts',(-44.8441428613021,19.143576506476,0.));
#82376=CARTESIAN_POINT('Ctrl Pts',(-44.8441428613021,19.143576506476,20.));
#82377=CARTESIAN_POINT('Ctrl Pts',(-44.8281357541891,19.1732950078168,0.));
#82378=CARTESIAN_POINT('Ctrl Pts',(-44.8281357541891,19.1732950078168,20.));
#82379=CARTESIAN_POINT('Ctrl Pts',(-44.8121086903447,19.2030014823748,0.));
#82380=CARTESIAN_POINT('Ctrl Pts',(-44.8121086903447,19.2030014823748,20.));
#82381=CARTESIAN_POINT('Ctrl Pts',(-44.7960616781431,19.2326959164344,0.));
#82382=CARTESIAN_POINT('Ctrl Pts',(-44.7960616781431,19.2326959164344,20.));
#82383=CARTESIAN_POINT('Ctrl Pts',(-44.7799947259683,19.2623782962858,0.));
#82384=CARTESIAN_POINT('Ctrl Pts',(-44.7799947259683,19.2623782962858,20.));
#82385=CARTESIAN_POINT('Ctrl Pts',(-44.7639078422139,19.2920486082247,0.));
#82386=CARTESIAN_POINT('Ctrl Pts',(-44.7639078422139,19.2920486082247,20.));
#82387=CARTESIAN_POINT('Ctrl Pts',(-44.7478010352831,19.3217068385519,0.));
#82388=CARTESIAN_POINT('Ctrl Pts',(-44.7478010352831,19.3217068385519,20.));
#82389=CARTESIAN_POINT('Ctrl Pts',(-44.731674313589,19.3513529735741,0.));
#82390=CARTESIAN_POINT('Ctrl Pts',(-44.731674313589,19.3513529735741,20.));
#82391=CARTESIAN_POINT('Ctrl Pts',(-44.7155276855546,19.3809869996033,0.));
#82392=CARTESIAN_POINT('Ctrl Pts',(-44.7155276855546,19.3809869996033,20.));
#82393=CARTESIAN_POINT('Ctrl Pts',(-44.6993611596123,19.4106089029568,0.));
#82394=CARTESIAN_POINT('Ctrl Pts',(-44.6993611596123,19.4106089029568,20.));
#82395=CARTESIAN_POINT('Ctrl Pts',(-44.6831747442042,19.4402186699576,0.));
#82396=CARTESIAN_POINT('Ctrl Pts',(-44.6831747442042,19.4402186699576,20.));
#82397=CARTESIAN_POINT('Ctrl Pts',(-44.666968447782,19.4698162869338,0.));
#82398=CARTESIAN_POINT('Ctrl Pts',(-44.666968447782,19.4698162869338,20.));
#82399=CARTESIAN_POINT('Ctrl Pts',(-44.6507422788067,19.4994017402193,0.));
#82400=CARTESIAN_POINT('Ctrl Pts',(-44.6507422788067,19.4994017402193,20.));
#82401=CARTESIAN_POINT('Ctrl Pts',(-44.6344962457493,19.5289750161533,0.));
#82402=CARTESIAN_POINT('Ctrl Pts',(-44.6344962457493,19.5289750161533,20.));
#82403=CARTESIAN_POINT('Ctrl Pts',(-44.6182303570903,19.5585361010809,0.));
#82404=CARTESIAN_POINT('Ctrl Pts',(-44.6182303570903,19.5585361010809,20.));
#82405=CARTESIAN_POINT('Ctrl Pts',(-44.60194462132,19.5880849813525,0.));
#82406=CARTESIAN_POINT('Ctrl Pts',(-44.60194462132,19.5880849813525,20.));
#82407=CARTESIAN_POINT('Ctrl Pts',(-44.5856390469384,19.6176216433241,0.));
#82408=CARTESIAN_POINT('Ctrl Pts',(-44.5856390469384,19.6176216433241,20.));
#82409=CARTESIAN_POINT('Ctrl Pts',(-44.5693136424549,19.6471460733568,0.));
#82410=CARTESIAN_POINT('Ctrl Pts',(-44.5693136424549,19.6471460733568,20.));
#82411=CARTESIAN_POINT('Ctrl Pts',(-44.5529684163885,19.6766582578175,0.));
#82412=CARTESIAN_POINT('Ctrl Pts',(-44.5529684163885,19.6766582578175,20.));
#82413=CARTESIAN_POINT('Ctrl Pts',(-44.5366033772682,19.7061581830785,0.));
#82414=CARTESIAN_POINT('Ctrl Pts',(-44.5366033772682,19.7061581830785,20.));
#82415=CARTESIAN_POINT('Ctrl Pts',(-44.5202185336324,19.7356458355178,0.));
#82416=CARTESIAN_POINT('Ctrl Pts',(-44.5202185336324,19.7356458355178,20.));
#82417=CARTESIAN_POINT('Ctrl Pts',(-44.5038138940293,19.7651212015191,0.));
#82418=CARTESIAN_POINT('Ctrl Pts',(-44.5038138940293,19.7651212015191,20.));
#82419=CARTESIAN_POINT('Ctrl Pts',(-44.4873894670167,19.7945842674717,0.));
#82420=CARTESIAN_POINT('Ctrl Pts',(-44.4873894670167,19.7945842674717,20.));
#82421=CARTESIAN_POINT('Ctrl Pts',(-44.4709452611615,19.8240350197702,0.));
#82422=CARTESIAN_POINT('Ctrl Pts',(-44.4709452611615,19.8240350197702,20.));
#82423=CARTESIAN_POINT('Ctrl Pts',(-44.4544812850403,19.8534734448146,0.));
#82424=CARTESIAN_POINT('Ctrl Pts',(-44.4544812850403,19.8534734448146,20.));
#82425=CARTESIAN_POINT('Ctrl Pts',(-44.4379975472397,19.8828995290107,0.));
#82426=CARTESIAN_POINT('Ctrl Pts',(-44.4379975472397,19.8828995290107,20.));
#82427=CARTESIAN_POINT('Ctrl Pts',(-44.4214940563557,19.9123132587697,0.));
#82428=CARTESIAN_POINT('Ctrl Pts',(-44.4214940563557,19.9123132587697,20.));
#82429=CARTESIAN_POINT('Ctrl Pts',(-44.4049708209939,19.9417146205087,0.));
#82430=CARTESIAN_POINT('Ctrl Pts',(-44.4049708209939,19.9417146205087,20.));
#82431=CARTESIAN_POINT('Ctrl Pts',(-44.3884278497697,19.9711036006503,0.));
#82432=CARTESIAN_POINT('Ctrl Pts',(-44.3884278497697,19.9711036006503,20.));
#82433=CARTESIAN_POINT('Ctrl Pts',(-44.371865151308,20.0004801856228,0.));
#82434=CARTESIAN_POINT('Ctrl Pts',(-44.371865151308,20.0004801856228,20.));
#82435=CARTESIAN_POINT('Ctrl Pts',(-44.3552827342435,20.0298443618602,0.));
#82436=CARTESIAN_POINT('Ctrl Pts',(-44.3552827342435,20.0298443618602,20.));
#82437=CARTESIAN_POINT('Ctrl Pts',(-44.3386806072204,20.0591961158018,0.));
#82438=CARTESIAN_POINT('Ctrl Pts',(-44.3386806072204,20.0591961158018,20.));
#82439=CARTESIAN_POINT('Ctrl Pts',(-44.3220587788923,20.0885354338929,0.));
#82440=CARTESIAN_POINT('Ctrl Pts',(-44.3220587788923,20.0885354338929,20.));
#82441=CARTESIAN_POINT('Ctrl Pts',(-44.3054172579222,20.117862302584,0.));
#82442=CARTESIAN_POINT('Ctrl Pts',(-44.3054172579222,20.117862302584,20.));
#82443=CARTESIAN_POINT('Ctrl Pts',(-44.2887560529826,20.1471767083313,0.));
#82444=CARTESIAN_POINT('Ctrl Pts',(-44.2887560529826,20.1471767083313,20.));
#82445=CARTESIAN_POINT('Ctrl Pts',(-44.2720751727557,20.1764786375963,0.));
#82446=CARTESIAN_POINT('Ctrl Pts',(-44.2720751727557,20.1764786375963,20.));
#82447=CARTESIAN_POINT('Ctrl Pts',(-44.2553746259333,20.2057680768465,0.));
#82448=CARTESIAN_POINT('Ctrl Pts',(-44.2553746259333,20.2057680768465,20.));
#82449=CARTESIAN_POINT('Ctrl Pts',(-44.238654421217,20.2350450125552,0.));
#82450=CARTESIAN_POINT('Ctrl Pts',(-44.238654421217,20.2350450125552,20.));
#82451=CARTESIAN_POINT('Ctrl Pts',(-44.221914567318,20.2643094312016,0.));
#82452=CARTESIAN_POINT('Ctrl Pts',(-44.221914567318,20.2643094312016,20.));
#82453=CARTESIAN_POINT('Ctrl Pts',(-44.205155072957,20.2935613192706,0.));
#82454=CARTESIAN_POINT('Ctrl Pts',(-44.205155072957,20.2935613192706,20.));
#82455=CARTESIAN_POINT('Ctrl Pts',(-44.1883759468646,20.3228006632528,0.));
#82456=CARTESIAN_POINT('Ctrl Pts',(-44.1883759468646,20.3228006632528,20.));
#82457=CARTESIAN_POINT('Ctrl Pts',(-44.1715771977807,20.3520274496443,0.));
#82458=CARTESIAN_POINT('Ctrl Pts',(-44.1715771977807,20.3520274496443,20.));
#82459=CARTESIAN_POINT('Ctrl Pts',(-44.1547588344544,20.3812416649468,0.));
#82460=CARTESIAN_POINT('Ctrl Pts',(-44.1547588344544,20.3812416649468,20.));
#82461=CARTESIAN_POINT('Ctrl Pts',(-44.1379208656442,20.4104432956673,0.));
#82462=CARTESIAN_POINT('Ctrl Pts',(-44.1379208656442,20.4104432956673,20.));
#82463=CARTESIAN_POINT('Ctrl Pts',(-44.1210633001184,20.4396323283186,0.));
#82464=CARTESIAN_POINT('Ctrl Pts',(-44.1210633001184,20.4396323283186,20.));
#82465=CARTESIAN_POINT('Ctrl Pts',(-44.1041861466545,20.468808749419,0.));
#82466=CARTESIAN_POINT('Ctrl Pts',(-44.1041861466545,20.468808749419,20.));
#82467=CARTESIAN_POINT('Ctrl Pts',(-44.0872894140398,20.4979725454932,0.));
#82468=CARTESIAN_POINT('Ctrl Pts',(-44.0872894140398,20.4979725454932,20.));
#82469=CARTESIAN_POINT('Ctrl Pts',(-44.0703731110714,20.5271237030716,0.));
#82470=CARTESIAN_POINT('Ctrl Pts',(-44.0703731110714,20.5271237030716,20.));
#82471=CARTESIAN_POINT('Ctrl Pts',(-44.053437246556,20.5562622086905,0.));
#82472=CARTESIAN_POINT('Ctrl Pts',(-44.053437246556,20.5562622086905,20.));
#82473=CARTESIAN_POINT('Ctrl Pts',(-44.03648182931,20.5853880488919,0.));
#82474=CARTESIAN_POINT('Ctrl Pts',(-44.03648182931,20.5853880488919,20.));
#82475=CARTESIAN_POINT('Ctrl Pts',(-44.0195068681592,20.6145012102233,0.));
#82476=CARTESIAN_POINT('Ctrl Pts',(-44.0195068681592,20.6145012102233,20.));
#82477=CARTESIAN_POINT('Ctrl Pts',(-44.0025123719387,20.6436016792381,0.));
#82478=CARTESIAN_POINT('Ctrl Pts',(-44.0025123719387,20.6436016792381,20.));
#82479=CARTESIAN_POINT('Ctrl Pts',(-43.9854983494929,20.6726894424949,0.));
#82480=CARTESIAN_POINT('Ctrl Pts',(-43.9854983494929,20.6726894424949,20.));
#82481=CARTESIAN_POINT('Ctrl Pts',(-43.9684648096756,20.7017644865584,0.));
#82482=CARTESIAN_POINT('Ctrl Pts',(-43.9684648096756,20.7017644865584,20.));
#82483=CARTESIAN_POINT('Ctrl Pts',(-43.9514117613501,20.7308267979991,0.));
#82484=CARTESIAN_POINT('Ctrl Pts',(-43.9514117613501,20.7308267979991,20.));
#82485=CARTESIAN_POINT('Ctrl Pts',(-43.9343392133895,20.7598763633934,0.));
#82486=CARTESIAN_POINT('Ctrl Pts',(-43.9343392133895,20.7598763633934,20.));
#82487=CARTESIAN_POINT('Ctrl Pts',(-43.9172471746767,20.7889131693233,0.));
#82488=CARTESIAN_POINT('Ctrl Pts',(-43.9172471746767,20.7889131693233,20.));
#82489=CARTESIAN_POINT('Ctrl Pts',(-43.9001356541037,20.817937202377,0.));
#82490=CARTESIAN_POINT('Ctrl Pts',(-43.9001356541037,20.817937202377,20.));
#82491=CARTESIAN_POINT('Ctrl Pts',(-43.8830046605723,20.8469484491482,0.));
#82492=CARTESIAN_POINT('Ctrl Pts',(-43.8830046605723,20.8469484491482,20.));
#82493=CARTESIAN_POINT('Ctrl Pts',(-43.8658542029936,20.8759468962364,0.));
#82494=CARTESIAN_POINT('Ctrl Pts',(-43.8658542029936,20.8759468962364,20.));
#82495=CARTESIAN_POINT('Ctrl Pts',(-43.8486842902882,20.9049325302471,0.));
#82496=CARTESIAN_POINT('Ctrl Pts',(-43.8486842902882,20.9049325302471,20.));
#82497=CARTESIAN_POINT('Ctrl Pts',(-43.8314949313861,20.9339053377913,0.));
#82498=CARTESIAN_POINT('Ctrl Pts',(-43.8314949313861,20.9339053377913,20.));
#82499=CARTESIAN_POINT('Ctrl Pts',(-43.8142861352268,20.9628653054863,0.));
#82500=CARTESIAN_POINT('Ctrl Pts',(-43.8142861352268,20.9628653054863,20.));
#82501=CARTESIAN_POINT('Ctrl Pts',(-43.7970579107591,20.9918124199547,0.));
#82502=CARTESIAN_POINT('Ctrl Pts',(-43.7970579107591,20.9918124199547,20.));
#82503=CARTESIAN_POINT('Ctrl Pts',(-43.7798102669417,21.0207466678254,0.));
#82504=CARTESIAN_POINT('Ctrl Pts',(-43.7798102669417,21.0207466678254,20.));
#82505=CARTESIAN_POINT('Ctrl Pts',(-43.7625432127426,21.0496680357328,0.));
#82506=CARTESIAN_POINT('Ctrl Pts',(-43.7625432127426,21.0496680357328,20.));
#82507=CARTESIAN_POINT('Ctrl Pts',(-43.7452567571393,21.0785765103172,0.));
#82508=CARTESIAN_POINT('Ctrl Pts',(-43.7452567571393,21.0785765103172,20.));
#82509=CARTESIAN_POINT('Ctrl Pts',(-43.7279509091188,21.1074720782252,0.));
#82510=CARTESIAN_POINT('Ctrl Pts',(-43.7279509091188,21.1074720782252,20.));
#82511=CARTESIAN_POINT('Ctrl Pts',(-43.7106256776774,21.1363547261089,0.));
#82512=CARTESIAN_POINT('Ctrl Pts',(-43.7106256776774,21.1363547261089,20.));
#82513=CARTESIAN_POINT('Ctrl Pts',(-43.6932810718209,21.1652244406266,0.));
#82514=CARTESIAN_POINT('Ctrl Pts',(-43.6932810718209,21.1652244406266,20.));
#82515=CARTESIAN_POINT('Ctrl Pts',(-43.6759171005642,21.1940812084419,0.));
#82516=CARTESIAN_POINT('Ctrl Pts',(-43.6759171005642,21.1940812084419,20.));
#82517=CARTESIAN_POINT('Ctrl Pts',(-43.658533772932,21.2229250162246,0.));
#82518=CARTESIAN_POINT('Ctrl Pts',(-43.658533772932,21.2229250162246,20.));
#82519=CARTESIAN_POINT('Ctrl Pts',(-43.6411310979585,21.2517558506503,0.));
#82520=CARTESIAN_POINT('Ctrl Pts',(-43.6411310979585,21.2517558506503,20.));
#82521=CARTESIAN_POINT('Ctrl Pts',(-43.6237090846874,21.2805736984007,0.));
#82522=CARTESIAN_POINT('Ctrl Pts',(-43.6237090846874,21.2805736984007,20.));
#82523=CARTESIAN_POINT('Ctrl Pts',(-43.6062677421718,21.3093785461635,0.));
#82524=CARTESIAN_POINT('Ctrl Pts',(-43.6062677421718,21.3093785461635,20.));
#82525=CARTESIAN_POINT('Ctrl Pts',(-43.5888070794743,21.3381703806323,0.));
#82526=CARTESIAN_POINT('Ctrl Pts',(-43.5888070794743,21.3381703806323,20.));
#82527=CARTESIAN_POINT('Ctrl Pts',(-43.571327105667,21.3669491885068,0.));
#82528=CARTESIAN_POINT('Ctrl Pts',(-43.571327105667,21.3669491885068,20.));
#82529=CARTESIAN_POINT('Ctrl Pts',(-43.5538278298311,21.3957149564922,0.));
#82530=CARTESIAN_POINT('Ctrl Pts',(-43.5538278298311,21.3957149564922,20.));
#82531=CARTESIAN_POINT('Ctrl Pts',(-43.5363092610574,21.4244676712999,0.));
#82532=CARTESIAN_POINT('Ctrl Pts',(-43.5363092610574,21.4244676712999,20.));
#82533=CARTESIAN_POINT('Ctrl Pts',(-43.5187714084458,21.4532073196468,0.));
#82534=CARTESIAN_POINT('Ctrl Pts',(-43.5187714084458,21.4532073196468,20.));
#82535=CARTESIAN_POINT('Ctrl Pts',(-43.5012142811058,21.4819338882558,0.));
#82536=CARTESIAN_POINT('Ctrl Pts',(-43.5012142811058,21.4819338882558,20.));
#82537=CARTESIAN_POINT('Ctrl Pts',(-43.4836378881563,21.5106473638561,0.));
#82538=CARTESIAN_POINT('Ctrl Pts',(-43.4836378881563,21.5106473638561,20.));
#82539=CARTESIAN_POINT('Ctrl Pts',(-43.4660422387257,21.5393477331829,0.));
#82540=CARTESIAN_POINT('Ctrl Pts',(-43.4660422387257,21.5393477331829,20.));
#82541=CARTESIAN_POINT('Ctrl Pts',(-43.4484273419519,21.5680349829773,0.));
#82542=CARTESIAN_POINT('Ctrl Pts',(-43.4484273419519,21.5680349829773,20.));
#82543=CARTESIAN_POINT('Ctrl Pts',(-43.4307932069824,21.5967090999869,0.));
#82544=CARTESIAN_POINT('Ctrl Pts',(-43.4307932069824,21.5967090999869,20.));
#82545=CARTESIAN_POINT('Ctrl Pts',(-43.4131398429739,21.6253700709647,0.));
#82546=CARTESIAN_POINT('Ctrl Pts',(-43.4131398429739,21.6253700709647,20.));
#82547=CARTESIAN_POINT('Ctrl Pts',(-43.3954672590924,21.6540178826698,0.));
#82548=CARTESIAN_POINT('Ctrl Pts',(-43.3954672590924,21.6540178826698,20.));
#82549=CARTESIAN_POINT('Ctrl Pts',(-43.3777754645132,21.682652521867,0.));
#82550=CARTESIAN_POINT('Ctrl Pts',(-43.3777754645132,21.682652521867,20.));
#82551=CARTESIAN_POINT('Ctrl Pts',(-43.3600644684208,21.7112739753274,0.));
#82552=CARTESIAN_POINT('Ctrl Pts',(-43.3600644684208,21.7112739753274,20.));
#82553=CARTESIAN_POINT('Ctrl Pts',(-43.3423342800096,21.7398822298281,0.));
#82554=CARTESIAN_POINT('Ctrl Pts',(-43.3423342800096,21.7398822298281,20.));
#82555=CARTESIAN_POINT('Ctrl Pts',(-43.3245849084831,21.7684772721522,0.));
#82556=CARTESIAN_POINT('Ctrl Pts',(-43.3245849084831,21.7684772721522,20.));
#82557=CARTESIAN_POINT('Ctrl Pts',(-43.3068163630542,21.7970590890891,0.));
#82558=CARTESIAN_POINT('Ctrl Pts',(-43.3068163630542,21.7970590890891,20.));
#82559=CARTESIAN_POINT('Ctrl Pts',(-43.2890286529453,21.8256276674339,0.));
#82560=CARTESIAN_POINT('Ctrl Pts',(-43.2890286529453,21.8256276674339,20.));
#82561=CARTESIAN_POINT('Ctrl Pts',(-43.271221787388,21.8541829939879,0.));
#82562=CARTESIAN_POINT('Ctrl Pts',(-43.271221787388,21.8541829939879,20.));
#82563=CARTESIAN_POINT('Ctrl Pts',(-43.2533957756234,21.8827250555583,0.));
#82564=CARTESIAN_POINT('Ctrl Pts',(-43.2533957756234,21.8827250555583,20.));
#82565=CARTESIAN_POINT('Ctrl Pts',(-43.2355506269018,21.9112538389585,0.));
#82566=CARTESIAN_POINT('Ctrl Pts',(-43.2355506269018,21.9112538389585,20.));
#82567=CARTESIAN_POINT('Ctrl Pts',(-43.217686350483,21.9397693310079,0.));
#82568=CARTESIAN_POINT('Ctrl Pts',(-43.217686350483,21.9397693310079,20.));
#82569=CARTESIAN_POINT('Ctrl Pts',(-43.1998029556363,21.9682715185322,0.));
#82570=CARTESIAN_POINT('Ctrl Pts',(-43.1998029556363,21.9682715185322,20.));
#82571=CARTESIAN_POINT('Ctrl Pts',(-43.1819004516401,21.9967603883628,0.));
#82572=CARTESIAN_POINT('Ctrl Pts',(-43.1819004516401,21.9967603883628,20.));
#82573=CARTESIAN_POINT('Ctrl Pts',(-43.1639788477821,22.0252359273373,0.));
#82574=CARTESIAN_POINT('Ctrl Pts',(-43.1639788477821,22.0252359273373,20.));
#82575=CARTESIAN_POINT('Ctrl Pts',(-43.1460381533594,22.0536981222997,0.));
#82576=CARTESIAN_POINT('Ctrl Pts',(-43.1460381533594,22.0536981222997,20.));
#82577=CARTESIAN_POINT('Ctrl Pts',(-43.1280783776785,22.0821469600997,0.));
#82578=CARTESIAN_POINT('Ctrl Pts',(-43.1280783776785,22.0821469600997,20.));
#82579=CARTESIAN_POINT('Ctrl Pts',(-43.1100995300552,22.1105824275933,0.));
#82580=CARTESIAN_POINT('Ctrl Pts',(-43.1100995300552,22.1105824275933,20.));
#82581=CARTESIAN_POINT('Ctrl Pts',(-43.0921016198148,22.1390045116426,0.));
#82582=CARTESIAN_POINT('Ctrl Pts',(-43.0921016198148,22.1390045116426,20.));
#82583=CARTESIAN_POINT('Ctrl Pts',(-43.0740846562917,22.1674131991155,0.));
#82584=CARTESIAN_POINT('Ctrl Pts',(-43.0740846562917,22.1674131991155,20.));
#82585=CARTESIAN_POINT('Ctrl Pts',(-43.0560486488298,22.1958084768867,0.));
#82586=CARTESIAN_POINT('Ctrl Pts',(-43.0560486488298,22.1958084768867,20.));
#82587=CARTESIAN_POINT('Ctrl Pts',(-43.0379936067822,22.2241903318366,0.));
#82588=CARTESIAN_POINT('Ctrl Pts',(-43.0379936067822,22.2241903318366,20.));
#82589=CARTESIAN_POINT('Ctrl Pts',(-43.0199195395115,22.252558750852,0.));
#82590=CARTESIAN_POINT('Ctrl Pts',(-43.0199195395115,22.252558750852,20.));
#82591=CARTESIAN_POINT('Ctrl Pts',(-43.0018264563892,22.2809137208256,0.));
#82592=CARTESIAN_POINT('Ctrl Pts',(-43.0018264563892,22.2809137208256,20.));
#82593=CARTESIAN_POINT('Ctrl Pts',(-42.9837143667966,22.3092552286564,0.));
#82594=CARTESIAN_POINT('Ctrl Pts',(-42.9837143667966,22.3092552286564,20.));
#82595=CARTESIAN_POINT('Ctrl Pts',(-42.965583280124,22.3375832612492,0.));
#82596=CARTESIAN_POINT('Ctrl Pts',(-42.965583280124,22.3375832612492,20.));
#82597=CARTESIAN_POINT('Ctrl Pts',(-42.947433205771,22.3658978055149,0.));
#82598=CARTESIAN_POINT('Ctrl Pts',(-42.947433205771,22.3658978055149,20.));
#82599=CARTESIAN_POINT('Ctrl Pts',(-42.9292641531465,22.3941988483709,0.));
#82600=CARTESIAN_POINT('Ctrl Pts',(-42.9292641531465,22.3941988483709,20.));
#82601=CARTESIAN_POINT('Ctrl Pts',(-42.9110761316689,22.4224863767407,0.));
#82602=CARTESIAN_POINT('Ctrl Pts',(-42.9110761316689,22.4224863767407,20.));
#82603=CARTESIAN_POINT('Ctrl Pts',(-42.8928691507659,22.4507603775546,0.));
#82604=CARTESIAN_POINT('Ctrl Pts',(-42.8928691507659,22.4507603775546,20.));
#82605=CARTESIAN_POINT('Ctrl Pts',(-42.8746432198744,22.4790208377488,0.));
#82606=CARTESIAN_POINT('Ctrl Pts',(-42.8746432198744,22.4790208377488,20.));
#82607=CARTESIAN_POINT('Ctrl Pts',(-42.8563983484404,22.5072677442656,0.));
#82608=CARTESIAN_POINT('Ctrl Pts',(-42.8563983484404,22.5072677442656,20.));
#82609=CARTESIAN_POINT('Ctrl Pts',(-42.8381345459193,22.535501084053,0.));
#82610=CARTESIAN_POINT('Ctrl Pts',(-42.8381345459193,22.535501084053,20.));
#82611=CARTESIAN_POINT('Ctrl Pts',(-42.8198518217756,22.5637208440656,0.));
#82612=CARTESIAN_POINT('Ctrl Pts',(-42.8198518217756,22.5637208440656,20.));
#82613=CARTESIAN_POINT('Ctrl Pts',(-42.8015501854832,22.5919270112639,0.));
#82614=CARTESIAN_POINT('Ctrl Pts',(-42.8015501854832,22.5919270112639,20.));
#82615=CARTESIAN_POINT('Ctrl Pts',(-42.7832296465255,22.620119572615,0.));
#82616=CARTESIAN_POINT('Ctrl Pts',(-42.7832296465255,22.620119572615,20.));
#82617=CARTESIAN_POINT('Ctrl Pts',(-42.7648902143955,22.6482985150925,0.));
#82618=CARTESIAN_POINT('Ctrl Pts',(-42.7648902143955,22.6482985150925,20.));
#82619=CARTESIAN_POINT('Ctrl Pts',(-42.7465318985949,22.6764638256759,0.));
#82620=CARTESIAN_POINT('Ctrl Pts',(-42.7465318985949,22.6764638256759,20.));
#82621=CARTESIAN_POINT('Ctrl Pts',(-42.7281547086347,22.7046154913511,0.));
#82622=CARTESIAN_POINT('Ctrl Pts',(-42.7281547086347,22.7046154913511,20.));
#82623=CARTESIAN_POINT('Ctrl Pts',(-42.7097586540349,22.73275349911,0.));
#82624=CARTESIAN_POINT('Ctrl Pts',(-42.7097586540349,22.73275349911,20.));
#82625=CARTESIAN_POINT('Ctrl Pts',(-42.6913437443248,22.7608778359508,0.));
#82626=CARTESIAN_POINT('Ctrl Pts',(-42.6913437443248,22.7608778359508,20.));
#82627=CARTESIAN_POINT('Ctrl Pts',(-42.6729099890431,22.788988488878,0.));
#82628=CARTESIAN_POINT('Ctrl Pts',(-42.6729099890431,22.788988488878,20.));
#82629=CARTESIAN_POINT('Ctrl Pts',(-42.6544573977378,22.8170854449023,0.));
#82630=CARTESIAN_POINT('Ctrl Pts',(-42.6544573977378,22.8170854449023,20.));
#82631=CARTESIAN_POINT('Ctrl Pts',(-42.6359859799663,22.845168691041,0.));
#82632=CARTESIAN_POINT('Ctrl Pts',(-42.6359859799663,22.845168691041,20.));
#82633=CARTESIAN_POINT('Ctrl Pts',(-42.6174957452953,22.8732382143174,0.));
#82634=CARTESIAN_POINT('Ctrl Pts',(-42.6174957452953,22.8732382143174,20.));
#82635=CARTESIAN_POINT('Ctrl Pts',(-42.5989867033005,22.9012940017616,0.));
#82636=CARTESIAN_POINT('Ctrl Pts',(-42.5989867033005,22.9012940017616,20.));
#82637=CARTESIAN_POINT('Ctrl Pts',(-42.5804588635669,22.9293360404094,0.));
#82638=CARTESIAN_POINT('Ctrl Pts',(-42.5804588635669,22.9293360404094,20.));
#82639=CARTESIAN_POINT('Ctrl Pts',(-42.5619122356886,22.9573643173033,0.));
#82640=CARTESIAN_POINT('Ctrl Pts',(-42.5619122356886,22.9573643173033,20.));
#82641=CARTESIAN_POINT('Ctrl Pts',(-42.5433468292689,22.9853788194919,0.));
#82642=CARTESIAN_POINT('Ctrl Pts',(-42.5433468292689,22.9853788194919,20.));
#82643=CARTESIAN_POINT('Ctrl Pts',(-42.5247626539203,23.0133795340298,0.));
#82644=CARTESIAN_POINT('Ctrl Pts',(-42.5247626539203,23.0133795340298,20.));
#82645=CARTESIAN_POINT('Ctrl Pts',(-42.5061597192647,23.0413664479785,0.));
#82646=CARTESIAN_POINT('Ctrl Pts',(-42.5061597192647,23.0413664479785,20.));
#82647=CARTESIAN_POINT('Ctrl Pts',(-42.4875380349329,23.0693395484056,0.));
#82648=CARTESIAN_POINT('Ctrl Pts',(-42.4875380349329,23.0693395484056,20.));
#82649=CARTESIAN_POINT('Ctrl Pts',(-42.4688976105654,23.0972988223849,0.));
#82650=CARTESIAN_POINT('Ctrl Pts',(-42.4688976105654,23.0972988223849,20.));
#82651=CARTESIAN_POINT('Ctrl Pts',(-42.4502384558115,23.125244256997,0.));
#82652=CARTESIAN_POINT('Ctrl Pts',(-42.4502384558115,23.125244256997,20.));
#82653=CARTESIAN_POINT('Ctrl Pts',(-42.4315605803298,23.1531758393284,0.));
#82654=CARTESIAN_POINT('Ctrl Pts',(-42.4315605803298,23.1531758393284,20.));
#82655=CARTESIAN_POINT('Ctrl Pts',(-42.4128639937879,23.1810935564721,0.));
#82656=CARTESIAN_POINT('Ctrl Pts',(-42.4128639937879,23.1810935564721,20.));
#82657=CARTESIAN_POINT('Ctrl Pts',(-42.3941487058631,23.2089973955278,0.));
#82658=CARTESIAN_POINT('Ctrl Pts',(-42.3941487058631,23.2089973955278,20.));
#82659=CARTESIAN_POINT('Ctrl Pts',(-42.3754147262417,23.2368873436013,0.));
#82660=CARTESIAN_POINT('Ctrl Pts',(-42.3754147262417,23.2368873436013,20.));
#82661=CARTESIAN_POINT('Ctrl Pts',(-42.3566620646188,23.2647633878047,0.));
#82662=CARTESIAN_POINT('Ctrl Pts',(-42.3566620646188,23.2647633878047,20.));
#82663=CARTESIAN_POINT('Ctrl Pts',(-42.3378907306988,23.2926255152563,0.));
#82664=CARTESIAN_POINT('Ctrl Pts',(-42.3378907306988,23.2926255152563,20.));
#82665=CARTESIAN_POINT('Ctrl Pts',(-42.3191007341954,23.320473713081,0.));
#82666=CARTESIAN_POINT('Ctrl Pts',(-42.3191007341954,23.320473713081,20.));
#82667=CARTESIAN_POINT('Ctrl Pts',(-42.3002920848317,23.3483079684103,0.));
#82668=CARTESIAN_POINT('Ctrl Pts',(-42.3002920848317,23.3483079684103,20.));
#82669=CARTESIAN_POINT('Ctrl Pts',(-42.2814647923395,23.3761282683822,0.));
#82670=CARTESIAN_POINT('Ctrl Pts',(-42.2814647923395,23.3761282683822,20.));
#82671=CARTESIAN_POINT('Ctrl Pts',(-42.2626188664603,23.4039346001409,0.));
#82672=CARTESIAN_POINT('Ctrl Pts',(-42.2626188664603,23.4039346001409,20.));
#82673=CARTESIAN_POINT('Ctrl Pts',(-42.2437543169442,23.4317269508371,0.));
#82674=CARTESIAN_POINT('Ctrl Pts',(-42.2437543169442,23.4317269508371,20.));
#82675=CARTESIAN_POINT('Ctrl Pts',(-42.2248711535508,23.4595053076277,0.));
#82676=CARTESIAN_POINT('Ctrl Pts',(-42.2248711535508,23.4595053076277,20.));
#82677=CARTESIAN_POINT('Ctrl Pts',(-42.2059693860486,23.4872696576759,0.));
#82678=CARTESIAN_POINT('Ctrl Pts',(-42.2059693860486,23.4872696576759,20.));
#82679=CARTESIAN_POINT('Ctrl Pts',(-42.1870490242153,23.5150199881514,0.));
#82680=CARTESIAN_POINT('Ctrl Pts',(-42.1870490242153,23.5150199881514,20.));
#82681=CARTESIAN_POINT('Ctrl Pts',(-42.1681100778379,23.5427562862307,0.));
#82682=CARTESIAN_POINT('Ctrl Pts',(-42.1681100778379,23.5427562862307,20.));
#82683=CARTESIAN_POINT('Ctrl Pts',(-42.1491525567126,23.5704785390969,0.));
#82684=CARTESIAN_POINT('Ctrl Pts',(-42.1491525567126,23.5704785390969,20.));
#82685=CARTESIAN_POINT('Ctrl Pts',(-42.1301764706447,23.5981867339394,0.));
#82686=CARTESIAN_POINT('Ctrl Pts',(-42.1301764706447,23.5981867339394,20.));
#82687=CARTESIAN_POINT('Ctrl Pts',(-42.1111818294483,23.6258808579542,0.));
#82688=CARTESIAN_POINT('Ctrl Pts',(-42.1111818294483,23.6258808579542,20.));
#82689=CARTESIAN_POINT('Ctrl Pts',(-42.0921686429469,23.6535608983435,0.));
#82690=CARTESIAN_POINT('Ctrl Pts',(-42.0921686429469,23.6535608983435,20.));
#82691=CARTESIAN_POINT('Ctrl Pts',(-42.0731369209731,23.6812268423159,0.));
#82692=CARTESIAN_POINT('Ctrl Pts',(-42.0731369209731,23.6812268423159,20.));
#82693=CARTESIAN_POINT('Ctrl Pts',(-42.0540866733685,23.7088786770864,0.));
#82694=CARTESIAN_POINT('Ctrl Pts',(-42.0540866733685,23.7088786770864,20.));
#82695=CARTESIAN_POINT('Ctrl Pts',(-42.0350179099839,23.7365163898767,0.));
#82696=CARTESIAN_POINT('Ctrl Pts',(-42.0350179099839,23.7365163898767,20.));
#82697=CARTESIAN_POINT('Ctrl Pts',(-42.0159306406794,23.7641399679152,0.));
#82698=CARTESIAN_POINT('Ctrl Pts',(-42.0159306406794,23.7641399679152,20.));
#82699=CARTESIAN_POINT('Ctrl Pts',(-41.9968248753238,23.7917493984363,0.));
#82700=CARTESIAN_POINT('Ctrl Pts',(-41.9968248753238,23.7917493984363,20.));
#82701=CARTESIAN_POINT('Ctrl Pts',(-41.9777006237952,23.8193446686815,0.));
#82702=CARTESIAN_POINT('Ctrl Pts',(-41.9777006237952,23.8193446686815,20.));
#82703=CARTESIAN_POINT('Ctrl Pts',(-41.9585578959807,23.8469257658985,0.));
#82704=CARTESIAN_POINT('Ctrl Pts',(-41.9585578959807,23.8469257658985,20.));
#82705=CARTESIAN_POINT('Ctrl Pts',(-41.9393967017767,23.8744926773418,0.));
#82706=CARTESIAN_POINT('Ctrl Pts',(-41.9393967017767,23.8744926773418,20.));
#82707=CARTESIAN_POINT('Ctrl Pts',(-41.9202170510888,23.9020453902722,0.));
#82708=CARTESIAN_POINT('Ctrl Pts',(-41.9202170510888,23.9020453902722,20.));
#82709=CARTESIAN_POINT('Ctrl Pts',(-41.9010189538314,23.9295838919572,0.));
#82710=CARTESIAN_POINT('Ctrl Pts',(-41.9010189538314,23.9295838919572,20.));
#82711=CARTESIAN_POINT('Ctrl Pts',(-41.8818024199281,23.9571081696707,0.));
#82712=CARTESIAN_POINT('Ctrl Pts',(-41.8818024199281,23.9571081696707,20.));
#82713=CARTESIAN_POINT('Ctrl Pts',(-41.8625674593112,23.984618210693,0.));
#82714=CARTESIAN_POINT('Ctrl Pts',(-41.8625674593112,23.984618210693,20.));
#82715=CARTESIAN_POINT('Ctrl Pts',(-41.8433140819226,24.0121140023113,0.));
#82716=CARTESIAN_POINT('Ctrl Pts',(-41.8433140819226,24.0121140023113,20.));
#82717=CARTESIAN_POINT('Ctrl Pts',(-41.824042297713,24.0395955318191,0.));
#82718=CARTESIAN_POINT('Ctrl Pts',(-41.824042297713,24.0395955318191,20.));
#82719=CARTESIAN_POINT('Ctrl Pts',(-41.8047521166422,24.0670627865166,0.));
#82720=CARTESIAN_POINT('Ctrl Pts',(-41.8047521166422,24.0670627865166,20.));
#82721=CARTESIAN_POINT('Ctrl Pts',(-41.785443548679,24.0945157537107,0.));
#82722=CARTESIAN_POINT('Ctrl Pts',(-41.785443548679,24.0945157537107,20.));
#82723=CARTESIAN_POINT('Ctrl Pts',(-41.7661166038015,24.1219544207148,0.));
#82724=CARTESIAN_POINT('Ctrl Pts',(-41.7661166038015,24.1219544207148,20.));
#82725=CARTESIAN_POINT('Ctrl Pts',(-41.7467712919966,24.1493787748488,0.));
#82726=CARTESIAN_POINT('Ctrl Pts',(-41.7467712919966,24.1493787748488,20.));
#82727=CARTESIAN_POINT('Ctrl Pts',(-41.7274076232605,24.1767888034393,0.));
#82728=CARTESIAN_POINT('Ctrl Pts',(-41.7274076232605,24.1767888034393,20.));
#82729=CARTESIAN_POINT('Ctrl Pts',(-41.7080256075983,24.2041844938197,0.));
#82730=CARTESIAN_POINT('Ctrl Pts',(-41.7080256075983,24.2041844938197,20.));
#82731=CARTESIAN_POINT('Ctrl Pts',(-41.688625255024,24.2315658333297,0.));
#82732=CARTESIAN_POINT('Ctrl Pts',(-41.688625255024,24.2315658333297,20.));
#82733=CARTESIAN_POINT('Ctrl Pts',(-41.6692065755608,24.2589328093159,0.));
#82734=CARTESIAN_POINT('Ctrl Pts',(-41.6692065755608,24.2589328093159,20.));
#82735=CARTESIAN_POINT('Ctrl Pts',(-41.6497695792407,24.2862854091312,0.));
#82736=CARTESIAN_POINT('Ctrl Pts',(-41.6497695792407,24.2862854091312,20.));
#82737=CARTESIAN_POINT('Ctrl Pts',(-41.630314276105,24.3136236201351,0.));
#82738=CARTESIAN_POINT('Ctrl Pts',(-41.630314276105,24.3136236201351,20.));
#82739=CARTESIAN_POINT('Ctrl Pts',(-41.610840676204,24.340947429694,0.));
#82740=CARTESIAN_POINT('Ctrl Pts',(-41.610840676204,24.340947429694,20.));
#82741=CARTESIAN_POINT('Ctrl Pts',(-41.5913487895971,24.368256825181,0.));
#82742=CARTESIAN_POINT('Ctrl Pts',(-41.5913487895971,24.368256825181,20.));
#82743=CARTESIAN_POINT('Ctrl Pts',(-41.5718386263526,24.3955517939756,0.));
#82744=CARTESIAN_POINT('Ctrl Pts',(-41.5718386263526,24.3955517939756,20.));
#82745=CARTESIAN_POINT('Ctrl Pts',(-41.5523101965477,24.4228323234645,0.));
#82746=CARTESIAN_POINT('Ctrl Pts',(-41.5523101965477,24.4228323234645,20.));
#82747=CARTESIAN_POINT('Ctrl Pts',(-41.5327635102685,24.4500984010406,0.));
#82748=CARTESIAN_POINT('Ctrl Pts',(-41.5327635102685,24.4500984010406,20.));
#82749=CARTESIAN_POINT('Ctrl Pts',(-41.5131985776101,24.4773500141036,0.));
#82750=CARTESIAN_POINT('Ctrl Pts',(-41.5131985776101,24.4773500141036,20.));
#82751=CARTESIAN_POINT('Ctrl Pts',(-41.4936154086768,24.5045871500598,0.));
#82752=CARTESIAN_POINT('Ctrl Pts',(-41.4936154086768,24.5045871500598,20.));
#82753=CARTESIAN_POINT('Ctrl Pts',(-41.4740140135823,24.5318097963222,0.));
#82754=CARTESIAN_POINT('Ctrl Pts',(-41.4740140135823,24.5318097963222,20.));
#82755=CARTESIAN_POINT('Ctrl Pts',(-41.4543944024488,24.5590179403106,0.));
#82756=CARTESIAN_POINT('Ctrl Pts',(-41.4543944024488,24.5590179403106,20.));
#82757=CARTESIAN_POINT('Ctrl Pts',(-41.4347565854076,24.5862115694513,0.));
#82758=CARTESIAN_POINT('Ctrl Pts',(-41.4347565854076,24.5862115694513,20.));
#82759=CARTESIAN_POINT('Ctrl Pts',(-41.4151005725989,24.6133906711774,0.));
#82760=CARTESIAN_POINT('Ctrl Pts',(-41.4151005725989,24.6133906711774,20.));
#82761=CARTESIAN_POINT('Ctrl Pts',(-41.3954263741717,24.6405552329288,0.));
#82762=CARTESIAN_POINT('Ctrl Pts',(-41.3954263741717,24.6405552329288,20.));
#82763=CARTESIAN_POINT('Ctrl Pts',(-41.3757340002844,24.6677052421523,0.));
#82764=CARTESIAN_POINT('Ctrl Pts',(-41.3757340002844,24.6677052421523,20.));
#82765=CARTESIAN_POINT('Ctrl Pts',(-41.3560234611038,24.694840686301,0.));
#82766=CARTESIAN_POINT('Ctrl Pts',(-41.3560234611038,24.694840686301,20.));
#82767=CARTESIAN_POINT('Ctrl Pts',(-41.3362947668064,24.7219615528352,0.));
#82768=CARTESIAN_POINT('Ctrl Pts',(-41.3362947668064,24.7219615528352,20.));
#82769=CARTESIAN_POINT('Ctrl Pts',(-41.3165479275773,24.7490678292217,0.));
#82770=CARTESIAN_POINT('Ctrl Pts',(-41.3165479275773,24.7490678292217,20.));
#82771=CARTESIAN_POINT('Ctrl Pts',(-41.2967829536105,24.776159502934,0.));
#82772=CARTESIAN_POINT('Ctrl Pts',(-41.2967829536105,24.776159502934,20.));
#82773=CARTESIAN_POINT('Ctrl Pts',(-41.276999855109,24.8032365614525,0.));
#82774=CARTESIAN_POINT('Ctrl Pts',(-41.276999855109,24.8032365614525,20.));
#82775=CARTESIAN_POINT('Ctrl Pts',(-41.2571986422843,24.8302989922639,0.));
#82776=CARTESIAN_POINT('Ctrl Pts',(-41.2571986422843,24.8302989922639,20.));
#82777=CARTESIAN_POINT('Ctrl Pts',(-41.2373793253577,24.8573467828623,0.));
#82778=CARTESIAN_POINT('Ctrl Pts',(-41.2373793253577,24.8573467828623,20.));
#82779=CARTESIAN_POINT('Ctrl Pts',(-41.2175419145589,24.8843799207482,0.));
#82780=CARTESIAN_POINT('Ctrl Pts',(-41.2175419145589,24.8843799207482,20.));
#82781=CARTESIAN_POINT('Ctrl Pts',(-41.1976864201268,24.9113983934293,0.));
#82782=CARTESIAN_POINT('Ctrl Pts',(-41.1976864201268,24.9113983934293,20.));
#82783=CARTESIAN_POINT('Ctrl Pts',(-41.1778128523092,24.9384021884197,0.));
#82784=CARTESIAN_POINT('Ctrl Pts',(-41.1778128523092,24.9384021884197,20.));
#82785=CARTESIAN_POINT('Ctrl Pts',(-41.1579212213625,24.9653912932402,0.));
#82786=CARTESIAN_POINT('Ctrl Pts',(-41.1579212213625,24.9653912932402,20.));
#82787=CARTESIAN_POINT('Ctrl Pts',(-41.1380115375521,24.9923656954187,0.));
#82788=CARTESIAN_POINT('Ctrl Pts',(-41.1380115375521,24.9923656954187,20.));
#82789=CARTESIAN_POINT('Ctrl Pts',(-41.1180838111525,25.0193253824897,0.));
#82790=CARTESIAN_POINT('Ctrl Pts',(-41.1180838111525,25.0193253824897,20.));
#82791=CARTESIAN_POINT('Ctrl Pts',(-41.0981380524472,25.0462703419947,0.));
#82792=CARTESIAN_POINT('Ctrl Pts',(-41.0981380524472,25.0462703419947,20.));
#82793=CARTESIAN_POINT('Ctrl Pts',(-41.0781742717283,25.0732005614819,0.));
#82794=CARTESIAN_POINT('Ctrl Pts',(-41.0781742717283,25.0732005614819,20.));
#82795=CARTESIAN_POINT('Ctrl Pts',(-41.058192479297,25.1001160285063,0.));
#82796=CARTESIAN_POINT('Ctrl Pts',(-41.058192479297,25.1001160285063,20.));
#82797=CARTESIAN_POINT('Ctrl Pts',(-41.0381926854636,25.1270167306298,0.));
#82798=CARTESIAN_POINT('Ctrl Pts',(-41.0381926854636,25.1270167306298,20.));
#82799=CARTESIAN_POINT('Ctrl Pts',(-41.0181749005471,25.1539026554213,0.));
#82800=CARTESIAN_POINT('Ctrl Pts',(-41.0181749005471,25.1539026554213,20.));
#82801=CARTESIAN_POINT('Ctrl Pts',(-40.9981391348755,25.1807737904566,0.));
#82802=CARTESIAN_POINT('Ctrl Pts',(-40.9981391348755,25.1807737904566,20.));
#82803=CARTESIAN_POINT('Ctrl Pts',(-40.9780853987856,25.2076301233182,0.));
#82804=CARTESIAN_POINT('Ctrl Pts',(-40.9780853987856,25.2076301233182,20.));
#82805=CARTESIAN_POINT('Ctrl Pts',(-40.9580137026228,25.2344716415952,0.));
#82806=CARTESIAN_POINT('Ctrl Pts',(-40.9580137026228,25.2344716415952,20.));
#82807=CARTESIAN_POINT('Ctrl Pts',(-40.9379240567416,25.2612983328836,0.));
#82808=CARTESIAN_POINT('Ctrl Pts',(-40.9379240567416,25.2612983328836,20.));
#82809=CARTESIAN_POINT('Ctrl Pts',(-40.9178164715051,25.2881101847861,0.));
#82810=CARTESIAN_POINT('Ctrl Pts',(-40.9178164715051,25.2881101847861,20.));
#82811=CARTESIAN_POINT('Ctrl Pts',(-40.8976909572856,25.3149071849127,0.));
#82812=CARTESIAN_POINT('Ctrl Pts',(-40.8976909572856,25.3149071849127,20.));
#82813=CARTESIAN_POINT('Ctrl Pts',(-40.8775475244644,25.3416893208802,0.));
#82814=CARTESIAN_POINT('Ctrl Pts',(-40.8775475244644,25.3416893208802,20.));
#82815=CARTESIAN_POINT('Ctrl Pts',(-40.8573861834316,25.3684565803126,0.));
#82816=CARTESIAN_POINT('Ctrl Pts',(-40.8573861834316,25.3684565803126,20.));
#82817=CARTESIAN_POINT('Ctrl Pts',(-40.8372069445862,25.3952089508407,0.));
#82818=CARTESIAN_POINT('Ctrl Pts',(-40.8372069445862,25.3952089508407,20.));
#82819=CARTESIAN_POINT('Ctrl Pts',(-40.8170098183362,25.4219464201024,0.));
#82820=CARTESIAN_POINT('Ctrl Pts',(-40.8170098183362,25.4219464201024,20.));
#82821=CARTESIAN_POINT('Ctrl Pts',(-40.7967948150981,25.4486689757422,0.));
#82822=CARTESIAN_POINT('Ctrl Pts',(-40.7967948150981,25.4486689757422,20.));
#82823=CARTESIAN_POINT('Ctrl Pts',(-40.7765619452973,25.4753766054114,0.));
#82824=CARTESIAN_POINT('Ctrl Pts',(-40.7765619452973,25.4753766054114,20.));
#82825=CARTESIAN_POINT('Ctrl Pts',(-40.7563112193678,25.5020692967677,0.));
#82826=CARTESIAN_POINT('Ctrl Pts',(-40.7563112193678,25.5020692967677,20.));
#82827=CARTESIAN_POINT('Ctrl Pts',(-40.7360426477524,25.528747037476,0.));
#82828=CARTESIAN_POINT('Ctrl Pts',(-40.7360426477524,25.528747037476,20.));
#82829=CARTESIAN_POINT('Ctrl Pts',(-40.715756240903,25.5554098152083,0.));
#82830=CARTESIAN_POINT('Ctrl Pts',(-40.715756240903,25.5554098152083,20.));
#82831=CARTESIAN_POINT('Ctrl Pts',(-40.6954520092804,25.5820576176439,0.));
#82832=CARTESIAN_POINT('Ctrl Pts',(-40.6954520092804,25.5820576176439,20.));
#82833=CARTESIAN_POINT('Ctrl Pts',(-40.6751299633543,25.6086904324689,0.));
#82834=CARTESIAN_POINT('Ctrl Pts',(-40.6751299633543,25.6086904324689,20.));
#82835=CARTESIAN_POINT('Ctrl Pts',(-40.6547901136033,25.6353082473768,0.));
#82836=CARTESIAN_POINT('Ctrl Pts',(-40.6547901136033,25.6353082473768,20.));
#82837=CARTESIAN_POINT('Ctrl Pts',(-40.6344324705148,25.6619110500677,0.));
#82838=CARTESIAN_POINT('Ctrl Pts',(-40.6344324705148,25.6619110500677,20.));
#82839=CARTESIAN_POINT('Ctrl Pts',(-40.6140570445847,25.6884988282486,0.));
#82840=CARTESIAN_POINT('Ctrl Pts',(-40.6140570445847,25.6884988282486,20.));
#82841=CARTESIAN_POINT('Ctrl Pts',(-40.5936638463177,25.7150715696332,0.));
#82842=CARTESIAN_POINT('Ctrl Pts',(-40.5936638463177,25.7150715696332,20.));
#82843=CARTESIAN_POINT('Ctrl Pts',(-40.5732528862276,25.7416292619425,0.));
#82844=CARTESIAN_POINT('Ctrl Pts',(-40.5732528862276,25.7416292619425,20.));
#82845=CARTESIAN_POINT('Ctrl Pts',(-40.5528241748366,25.768171892904,0.));
#82846=CARTESIAN_POINT('Ctrl Pts',(-40.5528241748366,25.768171892904,20.));
#82847=CARTESIAN_POINT('Ctrl Pts',(-40.5323777226758,25.7946994502526,0.));
#82848=CARTESIAN_POINT('Ctrl Pts',(-40.5323777226758,25.7946994502526,20.));
#82849=CARTESIAN_POINT('Ctrl Pts',(-40.5119135402853,25.8212119217304,0.));
#82850=CARTESIAN_POINT('Ctrl Pts',(-40.5119135402853,25.8212119217304,20.));
#82851=CARTESIAN_POINT('Ctrl Pts',(-40.4914316382141,25.8477092950863,0.));
#82852=CARTESIAN_POINT('Ctrl Pts',(-40.4914316382141,25.8477092950863,20.));
#82853=CARTESIAN_POINT('Ctrl Pts',(-40.4709320270197,25.8741915580762,0.));
#82854=CARTESIAN_POINT('Ctrl Pts',(-40.4709320270197,25.8741915580762,20.));
#82855=CARTESIAN_POINT('Ctrl Pts',(-40.4504147172684,25.900658698463,0.));
#82856=CARTESIAN_POINT('Ctrl Pts',(-40.4504147172684,25.900658698463,20.));
#82857=CARTESIAN_POINT('Ctrl Pts',(-40.4298797195353,25.9271107040168,0.));
#82858=CARTESIAN_POINT('Ctrl Pts',(-40.4298797195353,25.9271107040168,20.));
#82859=CARTESIAN_POINT('Ctrl Pts',(-40.4093270444043,25.953547562515,0.));
#82860=CARTESIAN_POINT('Ctrl Pts',(-40.4093270444043,25.953547562515,20.));
#82861=CARTESIAN_POINT('Ctrl Pts',(-40.3887567024682,25.9799692617416,0.));
#82862=CARTESIAN_POINT('Ctrl Pts',(-40.3887567024682,25.9799692617416,20.));
#82863=CARTESIAN_POINT('Ctrl Pts',(-40.3681687043284,26.0063757894875,0.));
#82864=CARTESIAN_POINT('Ctrl Pts',(-40.3681687043284,26.0063757894875,20.));
#82865=CARTESIAN_POINT('Ctrl Pts',(-40.347563060595,26.0327671335511,0.));
#82866=CARTESIAN_POINT('Ctrl Pts',(-40.347563060595,26.0327671335511,20.));
#82867=CARTESIAN_POINT('Ctrl Pts',(-40.326939781887,26.0591432817373,0.));
#82868=CARTESIAN_POINT('Ctrl Pts',(-40.326939781887,26.0591432817373,20.));
#82869=CARTESIAN_POINT('Ctrl Pts',(-40.3062988788318,26.0855042218583,0.));
#82870=CARTESIAN_POINT('Ctrl Pts',(-40.3062988788318,26.0855042218583,20.));
#82871=CARTESIAN_POINT('Ctrl Pts',(-40.2856403620657,26.1118499417334,0.));
#82872=CARTESIAN_POINT('Ctrl Pts',(-40.2856403620657,26.1118499417334,20.));
#82873=CARTESIAN_POINT('Ctrl Pts',(-40.2649642422341,26.1381804291892,0.));
#82874=CARTESIAN_POINT('Ctrl Pts',(-40.2649642422341,26.1381804291892,20.));
#82875=CARTESIAN_POINT('Ctrl Pts',(-40.2442705299908,26.1644956720595,0.));
#82876=CARTESIAN_POINT('Ctrl Pts',(-40.2442705299908,26.1644956720595,20.));
#82877=CARTESIAN_POINT('Ctrl Pts',(-40.2235592359986,26.1907956581851,0.));
#82878=CARTESIAN_POINT('Ctrl Pts',(-40.2235592359986,26.1907956581851,20.));
#82879=CARTESIAN_POINT('Ctrl Pts',(-40.2028303709288,26.217080375414,0.));
#82880=CARTESIAN_POINT('Ctrl Pts',(-40.2028303709288,26.217080375414,20.));
#82881=CARTESIAN_POINT('Ctrl Pts',(-40.1820839454613,26.2433498116008,0.));
#82882=CARTESIAN_POINT('Ctrl Pts',(-40.1820839454613,26.2433498116008,20.));
#82883=CARTESIAN_POINT('Ctrl Pts',(-40.161319970285,26.2696039546074,0.));
#82884=CARTESIAN_POINT('Ctrl Pts',(-40.161319970285,26.2696039546074,20.));
#82885=CARTESIAN_POINT('Ctrl Pts',(-40.1405384560971,26.2958427923028,0.));
#82886=CARTESIAN_POINT('Ctrl Pts',(-40.1405384560971,26.2958427923028,20.));
#82887=CARTESIAN_POINT('Ctrl Pts',(-40.1197394136039,26.3220663125631,0.));
#82888=CARTESIAN_POINT('Ctrl Pts',(-40.1197394136039,26.3220663125631,20.));
#82889=CARTESIAN_POINT('Ctrl Pts',(-40.0989228535202,26.3482745032719,0.));
#82890=CARTESIAN_POINT('Ctrl Pts',(-40.0989228535202,26.3482745032719,20.));
#82891=CARTESIAN_POINT('Ctrl Pts',(-40.0780887865696,26.3744673523197,0.));
#82892=CARTESIAN_POINT('Ctrl Pts',(-40.0780887865696,26.3744673523197,20.));
#82893=CARTESIAN_POINT('Ctrl Pts',(-40.0572372234844,26.4006448476041,0.));
#82894=CARTESIAN_POINT('Ctrl Pts',(-40.0572372234844,26.4006448476041,20.));
#82895=CARTESIAN_POINT('Ctrl Pts',(-40.0363681750053,26.4268069770299,0.));
#82896=CARTESIAN_POINT('Ctrl Pts',(-40.0363681750053,26.4268069770299,20.));
#82897=CARTESIAN_POINT('Ctrl Pts',(-40.015481651882,26.4529537285089,0.));
#82898=CARTESIAN_POINT('Ctrl Pts',(-40.015481651882,26.4529537285089,20.));
#82899=CARTESIAN_POINT('Ctrl Pts',(-39.9945776648731,26.4790850899607,0.));
#82900=CARTESIAN_POINT('Ctrl Pts',(-39.9945776648731,26.4790850899607,20.));
#82901=CARTESIAN_POINT('Ctrl Pts',(-39.9736562247456,26.5052010493117,0.));
#82902=CARTESIAN_POINT('Ctrl Pts',(-39.9736562247456,26.5052010493117,20.));
#82903=CARTESIAN_POINT('Ctrl Pts',(-39.9527173422752,26.5313015944953,0.));
#82904=CARTESIAN_POINT('Ctrl Pts',(-39.9527173422752,26.5313015944953,20.));
#82905=CARTESIAN_POINT('Ctrl Pts',(-39.9317610282459,26.5573867134521,0.));
#82906=CARTESIAN_POINT('Ctrl Pts',(-39.9317610282459,26.5573867134521,20.));
#82907=CARTESIAN_POINT('Ctrl Pts',(-39.9107872934506,26.5834563941296,0.));
#82908=CARTESIAN_POINT('Ctrl Pts',(-39.9107872934506,26.5834563941296,20.));
#82909=CARTESIAN_POINT('Ctrl Pts',(-39.8897961486907,26.6095106244829,0.));
#82910=CARTESIAN_POINT('Ctrl Pts',(-39.8897961486907,26.6095106244829,20.));
#82911=CARTESIAN_POINT('Ctrl Pts',(-39.8687876047769,26.6355493924743,0.));
#82912=CARTESIAN_POINT('Ctrl Pts',(-39.8687876047769,26.6355493924743,20.));
#82913=CARTESIAN_POINT('Ctrl Pts',(-39.847761672528,26.6615726860734,0.));
#82914=CARTESIAN_POINT('Ctrl Pts',(-39.847761672528,26.6615726860734,20.));
#82915=CARTESIAN_POINT('Ctrl Pts',(-39.8267183627717,26.687580493257,0.));
#82916=CARTESIAN_POINT('Ctrl Pts',(-39.8267183627717,26.687580493257,20.));
#82917=CARTESIAN_POINT('Ctrl Pts',(-39.8056576863443,26.713572802009,0.));
#82918=CARTESIAN_POINT('Ctrl Pts',(-39.8056576863443,26.713572802009,20.));
#82919=CARTESIAN_POINT('Ctrl Pts',(-39.7845796540903,26.7395496003209,0.));
#82920=CARTESIAN_POINT('Ctrl Pts',(-39.7845796540903,26.7395496003209,20.));
#82921=CARTESIAN_POINT('Ctrl Pts',(-39.7634842768632,26.7655108761908,0.));
#82922=CARTESIAN_POINT('Ctrl Pts',(-39.7634842768632,26.7655108761908,20.));
#82923=CARTESIAN_POINT('Ctrl Pts',(-39.7423715655248,26.7914566176244,0.));
#82924=CARTESIAN_POINT('Ctrl Pts',(-39.7423715655248,26.7914566176244,20.));
#82925=CARTESIAN_POINT('Ctrl Pts',(-39.7212415309462,26.8173868126344,0.));
#82926=CARTESIAN_POINT('Ctrl Pts',(-39.7212415309462,26.8173868126344,20.));
#82927=CARTESIAN_POINT('Ctrl Pts',(-39.7000941840066,26.843301449241,0.));
#82928=CARTESIAN_POINT('Ctrl Pts',(-39.7000941840066,26.843301449241,20.));
#82929=CARTESIAN_POINT('Ctrl Pts',(-39.6789295355942,26.8692005154716,0.));
#82930=CARTESIAN_POINT('Ctrl Pts',(-39.6789295355942,26.8692005154716,20.));
#82931=CARTESIAN_POINT('Ctrl Pts',(-39.6577475966055,26.8950839993609,0.));
#82932=CARTESIAN_POINT('Ctrl Pts',(-39.6577475966055,26.8950839993609,20.));
#82933=CARTESIAN_POINT('Ctrl Pts',(-39.6365483779458,26.9209518889509,0.));
#82934=CARTESIAN_POINT('Ctrl Pts',(-39.6365483779458,26.9209518889509,20.));
#82935=CARTESIAN_POINT('Ctrl Pts',(-39.6153318905283,26.9468041722907,0.));
#82936=CARTESIAN_POINT('Ctrl Pts',(-39.6153318905283,26.9468041722907,20.));
#82937=CARTESIAN_POINT('Ctrl Pts',(-39.5940981452753,26.972640837437,0.));
#82938=CARTESIAN_POINT('Ctrl Pts',(-39.5940981452753,26.972640837437,20.));
#82939=CARTESIAN_POINT('Ctrl Pts',(-39.5728471531178,26.9984618724537,0.));
#82940=CARTESIAN_POINT('Ctrl Pts',(-39.5728471531178,26.9984618724537,20.));
#82941=CARTESIAN_POINT('Ctrl Pts',(-39.5515789249953,27.0242672654118,0.));
#82942=CARTESIAN_POINT('Ctrl Pts',(-39.5515789249953,27.0242672654118,20.));
#82943=CARTESIAN_POINT('Ctrl Pts',(-39.5302934718558,27.0500570043898,0.));
#82944=CARTESIAN_POINT('Ctrl Pts',(-39.5302934718558,27.0500570043898,20.));
#82945=CARTESIAN_POINT('Ctrl Pts',(-39.5089908046561,27.0758310774732,0.));
#82946=CARTESIAN_POINT('Ctrl Pts',(-39.5089908046561,27.0758310774732,20.));
#82947=CARTESIAN_POINT('Ctrl Pts',(-39.4876709343614,27.1015894727552,0.));
#82948=CARTESIAN_POINT('Ctrl Pts',(-39.4876709343614,27.1015894727552,20.));
#82949=CARTESIAN_POINT('Ctrl Pts',(-39.4663338719455,27.1273321783362,0.));
#82950=CARTESIAN_POINT('Ctrl Pts',(-39.4663338719455,27.1273321783362,20.));
#82951=CARTESIAN_POINT('Ctrl Pts',(-39.4449796283908,27.153059182324,0.));
#82952=CARTESIAN_POINT('Ctrl Pts',(-39.4449796283908,27.153059182324,20.));
#82953=CARTESIAN_POINT('Ctrl Pts',(-39.4236082146882,27.1787704728336,0.));
#82954=CARTESIAN_POINT('Ctrl Pts',(-39.4236082146882,27.1787704728336,20.));
#82955=CARTESIAN_POINT('Ctrl Pts',(-39.4022196418372,27.2044660379877,0.));
#82956=CARTESIAN_POINT('Ctrl Pts',(-39.4022196418372,27.2044660379877,20.));
#82957=CARTESIAN_POINT('Ctrl Pts',(-39.3808139208456,27.2301458659157,0.));
#82958=CARTESIAN_POINT('Ctrl Pts',(-39.3808139208456,27.2301458659157,20.));
#82959=CARTESIAN_POINT('Ctrl Pts',(-39.3593910627297,27.2558099447548,0.));
#82960=CARTESIAN_POINT('Ctrl Pts',(-39.3593910627297,27.2558099447548,20.));
#82961=CARTESIAN_POINT('Ctrl Pts',(-39.3379510785145,27.2814582626492,0.));
#82962=CARTESIAN_POINT('Ctrl Pts',(-39.3379510785145,27.2814582626492,20.));
#82963=CARTESIAN_POINT('Ctrl Pts',(-39.3164939792334,27.3070908077508,0.));
#82964=CARTESIAN_POINT('Ctrl Pts',(-39.3164939792334,27.3070908077508,20.));
#82965=CARTESIAN_POINT('Ctrl Pts',(-39.2950197759285,27.3327075682187,0.));
#82966=CARTESIAN_POINT('Ctrl Pts',(-39.2950197759285,27.3327075682187,20.));
#82967=CARTESIAN_POINT('Ctrl Pts',(-39.2735284796508,27.3583085322198,0.));
#82968=CARTESIAN_POINT('Ctrl Pts',(-39.2735284796508,27.3583085322198,20.));
#82969=CARTESIAN_POINT('Ctrl Pts',(-39.25202010146,27.3838936879286,0.));
#82970=CARTESIAN_POINT('Ctrl Pts',(-39.25202010146,27.3838936879286,20.));
#82971=CARTESIAN_POINT('Ctrl Pts',(-39.2304946524241,27.4094630235265,0.));
#82972=CARTESIAN_POINT('Ctrl Pts',(-39.2304946524241,27.4094630235265,20.));
#82973=CARTESIAN_POINT('Ctrl Pts',(-39.2089521436188,27.4350165272023,0.));
#82974=CARTESIAN_POINT('Ctrl Pts',(-39.2089521436188,27.4350165272023,20.));
#82975=CARTESIAN_POINT('Ctrl Pts',(-39.1873925861285,27.4605541871518,0.));
#82976=CARTESIAN_POINT('Ctrl Pts',(-39.1873925861285,27.4605541871518,20.));
#82977=CARTESIAN_POINT('Ctrl Pts',(-39.1658159910458,27.4860759915783,0.));
#82978=CARTESIAN_POINT('Ctrl Pts',(-39.1658159910458,27.4860759915783,20.));
#82979=CARTESIAN_POINT('Ctrl Pts',(-39.1442223694722,27.5115819286926,0.));
#82980=CARTESIAN_POINT('Ctrl Pts',(-39.1442223694722,27.5115819286926,20.));
#82981=CARTESIAN_POINT('Ctrl Pts',(-39.1226117325183,27.5370719867136,0.));
#82982=CARTESIAN_POINT('Ctrl Pts',(-39.1226117325183,27.5370719867136,20.));
#82983=CARTESIAN_POINT('Ctrl Pts',(-39.100984091303,27.5625461538675,0.));
#82984=CARTESIAN_POINT('Ctrl Pts',(-39.100984091303,27.5625461538675,20.));
#82985=CARTESIAN_POINT('Ctrl Pts',(-39.0793394569537,27.5880044183879,0.));
#82986=CARTESIAN_POINT('Ctrl Pts',(-39.0793394569537,27.5880044183879,20.));
#82987=CARTESIAN_POINT('Ctrl Pts',(-39.057677840606,27.6134467685155,0.));
#82988=CARTESIAN_POINT('Ctrl Pts',(-39.057677840606,27.6134467685155,20.));
#82989=CARTESIAN_POINT('Ctrl Pts',(-39.0359992534037,27.6388731924983,0.));
#82990=CARTESIAN_POINT('Ctrl Pts',(-39.0359992534037,27.6388731924983,20.));
#82991=CARTESIAN_POINT('Ctrl Pts',(-39.0143037064988,27.6642836785915,0.));
#82992=CARTESIAN_POINT('Ctrl Pts',(-39.0143037064988,27.6642836785915,20.));
#82993=CARTESIAN_POINT('Ctrl Pts',(-38.9925912110523,27.6896782150583,0.));
#82994=CARTESIAN_POINT('Ctrl Pts',(-38.9925912110523,27.6896782150583,20.));
#82995=CARTESIAN_POINT('Ctrl Pts',(-38.9708617782339,27.7150567901695,0.));
#82996=CARTESIAN_POINT('Ctrl Pts',(-38.9708617782339,27.7150567901695,20.));
#82997=CARTESIAN_POINT('Ctrl Pts',(-38.9491154192216,27.7404193922036,0.));
#82998=CARTESIAN_POINT('Ctrl Pts',(-38.9491154192216,27.7404193922036,20.));
#82999=CARTESIAN_POINT('Ctrl Pts',(-38.9273521452022,27.7657660094466,0.));
#83000=CARTESIAN_POINT('Ctrl Pts',(-38.9273521452022,27.7657660094466,20.));
#83001=CARTESIAN_POINT('Ctrl Pts',(-38.9055719673706,27.7910966301919,0.));
#83002=CARTESIAN_POINT('Ctrl Pts',(-38.9055719673706,27.7910966301919,20.));
#83003=CARTESIAN_POINT('Ctrl Pts',(-38.8837748969299,27.8164112427396,0.));
#83004=CARTESIAN_POINT('Ctrl Pts',(-38.8837748969299,27.8164112427396,20.));
#83005=CARTESIAN_POINT('Ctrl Pts',(-38.8619609450913,27.8417098353975,0.));
#83006=CARTESIAN_POINT('Ctrl Pts',(-38.8619609450913,27.8417098353975,20.));
#83007=CARTESIAN_POINT('Ctrl Pts',(-38.8401301230745,27.866992396481,0.));
#83008=CARTESIAN_POINT('Ctrl Pts',(-38.8401301230745,27.866992396481,20.));
#83009=CARTESIAN_POINT('Ctrl Pts',(-38.8182824421082,27.8922589143132,0.));
#83010=CARTESIAN_POINT('Ctrl Pts',(-38.8182824421082,27.8922589143132,20.));
#83011=CARTESIAN_POINT('Ctrl Pts',(-38.7964179134294,27.917509377225,0.));
#83012=CARTESIAN_POINT('Ctrl Pts',(-38.7964179134294,27.917509377225,20.));
#83013=CARTESIAN_POINT('Ctrl Pts',(-38.7745365482838,27.9427437735546,0.));
#83014=CARTESIAN_POINT('Ctrl Pts',(-38.7745365482838,27.9427437735546,20.));
#83015=CARTESIAN_POINT('Ctrl Pts',(-38.752638357925,27.9679620916479,0.));
#83016=CARTESIAN_POINT('Ctrl Pts',(-38.752638357925,27.9679620916479,20.));
#83017=CARTESIAN_POINT('Ctrl Pts',(-38.7307233536152,27.993164319858,0.));
#83018=CARTESIAN_POINT('Ctrl Pts',(-38.7307233536152,27.993164319858,20.));
#83019=CARTESIAN_POINT('Ctrl Pts',(-38.7087915466247,28.0183504465458,0.));
#83020=CARTESIAN_POINT('Ctrl Pts',(-38.7087915466247,28.0183504465458,20.));
#83021=CARTESIAN_POINT('Ctrl Pts',(-38.6868429482325,28.0435204600798,0.));
#83022=CARTESIAN_POINT('Ctrl Pts',(-38.6868429482325,28.0435204600798,20.));
#83023=CARTESIAN_POINT('Ctrl Pts',(-38.6648775697261,28.0686743488361,0.));
#83024=CARTESIAN_POINT('Ctrl Pts',(-38.6648775697261,28.0686743488361,20.));
#83025=CARTESIAN_POINT('Ctrl Pts',(-38.6428954224012,28.0938121011982,0.));
#83026=CARTESIAN_POINT('Ctrl Pts',(-38.6428954224012,28.0938121011982,20.));
#83027=CARTESIAN_POINT('Ctrl Pts',(-38.6208965175619,28.1189337055566,0.));
#83028=CARTESIAN_POINT('Ctrl Pts',(-38.6208965175619,28.1189337055566,20.));
#83029=CARTESIAN_POINT('Ctrl Pts',(-38.5988808665205,28.14403915031,0.));
#83030=CARTESIAN_POINT('Ctrl Pts',(-38.5988808665205,28.14403915031,20.));
#83031=CARTESIAN_POINT('Ctrl Pts',(-38.5768484805979,28.1691284238645,0.));
#83032=CARTESIAN_POINT('Ctrl Pts',(-38.5768484805979,28.1691284238645,20.));
#83033=CARTESIAN_POINT('Ctrl Pts',(-38.5547993711231,28.194201514634,0.));
#83034=CARTESIAN_POINT('Ctrl Pts',(-38.5547993711231,28.194201514634,20.));
#83035=CARTESIAN_POINT('Ctrl Pts',(-38.5327335494335,28.2192584110398,0.));
#83036=CARTESIAN_POINT('Ctrl Pts',(-38.5327335494335,28.2192584110398,20.));
#83037=CARTESIAN_POINT('Ctrl Pts',(-38.5106510268752,28.2442991015113,0.));
#83038=CARTESIAN_POINT('Ctrl Pts',(-38.5106510268752,28.2442991015113,20.));
#83039=CARTESIAN_POINT('Ctrl Pts',(-38.4885518148031,28.2693235744854,0.));
#83040=CARTESIAN_POINT('Ctrl Pts',(-38.4885518148031,28.2693235744854,20.));
#83041=CARTESIAN_POINT('Ctrl Pts',(-38.4664359245797,28.2943318184065,0.));
#83042=CARTESIAN_POINT('Ctrl Pts',(-38.4664359245797,28.2943318184065,20.));
#83043=CARTESIAN_POINT('Ctrl Pts',(-38.444303367576,28.3193238217266,0.));
#83044=CARTESIAN_POINT('Ctrl Pts',(-38.444303367576,28.3193238217266,20.));
#83045=CARTESIAN_POINT('Ctrl Pts',(-38.422154155171,28.3442995729049,0.));
#83046=CARTESIAN_POINT('Ctrl Pts',(-38.422154155171,28.3442995729049,20.));
#83047=CARTESIAN_POINT('Ctrl Pts',(-38.3999882987522,28.3692590604082,0.));
#83048=CARTESIAN_POINT('Ctrl Pts',(-38.3999882987522,28.3692590604082,20.));
#83049=CARTESIAN_POINT('Ctrl Pts',(-38.3778058097152,28.3942022727108,0.));
#83050=CARTESIAN_POINT('Ctrl Pts',(-38.3778058097152,28.3942022727108,20.));
#83051=CARTESIAN_POINT('Ctrl Pts',(-38.3556066994642,28.419129198295,0.));
#83052=CARTESIAN_POINT('Ctrl Pts',(-38.3556066994642,28.419129198295,20.));
#83053=CARTESIAN_POINT('Ctrl Pts',(-38.333390979412,28.4440398256512,0.));
#83054=CARTESIAN_POINT('Ctrl Pts',(-38.333390979412,28.4440398256512,20.));
#83055=CARTESIAN_POINT('Ctrl Pts',(-38.3111586609795,28.4689341432774,0.));
#83056=CARTESIAN_POINT('Ctrl Pts',(-38.3111586609795,28.4689341432774,20.));
#83057=CARTESIAN_POINT('Ctrl Pts',(-38.2889097555964,28.4938121396793,0.));
#83058=CARTESIAN_POINT('Ctrl Pts',(-38.2889097555964,28.4938121396793,20.));
#83059=CARTESIAN_POINT('Ctrl Pts',(-38.2666442747002,28.5186738033703,0.));
#83060=CARTESIAN_POINT('Ctrl Pts',(-38.2666442747002,28.5186738033703,20.));
#83061=CARTESIAN_POINT('Ctrl Pts',(-38.2443622297368,28.543519122871,0.));
#83062=CARTESIAN_POINT('Ctrl Pts',(-38.2443622297368,28.543519122871,20.));
#83063=CARTESIAN_POINT('Ctrl Pts',(-38.2220636321601,28.5683480867097,0.));
#83064=CARTESIAN_POINT('Ctrl Pts',(-38.2220636321601,28.5683480867097,20.));
#83065=CARTESIAN_POINT('Ctrl Pts',(-38.1997484934321,28.5931606834223,0.));
#83066=CARTESIAN_POINT('Ctrl Pts',(-38.1997484934321,28.5931606834223,20.));
#83067=CARTESIAN_POINT('Ctrl Pts',(-38.1774168250235,28.6179569015525,0.));
#83068=CARTESIAN_POINT('Ctrl Pts',(-38.1774168250235,28.6179569015525,20.));
#83069=CARTESIAN_POINT('Ctrl Pts',(-38.1550686384134,28.6427367296518,0.));
#83070=CARTESIAN_POINT('Ctrl Pts',(-38.1550686384134,28.6427367296518,20.));
#83071=CARTESIAN_POINT('Ctrl Pts',(-38.1327039450889,28.6675001562794,0.));
#83072=CARTESIAN_POINT('Ctrl Pts',(-38.1327039450889,28.6675001562794,20.));
#83073=CARTESIAN_POINT('Ctrl Pts',(-38.1103227565456,28.6922471700024,0.));
#83074=CARTESIAN_POINT('Ctrl Pts',(-38.1103227565456,28.6922471700024,20.));
#83075=CARTESIAN_POINT('Ctrl Pts',(-38.0879250842874,28.7169777593955,0.));
#83076=CARTESIAN_POINT('Ctrl Pts',(-38.0879250842874,28.7169777593955,20.));
#83077=CARTESIAN_POINT('Ctrl Pts',(-38.0655109398262,28.7416919130413,0.));
#83078=CARTESIAN_POINT('Ctrl Pts',(-38.0655109398262,28.7416919130413,20.));
#83079=CARTESIAN_POINT('Ctrl Pts',(-38.0430803346823,28.76638961953,0.));
#83080=CARTESIAN_POINT('Ctrl Pts',(-38.0430803346823,28.76638961953,20.));
#83081=CARTESIAN_POINT('Ctrl Pts',(-38.020633280384,28.7910708674595,0.));
#83082=CARTESIAN_POINT('Ctrl Pts',(-38.020633280384,28.7910708674595,20.));
#83083=CARTESIAN_POINT('Ctrl Pts',(-37.9981697884679,28.8157356454354,0.));
#83084=CARTESIAN_POINT('Ctrl Pts',(-37.9981697884679,28.8157356454354,20.));
#83085=CARTESIAN_POINT('Ctrl Pts',(-37.975689870479,28.8403839420709,0.));
#83086=CARTESIAN_POINT('Ctrl Pts',(-37.975689870479,28.8403839420709,20.));
#83087=CARTESIAN_POINT('Ctrl Pts',(-37.9531935379708,28.8650157459871,0.));
#83088=CARTESIAN_POINT('Ctrl Pts',(-37.9531935379708,28.8650157459871,20.));
#83089=CARTESIAN_POINT('Ctrl Pts',(-37.9306808025049,28.8896310458131,0.));
#83090=CARTESIAN_POINT('Ctrl Pts',(-37.9306808025049,28.8896310458131,20.));
#83091=CARTESIAN_POINT('Ctrl Pts',(-37.9081516756509,28.9142298301853,0.));
#83092=CARTESIAN_POINT('Ctrl Pts',(-37.9081516756509,28.9142298301853,20.));
#83093=CARTESIAN_POINT('Ctrl Pts',(-37.8856061689868,28.9388120877483,0.));
#83094=CARTESIAN_POINT('Ctrl Pts',(-37.8856061689868,28.9388120877483,20.));
#83095=CARTESIAN_POINT('Ctrl Pts',(-37.8630442940985,28.9633778071544,0.));
#83096=CARTESIAN_POINT('Ctrl Pts',(-37.8630442940985,28.9633778071544,20.));
#83097=CARTESIAN_POINT('Ctrl Pts',(-37.8404660625803,28.9879269770637,0.));
#83098=CARTESIAN_POINT('Ctrl Pts',(-37.8404660625803,28.9879269770637,20.));
#83099=CARTESIAN_POINT('Ctrl Pts',(-37.8178714860345,29.0124595861441,0.));
#83100=CARTESIAN_POINT('Ctrl Pts',(-37.8178714860345,29.0124595861441,20.));
#83101=CARTESIAN_POINT('Ctrl Pts',(-37.7952605760716,29.0369756230713,0.));
#83102=CARTESIAN_POINT('Ctrl Pts',(-37.7952605760716,29.0369756230713,20.));
#83103=CARTESIAN_POINT('Ctrl Pts',(-37.7726333443105,29.0614750765285,0.));
#83104=CARTESIAN_POINT('Ctrl Pts',(-37.7726333443105,29.0614750765285,20.));
#83105=CARTESIAN_POINT('Ctrl Pts',(-37.7499898023785,29.0859579352069,0.));
#83106=CARTESIAN_POINT('Ctrl Pts',(-37.7499898023785,29.0859579352069,20.));
#83107=CARTESIAN_POINT('Ctrl Pts',(-37.7273299619109,29.1104241878056,0.));
#83108=CARTESIAN_POINT('Ctrl Pts',(-37.7273299619109,29.1104241878056,20.));
#83109=CARTESIAN_POINT('Ctrl Pts',(-37.7046538345516,29.1348738230316,0.));
#83110=CARTESIAN_POINT('Ctrl Pts',(-37.7046538345516,29.1348738230316,20.));
#83111=CARTESIAN_POINT('Ctrl Pts',(-37.6819614319523,29.1593068295997,0.));
#83112=CARTESIAN_POINT('Ctrl Pts',(-37.6819614319523,29.1593068295997,20.));
#83113=CARTESIAN_POINT('Ctrl Pts',(-37.6592527657727,29.1837231962328,0.));
#83114=CARTESIAN_POINT('Ctrl Pts',(-37.6592527657727,29.1837231962328,20.));
#83115=CARTESIAN_POINT('Ctrl Pts',(-37.6365278476807,29.208122911661,0.));
#83116=CARTESIAN_POINT('Ctrl Pts',(-37.6365278476807,29.208122911661,20.));
#83117=CARTESIAN_POINT('Ctrl Pts',(-37.613786689352,29.2325059646224,0.));
#83118=CARTESIAN_POINT('Ctrl Pts',(-37.613786689352,29.2325059646224,20.));
#83119=CARTESIAN_POINT('Ctrl Pts',(-37.5910293024705,29.2568723438631,0.));
#83120=CARTESIAN_POINT('Ctrl Pts',(-37.5910293024705,29.2568723438631,20.));
#83121=CARTESIAN_POINT('Ctrl Pts',(-37.5682556987287,29.2812220381372,0.));
#83122=CARTESIAN_POINT('Ctrl Pts',(-37.5682556987287,29.2812220381372,20.));
#83123=CARTESIAN_POINT('Ctrl Pts',(-37.5454658898274,29.3055550362067,0.));
#83124=CARTESIAN_POINT('Ctrl Pts',(-37.5454658898274,29.3055550362067,20.));
#83125=CARTESIAN_POINT('Ctrl Pts',(-37.5226598874754,29.3298713268414,0.));
#83126=CARTESIAN_POINT('Ctrl Pts',(-37.5226598874754,29.3298713268414,20.));
#83127=CARTESIAN_POINT('Ctrl Pts',(-37.4998377033899,29.3541708988191,0.));
#83128=CARTESIAN_POINT('Ctrl Pts',(-37.4998377033899,29.3541708988191,20.));
#83129=CARTESIAN_POINT('Ctrl Pts',(-37.4769993492958,29.378453740925,0.));
#83130=CARTESIAN_POINT('Ctrl Pts',(-37.4769993492958,29.378453740925,20.));
#83131=CARTESIAN_POINT('Ctrl Pts',(-37.4541448369259,29.4027198419524,0.));
#83132=CARTESIAN_POINT('Ctrl Pts',(-37.4541448369259,29.4027198419524,20.));
#83133=CARTESIAN_POINT('Ctrl Pts',(-37.4312741780213,29.4269691907023,0.));
#83134=CARTESIAN_POINT('Ctrl Pts',(-37.4312741780213,29.4269691907023,20.));
#83135=CARTESIAN_POINT('Ctrl Pts',(-37.4083873843313,29.4512017759842,0.));
#83136=CARTESIAN_POINT('Ctrl Pts',(-37.4083873843313,29.4512017759842,20.));
#83137=CARTESIAN_POINT('Ctrl Pts',(-37.3854844676135,29.4754175866156,0.));
#83138=CARTESIAN_POINT('Ctrl Pts',(-37.3854844676135,29.4754175866156,20.));
#83139=CARTESIAN_POINT('Ctrl Pts',(-37.3625654396335,29.4996166114217,0.));
#83140=CARTESIAN_POINT('Ctrl Pts',(-37.3625654396335,29.4996166114217,20.));
#83141=CARTESIAN_POINT('Ctrl Pts',(-37.3396303121646,29.5237988392353,0.));
#83142=CARTESIAN_POINT('Ctrl Pts',(-37.3396303121646,29.5237988392353,20.));
#83143=CARTESIAN_POINT('Ctrl Pts',(-37.3166790969884,29.5479642588972,0.));
#83144=CARTESIAN_POINT('Ctrl Pts',(-37.3166790969884,29.5479642588972,20.));
#83145=CARTESIAN_POINT('Ctrl Pts',(-37.2937118058947,29.5721128592559,0.));
#83146=CARTESIAN_POINT('Ctrl Pts',(-37.2937118058947,29.5721128592559,20.));
#83147=CARTESIAN_POINT('Ctrl Pts',(-37.2707284506814,29.5962446291682,0.));
#83148=CARTESIAN_POINT('Ctrl Pts',(-37.2707284506814,29.5962446291682,20.));
#83149=CARTESIAN_POINT('Ctrl Pts',(-37.2477290431548,29.6203595574991,0.));
#83150=CARTESIAN_POINT('Ctrl Pts',(-37.2477290431548,29.6203595574991,20.));
#83151=CARTESIAN_POINT('Ctrl Pts',(-37.2247135951292,29.6444576331214,0.));
#83152=CARTESIAN_POINT('Ctrl Pts',(-37.2247135951292,29.6444576331214,20.));
#83153=CARTESIAN_POINT('Ctrl Pts',(-37.2016821184267,29.668538844916,0.));
#83154=CARTESIAN_POINT('Ctrl Pts',(-37.2016821184267,29.668538844916,20.));
#83155=CARTESIAN_POINT('Ctrl Pts',(-37.1786346248774,29.6926031817715,0.));
#83156=CARTESIAN_POINT('Ctrl Pts',(-37.1786346248774,29.6926031817715,20.));
#83157=CARTESIAN_POINT('Ctrl Pts',(-37.155571126319,29.7166506325841,0.));
#83158=CARTESIAN_POINT('Ctrl Pts',(-37.155571126319,29.7166506325841,20.));
#83159=CARTESIAN_POINT('Ctrl Pts',(-37.1324916345976,29.7406811862582,0.));
#83160=CARTESIAN_POINT('Ctrl Pts',(-37.1324916345976,29.7406811862582,20.));
#83161=CARTESIAN_POINT('Ctrl Pts',(-37.1093961615672,29.7646948317061,0.));
#83162=CARTESIAN_POINT('Ctrl Pts',(-37.1093961615672,29.7646948317061,20.));
#83163=CARTESIAN_POINT('Ctrl Pts',(-37.0862847190902,29.7886915578485,0.));
#83164=CARTESIAN_POINT('Ctrl Pts',(-37.0862847190902,29.7886915578485,20.));
#83165=CARTESIAN_POINT('Ctrl Pts',(-37.0631573190374,29.8126713536142,0.));
#83166=CARTESIAN_POINT('Ctrl Pts',(-37.0631573190374,29.8126713536142,20.));
#83167=CARTESIAN_POINT('Ctrl Pts',(-37.0400139732874,29.83663420794,0.));
#83168=CARTESIAN_POINT('Ctrl Pts',(-37.0400139732874,29.83663420794,20.));
#83169=CARTESIAN_POINT('Ctrl Pts',(-37.0168546937273,29.8605801097708,0.));
#83170=CARTESIAN_POINT('Ctrl Pts',(-37.0168546937273,29.8605801097708,20.));
#83171=CARTESIAN_POINT('Ctrl Pts',(-36.9936794922513,29.884509048059,0.));
#83172=CARTESIAN_POINT('Ctrl Pts',(-36.9936794922513,29.884509048059,20.));
#83173=CARTESIAN_POINT('Ctrl Pts',(-36.9704883807614,29.9084210117647,0.));
#83174=CARTESIAN_POINT('Ctrl Pts',(-36.9704883807614,29.9084210117647,20.));
#83175=CARTESIAN_POINT('Ctrl Pts',(-36.9472813711676,29.9323159898562,0.));
#83176=CARTESIAN_POINT('Ctrl Pts',(-36.9472813711676,29.9323159898562,20.));
#83177=CARTESIAN_POINT('Ctrl Pts',(-36.9240584753883,29.9561939713102,0.));
#83178=CARTESIAN_POINT('Ctrl Pts',(-36.9240584753883,29.9561939713102,20.));
#83179=CARTESIAN_POINT('Ctrl Pts',(-36.9008197053507,29.9800549451122,0.));
#83180=CARTESIAN_POINT('Ctrl Pts',(-36.9008197053507,29.9800549451122,20.));
#83181=CARTESIAN_POINT('Ctrl Pts',(-36.8775650729895,30.0038989002549,0.));
#83182=CARTESIAN_POINT('Ctrl Pts',(-36.8775650729895,30.0038989002549,20.));
#83183=CARTESIAN_POINT('Ctrl Pts',(-36.8542945902473,30.0277258257393,0.));
#83184=CARTESIAN_POINT('Ctrl Pts',(-36.8542945902473,30.0277258257393,20.));
#83185=CARTESIAN_POINT('Ctrl Pts',(-36.8310082690741,30.0515357105739,0.));
#83186=CARTESIAN_POINT('Ctrl Pts',(-36.8310082690741,30.0515357105739,20.));
#83187=CARTESIAN_POINT('Ctrl Pts',(-36.8077061214283,30.0753285437754,0.));
#83188=CARTESIAN_POINT('Ctrl Pts',(-36.8077061214283,30.0753285437754,20.));
#83189=CARTESIAN_POINT('Ctrl Pts',(-36.784388159276,30.0991043143684,0.));
#83190=CARTESIAN_POINT('Ctrl Pts',(-36.784388159276,30.0991043143684,20.));
#83191=CARTESIAN_POINT('Ctrl Pts',(-36.7610543945915,30.1228630113862,0.));
#83192=CARTESIAN_POINT('Ctrl Pts',(-36.7610543945915,30.1228630113862,20.));
#83193=CARTESIAN_POINT('Ctrl Pts',(-36.7377048393574,30.14660462387,0.));
#83194=CARTESIAN_POINT('Ctrl Pts',(-36.7377048393574,30.14660462387,20.));
#83195=CARTESIAN_POINT('Ctrl Pts',(-36.7143395055641,30.1703291408693,0.));
#83196=CARTESIAN_POINT('Ctrl Pts',(-36.7143395055641,30.1703291408693,20.));
#83197=CARTESIAN_POINT('Ctrl Pts',(-36.6909584052099,30.1940365514414,0.));
#83198=CARTESIAN_POINT('Ctrl Pts',(-36.6909584052099,30.1940365514414,20.));
#83199=CARTESIAN_POINT('Ctrl Pts',(-36.6675615503012,30.2177268446518,0.));
#83200=CARTESIAN_POINT('Ctrl Pts',(-36.6675615503012,30.2177268446518,20.));
#83201=CARTESIAN_POINT('Ctrl Pts',(-36.6441489528521,30.2414000095742,0.));
#83202=CARTESIAN_POINT('Ctrl Pts',(-36.6441489528521,30.2414000095742,20.));
#83203=CARTESIAN_POINT('Ctrl Pts',(-36.6207206248849,30.2650560352902,0.));
#83204=CARTESIAN_POINT('Ctrl Pts',(-36.6207206248849,30.2650560352902,20.));
#83205=CARTESIAN_POINT('Ctrl Pts',(-36.5972765784293,30.2886949108895,0.));
#83206=CARTESIAN_POINT('Ctrl Pts',(-36.5972765784293,30.2886949108895,20.));
#83207=CARTESIAN_POINT('Ctrl Pts',(-36.5738168255233,30.3123166254701,0.));
#83208=CARTESIAN_POINT('Ctrl Pts',(-36.5738168255233,30.3123166254701,20.));
#83209=CARTESIAN_POINT('Ctrl Pts',(-36.5503413782123,30.3359211681375,0.));
#83210=CARTESIAN_POINT('Ctrl Pts',(-36.5503413782123,30.3359211681375,20.));
#83211=CARTESIAN_POINT('Ctrl Pts',(-36.5268502485502,30.3595085280058,0.));
#83212=CARTESIAN_POINT('Ctrl Pts',(-36.5268502485502,30.3595085280058,20.));
#83213=CARTESIAN_POINT('Ctrl Pts',(-36.5033434485984,30.3830786941972,0.));
#83214=CARTESIAN_POINT('Ctrl Pts',(-36.5033434485984,30.3830786941972,20.));
#83215=CARTESIAN_POINT('Ctrl Pts',(-36.4798209904267,30.4066316558423,0.));
#83216=CARTESIAN_POINT('Ctrl Pts',(-36.4798209904267,30.4066316558423,20.));
#83217=CARTESIAN_POINT('Ctrl Pts',(-36.456282886113,30.4301674020801,0.));
#83218=CARTESIAN_POINT('Ctrl Pts',(-36.456282886113,30.4301674020801,20.));
#83219=CARTESIAN_POINT('Ctrl Pts',(-36.4327291477429,30.4536859220576,0.));
#83220=CARTESIAN_POINT('Ctrl Pts',(-36.4327291477429,30.4536859220576,20.));
#83221=CARTESIAN_POINT('Ctrl Pts',(-36.4091597874097,30.4771872049298,0.));
#83222=CARTESIAN_POINT('Ctrl Pts',(-36.4091597874097,30.4771872049298,20.));
#83223=CARTESIAN_POINT('Ctrl Pts',(-36.3855748172148,30.5006712398601,0.));
#83224=CARTESIAN_POINT('Ctrl Pts',(-36.3855748172148,30.5006712398601,20.));
#83225=CARTESIAN_POINT('Ctrl Pts',(-36.3619742492671,30.5241380160195,0.));
#83226=CARTESIAN_POINT('Ctrl Pts',(-36.3619742492671,30.5241380160195,20.));
#83227=CARTESIAN_POINT('Ctrl Pts',(-36.3383580956833,30.5475875225872,0.));
#83228=CARTESIAN_POINT('Ctrl Pts',(-36.3383580956833,30.5475875225872,20.));
#83229=CARTESIAN_POINT('Ctrl Pts',(-36.3147263685875,30.5710197487502,0.));
#83230=CARTESIAN_POINT('Ctrl Pts',(-36.3147263685875,30.5710197487502,20.));
#83231=CARTESIAN_POINT('Ctrl Pts',(-36.2910790801119,30.5944346837039,0.));
#83232=CARTESIAN_POINT('Ctrl Pts',(-36.2910790801119,30.5944346837039,20.));
#83233=CARTESIAN_POINT('Ctrl Pts',(-36.2674162423973,30.6178323166527,0.));
#83234=CARTESIAN_POINT('Ctrl Pts',(-36.2674162423973,30.6178323166527,20.));
#83235=CARTESIAN_POINT('Ctrl Pts',(-36.2437378675924,30.6412126368094,0.));
#83236=CARTESIAN_POINT('Ctrl Pts',(-36.2437378675924,30.6412126368094,20.));
#83237=CARTESIAN_POINT('Ctrl Pts',(-36.2200439678543,30.6645756333954,0.));
#83238=CARTESIAN_POINT('Ctrl Pts',(-36.2200439678543,30.6645756333954,20.));
#83239=CARTESIAN_POINT('Ctrl Pts',(-36.1963345553471,30.6879212956391,0.));
#83240=CARTESIAN_POINT('Ctrl Pts',(-36.1963345553471,30.6879212956391,20.));
#83241=CARTESIAN_POINT('Ctrl Pts',(-36.1726096422428,30.7112496127774,0.));
#83242=CARTESIAN_POINT('Ctrl Pts',(-36.1726096422428,30.7112496127774,20.));
#83243=CARTESIAN_POINT('Ctrl Pts',(-36.1488692407204,30.7345605740544,0.));
#83244=CARTESIAN_POINT('Ctrl Pts',(-36.1488692407204,30.7345605740544,20.));
#83245=CARTESIAN_POINT('Ctrl Pts',(-36.125113362967,30.7578541687236,0.));
#83246=CARTESIAN_POINT('Ctrl Pts',(-36.125113362967,30.7578541687236,20.));
#83247=CARTESIAN_POINT('Ctrl Pts',(-36.1013420211777,30.7811303860468,0.));
#83248=CARTESIAN_POINT('Ctrl Pts',(-36.1013420211777,30.7811303860468,20.));
#83249=CARTESIAN_POINT('Ctrl Pts',(-36.0775552275565,30.8043892152943,0.));
#83250=CARTESIAN_POINT('Ctrl Pts',(-36.0775552275565,30.8043892152943,20.));
#83251=CARTESIAN_POINT('Ctrl Pts',(-36.0537529943146,30.8276306457446,0.));
#83252=CARTESIAN_POINT('Ctrl Pts',(-36.0537529943146,30.8276306457446,20.));
#83253=CARTESIAN_POINT('Ctrl Pts',(-36.0299353336712,30.8508546666841,0.));
#83254=CARTESIAN_POINT('Ctrl Pts',(-36.0299353336712,30.8508546666841,20.));
#83255=CARTESIAN_POINT('Ctrl Pts',(-36.0061022578528,30.8740612674075,0.));
#83256=CARTESIAN_POINT('Ctrl Pts',(-36.0061022578528,30.8740612674075,20.));
#83257=CARTESIAN_POINT('Ctrl Pts',(-35.9822537790931,30.8972504372171,0.));
#83258=CARTESIAN_POINT('Ctrl Pts',(-35.9822537790931,30.8972504372171,20.));
#83259=CARTESIAN_POINT('Ctrl Pts',(-35.9583899096339,30.9204221654236,0.));
#83260=CARTESIAN_POINT('Ctrl Pts',(-35.9583899096339,30.9204221654236,20.));
#83261=CARTESIAN_POINT('Ctrl Pts',(-35.9345106617251,30.9435764413467,0.));
#83262=CARTESIAN_POINT('Ctrl Pts',(-35.9345106617251,30.9435764413467,20.));
#83263=CARTESIAN_POINT('Ctrl Pts',(-35.9106160476245,30.9667132543142,0.));
#83264=CARTESIAN_POINT('Ctrl Pts',(-35.9106160476245,30.9667132543142,20.));
#83265=CARTESIAN_POINT('Ctrl Pts',(-35.886706079598,30.9898325936627,0.));
#83266=CARTESIAN_POINT('Ctrl Pts',(-35.886706079598,30.9898325936627,20.));
#83267=CARTESIAN_POINT('Ctrl Pts',(-35.8627807699193,31.0129344487367,0.));
#83268=CARTESIAN_POINT('Ctrl Pts',(-35.8627807699193,31.0129344487367,20.));
#83269=CARTESIAN_POINT('Ctrl Pts',(-35.8388401308696,31.036018808889,0.));
#83270=CARTESIAN_POINT('Ctrl Pts',(-35.8388401308696,31.036018808889,20.));
#83271=CARTESIAN_POINT('Ctrl Pts',(-35.8148841747376,31.0590856634804,0.));
#83272=CARTESIAN_POINT('Ctrl Pts',(-35.8148841747376,31.0590856634804,20.));
#83273=CARTESIAN_POINT('Ctrl Pts',(-35.7909129138202,31.0821350018809,0.));
#83274=CARTESIAN_POINT('Ctrl Pts',(-35.7909129138202,31.0821350018809,20.));
#83275=CARTESIAN_POINT('Ctrl Pts',(-35.7669263604212,31.1051668134678,0.));
#83276=CARTESIAN_POINT('Ctrl Pts',(-35.7669263604212,31.1051668134678,20.));
#83277=CARTESIAN_POINT('Ctrl Pts',(-35.7429245268523,31.1281810876267,0.));
#83278=CARTESIAN_POINT('Ctrl Pts',(-35.7429245268523,31.1281810876267,20.));
#83279=CARTESIAN_POINT('Ctrl Pts',(-35.7189074254331,31.1511778137516,0.));
#83280=CARTESIAN_POINT('Ctrl Pts',(-35.7189074254331,31.1511778137516,20.));
#83281=CARTESIAN_POINT('Ctrl Pts',(-35.6948750684911,31.1741569812451,0.));
#83282=CARTESIAN_POINT('Ctrl Pts',(-35.6948750684911,31.1741569812451,20.));
#83283=CARTESIAN_POINT('Ctrl Pts',(-35.6708274683619,31.1971185795181,0.));
#83284=CARTESIAN_POINT('Ctrl Pts',(-35.6708274683619,31.1971185795181,20.));
#83285=CARTESIAN_POINT('Ctrl Pts',(-35.6467646373884,31.2200625979904,0.));
#83286=CARTESIAN_POINT('Ctrl Pts',(-35.6467646373884,31.2200625979904,20.));
#83287=CARTESIAN_POINT('Ctrl Pts',(-35.6226865879214,31.24298902609,0.));
#83288=CARTESIAN_POINT('Ctrl Pts',(-35.6226865879214,31.24298902609,20.));
#83289=CARTESIAN_POINT('Ctrl Pts',(-35.5985933323195,31.2658978532533,0.));
#83290=CARTESIAN_POINT('Ctrl Pts',(-35.5985933323195,31.2658978532533,20.));
#83291=CARTESIAN_POINT('Ctrl Pts',(-35.5744848829488,31.288789068925,0.));
#83292=CARTESIAN_POINT('Ctrl Pts',(-35.5744848829488,31.288789068925,20.));
#83293=CARTESIAN_POINT('Ctrl Pts',(-35.5503612521832,31.3116626625581,0.));
#83294=CARTESIAN_POINT('Ctrl Pts',(-35.5503612521832,31.3116626625581,20.));
#83295=CARTESIAN_POINT('Ctrl Pts',(-35.5262224524039,31.3345186236135,0.));
#83296=CARTESIAN_POINT('Ctrl Pts',(-35.5262224524039,31.3345186236135,20.));
#83297=CARTESIAN_POINT('Ctrl Pts',(-35.502068496,31.3573569415605,0.));
#83298=CARTESIAN_POINT('Ctrl Pts',(-35.502068496,31.3573569415605,20.));
#83299=CARTESIAN_POINT('Ctrl Pts',(-35.4778993953681,31.3801776058767,0.));
#83300=CARTESIAN_POINT('Ctrl Pts',(-35.4778993953681,31.3801776058767,20.));
#83301=CARTESIAN_POINT('Ctrl Pts',(-35.4537151629127,31.4029806060482,0.));
#83302=CARTESIAN_POINT('Ctrl Pts',(-35.4537151629127,31.4029806060482,20.));
#83303=CARTESIAN_POINT('Ctrl Pts',(-35.4295158110455,31.4257659315696,0.));
#83304=CARTESIAN_POINT('Ctrl Pts',(-35.4295158110455,31.4257659315696,20.));
#83305=CARTESIAN_POINT('Ctrl Pts',(-35.4053013521866,31.4485335719446,0.));
#83306=CARTESIAN_POINT('Ctrl Pts',(-35.4053013521866,31.4485335719446,20.));
#83307=CARTESIAN_POINT('Ctrl Pts',(-35.3810717987641,31.4712835166857,0.));
#83308=CARTESIAN_POINT('Ctrl Pts',(-35.3810717987641,31.4712835166857,20.));
#83309=CARTESIAN_POINT('Ctrl Pts',(-35.3568271632136,31.4940157553136,0.));
#83310=CARTESIAN_POINT('Ctrl Pts',(-35.3568271632136,31.4940157553136,20.));
#83311=CARTESIAN_POINT('Ctrl Pts',(-35.3325674579779,31.5167302773569,0.));
#83312=CARTESIAN_POINT('Ctrl Pts',(-35.3325674579779,31.5167302773569,20.));
#83313=CARTESIAN_POINT('Ctrl Pts',(-35.3082926955072,31.5394270723526,0.));
#83314=CARTESIAN_POINT('Ctrl Pts',(-35.3082926955072,31.5394270723526,20.));
#83315=CARTESIAN_POINT('Ctrl Pts',(-35.2840028882593,31.5621061298453,0.));
#83316=CARTESIAN_POINT('Ctrl Pts',(-35.2840028882593,31.5621061298453,20.));
#83317=CARTESIAN_POINT('Ctrl Pts',(-35.2596980486997,31.5847674393884,0.));
#83318=CARTESIAN_POINT('Ctrl Pts',(-35.2596980486997,31.5847674393884,20.));
#83319=CARTESIAN_POINT('Ctrl Pts',(-35.2353781893015,31.6074109905439,0.));
#83320=CARTESIAN_POINT('Ctrl Pts',(-35.2353781893015,31.6074109905439,20.));
#83321=CARTESIAN_POINT('Ctrl Pts',(-35.2110433225459,31.6300367728826,0.));
#83322=CARTESIAN_POINT('Ctrl Pts',(-35.2110433225459,31.6300367728826,20.));
#83323=CARTESIAN_POINT('Ctrl Pts',(-35.1866934609214,31.6526447759839,0.));
#83324=CARTESIAN_POINT('Ctrl Pts',(-35.1866934609214,31.6526447759839,20.));
#83325=CARTESIAN_POINT('Ctrl Pts',(-35.1623286169245,31.6752349894358,0.));
#83326=CARTESIAN_POINT('Ctrl Pts',(-35.1623286169245,31.6752349894358,20.));
#83327=CARTESIAN_POINT('Ctrl Pts',(-35.1379488030591,31.6978074028349,0.));
#83328=CARTESIAN_POINT('Ctrl Pts',(-35.1379488030591,31.6978074028349,20.));
#83329=CARTESIAN_POINT('Ctrl Pts',(-35.1135540318367,31.7203620057864,0.));
#83330=CARTESIAN_POINT('Ctrl Pts',(-35.1135540318367,31.7203620057864,20.));
#83331=CARTESIAN_POINT('Ctrl Pts',(-35.0891443157764,31.7428987879034,0.));
#83332=CARTESIAN_POINT('Ctrl Pts',(-35.0891443157764,31.7428987879034,20.));
#83333=CARTESIAN_POINT('Ctrl Pts',(-35.0647196674044,31.7654177388073,0.));
#83334=CARTESIAN_POINT('Ctrl Pts',(-35.0647196674044,31.7654177388073,20.));
#83335=CARTESIAN_POINT('Ctrl Pts',(-35.0402800992547,31.7879188481277,0.));
#83336=CARTESIAN_POINT('Ctrl Pts',(-35.0402800992547,31.7879188481277,20.));
#83337=CARTESIAN_POINT('Ctrl Pts',(-35.0158256238691,31.8104021055032,0.));
#83338=CARTESIAN_POINT('Ctrl Pts',(-35.0158256238691,31.8104021055032,20.));
#83339=CARTESIAN_POINT('Ctrl Pts',(-34.991356253797,31.8328675005809,0.));
#83340=CARTESIAN_POINT('Ctrl Pts',(-34.991356253797,31.8328675005809,20.));
#83341=CARTESIAN_POINT('Ctrl Pts',(-34.9668720015954,31.8553150230168,0.));
#83342=CARTESIAN_POINT('Ctrl Pts',(-34.9668720015954,31.8553150230168,20.));
#83343=CARTESIAN_POINT('Ctrl Pts',(-34.9423728798289,31.8777446624754,0.));
#83344=CARTESIAN_POINT('Ctrl Pts',(-34.9423728798289,31.8777446624754,20.));
#83345=CARTESIAN_POINT('Ctrl Pts',(-34.9178589010694,31.9001564086295,0.));
#83346=CARTESIAN_POINT('Ctrl Pts',(-34.9178589010694,31.9001564086295,20.));
#83347=CARTESIAN_POINT('Ctrl Pts',(-34.8933300778963,31.9225502511603,0.));
#83348=CARTESIAN_POINT('Ctrl Pts',(-34.8933300778963,31.9225502511603,20.));
#83349=CARTESIAN_POINT('Ctrl Pts',(-34.8687864228965,31.9449261797574,0.));
#83350=CARTESIAN_POINT('Ctrl Pts',(-34.8687864228965,31.9449261797574,20.));
#83351=CARTESIAN_POINT('Ctrl Pts',(-34.8442279486644,31.967284184119,0.));
#83352=CARTESIAN_POINT('Ctrl Pts',(-34.8442279486644,31.967284184119,20.));
#83353=CARTESIAN_POINT('Ctrl Pts',(-34.8196546678026,31.9896242539524,0.));
#83354=CARTESIAN_POINT('Ctrl Pts',(-34.8196546678026,31.9896242539524,20.));
#83355=CARTESIAN_POINT('Ctrl Pts',(-34.7950665929206,32.0119463789729,0.));
#83356=CARTESIAN_POINT('Ctrl Pts',(-34.7950665929206,32.0119463789729,20.));
#83357=CARTESIAN_POINT('Ctrl Pts',(-34.7704637366357,32.0342505489048,0.));
#83358=CARTESIAN_POINT('Ctrl Pts',(-34.7704637366357,32.0342505489048,20.));
#83359=CARTESIAN_POINT('Ctrl Pts',(-34.7458461115727,32.0565367534806,0.));
#83360=CARTESIAN_POINT('Ctrl Pts',(-34.7458461115727,32.0565367534806,20.));
#83361=CARTESIAN_POINT('Ctrl Pts',(-34.7212137303638,32.0788049824416,0.));
#83362=CARTESIAN_POINT('Ctrl Pts',(-34.7212137303638,32.0788049824416,20.));
#83363=CARTESIAN_POINT('Ctrl Pts',(-34.6965666056491,32.1010552255378,0.));
#83364=CARTESIAN_POINT('Ctrl Pts',(-34.6965666056491,32.1010552255378,20.));
#83365=CARTESIAN_POINT('Ctrl Pts',(-34.6719047500757,32.1232874725276,0.));
#83366=CARTESIAN_POINT('Ctrl Pts',(-34.6719047500757,32.1232874725276,20.));
#83367=CARTESIAN_POINT('Ctrl Pts',(-34.6472281762982,32.145501713178,0.));
#83368=CARTESIAN_POINT('Ctrl Pts',(-34.6472281762982,32.145501713178,20.));
#83369=CARTESIAN_POINT('Ctrl Pts',(-34.6225368969784,32.167697937264,0.));
#83370=CARTESIAN_POINT('Ctrl Pts',(-34.6225368969784,32.167697937264,20.));
#83371=CARTESIAN_POINT('Ctrl Pts',(-34.5978309247855,32.1898761345694,0.));
#83372=CARTESIAN_POINT('Ctrl Pts',(-34.5978309247855,32.1898761345694,20.));
#83373=CARTESIAN_POINT('Ctrl Pts',(-34.5731102723969,32.212036294887,0.));
#83374=CARTESIAN_POINT('Ctrl Pts',(-34.5731102723969,32.212036294887,20.));
#83375=CARTESIAN_POINT('Ctrl Pts',(-34.5483749524972,32.2341784080183,0.));
#83376=CARTESIAN_POINT('Ctrl Pts',(-34.5483749524972,32.2341784080183,20.));
#83377=CARTESIAN_POINT('Ctrl Pts',(-34.5236249777791,32.2563024637739,0.));
#83378=CARTESIAN_POINT('Ctrl Pts',(-34.5236249777791,32.2563024637739,20.));
#83379=CARTESIAN_POINT('Ctrl Pts',(-34.4988603609427,32.2784084519728,0.));
#83380=CARTESIAN_POINT('Ctrl Pts',(-34.4988603609427,32.2784084519728,20.));
#83381=CARTESIAN_POINT('Ctrl Pts',(-34.474081114695,32.3004963624427,0.));
#83382=CARTESIAN_POINT('Ctrl Pts',(-34.474081114695,32.3004963624427,20.));
#83383=CARTESIAN_POINT('Ctrl Pts',(-34.4492872517507,32.3225661850195,0.));
#83384=CARTESIAN_POINT('Ctrl Pts',(-34.4492872517507,32.3225661850195,20.));
#83385=CARTESIAN_POINT('Ctrl Pts',(-34.4244787848311,32.3446179095473,0.));
#83386=CARTESIAN_POINT('Ctrl Pts',(-34.4244787848311,32.3446179095473,20.));
#83387=CARTESIAN_POINT('Ctrl Pts',(-34.3996557266651,32.3666515258787,0.));
#83388=CARTESIAN_POINT('Ctrl Pts',(-34.3996557266651,32.3666515258787,20.));
#83389=CARTESIAN_POINT('Ctrl Pts',(-34.3748180899889,32.388667023875,0.));
#83390=CARTESIAN_POINT('Ctrl Pts',(-34.3748180899889,32.388667023875,20.));
#83391=CARTESIAN_POINT('Ctrl Pts',(-34.3499658875467,32.4106643934066,0.));
#83392=CARTESIAN_POINT('Ctrl Pts',(-34.3499658875467,32.4106643934066,20.));
#83393=CARTESIAN_POINT('Ctrl Pts',(-34.3250991320905,32.4326436243532,0.));
#83394=CARTESIAN_POINT('Ctrl Pts',(-34.3250991320905,32.4326436243532,20.));
#83395=CARTESIAN_POINT('Ctrl Pts',(-34.3002178363797,32.4546047066033,0.));
#83396=CARTESIAN_POINT('Ctrl Pts',(-34.3002178363797,32.4546047066033,20.));
#83397=CARTESIAN_POINT('Ctrl Pts',(-34.2753220131812,32.4765476300538,0.));
#83398=CARTESIAN_POINT('Ctrl Pts',(-34.2753220131812,32.4765476300538,20.));
#83399=CARTESIAN_POINT('Ctrl Pts',(-34.2504116752689,32.4984723846097,0.));
#83400=CARTESIAN_POINT('Ctrl Pts',(-34.2504116752689,32.4984723846097,20.));
#83401=CARTESIAN_POINT('Ctrl Pts',(-34.2254868354237,32.5203789601849,0.));
#83402=CARTESIAN_POINT('Ctrl Pts',(-34.2254868354237,32.5203789601849,20.));
#83403=CARTESIAN_POINT('Ctrl Pts',(-34.2005475064343,32.542267346702,0.));
#83404=CARTESIAN_POINT('Ctrl Pts',(-34.2005475064343,32.542267346702,20.));
#83405=CARTESIAN_POINT('Ctrl Pts',(-34.1755937010963,32.564137534092,0.));
#83406=CARTESIAN_POINT('Ctrl Pts',(-34.1755937010963,32.564137534092,20.));
#83407=CARTESIAN_POINT('Ctrl Pts',(-34.1506254322131,32.585989512295,0.));
#83408=CARTESIAN_POINT('Ctrl Pts',(-34.1506254322131,32.585989512295,20.));
#83409=CARTESIAN_POINT('Ctrl Pts',(-34.1256427125956,32.6078232712594,0.));
#83410=CARTESIAN_POINT('Ctrl Pts',(-34.1256427125956,32.6078232712594,20.));
#83411=CARTESIAN_POINT('Ctrl Pts',(-34.1006455550618,32.6296388009428,0.));
#83412=CARTESIAN_POINT('Ctrl Pts',(-34.1006455550618,32.6296388009428,20.));
#83413=CARTESIAN_POINT('Ctrl Pts',(-34.0756339724376,32.6514360913116,0.));
#83414=CARTESIAN_POINT('Ctrl Pts',(-34.0756339724376,32.6514360913116,20.));
#83415=CARTESIAN_POINT('Ctrl Pts',(-34.0506079775557,32.6732151323407,0.));
#83416=CARTESIAN_POINT('Ctrl Pts',(-34.0506079775557,32.6732151323407,20.));
#83417=CARTESIAN_POINT('Ctrl Pts',(-34.0255675832564,32.694975914014,0.));
#83418=CARTESIAN_POINT('Ctrl Pts',(-34.0255675832564,32.694975914014,20.));
#83419=CARTESIAN_POINT('Ctrl Pts',(-34.0005128023872,32.7167184263237,0.));
#83420=CARTESIAN_POINT('Ctrl Pts',(-34.0005128023872,32.7167184263237,20.));
#83421=CARTESIAN_POINT('Ctrl Pts',(-33.9754436478026,32.7384426592708,0.));
#83422=CARTESIAN_POINT('Ctrl Pts',(-33.9754436478026,32.7384426592708,20.));
#83423=CARTESIAN_POINT('Ctrl Pts',(-33.9503601323651,32.7601486028652,0.));
#83424=CARTESIAN_POINT('Ctrl Pts',(-33.9503601323651,32.7601486028652,20.));
#83425=CARTESIAN_POINT('Ctrl Pts',(-33.9252622689445,32.781836247126,0.));
#83426=CARTESIAN_POINT('Ctrl Pts',(-33.9252622689445,32.781836247126,20.));
#83427=CARTESIAN_POINT('Ctrl Pts',(-33.9001500704179,32.8035055820805,0.));
#83428=CARTESIAN_POINT('Ctrl Pts',(-33.9001500704179,32.8035055820805,20.));
#83429=CARTESIAN_POINT('Ctrl Pts',(-33.8750235496691,32.8251565977646,0.));
#83430=CARTESIAN_POINT('Ctrl Pts',(-33.8750235496691,32.8251565977646,20.));
#83431=CARTESIAN_POINT('Ctrl Pts',(-33.8498827195893,32.8467892842227,0.));
#83432=CARTESIAN_POINT('Ctrl Pts',(-33.8498827195893,32.8467892842227,20.));
#83433=CARTESIAN_POINT('Ctrl Pts',(-33.8247275930774,32.8684036315085,0.));
#83434=CARTESIAN_POINT('Ctrl Pts',(-33.8247275930774,32.8684036315085,20.));
#83435=CARTESIAN_POINT('Ctrl Pts',(-33.7995581830395,32.8899996296849,0.));
#83436=CARTESIAN_POINT('Ctrl Pts',(-33.7995581830395,32.8899996296849,20.));
#83437=CARTESIAN_POINT('Ctrl Pts',(-33.7743745023893,32.9115772688235,0.));
#83438=CARTESIAN_POINT('Ctrl Pts',(-33.7743745023893,32.9115772688235,20.));
#83439=CARTESIAN_POINT('Ctrl Pts',(-33.7491765640476,32.9331365390046,0.));
#83440=CARTESIAN_POINT('Ctrl Pts',(-33.7491765640476,32.9331365390046,20.));
#83441=CARTESIAN_POINT('Ctrl Pts',(-33.723964380943,32.9546774303179,0.));
#83442=CARTESIAN_POINT('Ctrl Pts',(-33.723964380943,32.9546774303179,20.));
#83443=CARTESIAN_POINT('Ctrl Pts',(-33.6987379660104,32.9761999328604,0.));
#83444=CARTESIAN_POINT('Ctrl Pts',(-33.6987379660104,32.9761999328604,20.));
#83445=CARTESIAN_POINT('Ctrl Pts',(-33.673497332192,32.9977040367383,0.));
#83446=CARTESIAN_POINT('Ctrl Pts',(-33.673497332192,32.9977040367383,20.));
#83447=CARTESIAN_POINT('Ctrl Pts',(-33.6482424924373,33.0191897320665,0.));
#83448=CARTESIAN_POINT('Ctrl Pts',(-33.6482424924373,33.0191897320665,20.));
#83449=CARTESIAN_POINT('Ctrl Pts',(-33.6229734597032,33.0406570089692,0.));
#83450=CARTESIAN_POINT('Ctrl Pts',(-33.6229734597032,33.0406570089692,20.));
#83451=CARTESIAN_POINT('Ctrl Pts',(-33.5976902469543,33.0621058575797,0.));
#83452=CARTESIAN_POINT('Ctrl Pts',(-33.5976902469543,33.0621058575797,20.));
#83453=CARTESIAN_POINT('Ctrl Pts',(-33.572392867162,33.0835362680399,0.));
#83454=CARTESIAN_POINT('Ctrl Pts',(-33.572392867162,33.0835362680399,20.));
#83455=CARTESIAN_POINT('Ctrl Pts',(-33.5470813333053,33.1049482305003,0.));
#83456=CARTESIAN_POINT('Ctrl Pts',(-33.5470813333053,33.1049482305003,20.));
#83457=CARTESIAN_POINT('Ctrl Pts',(-33.5217556583704,33.1263417351207,0.));
#83458=CARTESIAN_POINT('Ctrl Pts',(-33.5217556583704,33.1263417351207,20.));
#83459=CARTESIAN_POINT('Ctrl Pts',(-33.4964158553506,33.1477167720697,0.));
#83460=CARTESIAN_POINT('Ctrl Pts',(-33.4964158553506,33.1477167720697,20.));
#83461=CARTESIAN_POINT('Ctrl Pts',(-33.4710619372468,33.1690733315248,0.));
#83462=CARTESIAN_POINT('Ctrl Pts',(-33.4710619372468,33.1690733315248,20.));
#83463=CARTESIAN_POINT('Ctrl Pts',(-33.4456939170666,33.1904114036721,0.));
#83464=CARTESIAN_POINT('Ctrl Pts',(-33.4456939170666,33.1904114036721,20.));
#83465=CARTESIAN_POINT('Ctrl Pts',(-33.4203118078248,33.2117309787063,0.));
#83466=CARTESIAN_POINT('Ctrl Pts',(-33.4203118078248,33.2117309787063,20.));
#83467=CARTESIAN_POINT('Ctrl Pts',(-33.3949156225429,33.233032046831,0.));
#83468=CARTESIAN_POINT('Ctrl Pts',(-33.3949156225429,33.233032046831,20.));
#83469=CARTESIAN_POINT('Ctrl Pts',(-33.3695053742505,33.2543145982587,0.));
#83470=CARTESIAN_POINT('Ctrl Pts',(-33.3695053742505,33.2543145982587,20.));
#83471=CARTESIAN_POINT('Ctrl Pts',(-33.3440810759838,33.2755786232108,0.));
#83472=CARTESIAN_POINT('Ctrl Pts',(-33.3440810759838,33.2755786232108,20.));
#83473=CARTESIAN_POINT('Ctrl Pts',(-33.3186427407863,33.2968241119176,0.));
#83474=CARTESIAN_POINT('Ctrl Pts',(-33.3186427407863,33.2968241119176,20.));
#83475=CARTESIAN_POINT('Ctrl Pts',(-33.2931903817093,33.318051054619,0.));
#83476=CARTESIAN_POINT('Ctrl Pts',(-33.2931903817093,33.318051054619,20.));
#83477=CARTESIAN_POINT('Ctrl Pts',(-33.2677240118112,33.3392594415636,0.));
#83478=CARTESIAN_POINT('Ctrl Pts',(-33.2677240118112,33.3392594415636,20.));
#83479=CARTESIAN_POINT('Ctrl Pts',(-33.2422436441578,33.3604492630093,0.));
#83480=CARTESIAN_POINT('Ctrl Pts',(-33.2422436441578,33.3604492630093,20.));
#83481=CARTESIAN_POINT('Ctrl Pts',(-33.2167492918215,33.3816205092222,0.));
#83482=CARTESIAN_POINT('Ctrl Pts',(-33.2167492918215,33.3816205092222,20.));
#83483=CARTESIAN_POINT('Ctrl Pts',(-33.1912409678819,33.4027731704774,0.));
#83484=CARTESIAN_POINT('Ctrl Pts',(-33.1912409678819,33.4027731704774,20.));
#83485=CARTESIAN_POINT('Ctrl Pts',(-33.1657186854252,33.4239072370581,0.));
#83486=CARTESIAN_POINT('Ctrl Pts',(-33.1657186854252,33.4239072370581,20.));
#83487=CARTESIAN_POINT('Ctrl Pts',(-33.1401824575448,33.4450226992567,0.));
#83488=CARTESIAN_POINT('Ctrl Pts',(-33.1401824575448,33.4450226992567,20.));
#83489=CARTESIAN_POINT('Ctrl Pts',(-33.1146322973416,33.4661195473749,0.));
#83490=CARTESIAN_POINT('Ctrl Pts',(-33.1146322973416,33.4661195473749,20.));
#83491=CARTESIAN_POINT('Ctrl Pts',(-33.0890682179239,33.4871977717238,0.));
#83492=CARTESIAN_POINT('Ctrl Pts',(-33.0890682179239,33.4871977717238,20.));
#83493=CARTESIAN_POINT('Ctrl Pts',(-33.063490232407,33.5082573626235,0.));
#83494=CARTESIAN_POINT('Ctrl Pts',(-33.063490232407,33.5082573626235,20.));
#83495=CARTESIAN_POINT('Ctrl Pts',(-33.0378983539138,33.5292983104032,0.));
#83496=CARTESIAN_POINT('Ctrl Pts',(-33.0378983539138,33.5292983104032,20.));
#83497=CARTESIAN_POINT('Ctrl Pts',(-33.0122925955739,33.5503206054003,0.));
#83498=CARTESIAN_POINT('Ctrl Pts',(-33.0122925955739,33.5503206054003,20.));
#83499=CARTESIAN_POINT('Ctrl Pts',(-32.986672970524,33.5713242379612,0.));
#83500=CARTESIAN_POINT('Ctrl Pts',(-32.986672970524,33.5713242379612,20.));
#83501=CARTESIAN_POINT('Ctrl Pts',(-32.9610394919081,33.5923091984411,0.));
#83502=CARTESIAN_POINT('Ctrl Pts',(-32.9610394919081,33.5923091984411,20.));
#83503=CARTESIAN_POINT('Ctrl Pts',(-32.935392172877,33.6132754772045,0.));
#83504=CARTESIAN_POINT('Ctrl Pts',(-32.935392172877,33.6132754772045,20.));
#83505=CARTESIAN_POINT('Ctrl Pts',(-32.9097310265884,33.6342230646254,0.));
#83506=CARTESIAN_POINT('Ctrl Pts',(-32.9097310265884,33.6342230646254,20.));
#83507=CARTESIAN_POINT('Ctrl Pts',(-32.8840560662069,33.6551519510862,0.));
#83508=CARTESIAN_POINT('Ctrl Pts',(-32.8840560662069,33.6551519510862,20.));
#83509=CARTESIAN_POINT('Ctrl Pts',(-32.8583673049046,33.6760621269785,0.));
#83510=CARTESIAN_POINT('Ctrl Pts',(-32.8583673049046,33.6760621269785,20.));
#83511=CARTESIAN_POINT('Ctrl Pts',(-32.8326647558606,33.6969535827028,0.));
#83512=CARTESIAN_POINT('Ctrl Pts',(-32.8326647558606,33.6969535827028,20.));
#83513=CARTESIAN_POINT('Ctrl Pts',(-32.8069484322617,33.717826308669,0.));
#83514=CARTESIAN_POINT('Ctrl Pts',(-32.8069484322617,33.717826308669,20.));
#83515=CARTESIAN_POINT('Ctrl Pts',(-32.7812183473018,33.7386802952956,0.));
#83516=CARTESIAN_POINT('Ctrl Pts',(-32.7812183473018,33.7386802952956,20.));
#83517=CARTESIAN_POINT('Ctrl Pts',(-32.7554745141811,33.7595155330097,0.));
#83518=CARTESIAN_POINT('Ctrl Pts',(-32.7554745141811,33.7595155330097,20.));
#83519=CARTESIAN_POINT('Ctrl Pts',(-32.7297169461065,33.7803320122473,0.));
#83520=CARTESIAN_POINT('Ctrl Pts',(-32.7297169461065,33.7803320122473,20.));
#83521=CARTESIAN_POINT('Ctrl Pts',(-32.7039456562922,33.8011297234537,0.));
#83522=CARTESIAN_POINT('Ctrl Pts',(-32.7039456562922,33.8011297234537,20.));
#83523=CARTESIAN_POINT('Ctrl Pts',(-32.6781606579598,33.8219086570836,0.));
#83524=CARTESIAN_POINT('Ctrl Pts',(-32.6781606579598,33.8219086570836,20.));
#83525=CARTESIAN_POINT('Ctrl Pts',(-32.652361964338,33.8426688036011,0.));
#83526=CARTESIAN_POINT('Ctrl Pts',(-32.652361964338,33.8426688036011,20.));
#83527=CARTESIAN_POINT('Ctrl Pts',(-32.6265495886629,33.8634101534794,0.));
#83528=CARTESIAN_POINT('Ctrl Pts',(-32.6265495886629,33.8634101534794,20.));
#83529=CARTESIAN_POINT('Ctrl Pts',(-32.6007235441777,33.8841326972007,0.));
#83530=CARTESIAN_POINT('Ctrl Pts',(-32.6007235441777,33.8841326972007,20.));
#83531=CARTESIAN_POINT('Ctrl Pts',(-32.5748838441319,33.9048364252556,0.));
#83532=CARTESIAN_POINT('Ctrl Pts',(-32.5748838441319,33.9048364252556,20.));
#83533=CARTESIAN_POINT('Ctrl Pts',(-32.5490305017817,33.9255213281433,0.));
#83534=CARTESIAN_POINT('Ctrl Pts',(-32.5490305017817,33.9255213281433,20.));
#83535=CARTESIAN_POINT('Ctrl Pts',(-32.5231635303904,33.9461873963724,0.));
#83536=CARTESIAN_POINT('Ctrl Pts',(-32.5231635303904,33.9461873963724,20.));
#83537=CARTESIAN_POINT('Ctrl Pts',(-32.4972829432285,33.9668346204604,0.));
#83538=CARTESIAN_POINT('Ctrl Pts',(-32.4972829432285,33.9668346204604,20.));
#83539=CARTESIAN_POINT('Ctrl Pts',(-32.4713887535742,33.987462990935,0.));
#83540=CARTESIAN_POINT('Ctrl Pts',(-32.4713887535742,33.987462990935,20.));
#83541=CARTESIAN_POINT('Ctrl Pts',(-32.4454809747123,34.0080724983324,0.));
#83542=CARTESIAN_POINT('Ctrl Pts',(-32.4454809747123,34.0080724983324,20.));
#83543=CARTESIAN_POINT('Ctrl Pts',(-32.4195596199345,34.0286631331978,0.));
#83544=CARTESIAN_POINT('Ctrl Pts',(-32.4195596199345,34.0286631331978,20.));
#83545=CARTESIAN_POINT('Ctrl Pts',(-32.3936247025393,34.0492348860854,0.));
#83546=CARTESIAN_POINT('Ctrl Pts',(-32.3936247025393,34.0492348860854,20.));
#83547=CARTESIAN_POINT('Ctrl Pts',(-32.3676762358321,34.0697877475586,0.));
#83548=CARTESIAN_POINT('Ctrl Pts',(-32.3676762358321,34.0697877475586,20.));
#83549=CARTESIAN_POINT('Ctrl Pts',(-32.3417142331257,34.0903217081898,0.));
#83550=CARTESIAN_POINT('Ctrl Pts',(-32.3417142331257,34.0903217081898,20.));
#83551=CARTESIAN_POINT('Ctrl Pts',(-32.3157387077392,34.1108367585604,0.));
#83552=CARTESIAN_POINT('Ctrl Pts',(-32.3157387077392,34.1108367585604,20.));
#83553=CARTESIAN_POINT('Ctrl Pts',(-32.2897496729991,34.131332889261,0.));
#83554=CARTESIAN_POINT('Ctrl Pts',(-32.2897496729991,34.131332889261,20.));
#83555=CARTESIAN_POINT('Ctrl Pts',(-32.2637471422389,34.1518100908915,0.));
#83556=CARTESIAN_POINT('Ctrl Pts',(-32.2637471422389,34.1518100908915,20.));
#83557=CARTESIAN_POINT('Ctrl Pts',(-32.2377311287994,34.1722683540613,0.));
#83558=CARTESIAN_POINT('Ctrl Pts',(-32.2377311287994,34.1722683540613,20.));
#83559=CARTESIAN_POINT('Ctrl Pts',(-32.2117016460282,34.1927076693883,0.));
#83560=CARTESIAN_POINT('Ctrl Pts',(-32.2117016460282,34.1927076693883,20.));
#83561=CARTESIAN_POINT('Ctrl Pts',(-32.1856587072789,34.2131280274994,0.));
#83562=CARTESIAN_POINT('Ctrl Pts',(-32.1856587072789,34.2131280274994,20.));
#83563=CARTESIAN_POINT('Ctrl Pts',(-32.1596023259127,34.233529419031,0.));
#83564=CARTESIAN_POINT('Ctrl Pts',(-32.1596023259127,34.233529419031,20.));
#83565=CARTESIAN_POINT('Ctrl Pts',(-32.1335325152974,34.2539118346284,0.));
#83566=CARTESIAN_POINT('Ctrl Pts',(-32.1335325152974,34.2539118346284,20.));
#83567=CARTESIAN_POINT('Ctrl Pts',(-32.1074492888083,34.2742752649465,0.));
#83568=CARTESIAN_POINT('Ctrl Pts',(-32.1074492888083,34.2742752649465,20.));
#83569=CARTESIAN_POINT('Ctrl Pts',(-32.081352659827,34.2946197006486,0.));
#83570=CARTESIAN_POINT('Ctrl Pts',(-32.081352659827,34.2946197006486,20.));
#83571=CARTESIAN_POINT('Ctrl Pts',(-32.0552426417428,34.3149451324081,0.));
#83572=CARTESIAN_POINT('Ctrl Pts',(-32.0552426417428,34.3149451324081,20.));
#83573=CARTESIAN_POINT('Ctrl Pts',(-32.0291192479513,34.335251550907,0.));
#83574=CARTESIAN_POINT('Ctrl Pts',(-32.0291192479513,34.335251550907,20.));
#83575=CARTESIAN_POINT('Ctrl Pts',(-32.0029824918551,34.3555389468366,0.));
#83576=CARTESIAN_POINT('Ctrl Pts',(-32.0029824918551,34.3555389468366,20.));
#83577=CARTESIAN_POINT('Ctrl Pts',(-31.9768323868632,34.3758073108972,0.));
#83578=CARTESIAN_POINT('Ctrl Pts',(-31.9768323868632,34.3758073108972,20.));
#83579=CARTESIAN_POINT('Ctrl Pts',(-31.9506689463919,34.3960566337982,0.));
#83580=CARTESIAN_POINT('Ctrl Pts',(-31.9506689463919,34.3960566337982,20.));
#83581=CARTESIAN_POINT('Ctrl Pts',(-31.9244921838641,34.4162869062583,0.));
#83582=CARTESIAN_POINT('Ctrl Pts',(-31.9244921838641,34.4162869062583,20.));
#83583=CARTESIAN_POINT('Ctrl Pts',(-31.8983021127102,34.4364981190057,0.));
#83584=CARTESIAN_POINT('Ctrl Pts',(-31.8983021127102,34.4364981190057,20.));
#83585=CARTESIAN_POINT('Ctrl Pts',(-31.8720987463673,34.4566902627777,0.));
#83586=CARTESIAN_POINT('Ctrl Pts',(-31.8720987463673,34.4566902627777,20.));
#83587=CARTESIAN_POINT('Ctrl Pts',(-31.8458820982794,34.4768633283209,0.));
#83588=CARTESIAN_POINT('Ctrl Pts',(-31.8458820982794,34.4768633283209,20.));
#83589=CARTESIAN_POINT('Ctrl Pts',(-31.819652181897,34.4970173063908,0.));
#83590=CARTESIAN_POINT('Ctrl Pts',(-31.819652181897,34.4970173063908,20.));
#83591=CARTESIAN_POINT('Ctrl Pts',(-31.7934090106771,34.5171521877518,0.));
#83592=CARTESIAN_POINT('Ctrl Pts',(-31.7934090106771,34.5171521877518,20.));
#83593=CARTESIAN_POINT('Ctrl Pts',(-31.7671525980838,34.5372679631777,0.));
#83594=CARTESIAN_POINT('Ctrl Pts',(-31.7671525980838,34.5372679631777,20.));
#83595=CARTESIAN_POINT('Ctrl Pts',(-31.7408829575879,34.5573646234518,0.));
#83596=CARTESIAN_POINT('Ctrl Pts',(-31.7408829575879,34.5573646234518,20.));
#83597=CARTESIAN_POINT('Ctrl Pts',(-31.7146001026678,34.5774421593669,0.));
#83598=CARTESIAN_POINT('Ctrl Pts',(-31.7146001026678,34.5774421593669,20.));
#83599=CARTESIAN_POINT('Ctrl Pts',(-31.6883040468088,34.5975005617252,0.));
#83600=CARTESIAN_POINT('Ctrl Pts',(-31.6883040468088,34.5975005617252,20.));
#83601=CARTESIAN_POINT('Ctrl Pts',(-31.6619948035027,34.6175398213376,0.));
#83602=CARTESIAN_POINT('Ctrl Pts',(-31.6619948035027,34.6175398213376,20.));
#83603=CARTESIAN_POINT('Ctrl Pts',(-31.6356723862475,34.6375599290242,0.));
#83604=CARTESIAN_POINT('Ctrl Pts',(-31.6356723862475,34.6375599290242,20.));
#83605=CARTESIAN_POINT('Ctrl Pts',(-31.609336808548,34.6575608756141,0.));
#83606=CARTESIAN_POINT('Ctrl Pts',(-31.609336808548,34.6575608756141,20.));
#83607=CARTESIAN_POINT('Ctrl Pts',(-31.5829880839157,34.6775426519456,0.));
#83608=CARTESIAN_POINT('Ctrl Pts',(-31.5829880839157,34.6775426519456,20.));
#83609=CARTESIAN_POINT('Ctrl Pts',(-31.556626225869,34.6975052488666,0.));
#83610=CARTESIAN_POINT('Ctrl Pts',(-31.556626225869,34.6975052488666,20.));
#83611=CARTESIAN_POINT('Ctrl Pts',(-31.5302512479332,34.7174486572342,0.));
#83612=CARTESIAN_POINT('Ctrl Pts',(-31.5302512479332,34.7174486572342,20.));
#83613=CARTESIAN_POINT('Ctrl Pts',(-31.5038631636409,34.7373728679152,0.));
#83614=CARTESIAN_POINT('Ctrl Pts',(-31.5038631636409,34.7373728679152,20.));
#83615=CARTESIAN_POINT('Ctrl Pts',(-31.4774619865312,34.7572778717852,0.));
#83616=CARTESIAN_POINT('Ctrl Pts',(-31.4774619865312,34.7572778717852,20.));
#83617=CARTESIAN_POINT('Ctrl Pts',(-31.4510477301503,34.7771636597296,0.));
#83618=CARTESIAN_POINT('Ctrl Pts',(-31.4510477301503,34.7771636597296,20.));
#83619=CARTESIAN_POINT('Ctrl Pts',(-31.4246204080513,34.7970302226433,0.));
#83620=CARTESIAN_POINT('Ctrl Pts',(-31.4246204080513,34.7970302226433,20.));
#83621=CARTESIAN_POINT('Ctrl Pts',(-31.3981800337935,34.8168775514299,0.));
#83622=CARTESIAN_POINT('Ctrl Pts',(-31.3981800337935,34.8168775514299,20.));
#83623=CARTESIAN_POINT('Ctrl Pts',(-31.3717266209434,34.8367056370026,0.));
#83624=CARTESIAN_POINT('Ctrl Pts',(-31.3717266209434,34.8367056370026,20.));
#83625=CARTESIAN_POINT('Ctrl Pts',(-31.3452601830726,34.856514470283,0.));
#83626=CARTESIAN_POINT('Ctrl Pts',(-31.3452601830726,34.856514470283,20.));
#83627=CARTESIAN_POINT('Ctrl Pts',(-31.3187807337598,34.8763040422018,0.));
#83628=CARTESIAN_POINT('Ctrl Pts',(-31.3187807337598,34.8763040422018,20.));
#83629=CARTESIAN_POINT('Ctrl Pts',(-31.2922882865907,34.8960743436995,0.));
#83630=CARTESIAN_POINT('Ctrl Pts',(-31.2922882865907,34.8960743436995,20.));
#83631=CARTESIAN_POINT('Ctrl Pts',(-31.2657828551579,34.9158253657262,0.));
#83632=CARTESIAN_POINT('Ctrl Pts',(-31.2657828551579,34.9158253657262,20.));
#83633=CARTESIAN_POINT('Ctrl Pts',(-31.2392644530613,34.9355570992414,0.));
#83634=CARTESIAN_POINT('Ctrl Pts',(-31.2392644530613,34.9355570992414,20.));
#83635=CARTESIAN_POINT('Ctrl Pts',(-31.2127330939086,34.9552695352152,0.));
#83636=CARTESIAN_POINT('Ctrl Pts',(-31.2127330939086,34.9552695352152,20.));
#83637=CARTESIAN_POINT('Ctrl Pts',(-31.1861887913133,34.9749626646259,0.));
#83638=CARTESIAN_POINT('Ctrl Pts',(-31.1861887913133,34.9749626646259,20.));
#83639=CARTESIAN_POINT('Ctrl Pts',(-31.1596315588953,34.9946364784612,0.));
#83640=CARTESIAN_POINT('Ctrl Pts',(-31.1596315588953,34.9946364784612,20.));
#83641=CARTESIAN_POINT('Ctrl Pts',(-31.1330614102809,35.0142909677175,0.));
#83642=CARTESIAN_POINT('Ctrl Pts',(-31.1330614102809,35.0142909677175,20.));
#83643=CARTESIAN_POINT('Ctrl Pts',(-31.1064783591027,35.0339261234012,0.));
#83644=CARTESIAN_POINT('Ctrl Pts',(-31.1064783591027,35.0339261234012,20.));
#83645=CARTESIAN_POINT('Ctrl Pts',(-31.0798824190004,35.0535419365277,0.));
#83646=CARTESIAN_POINT('Ctrl Pts',(-31.0798824190004,35.0535419365277,20.));
#83647=CARTESIAN_POINT('Ctrl Pts',(-31.0532736036193,35.0731383981212,0.));
#83648=CARTESIAN_POINT('Ctrl Pts',(-31.0532736036193,35.0731383981212,20.));
#83649=CARTESIAN_POINT('Ctrl Pts',(-31.026651926612,35.0927154992152,0.));
#83650=CARTESIAN_POINT('Ctrl Pts',(-31.026651926612,35.0927154992152,20.));
#83651=CARTESIAN_POINT('Ctrl Pts',(-31.0000174016378,35.1122732308527,0.));
#83652=CARTESIAN_POINT('Ctrl Pts',(-31.0000174016378,35.1122732308527,20.));
#83653=CARTESIAN_POINT('Ctrl Pts',(-30.9733700423633,35.131811584087,0.));
#83654=CARTESIAN_POINT('Ctrl Pts',(-30.9733700423633,35.131811584087,20.));
#83655=CARTESIAN_POINT('Ctrl Pts',(-30.9467098624624,35.1513305499814,0.));
#83656=CARTESIAN_POINT('Ctrl Pts',(-30.9467098624624,35.1513305499814,20.));
#83657=CARTESIAN_POINT('Ctrl Pts',(-30.9200368756162,35.170830119609,0.));
#83658=CARTESIAN_POINT('Ctrl Pts',(-30.9200368756162,35.170830119609,20.));
#83659=CARTESIAN_POINT('Ctrl Pts',(-30.8933510955116,35.1903102840518,0.));
#83660=CARTESIAN_POINT('Ctrl Pts',(-30.8933510955116,35.1903102840518,20.));
#83661=CARTESIAN_POINT('Ctrl Pts',(-30.8666525358408,35.2097710343997,0.));
#83662=CARTESIAN_POINT('Ctrl Pts',(-30.8666525358408,35.2097710343997,20.));
#83663=CARTESIAN_POINT('Ctrl Pts',(-30.8399412103027,35.2292123617517,0.));
#83664=CARTESIAN_POINT('Ctrl Pts',(-30.8399412103027,35.2292123617517,20.));
#83665=CARTESIAN_POINT('Ctrl Pts',(-30.8132171326021,35.2486342572162,0.));
#83666=CARTESIAN_POINT('Ctrl Pts',(-30.8132171326021,35.2486342572162,20.));
#83667=CARTESIAN_POINT('Ctrl Pts',(-30.7864803164511,35.2680367119112,0.));
#83668=CARTESIAN_POINT('Ctrl Pts',(-30.7864803164511,35.2680367119112,20.));
#83669=CARTESIAN_POINT('Ctrl Pts',(-30.7597307755696,35.2874197169657,0.));
#83670=CARTESIAN_POINT('Ctrl Pts',(-30.7597307755696,35.2874197169657,20.));
#83671=CARTESIAN_POINT('Ctrl Pts',(-30.732968523684,35.3067832635176,0.));
#83672=CARTESIAN_POINT('Ctrl Pts',(-30.732968523684,35.3067832635176,20.));
#83673=CARTESIAN_POINT('Ctrl Pts',(-30.7061935745273,35.3261273427148,0.));
#83674=CARTESIAN_POINT('Ctrl Pts',(-30.7061935745273,35.3261273427148,20.));
#83675=CARTESIAN_POINT('Ctrl Pts',(-30.6794059418388,35.3454519457137,0.));
#83676=CARTESIAN_POINT('Ctrl Pts',(-30.6794059418388,35.3454519457137,20.));
#83677=CARTESIAN_POINT('Ctrl Pts',(-30.6526056393639,35.3647570636798,0.));
#83678=CARTESIAN_POINT('Ctrl Pts',(-30.6526056393639,35.3647570636798,20.));
#83679=CARTESIAN_POINT('Ctrl Pts',(-30.6257926808542,35.3840426877879,0.));
#83680=CARTESIAN_POINT('Ctrl Pts',(-30.6257926808542,35.3840426877879,20.));
#83681=CARTESIAN_POINT('Ctrl Pts',(-30.5989670800681,35.4033088092225,0.));
#83682=CARTESIAN_POINT('Ctrl Pts',(-30.5989670800681,35.4033088092225,20.));
#83683=CARTESIAN_POINT('Ctrl Pts',(-30.5721288507715,35.4225554191786,0.));
#83684=CARTESIAN_POINT('Ctrl Pts',(-30.5721288507715,35.4225554191786,20.));
#83685=CARTESIAN_POINT('Ctrl Pts',(-30.5452780067369,35.4417825088605,0.));
#83686=CARTESIAN_POINT('Ctrl Pts',(-30.5452780067369,35.4417825088605,20.));
#83687=CARTESIAN_POINT('Ctrl Pts',(-30.5184145617425,35.4609900694812,0.));
#83688=CARTESIAN_POINT('Ctrl Pts',(-30.5184145617425,35.4609900694812,20.));
#83689=CARTESIAN_POINT('Ctrl Pts',(-30.4915385295724,35.4801780922625,0.));
#83690=CARTESIAN_POINT('Ctrl Pts',(-30.4915385295724,35.4801780922625,20.));
#83691=CARTESIAN_POINT('Ctrl Pts',(-30.4646499240178,35.4993465684361,0.));
#83692=CARTESIAN_POINT('Ctrl Pts',(-30.4646499240178,35.4993465684361,20.));
#83693=CARTESIAN_POINT('Ctrl Pts',(-30.437748758876,35.518495489243,0.));
#83694=CARTESIAN_POINT('Ctrl Pts',(-30.437748758876,35.518495489243,20.));
#83695=CARTESIAN_POINT('Ctrl Pts',(-30.4108350479521,35.5376248459348,0.));
#83696=CARTESIAN_POINT('Ctrl Pts',(-30.4108350479521,35.5376248459348,20.));
#83697=CARTESIAN_POINT('Ctrl Pts',(-30.3839088050584,35.5567346297736,0.));
#83698=CARTESIAN_POINT('Ctrl Pts',(-30.3839088050584,35.5567346297736,20.));
#83699=CARTESIAN_POINT('Ctrl Pts',(-30.3569700440131,35.5758248320301,0.));
#83700=CARTESIAN_POINT('Ctrl Pts',(-30.3569700440131,35.5758248320301,20.));
#83701=CARTESIAN_POINT('Ctrl Pts',(-30.3300187786403,35.5948954439837,0.));
#83702=CARTESIAN_POINT('Ctrl Pts',(-30.3300187786403,35.5948954439837,20.));
#83703=CARTESIAN_POINT('Ctrl Pts',(-30.3030550227693,35.6139464569223,0.));
#83704=CARTESIAN_POINT('Ctrl Pts',(-30.3030550227693,35.6139464569223,20.));
#83705=CARTESIAN_POINT('Ctrl Pts',(-30.2760787902362,35.6329778621436,0.));
#83706=CARTESIAN_POINT('Ctrl Pts',(-30.2760787902362,35.6329778621436,20.));
#83707=CARTESIAN_POINT('Ctrl Pts',(-30.2490900948838,35.6519896509552,0.));
#83708=CARTESIAN_POINT('Ctrl Pts',(-30.2490900948838,35.6519896509552,20.));
#83709=CARTESIAN_POINT('Ctrl Pts',(-30.2220889505625,35.6709818146751,0.));
#83710=CARTESIAN_POINT('Ctrl Pts',(-30.2220889505625,35.6709818146751,20.));
#83711=CARTESIAN_POINT('Ctrl Pts',(-30.1950753711288,35.6899543446308,0.));
#83712=CARTESIAN_POINT('Ctrl Pts',(-30.1950753711288,35.6899543446308,20.));
#83713=CARTESIAN_POINT('Ctrl Pts',(-30.1680493704465,35.7089072321597,0.));
#83714=CARTESIAN_POINT('Ctrl Pts',(-30.1680493704465,35.7089072321597,20.));
#83715=CARTESIAN_POINT('Ctrl Pts',(-30.141010962385,35.7278404686079,0.));
#83716=CARTESIAN_POINT('Ctrl Pts',(-30.141010962385,35.7278404686079,20.));
#83717=CARTESIAN_POINT('Ctrl Pts',(-30.1139601608197,35.7467540453308,0.));
#83718=CARTESIAN_POINT('Ctrl Pts',(-30.1139601608197,35.7467540453308,20.));
#83719=CARTESIAN_POINT('Ctrl Pts',(-30.0868969796328,35.7656479536938,0.));
#83720=CARTESIAN_POINT('Ctrl Pts',(-30.0868969796328,35.7656479536938,20.));
#83721=CARTESIAN_POINT('Ctrl Pts',(-30.0598214327127,35.7845221850715,0.));
#83722=CARTESIAN_POINT('Ctrl Pts',(-30.0598214327127,35.7845221850715,20.));
#83723=CARTESIAN_POINT('Ctrl Pts',(-30.0327335339539,35.8033767308478,0.));
#83724=CARTESIAN_POINT('Ctrl Pts',(-30.0327335339539,35.8033767308478,20.));
#83725=CARTESIAN_POINT('Ctrl Pts',(-30.005633297258,35.8222115824166,0.));
#83726=CARTESIAN_POINT('Ctrl Pts',(-30.005633297258,35.8222115824166,20.));
#83727=CARTESIAN_POINT('Ctrl Pts',(-29.9785207365333,35.841026731182,0.));
#83728=CARTESIAN_POINT('Ctrl Pts',(-29.9785207365333,35.841026731182,20.));
#83729=CARTESIAN_POINT('Ctrl Pts',(-29.9513958656946,35.8598221685576,0.));
#83730=CARTESIAN_POINT('Ctrl Pts',(-29.9513958656946,35.8598221685576,20.));
#83731=CARTESIAN_POINT('Ctrl Pts',(-29.9242586986624,35.8785978859658,0.));
#83732=CARTESIAN_POINT('Ctrl Pts',(-29.9242586986624,35.8785978859658,20.));
#83733=CARTESIAN_POINT('Ctrl Pts',(-29.8971092493635,35.8973538748387,0.));
#83734=CARTESIAN_POINT('Ctrl Pts',(-29.8971092493635,35.8973538748387,20.));
#83735=CARTESIAN_POINT('Ctrl Pts',(-29.869947531731,35.9160901266176,0.));
#83736=CARTESIAN_POINT('Ctrl Pts',(-29.869947531731,35.9160901266176,20.));
#83737=CARTESIAN_POINT('Ctrl Pts',(-29.8427735597049,35.9348066327539,0.));
#83738=CARTESIAN_POINT('Ctrl Pts',(-29.8427735597049,35.9348066327539,20.));
#83739=CARTESIAN_POINT('Ctrl Pts',(-29.8155873472308,35.9535033847081,0.));
#83740=CARTESIAN_POINT('Ctrl Pts',(-29.8155873472308,35.9535033847081,20.));
#83741=CARTESIAN_POINT('Ctrl Pts',(-29.7883889082614,35.9721803739509,0.));
#83742=CARTESIAN_POINT('Ctrl Pts',(-29.7883889082614,35.9721803739509,20.));
#83743=CARTESIAN_POINT('Ctrl Pts',(-29.7611782567557,35.9908375919623,0.));
#83744=CARTESIAN_POINT('Ctrl Pts',(-29.7611782567557,35.9908375919623,20.));
#83745=CARTESIAN_POINT('Ctrl Pts',(-29.7339554066796,36.009475030233,0.));
#83746=CARTESIAN_POINT('Ctrl Pts',(-29.7339554066796,36.009475030233,20.));
#83747=CARTESIAN_POINT('Ctrl Pts',(-29.7067203720053,36.0280926802632,0.));
#83748=CARTESIAN_POINT('Ctrl Pts',(-29.7067203720053,36.0280926802632,20.));
#83749=CARTESIAN_POINT('Ctrl Pts',(-29.6794731667107,36.0466905335617,0.));
#83750=CARTESIAN_POINT('Ctrl Pts',(-29.6794731667107,36.0466905335617,20.));
#83751=CARTESIAN_POINT('Ctrl Pts',(-29.6522138047794,36.0652685816464,0.));
#83752=CARTESIAN_POINT('Ctrl Pts',(-29.6522138047794,36.0652685816464,20.));
#83753=CARTESIAN_POINT('Ctrl Pts',(-29.6249423002017,36.0838268160451,0.));
#83754=CARTESIAN_POINT('Ctrl Pts',(-29.6249423002017,36.0838268160451,20.));
#83755=CARTESIAN_POINT('Ctrl Pts',(-29.5976586669748,36.1023652282957,0.));
#83756=CARTESIAN_POINT('Ctrl Pts',(-29.5976586669748,36.1023652282957,20.));
#83757=CARTESIAN_POINT('Ctrl Pts',(-29.5703629191022,36.120883809946,0.));
#83758=CARTESIAN_POINT('Ctrl Pts',(-29.5703629191022,36.120883809946,20.));
#83759=CARTESIAN_POINT('Ctrl Pts',(-29.5430550705938,36.1393825525541,0.));
#83760=CARTESIAN_POINT('Ctrl Pts',(-29.5430550705938,36.1393825525541,20.));
#83761=CARTESIAN_POINT('Ctrl Pts',(-29.5157351354652,36.1578614476865,0.));
#83762=CARTESIAN_POINT('Ctrl Pts',(-29.5157351354652,36.1578614476865,20.));
#83763=CARTESIAN_POINT('Ctrl Pts',(-29.4884031277381,36.1763204869192,0.));
#83764=CARTESIAN_POINT('Ctrl Pts',(-29.4884031277381,36.1763204869192,20.));
#83765=CARTESIAN_POINT('Ctrl Pts',(-29.4610590614411,36.1947596618382,0.));
#83766=CARTESIAN_POINT('Ctrl Pts',(-29.4610590614411,36.1947596618382,20.));
#83767=CARTESIAN_POINT('Ctrl Pts',(-29.4337029506094,36.2131789640396,0.));
#83768=CARTESIAN_POINT('Ctrl Pts',(-29.4337029506094,36.2131789640396,20.));
#83769=CARTESIAN_POINT('Ctrl Pts',(-29.4063348092849,36.2315783851295,0.));
#83770=CARTESIAN_POINT('Ctrl Pts',(-29.4063348092849,36.2315783851295,20.));
#83771=CARTESIAN_POINT('Ctrl Pts',(-29.3789546515147,36.2499579167227,0.));
#83772=CARTESIAN_POINT('Ctrl Pts',(-29.3789546515147,36.2499579167227,20.));
#83773=CARTESIAN_POINT('Ctrl Pts',(-29.3515624913523,36.2683175504441,0.));
#83774=CARTESIAN_POINT('Ctrl Pts',(-29.3515624913523,36.2683175504441,20.));
#83775=CARTESIAN_POINT('Ctrl Pts',(-29.3241583428569,36.286657277928,0.));
#83776=CARTESIAN_POINT('Ctrl Pts',(-29.3241583428569,36.286657277928,20.));
#83777=CARTESIAN_POINT('Ctrl Pts',(-29.2967422200943,36.3049770908188,0.));
#83778=CARTESIAN_POINT('Ctrl Pts',(-29.2967422200943,36.3049770908188,20.));
#83779=CARTESIAN_POINT('Ctrl Pts',(-29.2693141371364,36.3232769807701,0.));
#83780=CARTESIAN_POINT('Ctrl Pts',(-29.2693141371364,36.3232769807701,20.));
#83781=CARTESIAN_POINT('Ctrl Pts',(-29.241874108062,36.3415569394456,0.));
#83782=CARTESIAN_POINT('Ctrl Pts',(-29.241874108062,36.3415569394456,20.));
#83783=CARTESIAN_POINT('Ctrl Pts',(-29.2144221469563,36.3598169585186,0.));
#83784=CARTESIAN_POINT('Ctrl Pts',(-29.2144221469563,36.3598169585186,20.));
#83785=CARTESIAN_POINT('Ctrl Pts',(-29.186958267911,36.3780570296725,0.));
#83786=CARTESIAN_POINT('Ctrl Pts',(-29.186958267911,36.3780570296725,20.));
#83787=CARTESIAN_POINT('Ctrl Pts',(-29.1594824850239,36.3962771446002,0.));
#83788=CARTESIAN_POINT('Ctrl Pts',(-29.1594824850239,36.3962771446002,20.));
#83789=CARTESIAN_POINT('Ctrl Pts',(-29.1319948123985,36.4144772950043,0.));
#83790=CARTESIAN_POINT('Ctrl Pts',(-29.1319948123985,36.4144772950043,20.));
#83791=CARTESIAN_POINT('Ctrl Pts',(-29.1044952641443,36.4326574725969,0.));
#83792=CARTESIAN_POINT('Ctrl Pts',(-29.1044952641443,36.4326574725969,20.));
#83793=CARTESIAN_POINT('Ctrl Pts',(-29.0769838543763,36.4508176690994,0.));
#83794=CARTESIAN_POINT('Ctrl Pts',(-29.0769838543763,36.4508176690994,20.));
#83795=CARTESIAN_POINT('Ctrl Pts',(-29.0494605972165,36.4689578762435,0.));
#83796=CARTESIAN_POINT('Ctrl Pts',(-29.0494605972165,36.4689578762435,20.));
#83797=CARTESIAN_POINT('Ctrl Pts',(-29.0219255067927,36.4870780857703,0.));
#83798=CARTESIAN_POINT('Ctrl Pts',(-29.0219255067927,36.4870780857703,20.));
#83799=CARTESIAN_POINT('Ctrl Pts',(-28.99437859724,36.5051782894316,0.));
#83800=CARTESIAN_POINT('Ctrl Pts',(-28.99437859724,36.5051782894316,20.));
#83801=CARTESIAN_POINT('Ctrl Pts',(-28.9668198826995,36.5232584789885,0.));
#83802=CARTESIAN_POINT('Ctrl Pts',(-28.9668198826995,36.5232584789885,20.));
#83803=CARTESIAN_POINT('Ctrl Pts',(-28.9392493773185,36.5413186462123,0.));
#83804=CARTESIAN_POINT('Ctrl Pts',(-28.9392493773185,36.5413186462123,20.));
#83805=CARTESIAN_POINT('Ctrl Pts',(-28.9116670952497,36.5593587828826,0.));
#83806=CARTESIAN_POINT('Ctrl Pts',(-28.9116670952497,36.5593587828826,20.));
#83807=CARTESIAN_POINT('Ctrl Pts',(-28.8840730506515,36.577378880789,0.));
#83808=CARTESIAN_POINT('Ctrl Pts',(-28.8840730506515,36.577378880789,20.));
#83809=CARTESIAN_POINT('Ctrl Pts',(-28.8564672576885,36.5953789317305,0.));
#83810=CARTESIAN_POINT('Ctrl Pts',(-28.8564672576885,36.5953789317305,20.));
#83811=CARTESIAN_POINT('Ctrl Pts',(-28.8288497305324,36.6133589275174,0.));
#83812=CARTESIAN_POINT('Ctrl Pts',(-28.8288497305324,36.6133589275174,20.));
#83813=CARTESIAN_POINT('Ctrl Pts',(-28.8012204833609,36.6313188599694,0.));
#83814=CARTESIAN_POINT('Ctrl Pts',(-28.8012204833609,36.6313188599694,20.));
#83815=CARTESIAN_POINT('Ctrl Pts',(-28.7735795303585,36.6492587209167,0.));
#83816=CARTESIAN_POINT('Ctrl Pts',(-28.7735795303585,36.6492587209167,20.));
#83817=CARTESIAN_POINT('Ctrl Pts',(-28.7459268857152,36.6671785021988,0.));
#83818=CARTESIAN_POINT('Ctrl Pts',(-28.7459268857152,36.6671785021988,20.));
#83819=CARTESIAN_POINT('Ctrl Pts',(-28.7182625636274,36.6850781956649,0.));
#83820=CARTESIAN_POINT('Ctrl Pts',(-28.7182625636274,36.6850781956649,20.));
#83821=CARTESIAN_POINT('Ctrl Pts',(-28.6905865782966,36.7029577931733,0.));
#83822=CARTESIAN_POINT('Ctrl Pts',(-28.6905865782966,36.7029577931733,20.));
#83823=CARTESIAN_POINT('Ctrl Pts',(-28.6628989439305,36.7208172865919,0.));
#83824=CARTESIAN_POINT('Ctrl Pts',(-28.6628989439305,36.7208172865919,20.));
#83825=CARTESIAN_POINT('Ctrl Pts',(-28.6351996747428,36.738656667798,0.));
#83826=CARTESIAN_POINT('Ctrl Pts',(-28.6351996747428,36.738656667798,20.));
#83827=CARTESIAN_POINT('Ctrl Pts',(-28.6074887849535,36.7564759286795,0.));
#83828=CARTESIAN_POINT('Ctrl Pts',(-28.6074887849535,36.7564759286795,20.));
#83829=CARTESIAN_POINT('Ctrl Pts',(-28.5797662887891,36.774275061134,0.));
#83830=CARTESIAN_POINT('Ctrl Pts',(-28.5797662887891,36.774275061134,20.));
#83831=CARTESIAN_POINT('Ctrl Pts',(-28.5520322004825,36.7920540570698,0.));
#83832=CARTESIAN_POINT('Ctrl Pts',(-28.5520322004825,36.7920540570698,20.));
#83833=CARTESIAN_POINT('Ctrl Pts',(-28.5242865342725,36.809812908405,0.));
#83834=CARTESIAN_POINT('Ctrl Pts',(-28.5242865342725,36.809812908405,20.));
#83835=CARTESIAN_POINT('Ctrl Pts',(-28.496529304404,36.8275516070676,0.));
#83836=CARTESIAN_POINT('Ctrl Pts',(-28.496529304404,36.8275516070676,20.));
#83837=CARTESIAN_POINT('Ctrl Pts',(-28.4687605251277,36.8452701449948,0.));
#83838=CARTESIAN_POINT('Ctrl Pts',(-28.4687605251277,36.8452701449948,20.));
#83839=CARTESIAN_POINT('Ctrl Pts',(-28.4409802107003,36.8629685141338,0.));
#83840=CARTESIAN_POINT('Ctrl Pts',(-28.4409802107003,36.8629685141338,20.));
#83841=CARTESIAN_POINT('Ctrl Pts',(-28.4131883753841,36.8806467064409,0.));
#83842=CARTESIAN_POINT('Ctrl Pts',(-28.4131883753841,36.8806467064409,20.));
#83843=CARTESIAN_POINT('Ctrl Pts',(-28.3853850334476,36.8983047138822,0.));
#83844=CARTESIAN_POINT('Ctrl Pts',(-28.3853850334476,36.8983047138822,20.));
#83845=CARTESIAN_POINT('Ctrl Pts',(-28.3575701991656,36.9159425284342,0.));
#83846=CARTESIAN_POINT('Ctrl Pts',(-28.3575701991656,36.9159425284342,20.));
#83847=CARTESIAN_POINT('Ctrl Pts',(-28.3297438868192,36.9335601420835,0.));
#83848=CARTESIAN_POINT('Ctrl Pts',(-28.3297438868192,36.9335601420835,20.));
#83849=CARTESIAN_POINT('Ctrl Pts',(-28.3019061106957,36.9511575468269,0.));
#83850=CARTESIAN_POINT('Ctrl Pts',(-28.3019061106957,36.9511575468269,20.));
#83851=CARTESIAN_POINT('Ctrl Pts',(-28.2740568850882,36.9687347346709,0.));
#83852=CARTESIAN_POINT('Ctrl Pts',(-28.2740568850882,36.9687347346709,20.));
#83853=CARTESIAN_POINT('Ctrl Pts',(-28.2461962242955,36.9862916976318,0.));
#83854=CARTESIAN_POINT('Ctrl Pts',(-28.2461962242955,36.9862916976318,20.));
#83855=CARTESIAN_POINT('Ctrl Pts',(-28.2183241426219,37.0038284277349,0.));
#83856=CARTESIAN_POINT('Ctrl Pts',(-28.2183241426219,37.0038284277349,20.));
#83857=CARTESIAN_POINT('Ctrl Pts',(-28.1904406543778,37.0213449170157,0.));
#83858=CARTESIAN_POINT('Ctrl Pts',(-28.1904406543778,37.0213449170157,20.));
#83859=CARTESIAN_POINT('Ctrl Pts',(-28.1625457738798,37.0388411575197,0.));
#83860=CARTESIAN_POINT('Ctrl Pts',(-28.1625457738798,37.0388411575197,20.));
#83861=CARTESIAN_POINT('Ctrl Pts',(-28.1346395154507,37.0563171413025,0.));
#83862=CARTESIAN_POINT('Ctrl Pts',(-28.1346395154507,37.0563171413025,20.));
#83863=CARTESIAN_POINT('Ctrl Pts',(-28.1067218934195,37.0737728604297,0.));
#83864=CARTESIAN_POINT('Ctrl Pts',(-28.1067218934195,37.0737728604297,20.));
#83865=CARTESIAN_POINT('Ctrl Pts',(-28.0787929221219,37.0912083069771,0.));
#83866=CARTESIAN_POINT('Ctrl Pts',(-28.0787929221219,37.0912083069771,20.));
#83867=CARTESIAN_POINT('Ctrl Pts',(-28.0508526158994,37.1086234730311,0.));
#83868=CARTESIAN_POINT('Ctrl Pts',(-28.0508526158994,37.1086234730311,20.));
#83869=CARTESIAN_POINT('Ctrl Pts',(-28.0229009890986,37.1260183506872,0.));
#83870=CARTESIAN_POINT('Ctrl Pts',(-28.0229009890986,37.1260183506872,20.));
#83871=CARTESIAN_POINT('Ctrl Pts',(-27.994938056072,37.1433929320507,0.));
#83872=CARTESIAN_POINT('Ctrl Pts',(-27.994938056072,37.1433929320507,20.));
#83873=CARTESIAN_POINT('Ctrl Pts',(-27.9669638311771,37.1607472092352,0.));
#83874=CARTESIAN_POINT('Ctrl Pts',(-27.9669638311771,37.1607472092352,20.));
#83875=CARTESIAN_POINT('Ctrl Pts',(-27.9389783287777,37.1780811743651,0.));
#83876=CARTESIAN_POINT('Ctrl Pts',(-27.9389783287777,37.1780811743651,20.));
#83877=CARTESIAN_POINT('Ctrl Pts',(-27.9109815632437,37.1953948195748,0.));
#83878=CARTESIAN_POINT('Ctrl Pts',(-27.9109815632437,37.1953948195748,20.));
#83879=CARTESIAN_POINT('Ctrl Pts',(-27.8829735489517,37.2126881370093,0.));
#83880=CARTESIAN_POINT('Ctrl Pts',(-27.8829735489517,37.2126881370093,20.));
#83881=CARTESIAN_POINT('Ctrl Pts',(-27.8549543002843,37.2299611188238,0.));
#83882=CARTESIAN_POINT('Ctrl Pts',(-27.8549543002843,37.2299611188238,20.));
#83883=CARTESIAN_POINT('Ctrl Pts',(-27.8269238316305,37.2472137571841,0.));
#83884=CARTESIAN_POINT('Ctrl Pts',(-27.8269238316305,37.2472137571841,20.));
#83885=CARTESIAN_POINT('Ctrl Pts',(-27.7988821573847,37.2644460442654,0.));
#83886=CARTESIAN_POINT('Ctrl Pts',(-27.7988821573847,37.2644460442654,20.));
#83887=CARTESIAN_POINT('Ctrl Pts',(-27.7708292919468,37.2816579722525,0.));
#83888=CARTESIAN_POINT('Ctrl Pts',(-27.7708292919468,37.2816579722525,20.));
#83889=CARTESIAN_POINT('Ctrl Pts',(-27.7427652497224,37.2988495333397,0.));
#83890=CARTESIAN_POINT('Ctrl Pts',(-27.7427652497224,37.2988495333397,20.));
#83891=CARTESIAN_POINT('Ctrl Pts',(-27.7146900451229,37.3160207197314,0.));
#83892=CARTESIAN_POINT('Ctrl Pts',(-27.7146900451229,37.3160207197314,20.));
#83893=CARTESIAN_POINT('Ctrl Pts',(-27.6866036925651,37.3331715236413,0.));
#83894=CARTESIAN_POINT('Ctrl Pts',(-27.6866036925651,37.3331715236413,20.));
#83895=CARTESIAN_POINT('Ctrl Pts',(-27.6585062064726,37.3503019372939,0.));
#83896=CARTESIAN_POINT('Ctrl Pts',(-27.6585062064726,37.3503019372939,20.));
#83897=CARTESIAN_POINT('Ctrl Pts',(-27.6303976012745,37.3674119529233,0.));
#83898=CARTESIAN_POINT('Ctrl Pts',(-27.6303976012745,37.3674119529233,20.));
#83899=CARTESIAN_POINT('Ctrl Pts',(-27.6022778914064,37.384501562775,0.));
#83900=CARTESIAN_POINT('Ctrl Pts',(-27.6022778914064,37.384501562775,20.));
#83901=CARTESIAN_POINT('Ctrl Pts',(-27.5741470913095,37.4015707591036,0.));
#83902=CARTESIAN_POINT('Ctrl Pts',(-27.5741470913095,37.4015707591036,20.));
#83903=CARTESIAN_POINT('Ctrl Pts',(-27.5460052154308,37.418619534174,0.));
#83904=CARTESIAN_POINT('Ctrl Pts',(-27.5460052154308,37.418619534174,20.));
#83905=CARTESIAN_POINT('Ctrl Pts',(-27.5178522782226,37.4356478802604,0.));
#83906=CARTESIAN_POINT('Ctrl Pts',(-27.5178522782226,37.4356478802604,20.));
#83907=CARTESIAN_POINT('Ctrl Pts',(-27.489688294143,37.4526557896465,0.));
#83908=CARTESIAN_POINT('Ctrl Pts',(-27.489688294143,37.4526557896465,20.));
#83909=CARTESIAN_POINT('Ctrl Pts',(-27.4615132776558,37.4696432546266,0.));
#83910=CARTESIAN_POINT('Ctrl Pts',(-27.4615132776558,37.4696432546266,20.));
#83911=CARTESIAN_POINT('Ctrl Pts',(-27.4333272432311,37.4866102675047,0.));
#83912=CARTESIAN_POINT('Ctrl Pts',(-27.4333272432311,37.4866102675047,20.));
#83913=CARTESIAN_POINT('Ctrl Pts',(-27.4051302053449,37.5035568205959,0.));
#83914=CARTESIAN_POINT('Ctrl Pts',(-27.4051302053449,37.5035568205959,20.));
#83915=CARTESIAN_POINT('Ctrl Pts',(-27.3769221784798,37.5204829062256,0.));
#83916=CARTESIAN_POINT('Ctrl Pts',(-27.3769221784798,37.5204829062256,20.));
#83917=CARTESIAN_POINT('Ctrl Pts',(-27.3487031771241,37.5373885167297,0.));
#83918=CARTESIAN_POINT('Ctrl Pts',(-27.3487031771241,37.5373885167297,20.));
#83919=CARTESIAN_POINT('Ctrl Pts',(-27.3204732157704,37.5542736444521,0.));
#83920=CARTESIAN_POINT('Ctrl Pts',(-27.3204732157704,37.5542736444521,20.));
#83921=CARTESIAN_POINT('Ctrl Pts',(-27.2922323089174,37.571138281747,0.));
#83922=CARTESIAN_POINT('Ctrl Pts',(-27.2922323089174,37.571138281747,20.));
#83923=CARTESIAN_POINT('Ctrl Pts',(-27.2639804710687,37.5879824209777,0.));
#83924=CARTESIAN_POINT('Ctrl Pts',(-27.2639804710687,37.5879824209777,20.));
#83925=CARTESIAN_POINT('Ctrl Pts',(-27.2357177167352,37.6048060545188,0.));
#83926=CARTESIAN_POINT('Ctrl Pts',(-27.2357177167352,37.6048060545188,20.));
#83927=CARTESIAN_POINT('Ctrl Pts',(-27.2074440604332,37.6216091747552,0.));
#83928=CARTESIAN_POINT('Ctrl Pts',(-27.2074440604332,37.6216091747552,20.));
#83929=CARTESIAN_POINT('Ctrl Pts',(-27.1791595166856,37.6383917740821,0.));
#83930=CARTESIAN_POINT('Ctrl Pts',(-27.1791595166856,37.6383917740821,20.));
#83931=CARTESIAN_POINT('Ctrl Pts',(-27.15086410002,37.6551538449046,0.));
#83932=CARTESIAN_POINT('Ctrl Pts',(-27.15086410002,37.6551538449046,20.));
#83933=CARTESIAN_POINT('Ctrl Pts',(-27.1225578249703,37.6718953796384,0.));
#83934=CARTESIAN_POINT('Ctrl Pts',(-27.1225578249703,37.6718953796384,20.));
#83935=CARTESIAN_POINT('Ctrl Pts',(-27.0942407060752,37.6886163707084,0.));
#83936=CARTESIAN_POINT('Ctrl Pts',(-27.0942407060752,37.6886163707084,20.));
#83937=CARTESIAN_POINT('Ctrl Pts',(-27.0659127578793,37.705316810549,0.));
#83938=CARTESIAN_POINT('Ctrl Pts',(-27.0659127578793,37.705316810549,20.));
#83939=CARTESIAN_POINT('Ctrl Pts',(-27.0375739949332,37.7219966916053,0.));
#83940=CARTESIAN_POINT('Ctrl Pts',(-27.0375739949332,37.7219966916053,20.));
#83941=CARTESIAN_POINT('Ctrl Pts',(-27.0092244317934,37.7386560063324,0.));
#83942=CARTESIAN_POINT('Ctrl Pts',(-27.0092244317934,37.7386560063324,20.));
#83943=CARTESIAN_POINT('Ctrl Pts',(-26.9808640830224,37.755294747196,0.));
#83944=CARTESIAN_POINT('Ctrl Pts',(-26.9808640830224,37.755294747196,20.));
#83945=CARTESIAN_POINT('Ctrl Pts',(-26.9524929631885,37.7719129066715,0.));
#83946=CARTESIAN_POINT('Ctrl Pts',(-26.9524929631885,37.7719129066715,20.));
#83947=CARTESIAN_POINT('Ctrl Pts',(-26.9241110868652,37.7885104772446,0.));
#83948=CARTESIAN_POINT('Ctrl Pts',(-26.9241110868652,37.7885104772446,20.));
#83949=CARTESIAN_POINT('Ctrl Pts',(-26.8957184686315,37.8050874514106,0.));
#83950=CARTESIAN_POINT('Ctrl Pts',(-26.8957184686315,37.8050874514106,20.));
#83951=CARTESIAN_POINT('Ctrl Pts',(-26.8673151230714,37.8216438216745,0.));
#83952=CARTESIAN_POINT('Ctrl Pts',(-26.8673151230714,37.8216438216745,20.));
#83953=CARTESIAN_POINT('Ctrl Pts',(-26.8389010647754,37.8381795805523,0.));
#83954=CARTESIAN_POINT('Ctrl Pts',(-26.8389010647754,37.8381795805523,20.));
#83955=CARTESIAN_POINT('Ctrl Pts',(-26.8104763083398,37.8546947205707,0.));
#83956=CARTESIAN_POINT('Ctrl Pts',(-26.8104763083398,37.8546947205707,20.));
#83957=CARTESIAN_POINT('Ctrl Pts',(-26.782040868367,37.8711892342661,0.));
#83958=CARTESIAN_POINT('Ctrl Pts',(-26.782040868367,37.8711892342661,20.));
#83959=CARTESIAN_POINT('Ctrl Pts',(-26.7535947594648,37.887663114185,0.));
#83960=CARTESIAN_POINT('Ctrl Pts',(-26.7535947594648,37.887663114185,20.));
#83961=CARTESIAN_POINT('Ctrl Pts',(-26.7251379962461,37.904116352883,0.));
#83962=CARTESIAN_POINT('Ctrl Pts',(-26.7251379962461,37.904116352883,20.));
#83963=CARTESIAN_POINT('Ctrl Pts',(-26.6966705933291,37.9205489429259,0.));
#83964=CARTESIAN_POINT('Ctrl Pts',(-26.6966705933291,37.9205489429259,20.));
#83965=CARTESIAN_POINT('Ctrl Pts',(-26.6681925653377,37.9369608768896,0.));
#83966=CARTESIAN_POINT('Ctrl Pts',(-26.6681925653377,37.9369608768896,20.));
#83967=CARTESIAN_POINT('Ctrl Pts',(-26.6397039269022,37.9533521473617,0.));
#83968=CARTESIAN_POINT('Ctrl Pts',(-26.6397039269022,37.9533521473617,20.));
#83969=CARTESIAN_POINT('Ctrl Pts',(-26.6112046926582,37.9697227469388,0.));
#83970=CARTESIAN_POINT('Ctrl Pts',(-26.6112046926582,37.9697227469388,20.));
#83971=CARTESIAN_POINT('Ctrl Pts',(-26.5826948772472,37.9860726682286,0.));
#83972=CARTESIAN_POINT('Ctrl Pts',(-26.5826948772472,37.9860726682286,20.));
#83973=CARTESIAN_POINT('Ctrl Pts',(-26.5541744953163,38.0024019038486,0.));
#83974=CARTESIAN_POINT('Ctrl Pts',(-26.5541744953163,38.0024019038486,20.));
#83975=CARTESIAN_POINT('Ctrl Pts',(-26.5256435615177,38.0187104464255,0.));
#83976=CARTESIAN_POINT('Ctrl Pts',(-26.5256435615177,38.0187104464255,20.));
#83977=CARTESIAN_POINT('Ctrl Pts',(-26.4971020905092,38.0349982885963,0.));
#83978=CARTESIAN_POINT('Ctrl Pts',(-26.4971020905092,38.0349982885963,20.));
#83979=CARTESIAN_POINT('Ctrl Pts',(-26.4685500969542,38.0512654230085,0.));
#83980=CARTESIAN_POINT('Ctrl Pts',(-26.4685500969542,38.0512654230085,20.));
#83981=CARTESIAN_POINT('Ctrl Pts',(-26.439987595522,38.0675118423201,0.));
#83982=CARTESIAN_POINT('Ctrl Pts',(-26.439987595522,38.0675118423201,20.));
#83983=CARTESIAN_POINT('Ctrl Pts',(-26.4114146008872,38.0837375391992,0.));
#83984=CARTESIAN_POINT('Ctrl Pts',(-26.4114146008872,38.0837375391992,20.));
#83985=CARTESIAN_POINT('Ctrl Pts',(-26.3828311277301,38.0999425063245,0.));
#83986=CARTESIAN_POINT('Ctrl Pts',(-26.3828311277301,38.0999425063245,20.));
#83987=CARTESIAN_POINT('Ctrl Pts',(-26.3542371907363,38.1161267363846,0.));
#83988=CARTESIAN_POINT('Ctrl Pts',(-26.3542371907363,38.1161267363846,20.));
#83989=CARTESIAN_POINT('Ctrl Pts',(-26.3256328045976,38.1322902220784,0.));
#83990=CARTESIAN_POINT('Ctrl Pts',(-26.3256328045976,38.1322902220784,20.));
#83991=CARTESIAN_POINT('Ctrl Pts',(-26.2970179840108,38.1484329561142,0.));
#83992=CARTESIAN_POINT('Ctrl Pts',(-26.2970179840108,38.1484329561142,20.));
#83993=CARTESIAN_POINT('Ctrl Pts',(-26.2683927436784,38.1645549312104,0.));
#83994=CARTESIAN_POINT('Ctrl Pts',(-26.2683927436784,38.1645549312104,20.));
#83995=CARTESIAN_POINT('Ctrl Pts',(-26.2397570983077,38.1806561400953,0.));
#83996=CARTESIAN_POINT('Ctrl Pts',(-26.2397570983077,38.1806561400953,20.));
#83997=CARTESIAN_POINT('Ctrl Pts',(-26.2111110626121,38.196736575508,0.));
#83998=CARTESIAN_POINT('Ctrl Pts',(-26.2111110626121,38.196736575508,20.));
#83999=CARTESIAN_POINT('Ctrl Pts',(-26.1824546513102,38.2127962301983,0.));
#84000=CARTESIAN_POINT('Ctrl Pts',(-26.1824546513102,38.2127962301983,20.));
#84001=CARTESIAN_POINT('Ctrl Pts',(-26.1537878791271,38.2288350969267,0.));
#84002=CARTESIAN_POINT('Ctrl Pts',(-26.1537878791271,38.2288350969267,20.));
#84003=CARTESIAN_POINT('Ctrl Pts',(-26.1251107607929,38.244853168464,0.));
#84004=CARTESIAN_POINT('Ctrl Pts',(-26.1251107607929,38.244853168464,20.));
#84005=CARTESIAN_POINT('Ctrl Pts',(-26.0964233110434,38.2608504375906,0.));
#84006=CARTESIAN_POINT('Ctrl Pts',(-26.0964233110434,38.2608504375906,20.));
#84007=CARTESIAN_POINT('Ctrl Pts',(-26.0677255446196,38.276826897097,0.));
#84008=CARTESIAN_POINT('Ctrl Pts',(-26.0677255446196,38.276826897097,20.));
#84009=CARTESIAN_POINT('Ctrl Pts',(-26.0390174762676,38.2927825397833,0.));
#84010=CARTESIAN_POINT('Ctrl Pts',(-26.0390174762676,38.2927825397833,20.));
#84011=CARTESIAN_POINT('Ctrl Pts',(-26.0102991207387,38.3087173584599,0.));
#84012=CARTESIAN_POINT('Ctrl Pts',(-26.0102991207387,38.3087173584599,20.));
#84013=CARTESIAN_POINT('Ctrl Pts',(-25.9815704927901,38.3246313459476,0.));
#84014=CARTESIAN_POINT('Ctrl Pts',(-25.9815704927901,38.3246313459476,20.));
#84015=CARTESIAN_POINT('Ctrl Pts',(-25.9528316071847,38.3405244950781,0.));
#84016=CARTESIAN_POINT('Ctrl Pts',(-25.9528316071847,38.3405244950781,20.));
#84017=CARTESIAN_POINT('Ctrl Pts',(-25.9240824786909,38.3563967986931,0.));
#84018=CARTESIAN_POINT('Ctrl Pts',(-25.9240824786909,38.3563967986931,20.));
#84019=CARTESIAN_POINT('Ctrl Pts',(-25.8953231220827,38.3722482496454,0.));
#84020=CARTESIAN_POINT('Ctrl Pts',(-25.8953231220827,38.3722482496454,20.));
#84021=CARTESIAN_POINT('Ctrl Pts',(-25.8665535521392,38.3880788407969,0.));
#84022=CARTESIAN_POINT('Ctrl Pts',(-25.8665535521392,38.3880788407969,20.));
#84023=CARTESIAN_POINT('Ctrl Pts',(-25.8377737836446,38.4038885650199,0.));
#84024=CARTESIAN_POINT('Ctrl Pts',(-25.8377737836446,38.4038885650199,20.));
#84025=CARTESIAN_POINT('Ctrl Pts',(-25.8089838313888,38.4196774151969,0.));
#84026=CARTESIAN_POINT('Ctrl Pts',(-25.8089838313888,38.4196774151969,20.));
#84027=CARTESIAN_POINT('Ctrl Pts',(-25.7801837101667,38.4354453842206,0.));
#84028=CARTESIAN_POINT('Ctrl Pts',(-25.7801837101667,38.4354453842206,20.));
#84029=CARTESIAN_POINT('Ctrl Pts',(-25.7513734347795,38.4511924649945,0.));
#84030=CARTESIAN_POINT('Ctrl Pts',(-25.7513734347795,38.4511924649945,20.));
#84031=CARTESIAN_POINT('Ctrl Pts',(-25.7225530200332,38.4669186504318,0.));
#84032=CARTESIAN_POINT('Ctrl Pts',(-25.7225530200332,38.4669186504318,20.));
#84033=CARTESIAN_POINT('Ctrl Pts',(-25.6937224807392,38.4826239334567,0.));
#84034=CARTESIAN_POINT('Ctrl Pts',(-25.6937224807392,38.4826239334567,20.));
#84035=CARTESIAN_POINT('Ctrl Pts',(-25.6648818317151,38.4983083070042,0.));
#84036=CARTESIAN_POINT('Ctrl Pts',(-25.6648818317151,38.4983083070042,20.));
#84037=CARTESIAN_POINT('Ctrl Pts',(-25.6360310877836,38.5139717640192,0.));
#84038=CARTESIAN_POINT('Ctrl Pts',(-25.6360310877836,38.5139717640192,20.));
#84039=CARTESIAN_POINT('Ctrl Pts',(-25.6071702637723,38.5296142974561,0.));
#84040=CARTESIAN_POINT('Ctrl Pts',(-25.6071702637723,38.5296142974561,20.));
#84041=CARTESIAN_POINT('Ctrl Pts',(-25.5782993745137,38.5452359002793,0.));
#84042=CARTESIAN_POINT('Ctrl Pts',(-25.5782993745137,38.5452359002793,20.));
#84043=CARTESIAN_POINT('Ctrl Pts',(-25.5494184348457,38.5608365654634,0.));
#84044=CARTESIAN_POINT('Ctrl Pts',(-25.5494184348457,38.5608365654634,20.));
#84045=CARTESIAN_POINT('Ctrl Pts',(-25.5205274596115,38.5764162859939,0.));
#84046=CARTESIAN_POINT('Ctrl Pts',(-25.5205274596115,38.5764162859939,20.));
#84047=CARTESIAN_POINT('Ctrl Pts',(-25.4916264636604,38.591975054867,0.));
#84048=CARTESIAN_POINT('Ctrl Pts',(-25.4916264636604,38.591975054867,20.));
#84049=CARTESIAN_POINT('Ctrl Pts',(-25.462715461847,38.6075128650891,0.));
#84050=CARTESIAN_POINT('Ctrl Pts',(-25.462715461847,38.6075128650891,20.));
#84051=CARTESIAN_POINT('Ctrl Pts',(-25.4337944690316,38.6230297096774,0.));
#84052=CARTESIAN_POINT('Ctrl Pts',(-25.4337944690316,38.6230297096774,20.));
#84053=CARTESIAN_POINT('Ctrl Pts',(-25.4048635000795,38.6385255816593,0.));
#84054=CARTESIAN_POINT('Ctrl Pts',(-25.4048635000795,38.6385255816593,20.));
#84055=CARTESIAN_POINT('Ctrl Pts',(-25.3759225698613,38.6540004740723,0.));
#84056=CARTESIAN_POINT('Ctrl Pts',(-25.3759225698613,38.6540004740723,20.));
#84057=CARTESIAN_POINT('Ctrl Pts',(-25.3469716932528,38.6694543799641,0.));
#84058=CARTESIAN_POINT('Ctrl Pts',(-25.3469716932528,38.6694543799641,20.));
#84059=CARTESIAN_POINT('Ctrl Pts',(-25.3180108851341,38.6848872923919,0.));
#84060=CARTESIAN_POINT('Ctrl Pts',(-25.3180108851341,38.6848872923919,20.));
#84061=CARTESIAN_POINT('Ctrl Pts',(-25.2890401603913,38.7002992044241,0.));
#84062=CARTESIAN_POINT('Ctrl Pts',(-25.2890401603913,38.7002992044241,20.));
#84063=CARTESIAN_POINT('Ctrl Pts',(-25.2600595339159,38.7156901091392,0.));
#84064=CARTESIAN_POINT('Ctrl Pts',(-25.2600595339159,38.7156901091392,20.));
#84065=CARTESIAN_POINT('Ctrl Pts',(-25.231069020605,38.7310599996258,0.));
#84066=CARTESIAN_POINT('Ctrl Pts',(-25.231069020605,38.7310599996258,20.));
#84067=CARTESIAN_POINT('Ctrl Pts',(-25.2020686353608,38.7464088689836,0.));
#84068=CARTESIAN_POINT('Ctrl Pts',(-25.2020686353608,38.7464088689836,20.));
#84069=CARTESIAN_POINT('Ctrl Pts',(-25.1730583930911,38.7617367103228,0.));
#84070=CARTESIAN_POINT('Ctrl Pts',(-25.1730583930911,38.7617367103228,20.));
#84071=CARTESIAN_POINT('Ctrl Pts',(-25.1440383087085,38.7770435167639,0.));
#84072=CARTESIAN_POINT('Ctrl Pts',(-25.1440383087085,38.7770435167639,20.));
#84073=CARTESIAN_POINT('Ctrl Pts',(-25.1150083971302,38.7923292814368,0.));
#84074=CARTESIAN_POINT('Ctrl Pts',(-25.1150083971302,38.7923292814368,20.));
#84075=CARTESIAN_POINT('Ctrl Pts',(-25.0859686732795,38.8075939974829,0.));
#84076=CARTESIAN_POINT('Ctrl Pts',(-25.0859686732795,38.8075939974829,20.));
#84077=CARTESIAN_POINT('Ctrl Pts',(-25.0569191520845,38.8228376580533,0.));
#84078=CARTESIAN_POINT('Ctrl Pts',(-25.0569191520845,38.8228376580533,20.));
#84079=CARTESIAN_POINT('Ctrl Pts',(-25.0278598484791,38.8380602563098,0.));
#84080=CARTESIAN_POINT('Ctrl Pts',(-25.0278598484791,38.8380602563098,20.));
#84081=CARTESIAN_POINT('Ctrl Pts',(-24.9987907774025,38.8532617854245,0.));
#84082=CARTESIAN_POINT('Ctrl Pts',(-24.9987907774025,38.8532617854245,20.));
#84083=CARTESIAN_POINT('Ctrl Pts',(-24.9697119537989,38.8684422385799,0.));
#84084=CARTESIAN_POINT('Ctrl Pts',(-24.9697119537989,38.8684422385799,20.));
#84085=CARTESIAN_POINT('Ctrl Pts',(-24.9406233926168,38.883601608968,0.));
#84086=CARTESIAN_POINT('Ctrl Pts',(-24.9406233926168,38.883601608968,20.));
#84087=CARTESIAN_POINT('Ctrl Pts',(-24.9115251088108,38.8987398897918,0.));
#84088=CARTESIAN_POINT('Ctrl Pts',(-24.9115251088108,38.8987398897918,20.));
#84089=CARTESIAN_POINT('Ctrl Pts',(-24.8824171173402,38.9138570742648,0.));
#84090=CARTESIAN_POINT('Ctrl Pts',(-24.8824171173402,38.9138570742648,20.));
#84091=CARTESIAN_POINT('Ctrl Pts',(-24.8532994331703,38.9289531556117,0.));
#84092=CARTESIAN_POINT('Ctrl Pts',(-24.8532994331703,38.9289531556117,20.));
#84093=CARTESIAN_POINT('Ctrl Pts',(-24.8241720712716,38.9440281270684,0.));
#84094=CARTESIAN_POINT('Ctrl Pts',(-24.8241720712716,38.9440281270684,20.));
#84095=CARTESIAN_POINT('Ctrl Pts',(-24.7950350466188,38.9590819818797,0.));
#84096=CARTESIAN_POINT('Ctrl Pts',(-24.7950350466188,38.9590819818797,20.));
#84097=CARTESIAN_POINT('Ctrl Pts',(-24.7658883741919,38.9741147133012,0.));
#84098=CARTESIAN_POINT('Ctrl Pts',(-24.7658883741919,38.9741147133012,20.));
#84099=CARTESIAN_POINT('Ctrl Pts',(-24.736732068976,38.989126314598,0.));
#84100=CARTESIAN_POINT('Ctrl Pts',(-24.736732068976,38.989126314598,20.));
#84101=CARTESIAN_POINT('Ctrl Pts',(-24.7075661459617,39.0041167790461,0.));
#84102=CARTESIAN_POINT('Ctrl Pts',(-24.7075661459617,39.0041167790461,20.));
#84103=CARTESIAN_POINT('Ctrl Pts',(-24.6783906201452,39.019086099931,0.));
#84104=CARTESIAN_POINT('Ctrl Pts',(-24.6783906201452,39.019086099931,20.));
#84105=CARTESIAN_POINT('Ctrl Pts',(-24.6492055065285,39.0340342705498,0.));
#84106=CARTESIAN_POINT('Ctrl Pts',(-24.6492055065285,39.0340342705498,20.));
#84107=CARTESIAN_POINT('Ctrl Pts',(-24.6200108201182,39.0489612842095,0.));
#84108=CARTESIAN_POINT('Ctrl Pts',(-24.6200108201182,39.0489612842095,20.));
#84109=CARTESIAN_POINT('Ctrl Pts',(-24.5908065759258,39.0638671342286,0.));
#84110=CARTESIAN_POINT('Ctrl Pts',(-24.5908065759258,39.0638671342286,20.));
#84111=CARTESIAN_POINT('Ctrl Pts',(-24.5615927889669,39.0787518139362,0.));
#84112=CARTESIAN_POINT('Ctrl Pts',(-24.5615927889669,39.0787518139362,20.));
#84113=CARTESIAN_POINT('Ctrl Pts',(-24.5323694742617,39.0936153166722,0.));
#84114=CARTESIAN_POINT('Ctrl Pts',(-24.5323694742617,39.0936153166722,20.));
#84115=CARTESIAN_POINT('Ctrl Pts',(-24.5031366468345,39.1084576357871,0.));
#84116=CARTESIAN_POINT('Ctrl Pts',(-24.5031366468345,39.1084576357871,20.));
#84117=CARTESIAN_POINT('Ctrl Pts',(-24.4738943217155,39.1232787646414,0.));
#84118=CARTESIAN_POINT('Ctrl Pts',(-24.4738943217155,39.1232787646414,20.));
#84119=CARTESIAN_POINT('Ctrl Pts',(-24.4446425139409,39.1380786966047,0.));
#84120=CARTESIAN_POINT('Ctrl Pts',(-24.4446425139409,39.1380786966047,20.));
#84121=CARTESIAN_POINT('Ctrl Pts',(-24.4153812385543,39.1528574250568,0.));
#84122=CARTESIAN_POINT('Ctrl Pts',(-24.4153812385543,39.1528574250568,20.));
#84123=CARTESIAN_POINT('Ctrl Pts',(-24.3861105106067,39.1676149433869,0.));
#84124=CARTESIAN_POINT('Ctrl Pts',(-24.3861105106067,39.1676149433869,20.));
#84125=CARTESIAN_POINT('Ctrl Pts',(-24.3568303451549,39.1823512449951,0.));
#84126=CARTESIAN_POINT('Ctrl Pts',(-24.3568303451549,39.1823512449951,20.));
#84127=CARTESIAN_POINT('Ctrl Pts',(-24.3275407572588,39.197066323292,0.));
#84128=CARTESIAN_POINT('Ctrl Pts',(-24.3275407572588,39.197066323292,20.));
#84129=CARTESIAN_POINT('Ctrl Pts',(-24.2982417619806,39.2117601717005,0.));
#84130=CARTESIAN_POINT('Ctrl Pts',(-24.2982417619806,39.2117601717005,20.));
#84131=CARTESIAN_POINT('Ctrl Pts',(-24.2689333743823,39.2264327836562,0.));
#84132=CARTESIAN_POINT('Ctrl Pts',(-24.2689333743823,39.2264327836562,20.));
#84133=CARTESIAN_POINT('Ctrl Pts',(-24.2396156095261,39.2410841526077,0.));
#84134=CARTESIAN_POINT('Ctrl Pts',(-24.2396156095261,39.2410841526077,20.));
#84135=CARTESIAN_POINT('Ctrl Pts',(-24.2102884824784,39.2557142720138,0.));
#84136=CARTESIAN_POINT('Ctrl Pts',(-24.2102884824784,39.2557142720138,20.));
#84137=CARTESIAN_POINT('Ctrl Pts',(-24.1809520083147,39.2703231353422,0.));
#84138=CARTESIAN_POINT('Ctrl Pts',(-24.1809520083147,39.2703231353422,20.));
#84139=CARTESIAN_POINT('Ctrl Pts',(-24.1516062021224,39.2849107360681,0.));
#84140=CARTESIAN_POINT('Ctrl Pts',(-24.1516062021224,39.2849107360681,20.));
#84141=CARTESIAN_POINT('Ctrl Pts',(-24.1222510790066,39.2994770676712,0.));
#84142=CARTESIAN_POINT('Ctrl Pts',(-24.1222510790066,39.2994770676712,20.));
#84143=CARTESIAN_POINT('Ctrl Pts',(-24.0928866540882,39.3140221236369,0.));
#84144=CARTESIAN_POINT('Ctrl Pts',(-24.0928866540882,39.3140221236369,20.));
#84145=CARTESIAN_POINT('Ctrl Pts',(-24.0635129424931,39.3285458974612,0.));
#84146=CARTESIAN_POINT('Ctrl Pts',(-24.0635129424931,39.3285458974612,20.));
#84147=CARTESIAN_POINT('Ctrl Pts',(-24.0341299593437,39.3430483826555,0.));
#84148=CARTESIAN_POINT('Ctrl Pts',(-24.0341299593437,39.3430483826555,20.));
#84149=CARTESIAN_POINT('Ctrl Pts',(-24.0047377197503,39.3575295727493,0.));
#84150=CARTESIAN_POINT('Ctrl Pts',(-24.0047377197503,39.3575295727493,20.));
#84151=CARTESIAN_POINT('Ctrl Pts',(-23.9753362387978,39.3719894612957,0.));
#84152=CARTESIAN_POINT('Ctrl Pts',(-23.9753362387978,39.3719894612957,20.));
#84153=CARTESIAN_POINT('Ctrl Pts',(-23.9459255315518,39.3864280418676,0.));
#84154=CARTESIAN_POINT('Ctrl Pts',(-23.9459255315518,39.3864280418676,20.));
#84155=CARTESIAN_POINT('Ctrl Pts',(-23.9165056130837,39.4008453080481,0.));
#84156=CARTESIAN_POINT('Ctrl Pts',(-23.9165056130837,39.4008453080481,20.));
#84157=CARTESIAN_POINT('Ctrl Pts',(-23.8870764984925,39.4152412534209,0.));
#84158=CARTESIAN_POINT('Ctrl Pts',(-23.8870764984925,39.4152412534209,20.));
#84159=CARTESIAN_POINT('Ctrl Pts',(-23.8576382029238,39.4296158715627,0.));
#84160=CARTESIAN_POINT('Ctrl Pts',(-23.8576382029238,39.4296158715627,20.));
#84161=CARTESIAN_POINT('Ctrl Pts',(-23.8281907416005,39.4439691560298,0.));
#84162=CARTESIAN_POINT('Ctrl Pts',(-23.8281907416005,39.4439691560298,20.));
#84163=CARTESIAN_POINT('Ctrl Pts',(-23.7987341298022,39.4583011003674,0.));
#84164=CARTESIAN_POINT('Ctrl Pts',(-23.7987341298022,39.4583011003674,20.));
#84165=CARTESIAN_POINT('Ctrl Pts',(-23.7692683828081,39.4726116981337,0.));
#84166=CARTESIAN_POINT('Ctrl Pts',(-23.7692683828081,39.4726116981337,20.));
#84167=CARTESIAN_POINT('Ctrl Pts',(-23.7397935158457,39.4869009429217,0.));
#84168=CARTESIAN_POINT('Ctrl Pts',(-23.7397935158457,39.4869009429217,20.));
#84169=CARTESIAN_POINT('Ctrl Pts',(-23.7103095440476,39.5011688283778,0.));
#84170=CARTESIAN_POINT('Ctrl Pts',(-23.7103095440476,39.5011688283778,20.));
#84171=CARTESIAN_POINT('Ctrl Pts',(-23.6808164823786,39.5154153482324,0.));
#84172=CARTESIAN_POINT('Ctrl Pts',(-23.6808164823786,39.5154153482324,20.));
#84173=CARTESIAN_POINT('Ctrl Pts',(-23.651314345698,39.5296404962721,0.));
#84174=CARTESIAN_POINT('Ctrl Pts',(-23.651314345698,39.5296404962721,20.));
#84175=CARTESIAN_POINT('Ctrl Pts',(-23.6218031488905,39.5438442662853,0.));
#84176=CARTESIAN_POINT('Ctrl Pts',(-23.6218031488905,39.5438442662853,20.));
#84177=CARTESIAN_POINT('Ctrl Pts',(-23.5922829069852,39.5580266520107,0.));
#84178=CARTESIAN_POINT('Ctrl Pts',(-23.5922829069852,39.5580266520107,20.));
#84179=CARTESIAN_POINT('Ctrl Pts',(-23.5627536352592,39.5721876470956,0.));
#84180=CARTESIAN_POINT('Ctrl Pts',(-23.5627536352592,39.5721876470956,20.));
#84181=CARTESIAN_POINT('Ctrl Pts',(-23.533215349402,39.5863272450267,0.));
#84182=CARTESIAN_POINT('Ctrl Pts',(-23.533215349402,39.5863272450267,20.));
#84183=CARTESIAN_POINT('Ctrl Pts',(-23.5036680653391,39.6004454392038,0.));
#84184=CARTESIAN_POINT('Ctrl Pts',(-23.5036680653391,39.6004454392038,20.));
#84185=CARTESIAN_POINT('Ctrl Pts',(-23.4741117989348,39.6145422230651,0.));
#84186=CARTESIAN_POINT('Ctrl Pts',(-23.4741117989348,39.6145422230651,20.));
#84187=CARTESIAN_POINT('Ctrl Pts',(-23.4445465657147,39.6286175902046,0.));
#84188=CARTESIAN_POINT('Ctrl Pts',(-23.4445465657147,39.6286175902046,20.));
#84189=CARTESIAN_POINT('Ctrl Pts',(-23.4149723806221,39.6426715344742,0.));
#84190=CARTESIAN_POINT('Ctrl Pts',(-23.4149723806221,39.6426715344742,20.));
#84191=CARTESIAN_POINT('Ctrl Pts',(-23.385389257652,39.6567040501382,0.));
#84192=CARTESIAN_POINT('Ctrl Pts',(-23.385389257652,39.6567040501382,20.));
#84193=CARTESIAN_POINT('Ctrl Pts',(-23.3557972103217,39.670715131677,0.));
#84194=CARTESIAN_POINT('Ctrl Pts',(-23.3557972103217,39.670715131677,20.));
#84195=CARTESIAN_POINT('Ctrl Pts',(-23.3261962523444,39.6847047735001,0.));
#84196=CARTESIAN_POINT('Ctrl Pts',(-23.3261962523444,39.6847047735001,20.));
#84197=CARTESIAN_POINT('Ctrl Pts',(-23.2965863982648,39.6986729696788,0.));
#84198=CARTESIAN_POINT('Ctrl Pts',(-23.2965863982648,39.6986729696788,20.));
#84199=CARTESIAN_POINT('Ctrl Pts',(-23.2669676640418,39.712619713699,0.));
#84200=CARTESIAN_POINT('Ctrl Pts',(-23.2669676640418,39.712619713699,20.));
#84201=CARTESIAN_POINT('Ctrl Pts',(-23.2373400678346,39.7265449981305,0.));
#84202=CARTESIAN_POINT('Ctrl Pts',(-23.2373400678346,39.7265449981305,20.));
#84203=CARTESIAN_POINT('Ctrl Pts',(-23.2077036288598,39.7404488151086,0.));
#84204=CARTESIAN_POINT('Ctrl Pts',(-23.2077036288598,39.7404488151086,20.));
#84205=CARTESIAN_POINT('Ctrl Pts',(-23.1780583659508,39.7543311569459,0.));
#84206=CARTESIAN_POINT('Ctrl Pts',(-23.1780583659508,39.7543311569459,20.));
#84207=CARTESIAN_POINT('Ctrl Pts',(-23.1484042962029,39.7681920167058,0.));
#84208=CARTESIAN_POINT('Ctrl Pts',(-23.1484042962029,39.7681920167058,20.));
#84209=CARTESIAN_POINT('Ctrl Pts',(-23.1187414336251,39.7820313887737,0.));
#84210=CARTESIAN_POINT('Ctrl Pts',(-23.1187414336251,39.7820313887737,20.));
#84211=CARTESIAN_POINT('Ctrl Pts',(-23.089069787673,39.7958492694787,0.));
#84212=CARTESIAN_POINT('Ctrl Pts',(-23.089069787673,39.7958492694787,20.));
#84213=CARTESIAN_POINT('Ctrl Pts',(-23.0593893640427,39.8096456567259,0.));
#84214=CARTESIAN_POINT('Ctrl Pts',(-23.0593893640427,39.8096456567259,20.));
#84215=CARTESIAN_POINT('Ctrl Pts',(-23.0356380053139,39.8206655709903,0.));
#84216=CARTESIAN_POINT('Ctrl Pts',(-23.0356380053139,39.8206655709903,20.));
#84217=CARTESIAN_POINT('Ctrl Pts',(-23.0178205380655,39.8289208340947,0.));
#84218=CARTESIAN_POINT('Ctrl Pts',(-23.0178205380655,39.8289208340947,20.));
#84219=CARTESIAN_POINT('Ctrl Pts',(-23.005940471814,39.8344200439082,0.));
#84220=CARTESIAN_POINT('Ctrl Pts',(-23.005940471814,39.8344200439082,20.));
#84221=CARTESIAN_POINT('Ctrl Pts',(-23.,39.8371685740842,0.));
#84222=CARTESIAN_POINT('Ctrl Pts',(-23.,39.8371685740842,20.));
#84223=CARTESIAN_POINT('',(-23.,39.8371685740842,2.));
#84224=CARTESIAN_POINT('',(-23.,39.8371685740842,0.));
#84225=CARTESIAN_POINT('Ctrl Pts',(-23.,39.8371685740842,2.));
#84226=CARTESIAN_POINT('Ctrl Pts',(-25.2470089260756,38.797525254077,2.));
#84227=CARTESIAN_POINT('Ctrl Pts',(-27.4022761516233,37.5810556243015,2.));
#84228=CARTESIAN_POINT('Ctrl Pts',(-29.4485343857591,36.2031892014269,2.));
#84229=CARTESIAN_POINT('Ctrl Pts',(-8.50876070567958,48.2555798975982,0.));
#84230=CARTESIAN_POINT('Ctrl Pts',(-8.50876070567958,48.2555798975982,20.));
#84231=CARTESIAN_POINT('Ctrl Pts',(-8.50201591146282,48.2561497089132,0.));
#84232=CARTESIAN_POINT('Ctrl Pts',(-8.50201591146282,48.2561497089132,20.));
#84233=CARTESIAN_POINT('Ctrl Pts',(-8.48852624368609,48.2572870022174,0.));
#84234=CARTESIAN_POINT('Ctrl Pts',(-8.48852624368609,48.2572870022174,20.));
#84235=CARTESIAN_POINT('Ctrl Pts',(-8.46829150399134,48.2589859541967,0.));
#84236=CARTESIAN_POINT('Ctrl Pts',(-8.46829150399134,48.2589859541967,20.));
#84237=CARTESIAN_POINT('Ctrl Pts',(-8.44131137500422,48.2612372475269,0.));
#84238=CARTESIAN_POINT('Ctrl Pts',(-8.44131137500422,48.2612372475269,20.));
#84239=CARTESIAN_POINT('Ctrl Pts',(-8.40758542126,48.2640280707484,0.));
#84240=CARTESIAN_POINT('Ctrl Pts',(-8.40758542126,48.2640280707484,20.));
#84241=CARTESIAN_POINT('Ctrl Pts',(-8.37385867778171,48.2667956002972,0.));
#84242=CARTESIAN_POINT('Ctrl Pts',(-8.37385867778171,48.2667956002972,20.));
#84243=CARTESIAN_POINT('Ctrl Pts',(-8.34013115014498,48.2695398358687,0.));
#84244=CARTESIAN_POINT('Ctrl Pts',(-8.34013115014498,48.2695398358687,20.));
#84245=CARTESIAN_POINT('Ctrl Pts',(-8.30640284761837,48.2722607770974,0.));
#84246=CARTESIAN_POINT('Ctrl Pts',(-8.30640284761837,48.2722607770974,20.));
#84247=CARTESIAN_POINT('Ctrl Pts',(-8.2726737841987,48.274958423567,0.));
#84248=CARTESIAN_POINT('Ctrl Pts',(-8.2726737841987,48.274958423567,20.));
#84249=CARTESIAN_POINT('Ctrl Pts',(-8.23894397736023,48.2776327748283,0.));
#84250=CARTESIAN_POINT('Ctrl Pts',(-8.23894397736023,48.2776327748283,20.));
#84251=CARTESIAN_POINT('Ctrl Pts',(-8.20521344665195,48.2802838304168,0.));
#84252=CARTESIAN_POINT('Ctrl Pts',(-8.20521344665195,48.2802838304168,20.));
#84253=CARTESIAN_POINT('Ctrl Pts',(-8.17148221231955,48.2829115898716,0.));
#84254=CARTESIAN_POINT('Ctrl Pts',(-8.17148221231955,48.2829115898716,20.));
#84255=CARTESIAN_POINT('Ctrl Pts',(-8.13775029398595,48.2855160527521,0.));
#84256=CARTESIAN_POINT('Ctrl Pts',(-8.13775029398595,48.2855160527521,20.));
#84257=CARTESIAN_POINT('Ctrl Pts',(-8.10401770912493,48.288097218659,0.));
#84258=CARTESIAN_POINT('Ctrl Pts',(-8.10401770912493,48.288097218659,20.));
#84259=CARTESIAN_POINT('Ctrl Pts',(-8.07028447346159,48.2906550872281,0.));
#84260=CARTESIAN_POINT('Ctrl Pts',(-8.07028447346159,48.2906550872281,20.));
#84261=CARTESIAN_POINT('Ctrl Pts',(-8.03655060167525,48.2931896581208,0.));
#84262=CARTESIAN_POINT('Ctrl Pts',(-8.03655060167525,48.2931896581208,20.));
#84263=CARTESIAN_POINT('Ctrl Pts',(-8.00281610801474,48.2957009310153,0.));
#84264=CARTESIAN_POINT('Ctrl Pts',(-8.00281610801474,48.2957009310153,20.));
#84265=CARTESIAN_POINT('Ctrl Pts',(-7.96908100690894,48.2981889055984,0.));
#84266=CARTESIAN_POINT('Ctrl Pts',(-7.96908100690894,48.2981889055984,20.));
#84267=CARTESIAN_POINT('Ctrl Pts',(-7.93534531368691,48.300653581555,0.));
#84268=CARTESIAN_POINT('Ctrl Pts',(-7.93534531368691,48.300653581555,20.));
#84269=CARTESIAN_POINT('Ctrl Pts',(-7.90160904447353,48.3030949585702,0.));
#84270=CARTESIAN_POINT('Ctrl Pts',(-7.90160904447353,48.3030949585702,20.));
#84271=CARTESIAN_POINT('Ctrl Pts',(-7.86787221586447,48.3055130363337,0.));
#84272=CARTESIAN_POINT('Ctrl Pts',(-7.86787221586447,48.3055130363337,20.));
#84273=CARTESIAN_POINT('Ctrl Pts',(-7.83413484466695,48.3079078145432,0.));
#84274=CARTESIAN_POINT('Ctrl Pts',(-7.83413484466695,48.3079078145432,20.));
#84275=CARTESIAN_POINT('Ctrl Pts',(-7.80039694763398,48.3102792929086,0.));
#84276=CARTESIAN_POINT('Ctrl Pts',(-7.80039694763398,48.3102792929086,20.));
#84277=CARTESIAN_POINT('Ctrl Pts',(-7.76665854114747,48.3126274711557,0.));
#84278=CARTESIAN_POINT('Ctrl Pts',(-7.76665854114747,48.3126274711557,20.));
#84279=CARTESIAN_POINT('Ctrl Pts',(-7.7329196412329,48.3149523490266,0.));
#84280=CARTESIAN_POINT('Ctrl Pts',(-7.7329196412329,48.3149523490266,20.));
#84281=CARTESIAN_POINT('Ctrl Pts',(-7.69918026370737,48.3172539262766,0.));
#84282=CARTESIAN_POINT('Ctrl Pts',(-7.69918026370737,48.3172539262766,20.));
#84283=CARTESIAN_POINT('Ctrl Pts',(-7.66544042428834,48.3195322026739,0.));
#84284=CARTESIAN_POINT('Ctrl Pts',(-7.66544042428834,48.3195322026739,20.));
#84285=CARTESIAN_POINT('Ctrl Pts',(-7.63170013870894,48.3217871779975,0.));
#84286=CARTESIAN_POINT('Ctrl Pts',(-7.63170013870894,48.3217871779975,20.));
#84287=CARTESIAN_POINT('Ctrl Pts',(-7.59795942285541,48.3240188520354,0.));
#84288=CARTESIAN_POINT('Ctrl Pts',(-7.59795942285541,48.3240188520354,20.));
#84289=CARTESIAN_POINT('Ctrl Pts',(-7.56421829277371,48.3262272245847,0.));
#84290=CARTESIAN_POINT('Ctrl Pts',(-7.56421829277371,48.3262272245847,20.));
#84291=CARTESIAN_POINT('Ctrl Pts',(-7.53047676460328,48.328412295452,0.));
#84292=CARTESIAN_POINT('Ctrl Pts',(-7.53047676460328,48.328412295452,20.));
#84293=CARTESIAN_POINT('Ctrl Pts',(-7.4967348545312,48.3305740644544,0.));
#84294=CARTESIAN_POINT('Ctrl Pts',(-7.4967348545312,48.3305740644544,20.));
#84295=CARTESIAN_POINT('Ctrl Pts',(-7.4629925787421,48.3327125314199,0.));
#84296=CARTESIAN_POINT('Ctrl Pts',(-7.4629925787421,48.3327125314199,20.));
#84297=CARTESIAN_POINT('Ctrl Pts',(-7.42924995335919,48.3348276961881,0.));
#84298=CARTESIAN_POINT('Ctrl Pts',(-7.42924995335919,48.3348276961881,20.));
#84299=CARTESIAN_POINT('Ctrl Pts',(-7.39550699443534,48.3369195586108,0.));
#84300=CARTESIAN_POINT('Ctrl Pts',(-7.39550699443534,48.3369195586108,20.));
#84301=CARTESIAN_POINT('Ctrl Pts',(-7.36176371798263,48.3389881185516,0.));
#84302=CARTESIAN_POINT('Ctrl Pts',(-7.36176371798263,48.3389881185516,20.));
#84303=CARTESIAN_POINT('Ctrl Pts',(-7.32802013999148,48.3410333758855,0.));
#84304=CARTESIAN_POINT('Ctrl Pts',(-7.32802013999148,48.3410333758855,20.));
#84305=CARTESIAN_POINT('Ctrl Pts',(-7.2942762764527,48.3430553304987,0.));
#84306=CARTESIAN_POINT('Ctrl Pts',(-7.2942762764527,48.3430553304987,20.));
#84307=CARTESIAN_POINT('Ctrl Pts',(-7.26053214338257,48.3450539822883,0.));
#84308=CARTESIAN_POINT('Ctrl Pts',(-7.26053214338257,48.3450539822883,20.));
#84309=CARTESIAN_POINT('Ctrl Pts',(-7.22678775682933,48.3470293311619,0.));
#84310=CARTESIAN_POINT('Ctrl Pts',(-7.22678775682933,48.3470293311619,20.));
#84311=CARTESIAN_POINT('Ctrl Pts',(-7.19304313285999,48.3489813770376,0.));
#84312=CARTESIAN_POINT('Ctrl Pts',(-7.19304313285999,48.3489813770376,20.));
#84313=CARTESIAN_POINT('Ctrl Pts',(-7.15929828755241,48.3509101198447,0.));
#84314=CARTESIAN_POINT('Ctrl Pts',(-7.15929828755241,48.3509101198447,20.));
#84315=CARTESIAN_POINT('Ctrl Pts',(-7.12555323698551,48.3528155595232,0.));
#84316=CARTESIAN_POINT('Ctrl Pts',(-7.12555323698551,48.3528155595232,20.));
#84317=CARTESIAN_POINT('Ctrl Pts',(-7.09180799722882,48.354697696024,0.));
#84318=CARTESIAN_POINT('Ctrl Pts',(-7.09180799722882,48.354697696024,20.));
#84319=CARTESIAN_POINT('Ctrl Pts',(-7.05806258433803,48.3565565293095,0.));
#84320=CARTESIAN_POINT('Ctrl Pts',(-7.05806258433803,48.3565565293095,20.));
#84321=CARTESIAN_POINT('Ctrl Pts',(-7.02431701436127,48.3583920593534,0.));
#84322=CARTESIAN_POINT('Ctrl Pts',(-7.02431701436127,48.3583920593534,20.));
#84323=CARTESIAN_POINT('Ctrl Pts',(-6.99057130334228,48.3602042861407,0.));
#84324=CARTESIAN_POINT('Ctrl Pts',(-6.99057130334228,48.3602042861407,20.));
#84325=CARTESIAN_POINT('Ctrl Pts',(-6.95682546732485,48.3619932096677,0.));
#84326=CARTESIAN_POINT('Ctrl Pts',(-6.95682546732485,48.3619932096677,20.));
#84327=CARTESIAN_POINT('Ctrl Pts',(-6.9230795223571,48.3637588299416,0.));
#84328=CARTESIAN_POINT('Ctrl Pts',(-6.9230795223571,48.3637588299416,20.));
#84329=CARTESIAN_POINT('Ctrl Pts',(-6.88933348449371,48.3655011469807,0.));
#84330=CARTESIAN_POINT('Ctrl Pts',(-6.88933348449371,48.3655011469807,20.));
#84331=CARTESIAN_POINT('Ctrl Pts',(-6.8555873697933,48.3672201608141,0.));
#84332=CARTESIAN_POINT('Ctrl Pts',(-6.8555873697933,48.3672201608141,20.));
#84333=CARTESIAN_POINT('Ctrl Pts',(-6.82184119431719,48.3689158714816,0.));
#84334=CARTESIAN_POINT('Ctrl Pts',(-6.82184119431719,48.3689158714816,20.));
#84335=CARTESIAN_POINT('Ctrl Pts',(-6.78809497412715,48.370588279034,0.));
#84336=CARTESIAN_POINT('Ctrl Pts',(-6.78809497412715,48.370588279034,20.));
#84337=CARTESIAN_POINT('Ctrl Pts',(-6.75434872528386,48.3722373835335,0.));
#84338=CARTESIAN_POINT('Ctrl Pts',(-6.75434872528386,48.3722373835335,20.));
#84339=CARTESIAN_POINT('Ctrl Pts',(-6.72060246384581,48.3738631850533,0.));
#84340=CARTESIAN_POINT('Ctrl Pts',(-6.72060246384581,48.3738631850533,20.));
#84341=CARTESIAN_POINT('Ctrl Pts',(-6.68685620587016,48.3754656836776,0.));
#84342=CARTESIAN_POINT('Ctrl Pts',(-6.68685620587016,48.3754656836776,20.));
#84343=CARTESIAN_POINT('Ctrl Pts',(-6.65310996741334,48.3770448795022,0.));
#84344=CARTESIAN_POINT('Ctrl Pts',(-6.65310996741334,48.3770448795022,20.));
#84345=CARTESIAN_POINT('Ctrl Pts',(-6.61936376453196,48.3786007726338,0.));
#84346=CARTESIAN_POINT('Ctrl Pts',(-6.61936376453196,48.3786007726338,20.));
#84347=CARTESIAN_POINT('Ctrl Pts',(-6.58561761328368,48.3801333631899,0.));
#84348=CARTESIAN_POINT('Ctrl Pts',(-6.58561761328368,48.3801333631899,20.));
#84349=CARTESIAN_POINT('Ctrl Pts',(-6.55187152972773,48.3816426512994,0.));
#84350=CARTESIAN_POINT('Ctrl Pts',(-6.55187152972773,48.3816426512994,20.));
#84351=CARTESIAN_POINT('Ctrl Pts',(-6.51812552992425,48.3831286371024,0.));
#84352=CARTESIAN_POINT('Ctrl Pts',(-6.51812552992425,48.3831286371024,20.));
#84353=CARTESIAN_POINT('Ctrl Pts',(-6.48437962993407,48.3845913207494,0.));
#84354=CARTESIAN_POINT('Ctrl Pts',(-6.48437962993407,48.3845913207494,20.));
#84355=CARTESIAN_POINT('Ctrl Pts',(-6.45063384581846,48.3860307024022,0.));
#84356=CARTESIAN_POINT('Ctrl Pts',(-6.45063384581846,48.3860307024022,20.));
#84357=CARTESIAN_POINT('Ctrl Pts',(-6.41688819363866,48.3874467822337,0.));
#84358=CARTESIAN_POINT('Ctrl Pts',(-6.41688819363866,48.3874467822337,20.));
#84359=CARTESIAN_POINT('Ctrl Pts',(-6.38314268945589,48.388839560428,0.));
#84360=CARTESIAN_POINT('Ctrl Pts',(-6.38314268945589,48.388839560428,20.));
#84361=CARTESIAN_POINT('Ctrl Pts',(-6.34939734933123,48.3902090371802,0.));
#84362=CARTESIAN_POINT('Ctrl Pts',(-6.34939734933123,48.3902090371802,20.));
#84363=CARTESIAN_POINT('Ctrl Pts',(-6.3156521893259,48.3915552126968,0.));
#84364=CARTESIAN_POINT('Ctrl Pts',(-6.3156521893259,48.3915552126968,20.));
#84365=CARTESIAN_POINT('Ctrl Pts',(-6.28190722550134,48.3928780871951,0.));
#84366=CARTESIAN_POINT('Ctrl Pts',(-6.28190722550134,48.3928780871951,20.));
#84367=CARTESIAN_POINT('Ctrl Pts',(-6.24816247391921,48.3941776609035,0.));
#84368=CARTESIAN_POINT('Ctrl Pts',(-6.24816247391921,48.3941776609035,20.));
#84369=CARTESIAN_POINT('Ctrl Pts',(-6.21441795064169,48.3954539340615,0.));
#84370=CARTESIAN_POINT('Ctrl Pts',(-6.21441795064169,48.3954539340615,20.));
#84371=CARTESIAN_POINT('Ctrl Pts',(-6.18067367173125,48.3967069069196,0.));
#84372=CARTESIAN_POINT('Ctrl Pts',(-6.18067367173125,48.3967069069196,20.));
#84373=CARTESIAN_POINT('Ctrl Pts',(-6.1469296532508,48.3979365797396,0.));
#84374=CARTESIAN_POINT('Ctrl Pts',(-6.1469296532508,48.3979365797396,20.));
#84375=CARTESIAN_POINT('Ctrl Pts',(-6.11318591126344,48.3991429527941,0.));
#84376=CARTESIAN_POINT('Ctrl Pts',(-6.11318591126344,48.3991429527941,20.));
#84377=CARTESIAN_POINT('Ctrl Pts',(-6.07944246183268,48.400326026367,0.));
#84378=CARTESIAN_POINT('Ctrl Pts',(-6.07944246183268,48.400326026367,20.));
#84379=CARTESIAN_POINT('Ctrl Pts',(-6.04569932102201,48.4014858007534,0.));
#84380=CARTESIAN_POINT('Ctrl Pts',(-6.04569932102201,48.4014858007534,20.));
#84381=CARTESIAN_POINT('Ctrl Pts',(-6.01195650489506,48.4026222762592,0.));
#84382=CARTESIAN_POINT('Ctrl Pts',(-6.01195650489506,48.4026222762592,20.));
#84383=CARTESIAN_POINT('Ctrl Pts',(-5.97821402951549,48.4037354532013,0.));
#84384=CARTESIAN_POINT('Ctrl Pts',(-5.97821402951549,48.4037354532013,20.));
#84385=CARTESIAN_POINT('Ctrl Pts',(-5.94447191094723,48.404825331908,0.));
#84386=CARTESIAN_POINT('Ctrl Pts',(-5.94447191094723,48.404825331908,20.));
#84387=CARTESIAN_POINT('Ctrl Pts',(-5.91073016525427,48.4058919127185,0.));
#84388=CARTESIAN_POINT('Ctrl Pts',(-5.91073016525427,48.4058919127185,20.));
#84389=CARTESIAN_POINT('Ctrl Pts',(-5.87698880850096,48.4069351959835,0.));
#84390=CARTESIAN_POINT('Ctrl Pts',(-5.87698880850096,48.4069351959835,20.));
#84391=CARTESIAN_POINT('Ctrl Pts',(-5.8432478567519,48.4079551820642,0.));
#84392=CARTESIAN_POINT('Ctrl Pts',(-5.8432478567519,48.4079551820642,20.));
#84393=CARTESIAN_POINT('Ctrl Pts',(-5.80950732607179,48.4089518713336,0.));
#84394=CARTESIAN_POINT('Ctrl Pts',(-5.80950732607179,48.4089518713336,20.));
#84395=CARTESIAN_POINT('Ctrl Pts',(-5.77576723252553,48.4099252641753,0.));
#84396=CARTESIAN_POINT('Ctrl Pts',(-5.77576723252553,48.4099252641753,20.));
#84397=CARTESIAN_POINT('Ctrl Pts',(-5.74202759217814,48.4108753609837,0.));
#84398=CARTESIAN_POINT('Ctrl Pts',(-5.74202759217814,48.4108753609837,20.));
#84399=CARTESIAN_POINT('Ctrl Pts',(-5.70828842109461,48.4118021621647,0.));
#84400=CARTESIAN_POINT('Ctrl Pts',(-5.70828842109461,48.4118021621647,20.));
#84401=CARTESIAN_POINT('Ctrl Pts',(-5.67454973534015,48.412705668135,0.));
#84402=CARTESIAN_POINT('Ctrl Pts',(-5.67454973534015,48.412705668135,20.));
#84403=CARTESIAN_POINT('Ctrl Pts',(-5.64081155098006,48.4135858793227,0.));
#84404=CARTESIAN_POINT('Ctrl Pts',(-5.64081155098006,48.4135858793227,20.));
#84405=CARTESIAN_POINT('Ctrl Pts',(-5.60707388407982,48.414442796167,0.));
#84406=CARTESIAN_POINT('Ctrl Pts',(-5.60707388407982,48.414442796167,20.));
#84407=CARTESIAN_POINT('Ctrl Pts',(-5.57333675070493,48.4152764191183,0.));
#84408=CARTESIAN_POINT('Ctrl Pts',(-5.57333675070493,48.4152764191183,20.));
#84409=CARTESIAN_POINT('Ctrl Pts',(-5.53960016692118,48.4160867486381,0.));
#84410=CARTESIAN_POINT('Ctrl Pts',(-5.53960016692118,48.4160867486381,20.));
#84411=CARTESIAN_POINT('Ctrl Pts',(-5.50586414879431,48.4168737851989,0.));
#84412=CARTESIAN_POINT('Ctrl Pts',(-5.50586414879431,48.4168737851989,20.));
#84413=CARTESIAN_POINT('Ctrl Pts',(-5.47212871239031,48.417637529284,0.));
#84414=CARTESIAN_POINT('Ctrl Pts',(-5.47212871239031,48.417637529284,20.));
#84415=CARTESIAN_POINT('Ctrl Pts',(-5.43839387377499,48.4183779813881,0.));
#84416=CARTESIAN_POINT('Ctrl Pts',(-5.43839387377499,48.4183779813881,20.));
#84417=CARTESIAN_POINT('Ctrl Pts',(-5.40465964901426,48.4190951420167,0.));
#84418=CARTESIAN_POINT('Ctrl Pts',(-5.40465964901426,48.4190951420167,20.));
#84419=CARTESIAN_POINT('Ctrl Pts',(-5.37092605417403,48.4197890116867,0.));
#84420=CARTESIAN_POINT('Ctrl Pts',(-5.37092605417403,48.4197890116867,20.));
#84421=CARTESIAN_POINT('Ctrl Pts',(-5.33719310532028,48.4204595909261,0.));
#84422=CARTESIAN_POINT('Ctrl Pts',(-5.33719310532028,48.4204595909261,20.));
#84423=CARTESIAN_POINT('Ctrl Pts',(-5.3034608185191,48.4211068802741,0.));
#84424=CARTESIAN_POINT('Ctrl Pts',(-5.3034608185191,48.4211068802741,20.));
#84425=CARTESIAN_POINT('Ctrl Pts',(-5.26972920983671,48.4217308802807,0.));
#84426=CARTESIAN_POINT('Ctrl Pts',(-5.26972920983671,48.4217308802807,20.));
#84427=CARTESIAN_POINT('Ctrl Pts',(-5.23599829533945,48.4223315915069,0.));
#84428=CARTESIAN_POINT('Ctrl Pts',(-5.23599829533945,48.4223315915069,20.));
#84429=CARTESIAN_POINT('Ctrl Pts',(-5.20226809109352,48.4229090145253,0.));
#84430=CARTESIAN_POINT('Ctrl Pts',(-5.20226809109352,48.4229090145253,20.));
#84431=CARTESIAN_POINT('Ctrl Pts',(-5.16853861316522,48.4234631499193,0.));
#84432=CARTESIAN_POINT('Ctrl Pts',(-5.16853861316522,48.4234631499193,20.));
#84433=CARTESIAN_POINT('Ctrl Pts',(-5.13480987762072,48.4239939982838,0.));
#84434=CARTESIAN_POINT('Ctrl Pts',(-5.13480987762072,48.4239939982838,20.));
#84435=CARTESIAN_POINT('Ctrl Pts',(-5.10108190052608,48.4245015602246,0.));
#84436=CARTESIAN_POINT('Ctrl Pts',(-5.10108190052608,48.4245015602246,20.));
#84437=CARTESIAN_POINT('Ctrl Pts',(-5.06735469794743,48.4249858363582,0.));
#84438=CARTESIAN_POINT('Ctrl Pts',(-5.06735469794743,48.4249858363582,20.));
#84439=CARTESIAN_POINT('Ctrl Pts',(-5.03362828595094,48.4254468273122,0.));
#84440=CARTESIAN_POINT('Ctrl Pts',(-5.03362828595094,48.4254468273122,20.));
#84441=CARTESIAN_POINT('Ctrl Pts',(-4.99990268060293,48.4258845337255,0.));
#84442=CARTESIAN_POINT('Ctrl Pts',(-4.99990268060293,48.4258845337255,20.));
#84443=CARTESIAN_POINT('Ctrl Pts',(-4.96617789796954,48.4262989562483,0.));
#84444=CARTESIAN_POINT('Ctrl Pts',(-4.96617789796954,48.4262989562483,20.));
#84445=CARTESIAN_POINT('Ctrl Pts',(-4.93245395411686,48.4266900955418,0.));
#84446=CARTESIAN_POINT('Ctrl Pts',(-4.93245395411686,48.4266900955418,20.));
#84447=CARTESIAN_POINT('Ctrl Pts',(-4.89873086511077,48.4270579522784,0.));
#84448=CARTESIAN_POINT('Ctrl Pts',(-4.89873086511077,48.4270579522784,20.));
#84449=CARTESIAN_POINT('Ctrl Pts',(-4.86500864701731,48.4274025271416,0.));
#84450=CARTESIAN_POINT('Ctrl Pts',(-4.86500864701731,48.4274025271416,20.));
#84451=CARTESIAN_POINT('Ctrl Pts',(-4.8312873159023,48.4277238208263,0.));
#84452=CARTESIAN_POINT('Ctrl Pts',(-4.8312873159023,48.4277238208263,20.));
#84453=CARTESIAN_POINT('Ctrl Pts',(-4.79756688783169,48.4280218340382,0.));
#84454=CARTESIAN_POINT('Ctrl Pts',(-4.79756688783169,48.4280218340382,20.));
#84455=CARTESIAN_POINT('Ctrl Pts',(-4.76384737887107,48.4282965674942,0.));
#84456=CARTESIAN_POINT('Ctrl Pts',(-4.76384737887107,48.4282965674942,20.));
#84457=CARTESIAN_POINT('Ctrl Pts',(-4.73012880508602,48.4285480219221,0.));
#84458=CARTESIAN_POINT('Ctrl Pts',(-4.73012880508602,48.4285480219221,20.));
#84459=CARTESIAN_POINT('Ctrl Pts',(-4.69641118254227,48.4287761980604,0.));
#84460=CARTESIAN_POINT('Ctrl Pts',(-4.69641118254227,48.4287761980604,20.));
#84461=CARTESIAN_POINT('Ctrl Pts',(-4.66269452730544,48.4289810966589,0.));
#84462=CARTESIAN_POINT('Ctrl Pts',(-4.66269452730544,48.4289810966589,20.));
#84463=CARTESIAN_POINT('Ctrl Pts',(-4.62897885544098,48.4291627184787,0.));
#84464=CARTESIAN_POINT('Ctrl Pts',(-4.62897885544098,48.4291627184787,20.));
#84465=CARTESIAN_POINT('Ctrl Pts',(-4.5952641830141,48.4293210642923,0.));
#84466=CARTESIAN_POINT('Ctrl Pts',(-4.5952641830141,48.4293210642923,20.));
#84467=CARTESIAN_POINT('Ctrl Pts',(-4.56155052608981,48.4294561348833,0.));
#84468=CARTESIAN_POINT('Ctrl Pts',(-4.56155052608981,48.4294561348833,20.));
#84469=CARTESIAN_POINT('Ctrl Pts',(-4.52783790073295,48.4295679310466,0.));
#84470=CARTESIAN_POINT('Ctrl Pts',(-4.52783790073295,48.4295679310466,20.));
#84471=CARTESIAN_POINT('Ctrl Pts',(-4.49412632300816,48.4296564535884,0.));
#84472=CARTESIAN_POINT('Ctrl Pts',(-4.49412632300816,48.4296564535884,20.));
#84473=CARTESIAN_POINT('Ctrl Pts',(-4.46041580898013,48.4297217033257,0.));
#84474=CARTESIAN_POINT('Ctrl Pts',(-4.46041580898013,48.4297217033257,20.));
#84475=CARTESIAN_POINT('Ctrl Pts',(-4.42670637471342,48.4297636810863,0.));
#84476=CARTESIAN_POINT('Ctrl Pts',(-4.42670637471342,48.4297636810863,20.));
#84477=CARTESIAN_POINT('Ctrl Pts',(-4.39299803627247,48.4297823877088,0.));
#84478=CARTESIAN_POINT('Ctrl Pts',(-4.39299803627247,48.4297823877088,20.));
#84479=CARTESIAN_POINT('Ctrl Pts',(-4.35929080972167,48.4297778240431,0.));
#84480=CARTESIAN_POINT('Ctrl Pts',(-4.35929080972167,48.4297778240431,20.));
#84481=CARTESIAN_POINT('Ctrl Pts',(-4.32558471112518,48.42974999095,0.));
#84482=CARTESIAN_POINT('Ctrl Pts',(-4.32558471112518,48.42974999095,20.));
#84483=CARTESIAN_POINT('Ctrl Pts',(-4.29187975654678,48.4296988893018,0.));
#84484=CARTESIAN_POINT('Ctrl Pts',(-4.29187975654678,48.4296988893018,20.));
#84485=CARTESIAN_POINT('Ctrl Pts',(-4.25817596205002,48.4296245199823,0.));
#84486=CARTESIAN_POINT('Ctrl Pts',(-4.25817596205002,48.4296245199823,20.));
#84487=CARTESIAN_POINT('Ctrl Pts',(-4.22447334369802,48.4295268838864,0.));
#84488=CARTESIAN_POINT('Ctrl Pts',(-4.22447334369802,48.4295268838864,20.));
#84489=CARTESIAN_POINT('Ctrl Pts',(-4.19077191755407,48.4294059819202,0.));
#84490=CARTESIAN_POINT('Ctrl Pts',(-4.19077191755407,48.4294059819202,20.));
#84491=CARTESIAN_POINT('Ctrl Pts',(-4.15707169968116,48.4292618150011,0.));
#84492=CARTESIAN_POINT('Ctrl Pts',(-4.15707169968116,48.4292618150011,20.));
#84493=CARTESIAN_POINT('Ctrl Pts',(-4.12337270614212,48.429094384057,0.));
#84494=CARTESIAN_POINT('Ctrl Pts',(-4.12337270614212,48.429094384057,20.));
#84495=CARTESIAN_POINT('Ctrl Pts',(-4.08967495299953,48.4289036900268,0.));
#84496=CARTESIAN_POINT('Ctrl Pts',(-4.08967495299953,48.4289036900268,20.));
#84497=CARTESIAN_POINT('Ctrl Pts',(-4.0559784563157,48.4286897338604,0.));
#84498=CARTESIAN_POINT('Ctrl Pts',(-4.0559784563157,48.4286897338604,20.));
#84499=CARTESIAN_POINT('Ctrl Pts',(-4.02228323215261,48.4284525165189,0.));
#84500=CARTESIAN_POINT('Ctrl Pts',(-4.02228323215261,48.4284525165189,20.));
#84501=CARTESIAN_POINT('Ctrl Pts',(-3.98858929657202,48.4281920389749,0.));
#84502=CARTESIAN_POINT('Ctrl Pts',(-3.98858929657202,48.4281920389749,20.));
#84503=CARTESIAN_POINT('Ctrl Pts',(-3.9548966656355,48.427908302212,0.));
#84504=CARTESIAN_POINT('Ctrl Pts',(-3.9548966656355,48.427908302212,20.));
#84505=CARTESIAN_POINT('Ctrl Pts',(-3.92120535540421,48.4276013072253,0.));
#84506=CARTESIAN_POINT('Ctrl Pts',(-3.92120535540421,48.4276013072253,20.));
#84507=CARTESIAN_POINT('Ctrl Pts',(-3.88751538193921,48.4272710550206,0.));
#84508=CARTESIAN_POINT('Ctrl Pts',(-3.88751538193921,48.4272710550206,20.));
#84509=CARTESIAN_POINT('Ctrl Pts',(-3.85382676130116,48.4269175466151,0.));
#84510=CARTESIAN_POINT('Ctrl Pts',(-3.85382676130116,48.4269175466151,20.));
#84511=CARTESIAN_POINT('Ctrl Pts',(-3.82013950955044,48.4265407830367,0.));
#84512=CARTESIAN_POINT('Ctrl Pts',(-3.82013950955044,48.4265407830367,20.));
#84513=CARTESIAN_POINT('Ctrl Pts',(-3.78645364274707,48.4261407653249,0.));
#84514=CARTESIAN_POINT('Ctrl Pts',(-3.78645364274707,48.4261407653249,20.));
#84515=CARTESIAN_POINT('Ctrl Pts',(-3.75276917695086,48.4257174945299,0.));
#84516=CARTESIAN_POINT('Ctrl Pts',(-3.75276917695086,48.4257174945299,20.));
#84517=CARTESIAN_POINT('Ctrl Pts',(-3.7190861282211,48.4252709717129,0.));
#84518=CARTESIAN_POINT('Ctrl Pts',(-3.7190861282211,48.4252709717129,20.));
#84519=CARTESIAN_POINT('Ctrl Pts',(-3.68540451261697,48.424801197947,0.));
#84520=CARTESIAN_POINT('Ctrl Pts',(-3.68540451261697,48.424801197947,20.));
#84521=CARTESIAN_POINT('Ctrl Pts',(-3.65172434619742,48.4243081743158,0.));
#84522=CARTESIAN_POINT('Ctrl Pts',(-3.65172434619742,48.4243081743158,20.));
#84523=CARTESIAN_POINT('Ctrl Pts',(-3.61804564502098,48.4237919019141,0.));
#84524=CARTESIAN_POINT('Ctrl Pts',(-3.61804564502098,48.4237919019141,20.));
#84525=CARTESIAN_POINT('Ctrl Pts',(-3.58436842514565,48.4232523818483,0.));
#84526=CARTESIAN_POINT('Ctrl Pts',(-3.58436842514565,48.4232523818483,20.));
#84527=CARTESIAN_POINT('Ctrl Pts',(-3.55069270262909,48.4226896152354,0.));
#84528=CARTESIAN_POINT('Ctrl Pts',(-3.55069270262909,48.4226896152354,20.));
#84529=CARTESIAN_POINT('Ctrl Pts',(-3.51701849352855,48.422103603204,0.));
#84530=CARTESIAN_POINT('Ctrl Pts',(-3.51701849352855,48.422103603204,20.));
#84531=CARTESIAN_POINT('Ctrl Pts',(-3.48334581390102,48.4214943468927,0.));
#84532=CARTESIAN_POINT('Ctrl Pts',(-3.48334581390102,48.4214943468927,20.));
#84533=CARTESIAN_POINT('Ctrl Pts',(-3.44967467980324,48.4208618474523,0.));
#84534=CARTESIAN_POINT('Ctrl Pts',(-3.44967467980324,48.4208618474523,20.));
#84535=CARTESIAN_POINT('Ctrl Pts',(-3.4160051072915,48.4202061060442,0.));
#84536=CARTESIAN_POINT('Ctrl Pts',(-3.4160051072915,48.4202061060442,20.));
#84537=CARTESIAN_POINT('Ctrl Pts',(-3.38233711242168,48.4195271238417,0.));
#84538=CARTESIAN_POINT('Ctrl Pts',(-3.38233711242168,48.4195271238417,20.));
#84539=CARTESIAN_POINT('Ctrl Pts',(-3.34867071124919,48.4188249020284,0.));
#84540=CARTESIAN_POINT('Ctrl Pts',(-3.34867071124919,48.4188249020284,20.));
#84541=CARTESIAN_POINT('Ctrl Pts',(-3.31500591982889,48.4180994417999,0.));
#84542=CARTESIAN_POINT('Ctrl Pts',(-3.31500591982889,48.4180994417999,20.));
#84543=CARTESIAN_POINT('Ctrl Pts',(-3.28134275421533,48.4173507443625,0.));
#84544=CARTESIAN_POINT('Ctrl Pts',(-3.28134275421533,48.4173507443625,20.));
#84545=CARTESIAN_POINT('Ctrl Pts',(-3.24768123046267,48.4165788109335,0.));
#84546=CARTESIAN_POINT('Ctrl Pts',(-3.24768123046267,48.4165788109335,20.));
#84547=CARTESIAN_POINT('Ctrl Pts',(-3.21402136462459,48.4157836427414,0.));
#84548=CARTESIAN_POINT('Ctrl Pts',(-3.21402136462459,48.4157836427414,20.));
#84549=CARTESIAN_POINT('Ctrl Pts',(-3.18036317275455,48.4149652410254,0.));
#84550=CARTESIAN_POINT('Ctrl Pts',(-3.18036317275455,48.4149652410254,20.));
#84551=CARTESIAN_POINT('Ctrl Pts',(-3.14670667090557,48.414123607036,0.));
#84552=CARTESIAN_POINT('Ctrl Pts',(-3.14670667090557,48.414123607036,20.));
#84553=CARTESIAN_POINT('Ctrl Pts',(-3.11305187513001,48.4132587420349,0.));
#84554=CARTESIAN_POINT('Ctrl Pts',(-3.11305187513001,48.4132587420349,20.));
#84555=CARTESIAN_POINT('Ctrl Pts',(-3.0793988014797,48.4123706472953,0.));
#84556=CARTESIAN_POINT('Ctrl Pts',(-3.0793988014797,48.4123706472953,20.));
#84557=CARTESIAN_POINT('Ctrl Pts',(-3.04574746600609,48.4114593241014,0.));
#84558=CARTESIAN_POINT('Ctrl Pts',(-3.04574746600609,48.4114593241014,20.));
#84559=CARTESIAN_POINT('Ctrl Pts',(-3.01209788475996,48.4105247737488,0.));
#84560=CARTESIAN_POINT('Ctrl Pts',(-3.01209788475996,48.4105247737488,20.));
#84561=CARTESIAN_POINT('Ctrl Pts',(-2.97845007379182,48.4095669975441,0.));
#84562=CARTESIAN_POINT('Ctrl Pts',(-2.97845007379182,48.4095669975441,20.));
#84563=CARTESIAN_POINT('Ctrl Pts',(-2.94480404915165,48.4085859968048,0.));
#84564=CARTESIAN_POINT('Ctrl Pts',(-2.94480404915165,48.4085859968048,20.));
#84565=CARTESIAN_POINT('Ctrl Pts',(-2.91115982688905,48.4075817728593,0.));
#84566=CARTESIAN_POINT('Ctrl Pts',(-2.91115982688905,48.4075817728593,20.));
#84567=CARTESIAN_POINT('Ctrl Pts',(-2.87751742305295,48.4065543270471,0.));
#84568=CARTESIAN_POINT('Ctrl Pts',(-2.87751742305295,48.4065543270471,20.));
#84569=CARTESIAN_POINT('Ctrl Pts',(-2.84387685369182,48.4055036607195,0.));
#84570=CARTESIAN_POINT('Ctrl Pts',(-2.84387685369182,48.4055036607195,20.));
#84571=CARTESIAN_POINT('Ctrl Pts',(-2.81023813485357,48.4044297752383,0.));
#84572=CARTESIAN_POINT('Ctrl Pts',(-2.81023813485357,48.4044297752383,20.));
#84573=CARTESIAN_POINT('Ctrl Pts',(-2.77660128258548,48.4033326719771,0.));
#84574=CARTESIAN_POINT('Ctrl Pts',(-2.77660128258548,48.4033326719771,20.));
#84575=CARTESIAN_POINT('Ctrl Pts',(-2.74296631293438,48.4022123523201,0.));
#84576=CARTESIAN_POINT('Ctrl Pts',(-2.74296631293438,48.4022123523201,20.));
#84577=CARTESIAN_POINT('Ctrl Pts',(-2.70933324194662,48.4010688176627,0.));
#84578=CARTESIAN_POINT('Ctrl Pts',(-2.70933324194662,48.4010688176627,20.));
#84579=CARTESIAN_POINT('Ctrl Pts',(-2.67570208566795,48.3999020694116,0.));
#84580=CARTESIAN_POINT('Ctrl Pts',(-2.67570208566795,48.3999020694116,20.));
#84581=CARTESIAN_POINT('Ctrl Pts',(-2.64207286014351,48.3987121089844,0.));
#84582=CARTESIAN_POINT('Ctrl Pts',(-2.64207286014351,48.3987121089844,20.));
#84583=CARTESIAN_POINT('Ctrl Pts',(-2.60844558141791,48.3974989378103,0.));
#84584=CARTESIAN_POINT('Ctrl Pts',(-2.60844558141791,48.3974989378103,20.));
#84585=CARTESIAN_POINT('Ctrl Pts',(-2.57482026553517,48.3962625573292,0.));
#84586=CARTESIAN_POINT('Ctrl Pts',(-2.57482026553517,48.3962625573292,20.));
#84587=CARTESIAN_POINT('Ctrl Pts',(-2.54119692853862,48.3950029689925,0.));
#84588=CARTESIAN_POINT('Ctrl Pts',(-2.54119692853862,48.3950029689925,20.));
#84589=CARTESIAN_POINT('Ctrl Pts',(-2.50757558647122,48.3937201742621,0.));
#84590=CARTESIAN_POINT('Ctrl Pts',(-2.50757558647122,48.3937201742621,20.));
#84591=CARTESIAN_POINT('Ctrl Pts',(-2.47395625537496,48.3924141746117,0.));
#84592=CARTESIAN_POINT('Ctrl Pts',(-2.47395625537496,48.3924141746117,20.));
#84593=CARTESIAN_POINT('Ctrl Pts',(-2.44033895129154,48.3910849715258,0.));
#84594=CARTESIAN_POINT('Ctrl Pts',(-2.44033895129154,48.3910849715258,20.));
#84595=CARTESIAN_POINT('Ctrl Pts',(-2.40672369026198,48.3897325665,0.));
#84596=CARTESIAN_POINT('Ctrl Pts',(-2.40672369026198,48.3897325665,20.));
#84597=CARTESIAN_POINT('Ctrl Pts',(-2.37311048832666,48.3883569610415,0.));
#84598=CARTESIAN_POINT('Ctrl Pts',(-2.37311048832666,48.3883569610415,20.));
#84599=CARTESIAN_POINT('Ctrl Pts',(-2.33949936152535,48.3869581566679,0.));
#84600=CARTESIAN_POINT('Ctrl Pts',(-2.33949936152535,48.3869581566679,20.));
#84601=CARTESIAN_POINT('Ctrl Pts',(-2.30589032589701,48.3855361549086,0.));
#84602=CARTESIAN_POINT('Ctrl Pts',(-2.30589032589701,48.3855361549086,20.));
#84603=CARTESIAN_POINT('Ctrl Pts',(-2.2722833974801,48.3840909573039,0.));
#84604=CARTESIAN_POINT('Ctrl Pts',(-2.2722833974801,48.3840909573039,20.));
#84605=CARTESIAN_POINT('Ctrl Pts',(-2.23867859231222,48.3826225654055,0.));
#84606=CARTESIAN_POINT('Ctrl Pts',(-2.23867859231222,48.3826225654055,20.));
#84607=CARTESIAN_POINT('Ctrl Pts',(-2.20507592643043,48.3811309807756,0.));
#84608=CARTESIAN_POINT('Ctrl Pts',(-2.20507592643043,48.3811309807756,20.));
#84609=CARTESIAN_POINT('Ctrl Pts',(-2.17147541587105,48.3796162049883,0.));
#84610=CARTESIAN_POINT('Ctrl Pts',(-2.17147541587105,48.3796162049883,20.));
#84611=CARTESIAN_POINT('Ctrl Pts',(-2.13787707667014,48.3780782396279,0.));
#84612=CARTESIAN_POINT('Ctrl Pts',(-2.13787707667014,48.3780782396279,20.));
#84613=CARTESIAN_POINT('Ctrl Pts',(-2.10428092486295,48.3765170862905,0.));
#84614=CARTESIAN_POINT('Ctrl Pts',(-2.10428092486295,48.3765170862905,20.));
#84615=CARTESIAN_POINT('Ctrl Pts',(-2.07068697648389,48.374932746583,0.));
#84616=CARTESIAN_POINT('Ctrl Pts',(-2.07068697648389,48.374932746583,20.));
#84617=CARTESIAN_POINT('Ctrl Pts',(-2.03709524756656,48.3733252221237,0.));
#84618=CARTESIAN_POINT('Ctrl Pts',(-2.03709524756656,48.3733252221237,20.));
#84619=CARTESIAN_POINT('Ctrl Pts',(-2.00350575414356,48.3716945145424,0.));
#84620=CARTESIAN_POINT('Ctrl Pts',(-2.00350575414356,48.3716945145424,20.));
#84621=CARTESIAN_POINT('Ctrl Pts',(-1.96991851224693,48.3700406254798,0.));
#84622=CARTESIAN_POINT('Ctrl Pts',(-1.96991851224693,48.3700406254798,20.));
#84623=CARTESIAN_POINT('Ctrl Pts',(-1.93633353790814,48.3683635565876,0.));
#84624=CARTESIAN_POINT('Ctrl Pts',(-1.93633353790814,48.3683635565876,20.));
#84625=CARTESIAN_POINT('Ctrl Pts',(-1.90275084715797,48.3666633095284,0.));
#84626=CARTESIAN_POINT('Ctrl Pts',(-1.90275084715797,48.3666633095284,20.));
#84627=CARTESIAN_POINT('Ctrl Pts',(-1.86917045602653,48.3649398859758,0.));
#84628=CARTESIAN_POINT('Ctrl Pts',(-1.86917045602653,48.3649398859758,20.));
#84629=CARTESIAN_POINT('Ctrl Pts',(-1.83559238054324,48.3631932876149,0.));
#84630=CARTESIAN_POINT('Ctrl Pts',(-1.83559238054324,48.3631932876149,20.));
#84631=CARTESIAN_POINT('Ctrl Pts',(-1.80201663673657,48.3614235161422,0.));
#84632=CARTESIAN_POINT('Ctrl Pts',(-1.80201663673657,48.3614235161422,20.));
#84633=CARTESIAN_POINT('Ctrl Pts',(-1.76844324063427,48.3596305732653,0.));
#84634=CARTESIAN_POINT('Ctrl Pts',(-1.76844324063427,48.3596305732653,20.));
#84635=CARTESIAN_POINT('Ctrl Pts',(-1.73487220826327,48.357814460703,0.));
#84636=CARTESIAN_POINT('Ctrl Pts',(-1.73487220826327,48.357814460703,20.));
#84637=CARTESIAN_POINT('Ctrl Pts',(-1.70130355564958,48.3559751801849,0.));
#84638=CARTESIAN_POINT('Ctrl Pts',(-1.70130355564958,48.3559751801849,20.));
#84639=CARTESIAN_POINT('Ctrl Pts',(-1.66773729881857,48.3541127334515,0.));
#84640=CARTESIAN_POINT('Ctrl Pts',(-1.66773729881857,48.3541127334515,20.));
#84641=CARTESIAN_POINT('Ctrl Pts',(-1.63417345379483,48.3522271222546,0.));
#84642=CARTESIAN_POINT('Ctrl Pts',(-1.63417345379483,48.3522271222546,20.));
#84643=CARTESIAN_POINT('Ctrl Pts',(-1.60061203660208,48.350318348357,0.));
#84644=CARTESIAN_POINT('Ctrl Pts',(-1.60061203660208,48.350318348357,20.));
#84645=CARTESIAN_POINT('Ctrl Pts',(-1.56705306326333,48.3483864135332,0.));
#84646=CARTESIAN_POINT('Ctrl Pts',(-1.56705306326333,48.3483864135332,20.));
#84647=CARTESIAN_POINT('Ctrl Pts',(-1.53349654980078,48.3464313195685,0.));
#84648=CARTESIAN_POINT('Ctrl Pts',(-1.53349654980078,48.3464313195685,20.));
#84649=CARTESIAN_POINT('Ctrl Pts',(-1.49994251223572,48.3444530682597,0.));
#84650=CARTESIAN_POINT('Ctrl Pts',(-1.49994251223572,48.3444530682597,20.));
#84651=CARTESIAN_POINT('Ctrl Pts',(-1.46639096658853,48.3424516614145,0.));
#84652=CARTESIAN_POINT('Ctrl Pts',(-1.46639096658853,48.3424516614145,20.));
#84653=CARTESIAN_POINT('Ctrl Pts',(-1.4328419288788,48.3404271008519,0.));
#84654=CARTESIAN_POINT('Ctrl Pts',(-1.4328419288788,48.3404271008519,20.));
#84655=CARTESIAN_POINT('Ctrl Pts',(-1.39929541512521,48.3383793884017,0.));
#84656=CARTESIAN_POINT('Ctrl Pts',(-1.39929541512521,48.3383793884017,20.));
#84657=CARTESIAN_POINT('Ctrl Pts',(-1.36575144134572,48.336308525905,0.));
#84658=CARTESIAN_POINT('Ctrl Pts',(-1.36575144134572,48.336308525905,20.));
#84659=CARTESIAN_POINT('Ctrl Pts',(-1.33221002355744,48.3342145152137,0.));
#84660=CARTESIAN_POINT('Ctrl Pts',(-1.33221002355744,48.3342145152137,20.));
#84661=CARTESIAN_POINT('Ctrl Pts',(-1.29867117777653,48.3320973581913,0.));
#84662=CARTESIAN_POINT('Ctrl Pts',(-1.29867117777653,48.3320973581913,20.));
#84663=CARTESIAN_POINT('Ctrl Pts',(-1.26513492001823,48.3299570567123,0.));
#84664=CARTESIAN_POINT('Ctrl Pts',(-1.26513492001823,48.3299570567123,20.));
#84665=CARTESIAN_POINT('Ctrl Pts',(-1.23160126629694,48.3277936126623,0.));
#84666=CARTESIAN_POINT('Ctrl Pts',(-1.23160126629694,48.3277936126623,20.));
#84667=CARTESIAN_POINT('Ctrl Pts',(-1.19807023262612,48.3256070279384,0.));
#84668=CARTESIAN_POINT('Ctrl Pts',(-1.19807023262612,48.3256070279384,20.));
#84669=CARTESIAN_POINT('Ctrl Pts',(-1.1645418350184,48.3233973044482,0.));
#84670=CARTESIAN_POINT('Ctrl Pts',(-1.1645418350184,48.3233973044482,20.));
#84671=CARTESIAN_POINT('Ctrl Pts',(-1.13101608948536,48.3211644441107,0.));
#84672=CARTESIAN_POINT('Ctrl Pts',(-1.13101608948536,48.3211644441107,20.));
#84673=CARTESIAN_POINT('Ctrl Pts',(-1.09749301203764,48.3189084488565,0.));
#84674=CARTESIAN_POINT('Ctrl Pts',(-1.09749301203764,48.3189084488565,20.));
#84675=CARTESIAN_POINT('Ctrl Pts',(-1.06397261868501,48.3166293206271,0.));
#84676=CARTESIAN_POINT('Ctrl Pts',(-1.06397261868501,48.3166293206271,20.));
#84677=CARTESIAN_POINT('Ctrl Pts',(-1.03045492543642,48.3143270613748,0.));
#84678=CARTESIAN_POINT('Ctrl Pts',(-1.03045492543642,48.3143270613748,20.));
#84679=CARTESIAN_POINT('Ctrl Pts',(-0.996939948299871,48.312001673063,0.));
#84680=CARTESIAN_POINT('Ctrl Pts',(-0.996939948299871,48.312001673063,20.));
#84681=CARTESIAN_POINT('Ctrl Pts',(-0.963427703282371,48.3096531576664,
0.));
#84682=CARTESIAN_POINT('Ctrl Pts',(-0.963427703282371,48.3096531576664,
20.));
#84683=CARTESIAN_POINT('Ctrl Pts',(-0.929918206389844,48.3072815171712,
0.));
#84684=CARTESIAN_POINT('Ctrl Pts',(-0.929918206389844,48.3072815171712,
20.));
#84685=CARTESIAN_POINT('Ctrl Pts',(-0.896411473627245,48.3048867535745,
0.));
#84686=CARTESIAN_POINT('Ctrl Pts',(-0.896411473627245,48.3048867535745,
20.));
#84687=CARTESIAN_POINT('Ctrl Pts',(-0.862907520998508,48.3024688688845,
0.));
#84688=CARTESIAN_POINT('Ctrl Pts',(-0.862907520998508,48.3024688688845,
20.));
#84689=CARTESIAN_POINT('Ctrl Pts',(-0.829406364506684,48.3000278651208,
0.));
#84690=CARTESIAN_POINT('Ctrl Pts',(-0.829406364506684,48.3000278651208,
20.));
#84691=CARTESIAN_POINT('Ctrl Pts',(-0.79590802015391,48.2975637443136,0.));
#84692=CARTESIAN_POINT('Ctrl Pts',(-0.79590802015391,48.2975637443136,20.));
#84693=CARTESIAN_POINT('Ctrl Pts',(-0.762412503941543,48.2950765085043,
0.));
#84694=CARTESIAN_POINT('Ctrl Pts',(-0.762412503941543,48.2950765085043,
20.));
#84695=CARTESIAN_POINT('Ctrl Pts',(-0.728919831869663,48.2925661597457,
0.));
#84696=CARTESIAN_POINT('Ctrl Pts',(-0.728919831869663,48.2925661597457,
20.));
#84697=CARTESIAN_POINT('Ctrl Pts',(-0.695430019937358,48.2900327001016,
0.));
#84698=CARTESIAN_POINT('Ctrl Pts',(-0.695430019937358,48.2900327001016,
20.));
#84699=CARTESIAN_POINT('Ctrl Pts',(-0.66194308414246,48.2874761316474,0.));
#84700=CARTESIAN_POINT('Ctrl Pts',(-0.66194308414246,48.2874761316474,20.));
#84701=CARTESIAN_POINT('Ctrl Pts',(-0.628459040481846,48.2848964564694,
0.));
#84702=CARTESIAN_POINT('Ctrl Pts',(-0.628459040481846,48.2848964564694,
20.));
#84703=CARTESIAN_POINT('Ctrl Pts',(-0.594977904951284,48.282293676665,0.));
#84704=CARTESIAN_POINT('Ctrl Pts',(-0.594977904951284,48.282293676665,20.));
#84705=CARTESIAN_POINT('Ctrl Pts',(-0.561499693545691,48.2796677943426,
0.));
#84706=CARTESIAN_POINT('Ctrl Pts',(-0.561499693545691,48.2796677943426,
20.));
#84707=CARTESIAN_POINT('Ctrl Pts',(-0.528024422259037,48.2770188116216,
0.));
#84708=CARTESIAN_POINT('Ctrl Pts',(-0.528024422259037,48.2770188116216,
20.));
#84709=CARTESIAN_POINT('Ctrl Pts',(-0.494552107084227,48.2743467306329,
0.));
#84710=CARTESIAN_POINT('Ctrl Pts',(-0.494552107084227,48.2743467306329,
20.));
#84711=CARTESIAN_POINT('Ctrl Pts',(-0.461082764013003,48.2716515535183,
0.));
#84712=CARTESIAN_POINT('Ctrl Pts',(-0.461082764013003,48.2716515535183,
20.));
#84713=CARTESIAN_POINT('Ctrl Pts',(-0.427616409036058,48.2689332824309,
0.));
#84714=CARTESIAN_POINT('Ctrl Pts',(-0.427616409036058,48.2689332824309,
20.));
#84715=CARTESIAN_POINT('Ctrl Pts',(-0.394153058142925,48.2661919195348,
0.));
#84716=CARTESIAN_POINT('Ctrl Pts',(-0.394153058142925,48.2661919195348,
20.));
#84717=CARTESIAN_POINT('Ctrl Pts',(-0.360692727322003,48.2634274670053,
0.));
#84718=CARTESIAN_POINT('Ctrl Pts',(-0.360692727322003,48.2634274670053,
20.));
#84719=CARTESIAN_POINT('Ctrl Pts',(-0.327235432560555,48.2606399270286,
0.));
#84720=CARTESIAN_POINT('Ctrl Pts',(-0.327235432560555,48.2606399270286,
20.));
#84721=CARTESIAN_POINT('Ctrl Pts',(-0.293781189844835,48.2578293018028,
0.));
#84722=CARTESIAN_POINT('Ctrl Pts',(-0.293781189844835,48.2578293018028,
20.));
#84723=CARTESIAN_POINT('Ctrl Pts',(-0.260330015159953,48.2549955935366,
0.));
#84724=CARTESIAN_POINT('Ctrl Pts',(-0.260330015159953,48.2549955935366,
20.));
#84725=CARTESIAN_POINT('Ctrl Pts',(-0.22688192448987,48.2521388044499,0.));
#84726=CARTESIAN_POINT('Ctrl Pts',(-0.22688192448987,48.2521388044499,20.));
#84727=CARTESIAN_POINT('Ctrl Pts',(-0.193436933817472,48.2492589367737,
0.));
#84728=CARTESIAN_POINT('Ctrl Pts',(-0.193436933817472,48.2492589367737,
20.));
#84729=CARTESIAN_POINT('Ctrl Pts',(-0.159995059124576,48.2463559927498,
0.));
#84730=CARTESIAN_POINT('Ctrl Pts',(-0.159995059124576,48.2463559927498,
20.));
#84731=CARTESIAN_POINT('Ctrl Pts',(-0.126556316391682,48.2434299746318,
0.));
#84732=CARTESIAN_POINT('Ctrl Pts',(-0.126556316391682,48.2434299746318,
20.));
#84733=CARTESIAN_POINT('Ctrl Pts',(-0.0931207215982832,48.2404808846839,
0.));
#84734=CARTESIAN_POINT('Ctrl Pts',(-0.0931207215982832,48.2404808846839,
20.));
#84735=CARTESIAN_POINT('Ctrl Pts',(-0.0596882907225993,48.2375087251817,
0.));
#84736=CARTESIAN_POINT('Ctrl Pts',(-0.0596882907225993,48.2375087251817,
20.));
#84737=CARTESIAN_POINT('Ctrl Pts',(-0.0262590397416762,48.234513498412,
0.));
#84738=CARTESIAN_POINT('Ctrl Pts',(-0.0262590397416762,48.234513498412,
20.));
#84739=CARTESIAN_POINT('Ctrl Pts',(0.00716701536856768,48.2314952066725,
0.));
#84740=CARTESIAN_POINT('Ctrl Pts',(0.00716701536856768,48.2314952066725,
20.));
#84741=CARTESIAN_POINT('Ctrl Pts',(0.0405898586334352,48.2284538522724,
0.));
#84742=CARTESIAN_POINT('Ctrl Pts',(0.0405898586334352,48.2284538522724,
20.));
#84743=CARTESIAN_POINT('Ctrl Pts',(0.0740094740793884,48.2253894375317,
0.));
#84744=CARTESIAN_POINT('Ctrl Pts',(0.0740094740793884,48.2253894375317,
20.));
#84745=CARTESIAN_POINT('Ctrl Pts',(0.107425845734119,48.2223019647818,0.));
#84746=CARTESIAN_POINT('Ctrl Pts',(0.107425845734119,48.2223019647818,20.));
#84747=CARTESIAN_POINT('Ctrl Pts',(0.140838957626541,48.2191914363652,0.));
#84748=CARTESIAN_POINT('Ctrl Pts',(0.140838957626541,48.2191914363652,20.));
#84749=CARTESIAN_POINT('Ctrl Pts',(0.174248793786895,48.2160578546352,0.));
#84750=CARTESIAN_POINT('Ctrl Pts',(0.174248793786895,48.2160578546352,20.));
#84751=CARTESIAN_POINT('Ctrl Pts',(0.207655338246555,48.2129012219564,0.));
#84752=CARTESIAN_POINT('Ctrl Pts',(0.207655338246555,48.2129012219564,20.));
#84753=CARTESIAN_POINT('Ctrl Pts',(0.241058575037867,48.2097215407045,0.));
#84754=CARTESIAN_POINT('Ctrl Pts',(0.241058575037867,48.2097215407045,20.));
#84755=CARTESIAN_POINT('Ctrl Pts',(0.274458488194584,48.2065188132665,0.));
#84756=CARTESIAN_POINT('Ctrl Pts',(0.274458488194584,48.2065188132665,20.));
#84757=CARTESIAN_POINT('Ctrl Pts',(0.30785506175171,48.2032930420408,0.));
#84758=CARTESIAN_POINT('Ctrl Pts',(0.30785506175171,48.2032930420408,20.));
#84759=CARTESIAN_POINT('Ctrl Pts',(0.341248279745643,48.2000442294364,0.));
#84760=CARTESIAN_POINT('Ctrl Pts',(0.341248279745643,48.2000442294364,20.));
#84761=CARTESIAN_POINT('Ctrl Pts',(0.374638126214095,48.1967723778737,0.));
#84762=CARTESIAN_POINT('Ctrl Pts',(0.374638126214095,48.1967723778737,20.));
#84763=CARTESIAN_POINT('Ctrl Pts',(0.408024585196225,48.1934774897842,0.));
#84764=CARTESIAN_POINT('Ctrl Pts',(0.408024585196225,48.1934774897842,20.));
#84765=CARTESIAN_POINT('Ctrl Pts',(0.441407640732092,48.1901595676102,0.));
#84766=CARTESIAN_POINT('Ctrl Pts',(0.441407640732092,48.1901595676102,20.));
#84767=CARTESIAN_POINT('Ctrl Pts',(0.474787276863071,48.1868186138054,0.));
#84768=CARTESIAN_POINT('Ctrl Pts',(0.474787276863071,48.1868186138054,20.));
#84769=CARTESIAN_POINT('Ctrl Pts',(0.508163477631851,48.1834546308352,0.));
#84770=CARTESIAN_POINT('Ctrl Pts',(0.508163477631851,48.1834546308352,20.));
#84771=CARTESIAN_POINT('Ctrl Pts',(0.541536227082355,48.1800676211754,0.));
#84772=CARTESIAN_POINT('Ctrl Pts',(0.541536227082355,48.1800676211754,20.));
#84773=CARTESIAN_POINT('Ctrl Pts',(0.574905509259889,48.1766575873132,0.));
#84774=CARTESIAN_POINT('Ctrl Pts',(0.574905509259889,48.1766575873132,20.));
#84775=CARTESIAN_POINT('Ctrl Pts',(0.608271308211097,48.1732245317468,0.));
#84776=CARTESIAN_POINT('Ctrl Pts',(0.608271308211097,48.1732245317468,20.));
#84777=CARTESIAN_POINT('Ctrl Pts',(0.6416336079841,48.1697684569855,0.));
#84778=CARTESIAN_POINT('Ctrl Pts',(0.6416336079841,48.1697684569855,20.));
#84779=CARTESIAN_POINT('Ctrl Pts',(0.674992392628235,48.16628936555,0.));
#84780=CARTESIAN_POINT('Ctrl Pts',(0.674992392628235,48.16628936555,20.));
#84781=CARTESIAN_POINT('Ctrl Pts',(0.708347646194278,48.1627872599717,0.));
#84782=CARTESIAN_POINT('Ctrl Pts',(0.708347646194278,48.1627872599717,20.));
#84783=CARTESIAN_POINT('Ctrl Pts',(0.741699352734257,48.1592621427937,0.));
#84784=CARTESIAN_POINT('Ctrl Pts',(0.741699352734257,48.1592621427937,20.));
#84785=CARTESIAN_POINT('Ctrl Pts',(0.775047496301533,48.1557140165701,0.));
#84786=CARTESIAN_POINT('Ctrl Pts',(0.775047496301533,48.1557140165701,20.));
#84787=CARTESIAN_POINT('Ctrl Pts',(0.808392060950864,48.1521428838659,0.));
#84788=CARTESIAN_POINT('Ctrl Pts',(0.808392060950864,48.1521428838659,20.));
#84789=CARTESIAN_POINT('Ctrl Pts',(0.841733030738387,48.1485487472572,0.));
#84790=CARTESIAN_POINT('Ctrl Pts',(0.841733030738387,48.1485487472572,20.));
#84791=CARTESIAN_POINT('Ctrl Pts',(0.875070389721522,48.144931609331,0.));
#84792=CARTESIAN_POINT('Ctrl Pts',(0.875070389721522,48.144931609331,20.));
#84793=CARTESIAN_POINT('Ctrl Pts',(0.908404121959285,48.1412914726861,0.));
#84794=CARTESIAN_POINT('Ctrl Pts',(0.908404121959285,48.1412914726861,20.));
#84795=CARTESIAN_POINT('Ctrl Pts',(0.941734211511944,48.137628339932,0.));
#84796=CARTESIAN_POINT('Ctrl Pts',(0.941734211511944,48.137628339932,20.));
#84797=CARTESIAN_POINT('Ctrl Pts',(0.975060642441243,48.1339422136897,0.));
#84798=CARTESIAN_POINT('Ctrl Pts',(0.975060642441243,48.1339422136897,20.));
#84799=CARTESIAN_POINT('Ctrl Pts',(1.00838339881032,48.130233096591,0.));
#84800=CARTESIAN_POINT('Ctrl Pts',(1.00838339881032,48.130233096591,20.));
#84801=CARTESIAN_POINT('Ctrl Pts',(1.04170246468365,48.1265009912787,0.));
#84802=CARTESIAN_POINT('Ctrl Pts',(1.04170246468365,48.1265009912787,20.));
#84803=CARTESIAN_POINT('Ctrl Pts',(1.07501782412728,48.1227459004068,0.));
#84804=CARTESIAN_POINT('Ctrl Pts',(1.07501782412728,48.1227459004068,20.));
#84805=CARTESIAN_POINT('Ctrl Pts',(1.10832946120861,48.1189678266406,0.));
#84806=CARTESIAN_POINT('Ctrl Pts',(1.10832946120861,48.1189678266406,20.));
#84807=CARTESIAN_POINT('Ctrl Pts',(1.14163735999657,48.1151667726565,0.));
#84808=CARTESIAN_POINT('Ctrl Pts',(1.14163735999657,48.1151667726565,20.));
#84809=CARTESIAN_POINT('Ctrl Pts',(1.17494150456145,48.111342741142,0.));
#84810=CARTESIAN_POINT('Ctrl Pts',(1.17494150456145,48.111342741142,20.));
#84811=CARTESIAN_POINT('Ctrl Pts',(1.20824187897489,48.1074957347955,0.));
#84812=CARTESIAN_POINT('Ctrl Pts',(1.20824187897489,48.1074957347955,20.));
#84813=CARTESIAN_POINT('Ctrl Pts',(1.24153846731022,48.1036257563271,0.));
#84814=CARTESIAN_POINT('Ctrl Pts',(1.24153846731022,48.1036257563271,20.));
#84815=CARTESIAN_POINT('Ctrl Pts',(1.27483125364215,48.0997328084577,0.));
#84816=CARTESIAN_POINT('Ctrl Pts',(1.27483125364215,48.0997328084577,20.));
#84817=CARTESIAN_POINT('Ctrl Pts',(1.30812022204704,48.0958168939195,0.));
#84818=CARTESIAN_POINT('Ctrl Pts',(1.30812022204704,48.0958168939195,20.));
#84819=CARTESIAN_POINT('Ctrl Pts',(1.3414053566026,48.0918780154556,0.));
#84820=CARTESIAN_POINT('Ctrl Pts',(1.3414053566026,48.0918780154556,20.));
#84821=CARTESIAN_POINT('Ctrl Pts',(1.37468664138801,48.0879161758201,0.));
#84822=CARTESIAN_POINT('Ctrl Pts',(1.37468664138801,48.0879161758201,20.));
#84823=CARTESIAN_POINT('Ctrl Pts',(1.40796406048387,48.0839313777781,0.));
#84824=CARTESIAN_POINT('Ctrl Pts',(1.40796406048387,48.0839313777781,20.));
#84825=CARTESIAN_POINT('Ctrl Pts',(1.44123759797224,48.0799236241059,0.));
#84826=CARTESIAN_POINT('Ctrl Pts',(1.44123759797224,48.0799236241059,20.));
#84827=CARTESIAN_POINT('Ctrl Pts',(1.47450723793681,48.0758929175908,0.));
#84828=CARTESIAN_POINT('Ctrl Pts',(1.47450723793681,48.0758929175908,20.));
#84829=CARTESIAN_POINT('Ctrl Pts',(1.50777296446291,48.071839261032,0.));
#84830=CARTESIAN_POINT('Ctrl Pts',(1.50777296446291,48.071839261032,20.));
#84831=CARTESIAN_POINT('Ctrl Pts',(1.54103476163743,48.0677626572394,0.));
#84832=CARTESIAN_POINT('Ctrl Pts',(1.54103476163743,48.0677626572394,20.));
#84833=CARTESIAN_POINT('Ctrl Pts',(1.57429261354889,48.0636631090342,0.));
#84834=CARTESIAN_POINT('Ctrl Pts',(1.57429261354889,48.0636631090342,20.));
#84835=CARTESIAN_POINT('Ctrl Pts',(1.60754650428745,48.0595406192492,0.));
#84836=CARTESIAN_POINT('Ctrl Pts',(1.60754650428745,48.0595406192492,20.));
#84837=CARTESIAN_POINT('Ctrl Pts',(1.64079641794461,48.0553951907273,0.));
#84838=CARTESIAN_POINT('Ctrl Pts',(1.64079641794461,48.0553951907273,20.));
#84839=CARTESIAN_POINT('Ctrl Pts',(1.67404233861337,48.0512268263229,0.));
#84840=CARTESIAN_POINT('Ctrl Pts',(1.67404233861337,48.0512268263229,20.));
#84841=CARTESIAN_POINT('Ctrl Pts',(1.70728425038804,48.0470355289011,0.));
#84842=CARTESIAN_POINT('Ctrl Pts',(1.70728425038804,48.0470355289011,20.));
#84843=CARTESIAN_POINT('Ctrl Pts',(1.74052213736471,48.0428213013379,0.));
#84844=CARTESIAN_POINT('Ctrl Pts',(1.74052213736471,48.0428213013379,20.));
#84845=CARTESIAN_POINT('Ctrl Pts',(1.77375598364109,48.038584146521,0.));
#84846=CARTESIAN_POINT('Ctrl Pts',(1.77375598364109,48.038584146521,20.));
#84847=CARTESIAN_POINT('Ctrl Pts',(1.80698577331663,48.0343240673492,0.));
#84848=CARTESIAN_POINT('Ctrl Pts',(1.80698577331663,48.0343240673492,20.));
#84849=CARTESIAN_POINT('Ctrl Pts',(1.84021149049245,48.0300410667328,0.));
#84850=CARTESIAN_POINT('Ctrl Pts',(1.84021149049245,48.0300410667328,20.));
#84851=CARTESIAN_POINT('Ctrl Pts',(1.87343311927141,48.0257351475934,0.));
#84852=CARTESIAN_POINT('Ctrl Pts',(1.87343311927141,48.0257351475934,20.));
#84853=CARTESIAN_POINT('Ctrl Pts',(1.90665064375786,48.0214063128629,0.));
#84854=CARTESIAN_POINT('Ctrl Pts',(1.90665064375786,48.0214063128629,20.));
#84855=CARTESIAN_POINT('Ctrl Pts',(1.93986404805772,48.0170545654849,0.));
#84856=CARTESIAN_POINT('Ctrl Pts',(1.93986404805772,48.0170545654849,20.));
#84857=CARTESIAN_POINT('Ctrl Pts',(1.97307331627849,48.0126799084137,0.));
#84858=CARTESIAN_POINT('Ctrl Pts',(1.97307331627849,48.0126799084137,20.));
#84859=CARTESIAN_POINT('Ctrl Pts',(2.00627843252925,48.0082823446147,0.));
#84860=CARTESIAN_POINT('Ctrl Pts',(2.00627843252925,48.0082823446147,20.));
#84861=CARTESIAN_POINT('Ctrl Pts',(2.03947938092067,48.0038618770642,0.));
#84862=CARTESIAN_POINT('Ctrl Pts',(2.03947938092067,48.0038618770642,20.));
#84863=CARTESIAN_POINT('Ctrl Pts',(2.07267614556536,47.9994185087499,0.));
#84864=CARTESIAN_POINT('Ctrl Pts',(2.07267614556536,47.9994185087499,20.));
#84865=CARTESIAN_POINT('Ctrl Pts',(2.10586871057748,47.994952242671,0.));
#84866=CARTESIAN_POINT('Ctrl Pts',(2.10586871057748,47.994952242671,20.));
#84867=CARTESIAN_POINT('Ctrl Pts',(2.13905706007285,47.9904630818375,0.));
#84868=CARTESIAN_POINT('Ctrl Pts',(2.13905706007285,47.9904630818375,20.));
#84869=CARTESIAN_POINT('Ctrl Pts',(2.17224117816898,47.9859510292704,0.));
#84870=CARTESIAN_POINT('Ctrl Pts',(2.17224117816898,47.9859510292704,20.));
#84871=CARTESIAN_POINT('Ctrl Pts',(2.2054210489852,47.9814160880019,0.));
#84872=CARTESIAN_POINT('Ctrl Pts',(2.2054210489852,47.9814160880019,20.));
#84873=CARTESIAN_POINT('Ctrl Pts',(2.23859665664239,47.9768582610752,0.));
#84874=CARTESIAN_POINT('Ctrl Pts',(2.23859665664239,47.9768582610752,20.));
#84875=CARTESIAN_POINT('Ctrl Pts',(2.27176798526352,47.9722775515452,0.));
#84876=CARTESIAN_POINT('Ctrl Pts',(2.27176798526352,47.9722775515452,20.));
#84877=CARTESIAN_POINT('Ctrl Pts',(2.30493501897294,47.9676739624772,0.));
#84878=CARTESIAN_POINT('Ctrl Pts',(2.30493501897294,47.9676739624772,20.));
#84879=CARTESIAN_POINT('Ctrl Pts',(2.33809774189657,47.9630474969481,0.));
#84880=CARTESIAN_POINT('Ctrl Pts',(2.33809774189657,47.9630474969481,20.));
#84881=CARTESIAN_POINT('Ctrl Pts',(2.3712561381623,47.9583981580454,0.));
#84882=CARTESIAN_POINT('Ctrl Pts',(2.3712561381623,47.9583981580454,20.));
#84883=CARTESIAN_POINT('Ctrl Pts',(2.40441019189959,47.9537259488681,0.));
#84884=CARTESIAN_POINT('Ctrl Pts',(2.40441019189959,47.9537259488681,20.));
#84885=CARTESIAN_POINT('Ctrl Pts',(2.43755988723965,47.9490308725257,0.));
#84886=CARTESIAN_POINT('Ctrl Pts',(2.43755988723965,47.9490308725257,20.));
#84887=CARTESIAN_POINT('Ctrl Pts',(2.47070520831548,47.9443129321394,0.));
#84888=CARTESIAN_POINT('Ctrl Pts',(2.47070520831548,47.9443129321394,20.));
#84889=CARTESIAN_POINT('Ctrl Pts',(2.50384613926209,47.9395721308414,0.));
#84890=CARTESIAN_POINT('Ctrl Pts',(2.50384613926209,47.9395721308414,20.));
#84891=CARTESIAN_POINT('Ctrl Pts',(2.53698266421613,47.9348084717752,0.));
#84892=CARTESIAN_POINT('Ctrl Pts',(2.53698266421613,47.9348084717752,20.));
#84893=CARTESIAN_POINT('Ctrl Pts',(2.57011476731622,47.9300219580955,0.));
#84894=CARTESIAN_POINT('Ctrl Pts',(2.57011476731622,47.9300219580955,20.));
#84895=CARTESIAN_POINT('Ctrl Pts',(2.60324243270257,47.9252125929679,0.));
#84896=CARTESIAN_POINT('Ctrl Pts',(2.60324243270257,47.9252125929679,20.));
#84897=CARTESIAN_POINT('Ctrl Pts',(2.63636564451718,47.9203803795688,0.));
#84898=CARTESIAN_POINT('Ctrl Pts',(2.63636564451718,47.9203803795688,20.));
#84899=CARTESIAN_POINT('Ctrl Pts',(2.66948438690365,47.9155253210858,0.));
#84900=CARTESIAN_POINT('Ctrl Pts',(2.66948438690365,47.9155253210858,20.));
#84901=CARTESIAN_POINT('Ctrl Pts',(2.70259864400757,47.9106474207177,0.));
#84902=CARTESIAN_POINT('Ctrl Pts',(2.70259864400757,47.9106474207177,20.));
#84903=CARTESIAN_POINT('Ctrl Pts',(2.73570839997628,47.9057466816743,0.));
#84904=CARTESIAN_POINT('Ctrl Pts',(2.73570839997628,47.9057466816743,20.));
#84905=CARTESIAN_POINT('Ctrl Pts',(2.76881363895917,47.9008231071768,0.));
#84906=CARTESIAN_POINT('Ctrl Pts',(2.76881363895917,47.9008231071768,20.));
#84907=CARTESIAN_POINT('Ctrl Pts',(2.80191434510733,47.8958767004573,0.));
#84908=CARTESIAN_POINT('Ctrl Pts',(2.80191434510733,47.8958767004573,20.));
#84909=CARTESIAN_POINT('Ctrl Pts',(2.83501050257375,47.8909074647592,0.));
#84910=CARTESIAN_POINT('Ctrl Pts',(2.83501050257375,47.8909074647592,20.));
#84911=CARTESIAN_POINT('Ctrl Pts',(2.86810209551307,47.8859154033363,0.));
#84912=CARTESIAN_POINT('Ctrl Pts',(2.86810209551307,47.8859154033363,20.));
#84913=CARTESIAN_POINT('Ctrl Pts',(2.90118910808199,47.8809005194543,0.));
#84914=CARTESIAN_POINT('Ctrl Pts',(2.90118910808199,47.8809005194543,20.));
#84915=CARTESIAN_POINT('Ctrl Pts',(2.93427152443917,47.8758628163901,0.));
#84916=CARTESIAN_POINT('Ctrl Pts',(2.93427152443917,47.8758628163901,20.));
#84917=CARTESIAN_POINT('Ctrl Pts',(2.96734932874504,47.8708022974315,0.));
#84918=CARTESIAN_POINT('Ctrl Pts',(2.96734932874504,47.8708022974315,20.));
#84919=CARTESIAN_POINT('Ctrl Pts',(3.00042250516192,47.8657189658771,0.));
#84920=CARTESIAN_POINT('Ctrl Pts',(3.00042250516192,47.8657189658771,20.));
#84921=CARTESIAN_POINT('Ctrl Pts',(3.03349103785388,47.8606128250365,0.));
#84922=CARTESIAN_POINT('Ctrl Pts',(3.03349103785388,47.8606128250365,20.));
#84923=CARTESIAN_POINT('Ctrl Pts',(3.06655491098681,47.8554838782302,0.));
#84924=CARTESIAN_POINT('Ctrl Pts',(3.06655491098681,47.8554838782302,20.));
#84925=CARTESIAN_POINT('Ctrl Pts',(3.09961410872875,47.8503321287903,0.));
#84926=CARTESIAN_POINT('Ctrl Pts',(3.09961410872875,47.8503321287903,20.));
#84927=CARTESIAN_POINT('Ctrl Pts',(3.13266861524953,47.8451575800601,0.));
#84928=CARTESIAN_POINT('Ctrl Pts',(3.13266861524953,47.8451575800601,20.));
#84929=CARTESIAN_POINT('Ctrl Pts',(3.16571841472089,47.8399602353939,0.));
#84930=CARTESIAN_POINT('Ctrl Pts',(3.16571841472089,47.8399602353939,20.));
#84931=CARTESIAN_POINT('Ctrl Pts',(3.19876349131674,47.834740098157,0.));
#84932=CARTESIAN_POINT('Ctrl Pts',(3.19876349131674,47.834740098157,20.));
#84933=CARTESIAN_POINT('Ctrl Pts',(3.23180382921272,47.829497171726,0.));
#84934=CARTESIAN_POINT('Ctrl Pts',(3.23180382921272,47.829497171726,20.));
#84935=CARTESIAN_POINT('Ctrl Pts',(3.26483941258676,47.8242314594881,0.));
#84936=CARTESIAN_POINT('Ctrl Pts',(3.26483941258676,47.8242314594881,20.));
#84937=CARTESIAN_POINT('Ctrl Pts',(3.29787022561835,47.818942964842,0.));
#84938=CARTESIAN_POINT('Ctrl Pts',(3.29787022561835,47.818942964842,20.));
#84939=CARTESIAN_POINT('Ctrl Pts',(3.33089625248902,47.813631691197,0.));
#84940=CARTESIAN_POINT('Ctrl Pts',(3.33089625248902,47.813631691197,20.));
#84941=CARTESIAN_POINT('Ctrl Pts',(3.36391747738213,47.8082976419741,0.));
#84942=CARTESIAN_POINT('Ctrl Pts',(3.36391747738213,47.8082976419741,20.));
#84943=CARTESIAN_POINT('Ctrl Pts',(3.39693388448305,47.802940820605,0.));
#84944=CARTESIAN_POINT('Ctrl Pts',(3.39693388448305,47.802940820605,20.));
#84945=CARTESIAN_POINT('Ctrl Pts',(3.42994545797921,47.797561230533,0.));
#84946=CARTESIAN_POINT('Ctrl Pts',(3.42994545797921,47.797561230533,20.));
#84947=CARTESIAN_POINT('Ctrl Pts',(3.46295218206011,47.7921588752121,0.));
#84948=CARTESIAN_POINT('Ctrl Pts',(3.46295218206011,47.7921588752121,20.));
#84949=CARTESIAN_POINT('Ctrl Pts',(3.49595404091727,47.7867337581073,0.));
#84950=CARTESIAN_POINT('Ctrl Pts',(3.49595404091727,47.7867337581073,20.));
#84951=CARTESIAN_POINT('Ctrl Pts',(3.52895101874414,47.7812858826946,0.));
#84952=CARTESIAN_POINT('Ctrl Pts',(3.52895101874414,47.7812858826946,20.));
#84953=CARTESIAN_POINT('Ctrl Pts',(3.56194309973641,47.7758152524613,0.));
#84954=CARTESIAN_POINT('Ctrl Pts',(3.56194309973641,47.7758152524613,20.));
#84955=CARTESIAN_POINT('Ctrl Pts',(3.59493026809157,47.7703218709055,0.));
#84956=CARTESIAN_POINT('Ctrl Pts',(3.59493026809157,47.7703218709055,20.));
#84957=CARTESIAN_POINT('Ctrl Pts',(3.62791250800923,47.764805741537,0.));
#84958=CARTESIAN_POINT('Ctrl Pts',(3.62791250800923,47.764805741537,20.));
#84959=CARTESIAN_POINT('Ctrl Pts',(3.66088980369083,47.7592668678762,0.));
#84960=CARTESIAN_POINT('Ctrl Pts',(3.66088980369083,47.7592668678762,20.));
#84961=CARTESIAN_POINT('Ctrl Pts',(3.69386213933993,47.7537052534546,0.));
#84962=CARTESIAN_POINT('Ctrl Pts',(3.69386213933993,47.7537052534546,20.));
#84963=CARTESIAN_POINT('Ctrl Pts',(3.72682949916222,47.7481209018149,0.));
#84964=CARTESIAN_POINT('Ctrl Pts',(3.72682949916222,47.7481209018149,20.));
#84965=CARTESIAN_POINT('Ctrl Pts',(3.75979186736544,47.7425138165111,0.));
#84966=CARTESIAN_POINT('Ctrl Pts',(3.75979186736544,47.7425138165111,20.));
#84967=CARTESIAN_POINT('Ctrl Pts',(3.79274922815948,47.7368840011081,0.));
#84968=CARTESIAN_POINT('Ctrl Pts',(3.79274922815948,47.7368840011081,20.));
#84969=CARTESIAN_POINT('Ctrl Pts',(3.82570156575622,47.7312314591817,0.));
#84970=CARTESIAN_POINT('Ctrl Pts',(3.82570156575622,47.7312314591817,20.));
#84971=CARTESIAN_POINT('Ctrl Pts',(3.85864886436973,47.7255561943191,0.));
#84972=CARTESIAN_POINT('Ctrl Pts',(3.85864886436973,47.7255561943191,20.));
#84973=CARTESIAN_POINT('Ctrl Pts',(3.89159110821604,47.719858210118,0.));
#84974=CARTESIAN_POINT('Ctrl Pts',(3.89159110821604,47.719858210118,20.));
#84975=CARTESIAN_POINT('Ctrl Pts',(3.92452828151332,47.7141375101875,0.));
#84976=CARTESIAN_POINT('Ctrl Pts',(3.92452828151332,47.7141375101875,20.));
#84977=CARTESIAN_POINT('Ctrl Pts',(3.95746036848186,47.7083940981477,0.));
#84978=CARTESIAN_POINT('Ctrl Pts',(3.95746036848186,47.7083940981477,20.));
#84979=CARTESIAN_POINT('Ctrl Pts',(3.990387353344,47.7026279776294,0.));
#84980=CARTESIAN_POINT('Ctrl Pts',(3.990387353344,47.7026279776294,20.));
#84981=CARTESIAN_POINT('Ctrl Pts',(4.02330922032433,47.6968391522753,0.));
#84982=CARTESIAN_POINT('Ctrl Pts',(4.02330922032433,47.6968391522753,20.));
#84983=CARTESIAN_POINT('Ctrl Pts',(4.05622595364951,47.6910276257391,0.));
#84984=CARTESIAN_POINT('Ctrl Pts',(4.05622595364951,47.6910276257391,20.));
#84985=CARTESIAN_POINT('Ctrl Pts',(4.08913753754848,47.6851934016861,0.));
#84986=CARTESIAN_POINT('Ctrl Pts',(4.08913753754848,47.6851934016861,20.));
#84987=CARTESIAN_POINT('Ctrl Pts',(4.12204395625218,47.6793364837921,0.));
#84988=CARTESIAN_POINT('Ctrl Pts',(4.12204395625218,47.6793364837921,20.));
#84989=CARTESIAN_POINT('Ctrl Pts',(4.15494519399369,47.6734568757434,0.));
#84990=CARTESIAN_POINT('Ctrl Pts',(4.15494519399369,47.6734568757434,20.));
#84991=CARTESIAN_POINT('Ctrl Pts',(4.18784123500835,47.6675545812371,0.));
#84992=CARTESIAN_POINT('Ctrl Pts',(4.18784123500835,47.6675545812371,20.));
#84993=CARTESIAN_POINT('Ctrl Pts',(4.22073206353344,47.6616296039816,0.));
#84994=CARTESIAN_POINT('Ctrl Pts',(4.22073206353344,47.6616296039816,20.));
#84995=CARTESIAN_POINT('Ctrl Pts',(4.25361766380859,47.6556819476964,0.));
#84996=CARTESIAN_POINT('Ctrl Pts',(4.25361766380859,47.6556819476964,20.));
#84997=CARTESIAN_POINT('Ctrl Pts',(4.28649802007566,47.6497116161128,0.));
#84998=CARTESIAN_POINT('Ctrl Pts',(4.28649802007566,47.6497116161128,20.));
#84999=CARTESIAN_POINT('Ctrl Pts',(4.31937311657885,47.6437186129734,0.));
#85000=CARTESIAN_POINT('Ctrl Pts',(4.31937311657885,47.6437186129734,20.));
#85001=CARTESIAN_POINT('Ctrl Pts',(4.35224293756439,47.6377029420315,0.));
#85002=CARTESIAN_POINT('Ctrl Pts',(4.35224293756439,47.6377029420315,20.));
#85003=CARTESIAN_POINT('Ctrl Pts',(4.38510746728074,47.6316646070511,0.));
#85004=CARTESIAN_POINT('Ctrl Pts',(4.38510746728074,47.6316646070511,20.));
#85005=CARTESIAN_POINT('Ctrl Pts',(4.41796668997835,47.6256036118071,0.));
#85006=CARTESIAN_POINT('Ctrl Pts',(4.41796668997835,47.6256036118071,20.));
#85007=CARTESIAN_POINT('Ctrl Pts',(4.45082058991003,47.6195199600851,0.));
#85008=CARTESIAN_POINT('Ctrl Pts',(4.45082058991003,47.6195199600851,20.));
#85009=CARTESIAN_POINT('Ctrl Pts',(4.48366915133083,47.6134136556823,0.));
#85010=CARTESIAN_POINT('Ctrl Pts',(4.48366915133083,47.6134136556823,20.));
#85011=CARTESIAN_POINT('Ctrl Pts',(4.51651235849822,47.6072847024073,0.));
#85012=CARTESIAN_POINT('Ctrl Pts',(4.51651235849822,47.6072847024073,20.));
#85013=CARTESIAN_POINT('Ctrl Pts',(4.54935019567197,47.6011331040799,0.));
#85014=CARTESIAN_POINT('Ctrl Pts',(4.54935019567197,47.6011331040799,20.));
#85015=CARTESIAN_POINT('Ctrl Pts',(4.58218264711418,47.5949588645311,0.));
#85016=CARTESIAN_POINT('Ctrl Pts',(4.58218264711418,47.5949588645311,20.));
#85017=CARTESIAN_POINT('Ctrl Pts',(4.61500969708895,47.5887619876026,0.));
#85018=CARTESIAN_POINT('Ctrl Pts',(4.61500969708895,47.5887619876026,20.));
#85019=CARTESIAN_POINT('Ctrl Pts',(4.64783132986259,47.5825424771468,0.));
#85020=CARTESIAN_POINT('Ctrl Pts',(4.64783132986259,47.5825424771468,20.));
#85021=CARTESIAN_POINT('Ctrl Pts',(4.68064752970369,47.5763003370265,0.));
#85022=CARTESIAN_POINT('Ctrl Pts',(4.68064752970369,47.5763003370265,20.));
#85023=CARTESIAN_POINT('Ctrl Pts',(4.71345828088308,47.5700355711162,0.));
#85024=CARTESIAN_POINT('Ctrl Pts',(4.71345828088308,47.5700355711162,20.));
#85025=CARTESIAN_POINT('Ctrl Pts',(4.74626356767412,47.5637481833017,0.));
#85026=CARTESIAN_POINT('Ctrl Pts',(4.74626356767412,47.5637481833017,20.));
#85027=CARTESIAN_POINT('Ctrl Pts',(4.77906337435243,47.5574381774801,0.));
#85028=CARTESIAN_POINT('Ctrl Pts',(4.77906337435243,47.5574381774801,20.));
#85029=CARTESIAN_POINT('Ctrl Pts',(4.81185768519588,47.5511055575593,0.));
#85030=CARTESIAN_POINT('Ctrl Pts',(4.81185768519588,47.5511055575593,20.));
#85031=CARTESIAN_POINT('Ctrl Pts',(4.84464648448474,47.5447503274583,0.));
#85032=CARTESIAN_POINT('Ctrl Pts',(4.84464648448474,47.5447503274583,20.));
#85033=CARTESIAN_POINT('Ctrl Pts',(4.87742975650161,47.538372491107,0.));
#85034=CARTESIAN_POINT('Ctrl Pts',(4.87742975650161,47.538372491107,20.));
#85035=CARTESIAN_POINT('Ctrl Pts',(4.91020748553144,47.5319720524462,0.));
#85036=CARTESIAN_POINT('Ctrl Pts',(4.91020748553144,47.5319720524462,20.));
#85037=CARTESIAN_POINT('Ctrl Pts',(4.94297965586156,47.5255490154281,0.));
#85038=CARTESIAN_POINT('Ctrl Pts',(4.94297965586156,47.5255490154281,20.));
#85039=CARTESIAN_POINT('Ctrl Pts',(4.97574625178169,47.519103384016,0.));
#85040=CARTESIAN_POINT('Ctrl Pts',(4.97574625178169,47.519103384016,20.));
#85041=CARTESIAN_POINT('Ctrl Pts',(5.00850725758367,47.5126351621839,0.));
#85042=CARTESIAN_POINT('Ctrl Pts',(5.00850725758367,47.5126351621839,20.));
#85043=CARTESIAN_POINT('Ctrl Pts',(5.04126265756154,47.5061443539168,0.));
#85044=CARTESIAN_POINT('Ctrl Pts',(5.04126265756154,47.5061443539168,20.));
#85045=CARTESIAN_POINT('Ctrl Pts',(5.07401243601198,47.4996309632108,0.));
#85046=CARTESIAN_POINT('Ctrl Pts',(5.07401243601198,47.4996309632108,20.));
#85047=CARTESIAN_POINT('Ctrl Pts',(5.10675657723402,47.4930949940731,0.));
#85048=CARTESIAN_POINT('Ctrl Pts',(5.10675657723402,47.4930949940731,20.));
#85049=CARTESIAN_POINT('Ctrl Pts',(5.13949506552922,47.4865364505219,0.));
#85050=CARTESIAN_POINT('Ctrl Pts',(5.13949506552922,47.4865364505219,20.));
#85051=CARTESIAN_POINT('Ctrl Pts',(5.17222788520144,47.4799553365862,0.));
#85052=CARTESIAN_POINT('Ctrl Pts',(5.17222788520144,47.4799553365862,20.));
#85053=CARTESIAN_POINT('Ctrl Pts',(5.20495502055713,47.4733516563069,0.));
#85054=CARTESIAN_POINT('Ctrl Pts',(5.20495502055713,47.4733516563069,20.));
#85055=CARTESIAN_POINT('Ctrl Pts',(5.2376764559051,47.4667254137359,0.));
#85056=CARTESIAN_POINT('Ctrl Pts',(5.2376764559051,47.4667254137359,20.));
#85057=CARTESIAN_POINT('Ctrl Pts',(5.27039217555655,47.4600766129357,0.));
#85058=CARTESIAN_POINT('Ctrl Pts',(5.27039217555655,47.4600766129357,20.));
#85059=CARTESIAN_POINT('Ctrl Pts',(5.30310216382505,47.4534052579797,0.));
#85060=CARTESIAN_POINT('Ctrl Pts',(5.30310216382505,47.4534052579797,20.));
#85061=CARTESIAN_POINT('Ctrl Pts',(5.3358064050266,47.4467113529523,0.));
#85062=CARTESIAN_POINT('Ctrl Pts',(5.3358064050266,47.4467113529523,20.));
#85063=CARTESIAN_POINT('Ctrl Pts',(5.36850488347923,47.4399949019487,0.));
#85064=CARTESIAN_POINT('Ctrl Pts',(5.36850488347923,47.4399949019487,20.));
#85065=CARTESIAN_POINT('Ctrl Pts',(5.40119758350378,47.4332559090748,0.));
#85066=CARTESIAN_POINT('Ctrl Pts',(5.40119758350378,47.4332559090748,20.));
#85067=CARTESIAN_POINT('Ctrl Pts',(5.43388448942349,47.4264943784481,0.));
#85068=CARTESIAN_POINT('Ctrl Pts',(5.43388448942349,47.4264943784481,20.));
#85069=CARTESIAN_POINT('Ctrl Pts',(5.46656558556425,47.4197103141976,0.));
#85070=CARTESIAN_POINT('Ctrl Pts',(5.46656558556425,47.4197103141976,20.));
#85071=CARTESIAN_POINT('Ctrl Pts',(5.49924085625463,47.4129037204631,0.));
#85072=CARTESIAN_POINT('Ctrl Pts',(5.49924085625463,47.4129037204631,20.));
#85073=CARTESIAN_POINT('Ctrl Pts',(5.53191028582554,47.4060746013959,0.));
#85074=CARTESIAN_POINT('Ctrl Pts',(5.53191028582554,47.4060746013959,20.));
#85075=CARTESIAN_POINT('Ctrl Pts',(5.56457385861036,47.3992229611579,0.));
#85076=CARTESIAN_POINT('Ctrl Pts',(5.56457385861036,47.3992229611579,20.));
#85077=CARTESIAN_POINT('Ctrl Pts',(5.59723155894482,47.3923488039217,0.));
#85078=CARTESIAN_POINT('Ctrl Pts',(5.59723155894482,47.3923488039217,20.));
#85079=CARTESIAN_POINT('Ctrl Pts',(5.62988337116714,47.3854521338708,0.));
#85080=CARTESIAN_POINT('Ctrl Pts',(5.62988337116714,47.3854521338708,20.));
#85081=CARTESIAN_POINT('Ctrl Pts',(5.6625292796181,47.3785329551997,0.));
#85082=CARTESIAN_POINT('Ctrl Pts',(5.6625292796181,47.3785329551997,20.));
#85083=CARTESIAN_POINT('Ctrl Pts',(5.69516926864087,47.3715912721141,0.));
#85084=CARTESIAN_POINT('Ctrl Pts',(5.69516926864087,47.3715912721141,20.));
#85085=CARTESIAN_POINT('Ctrl Pts',(5.72780332258134,47.3646270888308,0.));
#85086=CARTESIAN_POINT('Ctrl Pts',(5.72780332258134,47.3646270888308,20.));
#85087=CARTESIAN_POINT('Ctrl Pts',(5.76043142578785,47.3576404095778,0.));
#85088=CARTESIAN_POINT('Ctrl Pts',(5.76043142578785,47.3576404095778,20.));
#85089=CARTESIAN_POINT('Ctrl Pts',(5.79305356261141,47.3506312385939,0.));
#85090=CARTESIAN_POINT('Ctrl Pts',(5.79305356261141,47.3506312385939,20.));
#85091=CARTESIAN_POINT('Ctrl Pts',(5.82566971740555,47.3435995801292,0.));
#85092=CARTESIAN_POINT('Ctrl Pts',(5.82566971740555,47.3435995801292,20.));
#85093=CARTESIAN_POINT('Ctrl Pts',(5.85827987452639,47.3365454384446,0.));
#85094=CARTESIAN_POINT('Ctrl Pts',(5.85827987452639,47.3365454384446,20.));
#85095=CARTESIAN_POINT('Ctrl Pts',(5.89088401833276,47.3294688178121,0.));
#85096=CARTESIAN_POINT('Ctrl Pts',(5.89088401833276,47.3294688178121,20.));
#85097=CARTESIAN_POINT('Ctrl Pts',(5.92348213318597,47.3223697225143,0.));
#85098=CARTESIAN_POINT('Ctrl Pts',(5.92348213318597,47.3223697225143,20.));
#85099=CARTESIAN_POINT('Ctrl Pts',(5.95607420344985,47.3152481568452,0.));
#85100=CARTESIAN_POINT('Ctrl Pts',(5.95607420344985,47.3152481568452,20.));
#85101=CARTESIAN_POINT('Ctrl Pts',(5.98866021349066,47.3081041251096,0.));
#85102=CARTESIAN_POINT('Ctrl Pts',(5.98866021349066,47.3081041251096,20.));
#85103=CARTESIAN_POINT('Ctrl Pts',(6.02124014767729,47.3009376316237,0.));
#85104=CARTESIAN_POINT('Ctrl Pts',(6.02124014767729,47.3009376316237,20.));
#85105=CARTESIAN_POINT('Ctrl Pts',(6.05381399038128,47.2937486807145,0.));
#85106=CARTESIAN_POINT('Ctrl Pts',(6.05381399038128,47.2937486807145,20.));
#85107=CARTESIAN_POINT('Ctrl Pts',(6.08638172597683,47.2865372767199,0.));
#85108=CARTESIAN_POINT('Ctrl Pts',(6.08638172597683,47.2865372767199,20.));
#85109=CARTESIAN_POINT('Ctrl Pts',(6.11894333884087,47.2793034239892,0.));
#85110=CARTESIAN_POINT('Ctrl Pts',(6.11894333884087,47.2793034239892,20.));
#85111=CARTESIAN_POINT('Ctrl Pts',(6.15149881335289,47.272047126882,0.));
#85112=CARTESIAN_POINT('Ctrl Pts',(6.15149881335289,47.272047126882,20.));
#85113=CARTESIAN_POINT('Ctrl Pts',(6.18404813389528,47.2647683897693,0.));
#85114=CARTESIAN_POINT('Ctrl Pts',(6.18404813389528,47.2647683897693,20.));
#85115=CARTESIAN_POINT('Ctrl Pts',(6.21659128485295,47.2574672170331,0.));
#85116=CARTESIAN_POINT('Ctrl Pts',(6.21659128485295,47.2574672170331,20.));
#85117=CARTESIAN_POINT('Ctrl Pts',(6.24912825061342,47.2501436130661,0.));
#85118=CARTESIAN_POINT('Ctrl Pts',(6.24912825061342,47.2501436130661,20.));
#85119=CARTESIAN_POINT('Ctrl Pts',(6.28165901556675,47.2427975822723,0.));
#85120=CARTESIAN_POINT('Ctrl Pts',(6.28165901556675,47.2427975822723,20.));
#85121=CARTESIAN_POINT('Ctrl Pts',(6.31418356410549,47.2354291290667,0.));
#85122=CARTESIAN_POINT('Ctrl Pts',(6.31418356410549,47.2354291290667,20.));
#85123=CARTESIAN_POINT('Ctrl Pts',(6.34670188062515,47.2280382578755,0.));
#85124=CARTESIAN_POINT('Ctrl Pts',(6.34670188062515,47.2280382578755,20.));
#85125=CARTESIAN_POINT('Ctrl Pts',(6.37921394952379,47.2206249731358,0.));
#85126=CARTESIAN_POINT('Ctrl Pts',(6.37921394952379,47.2206249731358,20.));
#85127=CARTESIAN_POINT('Ctrl Pts',(6.41171975520233,47.213189279296,0.));
#85128=CARTESIAN_POINT('Ctrl Pts',(6.41171975520233,47.213189279296,20.));
#85129=CARTESIAN_POINT('Ctrl Pts',(6.44421928206445,47.205731180815,0.));
#85130=CARTESIAN_POINT('Ctrl Pts',(6.44421928206445,47.205731180815,20.));
#85131=CARTESIAN_POINT('Ctrl Pts',(6.47671251451637,47.1982506821625,0.));
#85132=CARTESIAN_POINT('Ctrl Pts',(6.47671251451637,47.1982506821625,20.));
#85133=CARTESIAN_POINT('Ctrl Pts',(6.50919943696717,47.190747787819,0.));
#85134=CARTESIAN_POINT('Ctrl Pts',(6.50919943696717,47.190747787819,20.));
#85135=CARTESIAN_POINT('Ctrl Pts',(6.54168003382861,47.1832225022762,0.));
#85136=CARTESIAN_POINT('Ctrl Pts',(6.54168003382861,47.1832225022762,20.));
#85137=CARTESIAN_POINT('Ctrl Pts',(6.57415428951524,47.1756748300372,0.));
#85138=CARTESIAN_POINT('Ctrl Pts',(6.57415428951524,47.1756748300372,20.));
#85139=CARTESIAN_POINT('Ctrl Pts',(6.60662218844434,47.168104775616,0.));
#85140=CARTESIAN_POINT('Ctrl Pts',(6.60662218844434,47.168104775616,20.));
#85141=CARTESIAN_POINT('Ctrl Pts',(6.63908371503577,47.1605123435378,0.));
#85142=CARTESIAN_POINT('Ctrl Pts',(6.63908371503577,47.1605123435378,20.));
#85143=CARTESIAN_POINT('Ctrl Pts',(6.67153885371226,47.1528975383387,0.));
#85144=CARTESIAN_POINT('Ctrl Pts',(6.67153885371226,47.1528975383387,20.));
#85145=CARTESIAN_POINT('Ctrl Pts',(6.70398758889916,47.1452603645656,0.));
#85146=CARTESIAN_POINT('Ctrl Pts',(6.70398758889916,47.1452603645656,20.));
#85147=CARTESIAN_POINT('Ctrl Pts',(6.73642990502458,47.1376008267758,0.));
#85148=CARTESIAN_POINT('Ctrl Pts',(6.73642990502458,47.1376008267758,20.));
#85149=CARTESIAN_POINT('Ctrl Pts',(6.76886578651954,47.129918929538,0.));
#85150=CARTESIAN_POINT('Ctrl Pts',(6.76886578651954,47.129918929538,20.));
#85151=CARTESIAN_POINT('Ctrl Pts',(6.80129521781808,47.1222146774323,0.));
#85152=CARTESIAN_POINT('Ctrl Pts',(6.80129521781808,47.1222146774323,20.));
#85153=CARTESIAN_POINT('Ctrl Pts',(6.83371818335697,47.1144880750497,0.));
#85154=CARTESIAN_POINT('Ctrl Pts',(6.83371818335697,47.1144880750497,20.));
#85155=CARTESIAN_POINT('Ctrl Pts',(6.86613466757588,47.1067391269919,0.));
#85156=CARTESIAN_POINT('Ctrl Pts',(6.86613466757588,47.1067391269919,20.));
#85157=CARTESIAN_POINT('Ctrl Pts',(6.89854465491702,47.0989678378717,0.));
#85158=CARTESIAN_POINT('Ctrl Pts',(6.89854465491702,47.0989678378717,20.));
#85159=CARTESIAN_POINT('Ctrl Pts',(6.93094812982541,47.0911742123123,0.));
#85160=CARTESIAN_POINT('Ctrl Pts',(6.93094812982541,47.0911742123123,20.));
#85161=CARTESIAN_POINT('Ctrl Pts',(6.96334507674873,47.0833582549484,0.));
#85162=CARTESIAN_POINT('Ctrl Pts',(6.96334507674873,47.0833582549484,20.));
#85163=CARTESIAN_POINT('Ctrl Pts',(6.99573548013776,47.0755199704256,0.));
#85164=CARTESIAN_POINT('Ctrl Pts',(6.99573548013776,47.0755199704256,20.));
#85165=CARTESIAN_POINT('Ctrl Pts',(7.02811932444601,47.0676593634011,0.));
#85166=CARTESIAN_POINT('Ctrl Pts',(7.02811932444601,47.0676593634011,20.));
#85167=CARTESIAN_POINT('Ctrl Pts',(7.06049659413007,47.0597764385426,0.));
#85168=CARTESIAN_POINT('Ctrl Pts',(7.06049659413007,47.0597764385426,20.));
#85169=CARTESIAN_POINT('Ctrl Pts',(7.09286727364932,47.0518712005288,0.));
#85170=CARTESIAN_POINT('Ctrl Pts',(7.09286727364932,47.0518712005288,20.));
#85171=CARTESIAN_POINT('Ctrl Pts',(7.12523134746603,47.0439436540493,0.));
#85172=CARTESIAN_POINT('Ctrl Pts',(7.12523134746603,47.0439436540493,20.));
#85173=CARTESIAN_POINT('Ctrl Pts',(7.15758880004521,47.0359938038039,0.));
#85174=CARTESIAN_POINT('Ctrl Pts',(7.15758880004521,47.0359938038039,20.));
#85175=CARTESIAN_POINT('Ctrl Pts',(7.18993961585469,47.0280216545038,0.));
#85176=CARTESIAN_POINT('Ctrl Pts',(7.18993961585469,47.0280216545038,20.));
#85177=CARTESIAN_POINT('Ctrl Pts',(7.22228377936529,47.020027210871,0.));
#85178=CARTESIAN_POINT('Ctrl Pts',(7.22228377936529,47.020027210871,20.));
#85179=CARTESIAN_POINT('Ctrl Pts',(7.25462127505076,47.012010477639,0.));
#85180=CARTESIAN_POINT('Ctrl Pts',(7.25462127505076,47.012010477639,20.));
#85181=CARTESIAN_POINT('Ctrl Pts',(7.28695208738784,47.0039714595526,0.));
#85182=CARTESIAN_POINT('Ctrl Pts',(7.28695208738784,47.0039714595526,20.));
#85183=CARTESIAN_POINT('Ctrl Pts',(7.31927620085613,46.9959101613675,0.));
#85184=CARTESIAN_POINT('Ctrl Pts',(7.31927620085613,46.9959101613675,20.));
#85185=CARTESIAN_POINT('Ctrl Pts',(7.35159359993817,46.9878265878505,0.));
#85186=CARTESIAN_POINT('Ctrl Pts',(7.35159359993817,46.9878265878505,20.));
#85187=CARTESIAN_POINT('Ctrl Pts',(7.38390426911931,46.9797207437786,0.));
#85188=CARTESIAN_POINT('Ctrl Pts',(7.38390426911931,46.9797207437786,20.));
#85189=CARTESIAN_POINT('Ctrl Pts',(7.41620819288777,46.9715926339391,0.));
#85190=CARTESIAN_POINT('Ctrl Pts',(7.41620819288777,46.9715926339391,20.));
#85191=CARTESIAN_POINT('Ctrl Pts',(7.44850535573481,46.9634422631307,0.));
#85192=CARTESIAN_POINT('Ctrl Pts',(7.44850535573481,46.9634422631307,20.));
#85193=CARTESIAN_POINT('Ctrl Pts',(7.48079574215478,46.9552696361634,0.));
#85194=CARTESIAN_POINT('Ctrl Pts',(7.48079574215478,46.9552696361634,20.));
#85195=CARTESIAN_POINT('Ctrl Pts',(7.51307933664511,46.9470747578592,0.));
#85196=CARTESIAN_POINT('Ctrl Pts',(7.51307933664511,46.9470747578592,20.));
#85197=CARTESIAN_POINT('Ctrl Pts',(7.54535612370601,46.9388576330501,0.));
#85198=CARTESIAN_POINT('Ctrl Pts',(7.54535612370601,46.9388576330501,20.));
#85199=CARTESIAN_POINT('Ctrl Pts',(7.57762608784068,46.9306182665792,0.));
#85200=CARTESIAN_POINT('Ctrl Pts',(7.57762608784068,46.9306182665792,20.));
#85201=CARTESIAN_POINT('Ctrl Pts',(7.6098892135552,46.9223566632999,0.));
#85202=CARTESIAN_POINT('Ctrl Pts',(7.6098892135552,46.9223566632999,20.));
#85203=CARTESIAN_POINT('Ctrl Pts',(7.64214548535856,46.9140728280766,0.));
#85204=CARTESIAN_POINT('Ctrl Pts',(7.64214548535856,46.9140728280766,20.));
#85205=CARTESIAN_POINT('Ctrl Pts',(7.67439488776287,46.9057667657847,0.));
#85206=CARTESIAN_POINT('Ctrl Pts',(7.67439488776287,46.9057667657847,20.));
#85207=CARTESIAN_POINT('Ctrl Pts',(7.7066374052833,46.8974384813109,0.));
#85208=CARTESIAN_POINT('Ctrl Pts',(7.7066374052833,46.8974384813109,20.));
#85209=CARTESIAN_POINT('Ctrl Pts',(7.73887302243815,46.8890879795531,0.));
#85210=CARTESIAN_POINT('Ctrl Pts',(7.73887302243815,46.8890879795531,20.));
#85211=CARTESIAN_POINT('Ctrl Pts',(7.77110172374868,46.8807152654198,0.));
#85212=CARTESIAN_POINT('Ctrl Pts',(7.77110172374868,46.8807152654198,20.));
#85213=CARTESIAN_POINT('Ctrl Pts',(7.80332349373917,46.8723203438306,0.));
#85214=CARTESIAN_POINT('Ctrl Pts',(7.80332349373917,46.8723203438306,20.));
#85215=CARTESIAN_POINT('Ctrl Pts',(7.83553831693686,46.8639032197162,0.));
#85216=CARTESIAN_POINT('Ctrl Pts',(7.83553831693686,46.8639032197162,20.));
#85217=CARTESIAN_POINT('Ctrl Pts',(7.86774617787212,46.855463898018,0.));
#85218=CARTESIAN_POINT('Ctrl Pts',(7.86774617787212,46.855463898018,20.));
#85219=CARTESIAN_POINT('Ctrl Pts',(7.89994706107838,46.8470023836881,0.));
#85220=CARTESIAN_POINT('Ctrl Pts',(7.89994706107838,46.8470023836881,20.));
#85221=CARTESIAN_POINT('Ctrl Pts',(7.9321409510921,46.8385186816898,0.));
#85222=CARTESIAN_POINT('Ctrl Pts',(7.9321409510921,46.8385186816898,20.));
#85223=CARTESIAN_POINT('Ctrl Pts',(7.96432783245285,46.8300127969969,0.));
#85224=CARTESIAN_POINT('Ctrl Pts',(7.96432783245285,46.8300127969969,20.));
#85225=CARTESIAN_POINT('Ctrl Pts',(7.99650768970303,46.8214847345942,0.));
#85226=CARTESIAN_POINT('Ctrl Pts',(7.99650768970303,46.8214847345942,20.));
#85227=CARTESIAN_POINT('Ctrl Pts',(8.02868050738827,46.8129344994773,0.));
#85228=CARTESIAN_POINT('Ctrl Pts',(8.02868050738827,46.8129344994773,20.));
#85229=CARTESIAN_POINT('Ctrl Pts',(8.06084627005728,46.8043620966531,0.));
#85230=CARTESIAN_POINT('Ctrl Pts',(8.06084627005728,46.8043620966531,20.));
#85231=CARTESIAN_POINT('Ctrl Pts',(8.09300496226219,46.7957675311395,0.));
#85232=CARTESIAN_POINT('Ctrl Pts',(8.09300496226219,46.7957675311395,20.));
#85233=CARTESIAN_POINT('Ctrl Pts',(8.125156568558,46.7871508079658,0.));
#85234=CARTESIAN_POINT('Ctrl Pts',(8.125156568558,46.7871508079658,20.));
#85235=CARTESIAN_POINT('Ctrl Pts',(8.15730107350294,46.7785119321719,0.));
#85236=CARTESIAN_POINT('Ctrl Pts',(8.15730107350294,46.7785119321719,20.));
#85237=CARTESIAN_POINT('Ctrl Pts',(8.18943846165844,46.7698509088086,0.));
#85238=CARTESIAN_POINT('Ctrl Pts',(8.18943846165844,46.7698509088086,20.));
#85239=CARTESIAN_POINT('Ctrl Pts',(8.22156871758881,46.7611677429374,0.));
#85240=CARTESIAN_POINT('Ctrl Pts',(8.22156871758881,46.7611677429374,20.));
#85241=CARTESIAN_POINT('Ctrl Pts',(8.25369182586168,46.7524624396307,0.));
#85242=CARTESIAN_POINT('Ctrl Pts',(8.25369182586168,46.7524624396307,20.));
#85243=CARTESIAN_POINT('Ctrl Pts',(8.28580777104744,46.7437350039712,0.));
#85244=CARTESIAN_POINT('Ctrl Pts',(8.28580777104744,46.7437350039712,20.));
#85245=CARTESIAN_POINT('Ctrl Pts',(8.31791653771973,46.7349854410525,0.));
#85246=CARTESIAN_POINT('Ctrl Pts',(8.31791653771973,46.7349854410525,20.));
#85247=CARTESIAN_POINT('Ctrl Pts',(8.35001811045535,46.7262137559789,0.));
#85248=CARTESIAN_POINT('Ctrl Pts',(8.35001811045535,46.7262137559789,20.));
#85249=CARTESIAN_POINT('Ctrl Pts',(8.38211247383476,46.7174199538668,0.));
#85250=CARTESIAN_POINT('Ctrl Pts',(8.38211247383476,46.7174199538668,20.));
#85251=CARTESIAN_POINT('Ctrl Pts',(8.41419961244154,46.7086040398438,0.));
#85252=CARTESIAN_POINT('Ctrl Pts',(8.41419961244154,46.7086040398438,20.));
#85253=CARTESIAN_POINT('Ctrl Pts',(8.44627951086261,46.6997660190488,0.));
#85254=CARTESIAN_POINT('Ctrl Pts',(8.44627951086261,46.6997660190488,20.));
#85255=CARTESIAN_POINT('Ctrl Pts',(8.47835215368743,46.6909058966306,0.));
#85256=CARTESIAN_POINT('Ctrl Pts',(8.47835215368743,46.6909058966306,20.));
#85257=CARTESIAN_POINT('Ctrl Pts',(8.5104175255088,46.6820236777489,0.));
#85258=CARTESIAN_POINT('Ctrl Pts',(8.5104175255088,46.6820236777489,20.));
#85259=CARTESIAN_POINT('Ctrl Pts',(8.54247561092257,46.673119367573,0.));
#85260=CARTESIAN_POINT('Ctrl Pts',(8.54247561092257,46.673119367573,20.));
#85261=CARTESIAN_POINT('Ctrl Pts',(8.57452639452827,46.6641929712839,0.));
#85262=CARTESIAN_POINT('Ctrl Pts',(8.57452639452827,46.6641929712839,20.));
#85263=CARTESIAN_POINT('Ctrl Pts',(8.60656986092877,46.6552444940739,0.));
#85264=CARTESIAN_POINT('Ctrl Pts',(8.60656986092877,46.6552444940739,20.));
#85265=CARTESIAN_POINT('Ctrl Pts',(8.63860599473002,46.6462739411471,0.));
#85266=CARTESIAN_POINT('Ctrl Pts',(8.63860599473002,46.6462739411471,20.));
#85267=CARTESIAN_POINT('Ctrl Pts',(8.67063478054115,46.6372813177181,0.));
#85268=CARTESIAN_POINT('Ctrl Pts',(8.67063478054115,46.6372813177181,20.));
#85269=CARTESIAN_POINT('Ctrl Pts',(8.70265620297453,46.6282666290119,0.));
#85270=CARTESIAN_POINT('Ctrl Pts',(8.70265620297453,46.6282666290119,20.));
#85271=CARTESIAN_POINT('Ctrl Pts',(8.73467024664569,46.6192298802645,0.));
#85272=CARTESIAN_POINT('Ctrl Pts',(8.73467024664569,46.6192298802645,20.));
#85273=CARTESIAN_POINT('Ctrl Pts',(8.76667689617329,46.6101710767218,0.));
#85274=CARTESIAN_POINT('Ctrl Pts',(8.76667689617329,46.6101710767218,20.));
#85275=CARTESIAN_POINT('Ctrl Pts',(8.79867613617932,46.6010902236408,0.));
#85276=CARTESIAN_POINT('Ctrl Pts',(8.79867613617932,46.6010902236408,20.));
#85277=CARTESIAN_POINT('Ctrl Pts',(8.83066795128933,46.59198732629,0.));
#85278=CARTESIAN_POINT('Ctrl Pts',(8.83066795128933,46.59198732629,20.));
#85279=CARTESIAN_POINT('Ctrl Pts',(8.86265232613214,46.582862389949,0.));
#85280=CARTESIAN_POINT('Ctrl Pts',(8.86265232613214,46.582862389949,20.));
#85281=CARTESIAN_POINT('Ctrl Pts',(8.89462924533988,46.5737154199087,0.));
#85282=CARTESIAN_POINT('Ctrl Pts',(8.89462924533988,46.5737154199087,20.));
#85283=CARTESIAN_POINT('Ctrl Pts',(8.92659869354787,46.5645464214705,0.));
#85284=CARTESIAN_POINT('Ctrl Pts',(8.92659869354787,46.5645464214705,20.));
#85285=CARTESIAN_POINT('Ctrl Pts',(8.9585606553947,46.5553553999467,0.));
#85286=CARTESIAN_POINT('Ctrl Pts',(8.9585606553947,46.5553553999467,20.));
#85287=CARTESIAN_POINT('Ctrl Pts',(8.99051511552228,46.5461423606602,0.));
#85288=CARTESIAN_POINT('Ctrl Pts',(8.99051511552228,46.5461423606602,20.));
#85289=CARTESIAN_POINT('Ctrl Pts',(9.02246205857627,46.5369073089453,0.));
#85290=CARTESIAN_POINT('Ctrl Pts',(9.02246205857627,46.5369073089453,20.));
#85291=CARTESIAN_POINT('Ctrl Pts',(9.05440146920514,46.5276502501459,0.));
#85292=CARTESIAN_POINT('Ctrl Pts',(9.05440146920514,46.5276502501459,20.));
#85293=CARTESIAN_POINT('Ctrl Pts',(9.08633333206089,46.5183711896174,0.));
#85294=CARTESIAN_POINT('Ctrl Pts',(9.08633333206089,46.5183711896174,20.));
#85295=CARTESIAN_POINT('Ctrl Pts',(9.11825763179851,46.5090701327255,0.));
#85296=CARTESIAN_POINT('Ctrl Pts',(9.11825763179851,46.5090701327255,20.));
#85297=CARTESIAN_POINT('Ctrl Pts',(9.15017435307665,46.4997470848477,0.));
#85298=CARTESIAN_POINT('Ctrl Pts',(9.15017435307665,46.4997470848477,20.));
#85299=CARTESIAN_POINT('Ctrl Pts',(9.18208348055724,46.4904020513722,0.));
#85300=CARTESIAN_POINT('Ctrl Pts',(9.18208348055724,46.4904020513722,20.));
#85301=CARTESIAN_POINT('Ctrl Pts',(9.21398499890591,46.4810350376983,0.));
#85302=CARTESIAN_POINT('Ctrl Pts',(9.21398499890591,46.4810350376983,20.));
#85303=CARTESIAN_POINT('Ctrl Pts',(9.2458788927917,46.4716460492361,0.));
#85304=CARTESIAN_POINT('Ctrl Pts',(9.2458788927917,46.4716460492361,20.));
#85305=CARTESIAN_POINT('Ctrl Pts',(9.27776514688698,46.4622350914066,0.));
#85306=CARTESIAN_POINT('Ctrl Pts',(9.27776514688698,46.4622350914066,20.));
#85307=CARTESIAN_POINT('Ctrl Pts',(9.30964374586751,46.4528021696416,0.));
#85308=CARTESIAN_POINT('Ctrl Pts',(9.30964374586751,46.4528021696416,20.));
#85309=CARTESIAN_POINT('Ctrl Pts',(9.3415146744124,46.4433472893837,0.));
#85310=CARTESIAN_POINT('Ctrl Pts',(9.3415146744124,46.4433472893837,20.));
#85311=CARTESIAN_POINT('Ctrl Pts',(9.37337791720392,46.4338704560856,0.));
#85312=CARTESIAN_POINT('Ctrl Pts',(9.37337791720392,46.4338704560856,20.));
#85313=CARTESIAN_POINT('Ctrl Pts',(9.40523345892773,46.4243716752115,0.));
#85314=CARTESIAN_POINT('Ctrl Pts',(9.40523345892773,46.4243716752115,20.));
#85315=CARTESIAN_POINT('Ctrl Pts',(9.43708128427273,46.4148509522358,0.));
#85316=CARTESIAN_POINT('Ctrl Pts',(9.43708128427273,46.4148509522358,20.));
#85317=CARTESIAN_POINT('Ctrl Pts',(9.46892137793147,46.405308292644,0.));
#85318=CARTESIAN_POINT('Ctrl Pts',(9.46892137793147,46.405308292644,20.));
#85319=CARTESIAN_POINT('Ctrl Pts',(9.50075372460008,46.3957437019326,0.));
#85320=CARTESIAN_POINT('Ctrl Pts',(9.50075372460008,46.3957437019326,20.));
#85321=CARTESIAN_POINT('Ctrl Pts',(9.5325783089785,46.3861571856095,0.));
#85322=CARTESIAN_POINT('Ctrl Pts',(9.5325783089785,46.3861571856095,20.));
#85323=CARTESIAN_POINT('Ctrl Pts',(9.56439511577022,46.3765487491938,0.));
#85324=CARTESIAN_POINT('Ctrl Pts',(9.56439511577022,46.3765487491938,20.));
#85325=CARTESIAN_POINT('Ctrl Pts',(9.59620412968212,46.3669183982155,0.));
#85326=CARTESIAN_POINT('Ctrl Pts',(9.59620412968212,46.3669183982155,20.));
#85327=CARTESIAN_POINT('Ctrl Pts',(9.62800533542435,46.3572661382147,0.));
#85328=CARTESIAN_POINT('Ctrl Pts',(9.62800533542435,46.3572661382147,20.));
#85329=CARTESIAN_POINT('Ctrl Pts',(9.65979871771038,46.347591974742,0.));
#85330=CARTESIAN_POINT('Ctrl Pts',(9.65979871771038,46.347591974742,20.));
#85331=CARTESIAN_POINT('Ctrl Pts',(9.69158426125691,46.3378959133587,0.));
#85332=CARTESIAN_POINT('Ctrl Pts',(9.69158426125691,46.3378959133587,20.));
#85333=CARTESIAN_POINT('Ctrl Pts',(9.72336195078413,46.3281779596367,0.));
#85334=CARTESIAN_POINT('Ctrl Pts',(9.72336195078413,46.3281779596367,20.));
#85335=CARTESIAN_POINT('Ctrl Pts',(9.75513177101576,46.3184381191592,0.));
#85336=CARTESIAN_POINT('Ctrl Pts',(9.75513177101576,46.3184381191592,20.));
#85337=CARTESIAN_POINT('Ctrl Pts',(9.78689370667939,46.3086763975205,0.));
#85338=CARTESIAN_POINT('Ctrl Pts',(9.78689370667939,46.3086763975205,20.));
#85339=CARTESIAN_POINT('Ctrl Pts',(9.81864774250618,46.2988928003257,0.));
#85340=CARTESIAN_POINT('Ctrl Pts',(9.81864774250618,46.2988928003257,20.));
#85341=CARTESIAN_POINT('Ctrl Pts',(9.85039386323084,46.289087333191,0.));
#85342=CARTESIAN_POINT('Ctrl Pts',(9.85039386323084,46.289087333191,20.));
#85343=CARTESIAN_POINT('Ctrl Pts',(9.8821320535919,46.2792600017436,0.));
#85344=CARTESIAN_POINT('Ctrl Pts',(9.8821320535919,46.2792600017436,20.));
#85345=CARTESIAN_POINT('Ctrl Pts',(9.91386229833136,46.2694108116213,0.));
#85346=CARTESIAN_POINT('Ctrl Pts',(9.91386229833136,46.2694108116213,20.));
#85347=CARTESIAN_POINT('Ctrl Pts',(9.94558458219445,46.2595397684724,0.));
#85348=CARTESIAN_POINT('Ctrl Pts',(9.94558458219445,46.2595397684724,20.));
#85349=CARTESIAN_POINT('Ctrl Pts',(9.97729888992979,46.2496468779557,0.));
#85350=CARTESIAN_POINT('Ctrl Pts',(9.97729888992979,46.2496468779557,20.));
#85351=CARTESIAN_POINT('Ctrl Pts',(10.0090052062894,46.2397321457408,0.));
#85352=CARTESIAN_POINT('Ctrl Pts',(10.0090052062894,46.2397321457408,20.));
#85353=CARTESIAN_POINT('Ctrl Pts',(10.0407035160292,46.2297955775084,0.));
#85354=CARTESIAN_POINT('Ctrl Pts',(10.0407035160292,46.2297955775084,20.));
#85355=CARTESIAN_POINT('Ctrl Pts',(10.0723938039086,46.2198371789501,0.));
#85356=CARTESIAN_POINT('Ctrl Pts',(10.0723938039086,46.2198371789501,20.));
#85357=CARTESIAN_POINT('Ctrl Pts',(10.1040760546909,46.2098569557688,0.));
#85358=CARTESIAN_POINT('Ctrl Pts',(10.1040760546909,46.2098569557688,20.));
#85359=CARTESIAN_POINT('Ctrl Pts',(10.1357502531431,46.1998549136779,0.));
#85360=CARTESIAN_POINT('Ctrl Pts',(10.1357502531431,46.1998549136779,20.));
#85361=CARTESIAN_POINT('Ctrl Pts',(10.1674163840354,46.1898310584014,0.));
#85362=CARTESIAN_POINT('Ctrl Pts',(10.1674163840354,46.1898310584014,20.));
#85363=CARTESIAN_POINT('Ctrl Pts',(10.199074432142,46.179785395674,0.));
#85364=CARTESIAN_POINT('Ctrl Pts',(10.199074432142,46.179785395674,20.));
#85365=CARTESIAN_POINT('Ctrl Pts',(10.2307243822402,46.169717931241,0.));
#85366=CARTESIAN_POINT('Ctrl Pts',(10.2307243822402,46.169717931241,20.));
#85367=CARTESIAN_POINT('Ctrl Pts',(10.2623662191113,46.1596286708586,0.));
#85368=CARTESIAN_POINT('Ctrl Pts',(10.2623662191113,46.1596286708586,20.));
#85369=CARTESIAN_POINT('Ctrl Pts',(10.2939999275403,46.1495176202946,0.));
#85370=CARTESIAN_POINT('Ctrl Pts',(10.2939999275403,46.1495176202946,20.));
#85371=CARTESIAN_POINT('Ctrl Pts',(10.3256254923155,46.139384785327,0.));
#85372=CARTESIAN_POINT('Ctrl Pts',(10.3256254923155,46.139384785327,20.));
#85373=CARTESIAN_POINT('Ctrl Pts',(10.3572428982293,46.1292301717445,0.));
#85374=CARTESIAN_POINT('Ctrl Pts',(10.3572428982293,46.1292301717445,20.));
#85375=CARTESIAN_POINT('Ctrl Pts',(10.3888521300773,46.119053785347,0.));
#85376=CARTESIAN_POINT('Ctrl Pts',(10.3888521300773,46.119053785347,20.));
#85377=CARTESIAN_POINT('Ctrl Pts',(10.4204531726593,46.1088556319449,0.));
#85378=CARTESIAN_POINT('Ctrl Pts',(10.4204531726593,46.1088556319449,20.));
#85379=CARTESIAN_POINT('Ctrl Pts',(10.4520460107784,46.0986357173598,0.));
#85380=CARTESIAN_POINT('Ctrl Pts',(10.4520460107784,46.0986357173598,20.));
#85381=CARTESIAN_POINT('Ctrl Pts',(10.4836306292415,46.0883940474237,0.));
#85382=CARTESIAN_POINT('Ctrl Pts',(10.4836306292415,46.0883940474237,20.));
#85383=CARTESIAN_POINT('Ctrl Pts',(10.5152070128592,46.0781306279792,0.));
#85384=CARTESIAN_POINT('Ctrl Pts',(10.5152070128592,46.0781306279792,20.));
#85385=CARTESIAN_POINT('Ctrl Pts',(10.5467751464457,46.0678454648793,0.));
#85386=CARTESIAN_POINT('Ctrl Pts',(10.5467751464457,46.0678454648793,20.));
#85387=CARTESIAN_POINT('Ctrl Pts',(10.5783350148187,46.0575385639878,0.));
#85388=CARTESIAN_POINT('Ctrl Pts',(10.5783350148187,46.0575385639878,20.));
#85389=CARTESIAN_POINT('Ctrl Pts',(10.6098866028001,46.0472099311799,0.));
#85390=CARTESIAN_POINT('Ctrl Pts',(10.6098866028001,46.0472099311799,20.));
#85391=CARTESIAN_POINT('Ctrl Pts',(10.6414298952151,46.0368595723418,0.));
#85392=CARTESIAN_POINT('Ctrl Pts',(10.6414298952151,46.0368595723418,20.));
#85393=CARTESIAN_POINT('Ctrl Pts',(10.6729648768932,46.0264874933706,0.));
#85394=CARTESIAN_POINT('Ctrl Pts',(10.6729648768932,46.0264874933706,20.));
#85395=CARTESIAN_POINT('Ctrl Pts',(10.7044915326674,46.0160937001747,0.));
#85396=CARTESIAN_POINT('Ctrl Pts',(10.7044915326674,46.0160937001747,20.));
#85397=CARTESIAN_POINT('Ctrl Pts',(10.7360098473747,46.0056781986726,0.));
#85398=CARTESIAN_POINT('Ctrl Pts',(10.7360098473747,46.0056781986726,20.));
#85399=CARTESIAN_POINT('Ctrl Pts',(10.7675198058554,45.9952409947932,0.));
#85400=CARTESIAN_POINT('Ctrl Pts',(10.7675198058554,45.9952409947932,20.));
#85401=CARTESIAN_POINT('Ctrl Pts',(10.7990213929536,45.9847820944759,0.));
#85402=CARTESIAN_POINT('Ctrl Pts',(10.7990213929536,45.9847820944759,20.));
#85403=CARTESIAN_POINT('Ctrl Pts',(10.8305145935168,45.9743015036702,0.));
#85404=CARTESIAN_POINT('Ctrl Pts',(10.8305145935168,45.9743015036702,20.));
#85405=CARTESIAN_POINT('Ctrl Pts',(10.8619993923966,45.9637992283368,0.));
#85406=CARTESIAN_POINT('Ctrl Pts',(10.8619993923966,45.9637992283368,20.));
#85407=CARTESIAN_POINT('Ctrl Pts',(10.8934757744485,45.9532752744476,0.));
#85408=CARTESIAN_POINT('Ctrl Pts',(10.8934757744485,45.9532752744476,20.));
#85409=CARTESIAN_POINT('Ctrl Pts',(10.9249437245321,45.9427296479861,0.));
#85410=CARTESIAN_POINT('Ctrl Pts',(10.9249437245321,45.9427296479861,20.));
#85411=CARTESIAN_POINT('Ctrl Pts',(10.9564032275107,45.9321623549466,0.));
#85412=CARTESIAN_POINT('Ctrl Pts',(10.9564032275107,45.9321623549466,20.));
#85413=CARTESIAN_POINT('Ctrl Pts',(10.9878542682513,45.9215734013338,0.));
#85414=CARTESIAN_POINT('Ctrl Pts',(10.9878542682513,45.9215734013338,20.));
#85415=CARTESIAN_POINT('Ctrl Pts',(11.0192968316246,45.9109627931629,0.));
#85416=CARTESIAN_POINT('Ctrl Pts',(11.0192968316246,45.9109627931629,20.));
#85417=CARTESIAN_POINT('Ctrl Pts',(11.0507309025052,45.9003305364593,0.));
#85418=CARTESIAN_POINT('Ctrl Pts',(11.0507309025052,45.9003305364593,20.));
#85419=CARTESIAN_POINT('Ctrl Pts',(11.0821564657716,45.8896766372596,0.));
#85420=CARTESIAN_POINT('Ctrl Pts',(11.0821564657716,45.8896766372596,20.));
#85421=CARTESIAN_POINT('Ctrl Pts',(11.1135735063059,45.8790011016108,0.));
#85422=CARTESIAN_POINT('Ctrl Pts',(11.1135735063059,45.8790011016108,20.));
#85423=CARTESIAN_POINT('Ctrl Pts',(11.1449820089942,45.868303935571,0.));
#85424=CARTESIAN_POINT('Ctrl Pts',(11.1449820089942,45.868303935571,20.));
#85425=CARTESIAN_POINT('Ctrl Pts',(11.1763819587262,45.8575851452088,0.));
#85426=CARTESIAN_POINT('Ctrl Pts',(11.1763819587262,45.8575851452088,20.));
#85427=CARTESIAN_POINT('Ctrl Pts',(11.2077733403959,45.8468447366038,0.));
#85428=CARTESIAN_POINT('Ctrl Pts',(11.2077733403959,45.8468447366038,20.));
#85429=CARTESIAN_POINT('Ctrl Pts',(11.2391561389011,45.8360827158468,0.));
#85430=CARTESIAN_POINT('Ctrl Pts',(11.2391561389011,45.8360827158468,20.));
#85431=CARTESIAN_POINT('Ctrl Pts',(11.2705303391434,45.8252990890386,0.));
#85432=CARTESIAN_POINT('Ctrl Pts',(11.2705303391434,45.8252990890386,20.));
#85433=CARTESIAN_POINT('Ctrl Pts',(11.3018959260282,45.8144938622913,0.));
#85434=CARTESIAN_POINT('Ctrl Pts',(11.3018959260282,45.8144938622913,20.));
#85435=CARTESIAN_POINT('Ctrl Pts',(11.3332528844652,45.8036670417272,0.));
#85436=CARTESIAN_POINT('Ctrl Pts',(11.3332528844652,45.8036670417272,20.));
#85437=CARTESIAN_POINT('Ctrl Pts',(11.3646011993673,45.7928186334791,0.));
#85438=CARTESIAN_POINT('Ctrl Pts',(11.3646011993673,45.7928186334791,20.));
#85439=CARTESIAN_POINT('Ctrl Pts',(11.395940855652,45.7819486436912,0.));
#85440=CARTESIAN_POINT('Ctrl Pts',(11.395940855652,45.7819486436912,20.));
#85441=CARTESIAN_POINT('Ctrl Pts',(11.4272718382403,45.7710570785186,0.));
#85442=CARTESIAN_POINT('Ctrl Pts',(11.4272718382403,45.7710570785186,20.));
#85443=CARTESIAN_POINT('Ctrl Pts',(11.4585941320574,45.760143944127,0.));
#85444=CARTESIAN_POINT('Ctrl Pts',(11.4585941320574,45.760143944127,20.));
#85445=CARTESIAN_POINT('Ctrl Pts',(11.489907722032,45.7492092466918,0.));
#85446=CARTESIAN_POINT('Ctrl Pts',(11.489907722032,45.7492092466918,20.));
#85447=CARTESIAN_POINT('Ctrl Pts',(11.5212125930966,45.7382529923996,0.));
#85448=CARTESIAN_POINT('Ctrl Pts',(11.5212125930966,45.7382529923996,20.));
#85449=CARTESIAN_POINT('Ctrl Pts',(11.5525087301884,45.7272751874478,0.));
#85450=CARTESIAN_POINT('Ctrl Pts',(11.5525087301884,45.7272751874478,20.));
#85451=CARTESIAN_POINT('Ctrl Pts',(11.5837961182481,45.7162758380449,0.));
#85452=CARTESIAN_POINT('Ctrl Pts',(11.5837961182481,45.7162758380449,20.));
#85453=CARTESIAN_POINT('Ctrl Pts',(11.6150747422209,45.7052549504103,0.));
#85454=CARTESIAN_POINT('Ctrl Pts',(11.6150747422209,45.7052549504103,20.));
#85455=CARTESIAN_POINT('Ctrl Pts',(11.6463445870557,45.694212530774,0.));
#85456=CARTESIAN_POINT('Ctrl Pts',(11.6463445870557,45.694212530774,20.));
#85457=CARTESIAN_POINT('Ctrl Pts',(11.6776056377055,45.6831485853771,0.));
#85458=CARTESIAN_POINT('Ctrl Pts',(11.6776056377055,45.6831485853771,20.));
#85459=CARTESIAN_POINT('Ctrl Pts',(11.7088578791266,45.6720631204703,0.));
#85460=CARTESIAN_POINT('Ctrl Pts',(11.7088578791266,45.6720631204703,20.));
#85461=CARTESIAN_POINT('Ctrl Pts',(11.7401012962797,45.6609561423149,0.));
#85462=CARTESIAN_POINT('Ctrl Pts',(11.7401012962797,45.6609561423149,20.));
#85463=CARTESIAN_POINT('Ctrl Pts',(11.7713358741292,45.6498276571829,0.));
#85464=CARTESIAN_POINT('Ctrl Pts',(11.7713358741292,45.6498276571829,20.));
#85465=CARTESIAN_POINT('Ctrl Pts',(11.8025615976441,45.6386776713575,0.));
#85466=CARTESIAN_POINT('Ctrl Pts',(11.8025615976441,45.6386776713575,20.));
#85467=CARTESIAN_POINT('Ctrl Pts',(11.8337784517972,45.627506191133,0.));
#85468=CARTESIAN_POINT('Ctrl Pts',(11.8337784517972,45.627506191133,20.));
#85469=CARTESIAN_POINT('Ctrl Pts',(11.8649864215653,45.6163132228138,0.));
#85470=CARTESIAN_POINT('Ctrl Pts',(11.8649864215653,45.6163132228138,20.));
#85471=CARTESIAN_POINT('Ctrl Pts',(11.8961854919293,45.6050987727153,0.));
#85472=CARTESIAN_POINT('Ctrl Pts',(11.8961854919293,45.6050987727153,20.));
#85473=CARTESIAN_POINT('Ctrl Pts',(11.9273756478741,45.5938628471638,0.));
#85474=CARTESIAN_POINT('Ctrl Pts',(11.9273756478741,45.5938628471638,20.));
#85475=CARTESIAN_POINT('Ctrl Pts',(11.9585568743886,45.5826054524963,0.));
#85476=CARTESIAN_POINT('Ctrl Pts',(11.9585568743886,45.5826054524963,20.));
#85477=CARTESIAN_POINT('Ctrl Pts',(11.989729156466,45.5713265950605,0.));
#85478=CARTESIAN_POINT('Ctrl Pts',(11.989729156466,45.5713265950605,20.));
#85479=CARTESIAN_POINT('Ctrl Pts',(12.0208924791034,45.5600262812144,0.));
#85480=CARTESIAN_POINT('Ctrl Pts',(12.0208924791034,45.5600262812144,20.));
#85481=CARTESIAN_POINT('Ctrl Pts',(12.0520468273019,45.5487045173265,0.));
#85482=CARTESIAN_POINT('Ctrl Pts',(12.0520468273019,45.5487045173265,20.));
#85483=CARTESIAN_POINT('Ctrl Pts',(12.0831921860665,45.5373613097755,0.));
#85484=CARTESIAN_POINT('Ctrl Pts',(12.0831921860665,45.5373613097755,20.));
#85485=CARTESIAN_POINT('Ctrl Pts',(12.1143285404065,45.5259966649516,0.));
#85486=CARTESIAN_POINT('Ctrl Pts',(12.1143285404065,45.5259966649516,20.));
#85487=CARTESIAN_POINT('Ctrl Pts',(12.1454558753351,45.5146105892553,0.));
#85488=CARTESIAN_POINT('Ctrl Pts',(12.1454558753351,45.5146105892553,20.));
#85489=CARTESIAN_POINT('Ctrl Pts',(12.1765741758697,45.5032030890978,0.));
#85490=CARTESIAN_POINT('Ctrl Pts',(12.1765741758697,45.5032030890978,20.));
#85491=CARTESIAN_POINT('Ctrl Pts',(12.2076834270323,45.4917741709015,0.));
#85492=CARTESIAN_POINT('Ctrl Pts',(12.2076834270323,45.4917741709015,20.));
#85493=CARTESIAN_POINT('Ctrl Pts',(12.2387836138487,45.4803238410999,0.));
#85494=CARTESIAN_POINT('Ctrl Pts',(12.2387836138487,45.4803238410999,20.));
#85495=CARTESIAN_POINT('Ctrl Pts',(12.269874721349,45.4688521061371,0.));
#85496=CARTESIAN_POINT('Ctrl Pts',(12.269874721349,45.4688521061371,20.));
#85497=CARTESIAN_POINT('Ctrl Pts',(12.3009567345673,45.4573589724673,0.));
#85498=CARTESIAN_POINT('Ctrl Pts',(12.3009567345673,45.4573589724673,20.));
#85499=CARTESIAN_POINT('Ctrl Pts',(12.3320296385417,45.4458444465552,0.));
#85500=CARTESIAN_POINT('Ctrl Pts',(12.3320296385417,45.4458444465552,20.));
#85501=CARTESIAN_POINT('Ctrl Pts',(12.3630934183142,45.4343085348755,0.));
#85502=CARTESIAN_POINT('Ctrl Pts',(12.3630934183142,45.4343085348755,20.));
#85503=CARTESIAN_POINT('Ctrl Pts',(12.3941480589311,45.4227512439136,0.));
#85504=CARTESIAN_POINT('Ctrl Pts',(12.3941480589311,45.4227512439136,20.));
#85505=CARTESIAN_POINT('Ctrl Pts',(12.4251935454428,45.4111725801659,0.));
#85506=CARTESIAN_POINT('Ctrl Pts',(12.4251935454428,45.4111725801659,20.));
#85507=CARTESIAN_POINT('Ctrl Pts',(12.4562298629045,45.3995725501402,0.));
#85508=CARTESIAN_POINT('Ctrl Pts',(12.4562298629045,45.3995725501402,20.));
#85509=CARTESIAN_POINT('Ctrl Pts',(12.4872569963754,45.3879511603549,0.));
#85510=CARTESIAN_POINT('Ctrl Pts',(12.4872569963754,45.3879511603549,20.));
#85511=CARTESIAN_POINT('Ctrl Pts',(12.5182749309189,45.376308417339,0.));
#85512=CARTESIAN_POINT('Ctrl Pts',(12.5182749309189,45.376308417339,20.));
#85513=CARTESIAN_POINT('Ctrl Pts',(12.5492836516023,45.364644327632,0.));
#85514=CARTESIAN_POINT('Ctrl Pts',(12.5492836516023,45.364644327632,20.));
#85515=CARTESIAN_POINT('Ctrl Pts',(12.5802831434966,45.3529588977839,0.));
#85516=CARTESIAN_POINT('Ctrl Pts',(12.5802831434966,45.3529588977839,20.));
#85517=CARTESIAN_POINT('Ctrl Pts',(12.6112733916776,45.3412521343551,0.));
#85518=CARTESIAN_POINT('Ctrl Pts',(12.6112733916776,45.3412521343551,20.));
#85519=CARTESIAN_POINT('Ctrl Pts',(12.6422543812251,45.3295240439169,0.));
#85520=CARTESIAN_POINT('Ctrl Pts',(12.6422543812251,45.3295240439169,20.));
#85521=CARTESIAN_POINT('Ctrl Pts',(12.6732260972239,45.3177746330512,0.));
#85522=CARTESIAN_POINT('Ctrl Pts',(12.6732260972239,45.3177746330512,20.));
#85523=CARTESIAN_POINT('Ctrl Pts',(12.7041885247626,45.3060039083501,0.));
#85524=CARTESIAN_POINT('Ctrl Pts',(12.7041885247626,45.3060039083501,20.));
#85525=CARTESIAN_POINT('Ctrl Pts',(12.7351416489341,45.2942118764167,0.));
#85526=CARTESIAN_POINT('Ctrl Pts',(12.7351416489341,45.2942118764167,20.));
#85527=CARTESIAN_POINT('Ctrl Pts',(12.7660854548354,45.2823985438647,0.));
#85528=CARTESIAN_POINT('Ctrl Pts',(12.7660854548354,45.2823985438647,20.));
#85529=CARTESIAN_POINT('Ctrl Pts',(12.7970199275678,45.2705639173192,0.));
#85530=CARTESIAN_POINT('Ctrl Pts',(12.7970199275678,45.2705639173192,20.));
#85531=CARTESIAN_POINT('Ctrl Pts',(12.8279450522365,45.2587080034157,0.));
#85532=CARTESIAN_POINT('Ctrl Pts',(12.8279450522365,45.2587080034157,20.));
#85533=CARTESIAN_POINT('Ctrl Pts',(12.8588608139512,45.2468308087994,0.));
#85534=CARTESIAN_POINT('Ctrl Pts',(12.8588608139512,45.2468308087994,20.));
#85535=CARTESIAN_POINT('Ctrl Pts',(12.8897671978256,45.2349323401259,0.));
#85536=CARTESIAN_POINT('Ctrl Pts',(12.8897671978256,45.2349323401259,20.));
#85537=CARTESIAN_POINT('Ctrl Pts',(12.9206641889781,45.2230126040617,0.));
#85538=CARTESIAN_POINT('Ctrl Pts',(12.9206641889781,45.2230126040617,20.));
#85539=CARTESIAN_POINT('Ctrl Pts',(12.9515517725313,45.2110716072841,0.));
#85540=CARTESIAN_POINT('Ctrl Pts',(12.9515517725313,45.2110716072841,20.));
#85541=CARTESIAN_POINT('Ctrl Pts',(12.9824299336127,45.199109356482,0.));
#85542=CARTESIAN_POINT('Ctrl Pts',(12.9824299336127,45.199109356482,20.));
#85543=CARTESIAN_POINT('Ctrl Pts',(13.0132986573536,45.1871258583545,0.));
#85544=CARTESIAN_POINT('Ctrl Pts',(13.0132986573536,45.1871258583545,20.));
#85545=CARTESIAN_POINT('Ctrl Pts',(13.0441579288899,45.1751211196118,0.));
#85546=CARTESIAN_POINT('Ctrl Pts',(13.0441579288899,45.1751211196118,20.));
#85547=CARTESIAN_POINT('Ctrl Pts',(13.0750077333613,45.1630951469734,0.));
#85548=CARTESIAN_POINT('Ctrl Pts',(13.0750077333613,45.1630951469734,20.));
#85549=CARTESIAN_POINT('Ctrl Pts',(13.105848055912,45.1510479471692,0.));
#85550=CARTESIAN_POINT('Ctrl Pts',(13.105848055912,45.1510479471692,20.));
#85551=CARTESIAN_POINT('Ctrl Pts',(13.1366788816904,45.1389795269399,0.));
#85552=CARTESIAN_POINT('Ctrl Pts',(13.1366788816904,45.1389795269399,20.));
#85553=CARTESIAN_POINT('Ctrl Pts',(13.1675001958492,45.1268898930368,0.));
#85554=CARTESIAN_POINT('Ctrl Pts',(13.1675001958492,45.1268898930368,20.));
#85555=CARTESIAN_POINT('Ctrl Pts',(13.198311983546,45.114779052223,0.));
#85556=CARTESIAN_POINT('Ctrl Pts',(13.198311983546,45.114779052223,20.));
#85557=CARTESIAN_POINT('Ctrl Pts',(13.2291142299426,45.1026470112717,0.));
#85558=CARTESIAN_POINT('Ctrl Pts',(13.2291142299426,45.1026470112717,20.));
#85559=CARTESIAN_POINT('Ctrl Pts',(13.259906920205,45.0904937769663,0.));
#85560=CARTESIAN_POINT('Ctrl Pts',(13.259906920205,45.0904937769663,20.));
#85561=CARTESIAN_POINT('Ctrl Pts',(13.2906900395037,45.0783193561008,0.));
#85562=CARTESIAN_POINT('Ctrl Pts',(13.2906900395037,45.0783193561008,20.));
#85563=CARTESIAN_POINT('Ctrl Pts',(13.3214635730135,45.0661237554798,0.));
#85564=CARTESIAN_POINT('Ctrl Pts',(13.3214635730135,45.0661237554798,20.));
#85565=CARTESIAN_POINT('Ctrl Pts',(13.3522275059137,45.0539069819185,0.));
#85566=CARTESIAN_POINT('Ctrl Pts',(13.3522275059137,45.0539069819185,20.));
#85567=CARTESIAN_POINT('Ctrl Pts',(13.3829818233878,45.0416690422424,0.));
#85568=CARTESIAN_POINT('Ctrl Pts',(13.3829818233878,45.0416690422424,20.));
#85569=CARTESIAN_POINT('Ctrl Pts',(13.4137265106238,45.029409943288,0.));
#85570=CARTESIAN_POINT('Ctrl Pts',(13.4137265106238,45.029409943288,20.));
#85571=CARTESIAN_POINT('Ctrl Pts',(13.4444615528144,45.0171296919022,0.));
#85572=CARTESIAN_POINT('Ctrl Pts',(13.4444615528144,45.0171296919022,20.));
#85573=CARTESIAN_POINT('Ctrl Pts',(13.4751869351564,45.0048282949433,0.));
#85574=CARTESIAN_POINT('Ctrl Pts',(13.4751869351564,45.0048282949433,20.));
#85575=CARTESIAN_POINT('Ctrl Pts',(13.5059026428512,44.9925057592796,0.));
#85576=CARTESIAN_POINT('Ctrl Pts',(13.5059026428512,44.9925057592796,20.));
#85577=CARTESIAN_POINT('Ctrl Pts',(13.5366086611044,44.9801620917891,0.));
#85578=CARTESIAN_POINT('Ctrl Pts',(13.5366086611044,44.9801620917891,20.));
#85579=CARTESIAN_POINT('Ctrl Pts',(13.5673049751264,44.967797299361,0.));
#85580=CARTESIAN_POINT('Ctrl Pts',(13.5673049751264,44.967797299361,20.));
#85581=CARTESIAN_POINT('Ctrl Pts',(13.5979915701319,44.955411388895,0.));
#85582=CARTESIAN_POINT('Ctrl Pts',(13.5979915701319,44.955411388895,20.));
#85583=CARTESIAN_POINT('Ctrl Pts',(13.6286684313401,44.9430043673018,0.));
#85584=CARTESIAN_POINT('Ctrl Pts',(13.6286684313401,44.9430043673018,20.));
#85585=CARTESIAN_POINT('Ctrl Pts',(13.6593355439745,44.930576241502,0.));
#85586=CARTESIAN_POINT('Ctrl Pts',(13.6593355439745,44.930576241502,20.));
#85587=CARTESIAN_POINT('Ctrl Pts',(13.6899928932632,44.9181270184275,0.));
#85588=CARTESIAN_POINT('Ctrl Pts',(13.6899928932632,44.9181270184275,20.));
#85589=CARTESIAN_POINT('Ctrl Pts',(13.7206404644388,44.9056567050204,0.));
#85590=CARTESIAN_POINT('Ctrl Pts',(13.7206404644388,44.9056567050204,20.));
#85591=CARTESIAN_POINT('Ctrl Pts',(13.7512782427386,44.8931653082334,0.));
#85592=CARTESIAN_POINT('Ctrl Pts',(13.7512782427386,44.8931653082334,20.));
#85593=CARTESIAN_POINT('Ctrl Pts',(13.7819062134042,44.8806528350291,0.));
#85594=CARTESIAN_POINT('Ctrl Pts',(13.7819062134042,44.8806528350291,20.));
#85595=CARTESIAN_POINT('Ctrl Pts',(13.8125243616816,44.8681192923811,0.));
#85596=CARTESIAN_POINT('Ctrl Pts',(13.8125243616816,44.8681192923811,20.));
#85597=CARTESIAN_POINT('Ctrl Pts',(13.8431326728214,44.8555646872732,0.));
#85598=CARTESIAN_POINT('Ctrl Pts',(13.8431326728214,44.8555646872732,20.));
#85599=CARTESIAN_POINT('Ctrl Pts',(13.8737311320789,44.8429890267007,0.));
#85600=CARTESIAN_POINT('Ctrl Pts',(13.8737311320789,44.8429890267007,20.));
#85601=CARTESIAN_POINT('Ctrl Pts',(13.9043197247138,44.8303923176691,0.));
#85602=CARTESIAN_POINT('Ctrl Pts',(13.9043197247138,44.8303923176691,20.));
#85603=CARTESIAN_POINT('Ctrl Pts',(13.9348984359903,44.8177745671945,0.));
#85604=CARTESIAN_POINT('Ctrl Pts',(13.9348984359903,44.8177745671945,20.));
#85605=CARTESIAN_POINT('Ctrl Pts',(13.9654672511774,44.8051357823031,0.));
#85606=CARTESIAN_POINT('Ctrl Pts',(13.9654672511774,44.8051357823031,20.));
#85607=CARTESIAN_POINT('Ctrl Pts',(13.9960261555481,44.7924759700314,0.));
#85608=CARTESIAN_POINT('Ctrl Pts',(13.9960261555481,44.7924759700314,20.));
#85609=CARTESIAN_POINT('Ctrl Pts',(14.0265751343805,44.7797951374262,0.));
#85610=CARTESIAN_POINT('Ctrl Pts',(14.0265751343805,44.7797951374262,20.));
#85611=CARTESIAN_POINT('Ctrl Pts',(14.057114172957,44.7670932915455,0.));
#85612=CARTESIAN_POINT('Ctrl Pts',(14.057114172957,44.7670932915455,20.));
#85613=CARTESIAN_POINT('Ctrl Pts',(14.0876432565649,44.7543704394583,0.));
#85614=CARTESIAN_POINT('Ctrl Pts',(14.0876432565649,44.7543704394583,20.));
#85615=CARTESIAN_POINT('Ctrl Pts',(14.118162370496,44.7416265882443,0.));
#85616=CARTESIAN_POINT('Ctrl Pts',(14.118162370496,44.7416265882443,20.));
#85617=CARTESIAN_POINT('Ctrl Pts',(14.1486715000464,44.728861744993,0.));
#85618=CARTESIAN_POINT('Ctrl Pts',(14.1486715000464,44.728861744993,20.));
#85619=CARTESIAN_POINT('Ctrl Pts',(14.1791706305171,44.7160759168044,0.));
#85620=CARTESIAN_POINT('Ctrl Pts',(14.1791706305171,44.7160759168044,20.));
#85621=CARTESIAN_POINT('Ctrl Pts',(14.2096597472134,44.7032691107881,0.));
#85622=CARTESIAN_POINT('Ctrl Pts',(14.2096597472134,44.7032691107881,20.));
#85623=CARTESIAN_POINT('Ctrl Pts',(14.2401388354454,44.690441334065,0.));
#85624=CARTESIAN_POINT('Ctrl Pts',(14.2401388354454,44.690441334065,20.));
#85625=CARTESIAN_POINT('Ctrl Pts',(14.2706078805279,44.6775925937661,0.));
#85626=CARTESIAN_POINT('Ctrl Pts',(14.2706078805279,44.6775925937661,20.));
#85627=CARTESIAN_POINT('Ctrl Pts',(14.3010668677802,44.6647228970333,0.));
#85628=CARTESIAN_POINT('Ctrl Pts',(14.3010668677802,44.6647228970333,20.));
#85629=CARTESIAN_POINT('Ctrl Pts',(14.3315157825264,44.6518322510194,0.));
#85630=CARTESIAN_POINT('Ctrl Pts',(14.3315157825264,44.6518322510194,20.));
#85631=CARTESIAN_POINT('Ctrl Pts',(14.3619546100951,44.6389206628876,0.));
#85632=CARTESIAN_POINT('Ctrl Pts',(14.3619546100951,44.6389206628876,20.));
#85633=CARTESIAN_POINT('Ctrl Pts',(14.3923833358197,44.6259881398119,0.));
#85634=CARTESIAN_POINT('Ctrl Pts',(14.3923833358197,44.6259881398119,20.));
#85635=CARTESIAN_POINT('Ctrl Pts',(14.4228019450383,44.613034688977,0.));
#85636=CARTESIAN_POINT('Ctrl Pts',(14.4228019450383,44.613034688977,20.));
#85637=CARTESIAN_POINT('Ctrl Pts',(14.4532104230936,44.6000603175775,0.));
#85638=CARTESIAN_POINT('Ctrl Pts',(14.4532104230936,44.6000603175775,20.));
#85639=CARTESIAN_POINT('Ctrl Pts',(14.4836087553332,44.5870650328188,0.));
#85640=CARTESIAN_POINT('Ctrl Pts',(14.4836087553332,44.5870650328188,20.));
#85641=CARTESIAN_POINT('Ctrl Pts',(14.5139969271087,44.5740488419152,0.));
#85642=CARTESIAN_POINT('Ctrl Pts',(14.5139969271087,44.5740488419152,20.));
#85643=CARTESIAN_POINT('Ctrl Pts',(14.5443749237767,44.5610117520915,0.));
#85644=CARTESIAN_POINT('Ctrl Pts',(14.5443749237767,44.5610117520915,20.));
#85645=CARTESIAN_POINT('Ctrl Pts',(14.5747427306988,44.5479537705835,0.));
#85646=CARTESIAN_POINT('Ctrl Pts',(14.5747427306988,44.5479537705835,20.));
#85647=CARTESIAN_POINT('Ctrl Pts',(14.6051003332411,44.5348749046379,0.));
#85648=CARTESIAN_POINT('Ctrl Pts',(14.6051003332411,44.5348749046379,20.));
#85649=CARTESIAN_POINT('Ctrl Pts',(14.6354477167742,44.521775161512,0.));
#85650=CARTESIAN_POINT('Ctrl Pts',(14.6354477167742,44.521775161512,20.));
#85651=CARTESIAN_POINT('Ctrl Pts',(14.6657848666743,44.5086545484757,0.));
#85652=CARTESIAN_POINT('Ctrl Pts',(14.6657848666743,44.5086545484757,20.));
#85653=CARTESIAN_POINT('Ctrl Pts',(14.6961117683217,44.4955130728078,0.));
#85654=CARTESIAN_POINT('Ctrl Pts',(14.6961117683217,44.4955130728078,20.));
#85655=CARTESIAN_POINT('Ctrl Pts',(14.7264284071013,44.4823507417973,0.));
#85656=CARTESIAN_POINT('Ctrl Pts',(14.7264284071013,44.4823507417973,20.));
#85657=CARTESIAN_POINT('Ctrl Pts',(14.7567347684029,44.469167562743,0.));
#85658=CARTESIAN_POINT('Ctrl Pts',(14.7567347684029,44.469167562743,20.));
#85659=CARTESIAN_POINT('Ctrl Pts',(14.7870308376214,44.4559635429545,0.));
#85660=CARTESIAN_POINT('Ctrl Pts',(14.7870308376214,44.4559635429545,20.));
#85661=CARTESIAN_POINT('Ctrl Pts',(14.817316600156,44.4427386897515,0.));
#85662=CARTESIAN_POINT('Ctrl Pts',(14.817316600156,44.4427386897515,20.));
#85663=CARTESIAN_POINT('Ctrl Pts',(14.8475920414107,44.4294930104636,0.));
#85664=CARTESIAN_POINT('Ctrl Pts',(14.8475920414107,44.4294930104636,20.));
#85665=CARTESIAN_POINT('Ctrl Pts',(14.8778571467943,44.416226512431,0.));
#85666=CARTESIAN_POINT('Ctrl Pts',(14.8778571467943,44.416226512431,20.));
#85667=CARTESIAN_POINT('Ctrl Pts',(14.9081119017199,44.4029392030043,0.));
#85668=CARTESIAN_POINT('Ctrl Pts',(14.9081119017199,44.4029392030043,20.));
#85669=CARTESIAN_POINT('Ctrl Pts',(14.9383562916061,44.389631089546,0.));
#85670=CARTESIAN_POINT('Ctrl Pts',(14.9383562916061,44.389631089546,20.));
#85671=CARTESIAN_POINT('Ctrl Pts',(14.9685903018767,44.3763021794296,0.));
#85672=CARTESIAN_POINT('Ctrl Pts',(14.9685903018767,44.3763021794296,20.));
#85673=CARTESIAN_POINT('Ctrl Pts',(14.9988139179602,44.3629524800397,0.));
#85674=CARTESIAN_POINT('Ctrl Pts',(14.9988139179602,44.3629524800397,20.));
#85675=CARTESIAN_POINT('Ctrl Pts',(15.0290271252899,44.3495819987708,0.));
#85676=CARTESIAN_POINT('Ctrl Pts',(15.0290271252899,44.3495819987708,20.));
#85677=CARTESIAN_POINT('Ctrl Pts',(15.0592299093032,44.3361907430254,0.));
#85678=CARTESIAN_POINT('Ctrl Pts',(15.0592299093032,44.3361907430254,20.));
#85679=CARTESIAN_POINT('Ctrl Pts',(15.0894222554424,44.3227787202166,0.));
#85680=CARTESIAN_POINT('Ctrl Pts',(15.0894222554424,44.3227787202166,20.));
#85681=CARTESIAN_POINT('Ctrl Pts',(15.1196041491546,44.3093459377674,0.));
#85682=CARTESIAN_POINT('Ctrl Pts',(15.1196041491546,44.3093459377674,20.));
#85683=CARTESIAN_POINT('Ctrl Pts',(15.1497755758917,44.2958924031118,0.));
#85684=CARTESIAN_POINT('Ctrl Pts',(15.1497755758917,44.2958924031118,20.));
#85685=CARTESIAN_POINT('Ctrl Pts',(15.1799365211113,44.2824181236961,0.));
#85686=CARTESIAN_POINT('Ctrl Pts',(15.1799365211113,44.2824181236961,20.));
#85687=CARTESIAN_POINT('Ctrl Pts',(15.2100869702755,44.2689231069767,0.));
#85688=CARTESIAN_POINT('Ctrl Pts',(15.2100869702755,44.2689231069767,20.));
#85689=CARTESIAN_POINT('Ctrl Pts',(15.2402269088514,44.2554073604206,0.));
#85690=CARTESIAN_POINT('Ctrl Pts',(15.2402269088514,44.2554073604206,20.));
#85691=CARTESIAN_POINT('Ctrl Pts',(15.2703563223108,44.2418708915045,0.));
#85692=CARTESIAN_POINT('Ctrl Pts',(15.2703563223108,44.2418708915045,20.));
#85693=CARTESIAN_POINT('Ctrl Pts',(15.30047519613,44.2283137077152,0.));
#85694=CARTESIAN_POINT('Ctrl Pts',(15.30047519613,44.2283137077152,20.));
#85695=CARTESIAN_POINT('Ctrl Pts',(15.3305835157903,44.2147358165492,0.));
#85696=CARTESIAN_POINT('Ctrl Pts',(15.3305835157903,44.2147358165492,20.));
#85697=CARTESIAN_POINT('Ctrl Pts',(15.3606812667781,44.201137225514,0.));
#85698=CARTESIAN_POINT('Ctrl Pts',(15.3606812667781,44.201137225514,20.));
#85699=CARTESIAN_POINT('Ctrl Pts',(15.390768434585,44.1875179421286,0.));
#85700=CARTESIAN_POINT('Ctrl Pts',(15.390768434585,44.1875179421286,20.));
#85701=CARTESIAN_POINT('Ctrl Pts',(15.4208450047077,44.1738779739225,0.));
#85702=CARTESIAN_POINT('Ctrl Pts',(15.4208450047077,44.1738779739225,20.));
#85703=CARTESIAN_POINT('Ctrl Pts',(15.4509109626472,44.1602173284345,0.));
#85704=CARTESIAN_POINT('Ctrl Pts',(15.4509109626472,44.1602173284345,20.));
#85705=CARTESIAN_POINT('Ctrl Pts',(15.4809662939093,44.146536013213,0.));
#85706=CARTESIAN_POINT('Ctrl Pts',(15.4809662939093,44.146536013213,20.));
#85707=CARTESIAN_POINT('Ctrl Pts',(15.5110109840047,44.1328340358171,0.));
#85708=CARTESIAN_POINT('Ctrl Pts',(15.5110109840047,44.1328340358171,20.));
#85709=CARTESIAN_POINT('Ctrl Pts',(15.5410450184494,44.1191114038164,0.));
#85710=CARTESIAN_POINT('Ctrl Pts',(15.5410450184494,44.1191114038164,20.));
#85711=CARTESIAN_POINT('Ctrl Pts',(15.5710683827645,44.1053681247921,0.));
#85712=CARTESIAN_POINT('Ctrl Pts',(15.5710683827645,44.1053681247921,20.));
#85713=CARTESIAN_POINT('Ctrl Pts',(15.6010810624766,44.0916042063371,0.));
#85714=CARTESIAN_POINT('Ctrl Pts',(15.6010810624766,44.0916042063371,20.));
#85715=CARTESIAN_POINT('Ctrl Pts',(15.6310830431167,44.0778196560536,0.));
#85716=CARTESIAN_POINT('Ctrl Pts',(15.6310830431167,44.0778196560536,20.));
#85717=CARTESIAN_POINT('Ctrl Pts',(15.6610743102207,44.0640144815534,0.));
#85718=CARTESIAN_POINT('Ctrl Pts',(15.6610743102207,44.0640144815534,20.));
#85719=CARTESIAN_POINT('Ctrl Pts',(15.6910548493288,44.050188690457,0.));
#85720=CARTESIAN_POINT('Ctrl Pts',(15.6910548493288,44.050188690457,20.));
#85721=CARTESIAN_POINT('Ctrl Pts',(15.7210246459867,44.0363422903955,0.));
#85722=CARTESIAN_POINT('Ctrl Pts',(15.7210246459867,44.0363422903955,20.));
#85723=CARTESIAN_POINT('Ctrl Pts',(15.7509836857452,44.0224752890112,0.));
#85724=CARTESIAN_POINT('Ctrl Pts',(15.7509836857452,44.0224752890112,20.));
#85725=CARTESIAN_POINT('Ctrl Pts',(15.7809319541601,44.0085876939576,0.));
#85726=CARTESIAN_POINT('Ctrl Pts',(15.7809319541601,44.0085876939576,20.));
#85727=CARTESIAN_POINT('Ctrl Pts',(15.8108694367927,43.9946795128988,0.));
#85728=CARTESIAN_POINT('Ctrl Pts',(15.8108694367927,43.9946795128988,20.));
#85729=CARTESIAN_POINT('Ctrl Pts',(15.8407961192089,43.9807507535097,0.));
#85730=CARTESIAN_POINT('Ctrl Pts',(15.8407961192089,43.9807507535097,20.));
#85731=CARTESIAN_POINT('Ctrl Pts',(15.8707119869797,43.9668014234746,0.));
#85732=CARTESIAN_POINT('Ctrl Pts',(15.8707119869797,43.9668014234746,20.));
#85733=CARTESIAN_POINT('Ctrl Pts',(15.9006170256808,43.9528315304878,0.));
#85734=CARTESIAN_POINT('Ctrl Pts',(15.9006170256808,43.9528315304878,20.));
#85735=CARTESIAN_POINT('Ctrl Pts',(15.9305112208934,43.9388410822542,0.));
#85736=CARTESIAN_POINT('Ctrl Pts',(15.9305112208934,43.9388410822542,20.));
#85737=CARTESIAN_POINT('Ctrl Pts',(15.9603945582034,43.9248300864889,0.));
#85738=CARTESIAN_POINT('Ctrl Pts',(15.9603945582034,43.9248300864889,20.));
#85739=CARTESIAN_POINT('Ctrl Pts',(15.9902670232019,43.9107985509168,0.));
#85740=CARTESIAN_POINT('Ctrl Pts',(15.9902670232019,43.9107985509168,20.));
#85741=CARTESIAN_POINT('Ctrl Pts',(16.0201286014849,43.896746483274,0.));
#85742=CARTESIAN_POINT('Ctrl Pts',(16.0201286014849,43.896746483274,20.));
#85743=CARTESIAN_POINT('Ctrl Pts',(16.0499792786541,43.8826738913074,0.));
#85744=CARTESIAN_POINT('Ctrl Pts',(16.0499792786541,43.8826738913074,20.));
#85745=CARTESIAN_POINT('Ctrl Pts',(16.0798190403159,43.8685807827745,0.));
#85746=CARTESIAN_POINT('Ctrl Pts',(16.0798190403159,43.8685807827745,20.));
#85747=CARTESIAN_POINT('Ctrl Pts',(16.1096478720818,43.854467165442,0.));
#85748=CARTESIAN_POINT('Ctrl Pts',(16.1096478720818,43.854467165442,20.));
#85749=CARTESIAN_POINT('Ctrl Pts',(16.1394657595683,43.8403330470868,0.));
#85750=CARTESIAN_POINT('Ctrl Pts',(16.1394657595683,43.8403330470868,20.));
#85751=CARTESIAN_POINT('Ctrl Pts',(16.1692726883968,43.8261784354962,0.));
#85752=CARTESIAN_POINT('Ctrl Pts',(16.1692726883968,43.8261784354962,20.));
#85753=CARTESIAN_POINT('Ctrl Pts',(16.199068644194,43.8120033384679,0.));
#85754=CARTESIAN_POINT('Ctrl Pts',(16.199068644194,43.8120033384679,20.));
#85755=CARTESIAN_POINT('Ctrl Pts',(16.2288536125916,43.7978077638098,0.));
#85756=CARTESIAN_POINT('Ctrl Pts',(16.2288536125916,43.7978077638098,20.));
#85757=CARTESIAN_POINT('Ctrl Pts',(16.2586275792268,43.7835917193404,0.));
#85758=CARTESIAN_POINT('Ctrl Pts',(16.2586275792268,43.7835917193404,20.));
#85759=CARTESIAN_POINT('Ctrl Pts',(16.2883905297415,43.7693552128887,0.));
#85760=CARTESIAN_POINT('Ctrl Pts',(16.2883905297415,43.7693552128887,20.));
#85761=CARTESIAN_POINT('Ctrl Pts',(16.3181424497834,43.7550982522947,0.));
#85762=CARTESIAN_POINT('Ctrl Pts',(16.3181424497834,43.7550982522947,20.));
#85763=CARTESIAN_POINT('Ctrl Pts',(16.3478833250055,43.7408208454089,0.));
#85764=CARTESIAN_POINT('Ctrl Pts',(16.3478833250055,43.7408208454089,20.));
#85765=CARTESIAN_POINT('Ctrl Pts',(16.3776131410651,43.7265230000909,0.));
#85766=CARTESIAN_POINT('Ctrl Pts',(16.3776131410651,43.7265230000909,20.));
#85767=CARTESIAN_POINT('Ctrl Pts',(16.4073318836249,43.7122047242097,0.));
#85768=CARTESIAN_POINT('Ctrl Pts',(16.4073318836249,43.7122047242097,20.));
#85769=CARTESIAN_POINT('Ctrl Pts',(16.4370395383523,43.6978660256455,0.));
#85770=CARTESIAN_POINT('Ctrl Pts',(16.4370395383523,43.6978660256455,20.));
#85771=CARTESIAN_POINT('Ctrl Pts',(16.4667360909206,43.6835069122887,0.));
#85772=CARTESIAN_POINT('Ctrl Pts',(16.4667360909206,43.6835069122887,20.));
#85773=CARTESIAN_POINT('Ctrl Pts',(16.4964215270082,43.6691273920409,0.));
#85774=CARTESIAN_POINT('Ctrl Pts',(16.4964215270082,43.6691273920409,20.));
#85775=CARTESIAN_POINT('Ctrl Pts',(16.5260958322991,43.6547274728139,0.));
#85776=CARTESIAN_POINT('Ctrl Pts',(16.5260958322991,43.6547274728139,20.));
#85777=CARTESIAN_POINT('Ctrl Pts',(16.5557589924819,43.640307162529,0.));
#85778=CARTESIAN_POINT('Ctrl Pts',(16.5557589924819,43.640307162529,20.));
#85779=CARTESIAN_POINT('Ctrl Pts',(16.5854109932504,43.6258664691173,0.));
#85780=CARTESIAN_POINT('Ctrl Pts',(16.5854109932504,43.6258664691173,20.));
#85781=CARTESIAN_POINT('Ctrl Pts',(16.6150518203036,43.6114054005208,0.));
#85782=CARTESIAN_POINT('Ctrl Pts',(16.6150518203036,43.6114054005208,20.));
#85783=CARTESIAN_POINT('Ctrl Pts',(16.6446814593458,43.5969239646926,0.));
#85784=CARTESIAN_POINT('Ctrl Pts',(16.6446814593458,43.5969239646926,20.));
#85785=CARTESIAN_POINT('Ctrl Pts',(16.6742998960869,43.5824221695961,0.));
#85786=CARTESIAN_POINT('Ctrl Pts',(16.6742998960869,43.5824221695961,20.));
#85787=CARTESIAN_POINT('Ctrl Pts',(16.7039071162413,43.5679000232041,0.));
#85788=CARTESIAN_POINT('Ctrl Pts',(16.7039071162413,43.5679000232041,20.));
#85789=CARTESIAN_POINT('Ctrl Pts',(16.7335031055294,43.5533575334996,0.));
#85790=CARTESIAN_POINT('Ctrl Pts',(16.7335031055294,43.5533575334996,20.));
#85791=CARTESIAN_POINT('Ctrl Pts',(16.7630878496767,43.5387947084755,0.));
#85792=CARTESIAN_POINT('Ctrl Pts',(16.7630878496767,43.5387947084755,20.));
#85793=CARTESIAN_POINT('Ctrl Pts',(16.792661334414,43.5242115561352,0.));
#85794=CARTESIAN_POINT('Ctrl Pts',(16.792661334414,43.5242115561352,20.));
#85795=CARTESIAN_POINT('Ctrl Pts',(16.8222235454772,43.5096080844922,0.));
#85796=CARTESIAN_POINT('Ctrl Pts',(16.8222235454772,43.5096080844922,20.));
#85797=CARTESIAN_POINT('Ctrl Pts',(16.8517744686076,43.4949843015709,0.));
#85798=CARTESIAN_POINT('Ctrl Pts',(16.8517744686076,43.4949843015709,20.));
#85799=CARTESIAN_POINT('Ctrl Pts',(16.8813140895513,43.4803402154062,0.));
#85800=CARTESIAN_POINT('Ctrl Pts',(16.8813140895513,43.4803402154062,20.));
#85801=CARTESIAN_POINT('Ctrl Pts',(16.91084239406,43.4656758340435,0.));
#85802=CARTESIAN_POINT('Ctrl Pts',(16.91084239406,43.4656758340435,20.));
#85803=CARTESIAN_POINT('Ctrl Pts',(16.9403593678908,43.4509911655382,0.));
#85804=CARTESIAN_POINT('Ctrl Pts',(16.9403593678908,43.4509911655382,20.));
#85805=CARTESIAN_POINT('Ctrl Pts',(16.9698649968061,43.4362862179557,0.));
#85806=CARTESIAN_POINT('Ctrl Pts',(16.9698649968061,43.4362862179557,20.));
#85807=CARTESIAN_POINT('Ctrl Pts',(16.9993592665737,43.4215609993712,0.));
#85808=CARTESIAN_POINT('Ctrl Pts',(16.9993592665737,43.4215609993712,20.));
#85809=CARTESIAN_POINT('Ctrl Pts',(17.0288421629666,43.4068155178696,0.));
#85810=CARTESIAN_POINT('Ctrl Pts',(17.0288421629666,43.4068155178696,20.));
#85811=CARTESIAN_POINT('Ctrl Pts',(17.0583136717632,43.3920497815463,0.));
#85812=CARTESIAN_POINT('Ctrl Pts',(17.0583136717632,43.3920497815463,20.));
#85813=CARTESIAN_POINT('Ctrl Pts',(17.0877737787472,43.3772637985072,0.));
#85814=CARTESIAN_POINT('Ctrl Pts',(17.0877737787472,43.3772637985072,20.));
#85815=CARTESIAN_POINT('Ctrl Pts',(17.1172224697079,43.3624575768695,0.));
#85816=CARTESIAN_POINT('Ctrl Pts',(17.1172224697079,43.3624575768695,20.));
#85817=CARTESIAN_POINT('Ctrl Pts',(17.1466597304397,43.3476311247602,0.));
#85818=CARTESIAN_POINT('Ctrl Pts',(17.1466597304397,43.3476311247602,20.));
#85819=CARTESIAN_POINT('Ctrl Pts',(17.1760855467426,43.332784450317,0.));
#85820=CARTESIAN_POINT('Ctrl Pts',(17.1760855467426,43.332784450317,20.));
#85821=CARTESIAN_POINT('Ctrl Pts',(17.2054999044212,43.3179175616862,0.));
#85822=CARTESIAN_POINT('Ctrl Pts',(17.2054999044212,43.3179175616862,20.));
#85823=CARTESIAN_POINT('Ctrl Pts',(17.2349027892859,43.3030304670242,0.));
#85824=CARTESIAN_POINT('Ctrl Pts',(17.2349027892859,43.3030304670242,20.));
#85825=CARTESIAN_POINT('Ctrl Pts',(17.2642941871522,43.2881231744974,0.));
#85826=CARTESIAN_POINT('Ctrl Pts',(17.2642941871522,43.2881231744974,20.));
#85827=CARTESIAN_POINT('Ctrl Pts',(17.2936740838416,43.2731956922839,0.));
#85828=CARTESIAN_POINT('Ctrl Pts',(17.2936740838416,43.2731956922839,20.));
#85829=CARTESIAN_POINT('Ctrl Pts',(17.3230424651811,43.258248028572,0.));
#85830=CARTESIAN_POINT('Ctrl Pts',(17.3230424651811,43.258248028572,20.));
#85831=CARTESIAN_POINT('Ctrl Pts',(17.352399317003,43.2432801915607,0.));
#85832=CARTESIAN_POINT('Ctrl Pts',(17.352399317003,43.2432801915607,20.));
#85833=CARTESIAN_POINT('Ctrl Pts',(17.3817446251452,43.2282921894589,0.));
#85834=CARTESIAN_POINT('Ctrl Pts',(17.3817446251452,43.2282921894589,20.));
#85835=CARTESIAN_POINT('Ctrl Pts',(17.4110783754507,43.2132840304854,0.));
#85836=CARTESIAN_POINT('Ctrl Pts',(17.4110783754507,43.2132840304854,20.));
#85837=CARTESIAN_POINT('Ctrl Pts',(17.4404005537678,43.1982557228684,0.));
#85838=CARTESIAN_POINT('Ctrl Pts',(17.4404005537678,43.1982557228684,20.));
#85839=CARTESIAN_POINT('Ctrl Pts',(17.46971114595,43.1832072748459,0.));
#85840=CARTESIAN_POINT('Ctrl Pts',(17.46971114595,43.1832072748459,20.));
#85841=CARTESIAN_POINT('Ctrl Pts',(17.4990101378563,43.1681386946662,0.));
#85842=CARTESIAN_POINT('Ctrl Pts',(17.4990101378563,43.1681386946662,20.));
#85843=CARTESIAN_POINT('Ctrl Pts',(17.5282975153509,43.1530499905879,0.));
#85844=CARTESIAN_POINT('Ctrl Pts',(17.5282975153509,43.1530499905879,20.));
#85845=CARTESIAN_POINT('Ctrl Pts',(17.557573264304,43.1379411708804,0.));
#85846=CARTESIAN_POINT('Ctrl Pts',(17.557573264304,43.1379411708804,20.));
#85847=CARTESIAN_POINT('Ctrl Pts',(17.5868373705916,43.122812243824,0.));
#85848=CARTESIAN_POINT('Ctrl Pts',(17.5868373705916,43.122812243824,20.));
#85849=CARTESIAN_POINT('Ctrl Pts',(17.6160898200949,43.1076632177089,0.));
#85850=CARTESIAN_POINT('Ctrl Pts',(17.6160898200949,43.1076632177089,20.));
#85851=CARTESIAN_POINT('Ctrl Pts',(17.645330598701,43.0924941008354,0.));
#85852=CARTESIAN_POINT('Ctrl Pts',(17.645330598701,43.0924941008354,20.));
#85853=CARTESIAN_POINT('Ctrl Pts',(17.674559692302,43.0773049015137,0.));
#85854=CARTESIAN_POINT('Ctrl Pts',(17.674559692302,43.0773049015137,20.));
#85855=CARTESIAN_POINT('Ctrl Pts',(17.7037770867956,43.0620956280638,0.));
#85856=CARTESIAN_POINT('Ctrl Pts',(17.7037770867956,43.0620956280638,20.));
#85857=CARTESIAN_POINT('Ctrl Pts',(17.7329827680846,43.0468662888157,0.));
#85858=CARTESIAN_POINT('Ctrl Pts',(17.7329827680846,43.0468662888157,20.));
#85859=CARTESIAN_POINT('Ctrl Pts',(17.7621767220773,43.0316168921093,0.));
#85860=CARTESIAN_POINT('Ctrl Pts',(17.7621767220773,43.0316168921093,20.));
#85861=CARTESIAN_POINT('Ctrl Pts',(17.7913589346876,43.0163474462951,0.));
#85862=CARTESIAN_POINT('Ctrl Pts',(17.7913589346876,43.0163474462951,20.));
#85863=CARTESIAN_POINT('Ctrl Pts',(17.8205293918351,43.0010579597341,0.));
#85864=CARTESIAN_POINT('Ctrl Pts',(17.8205293918351,43.0010579597341,20.));
#85865=CARTESIAN_POINT('Ctrl Pts',(17.8496880794454,42.985748440798,0.));
#85866=CARTESIAN_POINT('Ctrl Pts',(17.8496880794454,42.985748440798,20.));
#85867=CARTESIAN_POINT('Ctrl Pts',(17.8788349834491,42.9704188978681,0.));
#85868=CARTESIAN_POINT('Ctrl Pts',(17.8788349834491,42.9704188978681,20.));
#85869=CARTESIAN_POINT('Ctrl Pts',(17.9079700897828,42.9550693393359,0.));
#85870=CARTESIAN_POINT('Ctrl Pts',(17.9079700897828,42.9550693393359,20.));
#85871=CARTESIAN_POINT('Ctrl Pts',(17.9370933843882,42.9396997736018,0.));
#85872=CARTESIAN_POINT('Ctrl Pts',(17.9370933843882,42.9396997736018,20.));
#85873=CARTESIAN_POINT('Ctrl Pts',(17.9662048532126,42.9243102090766,0.));
#85874=CARTESIAN_POINT('Ctrl Pts',(17.9662048532126,42.9243102090766,20.));
#85875=CARTESIAN_POINT('Ctrl Pts',(17.9953044822088,42.9089006541818,0.));
#85876=CARTESIAN_POINT('Ctrl Pts',(17.9953044822088,42.9089006541818,20.));
#85877=CARTESIAN_POINT('Ctrl Pts',(18.0243922573354,42.8934711173491,0.));
#85878=CARTESIAN_POINT('Ctrl Pts',(18.0243922573354,42.8934711173491,20.));
#85879=CARTESIAN_POINT('Ctrl Pts',(18.0534681645565,42.8780216070205,0.));
#85880=CARTESIAN_POINT('Ctrl Pts',(18.0534681645565,42.8780216070205,20.));
#85881=CARTESIAN_POINT('Ctrl Pts',(18.0825321898416,42.8625521316489,0.));
#85882=CARTESIAN_POINT('Ctrl Pts',(18.0825321898416,42.8625521316489,20.));
#85883=CARTESIAN_POINT('Ctrl Pts',(18.1115843191668,42.8470626996976,0.));
#85884=CARTESIAN_POINT('Ctrl Pts',(18.1115843191668,42.8470626996976,20.));
#85885=CARTESIAN_POINT('Ctrl Pts',(18.1406245385131,42.831553319639,0.));
#85886=CARTESIAN_POINT('Ctrl Pts',(18.1406245385131,42.831553319639,20.));
#85887=CARTESIAN_POINT('Ctrl Pts',(18.1696528338673,42.8160239999555,0.));
#85888=CARTESIAN_POINT('Ctrl Pts',(18.1696528338673,42.8160239999555,20.));
#85889=CARTESIAN_POINT('Ctrl Pts',(18.1986691912208,42.8004747491375,0.));
#85890=CARTESIAN_POINT('Ctrl Pts',(18.1986691912208,42.8004747491375,20.));
#85891=CARTESIAN_POINT('Ctrl Pts',(18.2276735965714,42.7849055756869,0.));
#85892=CARTESIAN_POINT('Ctrl Pts',(18.2276735965714,42.7849055756869,20.));
#85893=CARTESIAN_POINT('Ctrl Pts',(18.256666035922,42.7693164881155,0.));
#85894=CARTESIAN_POINT('Ctrl Pts',(18.256666035922,42.7693164881155,20.));
#85895=CARTESIAN_POINT('Ctrl Pts',(18.285646495282,42.7537074949463,0.));
#85896=CARTESIAN_POINT('Ctrl Pts',(18.285646495282,42.7537074949463,20.));
#85897=CARTESIAN_POINT('Ctrl Pts',(18.3146149606662,42.7380786047127,0.));
#85898=CARTESIAN_POINT('Ctrl Pts',(18.3146149606662,42.7380786047127,20.));
#85899=CARTESIAN_POINT('Ctrl Pts',(18.3435714180954,42.7224298259587,0.));
#85900=CARTESIAN_POINT('Ctrl Pts',(18.3435714180954,42.7224298259587,20.));
#85901=CARTESIAN_POINT('Ctrl Pts',(18.372515853596,42.7067611672378,0.));
#85902=CARTESIAN_POINT('Ctrl Pts',(18.372515853596,42.7067611672378,20.));
#85903=CARTESIAN_POINT('Ctrl Pts',(18.4014482531999,42.6910726371132,0.));
#85904=CARTESIAN_POINT('Ctrl Pts',(18.4014482531999,42.6910726371132,20.));
#85905=CARTESIAN_POINT('Ctrl Pts',(18.4303686029443,42.6753642441576,0.));
#85906=CARTESIAN_POINT('Ctrl Pts',(18.4303686029443,42.6753642441576,20.));
#85907=CARTESIAN_POINT('Ctrl Pts',(18.4592768888724,42.6596359969538,0.));
#85908=CARTESIAN_POINT('Ctrl Pts',(18.4592768888724,42.6596359969538,20.));
#85909=CARTESIAN_POINT('Ctrl Pts',(18.4881730970326,42.6438879040941,0.));
#85910=CARTESIAN_POINT('Ctrl Pts',(18.4881730970326,42.6438879040941,20.));
#85911=CARTESIAN_POINT('Ctrl Pts',(18.5170572134793,42.6281199741818,0.));
#85912=CARTESIAN_POINT('Ctrl Pts',(18.5170572134793,42.6281199741818,20.));
#85913=CARTESIAN_POINT('Ctrl Pts',(18.5459292242727,42.61233221583,0.));
#85914=CARTESIAN_POINT('Ctrl Pts',(18.5459292242727,42.61233221583,20.));
#85915=CARTESIAN_POINT('Ctrl Pts',(18.574789115479,42.596524637663,0.));
#85916=CARTESIAN_POINT('Ctrl Pts',(18.574789115479,42.596524637663,20.));
#85917=CARTESIAN_POINT('Ctrl Pts',(18.6036368731702,42.5806972483146,0.));
#85918=CARTESIAN_POINT('Ctrl Pts',(18.6036368731702,42.5806972483146,20.));
#85919=CARTESIAN_POINT('Ctrl Pts',(18.6324724834239,42.5648500564287,0.));
#85920=CARTESIAN_POINT('Ctrl Pts',(18.6324724834239,42.5648500564287,20.));
#85921=CARTESIAN_POINT('Ctrl Pts',(18.6612959323233,42.5489830706585,0.));
#85922=CARTESIAN_POINT('Ctrl Pts',(18.6612959323233,42.5489830706585,20.));
#85923=CARTESIAN_POINT('Ctrl Pts',(18.6901072059567,42.5330962996668,0.));
#85924=CARTESIAN_POINT('Ctrl Pts',(18.6901072059567,42.5330962996668,20.));
#85925=CARTESIAN_POINT('Ctrl Pts',(18.718906290419,42.517189752127,0.));
#85926=CARTESIAN_POINT('Ctrl Pts',(18.718906290419,42.517189752127,20.));
#85927=CARTESIAN_POINT('Ctrl Pts',(18.7476931718101,42.5012634367222,0.));
#85928=CARTESIAN_POINT('Ctrl Pts',(18.7476931718101,42.5012634367222,20.));
#85929=CARTESIAN_POINT('Ctrl Pts',(18.7764678362367,42.4853173621469,0.));
#85930=CARTESIAN_POINT('Ctrl Pts',(18.7764678362367,42.4853173621469,20.));
#85931=CARTESIAN_POINT('Ctrl Pts',(18.8052302698113,42.4693515371059,0.));
#85932=CARTESIAN_POINT('Ctrl Pts',(18.8052302698113,42.4693515371059,20.));
#85933=CARTESIAN_POINT('Ctrl Pts',(18.8339804586522,42.4533659703145,0.));
#85934=CARTESIAN_POINT('Ctrl Pts',(18.8339804586522,42.4533659703145,20.));
#85935=CARTESIAN_POINT('Ctrl Pts',(18.8627183888827,42.4373606704956,0.));
#85936=CARTESIAN_POINT('Ctrl Pts',(18.8627183888827,42.4373606704956,20.));
#85937=CARTESIAN_POINT('Ctrl Pts',(18.8914440466322,42.4213356463824,0.));
#85938=CARTESIAN_POINT('Ctrl Pts',(18.8914440466322,42.4213356463824,20.));
#85939=CARTESIAN_POINT('Ctrl Pts',(18.9201574180352,42.4052909067172,0.));
#85940=CARTESIAN_POINT('Ctrl Pts',(18.9201574180352,42.4052909067172,20.));
#85941=CARTESIAN_POINT('Ctrl Pts',(18.9488584892326,42.389226460254,0.));
#85942=CARTESIAN_POINT('Ctrl Pts',(18.9488584892326,42.389226460254,20.));
#85943=CARTESIAN_POINT('Ctrl Pts',(18.9775472463711,42.3731423157568,0.));
#85944=CARTESIAN_POINT('Ctrl Pts',(18.9775472463711,42.3731423157568,20.));
#85945=CARTESIAN_POINT('Ctrl Pts',(19.0062236756035,42.3570384820003,0.));
#85946=CARTESIAN_POINT('Ctrl Pts',(19.0062236756035,42.3570384820003,20.));
#85947=CARTESIAN_POINT('Ctrl Pts',(19.0348877630887,42.3409149677685,0.));
#85948=CARTESIAN_POINT('Ctrl Pts',(19.0348877630887,42.3409149677685,20.));
#85949=CARTESIAN_POINT('Ctrl Pts',(19.0635394949913,42.3247717818558,0.));
#85950=CARTESIAN_POINT('Ctrl Pts',(19.0635394949913,42.3247717818558,20.));
#85951=CARTESIAN_POINT('Ctrl Pts',(19.0921788574819,42.3086089330658,0.));
#85952=CARTESIAN_POINT('Ctrl Pts',(19.0921788574819,42.3086089330658,20.));
#85953=CARTESIAN_POINT('Ctrl Pts',(19.1208058367362,42.2924264302113,0.));
#85954=CARTESIAN_POINT('Ctrl Pts',(19.1208058367362,42.2924264302113,20.));
#85955=CARTESIAN_POINT('Ctrl Pts',(19.1494204189361,42.2762242821163,0.));
#85956=CARTESIAN_POINT('Ctrl Pts',(19.1494204189361,42.2762242821163,20.));
#85957=CARTESIAN_POINT('Ctrl Pts',(19.1780225902694,42.2600024976146,0.));
#85958=CARTESIAN_POINT('Ctrl Pts',(19.1780225902694,42.2600024976146,20.));
#85959=CARTESIAN_POINT('Ctrl Pts',(19.2066123369297,42.2437610855506,0.));
#85960=CARTESIAN_POINT('Ctrl Pts',(19.2066123369297,42.2437610855506,20.));
#85961=CARTESIAN_POINT('Ctrl Pts',(19.2351896451166,42.2275000547783,0.));
#85962=CARTESIAN_POINT('Ctrl Pts',(19.2351896451166,42.2275000547783,20.));
#85963=CARTESIAN_POINT('Ctrl Pts',(19.2637545010356,42.2112194141618,0.));
#85964=CARTESIAN_POINT('Ctrl Pts',(19.2637545010356,42.2112194141618,20.));
#85965=CARTESIAN_POINT('Ctrl Pts',(19.2923068908981,42.1949191725745,0.));
#85966=CARTESIAN_POINT('Ctrl Pts',(19.2923068908981,42.1949191725745,20.));
#85967=CARTESIAN_POINT('Ctrl Pts',(19.3208468009211,42.1785993388989,0.));
#85968=CARTESIAN_POINT('Ctrl Pts',(19.3208468009211,42.1785993388989,20.));
#85969=CARTESIAN_POINT('Ctrl Pts',(19.3493742173282,42.1622599220289,0.));
#85970=CARTESIAN_POINT('Ctrl Pts',(19.3493742173282,42.1622599220289,20.));
#85971=CARTESIAN_POINT('Ctrl Pts',(19.377889126349,42.1459009308685,0.));
#85972=CARTESIAN_POINT('Ctrl Pts',(19.377889126349,42.1459009308685,20.));
#85973=CARTESIAN_POINT('Ctrl Pts',(19.4063915142187,42.1295223743319,0.));
#85974=CARTESIAN_POINT('Ctrl Pts',(19.4063915142187,42.1295223743319,20.));
#85975=CARTESIAN_POINT('Ctrl Pts',(19.4348813671784,42.1131242613432,0.));
#85976=CARTESIAN_POINT('Ctrl Pts',(19.4348813671784,42.1131242613432,20.));
#85977=CARTESIAN_POINT('Ctrl Pts',(19.4633586714748,42.0967066008354,0.));
#85978=CARTESIAN_POINT('Ctrl Pts',(19.4633586714748,42.0967066008354,20.));
#85979=CARTESIAN_POINT('Ctrl Pts',(19.4918234133604,42.080269401751,0.));
#85980=CARTESIAN_POINT('Ctrl Pts',(19.4918234133604,42.080269401751,20.));
#85981=CARTESIAN_POINT('Ctrl Pts',(19.5202755790939,42.0638126730426,0.));
#85982=CARTESIAN_POINT('Ctrl Pts',(19.5202755790939,42.0638126730426,20.));
#85983=CARTESIAN_POINT('Ctrl Pts',(19.5487151549408,42.0473364236742,0.));
#85984=CARTESIAN_POINT('Ctrl Pts',(19.5487151549408,42.0473364236742,20.));
#85985=CARTESIAN_POINT('Ctrl Pts',(19.5771421271718,42.0308406626191,0.));
#85986=CARTESIAN_POINT('Ctrl Pts',(19.5771421271718,42.0308406626191,20.));
#85987=CARTESIAN_POINT('Ctrl Pts',(19.6055564820642,42.0143253988608,0.));
#85988=CARTESIAN_POINT('Ctrl Pts',(19.6055564820642,42.0143253988608,20.));
#85989=CARTESIAN_POINT('Ctrl Pts',(19.6339582059008,41.997790641393,0.));
#85990=CARTESIAN_POINT('Ctrl Pts',(19.6339582059008,41.997790641393,20.));
#85991=CARTESIAN_POINT('Ctrl Pts',(19.6623472849704,41.9812363992182,0.));
#85992=CARTESIAN_POINT('Ctrl Pts',(19.6623472849704,41.9812363992182,20.));
#85993=CARTESIAN_POINT('Ctrl Pts',(19.6907237055674,41.9646626813489,0.));
#85994=CARTESIAN_POINT('Ctrl Pts',(19.6907237055674,41.9646626813489,20.));
#85995=CARTESIAN_POINT('Ctrl Pts',(19.7190874539927,41.9480694968077,0.));
#85996=CARTESIAN_POINT('Ctrl Pts',(19.7190874539927,41.9480694968077,20.));
#85997=CARTESIAN_POINT('Ctrl Pts',(19.7474385165531,41.9314568546275,0.));
#85998=CARTESIAN_POINT('Ctrl Pts',(19.7474385165531,41.9314568546275,20.));
#85999=CARTESIAN_POINT('Ctrl Pts',(19.7757768795619,41.9148247638512,0.));
#86000=CARTESIAN_POINT('Ctrl Pts',(19.7757768795619,41.9148247638512,20.));
#86001=CARTESIAN_POINT('Ctrl Pts',(19.8041025293385,41.8981732335313,0.));
#86002=CARTESIAN_POINT('Ctrl Pts',(19.8041025293385,41.8981732335313,20.));
#86003=CARTESIAN_POINT('Ctrl Pts',(19.8324154522082,41.8815022727306,0.));
#86004=CARTESIAN_POINT('Ctrl Pts',(19.8324154522082,41.8815022727306,20.));
#86005=CARTESIAN_POINT('Ctrl Pts',(19.8607156345021,41.8648118905217,0.));
#86006=CARTESIAN_POINT('Ctrl Pts',(19.8607156345021,41.8648118905217,20.));
#86007=CARTESIAN_POINT('Ctrl Pts',(19.889003062557,41.8481020959867,0.));
#86008=CARTESIAN_POINT('Ctrl Pts',(19.889003062557,41.8481020959867,20.));
#86009=CARTESIAN_POINT('Ctrl Pts',(19.9172777227157,41.8313728982175,0.));
#86010=CARTESIAN_POINT('Ctrl Pts',(19.9172777227157,41.8313728982175,20.));
#86011=CARTESIAN_POINT('Ctrl Pts',(19.9455396013269,41.8146243063152,0.));
#86012=CARTESIAN_POINT('Ctrl Pts',(19.9455396013269,41.8146243063152,20.));
#86013=CARTESIAN_POINT('Ctrl Pts',(19.9737886847461,41.7978563293914,0.));
#86014=CARTESIAN_POINT('Ctrl Pts',(19.9737886847461,41.7978563293914,20.));
#86015=CARTESIAN_POINT('Ctrl Pts',(20.0020249593348,41.7810689765679,0.));
#86016=CARTESIAN_POINT('Ctrl Pts',(20.0020249593348,41.7810689765679,20.));
#86017=CARTESIAN_POINT('Ctrl Pts',(20.0302484114611,41.7642622569769,0.));
#86018=CARTESIAN_POINT('Ctrl Pts',(20.0302484114611,41.7642622569769,20.));
#86019=CARTESIAN_POINT('Ctrl Pts',(20.0584590274991,41.7474361797609,0.));
#86020=CARTESIAN_POINT('Ctrl Pts',(20.0584590274991,41.7474361797609,20.));
#86021=CARTESIAN_POINT('Ctrl Pts',(20.0866567938287,41.7305907540713,0.));
#86022=CARTESIAN_POINT('Ctrl Pts',(20.0866567938287,41.7305907540713,20.));
#86023=CARTESIAN_POINT('Ctrl Pts',(20.1148416968357,41.7137259890696,0.));
#86024=CARTESIAN_POINT('Ctrl Pts',(20.1148416968357,41.7137259890696,20.));
#86025=CARTESIAN_POINT('Ctrl Pts',(20.1430137229118,41.6968418939263,0.));
#86026=CARTESIAN_POINT('Ctrl Pts',(20.1430137229118,41.6968418939263,20.));
#86027=CARTESIAN_POINT('Ctrl Pts',(20.1711728584548,41.6799384778218,0.));
#86028=CARTESIAN_POINT('Ctrl Pts',(20.1711728584548,41.6799384778218,20.));
#86029=CARTESIAN_POINT('Ctrl Pts',(20.199319089869,41.6630157499462,0.));
#86030=CARTESIAN_POINT('Ctrl Pts',(20.199319089869,41.6630157499462,20.));
#86031=CARTESIAN_POINT('Ctrl Pts',(20.2274524035648,41.6460737195007,0.));
#86032=CARTESIAN_POINT('Ctrl Pts',(20.2274524035648,41.6460737195007,20.));
#86033=CARTESIAN_POINT('Ctrl Pts',(20.2555727859589,41.6291123956959,0.));
#86034=CARTESIAN_POINT('Ctrl Pts',(20.2555727859589,41.6291123956959,20.));
#86035=CARTESIAN_POINT('Ctrl Pts',(20.2836802234745,41.6121317877528,0.));
#86036=CARTESIAN_POINT('Ctrl Pts',(20.2836802234745,41.6121317877528,20.));
#86037=CARTESIAN_POINT('Ctrl Pts',(20.3117747025404,41.5951319049016,0.));
#86038=CARTESIAN_POINT('Ctrl Pts',(20.3117747025404,41.5951319049016,20.));
#86039=CARTESIAN_POINT('Ctrl Pts',(20.3398562095916,41.5781127563818,0.));
#86040=CARTESIAN_POINT('Ctrl Pts',(20.3398562095916,41.5781127563818,20.));
#86041=CARTESIAN_POINT('Ctrl Pts',(20.3679247310694,41.561074351443,0.));
#86042=CARTESIAN_POINT('Ctrl Pts',(20.3679247310694,41.561074351443,20.));
#86043=CARTESIAN_POINT('Ctrl Pts',(20.395980253421,41.5440166993445,0.));
#86044=CARTESIAN_POINT('Ctrl Pts',(20.395980253421,41.5440166993445,20.));
#86045=CARTESIAN_POINT('Ctrl Pts',(20.4240227631002,41.5269398093561,0.));
#86046=CARTESIAN_POINT('Ctrl Pts',(20.4240227631002,41.5269398093561,20.));
#86047=CARTESIAN_POINT('Ctrl Pts',(20.4520522465668,41.5098436907568,0.));
#86048=CARTESIAN_POINT('Ctrl Pts',(20.4520522465668,41.5098436907568,20.));
#86049=CARTESIAN_POINT('Ctrl Pts',(20.4800686902869,41.4927283528358,0.));
#86050=CARTESIAN_POINT('Ctrl Pts',(20.4800686902869,41.4927283528358,20.));
#86051=CARTESIAN_POINT('Ctrl Pts',(20.5080720807336,41.4755938048931,0.));
#86052=CARTESIAN_POINT('Ctrl Pts',(20.5080720807336,41.4755938048931,20.));
#86053=CARTESIAN_POINT('Ctrl Pts',(20.5360624043854,41.4584400562379,0.));
#86054=CARTESIAN_POINT('Ctrl Pts',(20.5360624043854,41.4584400562379,20.));
#86055=CARTESIAN_POINT('Ctrl Pts',(20.5640396477269,41.4412671161883,0.));
#86056=CARTESIAN_POINT('Ctrl Pts',(20.5640396477269,41.4412671161883,20.));
#86057=CARTESIAN_POINT('Ctrl Pts',(20.5920037972489,41.4240749940722,0.));
#86058=CARTESIAN_POINT('Ctrl Pts',(20.5920037972489,41.4240749940722,20.));
#86059=CARTESIAN_POINT('Ctrl Pts',(20.6199548394484,41.4068636992265,0.));
#86060=CARTESIAN_POINT('Ctrl Pts',(20.6199548394484,41.4068636992265,20.));
#86061=CARTESIAN_POINT('Ctrl Pts',(20.6478927608288,41.3896332409988,0.));
#86062=CARTESIAN_POINT('Ctrl Pts',(20.6478927608288,41.3896332409988,20.));
#86063=CARTESIAN_POINT('Ctrl Pts',(20.6758175479,41.3723836287471,0.));
#86064=CARTESIAN_POINT('Ctrl Pts',(20.6758175479,41.3723836287471,20.));
#86065=CARTESIAN_POINT('Ctrl Pts',(20.7037291871782,41.3551148718389,0.));
#86066=CARTESIAN_POINT('Ctrl Pts',(20.7037291871782,41.3551148718389,20.));
#86067=CARTESIAN_POINT('Ctrl Pts',(20.731627665186,41.3378269796522,0.));
#86068=CARTESIAN_POINT('Ctrl Pts',(20.731627665186,41.3378269796522,20.));
#86069=CARTESIAN_POINT('Ctrl Pts',(20.7595129684521,41.3205199615745,0.));
#86070=CARTESIAN_POINT('Ctrl Pts',(20.7595129684521,41.3205199615745,20.));
#86071=CARTESIAN_POINT('Ctrl Pts',(20.7873850835117,41.303193827003,0.));
#86072=CARTESIAN_POINT('Ctrl Pts',(20.7873850835117,41.303193827003,20.));
#86073=CARTESIAN_POINT('Ctrl Pts',(20.8152439969059,41.285848585344,0.));
#86074=CARTESIAN_POINT('Ctrl Pts',(20.8152439969059,41.285848585344,20.));
#86075=CARTESIAN_POINT('Ctrl Pts',(20.8430896951822,41.268484246013,0.));
#86076=CARTESIAN_POINT('Ctrl Pts',(20.8430896951822,41.268484246013,20.));
#86077=CARTESIAN_POINT('Ctrl Pts',(20.8709221648944,41.2511008184358,0.));
#86078=CARTESIAN_POINT('Ctrl Pts',(20.8709221648944,41.2511008184358,20.));
#86079=CARTESIAN_POINT('Ctrl Pts',(20.8987413926025,41.2336983120481,0.));
#86080=CARTESIAN_POINT('Ctrl Pts',(20.8987413926025,41.2336983120481,20.));
#86081=CARTESIAN_POINT('Ctrl Pts',(20.9265473648728,41.2162767362953,0.));
#86082=CARTESIAN_POINT('Ctrl Pts',(20.9265473648728,41.2162767362953,20.));
#86083=CARTESIAN_POINT('Ctrl Pts',(20.9543400682781,41.1988361006333,0.));
#86084=CARTESIAN_POINT('Ctrl Pts',(20.9543400682781,41.1988361006333,20.));
#86085=CARTESIAN_POINT('Ctrl Pts',(20.9821194893979,41.1813764145274,0.));
#86086=CARTESIAN_POINT('Ctrl Pts',(20.9821194893979,41.1813764145274,20.));
#86087=CARTESIAN_POINT('Ctrl Pts',(21.009885614818,41.1638976874526,0.));
#86088=CARTESIAN_POINT('Ctrl Pts',(21.009885614818,41.1638976874526,20.));
#86089=CARTESIAN_POINT('Ctrl Pts',(21.0376384311301,41.1463999288927,0.));
#86090=CARTESIAN_POINT('Ctrl Pts',(21.0376384311301,41.1463999288927,20.));
#86091=CARTESIAN_POINT('Ctrl Pts',(21.0653779249329,41.128883148342,0.));
#86092=CARTESIAN_POINT('Ctrl Pts',(21.0653779249329,41.128883148342,20.));
#86093=CARTESIAN_POINT('Ctrl Pts',(21.093104082831,41.1113473553046,0.));
#86094=CARTESIAN_POINT('Ctrl Pts',(21.093104082831,41.1113473553046,20.));
#86095=CARTESIAN_POINT('Ctrl Pts',(21.1208168914355,41.0937925592944,0.));
#86096=CARTESIAN_POINT('Ctrl Pts',(21.1208168914355,41.0937925592944,20.));
#86097=CARTESIAN_POINT('Ctrl Pts',(21.1485163373635,41.076218769835,0.));
#86098=CARTESIAN_POINT('Ctrl Pts',(21.1485163373635,41.076218769835,20.));
#86099=CARTESIAN_POINT('Ctrl Pts',(21.1762024072388,41.0586259964597,0.));
#86100=CARTESIAN_POINT('Ctrl Pts',(21.1762024072388,41.0586259964597,20.));
#86101=CARTESIAN_POINT('Ctrl Pts',(21.2038750876913,41.0410142487106,0.));
#86102=CARTESIAN_POINT('Ctrl Pts',(21.2038750876913,41.0410142487106,20.));
#86103=CARTESIAN_POINT('Ctrl Pts',(21.2315343653574,41.0233835361399,0.));
#86104=CARTESIAN_POINT('Ctrl Pts',(21.2315343653574,41.0233835361399,20.));
#86105=CARTESIAN_POINT('Ctrl Pts',(21.25918022688,41.0057338683097,0.));
#86106=CARTESIAN_POINT('Ctrl Pts',(21.25918022688,41.0057338683097,20.));
#86107=CARTESIAN_POINT('Ctrl Pts',(21.286812658909,40.9880652547928,0.));
#86108=CARTESIAN_POINT('Ctrl Pts',(21.286812658909,40.9880652547928,20.));
#86109=CARTESIAN_POINT('Ctrl Pts',(21.3144316481011,40.9703777051716,0.));
#86110=CARTESIAN_POINT('Ctrl Pts',(21.3144316481011,40.9703777051716,20.));
#86111=CARTESIAN_POINT('Ctrl Pts',(21.342037181119,40.9526712290373,0.));
#86112=CARTESIAN_POINT('Ctrl Pts',(21.342037181119,40.9526712290373,20.));
#86113=CARTESIAN_POINT('Ctrl Pts',(21.3696292446317,40.9349458359905,0.));
#86114=CARTESIAN_POINT('Ctrl Pts',(21.3696292446317,40.9349458359905,20.));
#86115=CARTESIAN_POINT('Ctrl Pts',(21.3972078253142,40.9172015356414,0.));
#86116=CARTESIAN_POINT('Ctrl Pts',(21.3972078253142,40.9172015356414,20.));
#86117=CARTESIAN_POINT('Ctrl Pts',(21.4247729098479,40.8994383376102,0.));
#86118=CARTESIAN_POINT('Ctrl Pts',(21.4247729098479,40.8994383376102,20.));
#86119=CARTESIAN_POINT('Ctrl Pts',(21.4523244849199,40.8816562515268,0.));
#86120=CARTESIAN_POINT('Ctrl Pts',(21.4523244849199,40.8816562515268,20.));
#86121=CARTESIAN_POINT('Ctrl Pts',(21.4798625372243,40.8638552870319,0.));
#86122=CARTESIAN_POINT('Ctrl Pts',(21.4798625372243,40.8638552870319,20.));
#86123=CARTESIAN_POINT('Ctrl Pts',(21.5073870534614,40.8460354537749,0.));
#86124=CARTESIAN_POINT('Ctrl Pts',(21.5073870534614,40.8460354537749,20.));
#86125=CARTESIAN_POINT('Ctrl Pts',(21.5348980203391,40.8281967614155,0.));
#86126=CARTESIAN_POINT('Ctrl Pts',(21.5348980203391,40.8281967614155,20.));
#86127=CARTESIAN_POINT('Ctrl Pts',(21.5623954245725,40.8103392196221,0.));
#86128=CARTESIAN_POINT('Ctrl Pts',(21.5623954245725,40.8103392196221,20.));
#86129=CARTESIAN_POINT('Ctrl Pts',(21.5898792528837,40.7924628380726,0.));
#86130=CARTESIAN_POINT('Ctrl Pts',(21.5898792528837,40.7924628380726,20.));
#86131=CARTESIAN_POINT('Ctrl Pts',(21.6173494920019,40.7745676264537,0.));
#86132=CARTESIAN_POINT('Ctrl Pts',(21.6173494920019,40.7745676264537,20.));
#86133=CARTESIAN_POINT('Ctrl Pts',(21.6448061286619,40.7566535944621,0.));
#86134=CARTESIAN_POINT('Ctrl Pts',(21.6448061286619,40.7566535944621,20.));
#86135=CARTESIAN_POINT('Ctrl Pts',(21.6722491496038,40.7387207518043,0.));
#86136=CARTESIAN_POINT('Ctrl Pts',(21.6722491496038,40.7387207518043,20.));
#86137=CARTESIAN_POINT('Ctrl Pts',(21.6996785415723,40.7207691081984,0.));
#86138=CARTESIAN_POINT('Ctrl Pts',(21.6996785415723,40.7207691081984,20.));
#86139=CARTESIAN_POINT('Ctrl Pts',(21.7270942913167,40.7027986733736,0.));
#86140=CARTESIAN_POINT('Ctrl Pts',(21.7270942913167,40.7027986733736,20.));
#86141=CARTESIAN_POINT('Ctrl Pts',(21.7544963855931,40.6848094570694,0.));
#86142=CARTESIAN_POINT('Ctrl Pts',(21.7544963855931,40.6848094570694,20.));
#86143=CARTESIAN_POINT('Ctrl Pts',(21.781884811165,40.6668014690334,0.));
#86144=CARTESIAN_POINT('Ctrl Pts',(21.781884811165,40.6668014690334,20.));
#86145=CARTESIAN_POINT('Ctrl Pts',(21.8092595548052,40.6487747190214,0.));
#86146=CARTESIAN_POINT('Ctrl Pts',(21.8092595548052,40.6487747190214,20.));
#86147=CARTESIAN_POINT('Ctrl Pts',(21.8366206032979,40.6307292167951,0.));
#86148=CARTESIAN_POINT('Ctrl Pts',(21.8366206032979,40.6307292167951,20.));
#86149=CARTESIAN_POINT('Ctrl Pts',(21.8639679434382,40.6126649721233,0.));
#86150=CARTESIAN_POINT('Ctrl Pts',(21.8639679434382,40.6126649721233,20.));
#86151=CARTESIAN_POINT('Ctrl Pts',(21.8913015620281,40.594581994783,0.));
#86152=CARTESIAN_POINT('Ctrl Pts',(21.8913015620281,40.594581994783,20.));
#86153=CARTESIAN_POINT('Ctrl Pts',(21.9186214458728,40.5764802945639,0.));
#86154=CARTESIAN_POINT('Ctrl Pts',(21.9186214458728,40.5764802945639,20.));
#86155=CARTESIAN_POINT('Ctrl Pts',(21.9459275817778,40.5583598812699,0.));
#86156=CARTESIAN_POINT('Ctrl Pts',(21.9459275817778,40.5583598812699,20.));
#86157=CARTESIAN_POINT('Ctrl Pts',(21.9732199565439,40.5402207647219,0.));
#86158=CARTESIAN_POINT('Ctrl Pts',(21.9732199565439,40.5402207647219,20.));
#86159=CARTESIAN_POINT('Ctrl Pts',(22.0004985569689,40.5220629547578,0.));
#86160=CARTESIAN_POINT('Ctrl Pts',(22.0004985569689,40.5220629547578,20.));
#86161=CARTESIAN_POINT('Ctrl Pts',(22.0277633698572,40.5038864612253,0.));
#86162=CARTESIAN_POINT('Ctrl Pts',(22.0277633698572,40.5038864612253,20.));
#86163=CARTESIAN_POINT('Ctrl Pts',(22.0550143820281,40.485691293976,0.));
#86164=CARTESIAN_POINT('Ctrl Pts',(22.0550143820281,40.485691293976,20.));
#86165=CARTESIAN_POINT('Ctrl Pts',(22.0822515803231,40.4674774628609,0.));
#86166=CARTESIAN_POINT('Ctrl Pts',(22.0822515803231,40.4674774628609,20.));
#86167=CARTESIAN_POINT('Ctrl Pts',(22.1094749516164,40.4492449777204,0.));
#86168=CARTESIAN_POINT('Ctrl Pts',(22.1094749516164,40.4492449777204,20.));
#86169=CARTESIAN_POINT('Ctrl Pts',(22.1366844828092,40.4309938483881,0.));
#86170=CARTESIAN_POINT('Ctrl Pts',(22.1366844828092,40.4309938483881,20.));
#86171=CARTESIAN_POINT('Ctrl Pts',(22.1638801608087,40.4127240847076,0.));
#86172=CARTESIAN_POINT('Ctrl Pts',(22.1638801608087,40.4127240847076,20.));
#86173=CARTESIAN_POINT('Ctrl Pts',(22.1910619725087,40.3944356965472,0.));
#86174=CARTESIAN_POINT('Ctrl Pts',(22.1910619725087,40.3944356965472,20.));
#86175=CARTESIAN_POINT('Ctrl Pts',(22.2182299047735,40.3761286938115,0.));
#86176=CARTESIAN_POINT('Ctrl Pts',(22.2182299047735,40.3761286938115,20.));
#86177=CARTESIAN_POINT('Ctrl Pts',(22.2453839444114,40.357803086462,0.));
#86178=CARTESIAN_POINT('Ctrl Pts',(22.2453839444114,40.357803086462,20.));
#86179=CARTESIAN_POINT('Ctrl Pts',(22.2725240781926,40.3394588845042,0.));
#86180=CARTESIAN_POINT('Ctrl Pts',(22.2725240781926,40.3394588845042,20.));
#86181=CARTESIAN_POINT('Ctrl Pts',(22.2996502928986,40.3210960979489,0.));
#86182=CARTESIAN_POINT('Ctrl Pts',(22.2996502928986,40.3210960979489,20.));
#86183=CARTESIAN_POINT('Ctrl Pts',(22.326762575367,40.3027147367804,0.));
#86184=CARTESIAN_POINT('Ctrl Pts',(22.326762575367,40.3027147367804,20.));
#86185=CARTESIAN_POINT('Ctrl Pts',(22.3538609125294,40.2843148109268,0.));
#86186=CARTESIAN_POINT('Ctrl Pts',(22.3538609125294,40.2843148109268,20.));
#86187=CARTESIAN_POINT('Ctrl Pts',(22.3809452914735,40.2658963302133,0.));
#86188=CARTESIAN_POINT('Ctrl Pts',(22.3809452914735,40.2658963302133,20.));
#86189=CARTESIAN_POINT('Ctrl Pts',(22.4080156993888,40.2474593044019,0.));
#86190=CARTESIAN_POINT('Ctrl Pts',(22.4080156993888,40.2474593044019,20.));
#86191=CARTESIAN_POINT('Ctrl Pts',(22.4350721234534,40.229003743277,0.));
#86192=CARTESIAN_POINT('Ctrl Pts',(22.4350721234534,40.229003743277,20.));
#86193=CARTESIAN_POINT('Ctrl Pts',(22.4621145507305,40.210529656724,0.));
#86194=CARTESIAN_POINT('Ctrl Pts',(22.4621145507305,40.210529656724,20.));
#86195=CARTESIAN_POINT('Ctrl Pts',(22.4891429680799,40.1920370547964,0.));
#86196=CARTESIAN_POINT('Ctrl Pts',(22.4891429680799,40.1920370547964,20.));
#86197=CARTESIAN_POINT('Ctrl Pts',(22.5161573620162,40.1735259478254,0.));
#86198=CARTESIAN_POINT('Ctrl Pts',(22.5161573620162,40.1735259478254,20.));
#86199=CARTESIAN_POINT('Ctrl Pts',(22.5431577188605,40.1549963463026,0.));
#86200=CARTESIAN_POINT('Ctrl Pts',(22.5431577188605,40.1549963463026,20.));
#86201=CARTESIAN_POINT('Ctrl Pts',(22.5701440249982,40.1364482606861,0.));
#86202=CARTESIAN_POINT('Ctrl Pts',(22.5701440249982,40.1364482606861,20.));
#86203=CARTESIAN_POINT('Ctrl Pts',(22.5971162671187,40.1178817012184,0.));
#86204=CARTESIAN_POINT('Ctrl Pts',(22.5971162671187,40.1178817012184,20.));
#86205=CARTESIAN_POINT('Ctrl Pts',(22.6240744324258,40.0992966777668,0.));
#86206=CARTESIAN_POINT('Ctrl Pts',(22.6240744324258,40.0992966777668,20.));
#86207=CARTESIAN_POINT('Ctrl Pts',(22.6510185089549,40.0806931995834,0.));
#86208=CARTESIAN_POINT('Ctrl Pts',(22.6510185089549,40.0806931995834,20.));
#86209=CARTESIAN_POINT('Ctrl Pts',(22.6779484851672,40.0620712756149,0.));
#86210=CARTESIAN_POINT('Ctrl Pts',(22.6779484851672,40.0620712756149,20.));
#86211=CARTESIAN_POINT('Ctrl Pts',(22.7048643493645,40.0434309149417,0.));
#86212=CARTESIAN_POINT('Ctrl Pts',(22.7048643493645,40.0434309149417,20.));
#86213=CARTESIAN_POINT('Ctrl Pts',(22.73176608914,40.0247721271957,0.));
#86214=CARTESIAN_POINT('Ctrl Pts',(22.73176608914,40.0247721271957,20.));
#86215=CARTESIAN_POINT('Ctrl Pts',(22.7586536908731,40.0060949229408,0.));
#86216=CARTESIAN_POINT('Ctrl Pts',(22.7586536908731,40.0060949229408,20.));
#86217=CARTESIAN_POINT('Ctrl Pts',(22.7855271390493,39.9873993141881,0.));
#86218=CARTESIAN_POINT('Ctrl Pts',(22.7855271390493,39.9873993141881,20.));
#86219=CARTESIAN_POINT('Ctrl Pts',(22.8123864172494,39.9686853136472,0.));
#86220=CARTESIAN_POINT('Ctrl Pts',(22.8123864172494,39.9686853136472,20.));
#86221=CARTESIAN_POINT('Ctrl Pts',(22.8392315093989,39.9499529337848,0.));
#86222=CARTESIAN_POINT('Ctrl Pts',(22.8392315093989,39.9499529337848,20.));
#86223=CARTESIAN_POINT('Ctrl Pts',(22.8660624009432,39.9312021859375,0.));
#86224=CARTESIAN_POINT('Ctrl Pts',(22.8660624009432,39.9312021859375,20.));
#86225=CARTESIAN_POINT('Ctrl Pts',(22.8928790800154,39.91243307943,0.));
#86226=CARTESIAN_POINT('Ctrl Pts',(22.8928790800154,39.91243307943,20.));
#86227=CARTESIAN_POINT('Ctrl Pts',(22.9196815387084,39.8936456206159,0.));
#86228=CARTESIAN_POINT('Ctrl Pts',(22.9196815387084,39.8936456206159,20.));
#86229=CARTESIAN_POINT('Ctrl Pts',(22.9464697723601,39.8748398133807,0.));
#86230=CARTESIAN_POINT('Ctrl Pts',(22.9464697723601,39.8748398133807,20.));
#86231=CARTESIAN_POINT('Ctrl Pts',(22.9678889774251,39.8597804904793,0.));
#86232=CARTESIAN_POINT('Ctrl Pts',(22.9678889774251,39.8597804904793,20.));
#86233=CARTESIAN_POINT('Ctrl Pts',(22.9839469786125,39.8484777427633,0.));
#86234=CARTESIAN_POINT('Ctrl Pts',(22.9839469786125,39.8484777427633,20.));
#86235=CARTESIAN_POINT('Ctrl Pts',(22.9946494671375,39.8409389084975,0.));
#86236=CARTESIAN_POINT('Ctrl Pts',(22.9946494671375,39.8409389084975,20.));
#86237=CARTESIAN_POINT('Ctrl Pts',(23.,39.8371685740842,0.));
#86238=CARTESIAN_POINT('Ctrl Pts',(23.,39.8371685740842,20.));
#86239=CARTESIAN_POINT('',(-8.50876070567958,48.2555798975982,2.));
#86240=CARTESIAN_POINT('Ctrl Pts',(10.7008281308626,46.0172966012412,2.));
#86241=CARTESIAN_POINT('Ctrl Pts',(9.93785043801569,46.269064380565,2.));
#86242=CARTESIAN_POINT('Ctrl Pts',(9.1675435200454,46.5017519909092,2.));
#86243=CARTESIAN_POINT('Ctrl Pts',(8.39088307367081,46.7150066081184,2.));
#86244=CARTESIAN_POINT('Ctrl Pts',(7.61536231145253,46.9279482920378,2.));
#86245=CARTESIAN_POINT('Ctrl Pts',(6.83350683128281,47.1215139493916,2.));
#86246=CARTESIAN_POINT('Ctrl Pts',(6.04630275161101,47.2954025498593,2.));
#86247=CARTESIAN_POINT('Ctrl Pts',(5.25841985133201,47.4694410976766,2.));
#86248=CARTESIAN_POINT('Ctrl Pts',(4.46517929614118,47.6237686035462,2.));
#86249=CARTESIAN_POINT('Ctrl Pts',(3.66758188329678,47.7581340930642,2.));
#86250=CARTESIAN_POINT('Ctrl Pts',(2.86929216217542,47.8926162107697,2.));
#86251=CARTESIAN_POINT('Ctrl Pts',(2.06663819084915,48.0071016174996,2.));
#86252=CARTESIAN_POINT('Ctrl Pts',(1.26063290971421,48.1013900403506,2.));
#86253=CARTESIAN_POINT('Ctrl Pts',(0.453491097353087,48.1958114173389,2.));
#86254=CARTESIAN_POINT('Ctrl Pts',(-0.357011308083155,48.2699787899167,
2.));
#86255=CARTESIAN_POINT('Ctrl Pts',(-1.16985013658731,48.3237428786942,2.));
#86256=CARTESIAN_POINT('Ctrl Pts',(-1.98327568803649,48.3775457754413,2.));
#86257=CARTESIAN_POINT('Ctrl Pts',(-2.79904086101009,48.4109159159145,2.));
#86258=CARTESIAN_POINT('Ctrl Pts',(-3.61611495486177,48.423755782707,2.));
#86259=CARTESIAN_POINT('Ctrl Pts',(-4.4303187583051,48.4365505444756,2.));
#86260=CARTESIAN_POINT('Ctrl Pts',(-5.24582212860677,48.4289590586956,2.));
#86261=CARTESIAN_POINT('Ctrl Pts',(-6.06160353104804,48.400936241801,2.));
#86262=CARTESIAN_POINT('Ctrl Pts',(-6.59891314705417,48.3824791784996,2.));
#86263=CARTESIAN_POINT('Ctrl Pts',(-7.13634335834826,48.3551598081879,2.));
#86264=CARTESIAN_POINT('Ctrl Pts',(-7.67360240784279,48.3189773727877,2.));
#86265=CARTESIAN_POINT('Ctrl Pts',(-7.95204798714075,48.3002250796529,2.));
#86266=CARTESIAN_POINT('Ctrl Pts',(-8.23044701858261,48.2790922958893,2.));
#86267=CARTESIAN_POINT('Ctrl Pts',(-8.50876070567958,48.2555798975982,2.));
#86268=CARTESIAN_POINT('',(-8.50876070567958,48.2555798975982,0.));
#86269=CARTESIAN_POINT('Origin',(43.358988599418,12.8159317895946,2.));
#86270=CARTESIAN_POINT('',(46.0771487394572,7.40158428109251,2.));
#86271=CARTESIAN_POINT('Ctrl Pts',(46.0771487393297,7.40158428157356,2.));
#86272=CARTESIAN_POINT('Ctrl Pts',(46.0771487393297,7.40158428157356,4.66666666666667));
#86273=CARTESIAN_POINT('Ctrl Pts',(46.0771487393297,7.40158428157356,7.33333333333333));
#86274=CARTESIAN_POINT('Ctrl Pts',(46.0771487393297,7.40158428157356,12.6666666666667));
#86275=CARTESIAN_POINT('Ctrl Pts',(46.0771487393297,7.40158428157356,15.3333333333333));
#86276=CARTESIAN_POINT('Ctrl Pts',(46.0771487393297,7.40158428157356,18.));
#86277=CARTESIAN_POINT('',(46.4996348579608,6.56002729234549,2.));
#86278=CARTESIAN_POINT('',(43.358988599418,12.8159317895946,2.));
#86279=CARTESIAN_POINT('',(46.4996348579608,6.56002729234549,2.));
#86280=CARTESIAN_POINT('Origin',(54.977096951452,18.6485605554598,2.));
#86281=CARTESIAN_POINT('',(45.2025619355918,13.741459297751,2.));
#86282=CARTESIAN_POINT('Ctrl Pts',(45.2025619355918,13.741459297751,18.));
#86283=CARTESIAN_POINT('Ctrl Pts',(45.2025619355918,13.741459297751,15.3333333333333));
#86284=CARTESIAN_POINT('Ctrl Pts',(45.2025619355918,13.741459297751,12.6666666666667));
#86285=CARTESIAN_POINT('Ctrl Pts',(45.2025619355918,13.741459297751,7.33333333333333));
#86286=CARTESIAN_POINT('Ctrl Pts',(45.2025619355918,13.741459297751,4.66666666666667));
#86287=CARTESIAN_POINT('Ctrl Pts',(45.2025619355918,13.741459297751,2.));
#86288=CARTESIAN_POINT('',(54.977096951452,18.6485605554598,2.));
#86289=CARTESIAN_POINT('',(54.977096951452,18.6485605554598,2.));
#86290=CARTESIAN_POINT('',(54.977096951452,18.6485605554598,2.));
#86291=CARTESIAN_POINT('Origin',(58.1177432099948,12.3926560582107,2.));
#86292=CARTESIAN_POINT('',(58.1177432099948,12.3926560582107,2.));
#86293=CARTESIAN_POINT('',(58.1177432099948,12.3926560582107,2.));
#86294=CARTESIAN_POINT('',(58.1177432099948,12.3926560582107,2.));
#86295=CARTESIAN_POINT('Origin',(46.4996348579608,6.56002729234549,2.));
#86296=CARTESIAN_POINT('',(46.4996348579608,6.56002729234549,2.));
#86297=CARTESIAN_POINT('Ctrl Pts',(37.5361777128299,31.4965928746404,0.));
#86298=CARTESIAN_POINT('Ctrl Pts',(37.5361777128299,31.4965928746404,20.));
#86299=CARTESIAN_POINT('Ctrl Pts',(37.5400435810124,31.4910366171629,0.));
#86300=CARTESIAN_POINT('Ctrl Pts',(37.5400435810124,31.4910366171629,20.));
#86301=CARTESIAN_POINT('Ctrl Pts',(37.5477733397938,31.4799228688318,0.));
#86302=CARTESIAN_POINT('Ctrl Pts',(37.5477733397938,31.4799228688318,20.));
#86303=CARTESIAN_POINT('Ctrl Pts',(37.5593620452151,31.4632485462068,0.));
#86304=CARTESIAN_POINT('Ctrl Pts',(37.5593620452151,31.4632485462068,20.));
#86305=CARTESIAN_POINT('Ctrl Pts',(37.574801786924,31.4410087157717,0.));
#86306=CARTESIAN_POINT('Ctrl Pts',(37.574801786924,31.4410087157717,20.));
#86307=CARTESIAN_POINT('Ctrl Pts',(37.5940816876034,31.4131965946731,0.));
#86308=CARTESIAN_POINT('Ctrl Pts',(37.5940816876034,31.4131965946731,20.));
#86309=CARTESIAN_POINT('Ctrl Pts',(37.6133418102375,31.3853721428083,0.));
#86310=CARTESIAN_POINT('Ctrl Pts',(37.6133418102375,31.3853721428083,20.));
#86311=CARTESIAN_POINT('Ctrl Pts',(37.6325821517747,31.3575353648538,0.));
#86312=CARTESIAN_POINT('Ctrl Pts',(37.6325821517747,31.3575353648538,20.));
#86313=CARTESIAN_POINT('Ctrl Pts',(37.6518027072643,31.3296862686536,0.));
#86314=CARTESIAN_POINT('Ctrl Pts',(37.6518027072643,31.3296862686536,20.));
#86315=CARTESIAN_POINT('Ctrl Pts',(37.6710034693473,31.3018248661211,0.));
#86316=CARTESIAN_POINT('Ctrl Pts',(37.6710034693473,31.3018248661211,20.));
#86317=CARTESIAN_POINT('Ctrl Pts',(37.6901844288974,31.2739511721649,0.));
#86318=CARTESIAN_POINT('Ctrl Pts',(37.6901844288974,31.2739511721649,20.));
#86319=CARTESIAN_POINT('Ctrl Pts',(37.7093455757381,31.2460652034827,0.));
#86320=CARTESIAN_POINT('Ctrl Pts',(37.7093455757381,31.2460652034827,20.));
#86321=CARTESIAN_POINT('Ctrl Pts',(37.7284868993471,31.2181669773772,0.));
#86322=CARTESIAN_POINT('Ctrl Pts',(37.7284868993471,31.2181669773772,20.));
#86323=CARTESIAN_POINT('Ctrl Pts',(37.7476083895316,31.1902565106222,0.));
#86324=CARTESIAN_POINT('Ctrl Pts',(37.7476083895316,31.1902565106222,20.));
#86325=CARTESIAN_POINT('Ctrl Pts',(37.7667100372089,31.1623338181506,0.));
#86326=CARTESIAN_POINT('Ctrl Pts',(37.7667100372089,31.1623338181506,20.));
#86327=CARTESIAN_POINT('Ctrl Pts',(37.7857918342009,31.1343989133989,0.));
#86328=CARTESIAN_POINT('Ctrl Pts',(37.7857918342009,31.1343989133989,20.));
#86329=CARTESIAN_POINT('Ctrl Pts',(37.8048537728749,31.1064518089103,0.));
#86330=CARTESIAN_POINT('Ctrl Pts',(37.8048537728749,31.1064518089103,20.));
#86331=CARTESIAN_POINT('Ctrl Pts',(37.8238958458276,31.0784925168637,0.));
#86332=CARTESIAN_POINT('Ctrl Pts',(37.8238958458276,31.0784925168637,20.));
#86333=CARTESIAN_POINT('Ctrl Pts',(37.8429180455734,31.0505210495984,0.));
#86334=CARTESIAN_POINT('Ctrl Pts',(37.8429180455734,31.0505210495984,20.));
#86335=CARTESIAN_POINT('Ctrl Pts',(37.861920364175,31.0225374202321,0.));
#86336=CARTESIAN_POINT('Ctrl Pts',(37.861920364175,31.0225374202321,20.));
#86337=CARTESIAN_POINT('Ctrl Pts',(37.8809027932971,30.9945416425721,0.));
#86338=CARTESIAN_POINT('Ctrl Pts',(37.8809027932971,30.9945416425721,20.));
#86339=CARTESIAN_POINT('Ctrl Pts',(37.8998653243731,30.9665337308352,0.));
#86340=CARTESIAN_POINT('Ctrl Pts',(37.8998653243731,30.9665337308352,20.));
#86341=CARTESIAN_POINT('Ctrl Pts',(37.9188079487378,30.9385136994261,0.));
#86342=CARTESIAN_POINT('Ctrl Pts',(37.9188079487378,30.9385136994261,20.));
#86343=CARTESIAN_POINT('Ctrl Pts',(37.9377306577632,30.9104815627079,0.));
#86344=CARTESIAN_POINT('Ctrl Pts',(37.9377306577632,30.9104815627079,20.));
#86345=CARTESIAN_POINT('Ctrl Pts',(37.9566334430211,30.882437334731,0.));
#86346=CARTESIAN_POINT('Ctrl Pts',(37.9566334430211,30.882437334731,20.));
#86347=CARTESIAN_POINT('Ctrl Pts',(37.9755162962752,30.8543810292446,0.));
#86348=CARTESIAN_POINT('Ctrl Pts',(37.9755162962752,30.8543810292446,20.));
#86349=CARTESIAN_POINT('Ctrl Pts',(37.9943792094053,30.8263126598247,0.));
#86350=CARTESIAN_POINT('Ctrl Pts',(37.9943792094053,30.8263126598247,20.));
#86351=CARTESIAN_POINT('Ctrl Pts',(38.0132221743517,30.7982322399668,0.));
#86352=CARTESIAN_POINT('Ctrl Pts',(38.0132221743517,30.7982322399668,20.));
#86353=CARTESIAN_POINT('Ctrl Pts',(38.0320451830565,30.7701397831859,0.));
#86354=CARTESIAN_POINT('Ctrl Pts',(38.0320451830565,30.7701397831859,20.));
#86355=CARTESIAN_POINT('Ctrl Pts',(38.0508482273931,30.7420353031339,0.));
#86356=CARTESIAN_POINT('Ctrl Pts',(38.0508482273931,30.7420353031339,20.));
#86357=CARTESIAN_POINT('Ctrl Pts',(38.0696312991626,30.7139188136053,0.));
#86358=CARTESIAN_POINT('Ctrl Pts',(38.0696312991626,30.7139188136053,20.));
#86359=CARTESIAN_POINT('Ctrl Pts',(38.088394390128,30.6857903284809,0.));
#86360=CARTESIAN_POINT('Ctrl Pts',(38.088394390128,30.6857903284809,20.));
#86361=CARTESIAN_POINT('Ctrl Pts',(38.1071374920373,30.6576498616875,0.));
#86362=CARTESIAN_POINT('Ctrl Pts',(38.1071374920373,30.6576498616875,20.));
#86363=CARTESIAN_POINT('Ctrl Pts',(38.125860596649,30.6294974271553,0.));
#86364=CARTESIAN_POINT('Ctrl Pts',(38.125860596649,30.6294974271553,20.));
#86365=CARTESIAN_POINT('Ctrl Pts',(38.1445636957629,30.6013330387675,0.));
#86366=CARTESIAN_POINT('Ctrl Pts',(38.1445636957629,30.6013330387675,20.));
#86367=CARTESIAN_POINT('Ctrl Pts',(38.1632467812242,30.5731567103519,0.));
#86368=CARTESIAN_POINT('Ctrl Pts',(38.1632467812242,30.5731567103519,20.));
#86369=CARTESIAN_POINT('Ctrl Pts',(38.1819098449085,30.5449684557073,0.));
#86370=CARTESIAN_POINT('Ctrl Pts',(38.1819098449085,30.5449684557073,20.));
#86371=CARTESIAN_POINT('Ctrl Pts',(38.2005528787125,30.5167682886194,0.));
#86372=CARTESIAN_POINT('Ctrl Pts',(38.2005528787125,30.5167682886194,20.));
#86373=CARTESIAN_POINT('Ctrl Pts',(38.2191758745422,30.4885562228796,0.));
#86374=CARTESIAN_POINT('Ctrl Pts',(38.2191758745422,30.4885562228796,20.));
#86375=CARTESIAN_POINT('Ctrl Pts',(38.2377788243005,30.460332272307,0.));
#86376=CARTESIAN_POINT('Ctrl Pts',(38.2377788243005,30.460332272307,20.));
#86377=CARTESIAN_POINT('Ctrl Pts',(38.2563617198829,30.4320964507535,0.));
#86378=CARTESIAN_POINT('Ctrl Pts',(38.2563617198829,30.4320964507535,20.));
#86379=CARTESIAN_POINT('Ctrl Pts',(38.2749245531853,30.4038487720928,0.));
#86380=CARTESIAN_POINT('Ctrl Pts',(38.2749245531853,30.4038487720928,20.));
#86381=CARTESIAN_POINT('Ctrl Pts',(38.2934673161074,30.3755892502132,0.));
#86382=CARTESIAN_POINT('Ctrl Pts',(38.2934673161074,30.3755892502132,20.));
#86383=CARTESIAN_POINT('Ctrl Pts',(38.3119900005578,30.3473178990095,0.));
#86384=CARTESIAN_POINT('Ctrl Pts',(38.3119900005578,30.3473178990095,20.));
#86385=CARTESIAN_POINT('Ctrl Pts',(38.3304925984593,30.3190347323738,0.));
#86386=CARTESIAN_POINT('Ctrl Pts',(38.3304925984593,30.3190347323738,20.));
#86387=CARTESIAN_POINT('Ctrl Pts',(38.3489751017513,30.2907397641919,0.));
#86388=CARTESIAN_POINT('Ctrl Pts',(38.3489751017513,30.2907397641919,20.));
#86389=CARTESIAN_POINT('Ctrl Pts',(38.3674375023871,30.2624330083488,0.));
#86390=CARTESIAN_POINT('Ctrl Pts',(38.3674375023871,30.2624330083488,20.));
#86391=CARTESIAN_POINT('Ctrl Pts',(38.3858797923318,30.2341144787313,0.));
#86392=CARTESIAN_POINT('Ctrl Pts',(38.3858797923318,30.2341144787313,20.));
#86393=CARTESIAN_POINT('Ctrl Pts',(38.4043019635603,30.2057841892317,0.));
#86394=CARTESIAN_POINT('Ctrl Pts',(38.4043019635603,30.2057841892317,20.));
#86395=CARTESIAN_POINT('Ctrl Pts',(38.4227040080549,30.1774421537519,0.));
#86396=CARTESIAN_POINT('Ctrl Pts',(38.4227040080549,30.1774421537519,20.));
#86397=CARTESIAN_POINT('Ctrl Pts',(38.4410859178038,30.1490883862047,0.));
#86398=CARTESIAN_POINT('Ctrl Pts',(38.4410859178038,30.1490883862047,20.));
#86399=CARTESIAN_POINT('Ctrl Pts',(38.4594476848032,30.1207229005118,0.));
#86400=CARTESIAN_POINT('Ctrl Pts',(38.4594476848032,30.1207229005118,20.));
#86401=CARTESIAN_POINT('Ctrl Pts',(38.4777893010568,30.0923457106027,0.));
#86402=CARTESIAN_POINT('Ctrl Pts',(38.4777893010568,30.0923457106027,20.));
#86403=CARTESIAN_POINT('Ctrl Pts',(38.4961107585777,30.0639568304126,0.));
#86404=CARTESIAN_POINT('Ctrl Pts',(38.4961107585777,30.0639568304126,20.));
#86405=CARTESIAN_POINT('Ctrl Pts',(38.5144120493894,30.0355562738816,0.));
#86406=CARTESIAN_POINT('Ctrl Pts',(38.5144120493894,30.0355562738816,20.));
#86407=CARTESIAN_POINT('Ctrl Pts',(38.532693165526,30.0071440549534,0.));
#86408=CARTESIAN_POINT('Ctrl Pts',(38.532693165526,30.0071440549534,20.));
#86409=CARTESIAN_POINT('Ctrl Pts',(38.5509540990321,29.978720187576,0.));
#86410=CARTESIAN_POINT('Ctrl Pts',(38.5509540990321,29.978720187576,20.));
#86411=CARTESIAN_POINT('Ctrl Pts',(38.5691948419622,29.9502846857025,0.));
#86412=CARTESIAN_POINT('Ctrl Pts',(38.5691948419622,29.9502846857025,20.));
#86413=CARTESIAN_POINT('Ctrl Pts',(38.5874153863803,29.9218375632918,0.));
#86414=CARTESIAN_POINT('Ctrl Pts',(38.5874153863803,29.9218375632918,20.));
#86415=CARTESIAN_POINT('Ctrl Pts',(38.6056157243597,29.8933788343089,0.));
#86416=CARTESIAN_POINT('Ctrl Pts',(38.6056157243597,29.8933788343089,20.));
#86417=CARTESIAN_POINT('Ctrl Pts',(38.6237958479822,29.864908512726,0.));
#86418=CARTESIAN_POINT('Ctrl Pts',(38.6237958479822,29.864908512726,20.));
#86419=CARTESIAN_POINT('Ctrl Pts',(38.6419557493389,29.8364266125215,0.));
#86420=CARTESIAN_POINT('Ctrl Pts',(38.6419557493389,29.8364266125215,20.));
#86421=CARTESIAN_POINT('Ctrl Pts',(38.66009542053,29.8079331476799,0.));
#86422=CARTESIAN_POINT('Ctrl Pts',(38.66009542053,29.8079331476799,20.));
#86423=CARTESIAN_POINT('Ctrl Pts',(38.6782148536649,29.7794281321916,0.));
#86424=CARTESIAN_POINT('Ctrl Pts',(38.6782148536649,29.7794281321916,20.));
#86425=CARTESIAN_POINT('Ctrl Pts',(38.6963140408627,29.7509115800524,0.));
#86426=CARTESIAN_POINT('Ctrl Pts',(38.6963140408627,29.7509115800524,20.));
#86427=CARTESIAN_POINT('Ctrl Pts',(38.7143929742521,29.7223835052637,0.));
#86428=CARTESIAN_POINT('Ctrl Pts',(38.7143929742521,29.7223835052637,20.));
#86429=CARTESIAN_POINT('Ctrl Pts',(38.7324516459718,29.6938439218325,0.));
#86430=CARTESIAN_POINT('Ctrl Pts',(38.7324516459718,29.6938439218325,20.));
#86431=CARTESIAN_POINT('Ctrl Pts',(38.7504900481697,29.6652928437714,0.));
#86432=CARTESIAN_POINT('Ctrl Pts',(38.7504900481697,29.6652928437714,20.));
#86433=CARTESIAN_POINT('Ctrl Pts',(38.7685081730036,29.6367302850988,0.));
#86434=CARTESIAN_POINT('Ctrl Pts',(38.7685081730036,29.6367302850988,20.));
#86435=CARTESIAN_POINT('Ctrl Pts',(38.7865060126402,29.6081562598384,0.));
#86436=CARTESIAN_POINT('Ctrl Pts',(38.7865060126402,29.6081562598384,20.));
#86437=CARTESIAN_POINT('Ctrl Pts',(38.8044835592559,29.5795707820205,0.));
#86438=CARTESIAN_POINT('Ctrl Pts',(38.8044835592559,29.5795707820205,20.));
#86439=CARTESIAN_POINT('Ctrl Pts',(38.8224408050366,29.5509738656807,0.));
#86440=CARTESIAN_POINT('Ctrl Pts',(38.8224408050366,29.5509738656807,20.));
#86441=CARTESIAN_POINT('Ctrl Pts',(38.8403777421773,29.5223655248609,0.));
#86442=CARTESIAN_POINT('Ctrl Pts',(38.8403777421773,29.5223655248609,20.));
#86443=CARTESIAN_POINT('Ctrl Pts',(38.8582943628826,29.4937457736083,0.));
#86444=CARTESIAN_POINT('Ctrl Pts',(38.8582943628826,29.4937457736083,20.));
#86445=CARTESIAN_POINT('Ctrl Pts',(38.8761906593666,29.4651146259764,0.));
#86446=CARTESIAN_POINT('Ctrl Pts',(38.8761906593666,29.4651146259764,20.));
#86447=CARTESIAN_POINT('Ctrl Pts',(38.8940666238532,29.4364720960241,0.));
#86448=CARTESIAN_POINT('Ctrl Pts',(38.8940666238532,29.4364720960241,20.));
#86449=CARTESIAN_POINT('Ctrl Pts',(38.9119222485755,29.4078181978158,0.));
#86450=CARTESIAN_POINT('Ctrl Pts',(38.9119222485755,29.4078181978158,20.));
#86451=CARTESIAN_POINT('Ctrl Pts',(38.9297575257761,29.3791529454216,0.));
#86452=CARTESIAN_POINT('Ctrl Pts',(38.9297575257761,29.3791529454216,20.));
#86453=CARTESIAN_POINT('Ctrl Pts',(38.9475724477072,29.3504763529173,0.));
#86454=CARTESIAN_POINT('Ctrl Pts',(38.9475724477072,29.3504763529173,20.));
#86455=CARTESIAN_POINT('Ctrl Pts',(38.9653670066308,29.3217884343845,0.));
#86456=CARTESIAN_POINT('Ctrl Pts',(38.9653670066308,29.3217884343845,20.));
#86457=CARTESIAN_POINT('Ctrl Pts',(38.9831411948182,29.2930892039104,0.));
#86458=CARTESIAN_POINT('Ctrl Pts',(38.9831411948182,29.2930892039104,20.));
#86459=CARTESIAN_POINT('Ctrl Pts',(39.0008950045502,29.2643786755883,0.));
#86460=CARTESIAN_POINT('Ctrl Pts',(39.0008950045502,29.2643786755883,20.));
#86461=CARTESIAN_POINT('Ctrl Pts',(39.0186284281173,29.2356568635168,0.));
#86462=CARTESIAN_POINT('Ctrl Pts',(39.0186284281173,29.2356568635168,20.));
#86463=CARTESIAN_POINT('Ctrl Pts',(39.0363414578191,29.2069237818005,0.));
#86464=CARTESIAN_POINT('Ctrl Pts',(39.0363414578191,29.2069237818005,20.));
#86465=CARTESIAN_POINT('Ctrl Pts',(39.054034085965,29.1781794445493,0.));
#86466=CARTESIAN_POINT('Ctrl Pts',(39.054034085965,29.1781794445493,20.));
#86467=CARTESIAN_POINT('Ctrl Pts',(39.0717063048737,29.1494238658788,0.));
#86468=CARTESIAN_POINT('Ctrl Pts',(39.0717063048737,29.1494238658788,20.));
#86469=CARTESIAN_POINT('Ctrl Pts',(39.0893581068737,29.1206570599103,0.));
#86470=CARTESIAN_POINT('Ctrl Pts',(39.0893581068737,29.1206570599103,20.));
#86471=CARTESIAN_POINT('Ctrl Pts',(39.106989484303,29.0918790407708,0.));
#86472=CARTESIAN_POINT('Ctrl Pts',(39.106989484303,29.0918790407708,20.));
#86473=CARTESIAN_POINT('Ctrl Pts',(39.1246004295092,29.0630898225929,0.));
#86474=CARTESIAN_POINT('Ctrl Pts',(39.1246004295092,29.0630898225929,20.));
#86475=CARTESIAN_POINT('Ctrl Pts',(39.1421909348497,29.034289419515,0.));
#86476=CARTESIAN_POINT('Ctrl Pts',(39.1421909348497,29.034289419515,20.));
#86477=CARTESIAN_POINT('Ctrl Pts',(39.1597609926911,29.0054778456813,0.));
#86478=CARTESIAN_POINT('Ctrl Pts',(39.1597609926911,29.0054778456813,20.));
#86479=CARTESIAN_POINT('Ctrl Pts',(39.1773105954099,28.9766551152413,0.));
#86480=CARTESIAN_POINT('Ctrl Pts',(39.1773105954099,28.9766551152413,20.));
#86481=CARTESIAN_POINT('Ctrl Pts',(39.1948397353916,28.9478212423503,0.));
#86482=CARTESIAN_POINT('Ctrl Pts',(39.1948397353916,28.9478212423503,20.));
#86483=CARTESIAN_POINT('Ctrl Pts',(39.2123484050317,28.9189762411689,0.));
#86484=CARTESIAN_POINT('Ctrl Pts',(39.2123484050317,28.9189762411689,20.));
#86485=CARTESIAN_POINT('Ctrl Pts',(39.2298365967351,28.8901201258634,0.));
#86486=CARTESIAN_POINT('Ctrl Pts',(39.2298365967351,28.8901201258634,20.));
#86487=CARTESIAN_POINT('Ctrl Pts',(39.2473043029163,28.8612529106058,0.));
#86488=CARTESIAN_POINT('Ctrl Pts',(39.2473043029163,28.8612529106058,20.));
#86489=CARTESIAN_POINT('Ctrl Pts',(39.2647515159997,28.8323746095736,0.));
#86490=CARTESIAN_POINT('Ctrl Pts',(39.2647515159997,28.8323746095736,20.));
#86491=CARTESIAN_POINT('Ctrl Pts',(39.2821782284193,28.80348523695,0.));
#86492=CARTESIAN_POINT('Ctrl Pts',(39.2821782284193,28.80348523695,20.));
#86493=CARTESIAN_POINT('Ctrl Pts',(39.2995844326181,28.7745848069238,0.));
#86494=CARTESIAN_POINT('Ctrl Pts',(39.2995844326181,28.7745848069238,20.));
#86495=CARTESIAN_POINT('Ctrl Pts',(39.316970121049,28.7456733336894,0.));
#86496=CARTESIAN_POINT('Ctrl Pts',(39.316970121049,28.7456733336894,20.));
#86497=CARTESIAN_POINT('Ctrl Pts',(39.3343352861746,28.7167508314468,0.));
#86498=CARTESIAN_POINT('Ctrl Pts',(39.3343352861746,28.7167508314468,20.));
#86499=CARTESIAN_POINT('Ctrl Pts',(39.3516799204672,28.6878173144015,0.));
#86500=CARTESIAN_POINT('Ctrl Pts',(39.3516799204672,28.6878173144015,20.));
#86501=CARTESIAN_POINT('Ctrl Pts',(39.3690040164086,28.6588727967647,0.));
#86502=CARTESIAN_POINT('Ctrl Pts',(39.3690040164086,28.6588727967647,20.));
#86503=CARTESIAN_POINT('Ctrl Pts',(39.3863075664906,28.6299172927529,0.));
#86504=CARTESIAN_POINT('Ctrl Pts',(39.3863075664906,28.6299172927529,20.));
#86505=CARTESIAN_POINT('Ctrl Pts',(39.4035905632141,28.600950816588,0.));
#86506=CARTESIAN_POINT('Ctrl Pts',(39.4035905632141,28.600950816588,20.));
#86507=CARTESIAN_POINT('Ctrl Pts',(39.4208529990894,28.5719733824975,0.));
#86508=CARTESIAN_POINT('Ctrl Pts',(39.4208529990894,28.5719733824975,20.));
#86509=CARTESIAN_POINT('Ctrl Pts',(39.4380948666368,28.5429850047148,0.));
#86510=CARTESIAN_POINT('Ctrl Pts',(39.4380948666368,28.5429850047148,20.));
#86511=CARTESIAN_POINT('Ctrl Pts',(39.4553161583861,28.5139856974786,0.));
#86512=CARTESIAN_POINT('Ctrl Pts',(39.4553161583861,28.5139856974786,20.));
#86513=CARTESIAN_POINT('Ctrl Pts',(39.472516866877,28.4849754750331,0.));
#86514=CARTESIAN_POINT('Ctrl Pts',(39.472516866877,28.4849754750331,20.));
#86515=CARTESIAN_POINT('Ctrl Pts',(39.4896969846589,28.455954351628,0.));
#86516=CARTESIAN_POINT('Ctrl Pts',(39.4896969846589,28.455954351628,20.));
#86517=CARTESIAN_POINT('Ctrl Pts',(39.5068565042907,28.4269223415187,0.));
#86518=CARTESIAN_POINT('Ctrl Pts',(39.5068565042907,28.4269223415187,20.));
#86519=CARTESIAN_POINT('Ctrl Pts',(39.5239954183412,28.3978794589661,0.));
#86520=CARTESIAN_POINT('Ctrl Pts',(39.5239954183412,28.3978794589661,20.));
#86521=CARTESIAN_POINT('Ctrl Pts',(39.5411137193887,28.3688257182364,0.));
#86522=CARTESIAN_POINT('Ctrl Pts',(39.5411137193887,28.3688257182364,20.));
#86523=CARTESIAN_POINT('Ctrl Pts',(39.5582114000212,28.3397611336014,0.));
#86524=CARTESIAN_POINT('Ctrl Pts',(39.5582114000212,28.3397611336014,20.));
#86525=CARTESIAN_POINT('Ctrl Pts',(39.5752884528361,28.3106857193381,0.));
#86526=CARTESIAN_POINT('Ctrl Pts',(39.5752884528361,28.3106857193381,20.));
#86527=CARTESIAN_POINT('Ctrl Pts',(39.5923448704403,28.2815994897291,0.));
#86528=CARTESIAN_POINT('Ctrl Pts',(39.5923448704403,28.2815994897291,20.));
#86529=CARTESIAN_POINT('Ctrl Pts',(39.6093806454502,28.2525024590626,0.));
#86530=CARTESIAN_POINT('Ctrl Pts',(39.6093806454502,28.2525024590626,20.));
#86531=CARTESIAN_POINT('Ctrl Pts',(39.6263957704923,28.2233946416323,0.));
#86532=CARTESIAN_POINT('Ctrl Pts',(39.6263957704923,28.2233946416323,20.));
#86533=CARTESIAN_POINT('Ctrl Pts',(39.6433902382029,28.1942760517371,0.));
#86534=CARTESIAN_POINT('Ctrl Pts',(39.6433902382029,28.1942760517371,20.));
#86535=CARTESIAN_POINT('Ctrl Pts',(39.6603640412281,28.1651467036817,0.));
#86536=CARTESIAN_POINT('Ctrl Pts',(39.6603640412281,28.1651467036817,20.));
#86537=CARTESIAN_POINT('Ctrl Pts',(39.6773171722241,28.136006611776,0.));
#86538=CARTESIAN_POINT('Ctrl Pts',(39.6773171722241,28.136006611776,20.));
#86539=CARTESIAN_POINT('Ctrl Pts',(39.6942496238565,28.1068557903356,0.));
#86540=CARTESIAN_POINT('Ctrl Pts',(39.6942496238565,28.1068557903356,20.));
#86541=CARTESIAN_POINT('Ctrl Pts',(39.7111613888006,28.0776942536814,0.));
#86542=CARTESIAN_POINT('Ctrl Pts',(39.7111613888006,28.0776942536814,20.));
#86543=CARTESIAN_POINT('Ctrl Pts',(39.728052459741,28.0485220161395,0.));
#86544=CARTESIAN_POINT('Ctrl Pts',(39.728052459741,28.0485220161395,20.));
#86545=CARTESIAN_POINT('Ctrl Pts',(39.7449228293718,28.0193390920415,0.));
#86546=CARTESIAN_POINT('Ctrl Pts',(39.7449228293718,28.0193390920415,20.));
#86547=CARTESIAN_POINT('Ctrl Pts',(39.7617724903968,27.9901454957246,0.));
#86548=CARTESIAN_POINT('Ctrl Pts',(39.7617724903968,27.9901454957246,20.));
#86549=CARTESIAN_POINT('Ctrl Pts',(39.7786014355293,27.960941241531,0.));
#86550=CARTESIAN_POINT('Ctrl Pts',(39.7786014355293,27.960941241531,20.));
#86551=CARTESIAN_POINT('Ctrl Pts',(39.795409657493,27.9317263438086,0.));
#86552=CARTESIAN_POINT('Ctrl Pts',(39.795409657493,27.9317263438086,20.));
#86553=CARTESIAN_POINT('Ctrl Pts',(39.8121971490214,27.9025008169107,0.));
#86554=CARTESIAN_POINT('Ctrl Pts',(39.8121971490214,27.9025008169107,20.));
#86555=CARTESIAN_POINT('Ctrl Pts',(39.828963902858,27.8732646751959,0.));
#86556=CARTESIAN_POINT('Ctrl Pts',(39.828963902858,27.8732646751959,20.));
#86557=CARTESIAN_POINT('Ctrl Pts',(39.8457099117559,27.8440179330284,0.));
#86558=CARTESIAN_POINT('Ctrl Pts',(39.8457099117559,27.8440179330284,20.));
#86559=CARTESIAN_POINT('Ctrl Pts',(39.862435168478,27.8147606047778,0.));
#86560=CARTESIAN_POINT('Ctrl Pts',(39.862435168478,27.8147606047778,20.));
#86561=CARTESIAN_POINT('Ctrl Pts',(39.8791396657966,27.785492704819,0.));
#86562=CARTESIAN_POINT('Ctrl Pts',(39.8791396657966,27.785492704819,20.));
#86563=CARTESIAN_POINT('Ctrl Pts',(39.8958233964934,27.7562142475319,0.));
#86564=CARTESIAN_POINT('Ctrl Pts',(39.8958233964934,27.7562142475319,20.));
#86565=CARTESIAN_POINT('Ctrl Pts',(39.9124863533599,27.726925247302,0.));
#86566=CARTESIAN_POINT('Ctrl Pts',(39.9124863533599,27.726925247302,20.));
#86567=CARTESIAN_POINT('Ctrl Pts',(39.9291285291975,27.6976257185198,0.));
#86568=CARTESIAN_POINT('Ctrl Pts',(39.9291285291975,27.6976257185198,20.));
#86569=CARTESIAN_POINT('Ctrl Pts',(39.9457499168175,27.6683156755815,0.));
#86570=CARTESIAN_POINT('Ctrl Pts',(39.9457499168175,27.6683156755815,20.));
#86571=CARTESIAN_POINT('Ctrl Pts',(39.9623505090412,27.6389951328887,0.));
#86572=CARTESIAN_POINT('Ctrl Pts',(39.9623505090412,27.6389951328887,20.));
#86573=CARTESIAN_POINT('Ctrl Pts',(39.9789302986995,27.6096641048483,0.));
#86574=CARTESIAN_POINT('Ctrl Pts',(39.9789302986995,27.6096641048483,20.));
#86575=CARTESIAN_POINT('Ctrl Pts',(39.9954892786331,27.5803226058725,0.));
#86576=CARTESIAN_POINT('Ctrl Pts',(39.9954892786331,27.5803226058725,20.));
#86577=CARTESIAN_POINT('Ctrl Pts',(40.0120274416924,27.5509706503786,0.));
#86578=CARTESIAN_POINT('Ctrl Pts',(40.0120274416924,27.5509706503786,20.));
#86579=CARTESIAN_POINT('Ctrl Pts',(40.0285447807378,27.5216082527897,0.));
#86580=CARTESIAN_POINT('Ctrl Pts',(40.0285447807378,27.5216082527897,20.));
#86581=CARTESIAN_POINT('Ctrl Pts',(40.045041288639,27.4922354275335,0.));
#86582=CARTESIAN_POINT('Ctrl Pts',(40.045041288639,27.4922354275335,20.));
#86583=CARTESIAN_POINT('Ctrl Pts',(40.0615169582759,27.4628521890436,0.));
#86584=CARTESIAN_POINT('Ctrl Pts',(40.0615169582759,27.4628521890436,20.));
#86585=CARTESIAN_POINT('Ctrl Pts',(40.077971782538,27.4334585517582,0.));
#86586=CARTESIAN_POINT('Ctrl Pts',(40.077971782538,27.4334585517582,20.));
#86587=CARTESIAN_POINT('Ctrl Pts',(40.0944057543248,27.4040545301216,0.));
#86588=CARTESIAN_POINT('Ctrl Pts',(40.0944057543248,27.4040545301216,20.));
#86589=CARTESIAN_POINT('Ctrl Pts',(40.1108188665452,27.374640138583,0.));
#86590=CARTESIAN_POINT('Ctrl Pts',(40.1108188665452,27.374640138583,20.));
#86591=CARTESIAN_POINT('Ctrl Pts',(40.1272111121183,27.3452153915969,0.));
#86592=CARTESIAN_POINT('Ctrl Pts',(40.1272111121183,27.3452153915969,20.));
#86593=CARTESIAN_POINT('Ctrl Pts',(40.1435824839731,27.3157803036231,0.));
#86594=CARTESIAN_POINT('Ctrl Pts',(40.1435824839731,27.3157803036231,20.));
#86595=CARTESIAN_POINT('Ctrl Pts',(40.1599329750483,27.2863348891265,0.));
#86596=CARTESIAN_POINT('Ctrl Pts',(40.1599329750483,27.2863348891265,20.));
#86597=CARTESIAN_POINT('Ctrl Pts',(40.1762625782924,27.2568791625774,0.));
#86598=CARTESIAN_POINT('Ctrl Pts',(40.1762625782924,27.2568791625774,20.));
#86599=CARTESIAN_POINT('Ctrl Pts',(40.1925712866631,27.2274131384508,0.));
#86600=CARTESIAN_POINT('Ctrl Pts',(40.1925712866631,27.2274131384508,20.));
#86601=CARTESIAN_POINT('Ctrl Pts',(40.2088590931287,27.1979368312277,0.));
#86602=CARTESIAN_POINT('Ctrl Pts',(40.2088590931287,27.1979368312277,20.));
#86603=CARTESIAN_POINT('Ctrl Pts',(40.2251259906669,27.1684502553939,0.));
#86604=CARTESIAN_POINT('Ctrl Pts',(40.2251259906669,27.1684502553939,20.));
#86605=CARTESIAN_POINT('Ctrl Pts',(40.2413719722657,27.1389534254409,0.));
#86606=CARTESIAN_POINT('Ctrl Pts',(40.2413719722657,27.1389534254409,20.));
#86607=CARTESIAN_POINT('Ctrl Pts',(40.2575970309226,27.1094463558649,0.));
#86608=CARTESIAN_POINT('Ctrl Pts',(40.2575970309226,27.1094463558649,20.));
#86609=CARTESIAN_POINT('Ctrl Pts',(40.2738011596454,27.0799290611676,0.));
#86610=CARTESIAN_POINT('Ctrl Pts',(40.2738011596454,27.0799290611676,20.));
#86611=CARTESIAN_POINT('Ctrl Pts',(40.2899843514517,27.0504015558557,0.));
#86612=CARTESIAN_POINT('Ctrl Pts',(40.2899843514517,27.0504015558557,20.));
#86613=CARTESIAN_POINT('Ctrl Pts',(40.3061465993685,27.0208638544413,0.));
#86614=CARTESIAN_POINT('Ctrl Pts',(40.3061465993685,27.0208638544413,20.));
#86615=CARTESIAN_POINT('Ctrl Pts',(40.3222878964329,26.9913159714415,0.));
#86616=CARTESIAN_POINT('Ctrl Pts',(40.3222878964329,26.9913159714415,20.));
#86617=CARTESIAN_POINT('Ctrl Pts',(40.3384082356913,26.9617579213786,0.));
#86618=CARTESIAN_POINT('Ctrl Pts',(40.3384082356913,26.9617579213786,20.));
#86619=CARTESIAN_POINT('Ctrl Pts',(40.3545076102003,26.9321897187802,0.));
#86620=CARTESIAN_POINT('Ctrl Pts',(40.3545076102003,26.9321897187802,20.));
#86621=CARTESIAN_POINT('Ctrl Pts',(40.3705860130263,26.9026113781788,0.));
#86622=CARTESIAN_POINT('Ctrl Pts',(40.3705860130263,26.9026113781788,20.));
#86623=CARTESIAN_POINT('Ctrl Pts',(40.386643437246,26.8730229141124,0.));
#86624=CARTESIAN_POINT('Ctrl Pts',(40.386643437246,26.8730229141124,20.));
#86625=CARTESIAN_POINT('Ctrl Pts',(40.4026798759458,26.8434243411241,0.));
#86626=CARTESIAN_POINT('Ctrl Pts',(40.4026798759458,26.8434243411241,20.));
#86627=CARTESIAN_POINT('Ctrl Pts',(40.4186953222224,26.8138156737619,0.));
#86628=CARTESIAN_POINT('Ctrl Pts',(40.4186953222224,26.8138156737619,20.));
#86629=CARTESIAN_POINT('Ctrl Pts',(40.4346897691821,26.7841969265794,0.));
#86630=CARTESIAN_POINT('Ctrl Pts',(40.4346897691821,26.7841969265794,20.));
#86631=CARTESIAN_POINT('Ctrl Pts',(40.4506632099408,26.754568114135,0.));
#86632=CARTESIAN_POINT('Ctrl Pts',(40.4506632099408,26.754568114135,20.));
#86633=CARTESIAN_POINT('Ctrl Pts',(40.4666156376241,26.7249292509923,0.));
#86634=CARTESIAN_POINT('Ctrl Pts',(40.4666156376241,26.7249292509923,20.));
#86635=CARTESIAN_POINT('Ctrl Pts',(40.4825470453679,26.6952803517197,0.));
#86636=CARTESIAN_POINT('Ctrl Pts',(40.4825470453679,26.6952803517197,20.));
#86637=CARTESIAN_POINT('Ctrl Pts',(40.4984574263178,26.6656214308914,0.));
#86638=CARTESIAN_POINT('Ctrl Pts',(40.4984574263178,26.6656214308914,20.));
#86639=CARTESIAN_POINT('Ctrl Pts',(40.5143467736295,26.6359525030862,0.));
#86640=CARTESIAN_POINT('Ctrl Pts',(40.5143467736295,26.6359525030862,20.));
#86641=CARTESIAN_POINT('Ctrl Pts',(40.5302150804687,26.606273582888,0.));
#86642=CARTESIAN_POINT('Ctrl Pts',(40.5302150804687,26.606273582888,20.));
#86643=CARTESIAN_POINT('Ctrl Pts',(40.546062340011,26.5765846848862,0.));
#86644=CARTESIAN_POINT('Ctrl Pts',(40.546062340011,26.5765846848862,20.));
#86645=CARTESIAN_POINT('Ctrl Pts',(40.5618885454414,26.5468858236748,0.));
#86646=CARTESIAN_POINT('Ctrl Pts',(40.5618885454414,26.5468858236748,20.));
#86647=CARTESIAN_POINT('Ctrl Pts',(40.5776936899555,26.5171770138532,0.));
#86648=CARTESIAN_POINT('Ctrl Pts',(40.5776936899555,26.5171770138532,20.));
#86649=CARTESIAN_POINT('Ctrl Pts',(40.5934777667583,26.4874582700259,0.));
#86650=CARTESIAN_POINT('Ctrl Pts',(40.5934777667583,26.4874582700259,20.));
#86651=CARTESIAN_POINT('Ctrl Pts',(40.6092407690651,26.4577296068023,0.));
#86652=CARTESIAN_POINT('Ctrl Pts',(40.6092407690651,26.4577296068023,20.));
#86653=CARTESIAN_POINT('Ctrl Pts',(40.6249826901011,26.4279910387971,0.));
#86654=CARTESIAN_POINT('Ctrl Pts',(40.6249826901011,26.4279910387971,20.));
#86655=CARTESIAN_POINT('Ctrl Pts',(40.6407035231015,26.3982425806297,0.));
#86656=CARTESIAN_POINT('Ctrl Pts',(40.6407035231015,26.3982425806297,20.));
#86657=CARTESIAN_POINT('Ctrl Pts',(40.6564032613109,26.3684842469248,0.));
#86658=CARTESIAN_POINT('Ctrl Pts',(40.6564032613109,26.3684842469248,20.));
#86659=CARTESIAN_POINT('Ctrl Pts',(40.6720818979844,26.338716052312,0.));
#86660=CARTESIAN_POINT('Ctrl Pts',(40.6720818979844,26.338716052312,20.));
#86661=CARTESIAN_POINT('Ctrl Pts',(40.6877394263869,26.308938011426,0.));
#86662=CARTESIAN_POINT('Ctrl Pts',(40.6877394263869,26.308938011426,20.));
#86663=CARTESIAN_POINT('Ctrl Pts',(40.7033758397932,26.2791501389067,0.));
#86664=CARTESIAN_POINT('Ctrl Pts',(40.7033758397932,26.2791501389067,20.));
#86665=CARTESIAN_POINT('Ctrl Pts',(40.7189911314882,26.2493524493989,0.));
#86666=CARTESIAN_POINT('Ctrl Pts',(40.7189911314882,26.2493524493989,20.));
#86667=CARTESIAN_POINT('Ctrl Pts',(40.7345852947663,26.2195449575524,0.));
#86668=CARTESIAN_POINT('Ctrl Pts',(40.7345852947663,26.2195449575524,20.));
#86669=CARTESIAN_POINT('Ctrl Pts',(40.7501583229328,26.1897276780219,0.));
#86670=CARTESIAN_POINT('Ctrl Pts',(40.7501583229328,26.1897276780219,20.));
#86671=CARTESIAN_POINT('Ctrl Pts',(40.7657102093021,26.1599006254674,0.));
#86672=CARTESIAN_POINT('Ctrl Pts',(40.7657102093021,26.1599006254674,20.));
#86673=CARTESIAN_POINT('Ctrl Pts',(40.7812409471992,26.1300638145535,0.));
#86674=CARTESIAN_POINT('Ctrl Pts',(40.7812409471992,26.1300638145535,20.));
#86675=CARTESIAN_POINT('Ctrl Pts',(40.7967505299588,26.1002172599501,0.));
#86676=CARTESIAN_POINT('Ctrl Pts',(40.7967505299588,26.1002172599501,20.));
#86677=CARTESIAN_POINT('Ctrl Pts',(40.8122389509256,26.0703609763318,0.));
#86678=CARTESIAN_POINT('Ctrl Pts',(40.8122389509256,26.0703609763318,20.));
#86679=CARTESIAN_POINT('Ctrl Pts',(40.8277062034539,26.0404949783787,0.));
#86680=CARTESIAN_POINT('Ctrl Pts',(40.8277062034539,26.0404949783787,20.));
#86681=CARTESIAN_POINT('Ctrl Pts',(40.843152280908,26.0106192807756,0.));
#86682=CARTESIAN_POINT('Ctrl Pts',(40.843152280908,26.0106192807756,20.));
#86683=CARTESIAN_POINT('Ctrl Pts',(40.8585771766627,25.9807338982121,0.));
#86684=CARTESIAN_POINT('Ctrl Pts',(40.8585771766627,25.9807338982121,20.));
#86685=CARTESIAN_POINT('Ctrl Pts',(40.8739808841024,25.9508388453831,0.));
#86686=CARTESIAN_POINT('Ctrl Pts',(40.8739808841024,25.9508388453831,20.));
#86687=CARTESIAN_POINT('Ctrl Pts',(40.8893633966224,25.9209341369879,0.));
#86688=CARTESIAN_POINT('Ctrl Pts',(40.8893633966224,25.9209341369879,20.));
#86689=CARTESIAN_POINT('Ctrl Pts',(40.9047247076274,25.891019787731,0.));
#86690=CARTESIAN_POINT('Ctrl Pts',(40.9047247076274,25.891019787731,20.));
#86691=CARTESIAN_POINT('Ctrl Pts',(40.9200648105322,25.861095812322,0.));
#86692=CARTESIAN_POINT('Ctrl Pts',(40.9200648105322,25.861095812322,20.));
#86693=CARTESIAN_POINT('Ctrl Pts',(40.9353836987613,25.8311622254754,0.));
#86694=CARTESIAN_POINT('Ctrl Pts',(40.9353836987613,25.8311622254754,20.));
#86695=CARTESIAN_POINT('Ctrl Pts',(40.9506813657491,25.8012190419102,0.));
#86696=CARTESIAN_POINT('Ctrl Pts',(40.9506813657491,25.8012190419102,20.));
#86697=CARTESIAN_POINT('Ctrl Pts',(40.9659578049399,25.7712662763511,0.));
#86698=CARTESIAN_POINT('Ctrl Pts',(40.9659578049399,25.7712662763511,20.));
#86699=CARTESIAN_POINT('Ctrl Pts',(40.981213009789,25.7413039435271,0.));
#86700=CARTESIAN_POINT('Ctrl Pts',(40.981213009789,25.7413039435271,20.));
#86701=CARTESIAN_POINT('Ctrl Pts',(40.9964469737612,25.7113320581728,0.));
#86702=CARTESIAN_POINT('Ctrl Pts',(40.9964469737612,25.7113320581728,20.));
#86703=CARTESIAN_POINT('Ctrl Pts',(41.0116596903316,25.6813506350271,0.));
#86704=CARTESIAN_POINT('Ctrl Pts',(41.0116596903316,25.6813506350271,20.));
#86705=CARTESIAN_POINT('Ctrl Pts',(41.0268511529852,25.6513596888338,0.));
#86706=CARTESIAN_POINT('Ctrl Pts',(41.0268511529852,25.6513596888338,20.));
#86707=CARTESIAN_POINT('Ctrl Pts',(41.0420213552163,25.6213592343415,0.));
#86708=CARTESIAN_POINT('Ctrl Pts',(41.0420213552163,25.6213592343415,20.));
#86709=CARTESIAN_POINT('Ctrl Pts',(41.05717029053,25.5913492863038,0.));
#86710=CARTESIAN_POINT('Ctrl Pts',(41.05717029053,25.5913492863038,20.));
#86711=CARTESIAN_POINT('Ctrl Pts',(41.072297952441,25.5613298594791,0.));
#86712=CARTESIAN_POINT('Ctrl Pts',(41.072297952441,25.5613298594791,20.));
#86713=CARTESIAN_POINT('Ctrl Pts',(41.0874043344745,25.5313009686309,0.));
#86714=CARTESIAN_POINT('Ctrl Pts',(41.0874043344745,25.5313009686309,20.));
#86715=CARTESIAN_POINT('Ctrl Pts',(41.1024894301655,25.5012626285275,0.));
#86716=CARTESIAN_POINT('Ctrl Pts',(41.1024894301655,25.5012626285275,20.));
#86717=CARTESIAN_POINT('Ctrl Pts',(41.1175532330596,25.4712148539422,0.));
#86718=CARTESIAN_POINT('Ctrl Pts',(41.1175532330596,25.4712148539422,20.));
#86719=CARTESIAN_POINT('Ctrl Pts',(41.1325957367119,25.4411576596529,0.));
#86720=CARTESIAN_POINT('Ctrl Pts',(41.1325957367119,25.4411576596529,20.));
#86721=CARTESIAN_POINT('Ctrl Pts',(41.1476169346881,25.4110910604425,0.));
#86722=CARTESIAN_POINT('Ctrl Pts',(41.1476169346881,25.4110910604425,20.));
#86723=CARTESIAN_POINT('Ctrl Pts',(41.1626168205634,25.3810150710984,0.));
#86724=CARTESIAN_POINT('Ctrl Pts',(41.1626168205634,25.3810150710984,20.));
#86725=CARTESIAN_POINT('Ctrl Pts',(41.1775953879232,25.3509297064131,0.));
#86726=CARTESIAN_POINT('Ctrl Pts',(41.1775953879232,25.3509297064131,20.));
#86727=CARTESIAN_POINT('Ctrl Pts',(41.1925526303629,25.3208349811839,0.));
#86728=CARTESIAN_POINT('Ctrl Pts',(41.1925526303629,25.3208349811839,20.));
#86729=CARTESIAN_POINT('Ctrl Pts',(41.2074885414881,25.2907309102128,0.));
#86730=CARTESIAN_POINT('Ctrl Pts',(41.2074885414881,25.2907309102128,20.));
#86731=CARTESIAN_POINT('Ctrl Pts',(41.2224031149147,25.2606175083067,0.));
#86732=CARTESIAN_POINT('Ctrl Pts',(41.2224031149147,25.2606175083067,20.));
#86733=CARTESIAN_POINT('Ctrl Pts',(41.2372963442684,25.2304947902774,0.));
#86734=CARTESIAN_POINT('Ctrl Pts',(41.2372963442684,25.2304947902774,20.));
#86735=CARTESIAN_POINT('Ctrl Pts',(41.2521682231854,25.2003627709414,0.));
#86736=CARTESIAN_POINT('Ctrl Pts',(41.2521682231854,25.2003627709414,20.));
#86737=CARTESIAN_POINT('Ctrl Pts',(41.2670187453114,25.1702214651198,0.));
#86738=CARTESIAN_POINT('Ctrl Pts',(41.2670187453114,25.1702214651198,20.));
#86739=CARTESIAN_POINT('Ctrl Pts',(41.2818479043026,25.1400708876386,0.));
#86740=CARTESIAN_POINT('Ctrl Pts',(41.2818479043026,25.1400708876386,20.));
#86741=CARTESIAN_POINT('Ctrl Pts',(41.2966556938255,25.1099110533288,0.));
#86742=CARTESIAN_POINT('Ctrl Pts',(41.2966556938255,25.1099110533288,20.));
#86743=CARTESIAN_POINT('Ctrl Pts',(41.3114421075567,25.0797419770258,0.));
#86744=CARTESIAN_POINT('Ctrl Pts',(41.3114421075567,25.0797419770258,20.));
#86745=CARTESIAN_POINT('Ctrl Pts',(41.3262071391823,25.0495636735701,0.));
#86746=CARTESIAN_POINT('Ctrl Pts',(41.3262071391823,25.0495636735701,20.));
#86747=CARTESIAN_POINT('Ctrl Pts',(41.3409507823989,25.0193761578067,0.));
#86748=CARTESIAN_POINT('Ctrl Pts',(41.3409507823989,25.0193761578067,20.));
#86749=CARTESIAN_POINT('Ctrl Pts',(41.3556730309131,24.9891794445855,0.));
#86750=CARTESIAN_POINT('Ctrl Pts',(41.3556730309131,24.9891794445855,20.));
#86751=CARTESIAN_POINT('Ctrl Pts',(41.3703738784418,24.9589735487609,0.));
#86752=CARTESIAN_POINT('Ctrl Pts',(41.3703738784418,24.9589735487609,20.));
#86753=CARTESIAN_POINT('Ctrl Pts',(41.3850533187123,24.9287584851923,0.));
#86754=CARTESIAN_POINT('Ctrl Pts',(41.3850533187123,24.9287584851923,20.));
#86755=CARTESIAN_POINT('Ctrl Pts',(41.3997113454618,24.8985342687436,0.));
#86756=CARTESIAN_POINT('Ctrl Pts',(41.3997113454618,24.8985342687436,20.));
#86757=CARTESIAN_POINT('Ctrl Pts',(41.4143479524375,24.8683009142837,0.));
#86758=CARTESIAN_POINT('Ctrl Pts',(41.4143479524375,24.8683009142837,20.));
#86759=CARTESIAN_POINT('Ctrl Pts',(41.4289631333969,24.8380584366859,0.));
#86760=CARTESIAN_POINT('Ctrl Pts',(41.4289631333969,24.8380584366859,20.));
#86761=CARTESIAN_POINT('Ctrl Pts',(41.443556882107,24.8078068508284,0.));
#86762=CARTESIAN_POINT('Ctrl Pts',(41.443556882107,24.8078068508284,20.));
#86763=CARTESIAN_POINT('Ctrl Pts',(41.4581291923457,24.7775461715943,0.));
#86764=CARTESIAN_POINT('Ctrl Pts',(41.4581291923457,24.7775461715943,20.));
#86765=CARTESIAN_POINT('Ctrl Pts',(41.4726800579006,24.7472764138709,0.));
#86766=CARTESIAN_POINT('Ctrl Pts',(41.4726800579006,24.7472764138709,20.));
#86767=CARTESIAN_POINT('Ctrl Pts',(41.4872094725701,24.7169975925505,0.));
#86768=CARTESIAN_POINT('Ctrl Pts',(41.4872094725701,24.7169975925505,20.));
#86769=CARTESIAN_POINT('Ctrl Pts',(41.5017174301628,24.68670972253,0.));
#86770=CARTESIAN_POINT('Ctrl Pts',(41.5017174301628,24.68670972253,20.));
#86771=CARTESIAN_POINT('Ctrl Pts',(41.516203924497,24.6564128187107,0.));
#86772=CARTESIAN_POINT('Ctrl Pts',(41.516203924497,24.6564128187107,20.));
#86773=CARTESIAN_POINT('Ctrl Pts',(41.5306689494012,24.626106895999,0.));
#86774=CARTESIAN_POINT('Ctrl Pts',(41.5306689494012,24.626106895999,20.));
#86775=CARTESIAN_POINT('Ctrl Pts',(41.545112498714,24.5957919693057,0.));
#86776=CARTESIAN_POINT('Ctrl Pts',(41.545112498714,24.5957919693057,20.));
#86777=CARTESIAN_POINT('Ctrl Pts',(41.5595345662842,24.5654680535465,0.));
#86778=CARTESIAN_POINT('Ctrl Pts',(41.5595345662842,24.5654680535465,20.));
#86779=CARTESIAN_POINT('Ctrl Pts',(41.5739351459709,24.5351351636416,0.));
#86780=CARTESIAN_POINT('Ctrl Pts',(41.5739351459709,24.5351351636416,20.));
#86781=CARTESIAN_POINT('Ctrl Pts',(41.5883142316433,24.5047933145158,0.));
#86782=CARTESIAN_POINT('Ctrl Pts',(41.5883142316433,24.5047933145158,20.));
#86783=CARTESIAN_POINT('Ctrl Pts',(41.6026718171809,24.4744425210985,0.));
#86784=CARTESIAN_POINT('Ctrl Pts',(41.6026718171809,24.4744425210985,20.));
#86785=CARTESIAN_POINT('Ctrl Pts',(41.6170078964732,24.4440827983238,0.));
#86786=CARTESIAN_POINT('Ctrl Pts',(41.6170078964732,24.4440827983238,20.));
#86787=CARTESIAN_POINT('Ctrl Pts',(41.6313224634201,24.4137141611302,0.));
#86788=CARTESIAN_POINT('Ctrl Pts',(41.6313224634201,24.4137141611302,20.));
#86789=CARTESIAN_POINT('Ctrl Pts',(41.6456155119319,24.3833366244611,0.));
#86790=CARTESIAN_POINT('Ctrl Pts',(41.6456155119319,24.3833366244611,20.));
#86791=CARTESIAN_POINT('Ctrl Pts',(41.6598870359289,24.3529502032644,0.));
#86792=CARTESIAN_POINT('Ctrl Pts',(41.6598870359289,24.3529502032644,20.));
#86793=CARTESIAN_POINT('Ctrl Pts',(41.6741370293416,24.3225549124927,0.));
#86794=CARTESIAN_POINT('Ctrl Pts',(41.6741370293416,24.3225549124927,20.));
#86795=CARTESIAN_POINT('Ctrl Pts',(41.6883654861106,24.292150767103,0.));
#86796=CARTESIAN_POINT('Ctrl Pts',(41.6883654861106,24.292150767103,20.));
#86797=CARTESIAN_POINT('Ctrl Pts',(41.7025724001866,24.2617377820568,0.));
#86798=CARTESIAN_POINT('Ctrl Pts',(41.7025724001866,24.2617377820568,20.));
#86799=CARTESIAN_POINT('Ctrl Pts',(41.7167577655309,24.2313159723205,0.));
#86800=CARTESIAN_POINT('Ctrl Pts',(41.7167577655309,24.2313159723205,20.));
#86801=CARTESIAN_POINT('Ctrl Pts',(41.7309215761147,24.2008853528648,0.));
#86802=CARTESIAN_POINT('Ctrl Pts',(41.7309215761147,24.2008853528648,20.));
#86803=CARTESIAN_POINT('Ctrl Pts',(41.7450638259196,24.1704459386651,0.));
#86804=CARTESIAN_POINT('Ctrl Pts',(41.7450638259196,24.1704459386651,20.));
#86805=CARTESIAN_POINT('Ctrl Pts',(41.7591845089374,24.1399977447013,0.));
#86806=CARTESIAN_POINT('Ctrl Pts',(41.7591845089374,24.1399977447013,20.));
#86807=CARTESIAN_POINT('Ctrl Pts',(41.7732836191701,24.1095407859578,0.));
#86808=CARTESIAN_POINT('Ctrl Pts',(41.7732836191701,24.1095407859578,20.));
#86809=CARTESIAN_POINT('Ctrl Pts',(41.78736115063,24.0790750774236,0.));
#86810=CARTESIAN_POINT('Ctrl Pts',(41.78736115063,24.0790750774236,20.));
#86811=CARTESIAN_POINT('Ctrl Pts',(41.8014170973399,24.0486006340924,0.));
#86812=CARTESIAN_POINT('Ctrl Pts',(41.8014170973399,24.0486006340924,20.));
#86813=CARTESIAN_POINT('Ctrl Pts',(41.8154514533324,24.0181174709622,0.));
#86814=CARTESIAN_POINT('Ctrl Pts',(41.8154514533324,24.0181174709622,20.));
#86815=CARTESIAN_POINT('Ctrl Pts',(41.8294642126506,23.9876256030355,0.));
#86816=CARTESIAN_POINT('Ctrl Pts',(41.8294642126506,23.9876256030355,20.));
#86817=CARTESIAN_POINT('Ctrl Pts',(41.8434553693478,23.9571250453194,0.));
#86818=CARTESIAN_POINT('Ctrl Pts',(41.8434553693478,23.9571250453194,20.));
#86819=CARTESIAN_POINT('Ctrl Pts',(41.8574249174873,23.9266158128252,0.));
#86820=CARTESIAN_POINT('Ctrl Pts',(41.8574249174873,23.9266158128252,20.));
#86821=CARTESIAN_POINT('Ctrl Pts',(41.8713728511429,23.8960979205694,0.));
#86822=CARTESIAN_POINT('Ctrl Pts',(41.8713728511429,23.8960979205694,20.));
#86823=CARTESIAN_POINT('Ctrl Pts',(41.8852991643986,23.8655713835725,0.));
#86824=CARTESIAN_POINT('Ctrl Pts',(41.8852991643986,23.8655713835725,20.));
#86825=CARTESIAN_POINT('Ctrl Pts',(41.8992038513488,23.8350362168598,0.));
#86826=CARTESIAN_POINT('Ctrl Pts',(41.8992038513488,23.8350362168598,20.));
#86827=CARTESIAN_POINT('Ctrl Pts',(41.9130869060982,23.8044924354607,0.));
#86828=CARTESIAN_POINT('Ctrl Pts',(41.9130869060982,23.8044924354607,20.));
#86829=CARTESIAN_POINT('Ctrl Pts',(41.9269483227618,23.7739400544092,0.));
#86830=CARTESIAN_POINT('Ctrl Pts',(41.9269483227618,23.7739400544092,20.));
#86831=CARTESIAN_POINT('Ctrl Pts',(41.9407880954647,23.7433790887435,0.));
#86832=CARTESIAN_POINT('Ctrl Pts',(41.9407880954647,23.7433790887435,20.));
#86833=CARTESIAN_POINT('Ctrl Pts',(41.9546062183422,23.7128095535066,0.));
#86834=CARTESIAN_POINT('Ctrl Pts',(41.9546062183422,23.7128095535066,20.));
#86835=CARTESIAN_POINT('Ctrl Pts',(41.9684026855399,23.6822314637457,0.));
#86836=CARTESIAN_POINT('Ctrl Pts',(41.9684026855399,23.6822314637457,20.));
#86837=CARTESIAN_POINT('Ctrl Pts',(41.9821774912141,23.651644834513,0.));
#86838=CARTESIAN_POINT('Ctrl Pts',(41.9821774912141,23.651644834513,20.));
#86839=CARTESIAN_POINT('Ctrl Pts',(41.9959306295311,23.6210496808648,0.));
#86840=CARTESIAN_POINT('Ctrl Pts',(41.9959306295311,23.6210496808648,20.));
#86841=CARTESIAN_POINT('Ctrl Pts',(42.0096620946675,23.5904460178619,0.));
#86842=CARTESIAN_POINT('Ctrl Pts',(42.0096620946675,23.5904460178619,20.));
#86843=CARTESIAN_POINT('Ctrl Pts',(42.02337188081,23.5598338605694,0.));
#86844=CARTESIAN_POINT('Ctrl Pts',(42.02337188081,23.5598338605694,20.));
#86845=CARTESIAN_POINT('Ctrl Pts',(42.0370599821558,23.5292132240567,0.));
#86846=CARTESIAN_POINT('Ctrl Pts',(42.0370599821558,23.5292132240567,20.));
#86847=CARTESIAN_POINT('Ctrl Pts',(42.0507263929126,23.4985841233977,0.));
#86848=CARTESIAN_POINT('Ctrl Pts',(42.0507263929126,23.4985841233977,20.));
#86849=CARTESIAN_POINT('Ctrl Pts',(42.0643711072981,23.4679465736707,0.));
#86850=CARTESIAN_POINT('Ctrl Pts',(42.0643711072981,23.4679465736707,20.));
#86851=CARTESIAN_POINT('Ctrl Pts',(42.0779941195407,23.4373005899585,0.));
#86852=CARTESIAN_POINT('Ctrl Pts',(42.0779941195407,23.4373005899585,20.));
#86853=CARTESIAN_POINT('Ctrl Pts',(42.0915954238788,23.4066461873484,0.));
#86854=CARTESIAN_POINT('Ctrl Pts',(42.0915954238788,23.4066461873484,20.));
#86855=CARTESIAN_POINT('Ctrl Pts',(42.1051750145614,23.3759833809318,0.));
#86856=CARTESIAN_POINT('Ctrl Pts',(42.1051750145614,23.3759833809318,20.));
#86857=CARTESIAN_POINT('Ctrl Pts',(42.1187328858474,23.3453121858047,0.));
#86858=CARTESIAN_POINT('Ctrl Pts',(42.1187328858474,23.3453121858047,20.));
#86859=CARTESIAN_POINT('Ctrl Pts',(42.1322690320059,23.3146326170671,0.));
#86860=CARTESIAN_POINT('Ctrl Pts',(42.1322690320059,23.3146326170671,20.));
#86861=CARTESIAN_POINT('Ctrl Pts',(42.1457834473169,23.2839446898238,0.));
#86862=CARTESIAN_POINT('Ctrl Pts',(42.1457834473169,23.2839446898238,20.));
#86863=CARTESIAN_POINT('Ctrl Pts',(42.1592761260708,23.2532484191837,0.));
#86864=CARTESIAN_POINT('Ctrl Pts',(42.1592761260708,23.2532484191837,20.));
#86865=CARTESIAN_POINT('Ctrl Pts',(42.1727470625681,23.2225438202604,0.));
#86866=CARTESIAN_POINT('Ctrl Pts',(42.1727470625681,23.2225438202604,20.));
#86867=CARTESIAN_POINT('Ctrl Pts',(42.1861962511195,23.1918309081713,0.));
#86868=CARTESIAN_POINT('Ctrl Pts',(42.1861962511195,23.1918309081713,20.));
#86869=CARTESIAN_POINT('Ctrl Pts',(42.1996236860461,23.1611096980384,0.));
#86870=CARTESIAN_POINT('Ctrl Pts',(42.1996236860461,23.1611096980384,20.));
#86871=CARTESIAN_POINT('Ctrl Pts',(42.2130293616794,23.1303802049881,0.));
#86872=CARTESIAN_POINT('Ctrl Pts',(42.2130293616794,23.1303802049881,20.));
#86873=CARTESIAN_POINT('Ctrl Pts',(42.2264132723611,23.0996424441509,0.));
#86874=CARTESIAN_POINT('Ctrl Pts',(42.2264132723611,23.0996424441509,20.));
#86875=CARTESIAN_POINT('Ctrl Pts',(42.2397754124437,23.0688964306618,0.));
#86876=CARTESIAN_POINT('Ctrl Pts',(42.2397754124437,23.0688964306618,20.));
#86877=CARTESIAN_POINT('Ctrl Pts',(42.2531157762897,23.0381421796601,0.));
#86878=CARTESIAN_POINT('Ctrl Pts',(42.2531157762897,23.0381421796601,20.));
#86879=CARTESIAN_POINT('Ctrl Pts',(42.2664343582719,23.0073797062893,0.));
#86880=CARTESIAN_POINT('Ctrl Pts',(42.2664343582719,23.0073797062893,20.));
#86881=CARTESIAN_POINT('Ctrl Pts',(42.2797311527738,22.9766090256973,0.));
#86882=CARTESIAN_POINT('Ctrl Pts',(42.2797311527738,22.9766090256973,20.));
#86883=CARTESIAN_POINT('Ctrl Pts',(42.2930061541893,22.9458301530364,0.));
#86884=CARTESIAN_POINT('Ctrl Pts',(42.2930061541893,22.9458301530364,20.));
#86885=CARTESIAN_POINT('Ctrl Pts',(42.3062593569225,22.9150431034629,0.));
#86886=CARTESIAN_POINT('Ctrl Pts',(42.3062593569225,22.9150431034629,20.));
#86887=CARTESIAN_POINT('Ctrl Pts',(42.3194907553882,22.8842478921374,0.));
#86888=CARTESIAN_POINT('Ctrl Pts',(42.3194907553882,22.8842478921374,20.));
#86889=CARTESIAN_POINT('Ctrl Pts',(42.3327003440108,22.8534445342249,0.));
#86890=CARTESIAN_POINT('Ctrl Pts',(42.3327003440108,22.8534445342249,20.));
#86891=CARTESIAN_POINT('Ctrl Pts',(42.3458881172255,22.8226330448945,0.));
#86892=CARTESIAN_POINT('Ctrl Pts',(42.3458881172255,22.8226330448945,20.));
#86893=CARTESIAN_POINT('Ctrl Pts',(42.3590540694774,22.7918134393197,0.));
#86894=CARTESIAN_POINT('Ctrl Pts',(42.3590540694774,22.7918134393197,20.));
#86895=CARTESIAN_POINT('Ctrl Pts',(42.3721981952224,22.7609857326781,0.));
#86896=CARTESIAN_POINT('Ctrl Pts',(42.3721981952224,22.7609857326781,20.));
#86897=CARTESIAN_POINT('Ctrl Pts',(42.3853204889273,22.7301499401517,0.));
#86898=CARTESIAN_POINT('Ctrl Pts',(42.3853204889273,22.7301499401517,20.));
#86899=CARTESIAN_POINT('Ctrl Pts',(42.398420945069,22.6993060769268,0.));
#86900=CARTESIAN_POINT('Ctrl Pts',(42.398420945069,22.6993060769268,20.));
#86901=CARTESIAN_POINT('Ctrl Pts',(42.411499558135,22.6684541581936,0.));
#86902=CARTESIAN_POINT('Ctrl Pts',(42.411499558135,22.6684541581936,20.));
#86903=CARTESIAN_POINT('Ctrl Pts',(42.4245563226236,22.6375941991468,0.));
#86904=CARTESIAN_POINT('Ctrl Pts',(42.4245563226236,22.6375941991468,20.));
#86905=CARTESIAN_POINT('Ctrl Pts',(42.4375912330427,22.6067262149851,0.));
#86906=CARTESIAN_POINT('Ctrl Pts',(42.4375912330427,22.6067262149851,20.));
#86907=CARTESIAN_POINT('Ctrl Pts',(42.4506042839107,22.5758502209116,0.));
#86908=CARTESIAN_POINT('Ctrl Pts',(42.4506042839107,22.5758502209116,20.));
#86909=CARTESIAN_POINT('Ctrl Pts',(42.4635954697559,22.5449662321334,0.));
#86910=CARTESIAN_POINT('Ctrl Pts',(42.4635954697559,22.5449662321334,20.));
#86911=CARTESIAN_POINT('Ctrl Pts',(42.4765647851171,22.5140742638619,0.));
#86912=CARTESIAN_POINT('Ctrl Pts',(42.4765647851171,22.5140742638619,20.));
#86913=CARTESIAN_POINT('Ctrl Pts',(42.4895122245441,22.4831743313126,0.));
#86914=CARTESIAN_POINT('Ctrl Pts',(42.4895122245441,22.4831743313126,20.));
#86915=CARTESIAN_POINT('Ctrl Pts',(42.502437782597,22.4522664497054,0.));
#86916=CARTESIAN_POINT('Ctrl Pts',(42.502437782597,22.4522664497054,20.));
#86917=CARTESIAN_POINT('Ctrl Pts',(42.5153414538467,22.4213506342639,0.));
#86918=CARTESIAN_POINT('Ctrl Pts',(42.5153414538467,22.4213506342639,20.));
#86919=CARTESIAN_POINT('Ctrl Pts',(42.5282232328747,22.3904269002165,0.));
#86920=CARTESIAN_POINT('Ctrl Pts',(42.5282232328747,22.3904269002165,20.));
#86921=CARTESIAN_POINT('Ctrl Pts',(42.5410831142726,22.3594952627952,0.));
#86922=CARTESIAN_POINT('Ctrl Pts',(42.5410831142726,22.3594952627952,20.));
#86923=CARTESIAN_POINT('Ctrl Pts',(42.5539210926424,22.3285557372364,0.));
#86924=CARTESIAN_POINT('Ctrl Pts',(42.5539210926424,22.3285557372364,20.));
#86925=CARTESIAN_POINT('Ctrl Pts',(42.5667371625962,22.2976083387805,0.));
#86926=CARTESIAN_POINT('Ctrl Pts',(42.5667371625962,22.2976083387805,20.));
#86927=CARTESIAN_POINT('Ctrl Pts',(42.5795313187569,22.2666530826722,0.));
#86928=CARTESIAN_POINT('Ctrl Pts',(42.5795313187569,22.2666530826722,20.));
#86929=CARTESIAN_POINT('Ctrl Pts',(42.5923035557573,22.2356899841602,0.));
#86930=CARTESIAN_POINT('Ctrl Pts',(42.5923035557573,22.2356899841602,20.));
#86931=CARTESIAN_POINT('Ctrl Pts',(42.6050538682411,22.2047190584974,0.));
#86932=CARTESIAN_POINT('Ctrl Pts',(42.6050538682411,22.2047190584974,20.));
#86933=CARTESIAN_POINT('Ctrl Pts',(42.6177822508627,22.1737403209406,0.));
#86934=CARTESIAN_POINT('Ctrl Pts',(42.6177822508627,22.1737403209406,20.));
#86935=CARTESIAN_POINT('Ctrl Pts',(42.6304886982869,22.1427537867512,0.));
#86936=CARTESIAN_POINT('Ctrl Pts',(42.6304886982869,22.1427537867512,20.));
#86937=CARTESIAN_POINT('Ctrl Pts',(42.6431732051887,22.1117594711942,0.));
#86938=CARTESIAN_POINT('Ctrl Pts',(42.6431732051887,22.1117594711942,20.));
#86939=CARTESIAN_POINT('Ctrl Pts',(42.6558357662536,22.0807573895388,0.));
#86940=CARTESIAN_POINT('Ctrl Pts',(42.6558357662536,22.0807573895388,20.));
#86941=CARTESIAN_POINT('Ctrl Pts',(42.6684763761777,22.0497475570584,0.));
#86942=CARTESIAN_POINT('Ctrl Pts',(42.6684763761777,22.0497475570584,20.));
#86943=CARTESIAN_POINT('Ctrl Pts',(42.6810950296678,22.0187299890302,0.));
#86944=CARTESIAN_POINT('Ctrl Pts',(42.6810950296678,22.0187299890302,20.));
#86945=CARTESIAN_POINT('Ctrl Pts',(42.6936917214411,21.9877047007357,0.));
#86946=CARTESIAN_POINT('Ctrl Pts',(42.6936917214411,21.9877047007357,20.));
#86947=CARTESIAN_POINT('Ctrl Pts',(42.7062664462249,21.9566717074606,0.));
#86948=CARTESIAN_POINT('Ctrl Pts',(42.7062664462249,21.9566717074606,20.));
#86949=CARTESIAN_POINT('Ctrl Pts',(42.7188191987573,21.9256310244944,0.));
#86950=CARTESIAN_POINT('Ctrl Pts',(42.7188191987573,21.9256310244944,20.));
#86951=CARTESIAN_POINT('Ctrl Pts',(42.7313499737866,21.8945826671308,0.));
#86952=CARTESIAN_POINT('Ctrl Pts',(42.7313499737866,21.8945826671308,20.));
#86953=CARTESIAN_POINT('Ctrl Pts',(42.7438587660714,21.8635266506674,0.));
#86954=CARTESIAN_POINT('Ctrl Pts',(42.7438587660714,21.8635266506674,20.));
#86955=CARTESIAN_POINT('Ctrl Pts',(42.7563455703812,21.832462990406,0.));
#86956=CARTESIAN_POINT('Ctrl Pts',(42.7563455703812,21.832462990406,20.));
#86957=CARTESIAN_POINT('Ctrl Pts',(42.7688103814962,21.8013917016521,0.));
#86958=CARTESIAN_POINT('Ctrl Pts',(42.7688103814962,21.8013917016521,20.));
#86959=CARTESIAN_POINT('Ctrl Pts',(42.7812531942069,21.7703127997157,0.));
#86960=CARTESIAN_POINT('Ctrl Pts',(42.7812531942069,21.7703127997157,20.));
#86961=CARTESIAN_POINT('Ctrl Pts',(42.7936740033148,21.7392262999104,0.));
#86962=CARTESIAN_POINT('Ctrl Pts',(42.7936740033148,21.7392262999104,20.));
#86963=CARTESIAN_POINT('Ctrl Pts',(42.8060728036313,21.7081322175539,0.));
#86964=CARTESIAN_POINT('Ctrl Pts',(42.8060728036313,21.7081322175539,20.));
#86965=CARTESIAN_POINT('Ctrl Pts',(42.8184495899785,21.677030567968,0.));
#86966=CARTESIAN_POINT('Ctrl Pts',(42.8184495899785,21.677030567968,20.));
#86967=CARTESIAN_POINT('Ctrl Pts',(42.8308043571886,21.6459213664784,0.));
#86968=CARTESIAN_POINT('Ctrl Pts',(42.8308043571886,21.6459213664784,20.));
#86969=CARTESIAN_POINT('Ctrl Pts',(42.8431371001047,21.6148046284149,0.));
#86970=CARTESIAN_POINT('Ctrl Pts',(42.8431371001047,21.6148046284149,20.));
#86971=CARTESIAN_POINT('Ctrl Pts',(42.8554478135801,21.5836803691112,0.));
#86972=CARTESIAN_POINT('Ctrl Pts',(42.8554478135801,21.5836803691112,20.));
#86973=CARTESIAN_POINT('Ctrl Pts',(42.8677364924793,21.5525486039049,0.));
#86974=CARTESIAN_POINT('Ctrl Pts',(42.8677364924793,21.5525486039049,20.));
#86975=CARTESIAN_POINT('Ctrl Pts',(42.8800031316769,21.5214093481377,0.));
#86976=CARTESIAN_POINT('Ctrl Pts',(42.8800031316769,21.5214093481377,20.));
#86977=CARTESIAN_POINT('Ctrl Pts',(42.8922477260581,21.490262617155,0.));
#86978=CARTESIAN_POINT('Ctrl Pts',(42.8922477260581,21.490262617155,20.));
#86979=CARTESIAN_POINT('Ctrl Pts',(42.9044702705183,21.4591084263065,0.));
#86980=CARTESIAN_POINT('Ctrl Pts',(42.9044702705183,21.4591084263065,20.));
#86981=CARTESIAN_POINT('Ctrl Pts',(42.916670759964,21.4279467909454,0.));
#86982=CARTESIAN_POINT('Ctrl Pts',(42.916670759964,21.4279467909454,20.));
#86983=CARTESIAN_POINT('Ctrl Pts',(42.9288491893122,21.3967777264295,0.));
#86984=CARTESIAN_POINT('Ctrl Pts',(42.9288491893122,21.3967777264295,20.));
#86985=CARTESIAN_POINT('Ctrl Pts',(42.9410055534907,21.3656012481199,0.));
#86986=CARTESIAN_POINT('Ctrl Pts',(42.9410055534907,21.3656012481199,20.));
#86987=CARTESIAN_POINT('Ctrl Pts',(42.9531398474371,21.3344173713818,0.));
#86988=CARTESIAN_POINT('Ctrl Pts',(42.9531398474371,21.3344173713818,20.));
#86989=CARTESIAN_POINT('Ctrl Pts',(42.9652520660998,21.3032261115844,0.));
#86990=CARTESIAN_POINT('Ctrl Pts',(42.9652520660998,21.3032261115844,20.));
#86991=CARTESIAN_POINT('Ctrl Pts',(42.9773422044374,21.2720274841006,0.));
#86992=CARTESIAN_POINT('Ctrl Pts',(42.9773422044374,21.2720274841006,20.));
#86993=CARTESIAN_POINT('Ctrl Pts',(42.9894102574195,21.2408215043074,0.));
#86994=CARTESIAN_POINT('Ctrl Pts',(42.9894102574195,21.2408215043074,20.));
#86995=CARTESIAN_POINT('Ctrl Pts',(43.0014562200264,21.2096081875857,0.));
#86996=CARTESIAN_POINT('Ctrl Pts',(43.0014562200264,21.2096081875857,20.));
#86997=CARTESIAN_POINT('Ctrl Pts',(43.0134800872489,21.1783875493205,0.));
#86998=CARTESIAN_POINT('Ctrl Pts',(43.0134800872489,21.1783875493205,20.));
#86999=CARTESIAN_POINT('Ctrl Pts',(43.0254818540885,21.1471596049,0.));
#87000=CARTESIAN_POINT('Ctrl Pts',(43.0254818540885,21.1471596049,20.));
#87001=CARTESIAN_POINT('Ctrl Pts',(43.037461515557,21.1159243697169,0.));
#87002=CARTESIAN_POINT('Ctrl Pts',(43.037461515557,21.1159243697169,20.));
#87003=CARTESIAN_POINT('Ctrl Pts',(43.049419066677,21.0846818591673,0.));
#87004=CARTESIAN_POINT('Ctrl Pts',(43.049419066677,21.0846818591673,20.));
#87005=CARTESIAN_POINT('Ctrl Pts',(43.0613545024815,21.0534320886512,0.));
#87006=CARTESIAN_POINT('Ctrl Pts',(43.0613545024815,21.0534320886512,20.));
#87007=CARTESIAN_POINT('Ctrl Pts',(43.0732678180139,21.0221750735727,0.));
#87008=CARTESIAN_POINT('Ctrl Pts',(43.0732678180139,21.0221750735727,20.));
#87009=CARTESIAN_POINT('Ctrl Pts',(43.0851590083283,20.9909108293397,0.));
#87010=CARTESIAN_POINT('Ctrl Pts',(43.0851590083283,20.9909108293397,20.));
#87011=CARTESIAN_POINT('Ctrl Pts',(43.0970280684896,20.959639371364,0.));
#87012=CARTESIAN_POINT('Ctrl Pts',(43.0970280684896,20.959639371364,20.));
#87013=CARTESIAN_POINT('Ctrl Pts',(43.1088749935734,20.9283607150615,0.));
#87014=CARTESIAN_POINT('Ctrl Pts',(43.1088749935734,20.9283607150615,20.));
#87015=CARTESIAN_POINT('Ctrl Pts',(43.1206997786656,20.8970748758512,0.));
#87016=CARTESIAN_POINT('Ctrl Pts',(43.1206997786656,20.8970748758512,20.));
#87017=CARTESIAN_POINT('Ctrl Pts',(43.132502418863,20.8657818691565,0.));
#87018=CARTESIAN_POINT('Ctrl Pts',(43.132502418863,20.8657818691565,20.));
#87019=CARTESIAN_POINT('Ctrl Pts',(43.1442829092724,20.8344817104039,0.));
#87020=CARTESIAN_POINT('Ctrl Pts',(43.1442829092724,20.8344817104039,20.));
#87021=CARTESIAN_POINT('Ctrl Pts',(43.1560412450117,20.8031744150242,0.));
#87022=CARTESIAN_POINT('Ctrl Pts',(43.1560412450117,20.8031744150242,20.));
#87023=CARTESIAN_POINT('Ctrl Pts',(43.1677774212093,20.7718599984519,0.));
#87024=CARTESIAN_POINT('Ctrl Pts',(43.1677774212093,20.7718599984519,20.));
#87025=CARTESIAN_POINT('Ctrl Pts',(43.1794914330045,20.7405384761252,0.));
#87026=CARTESIAN_POINT('Ctrl Pts',(43.1794914330045,20.7405384761252,20.));
#87027=CARTESIAN_POINT('Ctrl Pts',(43.1911832755467,20.7092098634864,0.));
#87028=CARTESIAN_POINT('Ctrl Pts',(43.1911832755467,20.7092098634864,20.));
#87029=CARTESIAN_POINT('Ctrl Pts',(43.202852943996,20.6778741759814,0.));
#87030=CARTESIAN_POINT('Ctrl Pts',(43.202852943996,20.6778741759814,20.));
#87031=CARTESIAN_POINT('Ctrl Pts',(43.2145004335236,20.6465314290598,0.));
#87032=CARTESIAN_POINT('Ctrl Pts',(43.2145004335236,20.6465314290598,20.));
#87033=CARTESIAN_POINT('Ctrl Pts',(43.2261257393109,20.615181638175,0.));
#87034=CARTESIAN_POINT('Ctrl Pts',(43.2261257393109,20.615181638175,20.));
#87035=CARTESIAN_POINT('Ctrl Pts',(43.2377288565503,20.5838248187841,0.));
#87036=CARTESIAN_POINT('Ctrl Pts',(43.2377288565503,20.5838248187841,20.));
#87037=CARTESIAN_POINT('Ctrl Pts',(43.2493097804445,20.5524609863481,0.));
#87038=CARTESIAN_POINT('Ctrl Pts',(43.2493097804445,20.5524609863481,20.));
#87039=CARTESIAN_POINT('Ctrl Pts',(43.2608685062069,20.5210901563314,0.));
#87040=CARTESIAN_POINT('Ctrl Pts',(43.2608685062069,20.5210901563314,20.));
#87041=CARTESIAN_POINT('Ctrl Pts',(43.2724050290617,20.4897123442023,0.));
#87042=CARTESIAN_POINT('Ctrl Pts',(43.2724050290617,20.4897123442023,20.));
#87043=CARTESIAN_POINT('Ctrl Pts',(43.283919344243,20.4583275654327,0.));
#87044=CARTESIAN_POINT('Ctrl Pts',(43.283919344243,20.4583275654327,20.));
#87045=CARTESIAN_POINT('Ctrl Pts',(43.2954114469964,20.4269358354984,0.));
#87046=CARTESIAN_POINT('Ctrl Pts',(43.2954114469964,20.4269358354984,20.));
#87047=CARTESIAN_POINT('Ctrl Pts',(43.3068813325774,20.3955371698787,0.));
#87048=CARTESIAN_POINT('Ctrl Pts',(43.3068813325774,20.3955371698787,20.));
#87049=CARTESIAN_POINT('Ctrl Pts',(43.3183289962528,20.3641315840566,0.));
#87050=CARTESIAN_POINT('Ctrl Pts',(43.3183289962528,20.3641315840566,20.));
#87051=CARTESIAN_POINT('Ctrl Pts',(43.3297544333003,20.3327190935193,0.));
#87052=CARTESIAN_POINT('Ctrl Pts',(43.3297544333003,20.3327190935193,20.));
#87053=CARTESIAN_POINT('Ctrl Pts',(43.3411576390085,20.3012997137575,0.));
#87054=CARTESIAN_POINT('Ctrl Pts',(43.3411576390085,20.3012997137575,20.));
#87055=CARTESIAN_POINT('Ctrl Pts',(43.3525386086763,20.2698734602656,0.));
#87056=CARTESIAN_POINT('Ctrl Pts',(43.3525386086763,20.2698734602656,20.));
#87057=CARTESIAN_POINT('Ctrl Pts',(43.3638973376125,20.2384403485411,0.));
#87058=CARTESIAN_POINT('Ctrl Pts',(43.3638973376125,20.2384403485411,20.));
#87059=CARTESIAN_POINT('Ctrl Pts',(43.3752338211368,20.2070003940853,0.));
#87060=CARTESIAN_POINT('Ctrl Pts',(43.3752338211368,20.2070003940853,20.));
#87061=CARTESIAN_POINT('Ctrl Pts',(43.3865480545792,20.1755536124033,0.));
#87062=CARTESIAN_POINT('Ctrl Pts',(43.3865480545792,20.1755536124033,20.));
#87063=CARTESIAN_POINT('Ctrl Pts',(43.3978400332808,20.1441000190037,0.));
#87064=CARTESIAN_POINT('Ctrl Pts',(43.3978400332808,20.1441000190037,20.));
#87065=CARTESIAN_POINT('Ctrl Pts',(43.409109752594,20.1126396293992,0.));
#87066=CARTESIAN_POINT('Ctrl Pts',(43.409109752594,20.1126396293992,20.));
#87067=CARTESIAN_POINT('Ctrl Pts',(43.4203572078819,20.0811724591059,0.));
#87068=CARTESIAN_POINT('Ctrl Pts',(43.4203572078819,20.0811724591059,20.));
#87069=CARTESIAN_POINT('Ctrl Pts',(43.4315823945181,20.0496985236436,0.));
#87070=CARTESIAN_POINT('Ctrl Pts',(43.4315823945181,20.0496985236436,20.));
#87071=CARTESIAN_POINT('Ctrl Pts',(43.4427853078868,20.0182178385356,0.));
#87072=CARTESIAN_POINT('Ctrl Pts',(43.4427853078868,20.0182178385356,20.));
#87073=CARTESIAN_POINT('Ctrl Pts',(43.4539659433821,19.9867304193089,0.));
#87074=CARTESIAN_POINT('Ctrl Pts',(43.4539659433821,19.9867304193089,20.));
#87075=CARTESIAN_POINT('Ctrl Pts',(43.4651242964088,19.9552362814936,0.));
#87076=CARTESIAN_POINT('Ctrl Pts',(43.4651242964088,19.9552362814936,20.));
#87077=CARTESIAN_POINT('Ctrl Pts',(43.4762603623832,19.923735440624,0.));
#87078=CARTESIAN_POINT('Ctrl Pts',(43.4762603623832,19.923735440624,20.));
#87079=CARTESIAN_POINT('Ctrl Pts',(43.4873741367321,19.8922279122378,0.));
#87080=CARTESIAN_POINT('Ctrl Pts',(43.4873741367321,19.8922279122378,20.));
#87081=CARTESIAN_POINT('Ctrl Pts',(43.4984656148935,19.8607137118763,0.));
#87082=CARTESIAN_POINT('Ctrl Pts',(43.4984656148935,19.8607137118763,20.));
#87083=CARTESIAN_POINT('Ctrl Pts',(43.5095347923164,19.8291928550844,0.));
#87084=CARTESIAN_POINT('Ctrl Pts',(43.5095347923164,19.8291928550844,20.));
#87085=CARTESIAN_POINT('Ctrl Pts',(43.5205816644596,19.7976653574108,0.));
#87086=CARTESIAN_POINT('Ctrl Pts',(43.5205816644596,19.7976653574108,20.));
#87087=CARTESIAN_POINT('Ctrl Pts',(43.5316062267925,19.7661312344072,0.));
#87088=CARTESIAN_POINT('Ctrl Pts',(43.5316062267925,19.7661312344072,20.));
#87089=CARTESIAN_POINT('Ctrl Pts',(43.542608474795,19.734590501629,0.));
#87090=CARTESIAN_POINT('Ctrl Pts',(43.542608474795,19.734590501629,20.));
#87091=CARTESIAN_POINT('Ctrl Pts',(43.5535884039576,19.7030431746352,0.));
#87092=CARTESIAN_POINT('Ctrl Pts',(43.5535884039576,19.7030431746352,20.));
#87093=CARTESIAN_POINT('Ctrl Pts',(43.5645460097823,19.6714892689885,0.));
#87094=CARTESIAN_POINT('Ctrl Pts',(43.5645460097823,19.6714892689885,20.));
#87095=CARTESIAN_POINT('Ctrl Pts',(43.5754812877819,19.639928800255,0.));
#87096=CARTESIAN_POINT('Ctrl Pts',(43.5754812877819,19.639928800255,20.));
#87097=CARTESIAN_POINT('Ctrl Pts',(43.5863942334797,19.6083617840046,0.));
#87098=CARTESIAN_POINT('Ctrl Pts',(43.5863942334797,19.6083617840046,20.));
#87099=CARTESIAN_POINT('Ctrl Pts',(43.5972848424097,19.5767882358104,0.));
#87100=CARTESIAN_POINT('Ctrl Pts',(43.5972848424097,19.5767882358104,20.));
#87101=CARTESIAN_POINT('Ctrl Pts',(43.6081531101168,19.545208171249,0.));
#87102=CARTESIAN_POINT('Ctrl Pts',(43.6081531101168,19.545208171249,20.));
#87103=CARTESIAN_POINT('Ctrl Pts',(43.6189990321561,19.5136216059004,0.));
#87104=CARTESIAN_POINT('Ctrl Pts',(43.6189990321561,19.5136216059004,20.));
#87105=CARTESIAN_POINT('Ctrl Pts',(43.629822604094,19.4820285553483,0.));
#87106=CARTESIAN_POINT('Ctrl Pts',(43.629822604094,19.4820285553483,20.));
#87107=CARTESIAN_POINT('Ctrl Pts',(43.6406238215078,19.4504290351799,0.));
#87108=CARTESIAN_POINT('Ctrl Pts',(43.6406238215078,19.4504290351799,20.));
#87109=CARTESIAN_POINT('Ctrl Pts',(43.6514026799849,19.4188230609858,0.));
#87110=CARTESIAN_POINT('Ctrl Pts',(43.6514026799849,19.4188230609858,20.));
#87111=CARTESIAN_POINT('Ctrl Pts',(43.6621591751234,19.3872106483603,0.));
#87112=CARTESIAN_POINT('Ctrl Pts',(43.6621591751234,19.3872106483603,20.));
#87113=CARTESIAN_POINT('Ctrl Pts',(43.6728933025325,19.3555918129009,0.));
#87114=CARTESIAN_POINT('Ctrl Pts',(43.6728933025325,19.3555918129009,20.));
#87115=CARTESIAN_POINT('Ctrl Pts',(43.6836050578319,19.3239665702086,0.));
#87116=CARTESIAN_POINT('Ctrl Pts',(43.6836050578319,19.3239665702086,20.));
#87117=CARTESIAN_POINT('Ctrl Pts',(43.6942944366523,19.2923349358879,0.));
#87118=CARTESIAN_POINT('Ctrl Pts',(43.6942944366523,19.2923349358879,20.));
#87119=CARTESIAN_POINT('Ctrl Pts',(43.7049614346349,19.2606969255464,0.));
#87120=CARTESIAN_POINT('Ctrl Pts',(43.7049614346349,19.2606969255464,20.));
#87121=CARTESIAN_POINT('Ctrl Pts',(43.7156060474324,19.2290525547956,0.));
#87122=CARTESIAN_POINT('Ctrl Pts',(43.7156060474324,19.2290525547956,20.));
#87123=CARTESIAN_POINT('Ctrl Pts',(43.7262282707082,19.1974018392505,0.));
#87124=CARTESIAN_POINT('Ctrl Pts',(43.7262282707082,19.1974018392505,20.));
#87125=CARTESIAN_POINT('Ctrl Pts',(43.7368281001363,19.1657447945291,0.));
#87126=CARTESIAN_POINT('Ctrl Pts',(43.7368281001363,19.1657447945291,20.));
#87127=CARTESIAN_POINT('Ctrl Pts',(43.747405531401,19.1340814362531,0.));
#87128=CARTESIAN_POINT('Ctrl Pts',(43.747405531401,19.1340814362531,20.));
#87129=CARTESIAN_POINT('Ctrl Pts',(43.7579605601976,19.1024117800474,0.));
#87130=CARTESIAN_POINT('Ctrl Pts',(43.7579605601976,19.1024117800474,20.));
#87131=CARTESIAN_POINT('Ctrl Pts',(43.7684931822314,19.0707358415405,0.));
#87132=CARTESIAN_POINT('Ctrl Pts',(43.7684931822314,19.0707358415405,20.));
#87133=CARTESIAN_POINT('Ctrl Pts',(43.779003393219,19.039053636364,0.));
#87134=CARTESIAN_POINT('Ctrl Pts',(43.779003393219,19.039053636364,20.));
#87135=CARTESIAN_POINT('Ctrl Pts',(43.7894911888877,19.0073651801531,0.));
#87136=CARTESIAN_POINT('Ctrl Pts',(43.7894911888877,19.0073651801531,20.));
#87137=CARTESIAN_POINT('Ctrl Pts',(43.7999565649762,18.9756704885464,0.));
#87138=CARTESIAN_POINT('Ctrl Pts',(43.7999565649762,18.9756704885464,20.));
#87139=CARTESIAN_POINT('Ctrl Pts',(43.8103995172341,18.9439695771858,0.));
#87140=CARTESIAN_POINT('Ctrl Pts',(43.8103995172341,18.9439695771858,20.));
#87141=CARTESIAN_POINT('Ctrl Pts',(43.8208200414219,18.9122624617166,0.));
#87142=CARTESIAN_POINT('Ctrl Pts',(43.8208200414219,18.9122624617166,20.));
#87143=CARTESIAN_POINT('Ctrl Pts',(43.8312181333106,18.8805491577876,0.));
#87144=CARTESIAN_POINT('Ctrl Pts',(43.8312181333106,18.8805491577876,20.));
#87145=CARTESIAN_POINT('Ctrl Pts',(43.8415937886817,18.8488296810507,0.));
#87146=CARTESIAN_POINT('Ctrl Pts',(43.8415937886817,18.8488296810507,20.));
#87147=CARTESIAN_POINT('Ctrl Pts',(43.8519470033272,18.8171040471611,0.));
#87148=CARTESIAN_POINT('Ctrl Pts',(43.8519470033272,18.8171040471611,20.));
#87149=CARTESIAN_POINT('Ctrl Pts',(43.8622777730502,18.7853722717774,0.));
#87150=CARTESIAN_POINT('Ctrl Pts',(43.8622777730502,18.7853722717774,20.));
#87151=CARTESIAN_POINT('Ctrl Pts',(43.8725860936644,18.7536343705616,0.));
#87152=CARTESIAN_POINT('Ctrl Pts',(43.8725860936644,18.7536343705616,20.));
#87153=CARTESIAN_POINT('Ctrl Pts',(43.8828719609947,18.721890359179,0.));
#87154=CARTESIAN_POINT('Ctrl Pts',(43.8828719609947,18.721890359179,20.));
#87155=CARTESIAN_POINT('Ctrl Pts',(43.8931353708767,18.6901402532984,0.));
#87156=CARTESIAN_POINT('Ctrl Pts',(43.8931353708767,18.6901402532984,20.));
#87157=CARTESIAN_POINT('Ctrl Pts',(43.903376319157,18.6583840685915,0.));
#87158=CARTESIAN_POINT('Ctrl Pts',(43.903376319157,18.6583840685915,20.));
#87159=CARTESIAN_POINT('Ctrl Pts',(43.913594801693,18.6266218207337,0.));
#87160=CARTESIAN_POINT('Ctrl Pts',(43.913594801693,18.6266218207337,20.));
#87161=CARTESIAN_POINT('Ctrl Pts',(43.9237908143526,18.5948535254034,0.));
#87162=CARTESIAN_POINT('Ctrl Pts',(43.9237908143526,18.5948535254034,20.));
#87163=CARTESIAN_POINT('Ctrl Pts',(43.9339643530151,18.5630791982821,0.));
#87164=CARTESIAN_POINT('Ctrl Pts',(43.9339643530151,18.5630791982821,20.));
#87165=CARTESIAN_POINT('Ctrl Pts',(43.94411541357,18.5312988550549,0.));
#87166=CARTESIAN_POINT('Ctrl Pts',(43.94411541357,18.5312988550549,20.));
#87167=CARTESIAN_POINT('Ctrl Pts',(43.9542439919177,18.4995125114099,0.));
#87168=CARTESIAN_POINT('Ctrl Pts',(43.9542439919177,18.4995125114099,20.));
#87169=CARTESIAN_POINT('Ctrl Pts',(43.9643500839697,18.4677201830388,0.));
#87170=CARTESIAN_POINT('Ctrl Pts',(43.9643500839697,18.4677201830388,20.));
#87171=CARTESIAN_POINT('Ctrl Pts',(43.9744336856481,18.4359218856365,0.));
#87172=CARTESIAN_POINT('Ctrl Pts',(43.9744336856481,18.4359218856365,20.));
#87173=CARTESIAN_POINT('Ctrl Pts',(43.9844947928861,18.4041176349014,0.));
#87174=CARTESIAN_POINT('Ctrl Pts',(43.9844947928861,18.4041176349014,20.));
#87175=CARTESIAN_POINT('Ctrl Pts',(43.9945334016277,18.3723074465347,0.));
#87176=CARTESIAN_POINT('Ctrl Pts',(43.9945334016277,18.3723074465347,20.));
#87177=CARTESIAN_POINT('Ctrl Pts',(44.0045495078276,18.3404913362408,0.));
#87178=CARTESIAN_POINT('Ctrl Pts',(44.0045495078276,18.3404913362408,20.));
#87179=CARTESIAN_POINT('Ctrl Pts',(44.0145431074514,18.3086693197275,0.));
#87180=CARTESIAN_POINT('Ctrl Pts',(44.0145431074514,18.3086693197275,20.));
#87181=CARTESIAN_POINT('Ctrl Pts',(44.0245141964756,18.2768414127056,0.));
#87182=CARTESIAN_POINT('Ctrl Pts',(44.0245141964756,18.2768414127056,20.));
#87183=CARTESIAN_POINT('Ctrl Pts',(44.0344627708874,18.245007630889,0.));
#87184=CARTESIAN_POINT('Ctrl Pts',(44.0344627708874,18.245007630889,20.));
#87185=CARTESIAN_POINT('Ctrl Pts',(44.044388826685,18.2131679899948,0.));
#87186=CARTESIAN_POINT('Ctrl Pts',(44.044388826685,18.2131679899948,20.));
#87187=CARTESIAN_POINT('Ctrl Pts',(44.0542923598772,18.1813225057438,0.));
#87188=CARTESIAN_POINT('Ctrl Pts',(44.0542923598772,18.1813225057438,20.));
#87189=CARTESIAN_POINT('Ctrl Pts',(44.0641733664839,18.1494711938598,0.));
#87190=CARTESIAN_POINT('Ctrl Pts',(44.0641733664839,18.1494711938598,20.));
#87191=CARTESIAN_POINT('Ctrl Pts',(44.0740318425361,18.1176140700699,0.));
#87192=CARTESIAN_POINT('Ctrl Pts',(44.0740318425361,18.1176140700699,20.));
#87193=CARTESIAN_POINT('Ctrl Pts',(44.0838677840754,18.0857511501043,0.));
#87194=CARTESIAN_POINT('Ctrl Pts',(44.0838677840754,18.0857511501043,20.));
#87195=CARTESIAN_POINT('Ctrl Pts',(44.0936811871546,18.0538824496962,0.));
#87196=CARTESIAN_POINT('Ctrl Pts',(44.0936811871546,18.0538824496962,20.));
#87197=CARTESIAN_POINT('Ctrl Pts',(44.1034720478372,18.0220079845822,0.));
#87198=CARTESIAN_POINT('Ctrl Pts',(44.1034720478372,18.0220079845822,20.));
#87199=CARTESIAN_POINT('Ctrl Pts',(44.1132403621971,17.9901277705015,0.));
#87200=CARTESIAN_POINT('Ctrl Pts',(44.1132403621971,17.9901277705015,20.));
#87201=CARTESIAN_POINT('Ctrl Pts',(44.1229861263191,17.9582418231966,0.));
#87202=CARTESIAN_POINT('Ctrl Pts',(44.1229861263191,17.9582418231966,20.));
#87203=CARTESIAN_POINT('Ctrl Pts',(44.1327093362991,17.9263501584131,0.));
#87204=CARTESIAN_POINT('Ctrl Pts',(44.1327093362991,17.9263501584131,20.));
#87205=CARTESIAN_POINT('Ctrl Pts',(44.1424099882439,17.8944527919,0.));
#87206=CARTESIAN_POINT('Ctrl Pts',(44.1424099882439,17.8944527919,20.));
#87207=CARTESIAN_POINT('Ctrl Pts',(44.1520880782717,17.8625497394092,0.));
#87208=CARTESIAN_POINT('Ctrl Pts',(44.1520880782717,17.8625497394092,20.));
#87209=CARTESIAN_POINT('Ctrl Pts',(44.1617436025112,17.8306410166963,0.));
#87210=CARTESIAN_POINT('Ctrl Pts',(44.1617436025112,17.8306410166963,20.));
#87211=CARTESIAN_POINT('Ctrl Pts',(44.1713765571021,17.7987266395196,0.));
#87212=CARTESIAN_POINT('Ctrl Pts',(44.1713765571021,17.7987266395196,20.));
#87213=CARTESIAN_POINT('Ctrl Pts',(44.1809869381949,17.7668066236405,0.));
#87214=CARTESIAN_POINT('Ctrl Pts',(44.1809869381949,17.7668066236405,20.));
#87215=CARTESIAN_POINT('Ctrl Pts',(44.1905747419505,17.7348809848234,0.));
#87216=CARTESIAN_POINT('Ctrl Pts',(44.1905747419505,17.7348809848234,20.));
#87217=CARTESIAN_POINT('Ctrl Pts',(44.2001399645408,17.7029497388358,0.));
#87218=CARTESIAN_POINT('Ctrl Pts',(44.2001399645408,17.7029497388358,20.));
#87219=CARTESIAN_POINT('Ctrl Pts',(44.2096826021493,17.6710129014481,0.));
#87220=CARTESIAN_POINT('Ctrl Pts',(44.2096826021493,17.6710129014481,20.));
#87221=CARTESIAN_POINT('Ctrl Pts',(44.2192026509705,17.6390704884341,0.));
#87222=CARTESIAN_POINT('Ctrl Pts',(44.2192026509705,17.6390704884341,20.));
#87223=CARTESIAN_POINT('Ctrl Pts',(44.2287001072093,17.6071225155702,0.));
#87224=CARTESIAN_POINT('Ctrl Pts',(44.2287001072093,17.6071225155702,20.));
#87225=CARTESIAN_POINT('Ctrl Pts',(44.2381749670816,17.5751689986363,0.));
#87226=CARTESIAN_POINT('Ctrl Pts',(44.2381749670816,17.5751689986363,20.));
#87227=CARTESIAN_POINT('Ctrl Pts',(44.2476272268138,17.5432099534151,0.));
#87228=CARTESIAN_POINT('Ctrl Pts',(44.2476272268138,17.5432099534151,20.));
#87229=CARTESIAN_POINT('Ctrl Pts',(44.2570568826434,17.5112453956925,0.));
#87230=CARTESIAN_POINT('Ctrl Pts',(44.2570568826434,17.5112453956925,20.));
#87231=CARTESIAN_POINT('Ctrl Pts',(44.2664639308191,17.4792753412574,0.));
#87232=CARTESIAN_POINT('Ctrl Pts',(44.2664639308191,17.4792753412574,20.));
#87233=CARTESIAN_POINT('Ctrl Pts',(44.2758483676008,17.447299805902,0.));
#87234=CARTESIAN_POINT('Ctrl Pts',(44.2758483676008,17.447299805902,20.));
#87235=CARTESIAN_POINT('Ctrl Pts',(44.2852101892593,17.4153188054211,0.));
#87236=CARTESIAN_POINT('Ctrl Pts',(44.2852101892593,17.4153188054211,20.));
#87237=CARTESIAN_POINT('Ctrl Pts',(44.294549392076,17.3833323556128,0.));
#87238=CARTESIAN_POINT('Ctrl Pts',(44.294549392076,17.3833323556128,20.));
#87239=CARTESIAN_POINT('Ctrl Pts',(44.3038659723435,17.3513404722779,0.));
#87240=CARTESIAN_POINT('Ctrl Pts',(44.3038659723435,17.3513404722779,20.));
#87241=CARTESIAN_POINT('Ctrl Pts',(44.3131599263642,17.3193431712198,0.));
#87242=CARTESIAN_POINT('Ctrl Pts',(44.3131599263642,17.3193431712198,20.));
#87243=CARTESIAN_POINT('Ctrl Pts',(44.3224312504523,17.2873404682456,0.));
#87244=CARTESIAN_POINT('Ctrl Pts',(44.3224312504523,17.2873404682456,20.));
#87245=CARTESIAN_POINT('Ctrl Pts',(44.3316799409325,17.2553323791649,0.));
#87246=CARTESIAN_POINT('Ctrl Pts',(44.3316799409325,17.2553323791649,20.));
#87247=CARTESIAN_POINT('Ctrl Pts',(44.340905994141,17.2233189197905,0.));
#87248=CARTESIAN_POINT('Ctrl Pts',(44.340905994141,17.2233189197905,20.));
#87249=CARTESIAN_POINT('Ctrl Pts',(44.3501094064252,17.1913001059384,0.));
#87250=CARTESIAN_POINT('Ctrl Pts',(44.3501094064252,17.1913001059384,20.));
#87251=CARTESIAN_POINT('Ctrl Pts',(44.3592901741436,17.1592759534275,0.));
#87252=CARTESIAN_POINT('Ctrl Pts',(44.3592901741436,17.1592759534275,20.));
#87253=CARTESIAN_POINT('Ctrl Pts',(44.3684482936655,17.1272464780797,0.));
#87254=CARTESIAN_POINT('Ctrl Pts',(44.3684482936655,17.1272464780797,20.));
#87255=CARTESIAN_POINT('Ctrl Pts',(44.3775837613707,17.0952116957196,0.));
#87256=CARTESIAN_POINT('Ctrl Pts',(44.3775837613707,17.0952116957196,20.));
#87257=CARTESIAN_POINT('Ctrl Pts',(44.3866965736492,17.0631716221745,0.));
#87258=CARTESIAN_POINT('Ctrl Pts',(44.3866965736492,17.0631716221745,20.));
#87259=CARTESIAN_POINT('Ctrl Pts',(44.3957867269024,17.0311262732746,0.));
#87260=CARTESIAN_POINT('Ctrl Pts',(44.3957867269024,17.0311262732746,20.));
#87261=CARTESIAN_POINT('Ctrl Pts',(44.404854217543,16.9990756648532,0.));
#87262=CARTESIAN_POINT('Ctrl Pts',(44.404854217543,16.9990756648532,20.));
#87263=CARTESIAN_POINT('Ctrl Pts',(44.4138990419958,16.967019812747,0.));
#87264=CARTESIAN_POINT('Ctrl Pts',(44.4138990419958,16.967019812747,20.));
#87265=CARTESIAN_POINT('Ctrl Pts',(44.4229211966955,16.9349587327952,0.));
#87266=CARTESIAN_POINT('Ctrl Pts',(44.4229211966955,16.9349587327952,20.));
#87267=CARTESIAN_POINT('Ctrl Pts',(44.4319206780879,16.9028924408399,0.));
#87268=CARTESIAN_POINT('Ctrl Pts',(44.4319206780879,16.9028924408399,20.));
#87269=CARTESIAN_POINT('Ctrl Pts',(44.4408974826293,16.870820952726,0.));
#87270=CARTESIAN_POINT('Ctrl Pts',(44.4408974826293,16.870820952726,20.));
#87271=CARTESIAN_POINT('Ctrl Pts',(44.4498516067869,16.8387442843012,0.));
#87272=CARTESIAN_POINT('Ctrl Pts',(44.4498516067869,16.8387442843012,20.));
#87273=CARTESIAN_POINT('Ctrl Pts',(44.4587830470388,16.8066624514163,0.));
#87274=CARTESIAN_POINT('Ctrl Pts',(44.4587830470388,16.8066624514163,20.));
#87275=CARTESIAN_POINT('Ctrl Pts',(44.4676917998748,16.7745754699247,0.));
#87276=CARTESIAN_POINT('Ctrl Pts',(44.4676917998748,16.7745754699247,20.));
#87277=CARTESIAN_POINT('Ctrl Pts',(44.4765778617956,16.742483355683,0.));
#87278=CARTESIAN_POINT('Ctrl Pts',(44.4765778617956,16.742483355683,20.));
#87279=CARTESIAN_POINT('Ctrl Pts',(44.4854412293128,16.7103861245505,0.));
#87280=CARTESIAN_POINT('Ctrl Pts',(44.4854412293128,16.7103861245505,20.));
#87281=CARTESIAN_POINT('Ctrl Pts',(44.4942818989491,16.6782837923893,0.));
#87282=CARTESIAN_POINT('Ctrl Pts',(44.4942818989491,16.6782837923893,20.));
#87283=CARTESIAN_POINT('Ctrl Pts',(44.503099867238,16.6461763750644,0.));
#87284=CARTESIAN_POINT('Ctrl Pts',(44.503099867238,16.6461763750644,20.));
#87285=CARTESIAN_POINT('Ctrl Pts',(44.5118951307243,16.6140638884438,0.));
#87286=CARTESIAN_POINT('Ctrl Pts',(44.5118951307243,16.6140638884438,20.));
#87287=CARTESIAN_POINT('Ctrl Pts',(44.5206676859632,16.581946348398,0.));
#87288=CARTESIAN_POINT('Ctrl Pts',(44.5206676859632,16.581946348398,20.));
#87289=CARTESIAN_POINT('Ctrl Pts',(44.5294175295214,16.5498237708003,0.));
#87290=CARTESIAN_POINT('Ctrl Pts',(44.5294175295214,16.5498237708003,20.));
#87291=CARTESIAN_POINT('Ctrl Pts',(44.5381446579761,16.5176961715269,0.));
#87292=CARTESIAN_POINT('Ctrl Pts',(44.5381446579761,16.5176961715269,20.));
#87293=CARTESIAN_POINT('Ctrl Pts',(44.5468490679154,16.4855635664567,0.));
#87294=CARTESIAN_POINT('Ctrl Pts',(44.5468490679154,16.4855635664567,20.));
#87295=CARTESIAN_POINT('Ctrl Pts',(44.5555307559385,16.4534259714715,0.));
#87296=CARTESIAN_POINT('Ctrl Pts',(44.5555307559385,16.4534259714715,20.));
#87297=CARTESIAN_POINT('Ctrl Pts',(44.5641897186557,16.4212834024559,0.));
#87298=CARTESIAN_POINT('Ctrl Pts',(44.5641897186557,16.4212834024559,20.));
#87299=CARTESIAN_POINT('Ctrl Pts',(44.5728259526889,16.3891358752972,0.));
#87300=CARTESIAN_POINT('Ctrl Pts',(44.5728259526889,16.3891358752972,20.));
#87301=CARTESIAN_POINT('Ctrl Pts',(44.581439454671,16.3569834058857,0.));
#87302=CARTESIAN_POINT('Ctrl Pts',(44.581439454671,16.3569834058857,20.));
#87303=CARTESIAN_POINT('Ctrl Pts',(44.5900302212458,16.3248260101143,0.));
#87304=CARTESIAN_POINT('Ctrl Pts',(44.5900302212458,16.3248260101143,20.));
#87305=CARTESIAN_POINT('Ctrl Pts',(44.5985982490682,16.2926637038787,0.));
#87306=CARTESIAN_POINT('Ctrl Pts',(44.5985982490682,16.2926637038787,20.));
#87307=CARTESIAN_POINT('Ctrl Pts',(44.6071435348036,16.2604965030773,0.));
#87308=CARTESIAN_POINT('Ctrl Pts',(44.6071435348036,16.2604965030773,20.));
#87309=CARTESIAN_POINT('Ctrl Pts',(44.6156660751288,16.2283244236112,0.));
#87310=CARTESIAN_POINT('Ctrl Pts',(44.6156660751288,16.2283244236112,20.));
#87311=CARTESIAN_POINT('Ctrl Pts',(44.6241658667307,16.196147481384,0.));
#87312=CARTESIAN_POINT('Ctrl Pts',(44.6241658667307,16.196147481384,20.));
#87313=CARTESIAN_POINT('Ctrl Pts',(44.6326429063072,16.1639656923023,0.));
#87314=CARTESIAN_POINT('Ctrl Pts',(44.6326429063072,16.1639656923023,20.));
#87315=CARTESIAN_POINT('Ctrl Pts',(44.6410971905673,16.131779072275,0.));
#87316=CARTESIAN_POINT('Ctrl Pts',(44.6410971905673,16.131779072275,20.));
#87317=CARTESIAN_POINT('Ctrl Pts',(44.649528716232,16.0995876372141,0.));
#87318=CARTESIAN_POINT('Ctrl Pts',(44.649528716232,16.0995876372141,20.));
#87319=CARTESIAN_POINT('Ctrl Pts',(44.6579374800339,16.0673914030343,0.));
#87320=CARTESIAN_POINT('Ctrl Pts',(44.6579374800339,16.0673914030343,20.));
#87321=CARTESIAN_POINT('Ctrl Pts',(44.6663234787169,16.0351903856534,0.));
#87322=CARTESIAN_POINT('Ctrl Pts',(44.6663234787169,16.0351903856534,20.));
#87323=CARTESIAN_POINT('Ctrl Pts',(44.6746867090345,16.0029846009915,0.));
#87324=CARTESIAN_POINT('Ctrl Pts',(44.6746867090345,16.0029846009915,20.));
#87325=CARTESIAN_POINT('Ctrl Pts',(44.6830271677516,15.9707740649715,0.));
#87326=CARTESIAN_POINT('Ctrl Pts',(44.6830271677516,15.9707740649715,20.));
#87327=CARTESIAN_POINT('Ctrl Pts',(44.691344851643,15.9385587935186,0.));
#87328=CARTESIAN_POINT('Ctrl Pts',(44.691344851643,15.9385587935186,20.));
#87329=CARTESIAN_POINT('Ctrl Pts',(44.6996397574952,15.9063388025603,0.));
#87330=CARTESIAN_POINT('Ctrl Pts',(44.6996397574952,15.9063388025603,20.));
#87331=CARTESIAN_POINT('Ctrl Pts',(44.7079118821065,15.8741141080272,0.));
#87332=CARTESIAN_POINT('Ctrl Pts',(44.7079118821065,15.8741141080272,20.));
#87333=CARTESIAN_POINT('Ctrl Pts',(44.7161612222865,15.8418847258528,0.));
#87334=CARTESIAN_POINT('Ctrl Pts',(44.7161612222865,15.8418847258528,20.));
#87335=CARTESIAN_POINT('Ctrl Pts',(44.7243877748558,15.8096506719735,0.));
#87336=CARTESIAN_POINT('Ctrl Pts',(44.7243877748558,15.8096506719735,20.));
#87337=CARTESIAN_POINT('Ctrl Pts',(44.7325915366458,15.7774119623278,0.));
#87338=CARTESIAN_POINT('Ctrl Pts',(44.7325915366458,15.7774119623278,20.));
#87339=CARTESIAN_POINT('Ctrl Pts',(44.7407725044985,15.745168612857,0.));
#87340=CARTESIAN_POINT('Ctrl Pts',(44.7407725044985,15.745168612857,20.));
#87341=CARTESIAN_POINT('Ctrl Pts',(44.7489306752664,15.7129206395047,0.));
#87342=CARTESIAN_POINT('Ctrl Pts',(44.7489306752664,15.7129206395047,20.));
#87343=CARTESIAN_POINT('Ctrl Pts',(44.7570660458133,15.6806680582172,0.));
#87344=CARTESIAN_POINT('Ctrl Pts',(44.7570660458133,15.6806680582172,20.));
#87345=CARTESIAN_POINT('Ctrl Pts',(44.7651786130144,15.6484108849434,0.));
#87346=CARTESIAN_POINT('Ctrl Pts',(44.7651786130144,15.6484108849434,20.));
#87347=CARTESIAN_POINT('Ctrl Pts',(44.7732683737566,15.6161491356348,0.));
#87348=CARTESIAN_POINT('Ctrl Pts',(44.7732683737566,15.6161491356348,20.));
#87349=CARTESIAN_POINT('Ctrl Pts',(44.7813353249379,15.583882826246,0.));
#87350=CARTESIAN_POINT('Ctrl Pts',(44.7813353249379,15.583882826246,20.));
#87351=CARTESIAN_POINT('Ctrl Pts',(44.7893794634672,15.5516119727338,0.));
#87352=CARTESIAN_POINT('Ctrl Pts',(44.7893794634672,15.5516119727338,20.));
#87353=CARTESIAN_POINT('Ctrl Pts',(44.7974007862643,15.5193365910578,0.));
#87354=CARTESIAN_POINT('Ctrl Pts',(44.7974007862643,15.5193365910578,20.));
#87355=CARTESIAN_POINT('Ctrl Pts',(44.8053992902599,15.4870566971799,0.));
#87356=CARTESIAN_POINT('Ctrl Pts',(44.8053992902599,15.4870566971799,20.));
#87357=CARTESIAN_POINT('Ctrl Pts',(44.8133749723964,15.4547723070643,0.));
#87358=CARTESIAN_POINT('Ctrl Pts',(44.8133749723964,15.4547723070643,20.));
#87359=CARTESIAN_POINT('Ctrl Pts',(44.8213278296263,15.4224834366782,0.));
#87360=CARTESIAN_POINT('Ctrl Pts',(44.8213278296263,15.4224834366782,20.));
#87361=CARTESIAN_POINT('Ctrl Pts',(44.8292578589132,15.3901901019906,0.));
#87362=CARTESIAN_POINT('Ctrl Pts',(44.8292578589132,15.3901901019906,20.));
#87363=CARTESIAN_POINT('Ctrl Pts',(44.8371650572316,15.3578923189739,0.));
#87364=CARTESIAN_POINT('Ctrl Pts',(44.8371650572316,15.3578923189739,20.));
#87365=CARTESIAN_POINT('Ctrl Pts',(44.8450494215678,15.3255901036026,0.));
#87366=CARTESIAN_POINT('Ctrl Pts',(44.8450494215678,15.3255901036026,20.));
#87367=CARTESIAN_POINT('Ctrl Pts',(44.8529109489191,15.2932834718541,0.));
#87368=CARTESIAN_POINT('Ctrl Pts',(44.8529109489191,15.2932834718541,20.));
#87369=CARTESIAN_POINT('Ctrl Pts',(44.8607496362943,15.2609724397079,0.));
#87370=CARTESIAN_POINT('Ctrl Pts',(44.8607496362943,15.2609724397079,20.));
#87371=CARTESIAN_POINT('Ctrl Pts',(44.8685654807131,15.2286570231461,0.));
#87372=CARTESIAN_POINT('Ctrl Pts',(44.8685654807131,15.2286570231461,20.));
#87373=CARTESIAN_POINT('Ctrl Pts',(44.8763584792064,15.1963372381533,0.));
#87374=CARTESIAN_POINT('Ctrl Pts',(44.8763584792064,15.1963372381533,20.));
#87375=CARTESIAN_POINT('Ctrl Pts',(44.8841286288163,15.1640131007166,0.));
#87376=CARTESIAN_POINT('Ctrl Pts',(44.8841286288163,15.1640131007166,20.));
#87377=CARTESIAN_POINT('Ctrl Pts',(44.8918759265956,15.1316846268256,0.));
#87378=CARTESIAN_POINT('Ctrl Pts',(44.8918759265956,15.1316846268256,20.));
#87379=CARTESIAN_POINT('Ctrl Pts',(44.8996003696078,15.0993518324721,0.));
#87380=CARTESIAN_POINT('Ctrl Pts',(44.8996003696078,15.0993518324721,20.));
#87381=CARTESIAN_POINT('Ctrl Pts',(44.9073019549277,15.0670147336509,0.));
#87382=CARTESIAN_POINT('Ctrl Pts',(44.9073019549277,15.0670147336509,20.));
#87383=CARTESIAN_POINT('Ctrl Pts',(44.9149806796409,15.034673346359,0.));
#87384=CARTESIAN_POINT('Ctrl Pts',(44.9149806796409,15.034673346359,20.));
#87385=CARTESIAN_POINT('Ctrl Pts',(44.9226365408441,15.0023276865958,0.));
#87386=CARTESIAN_POINT('Ctrl Pts',(44.9226365408441,15.0023276865958,20.));
#87387=CARTESIAN_POINT('Ctrl Pts',(44.9302695356455,14.969977770363,0.));
#87388=CARTESIAN_POINT('Ctrl Pts',(44.9302695356455,14.969977770363,20.));
#87389=CARTESIAN_POINT('Ctrl Pts',(44.9378796611651,14.9376236136649,0.));
#87390=CARTESIAN_POINT('Ctrl Pts',(44.9378796611651,14.9376236136649,20.));
#87391=CARTESIAN_POINT('Ctrl Pts',(44.9454669145344,14.9052652325081,0.));
#87392=CARTESIAN_POINT('Ctrl Pts',(44.9454669145344,14.9052652325081,20.));
#87393=CARTESIAN_POINT('Ctrl Pts',(44.9530312928957,14.8729026429019,0.));
#87394=CARTESIAN_POINT('Ctrl Pts',(44.9530312928957,14.8729026429019,20.));
#87395=CARTESIAN_POINT('Ctrl Pts',(44.9605727934022,14.8405358608577,0.));
#87396=CARTESIAN_POINT('Ctrl Pts',(44.9605727934022,14.8405358608577,20.));
#87397=CARTESIAN_POINT('Ctrl Pts',(44.9680914132176,14.8081649023895,0.));
#87398=CARTESIAN_POINT('Ctrl Pts',(44.9680914132176,14.8081649023895,20.));
#87399=CARTESIAN_POINT('Ctrl Pts',(44.9755871495162,14.7757897835134,0.));
#87400=CARTESIAN_POINT('Ctrl Pts',(44.9755871495162,14.7757897835134,20.));
#87401=CARTESIAN_POINT('Ctrl Pts',(44.9830599994838,14.7434105202483,0.));
#87402=CARTESIAN_POINT('Ctrl Pts',(44.9830599994838,14.7434105202483,20.));
#87403=CARTESIAN_POINT('Ctrl Pts',(44.9905099603172,14.7110271286153,0.));
#87404=CARTESIAN_POINT('Ctrl Pts',(44.9905099603172,14.7110271286153,20.));
#87405=CARTESIAN_POINT('Ctrl Pts',(44.9979370292252,14.6786396246378,0.));
#87406=CARTESIAN_POINT('Ctrl Pts',(44.9979370292252,14.6786396246378,20.));
#87407=CARTESIAN_POINT('Ctrl Pts',(45.0053412034276,14.6462480243418,0.));
#87408=CARTESIAN_POINT('Ctrl Pts',(45.0053412034276,14.6462480243418,20.));
#87409=CARTESIAN_POINT('Ctrl Pts',(45.0127224801553,14.6138523437553,0.));
#87410=CARTESIAN_POINT('Ctrl Pts',(45.0127224801553,14.6138523437553,20.));
#87411=CARTESIAN_POINT('Ctrl Pts',(45.020080856651,14.5814525989087,0.));
#87412=CARTESIAN_POINT('Ctrl Pts',(45.020080856651,14.5814525989087,20.));
#87413=CARTESIAN_POINT('Ctrl Pts',(45.0274163301681,14.5490488058349,0.));
#87414=CARTESIAN_POINT('Ctrl Pts',(45.0274163301681,14.5490488058349,20.));
#87415=CARTESIAN_POINT('Ctrl Pts',(45.0347288979708,14.516640980569,0.));
#87416=CARTESIAN_POINT('Ctrl Pts',(45.0347288979708,14.516640980569,20.));
#87417=CARTESIAN_POINT('Ctrl Pts',(45.0420185573341,14.4842291391484,0.));
#87418=CARTESIAN_POINT('Ctrl Pts',(45.0420185573341,14.4842291391484,20.));
#87419=CARTESIAN_POINT('Ctrl Pts',(45.0492853055441,14.451813297613,0.));
#87420=CARTESIAN_POINT('Ctrl Pts',(45.0492853055441,14.451813297613,20.));
#87421=CARTESIAN_POINT('Ctrl Pts',(45.0565291398984,14.4193934720051,0.));
#87422=CARTESIAN_POINT('Ctrl Pts',(45.0565291398984,14.4193934720051,20.));
#87423=CARTESIAN_POINT('Ctrl Pts',(45.0637500577056,14.3869696783692,0.));
#87424=CARTESIAN_POINT('Ctrl Pts',(45.0637500577056,14.3869696783692,20.));
#87425=CARTESIAN_POINT('Ctrl Pts',(45.0709480562863,14.354541932752,0.));
#87426=CARTESIAN_POINT('Ctrl Pts',(45.0709480562863,14.354541932752,20.));
#87427=CARTESIAN_POINT('Ctrl Pts',(45.0781231329719,14.3221102512025,0.));
#87428=CARTESIAN_POINT('Ctrl Pts',(45.0781231329719,14.3221102512025,20.));
#87429=CARTESIAN_POINT('Ctrl Pts',(45.0852752851048,14.2896746497719,0.));
#87430=CARTESIAN_POINT('Ctrl Pts',(45.0852752851048,14.2896746497719,20.));
#87431=CARTESIAN_POINT('Ctrl Pts',(45.0924045100383,14.2572351445137,0.));
#87432=CARTESIAN_POINT('Ctrl Pts',(45.0924045100383,14.2572351445137,20.));
#87433=CARTESIAN_POINT('Ctrl Pts',(45.0995108051367,14.2247917514836,0.));
#87434=CARTESIAN_POINT('Ctrl Pts',(45.0995108051367,14.2247917514836,20.));
#87435=CARTESIAN_POINT('Ctrl Pts',(45.1065941677758,14.1923444867396,0.));
#87436=CARTESIAN_POINT('Ctrl Pts',(45.1065941677758,14.1923444867396,20.));
#87437=CARTESIAN_POINT('Ctrl Pts',(45.1136545953429,14.1598933663423,0.));
#87438=CARTESIAN_POINT('Ctrl Pts',(45.1136545953429,14.1598933663423,20.));
#87439=CARTESIAN_POINT('Ctrl Pts',(45.1206920852361,14.127438406354,0.));
#87440=CARTESIAN_POINT('Ctrl Pts',(45.1206920852361,14.127438406354,20.));
#87441=CARTESIAN_POINT('Ctrl Pts',(45.127706634865,14.0949796228398,0.));
#87442=CARTESIAN_POINT('Ctrl Pts',(45.127706634865,14.0949796228398,20.));
#87443=CARTESIAN_POINT('Ctrl Pts',(45.1346982416501,14.0625170318665,0.));
#87444=CARTESIAN_POINT('Ctrl Pts',(45.1346982416501,14.0625170318665,20.));
#87445=CARTESIAN_POINT('Ctrl Pts',(45.1416669030232,14.0300506495033,0.));
#87446=CARTESIAN_POINT('Ctrl Pts',(45.1416669030232,14.0300506495033,20.));
#87447=CARTESIAN_POINT('Ctrl Pts',(45.1486126164275,13.997580491822,0.));
#87448=CARTESIAN_POINT('Ctrl Pts',(45.1486126164275,13.997580491822,20.));
#87449=CARTESIAN_POINT('Ctrl Pts',(45.1555353793172,13.9651065748961,0.));
#87450=CARTESIAN_POINT('Ctrl Pts',(45.1555353793172,13.9651065748961,20.));
#87451=CARTESIAN_POINT('Ctrl Pts',(45.1624351891574,13.9326289148012,0.));
#87452=CARTESIAN_POINT('Ctrl Pts',(45.1624351891574,13.9326289148012,20.));
#87453=CARTESIAN_POINT('Ctrl Pts',(45.1693120434241,13.9001475276153,0.));
#87454=CARTESIAN_POINT('Ctrl Pts',(45.1693120434241,13.9001475276153,20.));
#87455=CARTESIAN_POINT('Ctrl Pts',(45.1761659396043,13.8676624294184,0.));
#87456=CARTESIAN_POINT('Ctrl Pts',(45.1761659396043,13.8676624294184,20.));
#87457=CARTESIAN_POINT('Ctrl Pts',(45.1829968751969,13.8351736362929,0.));
#87458=CARTESIAN_POINT('Ctrl Pts',(45.1829968751969,13.8351736362929,20.));
#87459=CARTESIAN_POINT('Ctrl Pts',(45.1898048477123,13.8026811643234,0.));
#87460=CARTESIAN_POINT('Ctrl Pts',(45.1898048477123,13.8026811643234,20.));
#87461=CARTESIAN_POINT('Ctrl Pts',(45.1965898546723,13.7701850295968,0.));
#87462=CARTESIAN_POINT('Ctrl Pts',(45.1965898546723,13.7701850295968,20.));
#87463=CARTESIAN_POINT('Ctrl Pts',(45.2033518936101,13.7376852482019,0.));
#87464=CARTESIAN_POINT('Ctrl Pts',(45.2033518936101,13.7376852482019,20.));
#87465=CARTESIAN_POINT('Ctrl Pts',(45.2100909620697,13.7051818362299,0.));
#87466=CARTESIAN_POINT('Ctrl Pts',(45.2100909620697,13.7051818362299,20.));
#87467=CARTESIAN_POINT('Ctrl Pts',(45.2168070576061,13.6726748097738,0.));
#87468=CARTESIAN_POINT('Ctrl Pts',(45.2168070576061,13.6726748097738,20.));
#87469=CARTESIAN_POINT('Ctrl Pts',(45.2235001777847,13.6401641849286,0.));
#87470=CARTESIAN_POINT('Ctrl Pts',(45.2235001777847,13.6401641849286,20.));
#87471=CARTESIAN_POINT('Ctrl Pts',(45.2301703201819,13.6076499777915,0.));
#87472=CARTESIAN_POINT('Ctrl Pts',(45.2301703201819,13.6076499777915,20.));
#87473=CARTESIAN_POINT('Ctrl Pts',(45.2368174823856,13.5751322044618,0.));
#87474=CARTESIAN_POINT('Ctrl Pts',(45.2368174823856,13.5751322044618,20.));
#87475=CARTESIAN_POINT('Ctrl Pts',(45.2434416619952,13.542610881041,0.));
#87476=CARTESIAN_POINT('Ctrl Pts',(45.2434416619952,13.542610881041,20.));
#87477=CARTESIAN_POINT('Ctrl Pts',(45.2500428566225,13.5100860236329,0.));
#87478=CARTESIAN_POINT('Ctrl Pts',(45.2500428566225,13.5100860236329,20.));
#87479=CARTESIAN_POINT('Ctrl Pts',(45.2566210638904,13.4775576483433,0.));
#87480=CARTESIAN_POINT('Ctrl Pts',(45.2566210638904,13.4775576483433,20.));
#87481=CARTESIAN_POINT('Ctrl Pts',(45.2631762814325,13.44502577128,0.));
#87482=CARTESIAN_POINT('Ctrl Pts',(45.2631762814325,13.44502577128,20.));
#87483=CARTESIAN_POINT('Ctrl Pts',(45.2697085068935,13.4124904085531,0.));
#87484=CARTESIAN_POINT('Ctrl Pts',(45.2697085068935,13.4124904085531,20.));
#87485=CARTESIAN_POINT('Ctrl Pts',(45.276217737929,13.3799515762744,0.));
#87486=CARTESIAN_POINT('Ctrl Pts',(45.276217737929,13.3799515762744,20.));
#87487=CARTESIAN_POINT('Ctrl Pts',(45.2827039722059,13.3474092905576,0.));
#87488=CARTESIAN_POINT('Ctrl Pts',(45.2827039722059,13.3474092905576,20.));
#87489=CARTESIAN_POINT('Ctrl Pts',(45.2891672074022,13.3148635675188,0.));
#87490=CARTESIAN_POINT('Ctrl Pts',(45.2891672074022,13.3148635675188,20.));
#87491=CARTESIAN_POINT('Ctrl Pts',(45.2956074412073,13.282314423276,0.));
#87492=CARTESIAN_POINT('Ctrl Pts',(45.2956074412073,13.282314423276,20.));
#87493=CARTESIAN_POINT('Ctrl Pts',(45.3020246713218,13.2497618739494,0.));
#87494=CARTESIAN_POINT('Ctrl Pts',(45.3020246713218,13.2497618739494,20.));
#87495=CARTESIAN_POINT('Ctrl Pts',(45.3084188954577,13.217205935661,0.));
#87496=CARTESIAN_POINT('Ctrl Pts',(45.3084188954577,13.217205935661,20.));
#87497=CARTESIAN_POINT('Ctrl Pts',(45.3147901113387,13.1846466245352,0.));
#87498=CARTESIAN_POINT('Ctrl Pts',(45.3147901113387,13.1846466245352,20.));
#87499=CARTESIAN_POINT('Ctrl Pts',(45.321138316699,13.1520839566979,0.));
#87500=CARTESIAN_POINT('Ctrl Pts',(45.321138316699,13.1520839566979,20.));
#87501=CARTESIAN_POINT('Ctrl Pts',(45.3274635092846,13.1195179482773,0.));
#87502=CARTESIAN_POINT('Ctrl Pts',(45.3274635092846,13.1195179482773,20.));
#87503=CARTESIAN_POINT('Ctrl Pts',(45.3337656868523,13.0869486154035,0.));
#87504=CARTESIAN_POINT('Ctrl Pts',(45.3337656868523,13.0869486154035,20.));
#87505=CARTESIAN_POINT('Ctrl Pts',(45.3400448471699,13.0543759742083,0.));
#87506=CARTESIAN_POINT('Ctrl Pts',(45.3400448471699,13.0543759742083,20.));
#87507=CARTESIAN_POINT('Ctrl Pts',(45.3463009880171,13.021800040826,0.));
#87508=CARTESIAN_POINT('Ctrl Pts',(45.3463009880171,13.021800040826,20.));
#87509=CARTESIAN_POINT('Ctrl Pts',(45.3525341071849,12.9892208313927,0.));
#87510=CARTESIAN_POINT('Ctrl Pts',(45.3525341071849,12.9892208313927,20.));
#87511=CARTESIAN_POINT('Ctrl Pts',(45.3587442024753,12.9566383620464,0.));
#87512=CARTESIAN_POINT('Ctrl Pts',(45.3587442024753,12.9566383620464,20.));
#87513=CARTESIAN_POINT('Ctrl Pts',(45.364931271701,12.9240526489273,0.));
#87514=CARTESIAN_POINT('Ctrl Pts',(45.364931271701,12.9240526489273,20.));
#87515=CARTESIAN_POINT('Ctrl Pts',(45.371095312686,12.8914637081769,0.));
#87516=CARTESIAN_POINT('Ctrl Pts',(45.371095312686,12.8914637081769,20.));
#87517=CARTESIAN_POINT('Ctrl Pts',(45.3772363232658,12.8588715559393,0.));
#87518=CARTESIAN_POINT('Ctrl Pts',(45.3772363232658,12.8588715559393,20.));
#87519=CARTESIAN_POINT('Ctrl Pts',(45.3833543012877,12.82627620836,0.));
#87520=CARTESIAN_POINT('Ctrl Pts',(45.3833543012877,12.82627620836,20.));
#87521=CARTESIAN_POINT('Ctrl Pts',(45.3894492446102,12.7936776815868,0.));
#87522=CARTESIAN_POINT('Ctrl Pts',(45.3894492446102,12.7936776815868,20.));
#87523=CARTESIAN_POINT('Ctrl Pts',(45.3955211511033,12.7610759917694,0.));
#87524=CARTESIAN_POINT('Ctrl Pts',(45.3955211511033,12.7610759917694,20.));
#87525=CARTESIAN_POINT('Ctrl Pts',(45.4015700186485,12.7284711550592,0.));
#87526=CARTESIAN_POINT('Ctrl Pts',(45.4015700186485,12.7284711550592,20.));
#87527=CARTESIAN_POINT('Ctrl Pts',(45.407595845137,12.6958631876099,0.));
#87528=CARTESIAN_POINT('Ctrl Pts',(45.407595845137,12.6958631876099,20.));
#87529=CARTESIAN_POINT('Ctrl Pts',(45.4135986284717,12.6632521055766,0.));
#87530=CARTESIAN_POINT('Ctrl Pts',(45.4135986284717,12.6632521055766,20.));
#87531=CARTESIAN_POINT('Ctrl Pts',(45.4195783665665,12.6306379251165,0.));
#87532=CARTESIAN_POINT('Ctrl Pts',(45.4195783665665,12.6306379251165,20.));
#87533=CARTESIAN_POINT('Ctrl Pts',(45.4255350573473,12.5980206623884,0.));
#87534=CARTESIAN_POINT('Ctrl Pts',(45.4255350573473,12.5980206623884,20.));
#87535=CARTESIAN_POINT('Ctrl Pts',(45.4314686987515,12.5654003335533,0.));
#87536=CARTESIAN_POINT('Ctrl Pts',(45.4314686987515,12.5654003335533,20.));
#87537=CARTESIAN_POINT('Ctrl Pts',(45.4373792887274,12.5327769547739,0.));
#87538=CARTESIAN_POINT('Ctrl Pts',(45.4373792887274,12.5327769547739,20.));
#87539=CARTESIAN_POINT('Ctrl Pts',(45.4432668252347,12.500150542215,0.));
#87540=CARTESIAN_POINT('Ctrl Pts',(45.4432668252347,12.500150542215,20.));
#87541=CARTESIAN_POINT('Ctrl Pts',(45.4491313062444,12.4675211120431,0.));
#87542=CARTESIAN_POINT('Ctrl Pts',(45.4491313062444,12.4675211120431,20.));
#87543=CARTESIAN_POINT('Ctrl Pts',(45.4549727297392,12.4348886804266,0.));
#87544=CARTESIAN_POINT('Ctrl Pts',(45.4549727297392,12.4348886804266,20.));
#87545=CARTESIAN_POINT('Ctrl Pts',(45.4607910937128,12.4022532635357,0.));
#87546=CARTESIAN_POINT('Ctrl Pts',(45.4607910937128,12.4022532635357,20.));
#87547=CARTESIAN_POINT('Ctrl Pts',(45.4665863961701,12.3696148775423,0.));
#87548=CARTESIAN_POINT('Ctrl Pts',(45.4665863961701,12.3696148775423,20.));
#87549=CARTESIAN_POINT('Ctrl Pts',(45.4723586351267,12.3369735386201,0.));
#87550=CARTESIAN_POINT('Ctrl Pts',(45.4723586351267,12.3369735386201,20.));
#87551=CARTESIAN_POINT('Ctrl Pts',(45.4781078086095,12.3043292629445,0.));
#87552=CARTESIAN_POINT('Ctrl Pts',(45.4781078086095,12.3043292629445,20.));
#87553=CARTESIAN_POINT('Ctrl Pts',(45.483833914657,12.2716820666929,0.));
#87554=CARTESIAN_POINT('Ctrl Pts',(45.483833914657,12.2716820666929,20.));
#87555=CARTESIAN_POINT('Ctrl Pts',(45.4895369513189,12.2390319660445,0.));
#87556=CARTESIAN_POINT('Ctrl Pts',(45.4895369513189,12.2390319660445,20.));
#87557=CARTESIAN_POINT('Ctrl Pts',(45.4952169166561,12.2063789771801,0.));
#87558=CARTESIAN_POINT('Ctrl Pts',(45.4952169166561,12.2063789771801,20.));
#87559=CARTESIAN_POINT('Ctrl Pts',(45.5008738087416,12.1737231162825,0.));
#87560=CARTESIAN_POINT('Ctrl Pts',(45.5008738087416,12.1737231162825,20.));
#87561=CARTESIAN_POINT('Ctrl Pts',(45.5065076256599,12.1410643995363,0.));
#87562=CARTESIAN_POINT('Ctrl Pts',(45.5065076256599,12.1410643995363,20.));
#87563=CARTESIAN_POINT('Ctrl Pts',(45.5121183655068,12.1084028431278,0.));
#87564=CARTESIAN_POINT('Ctrl Pts',(45.5121183655068,12.1084028431278,20.));
#87565=CARTESIAN_POINT('Ctrl Pts',(45.5177060263888,12.0757384632451,0.));
#87566=CARTESIAN_POINT('Ctrl Pts',(45.5177060263888,12.0757384632451,20.));
#87567=CARTESIAN_POINT('Ctrl Pts',(45.5232706064237,12.0430712760779,0.));
#87568=CARTESIAN_POINT('Ctrl Pts',(45.5232706064237,12.0430712760779,20.));
#87569=CARTESIAN_POINT('Ctrl Pts',(45.5288121037394,12.0104012978174,0.));
#87570=CARTESIAN_POINT('Ctrl Pts',(45.5288121037394,12.0104012978174,20.));
#87571=CARTESIAN_POINT('Ctrl Pts',(45.5343305164759,11.9777285446569,0.));
#87572=CARTESIAN_POINT('Ctrl Pts',(45.5343305164759,11.9777285446569,20.));
#87573=CARTESIAN_POINT('Ctrl Pts',(45.5398258427844,11.9450530327911,0.));
#87574=CARTESIAN_POINT('Ctrl Pts',(45.5398258427844,11.9450530327911,20.));
#87575=CARTESIAN_POINT('Ctrl Pts',(45.5452980808284,11.9123747784165,0.));
#87576=CARTESIAN_POINT('Ctrl Pts',(45.5452980808284,11.9123747784165,20.));
#87577=CARTESIAN_POINT('Ctrl Pts',(45.5507472287824,11.8796937977314,0.));
#87578=CARTESIAN_POINT('Ctrl Pts',(45.5507472287824,11.8796937977314,20.));
#87579=CARTESIAN_POINT('Ctrl Pts',(45.5561732848327,11.8470101069358,0.));
#87580=CARTESIAN_POINT('Ctrl Pts',(45.5561732848327,11.8470101069358,20.));
#87581=CARTESIAN_POINT('Ctrl Pts',(45.5615762471761,11.8143237222317,0.));
#87582=CARTESIAN_POINT('Ctrl Pts',(45.5615762471761,11.8143237222317,20.));
#87583=CARTESIAN_POINT('Ctrl Pts',(45.5669561140206,11.7816346598227,0.));
#87584=CARTESIAN_POINT('Ctrl Pts',(45.5669561140206,11.7816346598227,20.));
#87585=CARTESIAN_POINT('Ctrl Pts',(45.5723128835857,11.748942935914,0.));
#87586=CARTESIAN_POINT('Ctrl Pts',(45.5723128835857,11.748942935914,20.));
#87587=CARTESIAN_POINT('Ctrl Pts',(45.5776465541021,11.7162485667124,0.));
#87588=CARTESIAN_POINT('Ctrl Pts',(45.5776465541021,11.7162485667124,20.));
#87589=CARTESIAN_POINT('Ctrl Pts',(45.5829571238122,11.6835515684258,0.));
#87590=CARTESIAN_POINT('Ctrl Pts',(45.5829571238122,11.6835515684258,20.));
#87591=CARTESIAN_POINT('Ctrl Pts',(45.5882445909695,11.6508519572639,0.));
#87592=CARTESIAN_POINT('Ctrl Pts',(45.5882445909695,11.6508519572639,20.));
#87593=CARTESIAN_POINT('Ctrl Pts',(45.5935089538387,11.6181497494382,0.));
#87594=CARTESIAN_POINT('Ctrl Pts',(45.5935089538387,11.6181497494382,20.));
#87595=CARTESIAN_POINT('Ctrl Pts',(45.598750210696,11.5854449611619,0.));
#87596=CARTESIAN_POINT('Ctrl Pts',(45.598750210696,11.5854449611619,20.));
#87597=CARTESIAN_POINT('Ctrl Pts',(45.6039683598295,11.5527376086502,0.));
#87598=CARTESIAN_POINT('Ctrl Pts',(45.6039683598295,11.5527376086502,20.));
#87599=CARTESIAN_POINT('Ctrl Pts',(45.6091633995383,11.5200277081201,0.));
#87600=CARTESIAN_POINT('Ctrl Pts',(45.6091633995383,11.5200277081201,20.));
#87601=CARTESIAN_POINT('Ctrl Pts',(45.6143353281323,11.4873152757897,0.));
#87602=CARTESIAN_POINT('Ctrl Pts',(45.6143353281323,11.4873152757897,20.));
#87603=CARTESIAN_POINT('Ctrl Pts',(45.6194841439321,11.4546003278786,0.));
#87604=CARTESIAN_POINT('Ctrl Pts',(45.6194841439321,11.4546003278786,20.));
#87605=CARTESIAN_POINT('Ctrl Pts',(45.6246098452703,11.421882880608,0.));
#87606=CARTESIAN_POINT('Ctrl Pts',(45.6246098452703,11.421882880608,20.));
#87607=CARTESIAN_POINT('Ctrl Pts',(45.6297124304911,11.3891629502006,0.));
#87608=CARTESIAN_POINT('Ctrl Pts',(45.6297124304911,11.3891629502006,20.));
#87609=CARTESIAN_POINT('Ctrl Pts',(45.6347918979506,11.3564405528809,0.));
#87610=CARTESIAN_POINT('Ctrl Pts',(45.6347918979506,11.3564405528809,20.));
#87611=CARTESIAN_POINT('Ctrl Pts',(45.6398482460165,11.3237157048751,0.));
#87612=CARTESIAN_POINT('Ctrl Pts',(45.6398482460165,11.3237157048751,20.));
#87613=CARTESIAN_POINT('Ctrl Pts',(45.6448814730676,11.290988422411,0.));
#87614=CARTESIAN_POINT('Ctrl Pts',(45.6448814730676,11.290988422411,20.));
#87615=CARTESIAN_POINT('Ctrl Pts',(45.6498915774933,11.2582587217178,0.));
#87616=CARTESIAN_POINT('Ctrl Pts',(45.6498915774933,11.2582587217178,20.));
#87617=CARTESIAN_POINT('Ctrl Pts',(45.6548785576938,11.2255266190259,0.));
#87618=CARTESIAN_POINT('Ctrl Pts',(45.6548785576938,11.2255266190259,20.));
#87619=CARTESIAN_POINT('Ctrl Pts',(45.6598424120808,11.1927921305675,0.));
#87620=CARTESIAN_POINT('Ctrl Pts',(45.6598424120808,11.1927921305675,20.));
#87621=CARTESIAN_POINT('Ctrl Pts',(45.6647831390778,11.1600552725764,0.));
#87622=CARTESIAN_POINT('Ctrl Pts',(45.6647831390778,11.1600552725764,20.));
#87623=CARTESIAN_POINT('Ctrl Pts',(45.6697007371202,11.1273160612881,0.));
#87624=CARTESIAN_POINT('Ctrl Pts',(45.6697007371202,11.1273160612881,20.));
#87625=CARTESIAN_POINT('Ctrl Pts',(45.6745952046549,11.0945745129393,0.));
#87626=CARTESIAN_POINT('Ctrl Pts',(45.6745952046549,11.0945745129393,20.));
#87627=CARTESIAN_POINT('Ctrl Pts',(45.6794665401395,11.0618306437685,0.));
#87628=CARTESIAN_POINT('Ctrl Pts',(45.6794665401395,11.0618306437685,20.));
#87629=CARTESIAN_POINT('Ctrl Pts',(45.684314742043,11.0290844700154,0.));
#87630=CARTESIAN_POINT('Ctrl Pts',(45.684314742043,11.0290844700154,20.));
#87631=CARTESIAN_POINT('Ctrl Pts',(45.6891398088456,10.9963360079212,0.));
#87632=CARTESIAN_POINT('Ctrl Pts',(45.6891398088456,10.9963360079212,20.));
#87633=CARTESIAN_POINT('Ctrl Pts',(45.6939417390393,10.9635852737287,0.));
#87634=CARTESIAN_POINT('Ctrl Pts',(45.6939417390393,10.9635852737287,20.));
#87635=CARTESIAN_POINT('Ctrl Pts',(45.698720531127,10.930832283682,0.));
#87636=CARTESIAN_POINT('Ctrl Pts',(45.698720531127,10.930832283682,20.));
#87637=CARTESIAN_POINT('Ctrl Pts',(45.7034761836229,10.898077054027,0.));
#87638=CARTESIAN_POINT('Ctrl Pts',(45.7034761836229,10.898077054027,20.));
#87639=CARTESIAN_POINT('Ctrl Pts',(45.7082086950532,10.8653196010107,0.));
#87640=CARTESIAN_POINT('Ctrl Pts',(45.7082086950532,10.8653196010107,20.));
#87641=CARTESIAN_POINT('Ctrl Pts',(45.7129180639558,10.832559940882,0.));
#87642=CARTESIAN_POINT('Ctrl Pts',(45.7129180639558,10.832559940882,20.));
#87643=CARTESIAN_POINT('Ctrl Pts',(45.7176042888794,10.7997980898913,0.));
#87644=CARTESIAN_POINT('Ctrl Pts',(45.7176042888794,10.7997980898913,20.));
#87645=CARTESIAN_POINT('Ctrl Pts',(45.7222673683833,10.7670340642896,0.));
#87646=CARTESIAN_POINT('Ctrl Pts',(45.7222673683833,10.7670340642896,20.));
#87647=CARTESIAN_POINT('Ctrl Pts',(45.7269073010391,10.73426788033,0.));
#87648=CARTESIAN_POINT('Ctrl Pts',(45.7269073010391,10.73426788033,20.));
#87649=CARTESIAN_POINT('Ctrl Pts',(45.7315240854293,10.7014995542666,0.));
#87650=CARTESIAN_POINT('Ctrl Pts',(45.7315240854293,10.7014995542666,20.));
#87651=CARTESIAN_POINT('Ctrl Pts',(45.7361177201484,10.6687291023553,0.));
#87652=CARTESIAN_POINT('Ctrl Pts',(45.7361177201484,10.6687291023553,20.));
#87653=CARTESIAN_POINT('Ctrl Pts',(45.7406882038015,10.6359565408533,0.));
#87654=CARTESIAN_POINT('Ctrl Pts',(45.7406882038015,10.6359565408533,20.));
#87655=CARTESIAN_POINT('Ctrl Pts',(45.745235535006,10.6031818860194,0.));
#87656=CARTESIAN_POINT('Ctrl Pts',(45.745235535006,10.6031818860194,20.));
#87657=CARTESIAN_POINT('Ctrl Pts',(45.7497597123901,10.5704051541135,0.));
#87658=CARTESIAN_POINT('Ctrl Pts',(45.7497597123901,10.5704051541135,20.));
#87659=CARTESIAN_POINT('Ctrl Pts',(45.7542607345937,10.5376263613969,0.));
#87660=CARTESIAN_POINT('Ctrl Pts',(45.7542607345937,10.5376263613969,20.));
#87661=CARTESIAN_POINT('Ctrl Pts',(45.7587386002674,10.504845524132,0.));
#87662=CARTESIAN_POINT('Ctrl Pts',(45.7587386002674,10.504845524132,20.));
#87663=CARTESIAN_POINT('Ctrl Pts',(45.7631933080735,10.4720626585828,0.));
#87664=CARTESIAN_POINT('Ctrl Pts',(45.7631933080735,10.4720626585828,20.));
#87665=CARTESIAN_POINT('Ctrl Pts',(45.7676248566855,10.4392777810149,0.));
#87666=CARTESIAN_POINT('Ctrl Pts',(45.7676248566855,10.4392777810149,20.));
#87667=CARTESIAN_POINT('Ctrl Pts',(45.772033244789,10.406490907695,0.));
#87668=CARTESIAN_POINT('Ctrl Pts',(45.772033244789,10.406490907695,20.));
#87669=CARTESIAN_POINT('Ctrl Pts',(45.7764184710811,10.3737020548914,0.));
#87670=CARTESIAN_POINT('Ctrl Pts',(45.7764184710811,10.3737020548914,20.));
#87671=CARTESIAN_POINT('Ctrl Pts',(45.7807805342697,10.3409112388736,0.));
#87672=CARTESIAN_POINT('Ctrl Pts',(45.7807805342697,10.3409112388736,20.));
#87673=CARTESIAN_POINT('Ctrl Pts',(45.7851194330743,10.3081184759123,0.));
#87674=CARTESIAN_POINT('Ctrl Pts',(45.7851194330743,10.3081184759123,20.));
#87675=CARTESIAN_POINT('Ctrl Pts',(45.7894351662253,10.2753237822796,0.));
#87676=CARTESIAN_POINT('Ctrl Pts',(45.7894351662253,10.2753237822796,20.));
#87677=CARTESIAN_POINT('Ctrl Pts',(45.7937277324642,10.2425271742485,0.));
#87678=CARTESIAN_POINT('Ctrl Pts',(45.7937277324642,10.2425271742485,20.));
#87679=CARTESIAN_POINT('Ctrl Pts',(45.7979971305449,10.2097286680937,0.));
#87680=CARTESIAN_POINT('Ctrl Pts',(45.7979971305449,10.2097286680937,20.));
#87681=CARTESIAN_POINT('Ctrl Pts',(45.8022433592327,10.1769282800914,0.));
#87682=CARTESIAN_POINT('Ctrl Pts',(45.8022433592327,10.1769282800914,20.));
#87683=CARTESIAN_POINT('Ctrl Pts',(45.8064664173048,10.1441260265191,0.));
#87684=CARTESIAN_POINT('Ctrl Pts',(45.8064664173048,10.1441260265191,20.));
#87685=CARTESIAN_POINT('Ctrl Pts',(45.8106663035491,10.1113219236554,0.));
#87686=CARTESIAN_POINT('Ctrl Pts',(45.8106663035491,10.1113219236554,20.));
#87687=CARTESIAN_POINT('Ctrl Pts',(45.8148430167647,10.0785159877801,0.));
#87688=CARTESIAN_POINT('Ctrl Pts',(45.8148430167647,10.0785159877801,20.));
#87689=CARTESIAN_POINT('Ctrl Pts',(45.8189965557614,10.0457082351741,0.));
#87690=CARTESIAN_POINT('Ctrl Pts',(45.8189965557614,10.0457082351741,20.));
#87691=CARTESIAN_POINT('Ctrl Pts',(45.8231269193611,10.0128986821194,0.));
#87692=CARTESIAN_POINT('Ctrl Pts',(45.8231269193611,10.0128986821194,20.));
#87693=CARTESIAN_POINT('Ctrl Pts',(45.8272341063969,9.98008734489948,0.));
#87694=CARTESIAN_POINT('Ctrl Pts',(45.8272341063969,9.98008734489948,20.));
#87695=CARTESIAN_POINT('Ctrl Pts',(45.8313181157134,9.94727423979906,0.));
#87696=CARTESIAN_POINT('Ctrl Pts',(45.8313181157134,9.94727423979906,20.));
#87697=CARTESIAN_POINT('Ctrl Pts',(45.8353789461673,9.91445938310424,0.));
#87698=CARTESIAN_POINT('Ctrl Pts',(45.8353789461673,9.91445938310424,20.));
#87699=CARTESIAN_POINT('Ctrl Pts',(45.8394165966264,9.88164279110241,0.));
#87700=CARTESIAN_POINT('Ctrl Pts',(45.8394165966264,9.88164279110241,20.));
#87701=CARTESIAN_POINT('Ctrl Pts',(45.84343106597,9.84882448008225,0.));
#87702=CARTESIAN_POINT('Ctrl Pts',(45.84343106597,9.84882448008225,20.));
#87703=CARTESIAN_POINT('Ctrl Pts',(45.8474223530896,9.81600446633368,0.));
#87704=CARTESIAN_POINT('Ctrl Pts',(45.8474223530896,9.81600446633368,20.));
#87705=CARTESIAN_POINT('Ctrl Pts',(45.8513904568872,9.78318276614762,0.));
#87706=CARTESIAN_POINT('Ctrl Pts',(45.8513904568872,9.78318276614762,20.));
#87707=CARTESIAN_POINT('Ctrl Pts',(45.8553353762765,9.75035939581619,0.));
#87708=CARTESIAN_POINT('Ctrl Pts',(45.8553353762765,9.75035939581619,20.));
#87709=CARTESIAN_POINT('Ctrl Pts',(45.8592571101812,9.71753437163221,0.));
#87710=CARTESIAN_POINT('Ctrl Pts',(45.8592571101812,9.71753437163221,20.));
#87711=CARTESIAN_POINT('Ctrl Pts',(45.8631556575366,9.68470770988976,0.));
#87712=CARTESIAN_POINT('Ctrl Pts',(45.8631556575366,9.68470770988976,20.));
#87713=CARTESIAN_POINT('Ctrl Pts',(45.8670310172895,9.65187942688401,0.));
#87714=CARTESIAN_POINT('Ctrl Pts',(45.8670310172895,9.65187942688401,20.));
#87715=CARTESIAN_POINT('Ctrl Pts',(45.870883188399,9.61904953891161,0.));
#87716=CARTESIAN_POINT('Ctrl Pts',(45.870883188399,9.61904953891161,20.));
#87717=CARTESIAN_POINT('Ctrl Pts',(45.8747121698355,9.58621806227057,0.));
#87718=CARTESIAN_POINT('Ctrl Pts',(45.8747121698355,9.58621806227057,20.));
#87719=CARTESIAN_POINT('Ctrl Pts',(45.8785179605829,9.55338501326048,0.));
#87720=CARTESIAN_POINT('Ctrl Pts',(45.8785179605829,9.55338501326048,20.));
#87721=CARTESIAN_POINT('Ctrl Pts',(45.882300559635,9.52055040818185,0.));
#87722=CARTESIAN_POINT('Ctrl Pts',(45.882300559635,9.52055040818185,20.));
#87723=CARTESIAN_POINT('Ctrl Pts',(45.8860599659967,9.4877142633361,0.));
#87724=CARTESIAN_POINT('Ctrl Pts',(45.8860599659967,9.4877142633361,20.));
#87725=CARTESIAN_POINT('Ctrl Pts',(45.8897961786838,9.45487659502548,0.));
#87726=CARTESIAN_POINT('Ctrl Pts',(45.8897961786838,9.45487659502548,20.));
#87727=CARTESIAN_POINT('Ctrl Pts',(45.8935091967241,9.42203741955325,0.));
#87728=CARTESIAN_POINT('Ctrl Pts',(45.8935091967241,9.42203741955325,20.));
#87729=CARTESIAN_POINT('Ctrl Pts',(45.8971990191563,9.38919675322381,0.));
#87730=CARTESIAN_POINT('Ctrl Pts',(45.8971990191563,9.38919675322381,20.));
#87731=CARTESIAN_POINT('Ctrl Pts',(45.90086564503,9.35635461234246,0.));
#87732=CARTESIAN_POINT('Ctrl Pts',(45.90086564503,9.35635461234246,20.));
#87733=CARTESIAN_POINT('Ctrl Pts',(45.9045090734063,9.3235110132158,0.));
#87734=CARTESIAN_POINT('Ctrl Pts',(45.9045090734063,9.3235110132158,20.));
#87735=CARTESIAN_POINT('Ctrl Pts',(45.9081293033576,9.29066597215163,0.));
#87736=CARTESIAN_POINT('Ctrl Pts',(45.9081293033576,9.29066597215163,20.));
#87737=CARTESIAN_POINT('Ctrl Pts',(45.9117263339694,9.25781950545902,0.));
#87738=CARTESIAN_POINT('Ctrl Pts',(45.9117263339694,9.25781950545902,20.));
#87739=CARTESIAN_POINT('Ctrl Pts',(45.9153001643391,9.22497162944821,0.));
#87740=CARTESIAN_POINT('Ctrl Pts',(45.9153001643391,9.22497162944821,20.));
#87741=CARTESIAN_POINT('Ctrl Pts',(45.9188507935764,9.19212236043074,0.));
#87742=CARTESIAN_POINT('Ctrl Pts',(45.9188507935764,9.19212236043074,20.));
#87743=CARTESIAN_POINT('Ctrl Pts',(45.9223782208015,9.15927171471892,0.));
#87744=CARTESIAN_POINT('Ctrl Pts',(45.9223782208015,9.15927171471892,20.));
#87745=CARTESIAN_POINT('Ctrl Pts',(45.9258824451441,9.12641970862567,0.));
#87746=CARTESIAN_POINT('Ctrl Pts',(45.9258824451441,9.12641970862567,20.));
#87747=CARTESIAN_POINT('Ctrl Pts',(45.9293634657451,9.09356635846486,0.));
#87748=CARTESIAN_POINT('Ctrl Pts',(45.9293634657451,9.09356635846486,20.));
#87749=CARTESIAN_POINT('Ctrl Pts',(45.9328212817567,9.06071168055121,0.));
#87750=CARTESIAN_POINT('Ctrl Pts',(45.9328212817567,9.06071168055121,20.));
#87751=CARTESIAN_POINT('Ctrl Pts',(45.9362558923428,9.02785569120062,0.));
#87752=CARTESIAN_POINT('Ctrl Pts',(45.9362558923428,9.02785569120062,20.));
#87753=CARTESIAN_POINT('Ctrl Pts',(45.939667296681,8.99499840673047,0.));
#87754=CARTESIAN_POINT('Ctrl Pts',(45.939667296681,8.99499840673047,20.));
#87755=CARTESIAN_POINT('Ctrl Pts',(45.9430554939595,8.96213984345905,0.));
#87756=CARTESIAN_POINT('Ctrl Pts',(45.9430554939595,8.96213984345905,20.));
#87757=CARTESIAN_POINT('Ctrl Pts',(45.9464204833787,8.92928001770576,0.));
#87758=CARTESIAN_POINT('Ctrl Pts',(45.9464204833787,8.92928001770576,20.));
#87759=CARTESIAN_POINT('Ctrl Pts',(45.9497622641496,8.89641894579083,0.));
#87760=CARTESIAN_POINT('Ctrl Pts',(45.9497622641496,8.89641894579083,20.));
#87761=CARTESIAN_POINT('Ctrl Pts',(45.9530808354938,8.86355664403535,0.));
#87762=CARTESIAN_POINT('Ctrl Pts',(45.9530808354938,8.86355664403535,20.));
#87763=CARTESIAN_POINT('Ctrl Pts',(45.9563761966444,8.83069312876128,0.));
#87764=CARTESIAN_POINT('Ctrl Pts',(45.9563761966444,8.83069312876128,20.));
#87765=CARTESIAN_POINT('Ctrl Pts',(45.9596483468462,8.79782841629148,0.));
#87766=CARTESIAN_POINT('Ctrl Pts',(45.9596483468462,8.79782841629148,20.));
#87767=CARTESIAN_POINT('Ctrl Pts',(45.9628972853566,8.76496252295002,0.));
#87768=CARTESIAN_POINT('Ctrl Pts',(45.9628972853566,8.76496252295002,20.));
#87769=CARTESIAN_POINT('Ctrl Pts',(45.9661230114446,8.732095465062,0.));
#87770=CARTESIAN_POINT('Ctrl Pts',(45.9661230114446,8.732095465062,20.));
#87771=CARTESIAN_POINT('Ctrl Pts',(45.9693255243897,8.69922725895329,0.));
#87772=CARTESIAN_POINT('Ctrl Pts',(45.9693255243897,8.69922725895329,20.));
#87773=CARTESIAN_POINT('Ctrl Pts',(45.9725048234817,8.66635792095044,0.));
#87774=CARTESIAN_POINT('Ctrl Pts',(45.9725048234817,8.66635792095044,20.));
#87775=CARTESIAN_POINT('Ctrl Pts',(45.9756609080225,8.633487467381,0.));
#87776=CARTESIAN_POINT('Ctrl Pts',(45.9756609080225,8.633487467381,20.));
#87777=CARTESIAN_POINT('Ctrl Pts',(45.9787937773254,8.6006159145734,0.));
#87778=CARTESIAN_POINT('Ctrl Pts',(45.9787937773254,8.6006159145734,20.));
#87779=CARTESIAN_POINT('Ctrl Pts',(45.9819034307166,8.56774327885726,0.));
#87780=CARTESIAN_POINT('Ctrl Pts',(45.9819034307166,8.56774327885726,20.));
#87781=CARTESIAN_POINT('Ctrl Pts',(45.9849898675351,8.53486957656348,0.));
#87782=CARTESIAN_POINT('Ctrl Pts',(45.9849898675351,8.53486957656348,20.));
#87783=CARTESIAN_POINT('Ctrl Pts',(45.9880530871298,8.50199482402355,0.));
#87784=CARTESIAN_POINT('Ctrl Pts',(45.9880530871298,8.50199482402355,20.));
#87785=CARTESIAN_POINT('Ctrl Pts',(45.991093088861,8.46911903756974,0.));
#87786=CARTESIAN_POINT('Ctrl Pts',(45.991093088861,8.46911903756974,20.));
#87787=CARTESIAN_POINT('Ctrl Pts',(45.9941098720982,8.43624223353472,0.));
#87788=CARTESIAN_POINT('Ctrl Pts',(45.9941098720982,8.43624223353472,20.));
#87789=CARTESIAN_POINT('Ctrl Pts',(45.9971034362229,8.403364428252,0.));
#87790=CARTESIAN_POINT('Ctrl Pts',(45.9971034362229,8.403364428252,20.));
#87791=CARTESIAN_POINT('Ctrl Pts',(46.000073780629,8.37048563805606,0.));
#87792=CARTESIAN_POINT('Ctrl Pts',(46.000073780629,8.37048563805606,20.));
#87793=CARTESIAN_POINT('Ctrl Pts',(46.0030209047226,8.33760587928254,0.));
#87794=CARTESIAN_POINT('Ctrl Pts',(46.0030209047226,8.33760587928254,20.));
#87795=CARTESIAN_POINT('Ctrl Pts',(46.0059448079215,8.30472516826798,0.));
#87796=CARTESIAN_POINT('Ctrl Pts',(46.0059448079215,8.30472516826798,20.));
#87797=CARTESIAN_POINT('Ctrl Pts',(46.0088454896554,8.27184352134995,0.));
#87798=CARTESIAN_POINT('Ctrl Pts',(46.0088454896554,8.27184352134995,20.));
#87799=CARTESIAN_POINT('Ctrl Pts',(46.0117229493647,8.2389609548667,0.));
#87800=CARTESIAN_POINT('Ctrl Pts',(46.0117229493647,8.2389609548667,20.));
#87801=CARTESIAN_POINT('Ctrl Pts',(46.0145771865005,8.20607748515696,0.));
#87802=CARTESIAN_POINT('Ctrl Pts',(46.0145771865005,8.20607748515696,20.));
#87803=CARTESIAN_POINT('Ctrl Pts',(46.0174082005262,8.17319312856043,0.));
#87804=CARTESIAN_POINT('Ctrl Pts',(46.0174082005262,8.17319312856043,20.));
#87805=CARTESIAN_POINT('Ctrl Pts',(46.0202159909161,8.1403079014174,0.));
#87806=CARTESIAN_POINT('Ctrl Pts',(46.0202159909161,8.1403079014174,20.));
#87807=CARTESIAN_POINT('Ctrl Pts',(46.0230005571558,8.10742182006901,0.));
#87808=CARTESIAN_POINT('Ctrl Pts',(46.0230005571558,8.10742182006901,20.));
#87809=CARTESIAN_POINT('Ctrl Pts',(46.025761898743,8.07453490085737,0.));
#87810=CARTESIAN_POINT('Ctrl Pts',(46.025761898743,8.07453490085737,20.));
#87811=CARTESIAN_POINT('Ctrl Pts',(46.0285000151874,8.04164716012546,0.));
#87812=CARTESIAN_POINT('Ctrl Pts',(46.0285000151874,8.04164716012546,20.));
#87813=CARTESIAN_POINT('Ctrl Pts',(46.0312149060105,8.00875861421695,0.));
#87814=CARTESIAN_POINT('Ctrl Pts',(46.0312149060105,8.00875861421695,20.));
#87815=CARTESIAN_POINT('Ctrl Pts',(46.0339065707442,7.97586927947621,0.));
#87816=CARTESIAN_POINT('Ctrl Pts',(46.0339065707442,7.97586927947621,20.));
#87817=CARTESIAN_POINT('Ctrl Pts',(46.0365750089318,7.94297917224816,0.));
#87818=CARTESIAN_POINT('Ctrl Pts',(46.0365750089318,7.94297917224816,20.));
#87819=CARTESIAN_POINT('Ctrl Pts',(46.0392202201278,7.91008830887856,0.));
#87820=CARTESIAN_POINT('Ctrl Pts',(46.0392202201278,7.91008830887856,20.));
#87821=CARTESIAN_POINT('Ctrl Pts',(46.0418422038989,7.87719670571401,0.));
#87822=CARTESIAN_POINT('Ctrl Pts',(46.0418422038989,7.87719670571401,20.));
#87823=CARTESIAN_POINT('Ctrl Pts',(46.0444409598224,7.84430437910167,0.));
#87824=CARTESIAN_POINT('Ctrl Pts',(46.0444409598224,7.84430437910167,20.));
#87825=CARTESIAN_POINT('Ctrl Pts',(46.0470164874882,7.81141134538955,0.));
#87826=CARTESIAN_POINT('Ctrl Pts',(46.0470164874882,7.81141134538955,20.));
#87827=CARTESIAN_POINT('Ctrl Pts',(46.0495687864972,7.77851762092637,0.));
#87828=CARTESIAN_POINT('Ctrl Pts',(46.0495687864972,7.77851762092637,20.));
#87829=CARTESIAN_POINT('Ctrl Pts',(46.052097856463,7.74562322206168,0.));
#87830=CARTESIAN_POINT('Ctrl Pts',(46.052097856463,7.74562322206168,20.));
#87831=CARTESIAN_POINT('Ctrl Pts',(46.0546036970108,7.71272816514572,0.));
#87832=CARTESIAN_POINT('Ctrl Pts',(46.0546036970108,7.71272816514572,20.));
#87833=CARTESIAN_POINT('Ctrl Pts',(46.0570863077758,7.67983246652918,0.));
#87834=CARTESIAN_POINT('Ctrl Pts',(46.0570863077758,7.67983246652918,20.));
#87835=CARTESIAN_POINT('Ctrl Pts',(46.0595456884042,7.64693614256336,0.));
#87836=CARTESIAN_POINT('Ctrl Pts',(46.0595456884042,7.64693614256336,20.));
#87837=CARTESIAN_POINT('Ctrl Pts',(46.0619818385541,7.61403920960036,0.));
#87838=CARTESIAN_POINT('Ctrl Pts',(46.0619818385541,7.61403920960036,20.));
#87839=CARTESIAN_POINT('Ctrl Pts',(46.0643947578955,7.58114168399302,0.));
#87840=CARTESIAN_POINT('Ctrl Pts',(46.0643947578955,7.58114168399302,20.));
#87841=CARTESIAN_POINT('Ctrl Pts',(46.0667844461104,7.54824358209485,0.));
#87842=CARTESIAN_POINT('Ctrl Pts',(46.0667844461104,7.54824358209485,20.));
#87843=CARTESIAN_POINT('Ctrl Pts',(46.0691509028928,7.51534492025983,0.));
#87844=CARTESIAN_POINT('Ctrl Pts',(46.0691509028928,7.51534492025983,20.));
#87845=CARTESIAN_POINT('Ctrl Pts',(46.0714941279471,7.48244571484251,0.));
#87846=CARTESIAN_POINT('Ctrl Pts',(46.0714941279471,7.48244571484251,20.));
#87847=CARTESIAN_POINT('Ctrl Pts',(46.0738141209885,7.4495459821981,0.));
#87848=CARTESIAN_POINT('Ctrl Pts',(46.0738141209885,7.4495459821981,20.));
#87849=CARTESIAN_POINT('Ctrl Pts',(46.0761108817447,7.41664573868261,0.));
#87850=CARTESIAN_POINT('Ctrl Pts',(46.0761108817447,7.41664573868261,20.));
#87851=CARTESIAN_POINT('Ctrl Pts',(46.0783844099553,7.38374500065295,0.));
#87852=CARTESIAN_POINT('Ctrl Pts',(46.0783844099553,7.38374500065295,20.));
#87853=CARTESIAN_POINT('Ctrl Pts',(46.0806347053718,7.35084378446662,0.));
#87854=CARTESIAN_POINT('Ctrl Pts',(46.0806347053718,7.35084378446662,20.));
#87855=CARTESIAN_POINT('Ctrl Pts',(46.0828617677561,7.3179421064814,0.));
#87856=CARTESIAN_POINT('Ctrl Pts',(46.0828617677561,7.3179421064814,20.));
#87857=CARTESIAN_POINT('Ctrl Pts',(46.0850655968817,7.28503998305551,0.));
#87858=CARTESIAN_POINT('Ctrl Pts',(46.0850655968817,7.28503998305551,20.));
#87859=CARTESIAN_POINT('Ctrl Pts',(46.0872461925336,7.2521374305475,0.));
#87860=CARTESIAN_POINT('Ctrl Pts',(46.0872461925336,7.2521374305475,20.));
#87861=CARTESIAN_POINT('Ctrl Pts',(46.0894035545083,7.21923446531641,0.));
#87862=CARTESIAN_POINT('Ctrl Pts',(46.0894035545083,7.21923446531641,20.));
#87863=CARTESIAN_POINT('Ctrl Pts',(46.0915376826137,7.18633110372212,0.));
#87864=CARTESIAN_POINT('Ctrl Pts',(46.0915376826137,7.18633110372212,20.));
#87865=CARTESIAN_POINT('Ctrl Pts',(46.0936485766695,7.1534273621253,0.));
#87866=CARTESIAN_POINT('Ctrl Pts',(46.0936485766695,7.1534273621253,20.));
#87867=CARTESIAN_POINT('Ctrl Pts',(46.0957362365075,7.12052325688753,0.));
#87868=CARTESIAN_POINT('Ctrl Pts',(46.0957362365075,7.12052325688753,20.));
#87869=CARTESIAN_POINT('Ctrl Pts',(46.097800661971,7.08761880437094,0.));
#87870=CARTESIAN_POINT('Ctrl Pts',(46.097800661971,7.08761880437094,20.));
#87871=CARTESIAN_POINT('Ctrl Pts',(46.0998418529147,7.05471402093802,0.));
#87872=CARTESIAN_POINT('Ctrl Pts',(46.0998418529147,7.05471402093802,20.));
#87873=CARTESIAN_POINT('Ctrl Pts',(46.1018598092046,7.02180892295148,0.));
#87874=CARTESIAN_POINT('Ctrl Pts',(46.1018598092046,7.02180892295148,20.));
#87875=CARTESIAN_POINT('Ctrl Pts',(46.103854530718,6.98890352677439,0.));
#87876=CARTESIAN_POINT('Ctrl Pts',(46.103854530718,6.98890352677439,20.));
#87877=CARTESIAN_POINT('Ctrl Pts',(46.1058260173429,6.95599784877019,0.));
#87878=CARTESIAN_POINT('Ctrl Pts',(46.1058260173429,6.95599784877019,20.));
#87879=CARTESIAN_POINT('Ctrl Pts',(46.1077742689797,6.92309190530285,0.));
#87880=CARTESIAN_POINT('Ctrl Pts',(46.1077742689797,6.92309190530285,20.));
#87881=CARTESIAN_POINT('Ctrl Pts',(46.1096992855399,6.8901857127369,0.));
#87882=CARTESIAN_POINT('Ctrl Pts',(46.1096992855399,6.8901857127369,20.));
#87883=CARTESIAN_POINT('Ctrl Pts',(46.111601066948,6.85727928743788,0.));
#87884=CARTESIAN_POINT('Ctrl Pts',(46.111601066948,6.85727928743788,20.));
#87885=CARTESIAN_POINT('Ctrl Pts',(46.1134796131392,6.82437264577169,0.));
#87886=CARTESIAN_POINT('Ctrl Pts',(46.1134796131392,6.82437264577169,20.));
#87887=CARTESIAN_POINT('Ctrl Pts',(46.1153349240611,6.7914658041047,0.));
#87888=CARTESIAN_POINT('Ctrl Pts',(46.1153349240611,6.7914658041047,20.));
#87889=CARTESIAN_POINT('Ctrl Pts',(46.1171669996709,6.75855877880357,0.));
#87890=CARTESIAN_POINT('Ctrl Pts',(46.1171669996709,6.75855877880357,20.));
#87891=CARTESIAN_POINT('Ctrl Pts',(46.1189758399374,6.72565158623521,0.));
#87892=CARTESIAN_POINT('Ctrl Pts',(46.1189758399374,6.72565158623521,20.));
#87893=CARTESIAN_POINT('Ctrl Pts',(46.1207614448407,6.69274424276688,0.));
#87894=CARTESIAN_POINT('Ctrl Pts',(46.1207614448407,6.69274424276688,20.));
#87895=CARTESIAN_POINT('Ctrl Pts',(46.122523814374,6.65983676476652,0.));
#87896=CARTESIAN_POINT('Ctrl Pts',(46.122523814374,6.65983676476652,20.));
#87897=CARTESIAN_POINT('Ctrl Pts',(46.124262948542,6.62692916860258,0.));
#87898=CARTESIAN_POINT('Ctrl Pts',(46.124262948542,6.62692916860258,20.));
#87899=CARTESIAN_POINT('Ctrl Pts',(46.1259788473615,6.594021470644,0.));
#87900=CARTESIAN_POINT('Ctrl Pts',(46.1259788473615,6.594021470644,20.));
#87901=CARTESIAN_POINT('Ctrl Pts',(46.1276715108604,6.5611136872601,0.));
#87902=CARTESIAN_POINT('Ctrl Pts',(46.1276715108604,6.5611136872601,20.));
#87903=CARTESIAN_POINT('Ctrl Pts',(46.1293409390781,6.5282058348205,0.));
#87904=CARTESIAN_POINT('Ctrl Pts',(46.1293409390781,6.5282058348205,20.));
#87905=CARTESIAN_POINT('Ctrl Pts',(46.1309871320644,6.49529792969509,0.));
#87906=CARTESIAN_POINT('Ctrl Pts',(46.1309871320644,6.49529792969509,20.));
#87907=CARTESIAN_POINT('Ctrl Pts',(46.1326100898806,6.46238998825408,0.));
#87908=CARTESIAN_POINT('Ctrl Pts',(46.1326100898806,6.46238998825408,20.));
#87909=CARTESIAN_POINT('Ctrl Pts',(46.134209812599,6.42948202686814,0.));
#87910=CARTESIAN_POINT('Ctrl Pts',(46.134209812599,6.42948202686814,20.));
#87911=CARTESIAN_POINT('Ctrl Pts',(46.1357863003044,6.39657406190845,0.));
#87912=CARTESIAN_POINT('Ctrl Pts',(46.1357863003044,6.39657406190845,20.));
#87913=CARTESIAN_POINT('Ctrl Pts',(46.1373395530931,6.36366610974648,0.));
#87914=CARTESIAN_POINT('Ctrl Pts',(46.1373395530931,6.36366610974648,20.));
#87915=CARTESIAN_POINT('Ctrl Pts',(46.138869571074,6.3307581867542,0.));
#87916=CARTESIAN_POINT('Ctrl Pts',(46.138869571074,6.3307581867542,20.));
#87917=CARTESIAN_POINT('Ctrl Pts',(46.1403763543673,6.29785030930382,0.));
#87918=CARTESIAN_POINT('Ctrl Pts',(46.1403763543673,6.29785030930382,20.));
#87919=CARTESIAN_POINT('Ctrl Pts',(46.141859903105,6.26494249376778,0.));
#87920=CARTESIAN_POINT('Ctrl Pts',(46.141859903105,6.26494249376778,20.));
#87921=CARTESIAN_POINT('Ctrl Pts',(46.1433202174297,6.23203475651883,0.));
#87922=CARTESIAN_POINT('Ctrl Pts',(46.1433202174297,6.23203475651883,20.));
#87923=CARTESIAN_POINT('Ctrl Pts',(46.1447572974959,6.19912711393004,0.));
#87924=CARTESIAN_POINT('Ctrl Pts',(46.1447572974959,6.19912711393004,20.));
#87925=CARTESIAN_POINT('Ctrl Pts',(46.1461711434687,6.16621958237488,0.));
#87926=CARTESIAN_POINT('Ctrl Pts',(46.1461711434687,6.16621958237488,20.));
#87927=CARTESIAN_POINT('Ctrl Pts',(46.1475617555249,6.1333121782271,0.));
#87928=CARTESIAN_POINT('Ctrl Pts',(46.1475617555249,6.1333121782271,20.));
#87929=CARTESIAN_POINT('Ctrl Pts',(46.1489291338532,6.10040491786086,0.));
#87930=CARTESIAN_POINT('Ctrl Pts',(46.1489291338532,6.10040491786086,20.));
#87931=CARTESIAN_POINT('Ctrl Pts',(46.1502732786543,6.06749781765058,0.));
#87932=CARTESIAN_POINT('Ctrl Pts',(46.1502732786543,6.06749781765058,20.));
#87933=CARTESIAN_POINT('Ctrl Pts',(46.151594190141,6.03459089397104,0.));
#87934=CARTESIAN_POINT('Ctrl Pts',(46.151594190141,6.03459089397104,20.));
#87935=CARTESIAN_POINT('Ctrl Pts',(46.1528918685373,6.0016841631972,0.));
#87936=CARTESIAN_POINT('Ctrl Pts',(46.1528918685373,6.0016841631972,20.));
#87937=CARTESIAN_POINT('Ctrl Pts',(46.1541663140783,5.96877764170412,0.));
#87938=CARTESIAN_POINT('Ctrl Pts',(46.1541663140783,5.96877764170412,20.));
#87939=CARTESIAN_POINT('Ctrl Pts',(46.1554175270101,5.9358713458669,0.));
#87940=CARTESIAN_POINT('Ctrl Pts',(46.1554175270101,5.9358713458669,20.));
#87941=CARTESIAN_POINT('Ctrl Pts',(46.1566455075904,5.90296529206097,0.));
#87942=CARTESIAN_POINT('Ctrl Pts',(46.1566455075904,5.90296529206097,20.));
#87943=CARTESIAN_POINT('Ctrl Pts',(46.1578502560886,5.87005949666212,0.));
#87944=CARTESIAN_POINT('Ctrl Pts',(46.1578502560886,5.87005949666212,20.));
#87945=CARTESIAN_POINT('Ctrl Pts',(46.1590317727861,5.83715397604653,0.));
#87946=CARTESIAN_POINT('Ctrl Pts',(46.1590317727861,5.83715397604653,20.));
#87947=CARTESIAN_POINT('Ctrl Pts',(46.160190057976,5.80424874659071,0.));
#87948=CARTESIAN_POINT('Ctrl Pts',(46.160190057976,5.80424874659071,20.));
#87949=CARTESIAN_POINT('Ctrl Pts',(46.1613251119636,5.77134382467173,0.));
#87950=CARTESIAN_POINT('Ctrl Pts',(46.1613251119636,5.77134382467173,20.));
#87951=CARTESIAN_POINT('Ctrl Pts',(46.1624369350662,5.73843922666648,0.));
#87952=CARTESIAN_POINT('Ctrl Pts',(46.1624369350662,5.73843922666648,20.));
#87953=CARTESIAN_POINT('Ctrl Pts',(46.1635255276116,5.70553496895185,0.));
#87954=CARTESIAN_POINT('Ctrl Pts',(46.1635255276116,5.70553496895185,20.));
#87955=CARTESIAN_POINT('Ctrl Pts',(46.1645908899393,5.67263106790479,0.));
#87956=CARTESIAN_POINT('Ctrl Pts',(46.1645908899393,5.67263106790479,20.));
#87957=CARTESIAN_POINT('Ctrl Pts',(46.1656330223979,5.63972753990236,0.));
#87958=CARTESIAN_POINT('Ctrl Pts',(46.1656330223979,5.63972753990236,20.));
#87959=CARTESIAN_POINT('Ctrl Pts',(46.166651925349,5.60682440132182,0.));
#87960=CARTESIAN_POINT('Ctrl Pts',(46.166651925349,5.60682440132182,20.));
#87961=CARTESIAN_POINT('Ctrl Pts',(46.1676475991657,5.57392166854075,0.));
#87962=CARTESIAN_POINT('Ctrl Pts',(46.1676475991657,5.57392166854075,20.));
#87963=CARTESIAN_POINT('Ctrl Pts',(46.1686200442337,5.5410193579371,0.));
#87964=CARTESIAN_POINT('Ctrl Pts',(46.1686200442337,5.5410193579371,20.));
#87965=CARTESIAN_POINT('Ctrl Pts',(46.1695692609505,5.50811748588894,0.));
#87966=CARTESIAN_POINT('Ctrl Pts',(46.1695692609505,5.50811748588894,20.));
#87967=CARTESIAN_POINT('Ctrl Pts',(46.170495249726,5.4752160687746,0.));
#87968=CARTESIAN_POINT('Ctrl Pts',(46.170495249726,5.4752160687746,20.));
#87969=CARTESIAN_POINT('Ctrl Pts',(46.1713980109807,5.44231512297239,0.));
#87970=CARTESIAN_POINT('Ctrl Pts',(46.1713980109807,5.44231512297239,20.));
#87971=CARTESIAN_POINT('Ctrl Pts',(46.1722775451467,5.40941466486069,0.));
#87972=CARTESIAN_POINT('Ctrl Pts',(46.1722775451467,5.40941466486069,20.));
#87973=CARTESIAN_POINT('Ctrl Pts',(46.1731338526667,5.37651471081787,0.));
#87974=CARTESIAN_POINT('Ctrl Pts',(46.1731338526667,5.37651471081787,20.));
#87975=CARTESIAN_POINT('Ctrl Pts',(46.1739669339953,5.3436152772224,0.));
#87976=CARTESIAN_POINT('Ctrl Pts',(46.1739669339953,5.3436152772224,20.));
#87977=CARTESIAN_POINT('Ctrl Pts',(46.1747767895978,5.31071638045279,0.));
#87978=CARTESIAN_POINT('Ctrl Pts',(46.1747767895978,5.31071638045279,20.));
#87979=CARTESIAN_POINT('Ctrl Pts',(46.1755634199519,5.27781803688791,0.));
#87980=CARTESIAN_POINT('Ctrl Pts',(46.1755634199519,5.27781803688791,20.));
#87981=CARTESIAN_POINT('Ctrl Pts',(46.1763268255471,5.24492026290663,0.));
#87982=CARTESIAN_POINT('Ctrl Pts',(46.1763268255471,5.24492026290663,20.));
#87983=CARTESIAN_POINT('Ctrl Pts',(46.1770670068854,5.21202307488802,0.));
#87984=CARTESIAN_POINT('Ctrl Pts',(46.1770670068854,5.21202307488802,20.));
#87985=CARTESIAN_POINT('Ctrl Pts',(46.1777839644797,5.17912648921102,0.));
#87986=CARTESIAN_POINT('Ctrl Pts',(46.1777839644797,5.17912648921102,20.));
#87987=CARTESIAN_POINT('Ctrl Pts',(46.1784776988548,5.14623052225472,0.));
#87988=CARTESIAN_POINT('Ctrl Pts',(46.1784776988548,5.14623052225472,20.));
#87989=CARTESIAN_POINT('Ctrl Pts',(46.1791482105459,5.11333519039809,0.));
#87990=CARTESIAN_POINT('Ctrl Pts',(46.1791482105459,5.11333519039809,20.));
#87991=CARTESIAN_POINT('Ctrl Pts',(46.1797955000997,5.08044051002026,0.));
#87992=CARTESIAN_POINT('Ctrl Pts',(46.1797955000997,5.08044051002026,20.));
#87993=CARTESIAN_POINT('Ctrl Pts',(46.1804195680748,5.04754649750031,0.));
#87994=CARTESIAN_POINT('Ctrl Pts',(46.1804195680748,5.04754649750031,20.));
#87995=CARTESIAN_POINT('Ctrl Pts',(46.1810204150412,5.01465316921749,0.));
#87996=CARTESIAN_POINT('Ctrl Pts',(46.1810204150412,5.01465316921749,20.));
#87997=CARTESIAN_POINT('Ctrl Pts',(46.1815980415817,4.98176054155101,0.));
#87998=CARTESIAN_POINT('Ctrl Pts',(46.1815980415817,4.98176054155101,20.));
#87999=CARTESIAN_POINT('Ctrl Pts',(46.182152448291,4.94886863088032,0.));
#88000=CARTESIAN_POINT('Ctrl Pts',(46.182152448291,4.94886863088032,20.));
#88001=CARTESIAN_POINT('Ctrl Pts',(46.1826836357763,4.91597745358481,0.));
#88002=CARTESIAN_POINT('Ctrl Pts',(46.1826836357763,4.91597745358481,20.));
#88003=CARTESIAN_POINT('Ctrl Pts',(46.1831916046531,4.8830870260435,0.));
#88004=CARTESIAN_POINT('Ctrl Pts',(46.1831916046531,4.8830870260435,20.));
#88005=CARTESIAN_POINT('Ctrl Pts',(46.1836763555496,4.85019736463544,0.));
#88006=CARTESIAN_POINT('Ctrl Pts',(46.1836763555496,4.85019736463544,20.));
#88007=CARTESIAN_POINT('Ctrl Pts',(46.1841378891039,4.81730848573954,0.));
#88008=CARTESIAN_POINT('Ctrl Pts',(46.1841378891039,4.81730848573954,20.));
#88009=CARTESIAN_POINT('Ctrl Pts',(46.1845762059678,4.78442040573515,0.));
#88010=CARTESIAN_POINT('Ctrl Pts',(46.1845762059678,4.78442040573515,20.));
#88011=CARTESIAN_POINT('Ctrl Pts',(46.1849913068043,4.75153314100161,0.));
#88012=CARTESIAN_POINT('Ctrl Pts',(46.1849913068043,4.75153314100161,20.));
#88013=CARTESIAN_POINT('Ctrl Pts',(46.1853831922891,4.71864670791826,0.));
#88014=CARTESIAN_POINT('Ctrl Pts',(46.1853831922891,4.71864670791826,20.));
#88015=CARTESIAN_POINT('Ctrl Pts',(46.1857518631086,4.68576112286394,0.));
#88016=CARTESIAN_POINT('Ctrl Pts',(46.1857518631086,4.68576112286394,20.));
#88017=CARTESIAN_POINT('Ctrl Pts',(46.1860973199616,4.65287640221748,0.));
#88018=CARTESIAN_POINT('Ctrl Pts',(46.1860973199616,4.65287640221748,20.));
#88019=CARTESIAN_POINT('Ctrl Pts',(46.1864195635571,4.61999256235741,0.));
#88020=CARTESIAN_POINT('Ctrl Pts',(46.1864195635571,4.61999256235741,20.));
#88021=CARTESIAN_POINT('Ctrl Pts',(46.1867185946155,4.58710961966233,0.));
#88022=CARTESIAN_POINT('Ctrl Pts',(46.1867185946155,4.58710961966233,20.));
#88023=CARTESIAN_POINT('Ctrl Pts',(46.1869944138693,4.55422759051101,0.));
#88024=CARTESIAN_POINT('Ctrl Pts',(46.1869944138693,4.55422759051101,20.));
#88025=CARTESIAN_POINT('Ctrl Pts',(46.1872470220627,4.52134649128218,0.));
#88026=CARTESIAN_POINT('Ctrl Pts',(46.1872470220627,4.52134649128218,20.));
#88027=CARTESIAN_POINT('Ctrl Pts',(46.1874764199521,4.48846633835459,0.));
#88028=CARTESIAN_POINT('Ctrl Pts',(46.1874764199521,4.48846633835459,20.));
#88029=CARTESIAN_POINT('Ctrl Pts',(46.1876826083051,4.45558714810681,0.));
#88030=CARTESIAN_POINT('Ctrl Pts',(46.1876826083051,4.45558714810681,20.));
#88031=CARTESIAN_POINT('Ctrl Pts',(46.1878655879008,4.42270893691724,0.));
#88032=CARTESIAN_POINT('Ctrl Pts',(46.1878655879008,4.42270893691724,20.));
#88033=CARTESIAN_POINT('Ctrl Pts',(46.1880253595296,4.38983172116389,0.));
#88034=CARTESIAN_POINT('Ctrl Pts',(46.1880253595296,4.38983172116389,20.));
#88035=CARTESIAN_POINT('Ctrl Pts',(46.1881619239926,4.35695551722447,0.));
#88036=CARTESIAN_POINT('Ctrl Pts',(46.1881619239926,4.35695551722447,20.));
#88037=CARTESIAN_POINT('Ctrl Pts',(46.1882752821036,4.32408034147655,0.));
#88038=CARTESIAN_POINT('Ctrl Pts',(46.1882752821036,4.32408034147655,20.));
#88039=CARTESIAN_POINT('Ctrl Pts',(46.1883654346888,4.29120621029777,0.));
#88040=CARTESIAN_POINT('Ctrl Pts',(46.1883654346888,4.29120621029777,20.));
#88041=CARTESIAN_POINT('Ctrl Pts',(46.1884323825857,4.25833314006578,0.));
#88042=CARTESIAN_POINT('Ctrl Pts',(46.1884323825857,4.25833314006578,20.));
#88043=CARTESIAN_POINT('Ctrl Pts',(46.1884761266433,4.22546114715825,0.));
#88044=CARTESIAN_POINT('Ctrl Pts',(46.1884761266433,4.22546114715825,20.));
#88045=CARTESIAN_POINT('Ctrl Pts',(46.1884966677209,4.19259024795239,0.));
#88046=CARTESIAN_POINT('Ctrl Pts',(46.1884966677209,4.19259024795239,20.));
#88047=CARTESIAN_POINT('Ctrl Pts',(46.1884940066895,4.15972045882509,0.));
#88048=CARTESIAN_POINT('Ctrl Pts',(46.1884940066895,4.15972045882509,20.));
#88049=CARTESIAN_POINT('Ctrl Pts',(46.1884681444317,4.12685179615294,0.));
#88050=CARTESIAN_POINT('Ctrl Pts',(46.1884681444317,4.12685179615294,20.));
#88051=CARTESIAN_POINT('Ctrl Pts',(46.188419081843,4.09398427631255,0.));
#88052=CARTESIAN_POINT('Ctrl Pts',(46.188419081843,4.09398427631255,20.));
#88053=CARTESIAN_POINT('Ctrl Pts',(46.18834681983,4.06111791568023,0.));
#88054=CARTESIAN_POINT('Ctrl Pts',(46.18834681983,4.06111791568023,20.));
#88055=CARTESIAN_POINT('Ctrl Pts',(46.1882513593113,4.02825273063218,0.));
#88056=CARTESIAN_POINT('Ctrl Pts',(46.1882513593113,4.02825273063218,20.));
#88057=CARTESIAN_POINT('Ctrl Pts',(46.1881327012171,3.99538873754443,0.));
#88058=CARTESIAN_POINT('Ctrl Pts',(46.1881327012171,3.99538873754443,20.));
#88059=CARTESIAN_POINT('Ctrl Pts',(46.1879908464881,3.96252595279274,0.));
#88060=CARTESIAN_POINT('Ctrl Pts',(46.1879908464881,3.96252595279274,20.));
#88061=CARTESIAN_POINT('Ctrl Pts',(46.1878257960766,3.92966439275257,0.));
#88062=CARTESIAN_POINT('Ctrl Pts',(46.1878257960766,3.92966439275257,20.));
#88063=CARTESIAN_POINT('Ctrl Pts',(46.1876375509469,3.89680407379914,0.));
#88064=CARTESIAN_POINT('Ctrl Pts',(46.1876375509469,3.89680407379914,20.));
#88065=CARTESIAN_POINT('Ctrl Pts',(46.1874261120751,3.86394501230744,0.));
#88066=CARTESIAN_POINT('Ctrl Pts',(46.1874261120751,3.86394501230744,20.));
#88067=CARTESIAN_POINT('Ctrl Pts',(46.1871914804492,3.83108722465199,0.));
#88068=CARTESIAN_POINT('Ctrl Pts',(46.1871914804492,3.83108722465199,20.));
#88069=CARTESIAN_POINT('Ctrl Pts',(46.1869336570686,3.79823072720685,0.));
#88070=CARTESIAN_POINT('Ctrl Pts',(46.1869336570686,3.79823072720685,20.));
#88071=CARTESIAN_POINT('Ctrl Pts',(46.1866526429445,3.76537553634596,0.));
#88072=CARTESIAN_POINT('Ctrl Pts',(46.1866526429445,3.76537553634596,20.));
#88073=CARTESIAN_POINT('Ctrl Pts',(46.1863484390996,3.73252166844328,0.));
#88074=CARTESIAN_POINT('Ctrl Pts',(46.1863484390996,3.73252166844328,20.));
#88075=CARTESIAN_POINT('Ctrl Pts',(46.1860210465678,3.69966913987253,0.));
#88076=CARTESIAN_POINT('Ctrl Pts',(46.1860210465678,3.69966913987253,20.));
#88077=CARTESIAN_POINT('Ctrl Pts',(46.185670466394,3.6668179670071,0.));
#88078=CARTESIAN_POINT('Ctrl Pts',(46.185670466394,3.6668179670071,20.));
#88079=CARTESIAN_POINT('Ctrl Pts',(46.1852966996347,3.6339681662199,0.));
#88080=CARTESIAN_POINT('Ctrl Pts',(46.1852966996347,3.6339681662199,20.));
#88081=CARTESIAN_POINT('Ctrl Pts',(46.1848997473582,3.60111975388339,0.));
#88082=CARTESIAN_POINT('Ctrl Pts',(46.1848997473582,3.60111975388339,20.));
#88083=CARTESIAN_POINT('Ctrl Pts',(46.1844796106451,3.56827274636958,0.));
#88084=CARTESIAN_POINT('Ctrl Pts',(46.1844796106451,3.56827274636958,20.));
#88085=CARTESIAN_POINT('Ctrl Pts',(46.1840362905882,3.53542716005025,0.));
#88086=CARTESIAN_POINT('Ctrl Pts',(46.1840362905882,3.53542716005025,20.));
#88087=CARTESIAN_POINT('Ctrl Pts',(46.1835697882921,3.50258301129689,0.));
#88088=CARTESIAN_POINT('Ctrl Pts',(46.1835697882921,3.50258301129689,20.));
#88089=CARTESIAN_POINT('Ctrl Pts',(46.1830801048722,3.4697403164807,0.));
#88090=CARTESIAN_POINT('Ctrl Pts',(46.1830801048722,3.4697403164807,20.));
#88091=CARTESIAN_POINT('Ctrl Pts',(46.1825672414553,3.43689909197262,0.));
#88092=CARTESIAN_POINT('Ctrl Pts',(46.1825672414553,3.43689909197262,20.));
#88093=CARTESIAN_POINT('Ctrl Pts',(46.1820311991793,3.40405935414302,0.));
#88094=CARTESIAN_POINT('Ctrl Pts',(46.1820311991793,3.40405935414302,20.));
#88095=CARTESIAN_POINT('Ctrl Pts',(46.1814719791936,3.37122111936182,0.));
#88096=CARTESIAN_POINT('Ctrl Pts',(46.1814719791936,3.37122111936182,20.));
#88097=CARTESIAN_POINT('Ctrl Pts',(46.1808895826591,3.33838440399861,0.));
#88098=CARTESIAN_POINT('Ctrl Pts',(46.1808895826591,3.33838440399861,20.));
#88099=CARTESIAN_POINT('Ctrl Pts',(46.1802840107495,3.30554922442266,0.));
#88100=CARTESIAN_POINT('Ctrl Pts',(46.1802840107495,3.30554922442266,20.));
#88101=CARTESIAN_POINT('Ctrl Pts',(46.1796552646498,3.27271559700279,0.));
#88102=CARTESIAN_POINT('Ctrl Pts',(46.1796552646498,3.27271559700279,20.));
#88103=CARTESIAN_POINT('Ctrl Pts',(46.1790033455572,3.23988353810748,0.));
#88104=CARTESIAN_POINT('Ctrl Pts',(46.1790033455572,3.23988353810748,20.));
#88105=CARTESIAN_POINT('Ctrl Pts',(46.1783282546796,3.20705306410471,0.));
#88106=CARTESIAN_POINT('Ctrl Pts',(46.1783282546796,3.20705306410471,20.));
#88107=CARTESIAN_POINT('Ctrl Pts',(46.1776299932363,3.17422419136187,0.));
#88108=CARTESIAN_POINT('Ctrl Pts',(46.1776299932363,3.17422419136187,20.));
#88109=CARTESIAN_POINT('Ctrl Pts',(46.1769085624582,3.14139693624605,0.));
#88110=CARTESIAN_POINT('Ctrl Pts',(46.1769085624582,3.14139693624605,20.));
#88111=CARTESIAN_POINT('Ctrl Pts',(46.1761639635878,3.10857131512384,0.));
#88112=CARTESIAN_POINT('Ctrl Pts',(46.1761639635878,3.10857131512384,20.));
#88113=CARTESIAN_POINT('Ctrl Pts',(46.1753961978798,3.0757473443616,0.));
#88114=CARTESIAN_POINT('Ctrl Pts',(46.1753961978798,3.0757473443616,20.));
#88115=CARTESIAN_POINT('Ctrl Pts',(46.1746052665999,3.04292504032497,0.));
#88116=CARTESIAN_POINT('Ctrl Pts',(46.1746052665999,3.04292504032497,20.));
#88117=CARTESIAN_POINT('Ctrl Pts',(46.1737911710261,3.01010441937913,0.));
#88118=CARTESIAN_POINT('Ctrl Pts',(46.1737911710261,3.01010441937913,20.));
#88119=CARTESIAN_POINT('Ctrl Pts',(46.1729539124487,2.9772854978889,0.));
#88120=CARTESIAN_POINT('Ctrl Pts',(46.1729539124487,2.9772854978889,20.));
#88121=CARTESIAN_POINT('Ctrl Pts',(46.172093492169,2.94446829221865,0.));
#88122=CARTESIAN_POINT('Ctrl Pts',(46.172093492169,2.94446829221865,20.));
#88123=CARTESIAN_POINT('Ctrl Pts',(46.1712099114993,2.91165281873225,0.));
#88124=CARTESIAN_POINT('Ctrl Pts',(46.1712099114993,2.91165281873225,20.));
#88125=CARTESIAN_POINT('Ctrl Pts',(46.1703031717627,2.87883909379287,0.));
#88126=CARTESIAN_POINT('Ctrl Pts',(46.1703031717627,2.87883909379287,20.));
#88127=CARTESIAN_POINT('Ctrl Pts',(46.169373274294,2.84602713376309,0.));
#88128=CARTESIAN_POINT('Ctrl Pts',(46.169373274294,2.84602713376309,20.));
#88129=CARTESIAN_POINT('Ctrl Pts',(46.1684202204402,2.81321695500492,0.));
#88130=CARTESIAN_POINT('Ctrl Pts',(46.1684202204402,2.81321695500492,20.));
#88131=CARTESIAN_POINT('Ctrl Pts',(46.1674440115603,2.78040857388008,0.));
#88132=CARTESIAN_POINT('Ctrl Pts',(46.1674440115603,2.78040857388008,20.));
#88133=CARTESIAN_POINT('Ctrl Pts',(46.1664446490252,2.7476020067498,0.));
#88134=CARTESIAN_POINT('Ctrl Pts',(46.1664446490252,2.7476020067498,20.));
#88135=CARTESIAN_POINT('Ctrl Pts',(46.1654221342175,2.71479726997479,0.));
#88136=CARTESIAN_POINT('Ctrl Pts',(46.1654221342175,2.71479726997479,20.));
#88137=CARTESIAN_POINT('Ctrl Pts',(46.1643764685316,2.68199437991524,0.));
#88138=CARTESIAN_POINT('Ctrl Pts',(46.1643764685316,2.68199437991524,20.));
#88139=CARTESIAN_POINT('Ctrl Pts',(46.163307653373,2.64919335293067,0.));
#88140=CARTESIAN_POINT('Ctrl Pts',(46.163307653373,2.64919335293067,20.));
#88141=CARTESIAN_POINT('Ctrl Pts',(46.1622156901587,2.61639420537995,0.));
#88142=CARTESIAN_POINT('Ctrl Pts',(46.1622156901587,2.61639420537995,20.));
#88143=CARTESIAN_POINT('Ctrl Pts',(46.1611005803162,2.58359695362108,0.));
#88144=CARTESIAN_POINT('Ctrl Pts',(46.1611005803162,2.58359695362108,20.));
#88145=CARTESIAN_POINT('Ctrl Pts',(46.1599623252856,2.55080161401166,0.));
#88146=CARTESIAN_POINT('Ctrl Pts',(46.1599623252856,2.55080161401166,20.));
#88147=CARTESIAN_POINT('Ctrl Pts',(46.1588009265184,2.51800820290892,0.));
#88148=CARTESIAN_POINT('Ctrl Pts',(46.1588009265184,2.51800820290892,20.));
#88149=CARTESIAN_POINT('Ctrl Pts',(46.1576163854777,2.48521673666957,0.));
#88150=CARTESIAN_POINT('Ctrl Pts',(46.1576163854777,2.48521673666957,20.));
#88151=CARTESIAN_POINT('Ctrl Pts',(46.1564087036389,2.4524272316497,0.));
#88152=CARTESIAN_POINT('Ctrl Pts',(46.1564087036389,2.4524272316497,20.));
#88153=CARTESIAN_POINT('Ctrl Pts',(46.155177882489,2.41963970420458,0.));
#88154=CARTESIAN_POINT('Ctrl Pts',(46.155177882489,2.41963970420458,20.));
#88155=CARTESIAN_POINT('Ctrl Pts',(46.1539239235264,2.38685417068871,0.));
#88156=CARTESIAN_POINT('Ctrl Pts',(46.1539239235264,2.38685417068871,20.));
#88157=CARTESIAN_POINT('Ctrl Pts',(46.1526468282603,2.35407064745589,0.));
#88158=CARTESIAN_POINT('Ctrl Pts',(46.1526468282603,2.35407064745589,20.));
#88159=CARTESIAN_POINT('Ctrl Pts',(46.1513465982124,2.3212891508592,0.));
#88160=CARTESIAN_POINT('Ctrl Pts',(46.1513465982124,2.3212891508592,20.));
#88161=CARTESIAN_POINT('Ctrl Pts',(46.1500232349155,2.28850969725138,0.));
#88162=CARTESIAN_POINT('Ctrl Pts',(46.1500232349155,2.28850969725138,20.));
#88163=CARTESIAN_POINT('Ctrl Pts',(46.1486767399146,2.25573230298459,0.));
#88164=CARTESIAN_POINT('Ctrl Pts',(46.1486767399146,2.25573230298459,20.));
#88165=CARTESIAN_POINT('Ctrl Pts',(46.147307114766,2.2229569844105,0.));
#88166=CARTESIAN_POINT('Ctrl Pts',(46.147307114766,2.2229569844105,20.));
#88167=CARTESIAN_POINT('Ctrl Pts',(46.1459143610377,2.19018375787987,0.));
#88168=CARTESIAN_POINT('Ctrl Pts',(46.1459143610377,2.19018375787987,20.));
#88169=CARTESIAN_POINT('Ctrl Pts',(46.1444984803082,2.15741263974263,0.));
#88170=CARTESIAN_POINT('Ctrl Pts',(46.1444984803082,2.15741263974263,20.));
#88171=CARTESIAN_POINT('Ctrl Pts',(46.1430594741682,2.12464364634813,0.));
#88172=CARTESIAN_POINT('Ctrl Pts',(46.1430594741682,2.12464364634813,20.));
#88173=CARTESIAN_POINT('Ctrl Pts',(46.1415973442202,2.09187679404497,0.));
#88174=CARTESIAN_POINT('Ctrl Pts',(46.1415973442202,2.09187679404497,20.));
#88175=CARTESIAN_POINT('Ctrl Pts',(46.1401120920793,2.05911209918102,0.));
#88176=CARTESIAN_POINT('Ctrl Pts',(46.1401120920793,2.05911209918102,20.));
#88177=CARTESIAN_POINT('Ctrl Pts',(46.1386037193727,2.02634957810318,0.));
#88178=CARTESIAN_POINT('Ctrl Pts',(46.1386037193727,2.02634957810318,20.));
#88179=CARTESIAN_POINT('Ctrl Pts',(46.1370722277379,1.99358924715754,0.));
#88180=CARTESIAN_POINT('Ctrl Pts',(46.1370722277379,1.99358924715754,20.));
#88181=CARTESIAN_POINT('Ctrl Pts',(46.1355176188236,1.96083112268931,0.));
#88182=CARTESIAN_POINT('Ctrl Pts',(46.1355176188236,1.96083112268931,20.));
#88183=CARTESIAN_POINT('Ctrl Pts',(46.1339398942902,1.9280752210434,0.));
#88184=CARTESIAN_POINT('Ctrl Pts',(46.1339398942902,1.9280752210434,20.));
#88185=CARTESIAN_POINT('Ctrl Pts',(46.1323390558096,1.89532155856415,0.));
#88186=CARTESIAN_POINT('Ctrl Pts',(46.1323390558096,1.89532155856415,20.));
#88187=CARTESIAN_POINT('Ctrl Pts',(46.1307151050651,1.86257015159583,0.));
#88188=CARTESIAN_POINT('Ctrl Pts',(46.1307151050651,1.86257015159583,20.));
#88189=CARTESIAN_POINT('Ctrl Pts',(46.1290680437528,1.82982101648207,0.));
#88190=CARTESIAN_POINT('Ctrl Pts',(46.1290680437528,1.82982101648207,20.));
#88191=CARTESIAN_POINT('Ctrl Pts',(46.1273978735796,1.79707416956535,0.));
#88192=CARTESIAN_POINT('Ctrl Pts',(46.1273978735796,1.79707416956535,20.));
#88193=CARTESIAN_POINT('Ctrl Pts',(46.1257045962649,1.76432962718686,0.));
#88194=CARTESIAN_POINT('Ctrl Pts',(46.1257045962649,1.76432962718686,20.));
#88195=CARTESIAN_POINT('Ctrl Pts',(46.1239882135394,1.73158740568598,0.));
#88196=CARTESIAN_POINT('Ctrl Pts',(46.1239882135394,1.73158740568598,20.));
#88197=CARTESIAN_POINT('Ctrl Pts',(46.1222487271454,1.6988475214004,0.));
#88198=CARTESIAN_POINT('Ctrl Pts',(46.1222487271454,1.6988475214004,20.));
#88199=CARTESIAN_POINT('Ctrl Pts',(46.1204861388364,1.66610999066656,0.));
#88200=CARTESIAN_POINT('Ctrl Pts',(46.1204861388364,1.66610999066656,20.));
#88201=CARTESIAN_POINT('Ctrl Pts',(46.1187004503775,1.63337482982071,0.));
#88202=CARTESIAN_POINT('Ctrl Pts',(46.1187004503775,1.63337482982071,20.));
#88203=CARTESIAN_POINT('Ctrl Pts',(46.1168916635447,1.60064205519959,0.));
#88204=CARTESIAN_POINT('Ctrl Pts',(46.1168916635447,1.60064205519959,20.));
#88205=CARTESIAN_POINT('Ctrl Pts',(46.1150597801266,1.56791168314158,0.));
#88206=CARTESIAN_POINT('Ctrl Pts',(46.1150597801266,1.56791168314158,20.));
#88207=CARTESIAN_POINT('Ctrl Pts',(46.1132048019234,1.53518372998667,0.));
#88208=CARTESIAN_POINT('Ctrl Pts',(46.1132048019234,1.53518372998667,20.));
#88209=CARTESIAN_POINT('Ctrl Pts',(46.111326730748,1.50245821207431,0.));
#88210=CARTESIAN_POINT('Ctrl Pts',(46.111326730748,1.50245821207431,20.));
#88211=CARTESIAN_POINT('Ctrl Pts',(46.1094255684237,1.46973514574144,0.));
#88212=CARTESIAN_POINT('Ctrl Pts',(46.1094255684237,1.46973514574144,20.));
#88213=CARTESIAN_POINT('Ctrl Pts',(46.1075013167858,1.43701454732091,0.));
#88214=CARTESIAN_POINT('Ctrl Pts',(46.1075013167858,1.43701454732091,20.));
#88215=CARTESIAN_POINT('Ctrl Pts',(46.1055539776801,1.40429643313894,0.));
#88216=CARTESIAN_POINT('Ctrl Pts',(46.1055539776801,1.40429643313894,20.));
#88217=CARTESIAN_POINT('Ctrl Pts',(46.1035835529643,1.37158081951552,0.));
#88218=CARTESIAN_POINT('Ctrl Pts',(46.1035835529643,1.37158081951552,20.));
#88219=CARTESIAN_POINT('Ctrl Pts',(46.1015900445065,1.33886772276919,0.));
#88220=CARTESIAN_POINT('Ctrl Pts',(46.1015900445065,1.33886772276919,20.));
#88221=CARTESIAN_POINT('Ctrl Pts',(46.0995734541875,1.30615715922173,0.));
#88222=CARTESIAN_POINT('Ctrl Pts',(46.0995734541875,1.30615715922173,20.));
#88223=CARTESIAN_POINT('Ctrl Pts',(46.0975337839002,1.27344914520176,0.));
#88224=CARTESIAN_POINT('Ctrl Pts',(46.0975337839002,1.27344914520176,20.));
#88225=CARTESIAN_POINT('Ctrl Pts',(46.0954710355506,1.24074369705073,0.));
#88226=CARTESIAN_POINT('Ctrl Pts',(46.0954710355506,1.24074369705073,20.));
#88227=CARTESIAN_POINT('Ctrl Pts',(46.0933852110571,1.20804083112097,0.));
#88228=CARTESIAN_POINT('Ctrl Pts',(46.0933852110571,1.20804083112097,20.));
#88229=CARTESIAN_POINT('Ctrl Pts',(46.0912763123502,1.17534056376402,0.));
#88230=CARTESIAN_POINT('Ctrl Pts',(46.0912763123502,1.17534056376402,20.));
#88231=CARTESIAN_POINT('Ctrl Pts',(46.0891443413718,1.14264291132053,0.));
#88232=CARTESIAN_POINT('Ctrl Pts',(46.0891443413718,1.14264291132053,20.));
#88233=CARTESIAN_POINT('Ctrl Pts',(46.0869893000733,1.10994789011163,0.));
#88234=CARTESIAN_POINT('Ctrl Pts',(46.0869893000733,1.10994789011163,20.));
#88235=CARTESIAN_POINT('Ctrl Pts',(46.0848111904142,1.07725551642471,0.));
#88236=CARTESIAN_POINT('Ctrl Pts',(46.0848111904142,1.07725551642471,20.));
#88237=CARTESIAN_POINT('Ctrl Pts',(46.0826100143611,1.04456580652048,0.));
#88238=CARTESIAN_POINT('Ctrl Pts',(46.0826100143611,1.04456580652048,20.));
#88239=CARTESIAN_POINT('Ctrl Pts',(46.0803857738924,1.01187877665955,0.));
#88240=CARTESIAN_POINT('Ctrl Pts',(46.0803857738924,1.01187877665955,20.));
#88241=CARTESIAN_POINT('Ctrl Pts',(46.0781384710012,0.979194443126295,0.));
#88242=CARTESIAN_POINT('Ctrl Pts',(46.0781384710012,0.979194443126295,20.));
#88243=CARTESIAN_POINT('Ctrl Pts',(46.0758681076973,0.946512822248755,0.));
#88244=CARTESIAN_POINT('Ctrl Pts',(46.0758681076973,0.946512822248755,20.));
#88245=CARTESIAN_POINT('Ctrl Pts',(46.0735746860119,0.913833930432277,0.));
#88246=CARTESIAN_POINT('Ctrl Pts',(46.0735746860119,0.913833930432277,20.));
#88247=CARTESIAN_POINT('Ctrl Pts',(46.0712582079948,0.881157784136745,0.));
#88248=CARTESIAN_POINT('Ctrl Pts',(46.0712582079948,0.881157784136745,20.));
#88249=CARTESIAN_POINT('Ctrl Pts',(46.0689186757066,0.848484399815189,0.));
#88250=CARTESIAN_POINT('Ctrl Pts',(46.0689186757066,0.848484399815189,20.));
#88251=CARTESIAN_POINT('Ctrl Pts',(46.0665560912128,0.815813793858643,0.));
#88252=CARTESIAN_POINT('Ctrl Pts',(46.0665560912128,0.815813793858643,20.));
#88253=CARTESIAN_POINT('Ctrl Pts',(46.064170456577,0.783145982548935,0.));
#88254=CARTESIAN_POINT('Ctrl Pts',(46.064170456577,0.783145982548935,20.));
#88255=CARTESIAN_POINT('Ctrl Pts',(46.0617617738521,0.750480981980926,0.));
#88256=CARTESIAN_POINT('Ctrl Pts',(46.0617617738521,0.750480981980926,20.));
#88257=CARTESIAN_POINT('Ctrl Pts',(46.0593300450868,0.71781880812973,0.));
#88258=CARTESIAN_POINT('Ctrl Pts',(46.0593300450868,0.71781880812973,20.));
#88259=CARTESIAN_POINT('Ctrl Pts',(46.0568752723439,0.685159476991768,0.));
#88260=CARTESIAN_POINT('Ctrl Pts',(46.0568752723439,0.685159476991768,20.));
#88261=CARTESIAN_POINT('Ctrl Pts',(46.0543974577158,0.652503004713265,0.));
#88262=CARTESIAN_POINT('Ctrl Pts',(46.0543974577158,0.652503004713265,20.));
#88263=CARTESIAN_POINT('Ctrl Pts',(46.0518966033391,0.619849407700868,0.));
#88264=CARTESIAN_POINT('Ctrl Pts',(46.0518966033391,0.619849407700868,20.));
#88265=CARTESIAN_POINT('Ctrl Pts',(46.0493727114182,0.587198702798626,0.));
#88266=CARTESIAN_POINT('Ctrl Pts',(46.0493727114182,0.587198702798626,20.));
#88267=CARTESIAN_POINT('Ctrl Pts',(46.0468257841997,0.554550907098833,0.));
#88268=CARTESIAN_POINT('Ctrl Pts',(46.0468257841997,0.554550907098833,20.));
#88269=CARTESIAN_POINT('Ctrl Pts',(46.044255823933,0.521906037621051,0.));
#88270=CARTESIAN_POINT('Ctrl Pts',(46.044255823933,0.521906037621051,20.));
#88271=CARTESIAN_POINT('Ctrl Pts',(46.0416628328334,0.489264111013841,0.));
#88272=CARTESIAN_POINT('Ctrl Pts',(46.0416628328334,0.489264111013841,20.));
#88273=CARTESIAN_POINT('Ctrl Pts',(46.0390468130479,0.456625143292617,0.));
#88274=CARTESIAN_POINT('Ctrl Pts',(46.0390468130479,0.456625143292617,20.));
#88275=CARTESIAN_POINT('Ctrl Pts',(46.0364077666069,0.42398914944525,0.));
#88276=CARTESIAN_POINT('Ctrl Pts',(46.0364077666069,0.42398914944525,20.));
#88277=CARTESIAN_POINT('Ctrl Pts',(46.0337456954889,0.391356143937839,0.));
#88278=CARTESIAN_POINT('Ctrl Pts',(46.0337456954889,0.391356143937839,20.));
#88279=CARTESIAN_POINT('Ctrl Pts',(46.0310606017089,0.358726141441572,0.));
#88280=CARTESIAN_POINT('Ctrl Pts',(46.0310606017089,0.358726141441572,20.));
#88281=CARTESIAN_POINT('Ctrl Pts',(46.0283524874048,0.32609915751696,0.));
#88282=CARTESIAN_POINT('Ctrl Pts',(46.0283524874048,0.32609915751696,20.));
#88283=CARTESIAN_POINT('Ctrl Pts',(46.025621354915,0.293475209241793,0.));
#88284=CARTESIAN_POINT('Ctrl Pts',(46.025621354915,0.293475209241793,20.));
#88285=CARTESIAN_POINT('Ctrl Pts',(46.022867206884,0.260854316057536,0.));
#88286=CARTESIAN_POINT('Ctrl Pts',(46.022867206884,0.260854316057536,20.));
#88287=CARTESIAN_POINT('Ctrl Pts',(46.0200900461091,0.228236498538563,0.));
#88288=CARTESIAN_POINT('Ctrl Pts',(46.0200900461091,0.228236498538563,20.));
#88289=CARTESIAN_POINT('Ctrl Pts',(46.0172898753497,0.195621776838885,0.));
#88290=CARTESIAN_POINT('Ctrl Pts',(46.0172898753497,0.195621776838885,20.));
#88291=CARTESIAN_POINT('Ctrl Pts',(46.0144666971462,0.163010169231708,0.));
#88292=CARTESIAN_POINT('Ctrl Pts',(46.0144666971462,0.163010169231708,20.));
#88293=CARTESIAN_POINT('Ctrl Pts',(46.0116205136405,0.130401690656321,0.));
#88294=CARTESIAN_POINT('Ctrl Pts',(46.0116205136405,0.130401690656321,20.));
#88295=CARTESIAN_POINT('Ctrl Pts',(46.0087513263814,0.0977963511372851,
0.));
#88296=CARTESIAN_POINT('Ctrl Pts',(46.0087513263814,0.0977963511372851,
20.));
#88297=CARTESIAN_POINT('Ctrl Pts',(46.0058591364029,0.0651941566547578,
0.));
#88298=CARTESIAN_POINT('Ctrl Pts',(46.0058591364029,0.0651941566547578,
20.));
#88299=CARTESIAN_POINT('Ctrl Pts',(46.0035269827389,0.0391149194889428,
0.));
#88300=CARTESIAN_POINT('Ctrl Pts',(46.0035269827389,0.0391149194889428,
20.));
#88301=CARTESIAN_POINT('Ctrl Pts',(46.0017675166781,0.0195569086685896,
0.));
#88302=CARTESIAN_POINT('Ctrl Pts',(46.0017675166781,0.0195569086685896,
20.));
#88303=CARTESIAN_POINT('Ctrl Pts',(46.0005899389515,0.0065188645893676,
0.));
#88304=CARTESIAN_POINT('Ctrl Pts',(46.0005899389515,0.0065188645893676,
20.));
#88305=CARTESIAN_POINT('Ctrl Pts',(46.,0.,0.));
#88306=CARTESIAN_POINT('Ctrl Pts',(46.,0.,20.));
#88307=CARTESIAN_POINT('',(37.5361777128299,31.4965928746404,2.));
#88308=CARTESIAN_POINT('Ctrl Pts',(45.2025619355895,13.7414592977624,2.));
#88309=CARTESIAN_POINT('Ctrl Pts',(45.039110381915,14.5281012519506,2.));
#88310=CARTESIAN_POINT('Ctrl Pts',(44.8554703046337,15.3115504167957,2.));
#88311=CARTESIAN_POINT('Ctrl Pts',(44.6518239974238,16.0907854020754,2.));
#88312=CARTESIAN_POINT('Ctrl Pts',(44.448476647749,16.8688764521982,2.));
#88313=CARTESIAN_POINT('Ctrl Pts',(44.2251818321296,17.6427655208206,2.));
#88314=CARTESIAN_POINT('Ctrl Pts',(43.9821719094461,18.4114480909826,2.));
#88315=CARTESIAN_POINT('Ctrl Pts',(43.7389521035327,19.1807945582349,2.));
#88316=CARTESIAN_POINT('Ctrl Pts',(43.4759831771533,19.9449253625111,2.));
#88317=CARTESIAN_POINT('Ctrl Pts',(43.1935481793562,20.7028482985112,2.));
#88318=CARTESIAN_POINT('Ctrl Pts',(42.910868013075,21.4614291516204,2.));
#88319=CARTESIAN_POINT('Ctrl Pts',(42.6086880302604,22.2137911905079,2.));
#88320=CARTESIAN_POINT('Ctrl Pts',(42.2873412605298,22.9589570442281,2.));
#88321=CARTESIAN_POINT('Ctrl Pts',(41.9655415206855,23.7051732830564,2.));
#88322=CARTESIAN_POINT('Ctrl Pts',(41.6245209894068,24.44417287288,2.));
#88323=CARTESIAN_POINT('Ctrl Pts',(41.2646624723933,25.1749942158169,2.));
#88324=CARTESIAN_POINT('Ctrl Pts',(40.9045439223885,25.9063436486862,2.));
#88325=CARTESIAN_POINT('Ctrl Pts',(40.5255602341407,26.6295028556231,2.));
#88326=CARTESIAN_POINT('Ctrl Pts',(40.1281423069477,27.3435304618815,2.));
#88327=CARTESIAN_POINT('Ctrl Pts',(39.7321213838807,28.0550481171695,2.));
#88328=CARTESIAN_POINT('Ctrl Pts',(39.3177957144339,28.7574981262846,2.));
#88329=CARTESIAN_POINT('Ctrl Pts',(38.8856370208255,29.4499732757602,2.));
#88330=CARTESIAN_POINT('Ctrl Pts',(38.6009980869291,29.9060682038772,2.));
#88331=CARTESIAN_POINT('Ctrl Pts',(38.3086238828692,30.3578364223247,2.));
#88332=CARTESIAN_POINT('Ctrl Pts',(38.0086596303984,30.8050248835235,2.));
#88333=CARTESIAN_POINT('Ctrl Pts',(37.8531972210893,31.0367891521673,2.));
#88334=CARTESIAN_POINT('Ctrl Pts',(37.6956965296231,31.2673228693602,2.));
#88335=CARTESIAN_POINT('Ctrl Pts',(37.5361777128299,31.4965928746404,2.));
#88336=CARTESIAN_POINT('',(37.5361777128299,31.4965928746404,0.));
#88337=CARTESIAN_POINT('Origin',(-1.19904086659517E-13,-1.4210854715202E-13,
0.));
#88338=CARTESIAN_POINT('',(-34.6009561857411,-30.3112822399915,2.));
#88339=CARTESIAN_POINT('',(-34.6009561857411,-30.3112822399915,0.));
#88340=CARTESIAN_POINT('Origin',(-1.19904086659517E-13,-1.4210854715202E-13,
2.));
#88341=CARTESIAN_POINT('Origin',(-35.3531508854311,-30.9702231582522,0.));
#88342=CARTESIAN_POINT('',(-35.9959384951176,-30.2041787151332,2.));
#88343=CARTESIAN_POINT('',(-35.9959384951176,-30.2041787151332,0.));
#88344=CARTESIAN_POINT('Origin',(-35.3531508854311,-30.9702231582522,2.));
#88345=CARTESIAN_POINT('Origin',(-35.238044383473,-29.5682300455808,0.));
#88346=CARTESIAN_POINT('',(-17.6190221917365,-14.7841150227904,2.));
#88347=CARTESIAN_POINT('Origin',(-1.83021655258307E-13,3.27857114887025E-14,
0.));
#88348=CARTESIAN_POINT('',(-43.5508185339833,14.8096659320883,2.));
#88349=CARTESIAN_POINT('',(-43.5508185339833,14.8096659320883,0.));
#88350=CARTESIAN_POINT('Origin',(-1.83021655258307E-13,3.27857114887025E-14,
2.));
#88351=CARTESIAN_POINT('Origin',(-44.4975754586351,15.1316151914815,0.));
#88352=CARTESIAN_POINT('',(-44.1555553153094,16.0713078122674,2.));
#88353=CARTESIAN_POINT('',(-44.1555553153094,16.0713078122674,0.));
#88354=CARTESIAN_POINT('Origin',(-44.4975754586351,15.1316151914815,2.));
#88355=CARTESIAN_POINT('Origin',(-43.2258605561518,15.7329265929808,0.));
#88356=CARTESIAN_POINT('',(-21.6129302780759,7.86646329649041,2.));
#88357=CARTESIAN_POINT('Origin',(-6.31175685987896E-14,1.74894258640722E-13,
0.));
#88358=CARTESIAN_POINT('',(-8.94986234824223,45.1209481720799,2.));
#88359=CARTESIAN_POINT('',(-8.94986234824223,45.1209481720799,0.));
#88360=CARTESIAN_POINT('Origin',(-6.31175685987896E-14,1.74894258640722E-13,
2.));
#88361=CARTESIAN_POINT('Origin',(-9.14442457320401,46.1018383497338,0.));
#88362=CARTESIAN_POINT('',(-8.1596168201918,46.2754865274007,2.));
#88363=CARTESIAN_POINT('',(-8.1596168201918,46.2754865274007,0.));
#88364=CARTESIAN_POINT('Origin',(-9.14442457320401,46.1018383497338,2.));
#88365=CARTESIAN_POINT('Origin',(-7.98781617267879,45.3011566385616,0.));
#88366=CARTESIAN_POINT('',(-3.99390808633937,22.6505783192808,2.));
#88367=CARTESIAN_POINT('Origin',(0.,0.,2.));
#88368=CARTESIAN_POINT('',(23.,-39.8371685740842,2.));
#88369=CARTESIAN_POINT('Ctrl Pts',(23.,-39.8371685740842,2.));
#88370=CARTESIAN_POINT('Ctrl Pts',(25.2470089248039,-38.7975252546671,2.));
#88371=CARTESIAN_POINT('Ctrl Pts',(27.402276150069,-37.5810556253098,2.));
#88372=CARTESIAN_POINT('Ctrl Pts',(29.4485343853537,-36.2031892016999,2.));
#88373=CARTESIAN_POINT('',(8.94986234824221,-45.1209481720799,2.));
#88374=CARTESIAN_POINT('Origin',(6.31175685987895E-14,-1.74894258640722E-13,
2.));
#88375=CARTESIAN_POINT('',(8.15961682019179,-46.2754865274007,2.));
#88376=CARTESIAN_POINT('Origin',(9.144424573204,-46.1018383497338,2.));
#88377=CARTESIAN_POINT('',(3.99390808633936,-22.6505783192808,2.));
#88378=CARTESIAN_POINT('',(23.,39.8371685740842,2.));
#88379=CARTESIAN_POINT('Ctrl Pts',(23.,39.8371685740842,2.));
#88380=CARTESIAN_POINT('Ctrl Pts',(20.9761380121528,41.2633137257534,2.));
#88381=CARTESIAN_POINT('Ctrl Pts',(18.8450107965655,42.5215950805976,2.));
#88382=CARTESIAN_POINT('Ctrl Pts',(16.6286143540096,43.6047734827858,2.));
#88383=CARTESIAN_POINT('',(34.6009561857411,30.3112822399915,2.));
#88384=CARTESIAN_POINT('Origin',(1.19904086659517E-13,1.4210854715202E-13,
2.));
#88385=CARTESIAN_POINT('',(35.9959384951176,30.2041787151333,2.));
#88386=CARTESIAN_POINT('Origin',(35.3531508854311,30.9702231582522,2.));
#88387=CARTESIAN_POINT('',(17.6190221917365,14.7841150227904,2.));
#88388=CARTESIAN_POINT('',(46.,0.,2.));
#88389=CARTESIAN_POINT('Ctrl Pts',(46.,0.,2.));
#88390=CARTESIAN_POINT('Ctrl Pts',(46.2231469368338,2.46578847026074,2.));
#88391=CARTESIAN_POINT('Ctrl Pts',(46.2472869475088,4.94053945592409,2.));
#88392=CARTESIAN_POINT('Ctrl Pts',(46.0771487393634,7.40158428108603,2.));
#88393=CARTESIAN_POINT('',(43.5508185339833,-14.8096659320883,2.));
#88394=CARTESIAN_POINT('Origin',(1.83021655258307E-13,-3.27857114887026E-14,
2.));
#88395=CARTESIAN_POINT('',(44.1555553153094,-16.0713078122675,2.));
#88396=CARTESIAN_POINT('Origin',(44.4975754586351,-15.1316151914816,2.));
#88397=CARTESIAN_POINT('',(21.6129302780759,-7.86646329649042,2.));
#88398=CARTESIAN_POINT('Origin',(0.,0.,2.));
#88399=CARTESIAN_POINT('Origin',(7.98781617267877,-45.3011566385616,0.));
#88400=CARTESIAN_POINT('',(8.15961682019179,-46.2754865274007,0.));
#88401=CARTESIAN_POINT('Origin',(9.144424573204,-46.1018383497338,0.));
#88402=CARTESIAN_POINT('',(8.94986234824221,-45.1209481720799,0.));
#88403=CARTESIAN_POINT('Origin',(6.31175685987895E-14,-1.74894258640722E-13,
0.));
#88404=CARTESIAN_POINT('',(23.,-39.8371685740842,0.));
#88405=CARTESIAN_POINT('Ctrl Pts',(46.0449384185095,-16.7589870229578,0.));
#88406=CARTESIAN_POINT('Ctrl Pts',(46.0449384185095,-16.7589870229578,20.));
#88407=CARTESIAN_POINT('Ctrl Pts',(46.0420594924752,-16.7651130917503,0.));
#88408=CARTESIAN_POINT('Ctrl Pts',(46.0420594924752,-16.7651130917503,20.));
#88409=CARTESIAN_POINT('Ctrl Pts',(46.0362995834799,-16.7773641333857,0.));
#88410=CARTESIAN_POINT('Ctrl Pts',(46.0362995834799,-16.7773641333857,20.));
#88411=CARTESIAN_POINT('Ctrl Pts',(46.0276535492064,-16.79573740799,0.));
#88412=CARTESIAN_POINT('Ctrl Pts',(46.0276535492064,-16.79573740799,20.));
#88413=CARTESIAN_POINT('Ctrl Pts',(46.0161131619282,-16.8202285317553,0.));
#88414=CARTESIAN_POINT('Ctrl Pts',(46.0161131619282,-16.8202285317553,20.));
#88415=CARTESIAN_POINT('Ctrl Pts',(46.0016671088634,-16.8508314760754,0.));
#88416=CARTESIAN_POINT('Ctrl Pts',(46.0016671088634,-16.8508314760754,20.));
#88417=CARTESIAN_POINT('Ctrl Pts',(45.9872004880192,-16.8814234574889,0.));
#88418=CARTESIAN_POINT('Ctrl Pts',(45.9872004880192,-16.8814234574889,20.));
#88419=CARTESIAN_POINT('Ctrl Pts',(45.9727133019197,-16.9120044710149,0.));
#88420=CARTESIAN_POINT('Ctrl Pts',(45.9727133019197,-16.9120044710149,20.));
#88421=CARTESIAN_POINT('Ctrl Pts',(45.9582055548827,-16.9425745084438,0.));
#88422=CARTESIAN_POINT('Ctrl Pts',(45.9582055548827,-16.9425745084438,20.));
#88423=CARTESIAN_POINT('Ctrl Pts',(45.9436772535459,-16.9731335574459,0.));
#88424=CARTESIAN_POINT('Ctrl Pts',(45.9436772535459,-16.9731335574459,20.));
#88425=CARTESIAN_POINT('Ctrl Pts',(45.9291284062576,-17.0036816026634,0.));
#88426=CARTESIAN_POINT('Ctrl Pts',(45.9291284062576,-17.0036816026634,20.));
#88427=CARTESIAN_POINT('Ctrl Pts',(45.91455902239,-17.0342186269342,0.));
#88428=CARTESIAN_POINT('Ctrl Pts',(45.91455902239,-17.0342186269342,20.));
#88429=CARTESIAN_POINT('Ctrl Pts',(45.8999691116666,-17.0647446124944,0.));
#88430=CARTESIAN_POINT('Ctrl Pts',(45.8999691116666,-17.0647446124944,20.));
#88431=CARTESIAN_POINT('Ctrl Pts',(45.8853586835176,-17.09525954213,0.));
#88432=CARTESIAN_POINT('Ctrl Pts',(45.8853586835176,-17.09525954213,20.));
#88433=CARTESIAN_POINT('Ctrl Pts',(45.8707277463338,-17.1257634005084,0.));
#88434=CARTESIAN_POINT('Ctrl Pts',(45.8707277463338,-17.1257634005084,20.));
#88435=CARTESIAN_POINT('Ctrl Pts',(45.8560763076625,-17.1562561738292,0.));
#88436=CARTESIAN_POINT('Ctrl Pts',(45.8560763076625,-17.1562561738292,20.));
#88437=CARTESIAN_POINT('Ctrl Pts',(45.8414043745501,-17.1867378492105,0.));
#88438=CARTESIAN_POINT('Ctrl Pts',(45.8414043745501,-17.1867378492105,20.));
#88439=CARTESIAN_POINT('Ctrl Pts',(45.8267119538424,-17.2172084141516,0.));
#88440=CARTESIAN_POINT('Ctrl Pts',(45.8267119538424,-17.2172084141516,20.));
#88441=CARTESIAN_POINT('Ctrl Pts',(45.8119990524823,-17.247667856,0.));
#88442=CARTESIAN_POINT('Ctrl Pts',(45.8119990524823,-17.247667856,20.));
#88443=CARTESIAN_POINT('Ctrl Pts',(45.7972656778619,-17.2781161613228,0.));
#88444=CARTESIAN_POINT('Ctrl Pts',(45.7972656778619,-17.2781161613228,20.));
#88445=CARTESIAN_POINT('Ctrl Pts',(45.7825118377706,-17.3085533159982,0.));
#88446=CARTESIAN_POINT('Ctrl Pts',(45.7825118377706,-17.3085533159982,20.));
#88447=CARTESIAN_POINT('Ctrl Pts',(45.7677375402375,-17.3389793054985,0.));
#88448=CARTESIAN_POINT('Ctrl Pts',(45.7677375402375,-17.3389793054985,20.));
#88449=CARTESIAN_POINT('Ctrl Pts',(45.7529427934047,-17.3693941151172,0.));
#88450=CARTESIAN_POINT('Ctrl Pts',(45.7529427934047,-17.3693941151172,20.));
#88451=CARTESIAN_POINT('Ctrl Pts',(45.7381276053971,-17.3997977302007,0.));
#88452=CARTESIAN_POINT('Ctrl Pts',(45.7381276053971,-17.3997977302007,20.));
#88453=CARTESIAN_POINT('Ctrl Pts',(45.7232919841685,-17.4301901364248,0.));
#88454=CARTESIAN_POINT('Ctrl Pts',(45.7232919841685,-17.4301901364248,20.));
#88455=CARTESIAN_POINT('Ctrl Pts',(45.7084359375081,-17.460571319782,0.));
#88456=CARTESIAN_POINT('Ctrl Pts',(45.7084359375081,-17.460571319782,20.));
#88457=CARTESIAN_POINT('Ctrl Pts',(45.6935594731126,-17.490941266452,0.));
#88458=CARTESIAN_POINT('Ctrl Pts',(45.6935594731126,-17.490941266452,20.));
#88459=CARTESIAN_POINT('Ctrl Pts',(45.67866259864,-17.5212999627071,0.));
#88460=CARTESIAN_POINT('Ctrl Pts',(45.67866259864,-17.5212999627071,20.));
#88461=CARTESIAN_POINT('Ctrl Pts',(45.6637453217655,-17.5516473948116,0.));
#88462=CARTESIAN_POINT('Ctrl Pts',(45.6637453217655,-17.5516473948116,20.));
#88463=CARTESIAN_POINT('Ctrl Pts',(45.6488076502485,-17.5819835489016,0.));
#88464=CARTESIAN_POINT('Ctrl Pts',(45.6488076502485,-17.5819835489016,20.));
#88465=CARTESIAN_POINT('Ctrl Pts',(45.6338495919363,-17.6123084109794,0.));
#88466=CARTESIAN_POINT('Ctrl Pts',(45.6338495919363,-17.6123084109794,20.));
#88467=CARTESIAN_POINT('Ctrl Pts',(45.6188711547313,-17.6426219669712,0.));
#88468=CARTESIAN_POINT('Ctrl Pts',(45.6188711547313,-17.6426219669712,20.));
#88469=CARTESIAN_POINT('Ctrl Pts',(45.6038723465685,-17.672924202767,0.));
#88470=CARTESIAN_POINT('Ctrl Pts',(45.6038723465685,-17.672924202767,20.));
#88471=CARTESIAN_POINT('Ctrl Pts',(45.5888531753911,-17.7032151042646,0.));
#88472=CARTESIAN_POINT('Ctrl Pts',(45.5888531753911,-17.7032151042646,20.));
#88473=CARTESIAN_POINT('Ctrl Pts',(45.5738136491221,-17.7334946574206,0.));
#88474=CARTESIAN_POINT('Ctrl Pts',(45.5738136491221,-17.7334946574206,20.));
#88475=CARTESIAN_POINT('Ctrl Pts',(45.5587537756595,-17.7637628482589,0.));
#88476=CARTESIAN_POINT('Ctrl Pts',(45.5587537756595,-17.7637628482589,20.));
#88477=CARTESIAN_POINT('Ctrl Pts',(45.5436735628911,-17.7940196628443,0.));
#88478=CARTESIAN_POINT('Ctrl Pts',(45.5436735628911,-17.7940196628443,20.));
#88479=CARTESIAN_POINT('Ctrl Pts',(45.528573018704,-17.8242650872661,0.));
#88480=CARTESIAN_POINT('Ctrl Pts',(45.528573018704,-17.8242650872661,20.));
#88481=CARTESIAN_POINT('Ctrl Pts',(45.5134521509949,-17.8544991076192,0.));
#88482=CARTESIAN_POINT('Ctrl Pts',(45.5134521509949,-17.8544991076192,20.));
#88483=CARTESIAN_POINT('Ctrl Pts',(45.498310967683,-17.8847217099814,0.));
#88484=CARTESIAN_POINT('Ctrl Pts',(45.498310967683,-17.8847217099814,20.));
#88485=CARTESIAN_POINT('Ctrl Pts',(45.4831494767122,-17.9149328804084,0.));
#88486=CARTESIAN_POINT('Ctrl Pts',(45.4831494767122,-17.9149328804084,20.));
#88487=CARTESIAN_POINT('Ctrl Pts',(45.4679676860453,-17.9451326049449,0.));
#88488=CARTESIAN_POINT('Ctrl Pts',(45.4679676860453,-17.9451326049449,20.));
#88489=CARTESIAN_POINT('Ctrl Pts',(45.4527656036598,-17.9753208696316,0.));
#88490=CARTESIAN_POINT('Ctrl Pts',(45.4527656036598,-17.9753208696316,20.));
#88491=CARTESIAN_POINT('Ctrl Pts',(45.4375432375433,-18.0054976605138,0.));
#88492=CARTESIAN_POINT('Ctrl Pts',(45.4375432375433,-18.0054976605138,20.));
#88493=CARTESIAN_POINT('Ctrl Pts',(45.4223005956881,-18.0356629636502,0.));
#88494=CARTESIAN_POINT('Ctrl Pts',(45.4223005956881,-18.0356629636502,20.));
#88495=CARTESIAN_POINT('Ctrl Pts',(45.4070376860893,-18.0658167651176,0.));
#88496=CARTESIAN_POINT('Ctrl Pts',(45.4070376860893,-18.0658167651176,20.));
#88497=CARTESIAN_POINT('Ctrl Pts',(45.3917545167484,-18.0959590510046,0.));
#88498=CARTESIAN_POINT('Ctrl Pts',(45.3917545167484,-18.0959590510046,20.));
#88499=CARTESIAN_POINT('Ctrl Pts',(45.3764510956741,-18.1260898074095,0.));
#88500=CARTESIAN_POINT('Ctrl Pts',(45.3764510956741,-18.1260898074095,20.));
#88501=CARTESIAN_POINT('Ctrl Pts',(45.3611274308852,-18.156209020436,0.));
#88502=CARTESIAN_POINT('Ctrl Pts',(45.3611274308852,-18.156209020436,20.));
#88503=CARTESIAN_POINT('Ctrl Pts',(45.3457835304119,-18.1863166761898,0.));
#88504=CARTESIAN_POINT('Ctrl Pts',(45.3457835304119,-18.1863166761898,20.));
#88505=CARTESIAN_POINT('Ctrl Pts',(45.3304194022976,-18.2164127607761,0.));
#88506=CARTESIAN_POINT('Ctrl Pts',(45.3304194022976,-18.2164127607761,20.));
#88507=CARTESIAN_POINT('Ctrl Pts',(45.3150350545965,-18.2464972603023,0.));
#88508=CARTESIAN_POINT('Ctrl Pts',(45.3150350545965,-18.2464972603023,20.));
#88509=CARTESIAN_POINT('Ctrl Pts',(45.299630495374,-18.276570160879,0.));
#88510=CARTESIAN_POINT('Ctrl Pts',(45.299630495374,-18.276570160879,20.));
#88511=CARTESIAN_POINT('Ctrl Pts',(45.2842057327048,-18.3066314486215,0.));
#88512=CARTESIAN_POINT('Ctrl Pts',(45.2842057327048,-18.3066314486215,20.));
#88513=CARTESIAN_POINT('Ctrl Pts',(45.2687607746732,-18.3366811096519,0.));
#88514=CARTESIAN_POINT('Ctrl Pts',(45.2687607746732,-18.3366811096519,20.));
#88515=CARTESIAN_POINT('Ctrl Pts',(45.2532956293718,-18.3667191300999,0.));
#88516=CARTESIAN_POINT('Ctrl Pts',(45.2532956293718,-18.3667191300999,20.));
#88517=CARTESIAN_POINT('Ctrl Pts',(45.2378103049022,-18.3967454961017,0.));
#88518=CARTESIAN_POINT('Ctrl Pts',(45.2378103049022,-18.3967454961017,20.));
#88519=CARTESIAN_POINT('Ctrl Pts',(45.2223048093755,-18.4267601937997,0.));
#88520=CARTESIAN_POINT('Ctrl Pts',(45.2223048093755,-18.4267601937997,20.));
#88521=CARTESIAN_POINT('Ctrl Pts',(45.2067791509123,-18.456763209342,0.));
#88522=CARTESIAN_POINT('Ctrl Pts',(45.2067791509123,-18.456763209342,20.));
#88523=CARTESIAN_POINT('Ctrl Pts',(45.1912333376434,-18.4867545288811,0.));
#88524=CARTESIAN_POINT('Ctrl Pts',(45.1912333376434,-18.4867545288811,20.));
#88525=CARTESIAN_POINT('Ctrl Pts',(45.1756673777099,-18.5167341385735,0.));
#88526=CARTESIAN_POINT('Ctrl Pts',(45.1756673777099,-18.5167341385735,20.));
#88527=CARTESIAN_POINT('Ctrl Pts',(45.1600812792631,-18.5467020245809,0.));
#88528=CARTESIAN_POINT('Ctrl Pts',(45.1600812792631,-18.5467020245809,20.));
#88529=CARTESIAN_POINT('Ctrl Pts',(45.144475050464,-18.5766581730695,0.));
#88530=CARTESIAN_POINT('Ctrl Pts',(45.144475050464,-18.5766581730695,20.));
#88531=CARTESIAN_POINT('Ctrl Pts',(45.1288486994834,-18.6066025702107,0.));
#88532=CARTESIAN_POINT('Ctrl Pts',(45.1288486994834,-18.6066025702107,20.));
#88533=CARTESIAN_POINT('Ctrl Pts',(45.1132022345013,-18.6365352021814,0.));
#88534=CARTESIAN_POINT('Ctrl Pts',(45.1132022345013,-18.6365352021814,20.));
#88535=CARTESIAN_POINT('Ctrl Pts',(45.097535663708,-18.6664560551643,0.));
#88536=CARTESIAN_POINT('Ctrl Pts',(45.097535663708,-18.6664560551643,20.));
#88537=CARTESIAN_POINT('Ctrl Pts',(45.081848995303,-18.6963651153477,0.));
#88538=CARTESIAN_POINT('Ctrl Pts',(45.081848995303,-18.6963651153477,20.));
#88539=CARTESIAN_POINT('Ctrl Pts',(45.0661422374956,-18.7262623689254,0.));
#88540=CARTESIAN_POINT('Ctrl Pts',(45.0661422374956,-18.7262623689254,20.));
#88541=CARTESIAN_POINT('Ctrl Pts',(45.050415398505,-18.7561478020964,0.));
#88542=CARTESIAN_POINT('Ctrl Pts',(45.050415398505,-18.7561478020964,20.));
#88543=CARTESIAN_POINT('Ctrl Pts',(45.0346684865594,-18.7860214010651,0.));
#88544=CARTESIAN_POINT('Ctrl Pts',(45.0346684865594,-18.7860214010651,20.));
#88545=CARTESIAN_POINT('Ctrl Pts',(45.0189015098976,-18.815883152041,0.));
#88546=CARTESIAN_POINT('Ctrl Pts',(45.0189015098976,-18.815883152041,20.));
#88547=CARTESIAN_POINT('Ctrl Pts',(45.0031144767678,-18.8457330412389,0.));
#88548=CARTESIAN_POINT('Ctrl Pts',(45.0031144767678,-18.8457330412389,20.));
#88549=CARTESIAN_POINT('Ctrl Pts',(44.987307395428,-18.8755710548788,0.));
#88550=CARTESIAN_POINT('Ctrl Pts',(44.987307395428,-18.8755710548788,20.));
#88551=CARTESIAN_POINT('Ctrl Pts',(44.971480274146,-18.9053971791858,0.));
#88552=CARTESIAN_POINT('Ctrl Pts',(44.971480274146,-18.9053971791858,20.));
#88553=CARTESIAN_POINT('Ctrl Pts',(44.9556331211993,-18.9352114003906,0.));
#88554=CARTESIAN_POINT('Ctrl Pts',(44.9556331211993,-18.9352114003906,20.));
#88555=CARTESIAN_POINT('Ctrl Pts',(44.9397659448752,-18.9650137047294,0.));
#88556=CARTESIAN_POINT('Ctrl Pts',(44.9397659448752,-18.9650137047294,20.));
#88557=CARTESIAN_POINT('Ctrl Pts',(44.9238787534705,-18.9948040784434,0.));
#88558=CARTESIAN_POINT('Ctrl Pts',(44.9238787534705,-18.9948040784434,20.));
#88559=CARTESIAN_POINT('Ctrl Pts',(44.9079715552916,-19.0245825077798,0.));
#88560=CARTESIAN_POINT('Ctrl Pts',(44.9079715552916,-19.0245825077798,20.));
#88561=CARTESIAN_POINT('Ctrl Pts',(44.8920443586544,-19.0543489789907,0.));
#88562=CARTESIAN_POINT('Ctrl Pts',(44.8920443586544,-19.0543489789907,20.));
#88563=CARTESIAN_POINT('Ctrl Pts',(44.8760971718851,-19.0841034783341,0.));
#88564=CARTESIAN_POINT('Ctrl Pts',(44.8760971718851,-19.0841034783341,20.));
#88565=CARTESIAN_POINT('Ctrl Pts',(44.8601300033192,-19.1138459920731,0.));
#88566=CARTESIAN_POINT('Ctrl Pts',(44.8601300033192,-19.1138459920731,20.));
#88567=CARTESIAN_POINT('Ctrl Pts',(44.8441428613021,-19.143576506476,0.));
#88568=CARTESIAN_POINT('Ctrl Pts',(44.8441428613021,-19.143576506476,20.));
#88569=CARTESIAN_POINT('Ctrl Pts',(44.8281357541891,-19.1732950078169,0.));
#88570=CARTESIAN_POINT('Ctrl Pts',(44.8281357541891,-19.1732950078169,20.));
#88571=CARTESIAN_POINT('Ctrl Pts',(44.8121086903447,-19.2030014823748,0.));
#88572=CARTESIAN_POINT('Ctrl Pts',(44.8121086903447,-19.2030014823748,20.));
#88573=CARTESIAN_POINT('Ctrl Pts',(44.7960616781431,-19.2326959164344,0.));
#88574=CARTESIAN_POINT('Ctrl Pts',(44.7960616781431,-19.2326959164344,20.));
#88575=CARTESIAN_POINT('Ctrl Pts',(44.7799947259683,-19.2623782962859,0.));
#88576=CARTESIAN_POINT('Ctrl Pts',(44.7799947259683,-19.2623782962859,20.));
#88577=CARTESIAN_POINT('Ctrl Pts',(44.7639078422139,-19.2920486082247,0.));
#88578=CARTESIAN_POINT('Ctrl Pts',(44.7639078422139,-19.2920486082247,20.));
#88579=CARTESIAN_POINT('Ctrl Pts',(44.7478010352831,-19.321706838552,0.));
#88580=CARTESIAN_POINT('Ctrl Pts',(44.7478010352831,-19.321706838552,20.));
#88581=CARTESIAN_POINT('Ctrl Pts',(44.731674313589,-19.3513529735741,0.));
#88582=CARTESIAN_POINT('Ctrl Pts',(44.731674313589,-19.3513529735741,20.));
#88583=CARTESIAN_POINT('Ctrl Pts',(44.7155276855546,-19.3809869996033,0.));
#88584=CARTESIAN_POINT('Ctrl Pts',(44.7155276855546,-19.3809869996033,20.));
#88585=CARTESIAN_POINT('Ctrl Pts',(44.6993611596123,-19.4106089029568,0.));
#88586=CARTESIAN_POINT('Ctrl Pts',(44.6993611596123,-19.4106089029568,20.));
#88587=CARTESIAN_POINT('Ctrl Pts',(44.6831747442042,-19.4402186699576,0.));
#88588=CARTESIAN_POINT('Ctrl Pts',(44.6831747442042,-19.4402186699576,20.));
#88589=CARTESIAN_POINT('Ctrl Pts',(44.6669684477819,-19.4698162869338,0.));
#88590=CARTESIAN_POINT('Ctrl Pts',(44.6669684477819,-19.4698162869338,20.));
#88591=CARTESIAN_POINT('Ctrl Pts',(44.6507422788067,-19.4994017402193,0.));
#88592=CARTESIAN_POINT('Ctrl Pts',(44.6507422788067,-19.4994017402193,20.));
#88593=CARTESIAN_POINT('Ctrl Pts',(44.6344962457493,-19.5289750161534,0.));
#88594=CARTESIAN_POINT('Ctrl Pts',(44.6344962457493,-19.5289750161534,20.));
#88595=CARTESIAN_POINT('Ctrl Pts',(44.6182303570903,-19.5585361010809,0.));
#88596=CARTESIAN_POINT('Ctrl Pts',(44.6182303570903,-19.5585361010809,20.));
#88597=CARTESIAN_POINT('Ctrl Pts',(44.60194462132,-19.5880849813526,0.));
#88598=CARTESIAN_POINT('Ctrl Pts',(44.60194462132,-19.5880849813526,20.));
#88599=CARTESIAN_POINT('Ctrl Pts',(44.5856390469384,-19.6176216433241,0.));
#88600=CARTESIAN_POINT('Ctrl Pts',(44.5856390469384,-19.6176216433241,20.));
#88601=CARTESIAN_POINT('Ctrl Pts',(44.5693136424548,-19.6471460733569,0.));
#88602=CARTESIAN_POINT('Ctrl Pts',(44.5693136424548,-19.6471460733569,20.));
#88603=CARTESIAN_POINT('Ctrl Pts',(44.5529684163885,-19.6766582578175,0.));
#88604=CARTESIAN_POINT('Ctrl Pts',(44.5529684163885,-19.6766582578175,20.));
#88605=CARTESIAN_POINT('Ctrl Pts',(44.5366033772681,-19.7061581830785,0.));
#88606=CARTESIAN_POINT('Ctrl Pts',(44.5366033772681,-19.7061581830785,20.));
#88607=CARTESIAN_POINT('Ctrl Pts',(44.5202185336324,-19.7356458355178,0.));
#88608=CARTESIAN_POINT('Ctrl Pts',(44.5202185336324,-19.7356458355178,20.));
#88609=CARTESIAN_POINT('Ctrl Pts',(44.5038138940293,-19.7651212015191,0.));
#88610=CARTESIAN_POINT('Ctrl Pts',(44.5038138940293,-19.7651212015191,20.));
#88611=CARTESIAN_POINT('Ctrl Pts',(44.4873894670167,-19.7945842674717,0.));
#88612=CARTESIAN_POINT('Ctrl Pts',(44.4873894670167,-19.7945842674717,20.));
#88613=CARTESIAN_POINT('Ctrl Pts',(44.4709452611615,-19.8240350197702,0.));
#88614=CARTESIAN_POINT('Ctrl Pts',(44.4709452611615,-19.8240350197702,20.));
#88615=CARTESIAN_POINT('Ctrl Pts',(44.4544812850403,-19.8534734448147,0.));
#88616=CARTESIAN_POINT('Ctrl Pts',(44.4544812850403,-19.8534734448147,20.));
#88617=CARTESIAN_POINT('Ctrl Pts',(44.4379975472397,-19.8828995290107,0.));
#88618=CARTESIAN_POINT('Ctrl Pts',(44.4379975472397,-19.8828995290107,20.));
#88619=CARTESIAN_POINT('Ctrl Pts',(44.4214940563556,-19.9123132587698,0.));
#88620=CARTESIAN_POINT('Ctrl Pts',(44.4214940563556,-19.9123132587698,20.));
#88621=CARTESIAN_POINT('Ctrl Pts',(44.4049708209939,-19.9417146205087,0.));
#88622=CARTESIAN_POINT('Ctrl Pts',(44.4049708209939,-19.9417146205087,20.));
#88623=CARTESIAN_POINT('Ctrl Pts',(44.3884278497697,-19.9711036006504,0.));
#88624=CARTESIAN_POINT('Ctrl Pts',(44.3884278497697,-19.9711036006504,20.));
#88625=CARTESIAN_POINT('Ctrl Pts',(44.371865151308,-20.0004801856229,0.));
#88626=CARTESIAN_POINT('Ctrl Pts',(44.371865151308,-20.0004801856229,20.));
#88627=CARTESIAN_POINT('Ctrl Pts',(44.3552827342435,-20.0298443618602,0.));
#88628=CARTESIAN_POINT('Ctrl Pts',(44.3552827342435,-20.0298443618602,20.));
#88629=CARTESIAN_POINT('Ctrl Pts',(44.3386806072204,-20.0591961158019,0.));
#88630=CARTESIAN_POINT('Ctrl Pts',(44.3386806072204,-20.0591961158019,20.));
#88631=CARTESIAN_POINT('Ctrl Pts',(44.3220587788923,-20.0885354338929,0.));
#88632=CARTESIAN_POINT('Ctrl Pts',(44.3220587788923,-20.0885354338929,20.));
#88633=CARTESIAN_POINT('Ctrl Pts',(44.3054172579221,-20.117862302584,0.));
#88634=CARTESIAN_POINT('Ctrl Pts',(44.3054172579221,-20.117862302584,20.));
#88635=CARTESIAN_POINT('Ctrl Pts',(44.2887560529826,-20.1471767083313,0.));
#88636=CARTESIAN_POINT('Ctrl Pts',(44.2887560529826,-20.1471767083313,20.));
#88637=CARTESIAN_POINT('Ctrl Pts',(44.2720751727557,-20.1764786375963,0.));
#88638=CARTESIAN_POINT('Ctrl Pts',(44.2720751727557,-20.1764786375963,20.));
#88639=CARTESIAN_POINT('Ctrl Pts',(44.2553746259333,-20.2057680768465,0.));
#88640=CARTESIAN_POINT('Ctrl Pts',(44.2553746259333,-20.2057680768465,20.));
#88641=CARTESIAN_POINT('Ctrl Pts',(44.238654421217,-20.2350450125552,0.));
#88642=CARTESIAN_POINT('Ctrl Pts',(44.238654421217,-20.2350450125552,20.));
#88643=CARTESIAN_POINT('Ctrl Pts',(44.221914567318,-20.2643094312016,0.));
#88644=CARTESIAN_POINT('Ctrl Pts',(44.221914567318,-20.2643094312016,20.));
#88645=CARTESIAN_POINT('Ctrl Pts',(44.205155072957,-20.2935613192706,0.));
#88646=CARTESIAN_POINT('Ctrl Pts',(44.205155072957,-20.2935613192706,20.));
#88647=CARTESIAN_POINT('Ctrl Pts',(44.1883759468646,-20.3228006632528,0.));
#88648=CARTESIAN_POINT('Ctrl Pts',(44.1883759468646,-20.3228006632528,20.));
#88649=CARTESIAN_POINT('Ctrl Pts',(44.1715771977807,-20.3520274496444,0.));
#88650=CARTESIAN_POINT('Ctrl Pts',(44.1715771977807,-20.3520274496444,20.));
#88651=CARTESIAN_POINT('Ctrl Pts',(44.1547588344544,-20.3812416649468,0.));
#88652=CARTESIAN_POINT('Ctrl Pts',(44.1547588344544,-20.3812416649468,20.));
#88653=CARTESIAN_POINT('Ctrl Pts',(44.1379208656442,-20.4104432956673,0.));
#88654=CARTESIAN_POINT('Ctrl Pts',(44.1379208656442,-20.4104432956673,20.));
#88655=CARTESIAN_POINT('Ctrl Pts',(44.1210633001184,-20.4396323283186,0.));
#88656=CARTESIAN_POINT('Ctrl Pts',(44.1210633001184,-20.4396323283186,20.));
#88657=CARTESIAN_POINT('Ctrl Pts',(44.1041861466545,-20.4688087494191,0.));
#88658=CARTESIAN_POINT('Ctrl Pts',(44.1041861466545,-20.4688087494191,20.));
#88659=CARTESIAN_POINT('Ctrl Pts',(44.0872894140398,-20.4979725454933,0.));
#88660=CARTESIAN_POINT('Ctrl Pts',(44.0872894140398,-20.4979725454933,20.));
#88661=CARTESIAN_POINT('Ctrl Pts',(44.0703731110714,-20.5271237030716,0.));
#88662=CARTESIAN_POINT('Ctrl Pts',(44.0703731110714,-20.5271237030716,20.));
#88663=CARTESIAN_POINT('Ctrl Pts',(44.053437246556,-20.5562622086905,0.));
#88664=CARTESIAN_POINT('Ctrl Pts',(44.053437246556,-20.5562622086905,20.));
#88665=CARTESIAN_POINT('Ctrl Pts',(44.03648182931,-20.5853880488919,0.));
#88666=CARTESIAN_POINT('Ctrl Pts',(44.03648182931,-20.5853880488919,20.));
#88667=CARTESIAN_POINT('Ctrl Pts',(44.0195068681592,-20.6145012102233,0.));
#88668=CARTESIAN_POINT('Ctrl Pts',(44.0195068681592,-20.6145012102233,20.));
#88669=CARTESIAN_POINT('Ctrl Pts',(44.0025123719387,-20.6436016792381,0.));
#88670=CARTESIAN_POINT('Ctrl Pts',(44.0025123719387,-20.6436016792381,20.));
#88671=CARTESIAN_POINT('Ctrl Pts',(43.9854983494929,-20.6726894424949,0.));
#88672=CARTESIAN_POINT('Ctrl Pts',(43.9854983494929,-20.6726894424949,20.));
#88673=CARTESIAN_POINT('Ctrl Pts',(43.9684648096756,-20.7017644865585,0.));
#88674=CARTESIAN_POINT('Ctrl Pts',(43.9684648096756,-20.7017644865585,20.));
#88675=CARTESIAN_POINT('Ctrl Pts',(43.9514117613501,-20.7308267979991,0.));
#88676=CARTESIAN_POINT('Ctrl Pts',(43.9514117613501,-20.7308267979991,20.));
#88677=CARTESIAN_POINT('Ctrl Pts',(43.9343392133895,-20.7598763633934,0.));
#88678=CARTESIAN_POINT('Ctrl Pts',(43.9343392133895,-20.7598763633934,20.));
#88679=CARTESIAN_POINT('Ctrl Pts',(43.9172471746767,-20.7889131693233,0.));
#88680=CARTESIAN_POINT('Ctrl Pts',(43.9172471746767,-20.7889131693233,20.));
#88681=CARTESIAN_POINT('Ctrl Pts',(43.9001356541037,-20.817937202377,0.));
#88682=CARTESIAN_POINT('Ctrl Pts',(43.9001356541037,-20.817937202377,20.));
#88683=CARTESIAN_POINT('Ctrl Pts',(43.8830046605723,-20.8469484491482,0.));
#88684=CARTESIAN_POINT('Ctrl Pts',(43.8830046605723,-20.8469484491482,20.));
#88685=CARTESIAN_POINT('Ctrl Pts',(43.8658542029936,-20.8759468962364,0.));
#88686=CARTESIAN_POINT('Ctrl Pts',(43.8658542029936,-20.8759468962364,20.));
#88687=CARTESIAN_POINT('Ctrl Pts',(43.8486842902882,-20.9049325302471,0.));
#88688=CARTESIAN_POINT('Ctrl Pts',(43.8486842902882,-20.9049325302471,20.));
#88689=CARTESIAN_POINT('Ctrl Pts',(43.8314949313861,-20.9339053377914,0.));
#88690=CARTESIAN_POINT('Ctrl Pts',(43.8314949313861,-20.9339053377914,20.));
#88691=CARTESIAN_POINT('Ctrl Pts',(43.8142861352268,-20.9628653054863,0.));
#88692=CARTESIAN_POINT('Ctrl Pts',(43.8142861352268,-20.9628653054863,20.));
#88693=CARTESIAN_POINT('Ctrl Pts',(43.7970579107591,-20.9918124199547,0.));
#88694=CARTESIAN_POINT('Ctrl Pts',(43.7970579107591,-20.9918124199547,20.));
#88695=CARTESIAN_POINT('Ctrl Pts',(43.7798102669417,-21.0207466678254,0.));
#88696=CARTESIAN_POINT('Ctrl Pts',(43.7798102669417,-21.0207466678254,20.));
#88697=CARTESIAN_POINT('Ctrl Pts',(43.7625432127426,-21.0496680357328,0.));
#88698=CARTESIAN_POINT('Ctrl Pts',(43.7625432127426,-21.0496680357328,20.));
#88699=CARTESIAN_POINT('Ctrl Pts',(43.7452567571393,-21.0785765103173,0.));
#88700=CARTESIAN_POINT('Ctrl Pts',(43.7452567571393,-21.0785765103173,20.));
#88701=CARTESIAN_POINT('Ctrl Pts',(43.7279509091188,-21.1074720782252,0.));
#88702=CARTESIAN_POINT('Ctrl Pts',(43.7279509091188,-21.1074720782252,20.));
#88703=CARTESIAN_POINT('Ctrl Pts',(43.7106256776774,-21.1363547261089,0.));
#88704=CARTESIAN_POINT('Ctrl Pts',(43.7106256776774,-21.1363547261089,20.));
#88705=CARTESIAN_POINT('Ctrl Pts',(43.6932810718209,-21.1652244406266,0.));
#88706=CARTESIAN_POINT('Ctrl Pts',(43.6932810718209,-21.1652244406266,20.));
#88707=CARTESIAN_POINT('Ctrl Pts',(43.6759171005641,-21.1940812084419,0.));
#88708=CARTESIAN_POINT('Ctrl Pts',(43.6759171005641,-21.1940812084419,20.));
#88709=CARTESIAN_POINT('Ctrl Pts',(43.658533772932,-21.2229250162246,0.));
#88710=CARTESIAN_POINT('Ctrl Pts',(43.658533772932,-21.2229250162246,20.));
#88711=CARTESIAN_POINT('Ctrl Pts',(43.6411310979584,-21.2517558506503,0.));
#88712=CARTESIAN_POINT('Ctrl Pts',(43.6411310979584,-21.2517558506503,20.));
#88713=CARTESIAN_POINT('Ctrl Pts',(43.6237090846874,-21.2805736984008,0.));
#88714=CARTESIAN_POINT('Ctrl Pts',(43.6237090846874,-21.2805736984008,20.));
#88715=CARTESIAN_POINT('Ctrl Pts',(43.6062677421718,-21.3093785461635,0.));
#88716=CARTESIAN_POINT('Ctrl Pts',(43.6062677421718,-21.3093785461635,20.));
#88717=CARTESIAN_POINT('Ctrl Pts',(43.5888070794743,-21.3381703806324,0.));
#88718=CARTESIAN_POINT('Ctrl Pts',(43.5888070794743,-21.3381703806324,20.));
#88719=CARTESIAN_POINT('Ctrl Pts',(43.571327105667,-21.3669491885068,0.));
#88720=CARTESIAN_POINT('Ctrl Pts',(43.571327105667,-21.3669491885068,20.));
#88721=CARTESIAN_POINT('Ctrl Pts',(43.5538278298311,-21.3957149564922,0.));
#88722=CARTESIAN_POINT('Ctrl Pts',(43.5538278298311,-21.3957149564922,20.));
#88723=CARTESIAN_POINT('Ctrl Pts',(43.5363092610574,-21.4244676712999,0.));
#88724=CARTESIAN_POINT('Ctrl Pts',(43.5363092610574,-21.4244676712999,20.));
#88725=CARTESIAN_POINT('Ctrl Pts',(43.5187714084458,-21.4532073196468,0.));
#88726=CARTESIAN_POINT('Ctrl Pts',(43.5187714084458,-21.4532073196468,20.));
#88727=CARTESIAN_POINT('Ctrl Pts',(43.5012142811058,-21.4819338882558,0.));
#88728=CARTESIAN_POINT('Ctrl Pts',(43.5012142811058,-21.4819338882558,20.));
#88729=CARTESIAN_POINT('Ctrl Pts',(43.4836378881563,-21.5106473638561,0.));
#88730=CARTESIAN_POINT('Ctrl Pts',(43.4836378881563,-21.5106473638561,20.));
#88731=CARTESIAN_POINT('Ctrl Pts',(43.4660422387257,-21.5393477331829,0.));
#88732=CARTESIAN_POINT('Ctrl Pts',(43.4660422387257,-21.5393477331829,20.));
#88733=CARTESIAN_POINT('Ctrl Pts',(43.4484273419519,-21.5680349829774,0.));
#88734=CARTESIAN_POINT('Ctrl Pts',(43.4484273419519,-21.5680349829774,20.));
#88735=CARTESIAN_POINT('Ctrl Pts',(43.4307932069823,-21.5967090999869,0.));
#88736=CARTESIAN_POINT('Ctrl Pts',(43.4307932069823,-21.5967090999869,20.));
#88737=CARTESIAN_POINT('Ctrl Pts',(43.4131398429739,-21.6253700709647,0.));
#88738=CARTESIAN_POINT('Ctrl Pts',(43.4131398429739,-21.6253700709647,20.));
#88739=CARTESIAN_POINT('Ctrl Pts',(43.3954672590924,-21.6540178826698,0.));
#88740=CARTESIAN_POINT('Ctrl Pts',(43.3954672590924,-21.6540178826698,20.));
#88741=CARTESIAN_POINT('Ctrl Pts',(43.3777754645132,-21.682652521867,0.));
#88742=CARTESIAN_POINT('Ctrl Pts',(43.3777754645132,-21.682652521867,20.));
#88743=CARTESIAN_POINT('Ctrl Pts',(43.3600644684208,-21.7112739753274,0.));
#88744=CARTESIAN_POINT('Ctrl Pts',(43.3600644684208,-21.7112739753274,20.));
#88745=CARTESIAN_POINT('Ctrl Pts',(43.3423342800096,-21.7398822298281,0.));
#88746=CARTESIAN_POINT('Ctrl Pts',(43.3423342800096,-21.7398822298281,20.));
#88747=CARTESIAN_POINT('Ctrl Pts',(43.3245849084831,-21.7684772721522,0.));
#88748=CARTESIAN_POINT('Ctrl Pts',(43.3245849084831,-21.7684772721522,20.));
#88749=CARTESIAN_POINT('Ctrl Pts',(43.3068163630542,-21.7970590890891,0.));
#88750=CARTESIAN_POINT('Ctrl Pts',(43.3068163630542,-21.7970590890891,20.));
#88751=CARTESIAN_POINT('Ctrl Pts',(43.2890286529453,-21.825627667434,0.));
#88752=CARTESIAN_POINT('Ctrl Pts',(43.2890286529453,-21.825627667434,20.));
#88753=CARTESIAN_POINT('Ctrl Pts',(43.271221787388,-21.854182993988,0.));
#88754=CARTESIAN_POINT('Ctrl Pts',(43.271221787388,-21.854182993988,20.));
#88755=CARTESIAN_POINT('Ctrl Pts',(43.2533957756234,-21.8827250555584,0.));
#88756=CARTESIAN_POINT('Ctrl Pts',(43.2533957756234,-21.8827250555584,20.));
#88757=CARTESIAN_POINT('Ctrl Pts',(43.2355506269018,-21.9112538389586,0.));
#88758=CARTESIAN_POINT('Ctrl Pts',(43.2355506269018,-21.9112538389586,20.));
#88759=CARTESIAN_POINT('Ctrl Pts',(43.217686350483,-21.939769331008,0.));
#88760=CARTESIAN_POINT('Ctrl Pts',(43.217686350483,-21.939769331008,20.));
#88761=CARTESIAN_POINT('Ctrl Pts',(43.1998029556363,-21.9682715185322,0.));
#88762=CARTESIAN_POINT('Ctrl Pts',(43.1998029556363,-21.9682715185322,20.));
#88763=CARTESIAN_POINT('Ctrl Pts',(43.1819004516401,-21.9967603883628,0.));
#88764=CARTESIAN_POINT('Ctrl Pts',(43.1819004516401,-21.9967603883628,20.));
#88765=CARTESIAN_POINT('Ctrl Pts',(43.1639788477821,-22.0252359273374,0.));
#88766=CARTESIAN_POINT('Ctrl Pts',(43.1639788477821,-22.0252359273374,20.));
#88767=CARTESIAN_POINT('Ctrl Pts',(43.1460381533593,-22.0536981222997,0.));
#88768=CARTESIAN_POINT('Ctrl Pts',(43.1460381533593,-22.0536981222997,20.));
#88769=CARTESIAN_POINT('Ctrl Pts',(43.1280783776784,-22.0821469600998,0.));
#88770=CARTESIAN_POINT('Ctrl Pts',(43.1280783776784,-22.0821469600998,20.));
#88771=CARTESIAN_POINT('Ctrl Pts',(43.1100995300552,-22.1105824275933,0.));
#88772=CARTESIAN_POINT('Ctrl Pts',(43.1100995300552,-22.1105824275933,20.));
#88773=CARTESIAN_POINT('Ctrl Pts',(43.0921016198148,-22.1390045116426,0.));
#88774=CARTESIAN_POINT('Ctrl Pts',(43.0921016198148,-22.1390045116426,20.));
#88775=CARTESIAN_POINT('Ctrl Pts',(43.0740846562917,-22.1674131991155,0.));
#88776=CARTESIAN_POINT('Ctrl Pts',(43.0740846562917,-22.1674131991155,20.));
#88777=CARTESIAN_POINT('Ctrl Pts',(43.0560486488298,-22.1958084768868,0.));
#88778=CARTESIAN_POINT('Ctrl Pts',(43.0560486488298,-22.1958084768868,20.));
#88779=CARTESIAN_POINT('Ctrl Pts',(43.0379936067822,-22.2241903318366,0.));
#88780=CARTESIAN_POINT('Ctrl Pts',(43.0379936067822,-22.2241903318366,20.));
#88781=CARTESIAN_POINT('Ctrl Pts',(43.0199195395114,-22.252558750852,0.));
#88782=CARTESIAN_POINT('Ctrl Pts',(43.0199195395114,-22.252558750852,20.));
#88783=CARTESIAN_POINT('Ctrl Pts',(43.0018264563892,-22.2809137208256,0.));
#88784=CARTESIAN_POINT('Ctrl Pts',(43.0018264563892,-22.2809137208256,20.));
#88785=CARTESIAN_POINT('Ctrl Pts',(42.9837143667967,-22.3092552286565,0.));
#88786=CARTESIAN_POINT('Ctrl Pts',(42.9837143667967,-22.3092552286565,20.));
#88787=CARTESIAN_POINT('Ctrl Pts',(42.965583280124,-22.3375832612492,0.));
#88788=CARTESIAN_POINT('Ctrl Pts',(42.965583280124,-22.3375832612492,20.));
#88789=CARTESIAN_POINT('Ctrl Pts',(42.947433205771,-22.3658978055149,0.));
#88790=CARTESIAN_POINT('Ctrl Pts',(42.947433205771,-22.3658978055149,20.));
#88791=CARTESIAN_POINT('Ctrl Pts',(42.9292641531465,-22.3941988483709,0.));
#88792=CARTESIAN_POINT('Ctrl Pts',(42.9292641531465,-22.3941988483709,20.));
#88793=CARTESIAN_POINT('Ctrl Pts',(42.9110761316689,-22.4224863767407,0.));
#88794=CARTESIAN_POINT('Ctrl Pts',(42.9110761316689,-22.4224863767407,20.));
#88795=CARTESIAN_POINT('Ctrl Pts',(42.8928691507659,-22.4507603775546,0.));
#88796=CARTESIAN_POINT('Ctrl Pts',(42.8928691507659,-22.4507603775546,20.));
#88797=CARTESIAN_POINT('Ctrl Pts',(42.8746432198743,-22.4790208377489,0.));
#88798=CARTESIAN_POINT('Ctrl Pts',(42.8746432198743,-22.4790208377489,20.));
#88799=CARTESIAN_POINT('Ctrl Pts',(42.8563983484404,-22.5072677442656,0.));
#88800=CARTESIAN_POINT('Ctrl Pts',(42.8563983484404,-22.5072677442656,20.));
#88801=CARTESIAN_POINT('Ctrl Pts',(42.8381345459193,-22.5355010840531,0.));
#88802=CARTESIAN_POINT('Ctrl Pts',(42.8381345459193,-22.5355010840531,20.));
#88803=CARTESIAN_POINT('Ctrl Pts',(42.8198518217756,-22.5637208440656,0.));
#88804=CARTESIAN_POINT('Ctrl Pts',(42.8198518217756,-22.5637208440656,20.));
#88805=CARTESIAN_POINT('Ctrl Pts',(42.8015501854832,-22.5919270112639,0.));
#88806=CARTESIAN_POINT('Ctrl Pts',(42.8015501854832,-22.5919270112639,20.));
#88807=CARTESIAN_POINT('Ctrl Pts',(42.7832296465255,-22.6201195726151,0.));
#88808=CARTESIAN_POINT('Ctrl Pts',(42.7832296465255,-22.6201195726151,20.));
#88809=CARTESIAN_POINT('Ctrl Pts',(42.7648902143955,-22.6482985150925,0.));
#88810=CARTESIAN_POINT('Ctrl Pts',(42.7648902143955,-22.6482985150925,20.));
#88811=CARTESIAN_POINT('Ctrl Pts',(42.7465318985949,-22.6764638256759,0.));
#88812=CARTESIAN_POINT('Ctrl Pts',(42.7465318985949,-22.6764638256759,20.));
#88813=CARTESIAN_POINT('Ctrl Pts',(42.7281547086347,-22.7046154913512,0.));
#88814=CARTESIAN_POINT('Ctrl Pts',(42.7281547086347,-22.7046154913512,20.));
#88815=CARTESIAN_POINT('Ctrl Pts',(42.7097586540349,-22.7327534991101,0.));
#88816=CARTESIAN_POINT('Ctrl Pts',(42.7097586540349,-22.7327534991101,20.));
#88817=CARTESIAN_POINT('Ctrl Pts',(42.6913437443248,-22.7608778359508,0.));
#88818=CARTESIAN_POINT('Ctrl Pts',(42.6913437443248,-22.7608778359508,20.));
#88819=CARTESIAN_POINT('Ctrl Pts',(42.6729099890431,-22.788988488878,0.));
#88820=CARTESIAN_POINT('Ctrl Pts',(42.6729099890431,-22.788988488878,20.));
#88821=CARTESIAN_POINT('Ctrl Pts',(42.6544573977378,-22.8170854449024,0.));
#88822=CARTESIAN_POINT('Ctrl Pts',(42.6544573977378,-22.8170854449024,20.));
#88823=CARTESIAN_POINT('Ctrl Pts',(42.6359859799663,-22.845168691041,0.));
#88824=CARTESIAN_POINT('Ctrl Pts',(42.6359859799663,-22.845168691041,20.));
#88825=CARTESIAN_POINT('Ctrl Pts',(42.6174957452953,-22.8732382143175,0.));
#88826=CARTESIAN_POINT('Ctrl Pts',(42.6174957452953,-22.8732382143175,20.));
#88827=CARTESIAN_POINT('Ctrl Pts',(42.5989867033005,-22.9012940017616,0.));
#88828=CARTESIAN_POINT('Ctrl Pts',(42.5989867033005,-22.9012940017616,20.));
#88829=CARTESIAN_POINT('Ctrl Pts',(42.5804588635669,-22.9293360404095,0.));
#88830=CARTESIAN_POINT('Ctrl Pts',(42.5804588635669,-22.9293360404095,20.));
#88831=CARTESIAN_POINT('Ctrl Pts',(42.5619122356886,-22.9573643173034,0.));
#88832=CARTESIAN_POINT('Ctrl Pts',(42.5619122356886,-22.9573643173034,20.));
#88833=CARTESIAN_POINT('Ctrl Pts',(42.5433468292689,-22.9853788194919,0.));
#88834=CARTESIAN_POINT('Ctrl Pts',(42.5433468292689,-22.9853788194919,20.));
#88835=CARTESIAN_POINT('Ctrl Pts',(42.5247626539203,-23.0133795340299,0.));
#88836=CARTESIAN_POINT('Ctrl Pts',(42.5247626539203,-23.0133795340299,20.));
#88837=CARTESIAN_POINT('Ctrl Pts',(42.5061597192647,-23.0413664479785,0.));
#88838=CARTESIAN_POINT('Ctrl Pts',(42.5061597192647,-23.0413664479785,20.));
#88839=CARTESIAN_POINT('Ctrl Pts',(42.4875380349329,-23.0693395484056,0.));
#88840=CARTESIAN_POINT('Ctrl Pts',(42.4875380349329,-23.0693395484056,20.));
#88841=CARTESIAN_POINT('Ctrl Pts',(42.4688976105654,-23.097298822385,0.));
#88842=CARTESIAN_POINT('Ctrl Pts',(42.4688976105654,-23.097298822385,20.));
#88843=CARTESIAN_POINT('Ctrl Pts',(42.4502384558115,-23.1252442569971,0.));
#88844=CARTESIAN_POINT('Ctrl Pts',(42.4502384558115,-23.1252442569971,20.));
#88845=CARTESIAN_POINT('Ctrl Pts',(42.4315605803297,-23.1531758393284,0.));
#88846=CARTESIAN_POINT('Ctrl Pts',(42.4315605803297,-23.1531758393284,20.));
#88847=CARTESIAN_POINT('Ctrl Pts',(42.4128639937879,-23.1810935564721,0.));
#88848=CARTESIAN_POINT('Ctrl Pts',(42.4128639937879,-23.1810935564721,20.));
#88849=CARTESIAN_POINT('Ctrl Pts',(42.3941487058631,-23.2089973955278,0.));
#88850=CARTESIAN_POINT('Ctrl Pts',(42.3941487058631,-23.2089973955278,20.));
#88851=CARTESIAN_POINT('Ctrl Pts',(42.3754147262417,-23.2368873436013,0.));
#88852=CARTESIAN_POINT('Ctrl Pts',(42.3754147262417,-23.2368873436013,20.));
#88853=CARTESIAN_POINT('Ctrl Pts',(42.3566620646188,-23.2647633878047,0.));
#88854=CARTESIAN_POINT('Ctrl Pts',(42.3566620646188,-23.2647633878047,20.));
#88855=CARTESIAN_POINT('Ctrl Pts',(42.3378907306988,-23.2926255152563,0.));
#88856=CARTESIAN_POINT('Ctrl Pts',(42.3378907306988,-23.2926255152563,20.));
#88857=CARTESIAN_POINT('Ctrl Pts',(42.3191007341954,-23.320473713081,0.));
#88858=CARTESIAN_POINT('Ctrl Pts',(42.3191007341954,-23.320473713081,20.));
#88859=CARTESIAN_POINT('Ctrl Pts',(42.3002920848317,-23.3483079684104,0.));
#88860=CARTESIAN_POINT('Ctrl Pts',(42.3002920848317,-23.3483079684104,20.));
#88861=CARTESIAN_POINT('Ctrl Pts',(42.2814647923395,-23.3761282683822,0.));
#88862=CARTESIAN_POINT('Ctrl Pts',(42.2814647923395,-23.3761282683822,20.));
#88863=CARTESIAN_POINT('Ctrl Pts',(42.2626188664603,-23.4039346001409,0.));
#88864=CARTESIAN_POINT('Ctrl Pts',(42.2626188664603,-23.4039346001409,20.));
#88865=CARTESIAN_POINT('Ctrl Pts',(42.2437543169442,-23.4317269508371,0.));
#88866=CARTESIAN_POINT('Ctrl Pts',(42.2437543169442,-23.4317269508371,20.));
#88867=CARTESIAN_POINT('Ctrl Pts',(42.2248711535508,-23.4595053076278,0.));
#88868=CARTESIAN_POINT('Ctrl Pts',(42.2248711535508,-23.4595053076278,20.));
#88869=CARTESIAN_POINT('Ctrl Pts',(42.2059693860486,-23.4872696576759,0.));
#88870=CARTESIAN_POINT('Ctrl Pts',(42.2059693860486,-23.4872696576759,20.));
#88871=CARTESIAN_POINT('Ctrl Pts',(42.1870490242153,-23.5150199881515,0.));
#88872=CARTESIAN_POINT('Ctrl Pts',(42.1870490242153,-23.5150199881515,20.));
#88873=CARTESIAN_POINT('Ctrl Pts',(42.1681100778379,-23.5427562862308,0.));
#88874=CARTESIAN_POINT('Ctrl Pts',(42.1681100778379,-23.5427562862308,20.));
#88875=CARTESIAN_POINT('Ctrl Pts',(42.1491525567126,-23.5704785390969,0.));
#88876=CARTESIAN_POINT('Ctrl Pts',(42.1491525567126,-23.5704785390969,20.));
#88877=CARTESIAN_POINT('Ctrl Pts',(42.1301764706447,-23.5981867339395,0.));
#88878=CARTESIAN_POINT('Ctrl Pts',(42.1301764706447,-23.5981867339395,20.));
#88879=CARTESIAN_POINT('Ctrl Pts',(42.1111818294483,-23.6258808579543,0.));
#88880=CARTESIAN_POINT('Ctrl Pts',(42.1111818294483,-23.6258808579543,20.));
#88881=CARTESIAN_POINT('Ctrl Pts',(42.0921686429469,-23.6535608983436,0.));
#88882=CARTESIAN_POINT('Ctrl Pts',(42.0921686429469,-23.6535608983436,20.));
#88883=CARTESIAN_POINT('Ctrl Pts',(42.0731369209731,-23.6812268423159,0.));
#88884=CARTESIAN_POINT('Ctrl Pts',(42.0731369209731,-23.6812268423159,20.));
#88885=CARTESIAN_POINT('Ctrl Pts',(42.0540866733685,-23.7088786770864,0.));
#88886=CARTESIAN_POINT('Ctrl Pts',(42.0540866733685,-23.7088786770864,20.));
#88887=CARTESIAN_POINT('Ctrl Pts',(42.0350179099839,-23.7365163898768,0.));
#88888=CARTESIAN_POINT('Ctrl Pts',(42.0350179099839,-23.7365163898768,20.));
#88889=CARTESIAN_POINT('Ctrl Pts',(42.0159306406794,-23.7641399679152,0.));
#88890=CARTESIAN_POINT('Ctrl Pts',(42.0159306406794,-23.7641399679152,20.));
#88891=CARTESIAN_POINT('Ctrl Pts',(41.9968248753238,-23.7917493984363,0.));
#88892=CARTESIAN_POINT('Ctrl Pts',(41.9968248753238,-23.7917493984363,20.));
#88893=CARTESIAN_POINT('Ctrl Pts',(41.9777006237952,-23.8193446686815,0.));
#88894=CARTESIAN_POINT('Ctrl Pts',(41.9777006237952,-23.8193446686815,20.));
#88895=CARTESIAN_POINT('Ctrl Pts',(41.9585578959806,-23.8469257658985,0.));
#88896=CARTESIAN_POINT('Ctrl Pts',(41.9585578959806,-23.8469257658985,20.));
#88897=CARTESIAN_POINT('Ctrl Pts',(41.9393967017767,-23.8744926773418,0.));
#88898=CARTESIAN_POINT('Ctrl Pts',(41.9393967017767,-23.8744926773418,20.));
#88899=CARTESIAN_POINT('Ctrl Pts',(41.9202170510888,-23.9020453902722,0.));
#88900=CARTESIAN_POINT('Ctrl Pts',(41.9202170510888,-23.9020453902722,20.));
#88901=CARTESIAN_POINT('Ctrl Pts',(41.9010189538314,-23.9295838919573,0.));
#88902=CARTESIAN_POINT('Ctrl Pts',(41.9010189538314,-23.9295838919573,20.));
#88903=CARTESIAN_POINT('Ctrl Pts',(41.8818024199281,-23.9571081696708,0.));
#88904=CARTESIAN_POINT('Ctrl Pts',(41.8818024199281,-23.9571081696708,20.));
#88905=CARTESIAN_POINT('Ctrl Pts',(41.8625674593112,-23.9846182106931,0.));
#88906=CARTESIAN_POINT('Ctrl Pts',(41.8625674593112,-23.9846182106931,20.));
#88907=CARTESIAN_POINT('Ctrl Pts',(41.8433140819226,-24.0121140023113,0.));
#88908=CARTESIAN_POINT('Ctrl Pts',(41.8433140819226,-24.0121140023113,20.));
#88909=CARTESIAN_POINT('Ctrl Pts',(41.824042297713,-24.0395955318191,0.));
#88910=CARTESIAN_POINT('Ctrl Pts',(41.824042297713,-24.0395955318191,20.));
#88911=CARTESIAN_POINT('Ctrl Pts',(41.8047521166422,-24.0670627865166,0.));
#88912=CARTESIAN_POINT('Ctrl Pts',(41.8047521166422,-24.0670627865166,20.));
#88913=CARTESIAN_POINT('Ctrl Pts',(41.785443548679,-24.0945157537107,0.));
#88914=CARTESIAN_POINT('Ctrl Pts',(41.785443548679,-24.0945157537107,20.));
#88915=CARTESIAN_POINT('Ctrl Pts',(41.7661166038015,-24.1219544207148,0.));
#88916=CARTESIAN_POINT('Ctrl Pts',(41.7661166038015,-24.1219544207148,20.));
#88917=CARTESIAN_POINT('Ctrl Pts',(41.7467712919966,-24.1493787748488,0.));
#88918=CARTESIAN_POINT('Ctrl Pts',(41.7467712919966,-24.1493787748488,20.));
#88919=CARTESIAN_POINT('Ctrl Pts',(41.7274076232604,-24.1767888034393,0.));
#88920=CARTESIAN_POINT('Ctrl Pts',(41.7274076232604,-24.1767888034393,20.));
#88921=CARTESIAN_POINT('Ctrl Pts',(41.7080256075983,-24.2041844938197,0.));
#88922=CARTESIAN_POINT('Ctrl Pts',(41.7080256075983,-24.2041844938197,20.));
#88923=CARTESIAN_POINT('Ctrl Pts',(41.688625255024,-24.2315658333297,0.));
#88924=CARTESIAN_POINT('Ctrl Pts',(41.688625255024,-24.2315658333297,20.));
#88925=CARTESIAN_POINT('Ctrl Pts',(41.6692065755608,-24.2589328093159,0.));
#88926=CARTESIAN_POINT('Ctrl Pts',(41.6692065755608,-24.2589328093159,20.));
#88927=CARTESIAN_POINT('Ctrl Pts',(41.6497695792407,-24.2862854091312,0.));
#88928=CARTESIAN_POINT('Ctrl Pts',(41.6497695792407,-24.2862854091312,20.));
#88929=CARTESIAN_POINT('Ctrl Pts',(41.630314276105,-24.3136236201351,0.));
#88930=CARTESIAN_POINT('Ctrl Pts',(41.630314276105,-24.3136236201351,20.));
#88931=CARTESIAN_POINT('Ctrl Pts',(41.610840676204,-24.3409474296941,0.));
#88932=CARTESIAN_POINT('Ctrl Pts',(41.610840676204,-24.3409474296941,20.));
#88933=CARTESIAN_POINT('Ctrl Pts',(41.5913487895971,-24.368256825181,0.));
#88934=CARTESIAN_POINT('Ctrl Pts',(41.5913487895971,-24.368256825181,20.));
#88935=CARTESIAN_POINT('Ctrl Pts',(41.5718386263526,-24.3955517939757,0.));
#88936=CARTESIAN_POINT('Ctrl Pts',(41.5718386263526,-24.3955517939757,20.));
#88937=CARTESIAN_POINT('Ctrl Pts',(41.5523101965477,-24.4228323234645,0.));
#88938=CARTESIAN_POINT('Ctrl Pts',(41.5523101965477,-24.4228323234645,20.));
#88939=CARTESIAN_POINT('Ctrl Pts',(41.5327635102685,-24.4500984010406,0.));
#88940=CARTESIAN_POINT('Ctrl Pts',(41.5327635102685,-24.4500984010406,20.));
#88941=CARTESIAN_POINT('Ctrl Pts',(41.5131985776101,-24.4773500141037,0.));
#88942=CARTESIAN_POINT('Ctrl Pts',(41.5131985776101,-24.4773500141037,20.));
#88943=CARTESIAN_POINT('Ctrl Pts',(41.4936154086768,-24.5045871500598,0.));
#88944=CARTESIAN_POINT('Ctrl Pts',(41.4936154086768,-24.5045871500598,20.));
#88945=CARTESIAN_POINT('Ctrl Pts',(41.4740140135823,-24.5318097963223,0.));
#88946=CARTESIAN_POINT('Ctrl Pts',(41.4740140135823,-24.5318097963223,20.));
#88947=CARTESIAN_POINT('Ctrl Pts',(41.4543944024488,-24.5590179403106,0.));
#88948=CARTESIAN_POINT('Ctrl Pts',(41.4543944024488,-24.5590179403106,20.));
#88949=CARTESIAN_POINT('Ctrl Pts',(41.4347565854076,-24.5862115694513,0.));
#88950=CARTESIAN_POINT('Ctrl Pts',(41.4347565854076,-24.5862115694513,20.));
#88951=CARTESIAN_POINT('Ctrl Pts',(41.4151005725989,-24.6133906711774,0.));
#88952=CARTESIAN_POINT('Ctrl Pts',(41.4151005725989,-24.6133906711774,20.));
#88953=CARTESIAN_POINT('Ctrl Pts',(41.3954263741717,-24.6405552329289,0.));
#88954=CARTESIAN_POINT('Ctrl Pts',(41.3954263741717,-24.6405552329289,20.));
#88955=CARTESIAN_POINT('Ctrl Pts',(41.3757340002844,-24.6677052421523,0.));
#88956=CARTESIAN_POINT('Ctrl Pts',(41.3757340002844,-24.6677052421523,20.));
#88957=CARTESIAN_POINT('Ctrl Pts',(41.3560234611038,-24.694840686301,0.));
#88958=CARTESIAN_POINT('Ctrl Pts',(41.3560234611038,-24.694840686301,20.));
#88959=CARTESIAN_POINT('Ctrl Pts',(41.3362947668064,-24.7219615528352,0.));
#88960=CARTESIAN_POINT('Ctrl Pts',(41.3362947668064,-24.7219615528352,20.));
#88961=CARTESIAN_POINT('Ctrl Pts',(41.3165479275773,-24.7490678292217,0.));
#88962=CARTESIAN_POINT('Ctrl Pts',(41.3165479275773,-24.7490678292217,20.));
#88963=CARTESIAN_POINT('Ctrl Pts',(41.2967829536105,-24.7761595029341,0.));
#88964=CARTESIAN_POINT('Ctrl Pts',(41.2967829536105,-24.7761595029341,20.));
#88965=CARTESIAN_POINT('Ctrl Pts',(41.276999855109,-24.8032365614526,0.));
#88966=CARTESIAN_POINT('Ctrl Pts',(41.276999855109,-24.8032365614526,20.));
#88967=CARTESIAN_POINT('Ctrl Pts',(41.2571986422843,-24.8302989922639,0.));
#88968=CARTESIAN_POINT('Ctrl Pts',(41.2571986422843,-24.8302989922639,20.));
#88969=CARTESIAN_POINT('Ctrl Pts',(41.2373793253577,-24.8573467828623,0.));
#88970=CARTESIAN_POINT('Ctrl Pts',(41.2373793253577,-24.8573467828623,20.));
#88971=CARTESIAN_POINT('Ctrl Pts',(41.2175419145588,-24.8843799207483,0.));
#88972=CARTESIAN_POINT('Ctrl Pts',(41.2175419145588,-24.8843799207483,20.));
#88973=CARTESIAN_POINT('Ctrl Pts',(41.1976864201268,-24.9113983934294,0.));
#88974=CARTESIAN_POINT('Ctrl Pts',(41.1976864201268,-24.9113983934294,20.));
#88975=CARTESIAN_POINT('Ctrl Pts',(41.1778128523092,-24.9384021884197,0.));
#88976=CARTESIAN_POINT('Ctrl Pts',(41.1778128523092,-24.9384021884197,20.));
#88977=CARTESIAN_POINT('Ctrl Pts',(41.1579212213625,-24.9653912932403,0.));
#88978=CARTESIAN_POINT('Ctrl Pts',(41.1579212213625,-24.9653912932403,20.));
#88979=CARTESIAN_POINT('Ctrl Pts',(41.1380115375521,-24.9923656954187,0.));
#88980=CARTESIAN_POINT('Ctrl Pts',(41.1380115375521,-24.9923656954187,20.));
#88981=CARTESIAN_POINT('Ctrl Pts',(41.1180838111525,-25.0193253824897,0.));
#88982=CARTESIAN_POINT('Ctrl Pts',(41.1180838111525,-25.0193253824897,20.));
#88983=CARTESIAN_POINT('Ctrl Pts',(41.0981380524472,-25.0462703419947,0.));
#88984=CARTESIAN_POINT('Ctrl Pts',(41.0981380524472,-25.0462703419947,20.));
#88985=CARTESIAN_POINT('Ctrl Pts',(41.0781742717283,-25.0732005614819,0.));
#88986=CARTESIAN_POINT('Ctrl Pts',(41.0781742717283,-25.0732005614819,20.));
#88987=CARTESIAN_POINT('Ctrl Pts',(41.058192479297,-25.1001160285063,0.));
#88988=CARTESIAN_POINT('Ctrl Pts',(41.058192479297,-25.1001160285063,20.));
#88989=CARTESIAN_POINT('Ctrl Pts',(41.0381926854635,-25.1270167306298,0.));
#88990=CARTESIAN_POINT('Ctrl Pts',(41.0381926854635,-25.1270167306298,20.));
#88991=CARTESIAN_POINT('Ctrl Pts',(41.0181749005471,-25.1539026554213,0.));
#88992=CARTESIAN_POINT('Ctrl Pts',(41.0181749005471,-25.1539026554213,20.));
#88993=CARTESIAN_POINT('Ctrl Pts',(40.9981391348755,-25.1807737904566,0.));
#88994=CARTESIAN_POINT('Ctrl Pts',(40.9981391348755,-25.1807737904566,20.));
#88995=CARTESIAN_POINT('Ctrl Pts',(40.9780853987856,-25.2076301233182,0.));
#88996=CARTESIAN_POINT('Ctrl Pts',(40.9780853987856,-25.2076301233182,20.));
#88997=CARTESIAN_POINT('Ctrl Pts',(40.9580137026228,-25.2344716415952,0.));
#88998=CARTESIAN_POINT('Ctrl Pts',(40.9580137026228,-25.2344716415952,20.));
#88999=CARTESIAN_POINT('Ctrl Pts',(40.9379240567416,-25.2612983328836,0.));
#89000=CARTESIAN_POINT('Ctrl Pts',(40.9379240567416,-25.2612983328836,20.));
#89001=CARTESIAN_POINT('Ctrl Pts',(40.9178164715051,-25.2881101847862,0.));
#89002=CARTESIAN_POINT('Ctrl Pts',(40.9178164715051,-25.2881101847862,20.));
#89003=CARTESIAN_POINT('Ctrl Pts',(40.8976909572856,-25.3149071849127,0.));
#89004=CARTESIAN_POINT('Ctrl Pts',(40.8976909572856,-25.3149071849127,20.));
#89005=CARTESIAN_POINT('Ctrl Pts',(40.8775475244644,-25.3416893208803,0.));
#89006=CARTESIAN_POINT('Ctrl Pts',(40.8775475244644,-25.3416893208803,20.));
#89007=CARTESIAN_POINT('Ctrl Pts',(40.8573861834315,-25.3684565803126,0.));
#89008=CARTESIAN_POINT('Ctrl Pts',(40.8573861834315,-25.3684565803126,20.));
#89009=CARTESIAN_POINT('Ctrl Pts',(40.8372069445861,-25.3952089508407,0.));
#89010=CARTESIAN_POINT('Ctrl Pts',(40.8372069445861,-25.3952089508407,20.));
#89011=CARTESIAN_POINT('Ctrl Pts',(40.8170098183361,-25.4219464201024,0.));
#89012=CARTESIAN_POINT('Ctrl Pts',(40.8170098183361,-25.4219464201024,20.));
#89013=CARTESIAN_POINT('Ctrl Pts',(40.796794815098,-25.4486689757422,0.));
#89014=CARTESIAN_POINT('Ctrl Pts',(40.796794815098,-25.4486689757422,20.));
#89015=CARTESIAN_POINT('Ctrl Pts',(40.7765619452973,-25.4753766054114,0.));
#89016=CARTESIAN_POINT('Ctrl Pts',(40.7765619452973,-25.4753766054114,20.));
#89017=CARTESIAN_POINT('Ctrl Pts',(40.7563112193678,-25.5020692967677,0.));
#89018=CARTESIAN_POINT('Ctrl Pts',(40.7563112193678,-25.5020692967677,20.));
#89019=CARTESIAN_POINT('Ctrl Pts',(40.7360426477524,-25.528747037476,0.));
#89020=CARTESIAN_POINT('Ctrl Pts',(40.7360426477524,-25.528747037476,20.));
#89021=CARTESIAN_POINT('Ctrl Pts',(40.715756240903,-25.5554098152083,0.));
#89022=CARTESIAN_POINT('Ctrl Pts',(40.715756240903,-25.5554098152083,20.));
#89023=CARTESIAN_POINT('Ctrl Pts',(40.6954520092804,-25.5820576176439,0.));
#89024=CARTESIAN_POINT('Ctrl Pts',(40.6954520092804,-25.5820576176439,20.));
#89025=CARTESIAN_POINT('Ctrl Pts',(40.6751299633542,-25.6086904324689,0.));
#89026=CARTESIAN_POINT('Ctrl Pts',(40.6751299633542,-25.6086904324689,20.));
#89027=CARTESIAN_POINT('Ctrl Pts',(40.6547901136033,-25.6353082473769,0.));
#89028=CARTESIAN_POINT('Ctrl Pts',(40.6547901136033,-25.6353082473769,20.));
#89029=CARTESIAN_POINT('Ctrl Pts',(40.6344324705148,-25.6619110500678,0.));
#89030=CARTESIAN_POINT('Ctrl Pts',(40.6344324705148,-25.6619110500678,20.));
#89031=CARTESIAN_POINT('Ctrl Pts',(40.6140570445846,-25.6884988282486,0.));
#89032=CARTESIAN_POINT('Ctrl Pts',(40.6140570445846,-25.6884988282486,20.));
#89033=CARTESIAN_POINT('Ctrl Pts',(40.5936638463177,-25.7150715696333,0.));
#89034=CARTESIAN_POINT('Ctrl Pts',(40.5936638463177,-25.7150715696333,20.));
#89035=CARTESIAN_POINT('Ctrl Pts',(40.5732528862276,-25.7416292619425,0.));
#89036=CARTESIAN_POINT('Ctrl Pts',(40.5732528862276,-25.7416292619425,20.));
#89037=CARTESIAN_POINT('Ctrl Pts',(40.5528241748366,-25.768171892904,0.));
#89038=CARTESIAN_POINT('Ctrl Pts',(40.5528241748366,-25.768171892904,20.));
#89039=CARTESIAN_POINT('Ctrl Pts',(40.5323777226757,-25.7946994502526,0.));
#89040=CARTESIAN_POINT('Ctrl Pts',(40.5323777226757,-25.7946994502526,20.));
#89041=CARTESIAN_POINT('Ctrl Pts',(40.5119135402852,-25.8212119217304,0.));
#89042=CARTESIAN_POINT('Ctrl Pts',(40.5119135402852,-25.8212119217304,20.));
#89043=CARTESIAN_POINT('Ctrl Pts',(40.491431638214,-25.8477092950863,0.));
#89044=CARTESIAN_POINT('Ctrl Pts',(40.491431638214,-25.8477092950863,20.));
#89045=CARTESIAN_POINT('Ctrl Pts',(40.4709320270197,-25.8741915580762,0.));
#89046=CARTESIAN_POINT('Ctrl Pts',(40.4709320270197,-25.8741915580762,20.));
#89047=CARTESIAN_POINT('Ctrl Pts',(40.4504147172684,-25.9006586984631,0.));
#89048=CARTESIAN_POINT('Ctrl Pts',(40.4504147172684,-25.9006586984631,20.));
#89049=CARTESIAN_POINT('Ctrl Pts',(40.4298797195352,-25.9271107040169,0.));
#89050=CARTESIAN_POINT('Ctrl Pts',(40.4298797195352,-25.9271107040169,20.));
#89051=CARTESIAN_POINT('Ctrl Pts',(40.4093270444043,-25.953547562515,0.));
#89052=CARTESIAN_POINT('Ctrl Pts',(40.4093270444043,-25.953547562515,20.));
#89053=CARTESIAN_POINT('Ctrl Pts',(40.3887567024682,-25.9799692617416,0.));
#89054=CARTESIAN_POINT('Ctrl Pts',(40.3887567024682,-25.9799692617416,20.));
#89055=CARTESIAN_POINT('Ctrl Pts',(40.3681687043283,-26.0063757894875,0.));
#89056=CARTESIAN_POINT('Ctrl Pts',(40.3681687043283,-26.0063757894875,20.));
#89057=CARTESIAN_POINT('Ctrl Pts',(40.347563060595,-26.0327671335511,0.));
#89058=CARTESIAN_POINT('Ctrl Pts',(40.347563060595,-26.0327671335511,20.));
#89059=CARTESIAN_POINT('Ctrl Pts',(40.326939781887,-26.0591432817373,0.));
#89060=CARTESIAN_POINT('Ctrl Pts',(40.326939781887,-26.0591432817373,20.));
#89061=CARTESIAN_POINT('Ctrl Pts',(40.3062988788318,-26.0855042218584,0.));
#89062=CARTESIAN_POINT('Ctrl Pts',(40.3062988788318,-26.0855042218584,20.));
#89063=CARTESIAN_POINT('Ctrl Pts',(40.2856403620657,-26.1118499417334,0.));
#89064=CARTESIAN_POINT('Ctrl Pts',(40.2856403620657,-26.1118499417334,20.));
#89065=CARTESIAN_POINT('Ctrl Pts',(40.2649642422341,-26.1381804291893,0.));
#89066=CARTESIAN_POINT('Ctrl Pts',(40.2649642422341,-26.1381804291893,20.));
#89067=CARTESIAN_POINT('Ctrl Pts',(40.2442705299908,-26.1644956720595,0.));
#89068=CARTESIAN_POINT('Ctrl Pts',(40.2442705299908,-26.1644956720595,20.));
#89069=CARTESIAN_POINT('Ctrl Pts',(40.2235592359986,-26.1907956581852,0.));
#89070=CARTESIAN_POINT('Ctrl Pts',(40.2235592359986,-26.1907956581852,20.));
#89071=CARTESIAN_POINT('Ctrl Pts',(40.2028303709288,-26.217080375414,0.));
#89072=CARTESIAN_POINT('Ctrl Pts',(40.2028303709288,-26.217080375414,20.));
#89073=CARTESIAN_POINT('Ctrl Pts',(40.1820839454613,-26.2433498116008,0.));
#89074=CARTESIAN_POINT('Ctrl Pts',(40.1820839454613,-26.2433498116008,20.));
#89075=CARTESIAN_POINT('Ctrl Pts',(40.161319970285,-26.2696039546074,0.));
#89076=CARTESIAN_POINT('Ctrl Pts',(40.161319970285,-26.2696039546074,20.));
#89077=CARTESIAN_POINT('Ctrl Pts',(40.1405384560971,-26.2958427923028,0.));
#89078=CARTESIAN_POINT('Ctrl Pts',(40.1405384560971,-26.2958427923028,20.));
#89079=CARTESIAN_POINT('Ctrl Pts',(40.1197394136039,-26.3220663125631,0.));
#89080=CARTESIAN_POINT('Ctrl Pts',(40.1197394136039,-26.3220663125631,20.));
#89081=CARTESIAN_POINT('Ctrl Pts',(40.0989228535202,-26.3482745032719,0.));
#89082=CARTESIAN_POINT('Ctrl Pts',(40.0989228535202,-26.3482745032719,20.));
#89083=CARTESIAN_POINT('Ctrl Pts',(40.0780887865696,-26.3744673523197,0.));
#89084=CARTESIAN_POINT('Ctrl Pts',(40.0780887865696,-26.3744673523197,20.));
#89085=CARTESIAN_POINT('Ctrl Pts',(40.0572372234843,-26.4006448476042,0.));
#89086=CARTESIAN_POINT('Ctrl Pts',(40.0572372234843,-26.4006448476042,20.));
#89087=CARTESIAN_POINT('Ctrl Pts',(40.0363681750052,-26.4268069770299,0.));
#89088=CARTESIAN_POINT('Ctrl Pts',(40.0363681750052,-26.4268069770299,20.));
#89089=CARTESIAN_POINT('Ctrl Pts',(40.015481651882,-26.4529537285089,0.));
#89090=CARTESIAN_POINT('Ctrl Pts',(40.015481651882,-26.4529537285089,20.));
#89091=CARTESIAN_POINT('Ctrl Pts',(39.994577664873,-26.4790850899607,0.));
#89092=CARTESIAN_POINT('Ctrl Pts',(39.994577664873,-26.4790850899607,20.));
#89093=CARTESIAN_POINT('Ctrl Pts',(39.9736562247456,-26.5052010493117,0.));
#89094=CARTESIAN_POINT('Ctrl Pts',(39.9736562247456,-26.5052010493117,20.));
#89095=CARTESIAN_POINT('Ctrl Pts',(39.9527173422752,-26.5313015944953,0.));
#89096=CARTESIAN_POINT('Ctrl Pts',(39.9527173422752,-26.5313015944953,20.));
#89097=CARTESIAN_POINT('Ctrl Pts',(39.9317610282459,-26.5573867134521,0.));
#89098=CARTESIAN_POINT('Ctrl Pts',(39.9317610282459,-26.5573867134521,20.));
#89099=CARTESIAN_POINT('Ctrl Pts',(39.9107872934506,-26.5834563941296,0.));
#89100=CARTESIAN_POINT('Ctrl Pts',(39.9107872934506,-26.5834563941296,20.));
#89101=CARTESIAN_POINT('Ctrl Pts',(39.8897961486907,-26.6095106244829,0.));
#89102=CARTESIAN_POINT('Ctrl Pts',(39.8897961486907,-26.6095106244829,20.));
#89103=CARTESIAN_POINT('Ctrl Pts',(39.8687876047769,-26.6355493924744,0.));
#89104=CARTESIAN_POINT('Ctrl Pts',(39.8687876047769,-26.6355493924744,20.));
#89105=CARTESIAN_POINT('Ctrl Pts',(39.847761672528,-26.6615726860735,0.));
#89106=CARTESIAN_POINT('Ctrl Pts',(39.847761672528,-26.6615726860735,20.));
#89107=CARTESIAN_POINT('Ctrl Pts',(39.8267183627717,-26.687580493257,0.));
#89108=CARTESIAN_POINT('Ctrl Pts',(39.8267183627717,-26.687580493257,20.));
#89109=CARTESIAN_POINT('Ctrl Pts',(39.8056576863443,-26.713572802009,0.));
#89110=CARTESIAN_POINT('Ctrl Pts',(39.8056576863443,-26.713572802009,20.));
#89111=CARTESIAN_POINT('Ctrl Pts',(39.7845796540903,-26.7395496003209,0.));
#89112=CARTESIAN_POINT('Ctrl Pts',(39.7845796540903,-26.7395496003209,20.));
#89113=CARTESIAN_POINT('Ctrl Pts',(39.7634842768631,-26.7655108761908,0.));
#89114=CARTESIAN_POINT('Ctrl Pts',(39.7634842768631,-26.7655108761908,20.));
#89115=CARTESIAN_POINT('Ctrl Pts',(39.7423715655248,-26.7914566176244,0.));
#89116=CARTESIAN_POINT('Ctrl Pts',(39.7423715655248,-26.7914566176244,20.));
#89117=CARTESIAN_POINT('Ctrl Pts',(39.7212415309462,-26.8173868126345,0.));
#89118=CARTESIAN_POINT('Ctrl Pts',(39.7212415309462,-26.8173868126345,20.));
#89119=CARTESIAN_POINT('Ctrl Pts',(39.7000941840065,-26.843301449241,0.));
#89120=CARTESIAN_POINT('Ctrl Pts',(39.7000941840065,-26.843301449241,20.));
#89121=CARTESIAN_POINT('Ctrl Pts',(39.6789295355942,-26.8692005154716,0.));
#89122=CARTESIAN_POINT('Ctrl Pts',(39.6789295355942,-26.8692005154716,20.));
#89123=CARTESIAN_POINT('Ctrl Pts',(39.6577475966055,-26.8950839993609,0.));
#89124=CARTESIAN_POINT('Ctrl Pts',(39.6577475966055,-26.8950839993609,20.));
#89125=CARTESIAN_POINT('Ctrl Pts',(39.6365483779457,-26.9209518889509,0.));
#89126=CARTESIAN_POINT('Ctrl Pts',(39.6365483779457,-26.9209518889509,20.));
#89127=CARTESIAN_POINT('Ctrl Pts',(39.6153318905282,-26.9468041722907,0.));
#89128=CARTESIAN_POINT('Ctrl Pts',(39.6153318905282,-26.9468041722907,20.));
#89129=CARTESIAN_POINT('Ctrl Pts',(39.5940981452753,-26.9726408374371,0.));
#89130=CARTESIAN_POINT('Ctrl Pts',(39.5940981452753,-26.9726408374371,20.));
#89131=CARTESIAN_POINT('Ctrl Pts',(39.5728471531177,-26.9984618724537,0.));
#89132=CARTESIAN_POINT('Ctrl Pts',(39.5728471531177,-26.9984618724537,20.));
#89133=CARTESIAN_POINT('Ctrl Pts',(39.5515789249952,-27.0242672654118,0.));
#89134=CARTESIAN_POINT('Ctrl Pts',(39.5515789249952,-27.0242672654118,20.));
#89135=CARTESIAN_POINT('Ctrl Pts',(39.5302934718558,-27.0500570043898,0.));
#89136=CARTESIAN_POINT('Ctrl Pts',(39.5302934718558,-27.0500570043898,20.));
#89137=CARTESIAN_POINT('Ctrl Pts',(39.5089908046561,-27.0758310774732,0.));
#89138=CARTESIAN_POINT('Ctrl Pts',(39.5089908046561,-27.0758310774732,20.));
#89139=CARTESIAN_POINT('Ctrl Pts',(39.4876709343614,-27.1015894727552,0.));
#89140=CARTESIAN_POINT('Ctrl Pts',(39.4876709343614,-27.1015894727552,20.));
#89141=CARTESIAN_POINT('Ctrl Pts',(39.4663338719455,-27.1273321783362,0.));
#89142=CARTESIAN_POINT('Ctrl Pts',(39.4663338719455,-27.1273321783362,20.));
#89143=CARTESIAN_POINT('Ctrl Pts',(39.4449796283908,-27.153059182324,0.));
#89144=CARTESIAN_POINT('Ctrl Pts',(39.4449796283908,-27.153059182324,20.));
#89145=CARTESIAN_POINT('Ctrl Pts',(39.4236082146882,-27.1787704728337,0.));
#89146=CARTESIAN_POINT('Ctrl Pts',(39.4236082146882,-27.1787704728337,20.));
#89147=CARTESIAN_POINT('Ctrl Pts',(39.4022196418372,-27.2044660379877,0.));
#89148=CARTESIAN_POINT('Ctrl Pts',(39.4022196418372,-27.2044660379877,20.));
#89149=CARTESIAN_POINT('Ctrl Pts',(39.3808139208456,-27.2301458659158,0.));
#89150=CARTESIAN_POINT('Ctrl Pts',(39.3808139208456,-27.2301458659158,20.));
#89151=CARTESIAN_POINT('Ctrl Pts',(39.3593910627297,-27.2558099447548,0.));
#89152=CARTESIAN_POINT('Ctrl Pts',(39.3593910627297,-27.2558099447548,20.));
#89153=CARTESIAN_POINT('Ctrl Pts',(39.3379510785145,-27.2814582626493,0.));
#89154=CARTESIAN_POINT('Ctrl Pts',(39.3379510785145,-27.2814582626493,20.));
#89155=CARTESIAN_POINT('Ctrl Pts',(39.3164939792334,-27.3070908077508,0.));
#89156=CARTESIAN_POINT('Ctrl Pts',(39.3164939792334,-27.3070908077508,20.));
#89157=CARTESIAN_POINT('Ctrl Pts',(39.2950197759285,-27.3327075682187,0.));
#89158=CARTESIAN_POINT('Ctrl Pts',(39.2950197759285,-27.3327075682187,20.));
#89159=CARTESIAN_POINT('Ctrl Pts',(39.2735284796508,-27.3583085322198,0.));
#89160=CARTESIAN_POINT('Ctrl Pts',(39.2735284796508,-27.3583085322198,20.));
#89161=CARTESIAN_POINT('Ctrl Pts',(39.25202010146,-27.3838936879286,0.));
#89162=CARTESIAN_POINT('Ctrl Pts',(39.25202010146,-27.3838936879286,20.));
#89163=CARTESIAN_POINT('Ctrl Pts',(39.2304946524241,-27.4094630235266,0.));
#89164=CARTESIAN_POINT('Ctrl Pts',(39.2304946524241,-27.4094630235266,20.));
#89165=CARTESIAN_POINT('Ctrl Pts',(39.2089521436188,-27.4350165272023,0.));
#89166=CARTESIAN_POINT('Ctrl Pts',(39.2089521436188,-27.4350165272023,20.));
#89167=CARTESIAN_POINT('Ctrl Pts',(39.1873925861285,-27.4605541871518,0.));
#89168=CARTESIAN_POINT('Ctrl Pts',(39.1873925861285,-27.4605541871518,20.));
#89169=CARTESIAN_POINT('Ctrl Pts',(39.1658159910457,-27.4860759915783,0.));
#89170=CARTESIAN_POINT('Ctrl Pts',(39.1658159910457,-27.4860759915783,20.));
#89171=CARTESIAN_POINT('Ctrl Pts',(39.1442223694722,-27.5115819286927,0.));
#89172=CARTESIAN_POINT('Ctrl Pts',(39.1442223694722,-27.5115819286927,20.));
#89173=CARTESIAN_POINT('Ctrl Pts',(39.1226117325183,-27.5370719867137,0.));
#89174=CARTESIAN_POINT('Ctrl Pts',(39.1226117325183,-27.5370719867137,20.));
#89175=CARTESIAN_POINT('Ctrl Pts',(39.100984091303,-27.5625461538676,0.));
#89176=CARTESIAN_POINT('Ctrl Pts',(39.100984091303,-27.5625461538676,20.));
#89177=CARTESIAN_POINT('Ctrl Pts',(39.0793394569537,-27.5880044183879,0.));
#89178=CARTESIAN_POINT('Ctrl Pts',(39.0793394569537,-27.5880044183879,20.));
#89179=CARTESIAN_POINT('Ctrl Pts',(39.057677840606,-27.6134467685156,0.));
#89180=CARTESIAN_POINT('Ctrl Pts',(39.057677840606,-27.6134467685156,20.));
#89181=CARTESIAN_POINT('Ctrl Pts',(39.0359992534037,-27.6388731924983,0.));
#89182=CARTESIAN_POINT('Ctrl Pts',(39.0359992534037,-27.6388731924983,20.));
#89183=CARTESIAN_POINT('Ctrl Pts',(39.0143037064988,-27.6642836785915,0.));
#89184=CARTESIAN_POINT('Ctrl Pts',(39.0143037064988,-27.6642836785915,20.));
#89185=CARTESIAN_POINT('Ctrl Pts',(38.9925912110523,-27.6896782150583,0.));
#89186=CARTESIAN_POINT('Ctrl Pts',(38.9925912110523,-27.6896782150583,20.));
#89187=CARTESIAN_POINT('Ctrl Pts',(38.9708617782339,-27.7150567901695,0.));
#89188=CARTESIAN_POINT('Ctrl Pts',(38.9708617782339,-27.7150567901695,20.));
#89189=CARTESIAN_POINT('Ctrl Pts',(38.9491154192216,-27.7404193922036,0.));
#89190=CARTESIAN_POINT('Ctrl Pts',(38.9491154192216,-27.7404193922036,20.));
#89191=CARTESIAN_POINT('Ctrl Pts',(38.9273521452022,-27.7657660094467,0.));
#89192=CARTESIAN_POINT('Ctrl Pts',(38.9273521452022,-27.7657660094467,20.));
#89193=CARTESIAN_POINT('Ctrl Pts',(38.9055719673706,-27.7910966301919,0.));
#89194=CARTESIAN_POINT('Ctrl Pts',(38.9055719673706,-27.7910966301919,20.));
#89195=CARTESIAN_POINT('Ctrl Pts',(38.8837748969299,-27.8164112427396,0.));
#89196=CARTESIAN_POINT('Ctrl Pts',(38.8837748969299,-27.8164112427396,20.));
#89197=CARTESIAN_POINT('Ctrl Pts',(38.8619609450912,-27.8417098353976,0.));
#89198=CARTESIAN_POINT('Ctrl Pts',(38.8619609450912,-27.8417098353976,20.));
#89199=CARTESIAN_POINT('Ctrl Pts',(38.8401301230745,-27.866992396481,0.));
#89200=CARTESIAN_POINT('Ctrl Pts',(38.8401301230745,-27.866992396481,20.));
#89201=CARTESIAN_POINT('Ctrl Pts',(38.8182824421081,-27.8922589143132,0.));
#89202=CARTESIAN_POINT('Ctrl Pts',(38.8182824421081,-27.8922589143132,20.));
#89203=CARTESIAN_POINT('Ctrl Pts',(38.7964179134294,-27.917509377225,0.));
#89204=CARTESIAN_POINT('Ctrl Pts',(38.7964179134294,-27.917509377225,20.));
#89205=CARTESIAN_POINT('Ctrl Pts',(38.7745365482837,-27.9427437735547,0.));
#89206=CARTESIAN_POINT('Ctrl Pts',(38.7745365482837,-27.9427437735547,20.));
#89207=CARTESIAN_POINT('Ctrl Pts',(38.752638357925,-27.9679620916479,0.));
#89208=CARTESIAN_POINT('Ctrl Pts',(38.752638357925,-27.9679620916479,20.));
#89209=CARTESIAN_POINT('Ctrl Pts',(38.7307233536152,-27.9931643198581,0.));
#89210=CARTESIAN_POINT('Ctrl Pts',(38.7307233536152,-27.9931643198581,20.));
#89211=CARTESIAN_POINT('Ctrl Pts',(38.7087915466246,-28.0183504465459,0.));
#89212=CARTESIAN_POINT('Ctrl Pts',(38.7087915466246,-28.0183504465459,20.));
#89213=CARTESIAN_POINT('Ctrl Pts',(38.6868429482324,-28.0435204600798,0.));
#89214=CARTESIAN_POINT('Ctrl Pts',(38.6868429482324,-28.0435204600798,20.));
#89215=CARTESIAN_POINT('Ctrl Pts',(38.6648775697261,-28.0686743488362,0.));
#89216=CARTESIAN_POINT('Ctrl Pts',(38.6648775697261,-28.0686743488362,20.));
#89217=CARTESIAN_POINT('Ctrl Pts',(38.6428954224012,-28.0938121011982,0.));
#89218=CARTESIAN_POINT('Ctrl Pts',(38.6428954224012,-28.0938121011982,20.));
#89219=CARTESIAN_POINT('Ctrl Pts',(38.6208965175619,-28.1189337055566,0.));
#89220=CARTESIAN_POINT('Ctrl Pts',(38.6208965175619,-28.1189337055566,20.));
#89221=CARTESIAN_POINT('Ctrl Pts',(38.5988808665205,-28.14403915031,0.));
#89222=CARTESIAN_POINT('Ctrl Pts',(38.5988808665205,-28.14403915031,20.));
#89223=CARTESIAN_POINT('Ctrl Pts',(38.5768484805978,-28.1691284238645,0.));
#89224=CARTESIAN_POINT('Ctrl Pts',(38.5768484805978,-28.1691284238645,20.));
#89225=CARTESIAN_POINT('Ctrl Pts',(38.5547993711231,-28.1942015146341,0.));
#89226=CARTESIAN_POINT('Ctrl Pts',(38.5547993711231,-28.1942015146341,20.));
#89227=CARTESIAN_POINT('Ctrl Pts',(38.5327335494334,-28.2192584110398,0.));
#89228=CARTESIAN_POINT('Ctrl Pts',(38.5327335494334,-28.2192584110398,20.));
#89229=CARTESIAN_POINT('Ctrl Pts',(38.5106510268752,-28.2442991015113,0.));
#89230=CARTESIAN_POINT('Ctrl Pts',(38.5106510268752,-28.2442991015113,20.));
#89231=CARTESIAN_POINT('Ctrl Pts',(38.4885518148031,-28.2693235744854,0.));
#89232=CARTESIAN_POINT('Ctrl Pts',(38.4885518148031,-28.2693235744854,20.));
#89233=CARTESIAN_POINT('Ctrl Pts',(38.4664359245797,-28.2943318184066,0.));
#89234=CARTESIAN_POINT('Ctrl Pts',(38.4664359245797,-28.2943318184066,20.));
#89235=CARTESIAN_POINT('Ctrl Pts',(38.4443033675759,-28.3193238217266,0.));
#89236=CARTESIAN_POINT('Ctrl Pts',(38.4443033675759,-28.3193238217266,20.));
#89237=CARTESIAN_POINT('Ctrl Pts',(38.4221541551709,-28.344299572905,0.));
#89238=CARTESIAN_POINT('Ctrl Pts',(38.4221541551709,-28.344299572905,20.));
#89239=CARTESIAN_POINT('Ctrl Pts',(38.3999882987522,-28.3692590604082,0.));
#89240=CARTESIAN_POINT('Ctrl Pts',(38.3999882987522,-28.3692590604082,20.));
#89241=CARTESIAN_POINT('Ctrl Pts',(38.3778058097152,-28.3942022727108,0.));
#89242=CARTESIAN_POINT('Ctrl Pts',(38.3778058097152,-28.3942022727108,20.));
#89243=CARTESIAN_POINT('Ctrl Pts',(38.3556066994642,-28.4191291982951,0.));
#89244=CARTESIAN_POINT('Ctrl Pts',(38.3556066994642,-28.4191291982951,20.));
#89245=CARTESIAN_POINT('Ctrl Pts',(38.3333909794119,-28.4440398256512,0.));
#89246=CARTESIAN_POINT('Ctrl Pts',(38.3333909794119,-28.4440398256512,20.));
#89247=CARTESIAN_POINT('Ctrl Pts',(38.3111586609794,-28.4689341432774,0.));
#89248=CARTESIAN_POINT('Ctrl Pts',(38.3111586609794,-28.4689341432774,20.));
#89249=CARTESIAN_POINT('Ctrl Pts',(38.2889097555964,-28.4938121396793,0.));
#89250=CARTESIAN_POINT('Ctrl Pts',(38.2889097555964,-28.4938121396793,20.));
#89251=CARTESIAN_POINT('Ctrl Pts',(38.2666442747002,-28.5186738033704,0.));
#89252=CARTESIAN_POINT('Ctrl Pts',(38.2666442747002,-28.5186738033704,20.));
#89253=CARTESIAN_POINT('Ctrl Pts',(38.2443622297368,-28.5435191228711,0.));
#89254=CARTESIAN_POINT('Ctrl Pts',(38.2443622297368,-28.5435191228711,20.));
#89255=CARTESIAN_POINT('Ctrl Pts',(38.2220636321601,-28.5683480867098,0.));
#89256=CARTESIAN_POINT('Ctrl Pts',(38.2220636321601,-28.5683480867098,20.));
#89257=CARTESIAN_POINT('Ctrl Pts',(38.1997484934321,-28.5931606834224,0.));
#89258=CARTESIAN_POINT('Ctrl Pts',(38.1997484934321,-28.5931606834224,20.));
#89259=CARTESIAN_POINT('Ctrl Pts',(38.1774168250235,-28.6179569015525,0.));
#89260=CARTESIAN_POINT('Ctrl Pts',(38.1774168250235,-28.6179569015525,20.));
#89261=CARTESIAN_POINT('Ctrl Pts',(38.1550686384134,-28.6427367296518,0.));
#89262=CARTESIAN_POINT('Ctrl Pts',(38.1550686384134,-28.6427367296518,20.));
#89263=CARTESIAN_POINT('Ctrl Pts',(38.1327039450889,-28.6675001562794,0.));
#89264=CARTESIAN_POINT('Ctrl Pts',(38.1327039450889,-28.6675001562794,20.));
#89265=CARTESIAN_POINT('Ctrl Pts',(38.1103227565456,-28.6922471700024,0.));
#89266=CARTESIAN_POINT('Ctrl Pts',(38.1103227565456,-28.6922471700024,20.));
#89267=CARTESIAN_POINT('Ctrl Pts',(38.0879250842874,-28.7169777593956,0.));
#89268=CARTESIAN_POINT('Ctrl Pts',(38.0879250842874,-28.7169777593956,20.));
#89269=CARTESIAN_POINT('Ctrl Pts',(38.0655109398262,-28.7416919130413,0.));
#89270=CARTESIAN_POINT('Ctrl Pts',(38.0655109398262,-28.7416919130413,20.));
#89271=CARTESIAN_POINT('Ctrl Pts',(38.0430803346823,-28.76638961953,0.));
#89272=CARTESIAN_POINT('Ctrl Pts',(38.0430803346823,-28.76638961953,20.));
#89273=CARTESIAN_POINT('Ctrl Pts',(38.020633280384,-28.7910708674595,0.));
#89274=CARTESIAN_POINT('Ctrl Pts',(38.020633280384,-28.7910708674595,20.));
#89275=CARTESIAN_POINT('Ctrl Pts',(37.9981697884679,-28.8157356454354,0.));
#89276=CARTESIAN_POINT('Ctrl Pts',(37.9981697884679,-28.8157356454354,20.));
#89277=CARTESIAN_POINT('Ctrl Pts',(37.975689870479,-28.8403839420709,0.));
#89278=CARTESIAN_POINT('Ctrl Pts',(37.975689870479,-28.8403839420709,20.));
#89279=CARTESIAN_POINT('Ctrl Pts',(37.9531935379708,-28.8650157459872,0.));
#89280=CARTESIAN_POINT('Ctrl Pts',(37.9531935379708,-28.8650157459872,20.));
#89281=CARTESIAN_POINT('Ctrl Pts',(37.9306808025048,-28.8896310458131,0.));
#89282=CARTESIAN_POINT('Ctrl Pts',(37.9306808025048,-28.8896310458131,20.));
#89283=CARTESIAN_POINT('Ctrl Pts',(37.9081516756509,-28.9142298301853,0.));
#89284=CARTESIAN_POINT('Ctrl Pts',(37.9081516756509,-28.9142298301853,20.));
#89285=CARTESIAN_POINT('Ctrl Pts',(37.8856061689868,-28.9388120877484,0.));
#89286=CARTESIAN_POINT('Ctrl Pts',(37.8856061689868,-28.9388120877484,20.));
#89287=CARTESIAN_POINT('Ctrl Pts',(37.8630442940985,-28.9633778071544,0.));
#89288=CARTESIAN_POINT('Ctrl Pts',(37.8630442940985,-28.9633778071544,20.));
#89289=CARTESIAN_POINT('Ctrl Pts',(37.8404660625803,-28.9879269770638,0.));
#89290=CARTESIAN_POINT('Ctrl Pts',(37.8404660625803,-28.9879269770638,20.));
#89291=CARTESIAN_POINT('Ctrl Pts',(37.8178714860345,-29.0124595861442,0.));
#89292=CARTESIAN_POINT('Ctrl Pts',(37.8178714860345,-29.0124595861442,20.));
#89293=CARTESIAN_POINT('Ctrl Pts',(37.7952605760716,-29.0369756230713,0.));
#89294=CARTESIAN_POINT('Ctrl Pts',(37.7952605760716,-29.0369756230713,20.));
#89295=CARTESIAN_POINT('Ctrl Pts',(37.7726333443105,-29.0614750765285,0.));
#89296=CARTESIAN_POINT('Ctrl Pts',(37.7726333443105,-29.0614750765285,20.));
#89297=CARTESIAN_POINT('Ctrl Pts',(37.7499898023784,-29.0859579352069,0.));
#89298=CARTESIAN_POINT('Ctrl Pts',(37.7499898023784,-29.0859579352069,20.));
#89299=CARTESIAN_POINT('Ctrl Pts',(37.7273299619109,-29.1104241878056,0.));
#89300=CARTESIAN_POINT('Ctrl Pts',(37.7273299619109,-29.1104241878056,20.));
#89301=CARTESIAN_POINT('Ctrl Pts',(37.7046538345516,-29.1348738230316,0.));
#89302=CARTESIAN_POINT('Ctrl Pts',(37.7046538345516,-29.1348738230316,20.));
#89303=CARTESIAN_POINT('Ctrl Pts',(37.6819614319522,-29.1593068295998,0.));
#89304=CARTESIAN_POINT('Ctrl Pts',(37.6819614319522,-29.1593068295998,20.));
#89305=CARTESIAN_POINT('Ctrl Pts',(37.6592527657727,-29.1837231962329,0.));
#89306=CARTESIAN_POINT('Ctrl Pts',(37.6592527657727,-29.1837231962329,20.));
#89307=CARTESIAN_POINT('Ctrl Pts',(37.6365278476807,-29.208122911661,0.));
#89308=CARTESIAN_POINT('Ctrl Pts',(37.6365278476807,-29.208122911661,20.));
#89309=CARTESIAN_POINT('Ctrl Pts',(37.6137866893519,-29.2325059646225,0.));
#89310=CARTESIAN_POINT('Ctrl Pts',(37.6137866893519,-29.2325059646225,20.));
#89311=CARTESIAN_POINT('Ctrl Pts',(37.5910293024705,-29.2568723438632,0.));
#89312=CARTESIAN_POINT('Ctrl Pts',(37.5910293024705,-29.2568723438632,20.));
#89313=CARTESIAN_POINT('Ctrl Pts',(37.5682556987287,-29.2812220381373,0.));
#89314=CARTESIAN_POINT('Ctrl Pts',(37.5682556987287,-29.2812220381373,20.));
#89315=CARTESIAN_POINT('Ctrl Pts',(37.5454658898273,-29.3055550362068,0.));
#89316=CARTESIAN_POINT('Ctrl Pts',(37.5454658898273,-29.3055550362068,20.));
#89317=CARTESIAN_POINT('Ctrl Pts',(37.5226598874754,-29.3298713268414,0.));
#89318=CARTESIAN_POINT('Ctrl Pts',(37.5226598874754,-29.3298713268414,20.));
#89319=CARTESIAN_POINT('Ctrl Pts',(37.4998377033899,-29.3541708988191,0.));
#89320=CARTESIAN_POINT('Ctrl Pts',(37.4998377033899,-29.3541708988191,20.));
#89321=CARTESIAN_POINT('Ctrl Pts',(37.4769993492958,-29.3784537409251,0.));
#89322=CARTESIAN_POINT('Ctrl Pts',(37.4769993492958,-29.3784537409251,20.));
#89323=CARTESIAN_POINT('Ctrl Pts',(37.4541448369259,-29.4027198419524,0.));
#89324=CARTESIAN_POINT('Ctrl Pts',(37.4541448369259,-29.4027198419524,20.));
#89325=CARTESIAN_POINT('Ctrl Pts',(37.4312741780212,-29.4269691907023,0.));
#89326=CARTESIAN_POINT('Ctrl Pts',(37.4312741780212,-29.4269691907023,20.));
#89327=CARTESIAN_POINT('Ctrl Pts',(37.4083873843312,-29.4512017759842,0.));
#89328=CARTESIAN_POINT('Ctrl Pts',(37.4083873843312,-29.4512017759842,20.));
#89329=CARTESIAN_POINT('Ctrl Pts',(37.3854844676135,-29.4754175866156,0.));
#89330=CARTESIAN_POINT('Ctrl Pts',(37.3854844676135,-29.4754175866156,20.));
#89331=CARTESIAN_POINT('Ctrl Pts',(37.3625654396334,-29.4996166114217,0.));
#89332=CARTESIAN_POINT('Ctrl Pts',(37.3625654396334,-29.4996166114217,20.));
#89333=CARTESIAN_POINT('Ctrl Pts',(37.3396303121646,-29.5237988392353,0.));
#89334=CARTESIAN_POINT('Ctrl Pts',(37.3396303121646,-29.5237988392353,20.));
#89335=CARTESIAN_POINT('Ctrl Pts',(37.3166790969884,-29.5479642588972,0.));
#89336=CARTESIAN_POINT('Ctrl Pts',(37.3166790969884,-29.5479642588972,20.));
#89337=CARTESIAN_POINT('Ctrl Pts',(37.2937118058947,-29.5721128592559,0.));
#89338=CARTESIAN_POINT('Ctrl Pts',(37.2937118058947,-29.5721128592559,20.));
#89339=CARTESIAN_POINT('Ctrl Pts',(37.2707284506814,-29.5962446291683,0.));
#89340=CARTESIAN_POINT('Ctrl Pts',(37.2707284506814,-29.5962446291683,20.));
#89341=CARTESIAN_POINT('Ctrl Pts',(37.2477290431548,-29.6203595574991,0.));
#89342=CARTESIAN_POINT('Ctrl Pts',(37.2477290431548,-29.6203595574991,20.));
#89343=CARTESIAN_POINT('Ctrl Pts',(37.2247135951292,-29.6444576331215,0.));
#89344=CARTESIAN_POINT('Ctrl Pts',(37.2247135951292,-29.6444576331215,20.));
#89345=CARTESIAN_POINT('Ctrl Pts',(37.2016821184267,-29.668538844916,0.));
#89346=CARTESIAN_POINT('Ctrl Pts',(37.2016821184267,-29.668538844916,20.));
#89347=CARTESIAN_POINT('Ctrl Pts',(37.1786346248774,-29.6926031817715,0.));
#89348=CARTESIAN_POINT('Ctrl Pts',(37.1786346248774,-29.6926031817715,20.));
#89349=CARTESIAN_POINT('Ctrl Pts',(37.155571126319,-29.7166506325841,0.));
#89350=CARTESIAN_POINT('Ctrl Pts',(37.155571126319,-29.7166506325841,20.));
#89351=CARTESIAN_POINT('Ctrl Pts',(37.1324916345976,-29.7406811862582,0.));
#89352=CARTESIAN_POINT('Ctrl Pts',(37.1324916345976,-29.7406811862582,20.));
#89353=CARTESIAN_POINT('Ctrl Pts',(37.1093961615672,-29.7646948317062,0.));
#89354=CARTESIAN_POINT('Ctrl Pts',(37.1093961615672,-29.7646948317062,20.));
#89355=CARTESIAN_POINT('Ctrl Pts',(37.0862847190902,-29.7886915578486,0.));
#89356=CARTESIAN_POINT('Ctrl Pts',(37.0862847190902,-29.7886915578486,20.));
#89357=CARTESIAN_POINT('Ctrl Pts',(37.0631573190373,-29.8126713536142,0.));
#89358=CARTESIAN_POINT('Ctrl Pts',(37.0631573190373,-29.8126713536142,20.));
#89359=CARTESIAN_POINT('Ctrl Pts',(37.0400139732874,-29.8366342079401,0.));
#89360=CARTESIAN_POINT('Ctrl Pts',(37.0400139732874,-29.8366342079401,20.));
#89361=CARTESIAN_POINT('Ctrl Pts',(37.0168546937273,-29.8605801097708,0.));
#89362=CARTESIAN_POINT('Ctrl Pts',(37.0168546937273,-29.8605801097708,20.));
#89363=CARTESIAN_POINT('Ctrl Pts',(36.9936794922513,-29.884509048059,0.));
#89364=CARTESIAN_POINT('Ctrl Pts',(36.9936794922513,-29.884509048059,20.));
#89365=CARTESIAN_POINT('Ctrl Pts',(36.9704883807614,-29.9084210117647,0.));
#89366=CARTESIAN_POINT('Ctrl Pts',(36.9704883807614,-29.9084210117647,20.));
#89367=CARTESIAN_POINT('Ctrl Pts',(36.9472813711676,-29.9323159898562,0.));
#89368=CARTESIAN_POINT('Ctrl Pts',(36.9472813711676,-29.9323159898562,20.));
#89369=CARTESIAN_POINT('Ctrl Pts',(36.9240584753882,-29.9561939713103,0.));
#89370=CARTESIAN_POINT('Ctrl Pts',(36.9240584753882,-29.9561939713103,20.));
#89371=CARTESIAN_POINT('Ctrl Pts',(36.9008197053507,-29.9800549451122,0.));
#89372=CARTESIAN_POINT('Ctrl Pts',(36.9008197053507,-29.9800549451122,20.));
#89373=CARTESIAN_POINT('Ctrl Pts',(36.8775650729895,-30.003898900255,0.));
#89374=CARTESIAN_POINT('Ctrl Pts',(36.8775650729895,-30.003898900255,20.));
#89375=CARTESIAN_POINT('Ctrl Pts',(36.8542945902472,-30.0277258257394,0.));
#89376=CARTESIAN_POINT('Ctrl Pts',(36.8542945902472,-30.0277258257394,20.));
#89377=CARTESIAN_POINT('Ctrl Pts',(36.8310082690741,-30.051535710574,0.));
#89378=CARTESIAN_POINT('Ctrl Pts',(36.8310082690741,-30.051535710574,20.));
#89379=CARTESIAN_POINT('Ctrl Pts',(36.8077061214283,-30.0753285437754,0.));
#89380=CARTESIAN_POINT('Ctrl Pts',(36.8077061214283,-30.0753285437754,20.));
#89381=CARTESIAN_POINT('Ctrl Pts',(36.7843881592759,-30.0991043143685,0.));
#89382=CARTESIAN_POINT('Ctrl Pts',(36.7843881592759,-30.0991043143685,20.));
#89383=CARTESIAN_POINT('Ctrl Pts',(36.7610543945915,-30.1228630113862,0.));
#89384=CARTESIAN_POINT('Ctrl Pts',(36.7610543945915,-30.1228630113862,20.));
#89385=CARTESIAN_POINT('Ctrl Pts',(36.7377048393574,-30.1466046238701,0.));
#89386=CARTESIAN_POINT('Ctrl Pts',(36.7377048393574,-30.1466046238701,20.));
#89387=CARTESIAN_POINT('Ctrl Pts',(36.7143395055641,-30.1703291408693,0.));
#89388=CARTESIAN_POINT('Ctrl Pts',(36.7143395055641,-30.1703291408693,20.));
#89389=CARTESIAN_POINT('Ctrl Pts',(36.6909584052099,-30.1940365514414,0.));
#89390=CARTESIAN_POINT('Ctrl Pts',(36.6909584052099,-30.1940365514414,20.));
#89391=CARTESIAN_POINT('Ctrl Pts',(36.6675615503012,-30.2177268446518,0.));
#89392=CARTESIAN_POINT('Ctrl Pts',(36.6675615503012,-30.2177268446518,20.));
#89393=CARTESIAN_POINT('Ctrl Pts',(36.6441489528521,-30.2414000095742,0.));
#89394=CARTESIAN_POINT('Ctrl Pts',(36.6441489528521,-30.2414000095742,20.));
#89395=CARTESIAN_POINT('Ctrl Pts',(36.6207206248848,-30.2650560352902,0.));
#89396=CARTESIAN_POINT('Ctrl Pts',(36.6207206248848,-30.2650560352902,20.));
#89397=CARTESIAN_POINT('Ctrl Pts',(36.5972765784293,-30.2886949108895,0.));
#89398=CARTESIAN_POINT('Ctrl Pts',(36.5972765784293,-30.2886949108895,20.));
#89399=CARTESIAN_POINT('Ctrl Pts',(36.5738168255233,-30.3123166254701,0.));
#89400=CARTESIAN_POINT('Ctrl Pts',(36.5738168255233,-30.3123166254701,20.));
#89401=CARTESIAN_POINT('Ctrl Pts',(36.5503413782123,-30.3359211681376,0.));
#89402=CARTESIAN_POINT('Ctrl Pts',(36.5503413782123,-30.3359211681376,20.));
#89403=CARTESIAN_POINT('Ctrl Pts',(36.5268502485502,-30.3595085280059,0.));
#89404=CARTESIAN_POINT('Ctrl Pts',(36.5268502485502,-30.3595085280059,20.));
#89405=CARTESIAN_POINT('Ctrl Pts',(36.5033434485984,-30.3830786941972,0.));
#89406=CARTESIAN_POINT('Ctrl Pts',(36.5033434485984,-30.3830786941972,20.));
#89407=CARTESIAN_POINT('Ctrl Pts',(36.4798209904267,-30.4066316558424,0.));
#89408=CARTESIAN_POINT('Ctrl Pts',(36.4798209904267,-30.4066316558424,20.));
#89409=CARTESIAN_POINT('Ctrl Pts',(36.456282886113,-30.4301674020802,0.));
#89410=CARTESIAN_POINT('Ctrl Pts',(36.456282886113,-30.4301674020802,20.));
#89411=CARTESIAN_POINT('Ctrl Pts',(36.4327291477428,-30.4536859220576,0.));
#89412=CARTESIAN_POINT('Ctrl Pts',(36.4327291477428,-30.4536859220576,20.));
#89413=CARTESIAN_POINT('Ctrl Pts',(36.4091597874097,-30.4771872049299,0.));
#89414=CARTESIAN_POINT('Ctrl Pts',(36.4091597874097,-30.4771872049299,20.));
#89415=CARTESIAN_POINT('Ctrl Pts',(36.3855748172148,-30.5006712398601,0.));
#89416=CARTESIAN_POINT('Ctrl Pts',(36.3855748172148,-30.5006712398601,20.));
#89417=CARTESIAN_POINT('Ctrl Pts',(36.3619742492671,-30.5241380160195,0.));
#89418=CARTESIAN_POINT('Ctrl Pts',(36.3619742492671,-30.5241380160195,20.));
#89419=CARTESIAN_POINT('Ctrl Pts',(36.3383580956832,-30.5475875225872,0.));
#89420=CARTESIAN_POINT('Ctrl Pts',(36.3383580956832,-30.5475875225872,20.));
#89421=CARTESIAN_POINT('Ctrl Pts',(36.3147263685874,-30.5710197487502,0.));
#89422=CARTESIAN_POINT('Ctrl Pts',(36.3147263685874,-30.5710197487502,20.));
#89423=CARTESIAN_POINT('Ctrl Pts',(36.2910790801119,-30.5944346837039,0.));
#89424=CARTESIAN_POINT('Ctrl Pts',(36.2910790801119,-30.5944346837039,20.));
#89425=CARTESIAN_POINT('Ctrl Pts',(36.2674162423973,-30.6178323166527,0.));
#89426=CARTESIAN_POINT('Ctrl Pts',(36.2674162423973,-30.6178323166527,20.));
#89427=CARTESIAN_POINT('Ctrl Pts',(36.2437378675924,-30.6412126368095,0.));
#89428=CARTESIAN_POINT('Ctrl Pts',(36.2437378675924,-30.6412126368095,20.));
#89429=CARTESIAN_POINT('Ctrl Pts',(36.2200439678542,-30.6645756333955,0.));
#89430=CARTESIAN_POINT('Ctrl Pts',(36.2200439678542,-30.6645756333955,20.));
#89431=CARTESIAN_POINT('Ctrl Pts',(36.196334555347,-30.6879212956392,0.));
#89432=CARTESIAN_POINT('Ctrl Pts',(36.196334555347,-30.6879212956392,20.));
#89433=CARTESIAN_POINT('Ctrl Pts',(36.1726096422428,-30.7112496127774,0.));
#89434=CARTESIAN_POINT('Ctrl Pts',(36.1726096422428,-30.7112496127774,20.));
#89435=CARTESIAN_POINT('Ctrl Pts',(36.1488692407204,-30.7345605740545,0.));
#89436=CARTESIAN_POINT('Ctrl Pts',(36.1488692407204,-30.7345605740545,20.));
#89437=CARTESIAN_POINT('Ctrl Pts',(36.1251133629669,-30.7578541687236,0.));
#89438=CARTESIAN_POINT('Ctrl Pts',(36.1251133629669,-30.7578541687236,20.));
#89439=CARTESIAN_POINT('Ctrl Pts',(36.1013420211777,-30.7811303860468,0.));
#89440=CARTESIAN_POINT('Ctrl Pts',(36.1013420211777,-30.7811303860468,20.));
#89441=CARTESIAN_POINT('Ctrl Pts',(36.0775552275565,-30.8043892152943,0.));
#89442=CARTESIAN_POINT('Ctrl Pts',(36.0775552275565,-30.8043892152943,20.));
#89443=CARTESIAN_POINT('Ctrl Pts',(36.0537529943146,-30.8276306457446,0.));
#89444=CARTESIAN_POINT('Ctrl Pts',(36.0537529943146,-30.8276306457446,20.));
#89445=CARTESIAN_POINT('Ctrl Pts',(36.0299353336712,-30.8508546666841,0.));
#89446=CARTESIAN_POINT('Ctrl Pts',(36.0299353336712,-30.8508546666841,20.));
#89447=CARTESIAN_POINT('Ctrl Pts',(36.0061022578528,-30.8740612674075,0.));
#89448=CARTESIAN_POINT('Ctrl Pts',(36.0061022578528,-30.8740612674075,20.));
#89449=CARTESIAN_POINT('Ctrl Pts',(35.9822537790931,-30.8972504372171,0.));
#89450=CARTESIAN_POINT('Ctrl Pts',(35.9822537790931,-30.8972504372171,20.));
#89451=CARTESIAN_POINT('Ctrl Pts',(35.9583899096339,-30.9204221654236,0.));
#89452=CARTESIAN_POINT('Ctrl Pts',(35.9583899096339,-30.9204221654236,20.));
#89453=CARTESIAN_POINT('Ctrl Pts',(35.9345106617251,-30.9435764413467,0.));
#89454=CARTESIAN_POINT('Ctrl Pts',(35.9345106617251,-30.9435764413467,20.));
#89455=CARTESIAN_POINT('Ctrl Pts',(35.9106160476245,-30.9667132543142,0.));
#89456=CARTESIAN_POINT('Ctrl Pts',(35.9106160476245,-30.9667132543142,20.));
#89457=CARTESIAN_POINT('Ctrl Pts',(35.886706079598,-30.9898325936627,0.));
#89458=CARTESIAN_POINT('Ctrl Pts',(35.886706079598,-30.9898325936627,20.));
#89459=CARTESIAN_POINT('Ctrl Pts',(35.8627807699193,-31.0129344487367,0.));
#89460=CARTESIAN_POINT('Ctrl Pts',(35.8627807699193,-31.0129344487367,20.));
#89461=CARTESIAN_POINT('Ctrl Pts',(35.8388401308696,-31.036018808889,0.));
#89462=CARTESIAN_POINT('Ctrl Pts',(35.8388401308696,-31.036018808889,20.));
#89463=CARTESIAN_POINT('Ctrl Pts',(35.8148841747376,-31.0590856634804,0.));
#89464=CARTESIAN_POINT('Ctrl Pts',(35.8148841747376,-31.0590856634804,20.));
#89465=CARTESIAN_POINT('Ctrl Pts',(35.7909129138202,-31.082135001881,0.));
#89466=CARTESIAN_POINT('Ctrl Pts',(35.7909129138202,-31.082135001881,20.));
#89467=CARTESIAN_POINT('Ctrl Pts',(35.7669263604212,-31.1051668134678,0.));
#89468=CARTESIAN_POINT('Ctrl Pts',(35.7669263604212,-31.1051668134678,20.));
#89469=CARTESIAN_POINT('Ctrl Pts',(35.7429245268523,-31.1281810876267,0.));
#89470=CARTESIAN_POINT('Ctrl Pts',(35.7429245268523,-31.1281810876267,20.));
#89471=CARTESIAN_POINT('Ctrl Pts',(35.7189074254331,-31.1511778137516,0.));
#89472=CARTESIAN_POINT('Ctrl Pts',(35.7189074254331,-31.1511778137516,20.));
#89473=CARTESIAN_POINT('Ctrl Pts',(35.6948750684911,-31.1741569812451,0.));
#89474=CARTESIAN_POINT('Ctrl Pts',(35.6948750684911,-31.1741569812451,20.));
#89475=CARTESIAN_POINT('Ctrl Pts',(35.6708274683619,-31.1971185795181,0.));
#89476=CARTESIAN_POINT('Ctrl Pts',(35.6708274683619,-31.1971185795181,20.));
#89477=CARTESIAN_POINT('Ctrl Pts',(35.6467646373883,-31.2200625979904,0.));
#89478=CARTESIAN_POINT('Ctrl Pts',(35.6467646373883,-31.2200625979904,20.));
#89479=CARTESIAN_POINT('Ctrl Pts',(35.6226865879214,-31.24298902609,0.));
#89480=CARTESIAN_POINT('Ctrl Pts',(35.6226865879214,-31.24298902609,20.));
#89481=CARTESIAN_POINT('Ctrl Pts',(35.5985933323194,-31.2658978532533,0.));
#89482=CARTESIAN_POINT('Ctrl Pts',(35.5985933323194,-31.2658978532533,20.));
#89483=CARTESIAN_POINT('Ctrl Pts',(35.5744848829487,-31.288789068925,0.));
#89484=CARTESIAN_POINT('Ctrl Pts',(35.5744848829487,-31.288789068925,20.));
#89485=CARTESIAN_POINT('Ctrl Pts',(35.5503612521832,-31.3116626625581,0.));
#89486=CARTESIAN_POINT('Ctrl Pts',(35.5503612521832,-31.3116626625581,20.));
#89487=CARTESIAN_POINT('Ctrl Pts',(35.5262224524039,-31.3345186236135,0.));
#89488=CARTESIAN_POINT('Ctrl Pts',(35.5262224524039,-31.3345186236135,20.));
#89489=CARTESIAN_POINT('Ctrl Pts',(35.502068496,-31.3573569415606,0.));
#89490=CARTESIAN_POINT('Ctrl Pts',(35.502068496,-31.3573569415606,20.));
#89491=CARTESIAN_POINT('Ctrl Pts',(35.4778993953681,-31.3801776058768,0.));
#89492=CARTESIAN_POINT('Ctrl Pts',(35.4778993953681,-31.3801776058768,20.));
#89493=CARTESIAN_POINT('Ctrl Pts',(35.4537151629126,-31.4029806060482,0.));
#89494=CARTESIAN_POINT('Ctrl Pts',(35.4537151629126,-31.4029806060482,20.));
#89495=CARTESIAN_POINT('Ctrl Pts',(35.4295158110454,-31.4257659315696,0.));
#89496=CARTESIAN_POINT('Ctrl Pts',(35.4295158110454,-31.4257659315696,20.));
#89497=CARTESIAN_POINT('Ctrl Pts',(35.4053013521866,-31.4485335719447,0.));
#89498=CARTESIAN_POINT('Ctrl Pts',(35.4053013521866,-31.4485335719447,20.));
#89499=CARTESIAN_POINT('Ctrl Pts',(35.3810717987641,-31.4712835166857,0.));
#89500=CARTESIAN_POINT('Ctrl Pts',(35.3810717987641,-31.4712835166857,20.));
#89501=CARTESIAN_POINT('Ctrl Pts',(35.3568271632136,-31.4940157553136,0.));
#89502=CARTESIAN_POINT('Ctrl Pts',(35.3568271632136,-31.4940157553136,20.));
#89503=CARTESIAN_POINT('Ctrl Pts',(35.3325674579779,-31.516730277357,0.));
#89504=CARTESIAN_POINT('Ctrl Pts',(35.3325674579779,-31.516730277357,20.));
#89505=CARTESIAN_POINT('Ctrl Pts',(35.3082926955072,-31.5394270723526,0.));
#89506=CARTESIAN_POINT('Ctrl Pts',(35.3082926955072,-31.5394270723526,20.));
#89507=CARTESIAN_POINT('Ctrl Pts',(35.2840028882593,-31.5621061298453,0.));
#89508=CARTESIAN_POINT('Ctrl Pts',(35.2840028882593,-31.5621061298453,20.));
#89509=CARTESIAN_POINT('Ctrl Pts',(35.2596980486996,-31.5847674393885,0.));
#89510=CARTESIAN_POINT('Ctrl Pts',(35.2596980486996,-31.5847674393885,20.));
#89511=CARTESIAN_POINT('Ctrl Pts',(35.2353781893014,-31.6074109905439,0.));
#89512=CARTESIAN_POINT('Ctrl Pts',(35.2353781893014,-31.6074109905439,20.));
#89513=CARTESIAN_POINT('Ctrl Pts',(35.2110433225458,-31.6300367728827,0.));
#89514=CARTESIAN_POINT('Ctrl Pts',(35.2110433225458,-31.6300367728827,20.));
#89515=CARTESIAN_POINT('Ctrl Pts',(35.1866934609214,-31.652644775984,0.));
#89516=CARTESIAN_POINT('Ctrl Pts',(35.1866934609214,-31.652644775984,20.));
#89517=CARTESIAN_POINT('Ctrl Pts',(35.1623286169245,-31.6752349894358,0.));
#89518=CARTESIAN_POINT('Ctrl Pts',(35.1623286169245,-31.6752349894358,20.));
#89519=CARTESIAN_POINT('Ctrl Pts',(35.1379488030591,-31.6978074028349,0.));
#89520=CARTESIAN_POINT('Ctrl Pts',(35.1379488030591,-31.6978074028349,20.));
#89521=CARTESIAN_POINT('Ctrl Pts',(35.1135540318367,-31.7203620057864,0.));
#89522=CARTESIAN_POINT('Ctrl Pts',(35.1135540318367,-31.7203620057864,20.));
#89523=CARTESIAN_POINT('Ctrl Pts',(35.0891443157764,-31.7428987879035,0.));
#89524=CARTESIAN_POINT('Ctrl Pts',(35.0891443157764,-31.7428987879035,20.));
#89525=CARTESIAN_POINT('Ctrl Pts',(35.0647196674043,-31.7654177388073,0.));
#89526=CARTESIAN_POINT('Ctrl Pts',(35.0647196674043,-31.7654177388073,20.));
#89527=CARTESIAN_POINT('Ctrl Pts',(35.0402800992547,-31.7879188481278,0.));
#89528=CARTESIAN_POINT('Ctrl Pts',(35.0402800992547,-31.7879188481278,20.));
#89529=CARTESIAN_POINT('Ctrl Pts',(35.0158256238691,-31.8104021055033,0.));
#89530=CARTESIAN_POINT('Ctrl Pts',(35.0158256238691,-31.8104021055033,20.));
#89531=CARTESIAN_POINT('Ctrl Pts',(34.991356253797,-31.8328675005809,0.));
#89532=CARTESIAN_POINT('Ctrl Pts',(34.991356253797,-31.8328675005809,20.));
#89533=CARTESIAN_POINT('Ctrl Pts',(34.9668720015954,-31.8553150230168,0.));
#89534=CARTESIAN_POINT('Ctrl Pts',(34.9668720015954,-31.8553150230168,20.));
#89535=CARTESIAN_POINT('Ctrl Pts',(34.9423728798289,-31.8777446624754,0.));
#89536=CARTESIAN_POINT('Ctrl Pts',(34.9423728798289,-31.8777446624754,20.));
#89537=CARTESIAN_POINT('Ctrl Pts',(34.9178589010694,-31.9001564086295,0.));
#89538=CARTESIAN_POINT('Ctrl Pts',(34.9178589010694,-31.9001564086295,20.));
#89539=CARTESIAN_POINT('Ctrl Pts',(34.8933300778963,-31.9225502511603,0.));
#89540=CARTESIAN_POINT('Ctrl Pts',(34.8933300778963,-31.9225502511603,20.));
#89541=CARTESIAN_POINT('Ctrl Pts',(34.8687864228965,-31.9449261797574,0.));
#89542=CARTESIAN_POINT('Ctrl Pts',(34.8687864228965,-31.9449261797574,20.));
#89543=CARTESIAN_POINT('Ctrl Pts',(34.8442279486644,-31.967284184119,0.));
#89544=CARTESIAN_POINT('Ctrl Pts',(34.8442279486644,-31.967284184119,20.));
#89545=CARTESIAN_POINT('Ctrl Pts',(34.8196546678026,-31.9896242539524,0.));
#89546=CARTESIAN_POINT('Ctrl Pts',(34.8196546678026,-31.9896242539524,20.));
#89547=CARTESIAN_POINT('Ctrl Pts',(34.7950665929206,-32.011946378973,0.));
#89548=CARTESIAN_POINT('Ctrl Pts',(34.7950665929206,-32.011946378973,20.));
#89549=CARTESIAN_POINT('Ctrl Pts',(34.7704637366357,-32.0342505489048,0.));
#89550=CARTESIAN_POINT('Ctrl Pts',(34.7704637366357,-32.0342505489048,20.));
#89551=CARTESIAN_POINT('Ctrl Pts',(34.7458461115727,-32.0565367534806,0.));
#89552=CARTESIAN_POINT('Ctrl Pts',(34.7458461115727,-32.0565367534806,20.));
#89553=CARTESIAN_POINT('Ctrl Pts',(34.7212137303638,-32.0788049824416,0.));
#89554=CARTESIAN_POINT('Ctrl Pts',(34.7212137303638,-32.0788049824416,20.));
#89555=CARTESIAN_POINT('Ctrl Pts',(34.6965666056491,-32.1010552255379,0.));
#89556=CARTESIAN_POINT('Ctrl Pts',(34.6965666056491,-32.1010552255379,20.));
#89557=CARTESIAN_POINT('Ctrl Pts',(34.6719047500757,-32.1232874725277,0.));
#89558=CARTESIAN_POINT('Ctrl Pts',(34.6719047500757,-32.1232874725277,20.));
#89559=CARTESIAN_POINT('Ctrl Pts',(34.6472281762982,-32.145501713178,0.));
#89560=CARTESIAN_POINT('Ctrl Pts',(34.6472281762982,-32.145501713178,20.));
#89561=CARTESIAN_POINT('Ctrl Pts',(34.6225368969784,-32.167697937264,0.));
#89562=CARTESIAN_POINT('Ctrl Pts',(34.6225368969784,-32.167697937264,20.));
#89563=CARTESIAN_POINT('Ctrl Pts',(34.5978309247855,-32.1898761345694,0.));
#89564=CARTESIAN_POINT('Ctrl Pts',(34.5978309247855,-32.1898761345694,20.));
#89565=CARTESIAN_POINT('Ctrl Pts',(34.5731102723969,-32.212036294887,0.));
#89566=CARTESIAN_POINT('Ctrl Pts',(34.5731102723969,-32.212036294887,20.));
#89567=CARTESIAN_POINT('Ctrl Pts',(34.5483749524972,-32.2341784080184,0.));
#89568=CARTESIAN_POINT('Ctrl Pts',(34.5483749524972,-32.2341784080184,20.));
#89569=CARTESIAN_POINT('Ctrl Pts',(34.5236249777791,-32.2563024637739,0.));
#89570=CARTESIAN_POINT('Ctrl Pts',(34.5236249777791,-32.2563024637739,20.));
#89571=CARTESIAN_POINT('Ctrl Pts',(34.4988603609426,-32.2784084519728,0.));
#89572=CARTESIAN_POINT('Ctrl Pts',(34.4988603609426,-32.2784084519728,20.));
#89573=CARTESIAN_POINT('Ctrl Pts',(34.474081114695,-32.3004963624427,0.));
#89574=CARTESIAN_POINT('Ctrl Pts',(34.474081114695,-32.3004963624427,20.));
#89575=CARTESIAN_POINT('Ctrl Pts',(34.4492872517507,-32.3225661850195,0.));
#89576=CARTESIAN_POINT('Ctrl Pts',(34.4492872517507,-32.3225661850195,20.));
#89577=CARTESIAN_POINT('Ctrl Pts',(34.4244787848311,-32.3446179095474,0.));
#89578=CARTESIAN_POINT('Ctrl Pts',(34.4244787848311,-32.3446179095474,20.));
#89579=CARTESIAN_POINT('Ctrl Pts',(34.3996557266651,-32.3666515258788,0.));
#89580=CARTESIAN_POINT('Ctrl Pts',(34.3996557266651,-32.3666515258788,20.));
#89581=CARTESIAN_POINT('Ctrl Pts',(34.3748180899889,-32.388667023875,0.));
#89582=CARTESIAN_POINT('Ctrl Pts',(34.3748180899889,-32.388667023875,20.));
#89583=CARTESIAN_POINT('Ctrl Pts',(34.3499658875467,-32.4106643934066,0.));
#89584=CARTESIAN_POINT('Ctrl Pts',(34.3499658875467,-32.4106643934066,20.));
#89585=CARTESIAN_POINT('Ctrl Pts',(34.3250991320904,-32.4326436243533,0.));
#89586=CARTESIAN_POINT('Ctrl Pts',(34.3250991320904,-32.4326436243533,20.));
#89587=CARTESIAN_POINT('Ctrl Pts',(34.3002178363797,-32.4546047066034,0.));
#89588=CARTESIAN_POINT('Ctrl Pts',(34.3002178363797,-32.4546047066034,20.));
#89589=CARTESIAN_POINT('Ctrl Pts',(34.2753220131812,-32.4765476300538,0.));
#89590=CARTESIAN_POINT('Ctrl Pts',(34.2753220131812,-32.4765476300538,20.));
#89591=CARTESIAN_POINT('Ctrl Pts',(34.2504116752689,-32.4984723846098,0.));
#89592=CARTESIAN_POINT('Ctrl Pts',(34.2504116752689,-32.4984723846098,20.));
#89593=CARTESIAN_POINT('Ctrl Pts',(34.2254868354237,-32.5203789601849,0.));
#89594=CARTESIAN_POINT('Ctrl Pts',(34.2254868354237,-32.5203789601849,20.));
#89595=CARTESIAN_POINT('Ctrl Pts',(34.2005475064343,-32.542267346702,0.));
#89596=CARTESIAN_POINT('Ctrl Pts',(34.2005475064343,-32.542267346702,20.));
#89597=CARTESIAN_POINT('Ctrl Pts',(34.1755937010962,-32.564137534092,0.));
#89598=CARTESIAN_POINT('Ctrl Pts',(34.1755937010962,-32.564137534092,20.));
#89599=CARTESIAN_POINT('Ctrl Pts',(34.1506254322131,-32.585989512295,0.));
#89600=CARTESIAN_POINT('Ctrl Pts',(34.1506254322131,-32.585989512295,20.));
#89601=CARTESIAN_POINT('Ctrl Pts',(34.1256427125955,-32.6078232712594,0.));
#89602=CARTESIAN_POINT('Ctrl Pts',(34.1256427125955,-32.6078232712594,20.));
#89603=CARTESIAN_POINT('Ctrl Pts',(34.1006455550618,-32.6296388009428,0.));
#89604=CARTESIAN_POINT('Ctrl Pts',(34.1006455550618,-32.6296388009428,20.));
#89605=CARTESIAN_POINT('Ctrl Pts',(34.0756339724376,-32.6514360913116,0.));
#89606=CARTESIAN_POINT('Ctrl Pts',(34.0756339724376,-32.6514360913116,20.));
#89607=CARTESIAN_POINT('Ctrl Pts',(34.0506079775557,-32.6732151323407,0.));
#89608=CARTESIAN_POINT('Ctrl Pts',(34.0506079775557,-32.6732151323407,20.));
#89609=CARTESIAN_POINT('Ctrl Pts',(34.0255675832564,-32.694975914014,0.));
#89610=CARTESIAN_POINT('Ctrl Pts',(34.0255675832564,-32.694975914014,20.));
#89611=CARTESIAN_POINT('Ctrl Pts',(34.0005128023871,-32.7167184263237,0.));
#89612=CARTESIAN_POINT('Ctrl Pts',(34.0005128023871,-32.7167184263237,20.));
#89613=CARTESIAN_POINT('Ctrl Pts',(33.9754436478026,-32.7384426592708,0.));
#89614=CARTESIAN_POINT('Ctrl Pts',(33.9754436478026,-32.7384426592708,20.));
#89615=CARTESIAN_POINT('Ctrl Pts',(33.950360132365,-32.7601486028652,0.));
#89616=CARTESIAN_POINT('Ctrl Pts',(33.950360132365,-32.7601486028652,20.));
#89617=CARTESIAN_POINT('Ctrl Pts',(33.9252622689445,-32.781836247126,0.));
#89618=CARTESIAN_POINT('Ctrl Pts',(33.9252622689445,-32.781836247126,20.));
#89619=CARTESIAN_POINT('Ctrl Pts',(33.9001500704179,-32.8035055820806,0.));
#89620=CARTESIAN_POINT('Ctrl Pts',(33.9001500704179,-32.8035055820806,20.));
#89621=CARTESIAN_POINT('Ctrl Pts',(33.8750235496691,-32.8251565977646,0.));
#89622=CARTESIAN_POINT('Ctrl Pts',(33.8750235496691,-32.8251565977646,20.));
#89623=CARTESIAN_POINT('Ctrl Pts',(33.8498827195893,-32.8467892842227,0.));
#89624=CARTESIAN_POINT('Ctrl Pts',(33.8498827195893,-32.8467892842227,20.));
#89625=CARTESIAN_POINT('Ctrl Pts',(33.8247275930774,-32.8684036315086,0.));
#89626=CARTESIAN_POINT('Ctrl Pts',(33.8247275930774,-32.8684036315086,20.));
#89627=CARTESIAN_POINT('Ctrl Pts',(33.7995581830395,-32.8899996296849,0.));
#89628=CARTESIAN_POINT('Ctrl Pts',(33.7995581830395,-32.8899996296849,20.));
#89629=CARTESIAN_POINT('Ctrl Pts',(33.7743745023893,-32.9115772688235,0.));
#89630=CARTESIAN_POINT('Ctrl Pts',(33.7743745023893,-32.9115772688235,20.));
#89631=CARTESIAN_POINT('Ctrl Pts',(33.7491765640476,-32.9331365390046,0.));
#89632=CARTESIAN_POINT('Ctrl Pts',(33.7491765640476,-32.9331365390046,20.));
#89633=CARTESIAN_POINT('Ctrl Pts',(33.723964380943,-32.9546774303179,0.));
#89634=CARTESIAN_POINT('Ctrl Pts',(33.723964380943,-32.9546774303179,20.));
#89635=CARTESIAN_POINT('Ctrl Pts',(33.6987379660104,-32.9761999328605,0.));
#89636=CARTESIAN_POINT('Ctrl Pts',(33.6987379660104,-32.9761999328605,20.));
#89637=CARTESIAN_POINT('Ctrl Pts',(33.6734973321919,-32.9977040367383,0.));
#89638=CARTESIAN_POINT('Ctrl Pts',(33.6734973321919,-32.9977040367383,20.));
#89639=CARTESIAN_POINT('Ctrl Pts',(33.6482424924372,-33.0191897320665,0.));
#89640=CARTESIAN_POINT('Ctrl Pts',(33.6482424924372,-33.0191897320665,20.));
#89641=CARTESIAN_POINT('Ctrl Pts',(33.6229734597032,-33.0406570089692,0.));
#89642=CARTESIAN_POINT('Ctrl Pts',(33.6229734597032,-33.0406570089692,20.));
#89643=CARTESIAN_POINT('Ctrl Pts',(33.5976902469543,-33.0621058575797,0.));
#89644=CARTESIAN_POINT('Ctrl Pts',(33.5976902469543,-33.0621058575797,20.));
#89645=CARTESIAN_POINT('Ctrl Pts',(33.572392867162,-33.0835362680399,0.));
#89646=CARTESIAN_POINT('Ctrl Pts',(33.572392867162,-33.0835362680399,20.));
#89647=CARTESIAN_POINT('Ctrl Pts',(33.5470813333053,-33.1049482305004,0.));
#89648=CARTESIAN_POINT('Ctrl Pts',(33.5470813333053,-33.1049482305004,20.));
#89649=CARTESIAN_POINT('Ctrl Pts',(33.5217556583703,-33.1263417351208,0.));
#89650=CARTESIAN_POINT('Ctrl Pts',(33.5217556583703,-33.1263417351208,20.));
#89651=CARTESIAN_POINT('Ctrl Pts',(33.4964158553505,-33.1477167720697,0.));
#89652=CARTESIAN_POINT('Ctrl Pts',(33.4964158553505,-33.1477167720697,20.));
#89653=CARTESIAN_POINT('Ctrl Pts',(33.4710619372468,-33.1690733315248,0.));
#89654=CARTESIAN_POINT('Ctrl Pts',(33.4710619372468,-33.1690733315248,20.));
#89655=CARTESIAN_POINT('Ctrl Pts',(33.4456939170666,-33.1904114036721,0.));
#89656=CARTESIAN_POINT('Ctrl Pts',(33.4456939170666,-33.1904114036721,20.));
#89657=CARTESIAN_POINT('Ctrl Pts',(33.4203118078248,-33.2117309787064,0.));
#89658=CARTESIAN_POINT('Ctrl Pts',(33.4203118078248,-33.2117309787064,20.));
#89659=CARTESIAN_POINT('Ctrl Pts',(33.3949156225429,-33.233032046831,0.));
#89660=CARTESIAN_POINT('Ctrl Pts',(33.3949156225429,-33.233032046831,20.));
#89661=CARTESIAN_POINT('Ctrl Pts',(33.3695053742505,-33.2543145982587,0.));
#89662=CARTESIAN_POINT('Ctrl Pts',(33.3695053742505,-33.2543145982587,20.));
#89663=CARTESIAN_POINT('Ctrl Pts',(33.3440810759838,-33.2755786232108,0.));
#89664=CARTESIAN_POINT('Ctrl Pts',(33.3440810759838,-33.2755786232108,20.));
#89665=CARTESIAN_POINT('Ctrl Pts',(33.3186427407863,-33.2968241119177,0.));
#89666=CARTESIAN_POINT('Ctrl Pts',(33.3186427407863,-33.2968241119177,20.));
#89667=CARTESIAN_POINT('Ctrl Pts',(33.2931903817093,-33.318051054619,0.));
#89668=CARTESIAN_POINT('Ctrl Pts',(33.2931903817093,-33.318051054619,20.));
#89669=CARTESIAN_POINT('Ctrl Pts',(33.2677240118112,-33.3392594415636,0.));
#89670=CARTESIAN_POINT('Ctrl Pts',(33.2677240118112,-33.3392594415636,20.));
#89671=CARTESIAN_POINT('Ctrl Pts',(33.2422436441578,-33.3604492630093,0.));
#89672=CARTESIAN_POINT('Ctrl Pts',(33.2422436441578,-33.3604492630093,20.));
#89673=CARTESIAN_POINT('Ctrl Pts',(33.2167492918215,-33.3816205092222,0.));
#89674=CARTESIAN_POINT('Ctrl Pts',(33.2167492918215,-33.3816205092222,20.));
#89675=CARTESIAN_POINT('Ctrl Pts',(33.1912409678819,-33.4027731704774,0.));
#89676=CARTESIAN_POINT('Ctrl Pts',(33.1912409678819,-33.4027731704774,20.));
#89677=CARTESIAN_POINT('Ctrl Pts',(33.1657186854252,-33.4239072370581,0.));
#89678=CARTESIAN_POINT('Ctrl Pts',(33.1657186854252,-33.4239072370581,20.));
#89679=CARTESIAN_POINT('Ctrl Pts',(33.1401824575448,-33.4450226992568,0.));
#89680=CARTESIAN_POINT('Ctrl Pts',(33.1401824575448,-33.4450226992568,20.));
#89681=CARTESIAN_POINT('Ctrl Pts',(33.1146322973416,-33.4661195473749,0.));
#89682=CARTESIAN_POINT('Ctrl Pts',(33.1146322973416,-33.4661195473749,20.));
#89683=CARTESIAN_POINT('Ctrl Pts',(33.0890682179238,-33.4871977717238,0.));
#89684=CARTESIAN_POINT('Ctrl Pts',(33.0890682179238,-33.4871977717238,20.));
#89685=CARTESIAN_POINT('Ctrl Pts',(33.063490232407,-33.5082573626235,0.));
#89686=CARTESIAN_POINT('Ctrl Pts',(33.063490232407,-33.5082573626235,20.));
#89687=CARTESIAN_POINT('Ctrl Pts',(33.0378983539137,-33.5292983104032,0.));
#89688=CARTESIAN_POINT('Ctrl Pts',(33.0378983539137,-33.5292983104032,20.));
#89689=CARTESIAN_POINT('Ctrl Pts',(33.0122925955738,-33.5503206054004,0.));
#89690=CARTESIAN_POINT('Ctrl Pts',(33.0122925955738,-33.5503206054004,20.));
#89691=CARTESIAN_POINT('Ctrl Pts',(32.986672970524,-33.5713242379612,0.));
#89692=CARTESIAN_POINT('Ctrl Pts',(32.986672970524,-33.5713242379612,20.));
#89693=CARTESIAN_POINT('Ctrl Pts',(32.9610394919081,-33.5923091984411,0.));
#89694=CARTESIAN_POINT('Ctrl Pts',(32.9610394919081,-33.5923091984411,20.));
#89695=CARTESIAN_POINT('Ctrl Pts',(32.935392172877,-33.6132754772046,0.));
#89696=CARTESIAN_POINT('Ctrl Pts',(32.935392172877,-33.6132754772046,20.));
#89697=CARTESIAN_POINT('Ctrl Pts',(32.9097310265884,-33.6342230646254,0.));
#89698=CARTESIAN_POINT('Ctrl Pts',(32.9097310265884,-33.6342230646254,20.));
#89699=CARTESIAN_POINT('Ctrl Pts',(32.8840560662069,-33.6551519510862,0.));
#89700=CARTESIAN_POINT('Ctrl Pts',(32.8840560662069,-33.6551519510862,20.));
#89701=CARTESIAN_POINT('Ctrl Pts',(32.8583673049046,-33.6760621269785,0.));
#89702=CARTESIAN_POINT('Ctrl Pts',(32.8583673049046,-33.6760621269785,20.));
#89703=CARTESIAN_POINT('Ctrl Pts',(32.8326647558605,-33.6969535827028,0.));
#89704=CARTESIAN_POINT('Ctrl Pts',(32.8326647558605,-33.6969535827028,20.));
#89705=CARTESIAN_POINT('Ctrl Pts',(32.8069484322617,-33.717826308669,0.));
#89706=CARTESIAN_POINT('Ctrl Pts',(32.8069484322617,-33.717826308669,20.));
#89707=CARTESIAN_POINT('Ctrl Pts',(32.7812183473018,-33.7386802952956,0.));
#89708=CARTESIAN_POINT('Ctrl Pts',(32.7812183473018,-33.7386802952956,20.));
#89709=CARTESIAN_POINT('Ctrl Pts',(32.755474514181,-33.7595155330097,0.));
#89710=CARTESIAN_POINT('Ctrl Pts',(32.755474514181,-33.7595155330097,20.));
#89711=CARTESIAN_POINT('Ctrl Pts',(32.7297169461064,-33.7803320122473,0.));
#89712=CARTESIAN_POINT('Ctrl Pts',(32.7297169461064,-33.7803320122473,20.));
#89713=CARTESIAN_POINT('Ctrl Pts',(32.7039456562922,-33.8011297234537,0.));
#89714=CARTESIAN_POINT('Ctrl Pts',(32.7039456562922,-33.8011297234537,20.));
#89715=CARTESIAN_POINT('Ctrl Pts',(32.6781606579597,-33.8219086570836,0.));
#89716=CARTESIAN_POINT('Ctrl Pts',(32.6781606579597,-33.8219086570836,20.));
#89717=CARTESIAN_POINT('Ctrl Pts',(32.652361964338,-33.8426688036011,0.));
#89718=CARTESIAN_POINT('Ctrl Pts',(32.652361964338,-33.8426688036011,20.));
#89719=CARTESIAN_POINT('Ctrl Pts',(32.6265495886629,-33.8634101534794,0.));
#89720=CARTESIAN_POINT('Ctrl Pts',(32.6265495886629,-33.8634101534794,20.));
#89721=CARTESIAN_POINT('Ctrl Pts',(32.6007235441777,-33.8841326972008,0.));
#89722=CARTESIAN_POINT('Ctrl Pts',(32.6007235441777,-33.8841326972008,20.));
#89723=CARTESIAN_POINT('Ctrl Pts',(32.5748838441319,-33.9048364252556,0.));
#89724=CARTESIAN_POINT('Ctrl Pts',(32.5748838441319,-33.9048364252556,20.));
#89725=CARTESIAN_POINT('Ctrl Pts',(32.5490305017817,-33.9255213281434,0.));
#89726=CARTESIAN_POINT('Ctrl Pts',(32.5490305017817,-33.9255213281434,20.));
#89727=CARTESIAN_POINT('Ctrl Pts',(32.5231635303904,-33.9461873963724,0.));
#89728=CARTESIAN_POINT('Ctrl Pts',(32.5231635303904,-33.9461873963724,20.));
#89729=CARTESIAN_POINT('Ctrl Pts',(32.4972829432285,-33.9668346204605,0.));
#89730=CARTESIAN_POINT('Ctrl Pts',(32.4972829432285,-33.9668346204605,20.));
#89731=CARTESIAN_POINT('Ctrl Pts',(32.4713887535741,-33.987462990935,0.));
#89732=CARTESIAN_POINT('Ctrl Pts',(32.4713887535741,-33.987462990935,20.));
#89733=CARTESIAN_POINT('Ctrl Pts',(32.4454809747123,-34.0080724983324,0.));
#89734=CARTESIAN_POINT('Ctrl Pts',(32.4454809747123,-34.0080724983324,20.));
#89735=CARTESIAN_POINT('Ctrl Pts',(32.4195596199344,-34.0286631331978,0.));
#89736=CARTESIAN_POINT('Ctrl Pts',(32.4195596199344,-34.0286631331978,20.));
#89737=CARTESIAN_POINT('Ctrl Pts',(32.3936247025392,-34.0492348860855,0.));
#89738=CARTESIAN_POINT('Ctrl Pts',(32.3936247025392,-34.0492348860855,20.));
#89739=CARTESIAN_POINT('Ctrl Pts',(32.3676762358321,-34.0697877475586,0.));
#89740=CARTESIAN_POINT('Ctrl Pts',(32.3676762358321,-34.0697877475586,20.));
#89741=CARTESIAN_POINT('Ctrl Pts',(32.3417142331256,-34.0903217081898,0.));
#89742=CARTESIAN_POINT('Ctrl Pts',(32.3417142331256,-34.0903217081898,20.));
#89743=CARTESIAN_POINT('Ctrl Pts',(32.3157387077392,-34.1108367585604,0.));
#89744=CARTESIAN_POINT('Ctrl Pts',(32.3157387077392,-34.1108367585604,20.));
#89745=CARTESIAN_POINT('Ctrl Pts',(32.289749672999,-34.131332889261,0.));
#89746=CARTESIAN_POINT('Ctrl Pts',(32.289749672999,-34.131332889261,20.));
#89747=CARTESIAN_POINT('Ctrl Pts',(32.2637471422388,-34.1518100908915,0.));
#89748=CARTESIAN_POINT('Ctrl Pts',(32.2637471422388,-34.1518100908915,20.));
#89749=CARTESIAN_POINT('Ctrl Pts',(32.2377311287994,-34.1722683540613,0.));
#89750=CARTESIAN_POINT('Ctrl Pts',(32.2377311287994,-34.1722683540613,20.));
#89751=CARTESIAN_POINT('Ctrl Pts',(32.2117016460282,-34.1927076693884,0.));
#89752=CARTESIAN_POINT('Ctrl Pts',(32.2117016460282,-34.1927076693884,20.));
#89753=CARTESIAN_POINT('Ctrl Pts',(32.1856587072789,-34.2131280274994,0.));
#89754=CARTESIAN_POINT('Ctrl Pts',(32.1856587072789,-34.2131280274994,20.));
#89755=CARTESIAN_POINT('Ctrl Pts',(32.1596023259127,-34.233529419031,0.));
#89756=CARTESIAN_POINT('Ctrl Pts',(32.1596023259127,-34.233529419031,20.));
#89757=CARTESIAN_POINT('Ctrl Pts',(32.1335325152974,-34.2539118346284,0.));
#89758=CARTESIAN_POINT('Ctrl Pts',(32.1335325152974,-34.2539118346284,20.));
#89759=CARTESIAN_POINT('Ctrl Pts',(32.1074492888083,-34.2742752649465,0.));
#89760=CARTESIAN_POINT('Ctrl Pts',(32.1074492888083,-34.2742752649465,20.));
#89761=CARTESIAN_POINT('Ctrl Pts',(32.081352659827,-34.2946197006486,0.));
#89762=CARTESIAN_POINT('Ctrl Pts',(32.081352659827,-34.2946197006486,20.));
#89763=CARTESIAN_POINT('Ctrl Pts',(32.0552426417428,-34.3149451324082,0.));
#89764=CARTESIAN_POINT('Ctrl Pts',(32.0552426417428,-34.3149451324082,20.));
#89765=CARTESIAN_POINT('Ctrl Pts',(32.0291192479513,-34.335251550907,0.));
#89766=CARTESIAN_POINT('Ctrl Pts',(32.0291192479513,-34.335251550907,20.));
#89767=CARTESIAN_POINT('Ctrl Pts',(32.0029824918551,-34.3555389468366,0.));
#89768=CARTESIAN_POINT('Ctrl Pts',(32.0029824918551,-34.3555389468366,20.));
#89769=CARTESIAN_POINT('Ctrl Pts',(31.9768323868632,-34.3758073108972,0.));
#89770=CARTESIAN_POINT('Ctrl Pts',(31.9768323868632,-34.3758073108972,20.));
#89771=CARTESIAN_POINT('Ctrl Pts',(31.9506689463919,-34.3960566337983,0.));
#89772=CARTESIAN_POINT('Ctrl Pts',(31.9506689463919,-34.3960566337983,20.));
#89773=CARTESIAN_POINT('Ctrl Pts',(31.9244921838641,-34.4162869062584,0.));
#89774=CARTESIAN_POINT('Ctrl Pts',(31.9244921838641,-34.4162869062584,20.));
#89775=CARTESIAN_POINT('Ctrl Pts',(31.8983021127101,-34.4364981190057,0.));
#89776=CARTESIAN_POINT('Ctrl Pts',(31.8983021127101,-34.4364981190057,20.));
#89777=CARTESIAN_POINT('Ctrl Pts',(31.8720987463673,-34.4566902627777,0.));
#89778=CARTESIAN_POINT('Ctrl Pts',(31.8720987463673,-34.4566902627777,20.));
#89779=CARTESIAN_POINT('Ctrl Pts',(31.8458820982794,-34.4768633283209,0.));
#89780=CARTESIAN_POINT('Ctrl Pts',(31.8458820982794,-34.4768633283209,20.));
#89781=CARTESIAN_POINT('Ctrl Pts',(31.819652181897,-34.4970173063908,0.));
#89782=CARTESIAN_POINT('Ctrl Pts',(31.819652181897,-34.4970173063908,20.));
#89783=CARTESIAN_POINT('Ctrl Pts',(31.7934090106771,-34.5171521877519,0.));
#89784=CARTESIAN_POINT('Ctrl Pts',(31.7934090106771,-34.5171521877519,20.));
#89785=CARTESIAN_POINT('Ctrl Pts',(31.7671525980837,-34.5372679631778,0.));
#89786=CARTESIAN_POINT('Ctrl Pts',(31.7671525980837,-34.5372679631778,20.));
#89787=CARTESIAN_POINT('Ctrl Pts',(31.7408829575878,-34.5573646234518,0.));
#89788=CARTESIAN_POINT('Ctrl Pts',(31.7408829575878,-34.5573646234518,20.));
#89789=CARTESIAN_POINT('Ctrl Pts',(31.7146001026678,-34.5774421593669,0.));
#89790=CARTESIAN_POINT('Ctrl Pts',(31.7146001026678,-34.5774421593669,20.));
#89791=CARTESIAN_POINT('Ctrl Pts',(31.6883040468088,-34.5975005617252,0.));
#89792=CARTESIAN_POINT('Ctrl Pts',(31.6883040468088,-34.5975005617252,20.));
#89793=CARTESIAN_POINT('Ctrl Pts',(31.6619948035026,-34.6175398213376,0.));
#89794=CARTESIAN_POINT('Ctrl Pts',(31.6619948035026,-34.6175398213376,20.));
#89795=CARTESIAN_POINT('Ctrl Pts',(31.6356723862475,-34.6375599290243,0.));
#89796=CARTESIAN_POINT('Ctrl Pts',(31.6356723862475,-34.6375599290243,20.));
#89797=CARTESIAN_POINT('Ctrl Pts',(31.609336808548,-34.6575608756141,0.));
#89798=CARTESIAN_POINT('Ctrl Pts',(31.609336808548,-34.6575608756141,20.));
#89799=CARTESIAN_POINT('Ctrl Pts',(31.5829880839157,-34.6775426519456,0.));
#89800=CARTESIAN_POINT('Ctrl Pts',(31.5829880839157,-34.6775426519456,20.));
#89801=CARTESIAN_POINT('Ctrl Pts',(31.556626225869,-34.6975052488666,0.));
#89802=CARTESIAN_POINT('Ctrl Pts',(31.556626225869,-34.6975052488666,20.));
#89803=CARTESIAN_POINT('Ctrl Pts',(31.5302512479332,-34.7174486572342,0.));
#89804=CARTESIAN_POINT('Ctrl Pts',(31.5302512479332,-34.7174486572342,20.));
#89805=CARTESIAN_POINT('Ctrl Pts',(31.5038631636409,-34.7373728679152,0.));
#89806=CARTESIAN_POINT('Ctrl Pts',(31.5038631636409,-34.7373728679152,20.));
#89807=CARTESIAN_POINT('Ctrl Pts',(31.4774619865312,-34.7572778717853,0.));
#89808=CARTESIAN_POINT('Ctrl Pts',(31.4774619865312,-34.7572778717853,20.));
#89809=CARTESIAN_POINT('Ctrl Pts',(31.4510477301503,-34.7771636597296,0.));
#89810=CARTESIAN_POINT('Ctrl Pts',(31.4510477301503,-34.7771636597296,20.));
#89811=CARTESIAN_POINT('Ctrl Pts',(31.4246204080513,-34.7970302226433,0.));
#89812=CARTESIAN_POINT('Ctrl Pts',(31.4246204080513,-34.7970302226433,20.));
#89813=CARTESIAN_POINT('Ctrl Pts',(31.3981800337935,-34.8168775514299,0.));
#89814=CARTESIAN_POINT('Ctrl Pts',(31.3981800337935,-34.8168775514299,20.));
#89815=CARTESIAN_POINT('Ctrl Pts',(31.3717266209433,-34.8367056370027,0.));
#89816=CARTESIAN_POINT('Ctrl Pts',(31.3717266209433,-34.8367056370027,20.));
#89817=CARTESIAN_POINT('Ctrl Pts',(31.3452601830725,-34.856514470283,0.));
#89818=CARTESIAN_POINT('Ctrl Pts',(31.3452601830725,-34.856514470283,20.));
#89819=CARTESIAN_POINT('Ctrl Pts',(31.3187807337598,-34.8763040422018,0.));
#89820=CARTESIAN_POINT('Ctrl Pts',(31.3187807337598,-34.8763040422018,20.));
#89821=CARTESIAN_POINT('Ctrl Pts',(31.2922882865907,-34.8960743436995,0.));
#89822=CARTESIAN_POINT('Ctrl Pts',(31.2922882865907,-34.8960743436995,20.));
#89823=CARTESIAN_POINT('Ctrl Pts',(31.2657828551579,-34.9158253657263,0.));
#89824=CARTESIAN_POINT('Ctrl Pts',(31.2657828551579,-34.9158253657263,20.));
#89825=CARTESIAN_POINT('Ctrl Pts',(31.2392644530613,-34.9355570992414,0.));
#89826=CARTESIAN_POINT('Ctrl Pts',(31.2392644530613,-34.9355570992414,20.));
#89827=CARTESIAN_POINT('Ctrl Pts',(31.2127330939085,-34.9552695352152,0.));
#89828=CARTESIAN_POINT('Ctrl Pts',(31.2127330939085,-34.9552695352152,20.));
#89829=CARTESIAN_POINT('Ctrl Pts',(31.1861887913133,-34.974962664626,0.));
#89830=CARTESIAN_POINT('Ctrl Pts',(31.1861887913133,-34.974962664626,20.));
#89831=CARTESIAN_POINT('Ctrl Pts',(31.1596315588953,-34.9946364784612,0.));
#89832=CARTESIAN_POINT('Ctrl Pts',(31.1596315588953,-34.9946364784612,20.));
#89833=CARTESIAN_POINT('Ctrl Pts',(31.1330614102809,-35.0142909677175,0.));
#89834=CARTESIAN_POINT('Ctrl Pts',(31.1330614102809,-35.0142909677175,20.));
#89835=CARTESIAN_POINT('Ctrl Pts',(31.1064783591027,-35.0339261234013,0.));
#89836=CARTESIAN_POINT('Ctrl Pts',(31.1064783591027,-35.0339261234013,20.));
#89837=CARTESIAN_POINT('Ctrl Pts',(31.0798824190003,-35.0535419365277,0.));
#89838=CARTESIAN_POINT('Ctrl Pts',(31.0798824190003,-35.0535419365277,20.));
#89839=CARTESIAN_POINT('Ctrl Pts',(31.0532736036193,-35.0731383981212,0.));
#89840=CARTESIAN_POINT('Ctrl Pts',(31.0532736036193,-35.0731383981212,20.));
#89841=CARTESIAN_POINT('Ctrl Pts',(31.026651926612,-35.0927154992152,0.));
#89842=CARTESIAN_POINT('Ctrl Pts',(31.026651926612,-35.0927154992152,20.));
#89843=CARTESIAN_POINT('Ctrl Pts',(31.0000174016378,-35.1122732308527,0.));
#89844=CARTESIAN_POINT('Ctrl Pts',(31.0000174016378,-35.1122732308527,20.));
#89845=CARTESIAN_POINT('Ctrl Pts',(30.9733700423633,-35.131811584087,0.));
#89846=CARTESIAN_POINT('Ctrl Pts',(30.9733700423633,-35.131811584087,20.));
#89847=CARTESIAN_POINT('Ctrl Pts',(30.9467098624624,-35.1513305499814,0.));
#89848=CARTESIAN_POINT('Ctrl Pts',(30.9467098624624,-35.1513305499814,20.));
#89849=CARTESIAN_POINT('Ctrl Pts',(30.9200368756162,-35.170830119609,0.));
#89850=CARTESIAN_POINT('Ctrl Pts',(30.9200368756162,-35.170830119609,20.));
#89851=CARTESIAN_POINT('Ctrl Pts',(30.8933510955115,-35.1903102840519,0.));
#89852=CARTESIAN_POINT('Ctrl Pts',(30.8933510955115,-35.1903102840519,20.));
#89853=CARTESIAN_POINT('Ctrl Pts',(30.8666525358408,-35.2097710343998,0.));
#89854=CARTESIAN_POINT('Ctrl Pts',(30.8666525358408,-35.2097710343998,20.));
#89855=CARTESIAN_POINT('Ctrl Pts',(30.8399412103026,-35.2292123617517,0.));
#89856=CARTESIAN_POINT('Ctrl Pts',(30.8399412103026,-35.2292123617517,20.));
#89857=CARTESIAN_POINT('Ctrl Pts',(30.8132171326021,-35.2486342572162,0.));
#89858=CARTESIAN_POINT('Ctrl Pts',(30.8132171326021,-35.2486342572162,20.));
#89859=CARTESIAN_POINT('Ctrl Pts',(30.786480316451,-35.2680367119112,0.));
#89860=CARTESIAN_POINT('Ctrl Pts',(30.786480316451,-35.2680367119112,20.));
#89861=CARTESIAN_POINT('Ctrl Pts',(30.7597307755696,-35.2874197169657,0.));
#89862=CARTESIAN_POINT('Ctrl Pts',(30.7597307755696,-35.2874197169657,20.));
#89863=CARTESIAN_POINT('Ctrl Pts',(30.732968523684,-35.3067832635177,0.));
#89864=CARTESIAN_POINT('Ctrl Pts',(30.732968523684,-35.3067832635177,20.));
#89865=CARTESIAN_POINT('Ctrl Pts',(30.7061935745273,-35.3261273427148,0.));
#89866=CARTESIAN_POINT('Ctrl Pts',(30.7061935745273,-35.3261273427148,20.));
#89867=CARTESIAN_POINT('Ctrl Pts',(30.6794059418388,-35.3454519457137,0.));
#89868=CARTESIAN_POINT('Ctrl Pts',(30.6794059418388,-35.3454519457137,20.));
#89869=CARTESIAN_POINT('Ctrl Pts',(30.6526056393638,-35.3647570636798,0.));
#89870=CARTESIAN_POINT('Ctrl Pts',(30.6526056393638,-35.3647570636798,20.));
#89871=CARTESIAN_POINT('Ctrl Pts',(30.6257926808541,-35.3840426877879,0.));
#89872=CARTESIAN_POINT('Ctrl Pts',(30.6257926808541,-35.3840426877879,20.));
#89873=CARTESIAN_POINT('Ctrl Pts',(30.5989670800681,-35.4033088092226,0.));
#89874=CARTESIAN_POINT('Ctrl Pts',(30.5989670800681,-35.4033088092226,20.));
#89875=CARTESIAN_POINT('Ctrl Pts',(30.5721288507715,-35.4225554191786,0.));
#89876=CARTESIAN_POINT('Ctrl Pts',(30.5721288507715,-35.4225554191786,20.));
#89877=CARTESIAN_POINT('Ctrl Pts',(30.5452780067368,-35.4417825088605,0.));
#89878=CARTESIAN_POINT('Ctrl Pts',(30.5452780067368,-35.4417825088605,20.));
#89879=CARTESIAN_POINT('Ctrl Pts',(30.5184145617424,-35.4609900694812,0.));
#89880=CARTESIAN_POINT('Ctrl Pts',(30.5184145617424,-35.4609900694812,20.));
#89881=CARTESIAN_POINT('Ctrl Pts',(30.4915385295724,-35.4801780922626,0.));
#89882=CARTESIAN_POINT('Ctrl Pts',(30.4915385295724,-35.4801780922626,20.));
#89883=CARTESIAN_POINT('Ctrl Pts',(30.4646499240177,-35.4993465684362,0.));
#89884=CARTESIAN_POINT('Ctrl Pts',(30.4646499240177,-35.4993465684362,20.));
#89885=CARTESIAN_POINT('Ctrl Pts',(30.437748758876,-35.518495489243,0.));
#89886=CARTESIAN_POINT('Ctrl Pts',(30.437748758876,-35.518495489243,20.));
#89887=CARTESIAN_POINT('Ctrl Pts',(30.4108350479521,-35.5376248459348,0.));
#89888=CARTESIAN_POINT('Ctrl Pts',(30.4108350479521,-35.5376248459348,20.));
#89889=CARTESIAN_POINT('Ctrl Pts',(30.3839088050584,-35.5567346297737,0.));
#89890=CARTESIAN_POINT('Ctrl Pts',(30.3839088050584,-35.5567346297737,20.));
#89891=CARTESIAN_POINT('Ctrl Pts',(30.3569700440131,-35.5758248320301,0.));
#89892=CARTESIAN_POINT('Ctrl Pts',(30.3569700440131,-35.5758248320301,20.));
#89893=CARTESIAN_POINT('Ctrl Pts',(30.3300187786403,-35.5948954439837,0.));
#89894=CARTESIAN_POINT('Ctrl Pts',(30.3300187786403,-35.5948954439837,20.));
#89895=CARTESIAN_POINT('Ctrl Pts',(30.3030550227693,-35.6139464569223,0.));
#89896=CARTESIAN_POINT('Ctrl Pts',(30.3030550227693,-35.6139464569223,20.));
#89897=CARTESIAN_POINT('Ctrl Pts',(30.2760787902362,-35.6329778621436,0.));
#89898=CARTESIAN_POINT('Ctrl Pts',(30.2760787902362,-35.6329778621436,20.));
#89899=CARTESIAN_POINT('Ctrl Pts',(30.2490900948838,-35.6519896509552,0.));
#89900=CARTESIAN_POINT('Ctrl Pts',(30.2490900948838,-35.6519896509552,20.));
#89901=CARTESIAN_POINT('Ctrl Pts',(30.2220889505625,-35.6709818146751,0.));
#89902=CARTESIAN_POINT('Ctrl Pts',(30.2220889505625,-35.6709818146751,20.));
#89903=CARTESIAN_POINT('Ctrl Pts',(30.1950753711288,-35.6899543446309,0.));
#89904=CARTESIAN_POINT('Ctrl Pts',(30.1950753711288,-35.6899543446309,20.));
#89905=CARTESIAN_POINT('Ctrl Pts',(30.1680493704465,-35.7089072321597,0.));
#89906=CARTESIAN_POINT('Ctrl Pts',(30.1680493704465,-35.7089072321597,20.));
#89907=CARTESIAN_POINT('Ctrl Pts',(30.141010962385,-35.727840468608,0.));
#89908=CARTESIAN_POINT('Ctrl Pts',(30.141010962385,-35.727840468608,20.));
#89909=CARTESIAN_POINT('Ctrl Pts',(30.1139601608197,-35.7467540453308,0.));
#89910=CARTESIAN_POINT('Ctrl Pts',(30.1139601608197,-35.7467540453308,20.));
#89911=CARTESIAN_POINT('Ctrl Pts',(30.0868969796328,-35.7656479536939,0.));
#89912=CARTESIAN_POINT('Ctrl Pts',(30.0868969796328,-35.7656479536939,20.));
#89913=CARTESIAN_POINT('Ctrl Pts',(30.0598214327127,-35.7845221850715,0.));
#89914=CARTESIAN_POINT('Ctrl Pts',(30.0598214327127,-35.7845221850715,20.));
#89915=CARTESIAN_POINT('Ctrl Pts',(30.0327335339539,-35.8033767308478,0.));
#89916=CARTESIAN_POINT('Ctrl Pts',(30.0327335339539,-35.8033767308478,20.));
#89917=CARTESIAN_POINT('Ctrl Pts',(30.005633297258,-35.8222115824167,0.));
#89918=CARTESIAN_POINT('Ctrl Pts',(30.005633297258,-35.8222115824167,20.));
#89919=CARTESIAN_POINT('Ctrl Pts',(29.9785207365333,-35.841026731182,0.));
#89920=CARTESIAN_POINT('Ctrl Pts',(29.9785207365333,-35.841026731182,20.));
#89921=CARTESIAN_POINT('Ctrl Pts',(29.9513958656946,-35.8598221685576,0.));
#89922=CARTESIAN_POINT('Ctrl Pts',(29.9513958656946,-35.8598221685576,20.));
#89923=CARTESIAN_POINT('Ctrl Pts',(29.9242586986624,-35.8785978859658,0.));
#89924=CARTESIAN_POINT('Ctrl Pts',(29.9242586986624,-35.8785978859658,20.));
#89925=CARTESIAN_POINT('Ctrl Pts',(29.8971092493634,-35.8973538748387,0.));
#89926=CARTESIAN_POINT('Ctrl Pts',(29.8971092493634,-35.8973538748387,20.));
#89927=CARTESIAN_POINT('Ctrl Pts',(29.869947531731,-35.9160901266177,0.));
#89928=CARTESIAN_POINT('Ctrl Pts',(29.869947531731,-35.9160901266177,20.));
#89929=CARTESIAN_POINT('Ctrl Pts',(29.8427735597048,-35.934806632754,0.));
#89930=CARTESIAN_POINT('Ctrl Pts',(29.8427735597048,-35.934806632754,20.));
#89931=CARTESIAN_POINT('Ctrl Pts',(29.8155873472308,-35.9535033847082,0.));
#89932=CARTESIAN_POINT('Ctrl Pts',(29.8155873472308,-35.9535033847082,20.));
#89933=CARTESIAN_POINT('Ctrl Pts',(29.7883889082614,-35.9721803739509,0.));
#89934=CARTESIAN_POINT('Ctrl Pts',(29.7883889082614,-35.9721803739509,20.));
#89935=CARTESIAN_POINT('Ctrl Pts',(29.7611782567557,-35.9908375919623,0.));
#89936=CARTESIAN_POINT('Ctrl Pts',(29.7611782567557,-35.9908375919623,20.));
#89937=CARTESIAN_POINT('Ctrl Pts',(29.7339554066796,-36.0094750302331,0.));
#89938=CARTESIAN_POINT('Ctrl Pts',(29.7339554066796,-36.0094750302331,20.));
#89939=CARTESIAN_POINT('Ctrl Pts',(29.7067203720053,-36.0280926802632,0.));
#89940=CARTESIAN_POINT('Ctrl Pts',(29.7067203720053,-36.0280926802632,20.));
#89941=CARTESIAN_POINT('Ctrl Pts',(29.6794731667106,-36.0466905335617,0.));
#89942=CARTESIAN_POINT('Ctrl Pts',(29.6794731667106,-36.0466905335617,20.));
#89943=CARTESIAN_POINT('Ctrl Pts',(29.6522138047793,-36.0652685816464,0.));
#89944=CARTESIAN_POINT('Ctrl Pts',(29.6522138047793,-36.0652685816464,20.));
#89945=CARTESIAN_POINT('Ctrl Pts',(29.6249423002017,-36.0838268160451,0.));
#89946=CARTESIAN_POINT('Ctrl Pts',(29.6249423002017,-36.0838268160451,20.));
#89947=CARTESIAN_POINT('Ctrl Pts',(29.5976586669748,-36.1023652282957,0.));
#89948=CARTESIAN_POINT('Ctrl Pts',(29.5976586669748,-36.1023652282957,20.));
#89949=CARTESIAN_POINT('Ctrl Pts',(29.5703629191022,-36.1208838099461,0.));
#89950=CARTESIAN_POINT('Ctrl Pts',(29.5703629191022,-36.1208838099461,20.));
#89951=CARTESIAN_POINT('Ctrl Pts',(29.5430550705937,-36.1393825525541,0.));
#89952=CARTESIAN_POINT('Ctrl Pts',(29.5430550705937,-36.1393825525541,20.));
#89953=CARTESIAN_POINT('Ctrl Pts',(29.5157351354651,-36.1578614476865,0.));
#89954=CARTESIAN_POINT('Ctrl Pts',(29.5157351354651,-36.1578614476865,20.));
#89955=CARTESIAN_POINT('Ctrl Pts',(29.4884031277381,-36.1763204869193,0.));
#89956=CARTESIAN_POINT('Ctrl Pts',(29.4884031277381,-36.1763204869193,20.));
#89957=CARTESIAN_POINT('Ctrl Pts',(29.4610590614411,-36.1947596618382,0.));
#89958=CARTESIAN_POINT('Ctrl Pts',(29.4610590614411,-36.1947596618382,20.));
#89959=CARTESIAN_POINT('Ctrl Pts',(29.4337029506094,-36.2131789640397,0.));
#89960=CARTESIAN_POINT('Ctrl Pts',(29.4337029506094,-36.2131789640397,20.));
#89961=CARTESIAN_POINT('Ctrl Pts',(29.4063348092849,-36.2315783851295,0.));
#89962=CARTESIAN_POINT('Ctrl Pts',(29.4063348092849,-36.2315783851295,20.));
#89963=CARTESIAN_POINT('Ctrl Pts',(29.3789546515147,-36.2499579167227,0.));
#89964=CARTESIAN_POINT('Ctrl Pts',(29.3789546515147,-36.2499579167227,20.));
#89965=CARTESIAN_POINT('Ctrl Pts',(29.3515624913523,-36.2683175504441,0.));
#89966=CARTESIAN_POINT('Ctrl Pts',(29.3515624913523,-36.2683175504441,20.));
#89967=CARTESIAN_POINT('Ctrl Pts',(29.3241583428569,-36.286657277928,0.));
#89968=CARTESIAN_POINT('Ctrl Pts',(29.3241583428569,-36.286657277928,20.));
#89969=CARTESIAN_POINT('Ctrl Pts',(29.2967422200943,-36.3049770908188,0.));
#89970=CARTESIAN_POINT('Ctrl Pts',(29.2967422200943,-36.3049770908188,20.));
#89971=CARTESIAN_POINT('Ctrl Pts',(29.2693141371364,-36.3232769807701,0.));
#89972=CARTESIAN_POINT('Ctrl Pts',(29.2693141371364,-36.3232769807701,20.));
#89973=CARTESIAN_POINT('Ctrl Pts',(29.241874108062,-36.3415569394456,0.));
#89974=CARTESIAN_POINT('Ctrl Pts',(29.241874108062,-36.3415569394456,20.));
#89975=CARTESIAN_POINT('Ctrl Pts',(29.2144221469562,-36.3598169585187,0.));
#89976=CARTESIAN_POINT('Ctrl Pts',(29.2144221469562,-36.3598169585187,20.));
#89977=CARTESIAN_POINT('Ctrl Pts',(29.186958267911,-36.3780570296726,0.));
#89978=CARTESIAN_POINT('Ctrl Pts',(29.186958267911,-36.3780570296726,20.));
#89979=CARTESIAN_POINT('Ctrl Pts',(29.1594824850239,-36.3962771446002,0.));
#89980=CARTESIAN_POINT('Ctrl Pts',(29.1594824850239,-36.3962771446002,20.));
#89981=CARTESIAN_POINT('Ctrl Pts',(29.1319948123985,-36.4144772950043,0.));
#89982=CARTESIAN_POINT('Ctrl Pts',(29.1319948123985,-36.4144772950043,20.));
#89983=CARTESIAN_POINT('Ctrl Pts',(29.1044952641442,-36.4326574725969,0.));
#89984=CARTESIAN_POINT('Ctrl Pts',(29.1044952641442,-36.4326574725969,20.));
#89985=CARTESIAN_POINT('Ctrl Pts',(29.0769838543763,-36.4508176690994,0.));
#89986=CARTESIAN_POINT('Ctrl Pts',(29.0769838543763,-36.4508176690994,20.));
#89987=CARTESIAN_POINT('Ctrl Pts',(29.0494605972165,-36.4689578762435,0.));
#89988=CARTESIAN_POINT('Ctrl Pts',(29.0494605972165,-36.4689578762435,20.));
#89989=CARTESIAN_POINT('Ctrl Pts',(29.0219255067927,-36.4870780857703,0.));
#89990=CARTESIAN_POINT('Ctrl Pts',(29.0219255067927,-36.4870780857703,20.));
#89991=CARTESIAN_POINT('Ctrl Pts',(28.99437859724,-36.5051782894317,0.));
#89992=CARTESIAN_POINT('Ctrl Pts',(28.99437859724,-36.5051782894317,20.));
#89993=CARTESIAN_POINT('Ctrl Pts',(28.9668198826995,-36.5232584789886,0.));
#89994=CARTESIAN_POINT('Ctrl Pts',(28.9668198826995,-36.5232584789886,20.));
#89995=CARTESIAN_POINT('Ctrl Pts',(28.9392493773185,-36.5413186462123,0.));
#89996=CARTESIAN_POINT('Ctrl Pts',(28.9392493773185,-36.5413186462123,20.));
#89997=CARTESIAN_POINT('Ctrl Pts',(28.9116670952497,-36.5593587828826,0.));
#89998=CARTESIAN_POINT('Ctrl Pts',(28.9116670952497,-36.5593587828826,20.));
#89999=CARTESIAN_POINT('Ctrl Pts',(28.8840730506515,-36.577378880789,0.));
#90000=CARTESIAN_POINT('Ctrl Pts',(28.8840730506515,-36.577378880789,20.));
#90001=CARTESIAN_POINT('Ctrl Pts',(28.8564672576885,-36.5953789317306,0.));
#90002=CARTESIAN_POINT('Ctrl Pts',(28.8564672576885,-36.5953789317306,20.));
#90003=CARTESIAN_POINT('Ctrl Pts',(28.8288497305324,-36.6133589275174,0.));
#90004=CARTESIAN_POINT('Ctrl Pts',(28.8288497305324,-36.6133589275174,20.));
#90005=CARTESIAN_POINT('Ctrl Pts',(28.8012204833609,-36.6313188599694,0.));
#90006=CARTESIAN_POINT('Ctrl Pts',(28.8012204833609,-36.6313188599694,20.));
#90007=CARTESIAN_POINT('Ctrl Pts',(28.7735795303585,-36.6492587209168,0.));
#90008=CARTESIAN_POINT('Ctrl Pts',(28.7735795303585,-36.6492587209168,20.));
#90009=CARTESIAN_POINT('Ctrl Pts',(28.7459268857152,-36.6671785021988,0.));
#90010=CARTESIAN_POINT('Ctrl Pts',(28.7459268857152,-36.6671785021988,20.));
#90011=CARTESIAN_POINT('Ctrl Pts',(28.7182625636274,-36.6850781956649,0.));
#90012=CARTESIAN_POINT('Ctrl Pts',(28.7182625636274,-36.6850781956649,20.));
#90013=CARTESIAN_POINT('Ctrl Pts',(28.6905865782966,-36.7029577931733,0.));
#90014=CARTESIAN_POINT('Ctrl Pts',(28.6905865782966,-36.7029577931733,20.));
#90015=CARTESIAN_POINT('Ctrl Pts',(28.6628989439305,-36.7208172865919,0.));
#90016=CARTESIAN_POINT('Ctrl Pts',(28.6628989439305,-36.7208172865919,20.));
#90017=CARTESIAN_POINT('Ctrl Pts',(28.6351996747428,-36.7386566677981,0.));
#90018=CARTESIAN_POINT('Ctrl Pts',(28.6351996747428,-36.7386566677981,20.));
#90019=CARTESIAN_POINT('Ctrl Pts',(28.6074887849535,-36.7564759286795,0.));
#90020=CARTESIAN_POINT('Ctrl Pts',(28.6074887849535,-36.7564759286795,20.));
#90021=CARTESIAN_POINT('Ctrl Pts',(28.5797662887891,-36.774275061134,0.));
#90022=CARTESIAN_POINT('Ctrl Pts',(28.5797662887891,-36.774275061134,20.));
#90023=CARTESIAN_POINT('Ctrl Pts',(28.5520322004824,-36.7920540570698,0.));
#90024=CARTESIAN_POINT('Ctrl Pts',(28.5520322004824,-36.7920540570698,20.));
#90025=CARTESIAN_POINT('Ctrl Pts',(28.5242865342724,-36.8098129084051,0.));
#90026=CARTESIAN_POINT('Ctrl Pts',(28.5242865342724,-36.8098129084051,20.));
#90027=CARTESIAN_POINT('Ctrl Pts',(28.496529304404,-36.8275516070676,0.));
#90028=CARTESIAN_POINT('Ctrl Pts',(28.496529304404,-36.8275516070676,20.));
#90029=CARTESIAN_POINT('Ctrl Pts',(28.4687605251277,-36.8452701449948,0.));
#90030=CARTESIAN_POINT('Ctrl Pts',(28.4687605251277,-36.8452701449948,20.));
#90031=CARTESIAN_POINT('Ctrl Pts',(28.4409802107002,-36.8629685141338,0.));
#90032=CARTESIAN_POINT('Ctrl Pts',(28.4409802107002,-36.8629685141338,20.));
#90033=CARTESIAN_POINT('Ctrl Pts',(28.413188375384,-36.8806467064409,0.));
#90034=CARTESIAN_POINT('Ctrl Pts',(28.413188375384,-36.8806467064409,20.));
#90035=CARTESIAN_POINT('Ctrl Pts',(28.3853850334475,-36.8983047138822,0.));
#90036=CARTESIAN_POINT('Ctrl Pts',(28.3853850334475,-36.8983047138822,20.));
#90037=CARTESIAN_POINT('Ctrl Pts',(28.3575701991656,-36.9159425284342,0.));
#90038=CARTESIAN_POINT('Ctrl Pts',(28.3575701991656,-36.9159425284342,20.));
#90039=CARTESIAN_POINT('Ctrl Pts',(28.3297438868192,-36.9335601420835,0.));
#90040=CARTESIAN_POINT('Ctrl Pts',(28.3297438868192,-36.9335601420835,20.));
#90041=CARTESIAN_POINT('Ctrl Pts',(28.3019061106957,-36.9511575468269,0.));
#90042=CARTESIAN_POINT('Ctrl Pts',(28.3019061106957,-36.9511575468269,20.));
#90043=CARTESIAN_POINT('Ctrl Pts',(28.2740568850881,-36.968734734671,0.));
#90044=CARTESIAN_POINT('Ctrl Pts',(28.2740568850881,-36.968734734671,20.));
#90045=CARTESIAN_POINT('Ctrl Pts',(28.2461962242955,-36.9862916976318,0.));
#90046=CARTESIAN_POINT('Ctrl Pts',(28.2461962242955,-36.9862916976318,20.));
#90047=CARTESIAN_POINT('Ctrl Pts',(28.2183241426219,-37.0038284277349,0.));
#90048=CARTESIAN_POINT('Ctrl Pts',(28.2183241426219,-37.0038284277349,20.));
#90049=CARTESIAN_POINT('Ctrl Pts',(28.1904406543778,-37.0213449170157,0.));
#90050=CARTESIAN_POINT('Ctrl Pts',(28.1904406543778,-37.0213449170157,20.));
#90051=CARTESIAN_POINT('Ctrl Pts',(28.1625457738797,-37.0388411575197,0.));
#90052=CARTESIAN_POINT('Ctrl Pts',(28.1625457738797,-37.0388411575197,20.));
#90053=CARTESIAN_POINT('Ctrl Pts',(28.1346395154506,-37.0563171413026,0.));
#90054=CARTESIAN_POINT('Ctrl Pts',(28.1346395154506,-37.0563171413026,20.));
#90055=CARTESIAN_POINT('Ctrl Pts',(28.1067218934195,-37.0737728604298,0.));
#90056=CARTESIAN_POINT('Ctrl Pts',(28.1067218934195,-37.0737728604298,20.));
#90057=CARTESIAN_POINT('Ctrl Pts',(28.0787929221219,-37.0912083069772,0.));
#90058=CARTESIAN_POINT('Ctrl Pts',(28.0787929221219,-37.0912083069772,20.));
#90059=CARTESIAN_POINT('Ctrl Pts',(28.0508526158994,-37.1086234730312,0.));
#90060=CARTESIAN_POINT('Ctrl Pts',(28.0508526158994,-37.1086234730312,20.));
#90061=CARTESIAN_POINT('Ctrl Pts',(28.0229009890985,-37.1260183506872,0.));
#90062=CARTESIAN_POINT('Ctrl Pts',(28.0229009890985,-37.1260183506872,20.));
#90063=CARTESIAN_POINT('Ctrl Pts',(27.994938056072,-37.1433929320507,0.));
#90064=CARTESIAN_POINT('Ctrl Pts',(27.994938056072,-37.1433929320507,20.));
#90065=CARTESIAN_POINT('Ctrl Pts',(27.9669638311771,-37.1607472092352,0.));
#90066=CARTESIAN_POINT('Ctrl Pts',(27.9669638311771,-37.1607472092352,20.));
#90067=CARTESIAN_POINT('Ctrl Pts',(27.9389783287777,-37.1780811743652,0.));
#90068=CARTESIAN_POINT('Ctrl Pts',(27.9389783287777,-37.1780811743652,20.));
#90069=CARTESIAN_POINT('Ctrl Pts',(27.9109815632437,-37.1953948195748,0.));
#90070=CARTESIAN_POINT('Ctrl Pts',(27.9109815632437,-37.1953948195748,20.));
#90071=CARTESIAN_POINT('Ctrl Pts',(27.8829735489517,-37.2126881370093,0.));
#90072=CARTESIAN_POINT('Ctrl Pts',(27.8829735489517,-37.2126881370093,20.));
#90073=CARTESIAN_POINT('Ctrl Pts',(27.8549543002843,-37.2299611188238,0.));
#90074=CARTESIAN_POINT('Ctrl Pts',(27.8549543002843,-37.2299611188238,20.));
#90075=CARTESIAN_POINT('Ctrl Pts',(27.8269238316305,-37.2472137571842,0.));
#90076=CARTESIAN_POINT('Ctrl Pts',(27.8269238316305,-37.2472137571842,20.));
#90077=CARTESIAN_POINT('Ctrl Pts',(27.7988821573846,-37.2644460442654,0.));
#90078=CARTESIAN_POINT('Ctrl Pts',(27.7988821573846,-37.2644460442654,20.));
#90079=CARTESIAN_POINT('Ctrl Pts',(27.7708292919468,-37.2816579722525,0.));
#90080=CARTESIAN_POINT('Ctrl Pts',(27.7708292919468,-37.2816579722525,20.));
#90081=CARTESIAN_POINT('Ctrl Pts',(27.7427652497224,-37.2988495333397,0.));
#90082=CARTESIAN_POINT('Ctrl Pts',(27.7427652497224,-37.2988495333397,20.));
#90083=CARTESIAN_POINT('Ctrl Pts',(27.7146900451228,-37.3160207197314,0.));
#90084=CARTESIAN_POINT('Ctrl Pts',(27.7146900451228,-37.3160207197314,20.));
#90085=CARTESIAN_POINT('Ctrl Pts',(27.6866036925651,-37.3331715236414,0.));
#90086=CARTESIAN_POINT('Ctrl Pts',(27.6866036925651,-37.3331715236414,20.));
#90087=CARTESIAN_POINT('Ctrl Pts',(27.6585062064726,-37.3503019372939,0.));
#90088=CARTESIAN_POINT('Ctrl Pts',(27.6585062064726,-37.3503019372939,20.));
#90089=CARTESIAN_POINT('Ctrl Pts',(27.6303976012744,-37.3674119529234,0.));
#90090=CARTESIAN_POINT('Ctrl Pts',(27.6303976012744,-37.3674119529234,20.));
#90091=CARTESIAN_POINT('Ctrl Pts',(27.6022778914064,-37.384501562775,0.));
#90092=CARTESIAN_POINT('Ctrl Pts',(27.6022778914064,-37.384501562775,20.));
#90093=CARTESIAN_POINT('Ctrl Pts',(27.5741470913094,-37.4015707591036,0.));
#90094=CARTESIAN_POINT('Ctrl Pts',(27.5741470913094,-37.4015707591036,20.));
#90095=CARTESIAN_POINT('Ctrl Pts',(27.5460052154308,-37.4186195341741,0.));
#90096=CARTESIAN_POINT('Ctrl Pts',(27.5460052154308,-37.4186195341741,20.));
#90097=CARTESIAN_POINT('Ctrl Pts',(27.5178522782226,-37.4356478802604,0.));
#90098=CARTESIAN_POINT('Ctrl Pts',(27.5178522782226,-37.4356478802604,20.));
#90099=CARTESIAN_POINT('Ctrl Pts',(27.4896882941429,-37.4526557896465,0.));
#90100=CARTESIAN_POINT('Ctrl Pts',(27.4896882941429,-37.4526557896465,20.));
#90101=CARTESIAN_POINT('Ctrl Pts',(27.4615132776558,-37.4696432546267,0.));
#90102=CARTESIAN_POINT('Ctrl Pts',(27.4615132776558,-37.4696432546267,20.));
#90103=CARTESIAN_POINT('Ctrl Pts',(27.4333272432311,-37.4866102675048,0.));
#90104=CARTESIAN_POINT('Ctrl Pts',(27.4333272432311,-37.4866102675048,20.));
#90105=CARTESIAN_POINT('Ctrl Pts',(27.4051302053449,-37.5035568205959,0.));
#90106=CARTESIAN_POINT('Ctrl Pts',(27.4051302053449,-37.5035568205959,20.));
#90107=CARTESIAN_POINT('Ctrl Pts',(27.3769221784798,-37.5204829062256,0.));
#90108=CARTESIAN_POINT('Ctrl Pts',(27.3769221784798,-37.5204829062256,20.));
#90109=CARTESIAN_POINT('Ctrl Pts',(27.3487031771241,-37.5373885167297,0.));
#90110=CARTESIAN_POINT('Ctrl Pts',(27.3487031771241,-37.5373885167297,20.));
#90111=CARTESIAN_POINT('Ctrl Pts',(27.3204732157704,-37.5542736444521,0.));
#90112=CARTESIAN_POINT('Ctrl Pts',(27.3204732157704,-37.5542736444521,20.));
#90113=CARTESIAN_POINT('Ctrl Pts',(27.2922323089174,-37.571138281747,0.));
#90114=CARTESIAN_POINT('Ctrl Pts',(27.2922323089174,-37.571138281747,20.));
#90115=CARTESIAN_POINT('Ctrl Pts',(27.2639804710687,-37.5879824209777,0.));
#90116=CARTESIAN_POINT('Ctrl Pts',(27.2639804710687,-37.5879824209777,20.));
#90117=CARTESIAN_POINT('Ctrl Pts',(27.2357177167352,-37.6048060545189,0.));
#90118=CARTESIAN_POINT('Ctrl Pts',(27.2357177167352,-37.6048060545189,20.));
#90119=CARTESIAN_POINT('Ctrl Pts',(27.2074440604332,-37.6216091747552,0.));
#90120=CARTESIAN_POINT('Ctrl Pts',(27.2074440604332,-37.6216091747552,20.));
#90121=CARTESIAN_POINT('Ctrl Pts',(27.1791595166855,-37.6383917740821,0.));
#90122=CARTESIAN_POINT('Ctrl Pts',(27.1791595166855,-37.6383917740821,20.));
#90123=CARTESIAN_POINT('Ctrl Pts',(27.15086410002,-37.6551538449046,0.));
#90124=CARTESIAN_POINT('Ctrl Pts',(27.15086410002,-37.6551538449046,20.));
#90125=CARTESIAN_POINT('Ctrl Pts',(27.1225578249702,-37.6718953796384,0.));
#90126=CARTESIAN_POINT('Ctrl Pts',(27.1225578249702,-37.6718953796384,20.));
#90127=CARTESIAN_POINT('Ctrl Pts',(27.0942407060752,-37.6886163707084,0.));
#90128=CARTESIAN_POINT('Ctrl Pts',(27.0942407060752,-37.6886163707084,20.));
#90129=CARTESIAN_POINT('Ctrl Pts',(27.0659127578793,-37.705316810549,0.));
#90130=CARTESIAN_POINT('Ctrl Pts',(27.0659127578793,-37.705316810549,20.));
#90131=CARTESIAN_POINT('Ctrl Pts',(27.0375739949332,-37.7219966916053,0.));
#90132=CARTESIAN_POINT('Ctrl Pts',(27.0375739949332,-37.7219966916053,20.));
#90133=CARTESIAN_POINT('Ctrl Pts',(27.0092244317933,-37.7386560063324,0.));
#90134=CARTESIAN_POINT('Ctrl Pts',(27.0092244317933,-37.7386560063324,20.));
#90135=CARTESIAN_POINT('Ctrl Pts',(26.9808640830224,-37.755294747196,0.));
#90136=CARTESIAN_POINT('Ctrl Pts',(26.9808640830224,-37.755294747196,20.));
#90137=CARTESIAN_POINT('Ctrl Pts',(26.9524929631885,-37.7719129066716,0.));
#90138=CARTESIAN_POINT('Ctrl Pts',(26.9524929631885,-37.7719129066716,20.));
#90139=CARTESIAN_POINT('Ctrl Pts',(26.9241110868652,-37.7885104772446,0.));
#90140=CARTESIAN_POINT('Ctrl Pts',(26.9241110868652,-37.7885104772446,20.));
#90141=CARTESIAN_POINT('Ctrl Pts',(26.8957184686315,-37.8050874514106,0.));
#90142=CARTESIAN_POINT('Ctrl Pts',(26.8957184686315,-37.8050874514106,20.));
#90143=CARTESIAN_POINT('Ctrl Pts',(26.8673151230714,-37.8216438216745,0.));
#90144=CARTESIAN_POINT('Ctrl Pts',(26.8673151230714,-37.8216438216745,20.));
#90145=CARTESIAN_POINT('Ctrl Pts',(26.8389010647754,-37.8381795805523,0.));
#90146=CARTESIAN_POINT('Ctrl Pts',(26.8389010647754,-37.8381795805523,20.));
#90147=CARTESIAN_POINT('Ctrl Pts',(26.8104763083398,-37.8546947205707,0.));
#90148=CARTESIAN_POINT('Ctrl Pts',(26.8104763083398,-37.8546947205707,20.));
#90149=CARTESIAN_POINT('Ctrl Pts',(26.7820408683669,-37.8711892342661,0.));
#90150=CARTESIAN_POINT('Ctrl Pts',(26.7820408683669,-37.8711892342661,20.));
#90151=CARTESIAN_POINT('Ctrl Pts',(26.7535947594648,-37.887663114185,0.));
#90152=CARTESIAN_POINT('Ctrl Pts',(26.7535947594648,-37.887663114185,20.));
#90153=CARTESIAN_POINT('Ctrl Pts',(26.7251379962461,-37.904116352883,0.));
#90154=CARTESIAN_POINT('Ctrl Pts',(26.7251379962461,-37.904116352883,20.));
#90155=CARTESIAN_POINT('Ctrl Pts',(26.6966705933291,-37.9205489429259,0.));
#90156=CARTESIAN_POINT('Ctrl Pts',(26.6966705933291,-37.9205489429259,20.));
#90157=CARTESIAN_POINT('Ctrl Pts',(26.6681925653377,-37.9369608768897,0.));
#90158=CARTESIAN_POINT('Ctrl Pts',(26.6681925653377,-37.9369608768897,20.));
#90159=CARTESIAN_POINT('Ctrl Pts',(26.6397039269022,-37.9533521473617,0.));
#90160=CARTESIAN_POINT('Ctrl Pts',(26.6397039269022,-37.9533521473617,20.));
#90161=CARTESIAN_POINT('Ctrl Pts',(26.6112046926582,-37.9697227469389,0.));
#90162=CARTESIAN_POINT('Ctrl Pts',(26.6112046926582,-37.9697227469389,20.));
#90163=CARTESIAN_POINT('Ctrl Pts',(26.5826948772471,-37.9860726682287,0.));
#90164=CARTESIAN_POINT('Ctrl Pts',(26.5826948772471,-37.9860726682287,20.));
#90165=CARTESIAN_POINT('Ctrl Pts',(26.5541744953162,-38.0024019038486,0.));
#90166=CARTESIAN_POINT('Ctrl Pts',(26.5541744953162,-38.0024019038486,20.));
#90167=CARTESIAN_POINT('Ctrl Pts',(26.5256435615177,-38.0187104464255,0.));
#90168=CARTESIAN_POINT('Ctrl Pts',(26.5256435615177,-38.0187104464255,20.));
#90169=CARTESIAN_POINT('Ctrl Pts',(26.4971020905092,-38.0349982885963,0.));
#90170=CARTESIAN_POINT('Ctrl Pts',(26.4971020905092,-38.0349982885963,20.));
#90171=CARTESIAN_POINT('Ctrl Pts',(26.4685500969542,-38.0512654230086,0.));
#90172=CARTESIAN_POINT('Ctrl Pts',(26.4685500969542,-38.0512654230086,20.));
#90173=CARTESIAN_POINT('Ctrl Pts',(26.4399875955219,-38.0675118423201,0.));
#90174=CARTESIAN_POINT('Ctrl Pts',(26.4399875955219,-38.0675118423201,20.));
#90175=CARTESIAN_POINT('Ctrl Pts',(26.4114146008872,-38.0837375391992,0.));
#90176=CARTESIAN_POINT('Ctrl Pts',(26.4114146008872,-38.0837375391992,20.));
#90177=CARTESIAN_POINT('Ctrl Pts',(26.38283112773,-38.0999425063245,0.));
#90178=CARTESIAN_POINT('Ctrl Pts',(26.38283112773,-38.0999425063245,20.));
#90179=CARTESIAN_POINT('Ctrl Pts',(26.3542371907363,-38.1161267363846,0.));
#90180=CARTESIAN_POINT('Ctrl Pts',(26.3542371907363,-38.1161267363846,20.));
#90181=CARTESIAN_POINT('Ctrl Pts',(26.3256328045975,-38.1322902220784,0.));
#90182=CARTESIAN_POINT('Ctrl Pts',(26.3256328045975,-38.1322902220784,20.));
#90183=CARTESIAN_POINT('Ctrl Pts',(26.2970179840108,-38.1484329561142,0.));
#90184=CARTESIAN_POINT('Ctrl Pts',(26.2970179840108,-38.1484329561142,20.));
#90185=CARTESIAN_POINT('Ctrl Pts',(26.2683927436784,-38.1645549312104,0.));
#90186=CARTESIAN_POINT('Ctrl Pts',(26.2683927436784,-38.1645549312104,20.));
#90187=CARTESIAN_POINT('Ctrl Pts',(26.2397570983077,-38.1806561400953,0.));
#90188=CARTESIAN_POINT('Ctrl Pts',(26.2397570983077,-38.1806561400953,20.));
#90189=CARTESIAN_POINT('Ctrl Pts',(26.2111110626121,-38.1967365755081,0.));
#90190=CARTESIAN_POINT('Ctrl Pts',(26.2111110626121,-38.1967365755081,20.));
#90191=CARTESIAN_POINT('Ctrl Pts',(26.1824546513102,-38.2127962301983,0.));
#90192=CARTESIAN_POINT('Ctrl Pts',(26.1824546513102,-38.2127962301983,20.));
#90193=CARTESIAN_POINT('Ctrl Pts',(26.1537878791271,-38.2288350969267,0.));
#90194=CARTESIAN_POINT('Ctrl Pts',(26.1537878791271,-38.2288350969267,20.));
#90195=CARTESIAN_POINT('Ctrl Pts',(26.1251107607929,-38.244853168464,0.));
#90196=CARTESIAN_POINT('Ctrl Pts',(26.1251107607929,-38.244853168464,20.));
#90197=CARTESIAN_POINT('Ctrl Pts',(26.0964233110434,-38.2608504375907,0.));
#90198=CARTESIAN_POINT('Ctrl Pts',(26.0964233110434,-38.2608504375907,20.));
#90199=CARTESIAN_POINT('Ctrl Pts',(26.0677255446196,-38.276826897097,0.));
#90200=CARTESIAN_POINT('Ctrl Pts',(26.0677255446196,-38.276826897097,20.));
#90201=CARTESIAN_POINT('Ctrl Pts',(26.0390174762675,-38.2927825397833,0.));
#90202=CARTESIAN_POINT('Ctrl Pts',(26.0390174762675,-38.2927825397833,20.));
#90203=CARTESIAN_POINT('Ctrl Pts',(26.0102991207387,-38.30871735846,0.));
#90204=CARTESIAN_POINT('Ctrl Pts',(26.0102991207387,-38.30871735846,20.));
#90205=CARTESIAN_POINT('Ctrl Pts',(25.9815704927901,-38.3246313459476,0.));
#90206=CARTESIAN_POINT('Ctrl Pts',(25.9815704927901,-38.3246313459476,20.));
#90207=CARTESIAN_POINT('Ctrl Pts',(25.9528316071847,-38.3405244950781,0.));
#90208=CARTESIAN_POINT('Ctrl Pts',(25.9528316071847,-38.3405244950781,20.));
#90209=CARTESIAN_POINT('Ctrl Pts',(25.9240824786908,-38.3563967986932,0.));
#90210=CARTESIAN_POINT('Ctrl Pts',(25.9240824786908,-38.3563967986932,20.));
#90211=CARTESIAN_POINT('Ctrl Pts',(25.8953231220827,-38.3722482496454,0.));
#90212=CARTESIAN_POINT('Ctrl Pts',(25.8953231220827,-38.3722482496454,20.));
#90213=CARTESIAN_POINT('Ctrl Pts',(25.8665535521392,-38.3880788407969,0.));
#90214=CARTESIAN_POINT('Ctrl Pts',(25.8665535521392,-38.3880788407969,20.));
#90215=CARTESIAN_POINT('Ctrl Pts',(25.8377737836446,-38.4038885650199,0.));
#90216=CARTESIAN_POINT('Ctrl Pts',(25.8377737836446,-38.4038885650199,20.));
#90217=CARTESIAN_POINT('Ctrl Pts',(25.8089838313888,-38.419677415197,0.));
#90218=CARTESIAN_POINT('Ctrl Pts',(25.8089838313888,-38.419677415197,20.));
#90219=CARTESIAN_POINT('Ctrl Pts',(25.7801837101667,-38.4354453842206,0.));
#90220=CARTESIAN_POINT('Ctrl Pts',(25.7801837101667,-38.4354453842206,20.));
#90221=CARTESIAN_POINT('Ctrl Pts',(25.7513734347795,-38.4511924649945,0.));
#90222=CARTESIAN_POINT('Ctrl Pts',(25.7513734347795,-38.4511924649945,20.));
#90223=CARTESIAN_POINT('Ctrl Pts',(25.7225530200331,-38.4669186504318,0.));
#90224=CARTESIAN_POINT('Ctrl Pts',(25.7225530200331,-38.4669186504318,20.));
#90225=CARTESIAN_POINT('Ctrl Pts',(25.6937224807392,-38.4826239334567,0.));
#90226=CARTESIAN_POINT('Ctrl Pts',(25.6937224807392,-38.4826239334567,20.));
#90227=CARTESIAN_POINT('Ctrl Pts',(25.6648818317151,-38.4983083070042,0.));
#90228=CARTESIAN_POINT('Ctrl Pts',(25.6648818317151,-38.4983083070042,20.));
#90229=CARTESIAN_POINT('Ctrl Pts',(25.6360310877836,-38.5139717640192,0.));
#90230=CARTESIAN_POINT('Ctrl Pts',(25.6360310877836,-38.5139717640192,20.));
#90231=CARTESIAN_POINT('Ctrl Pts',(25.6071702637723,-38.5296142974561,0.));
#90232=CARTESIAN_POINT('Ctrl Pts',(25.6071702637723,-38.5296142974561,20.));
#90233=CARTESIAN_POINT('Ctrl Pts',(25.5782993745137,-38.5452359002793,0.));
#90234=CARTESIAN_POINT('Ctrl Pts',(25.5782993745137,-38.5452359002793,20.));
#90235=CARTESIAN_POINT('Ctrl Pts',(25.5494184348456,-38.5608365654634,0.));
#90236=CARTESIAN_POINT('Ctrl Pts',(25.5494184348456,-38.5608365654634,20.));
#90237=CARTESIAN_POINT('Ctrl Pts',(25.5205274596115,-38.576416285994,0.));
#90238=CARTESIAN_POINT('Ctrl Pts',(25.5205274596115,-38.576416285994,20.));
#90239=CARTESIAN_POINT('Ctrl Pts',(25.4916264636604,-38.591975054867,0.));
#90240=CARTESIAN_POINT('Ctrl Pts',(25.4916264636604,-38.591975054867,20.));
#90241=CARTESIAN_POINT('Ctrl Pts',(25.462715461847,-38.6075128650891,0.));
#90242=CARTESIAN_POINT('Ctrl Pts',(25.462715461847,-38.6075128650891,20.));
#90243=CARTESIAN_POINT('Ctrl Pts',(25.4337944690316,-38.6230297096774,0.));
#90244=CARTESIAN_POINT('Ctrl Pts',(25.4337944690316,-38.6230297096774,20.));
#90245=CARTESIAN_POINT('Ctrl Pts',(25.4048635000794,-38.6385255816593,0.));
#90246=CARTESIAN_POINT('Ctrl Pts',(25.4048635000794,-38.6385255816593,20.));
#90247=CARTESIAN_POINT('Ctrl Pts',(25.3759225698613,-38.6540004740723,0.));
#90248=CARTESIAN_POINT('Ctrl Pts',(25.3759225698613,-38.6540004740723,20.));
#90249=CARTESIAN_POINT('Ctrl Pts',(25.3469716932528,-38.6694543799641,0.));
#90250=CARTESIAN_POINT('Ctrl Pts',(25.3469716932528,-38.6694543799641,20.));
#90251=CARTESIAN_POINT('Ctrl Pts',(25.318010885134,-38.6848872923919,0.));
#90252=CARTESIAN_POINT('Ctrl Pts',(25.318010885134,-38.6848872923919,20.));
#90253=CARTESIAN_POINT('Ctrl Pts',(25.2890401603912,-38.7002992044242,0.));
#90254=CARTESIAN_POINT('Ctrl Pts',(25.2890401603912,-38.7002992044242,20.));
#90255=CARTESIAN_POINT('Ctrl Pts',(25.2600595339159,-38.7156901091392,0.));
#90256=CARTESIAN_POINT('Ctrl Pts',(25.2600595339159,-38.7156901091392,20.));
#90257=CARTESIAN_POINT('Ctrl Pts',(25.2310690206049,-38.7310599996258,0.));
#90258=CARTESIAN_POINT('Ctrl Pts',(25.2310690206049,-38.7310599996258,20.));
#90259=CARTESIAN_POINT('Ctrl Pts',(25.2020686353608,-38.7464088689837,0.));
#90260=CARTESIAN_POINT('Ctrl Pts',(25.2020686353608,-38.7464088689837,20.));
#90261=CARTESIAN_POINT('Ctrl Pts',(25.1730583930911,-38.7617367103229,0.));
#90262=CARTESIAN_POINT('Ctrl Pts',(25.1730583930911,-38.7617367103229,20.));
#90263=CARTESIAN_POINT('Ctrl Pts',(25.1440383087084,-38.7770435167639,0.));
#90264=CARTESIAN_POINT('Ctrl Pts',(25.1440383087084,-38.7770435167639,20.));
#90265=CARTESIAN_POINT('Ctrl Pts',(25.1150083971302,-38.7923292814368,0.));
#90266=CARTESIAN_POINT('Ctrl Pts',(25.1150083971302,-38.7923292814368,20.));
#90267=CARTESIAN_POINT('Ctrl Pts',(25.0859686732794,-38.8075939974829,0.));
#90268=CARTESIAN_POINT('Ctrl Pts',(25.0859686732794,-38.8075939974829,20.));
#90269=CARTESIAN_POINT('Ctrl Pts',(25.0569191520845,-38.8228376580533,0.));
#90270=CARTESIAN_POINT('Ctrl Pts',(25.0569191520845,-38.8228376580533,20.));
#90271=CARTESIAN_POINT('Ctrl Pts',(25.0278598484791,-38.8380602563098,0.));
#90272=CARTESIAN_POINT('Ctrl Pts',(25.0278598484791,-38.8380602563098,20.));
#90273=CARTESIAN_POINT('Ctrl Pts',(24.9987907774025,-38.8532617854245,0.));
#90274=CARTESIAN_POINT('Ctrl Pts',(24.9987907774025,-38.8532617854245,20.));
#90275=CARTESIAN_POINT('Ctrl Pts',(24.9697119537988,-38.8684422385799,0.));
#90276=CARTESIAN_POINT('Ctrl Pts',(24.9697119537988,-38.8684422385799,20.));
#90277=CARTESIAN_POINT('Ctrl Pts',(24.9406233926168,-38.883601608968,0.));
#90278=CARTESIAN_POINT('Ctrl Pts',(24.9406233926168,-38.883601608968,20.));
#90279=CARTESIAN_POINT('Ctrl Pts',(24.9115251088107,-38.8987398897918,0.));
#90280=CARTESIAN_POINT('Ctrl Pts',(24.9115251088107,-38.8987398897918,20.));
#90281=CARTESIAN_POINT('Ctrl Pts',(24.8824171173401,-38.9138570742648,0.));
#90282=CARTESIAN_POINT('Ctrl Pts',(24.8824171173401,-38.9138570742648,20.));
#90283=CARTESIAN_POINT('Ctrl Pts',(24.8532994331703,-38.9289531556118,0.));
#90284=CARTESIAN_POINT('Ctrl Pts',(24.8532994331703,-38.9289531556118,20.));
#90285=CARTESIAN_POINT('Ctrl Pts',(24.8241720712716,-38.9440281270684,0.));
#90286=CARTESIAN_POINT('Ctrl Pts',(24.8241720712716,-38.9440281270684,20.));
#90287=CARTESIAN_POINT('Ctrl Pts',(24.7950350466188,-38.9590819818798,0.));
#90288=CARTESIAN_POINT('Ctrl Pts',(24.7950350466188,-38.9590819818798,20.));
#90289=CARTESIAN_POINT('Ctrl Pts',(24.7658883741919,-38.9741147133012,0.));
#90290=CARTESIAN_POINT('Ctrl Pts',(24.7658883741919,-38.9741147133012,20.));
#90291=CARTESIAN_POINT('Ctrl Pts',(24.736732068976,-38.989126314598,0.));
#90292=CARTESIAN_POINT('Ctrl Pts',(24.736732068976,-38.989126314598,20.));
#90293=CARTESIAN_POINT('Ctrl Pts',(24.7075661459616,-39.0041167790461,0.));
#90294=CARTESIAN_POINT('Ctrl Pts',(24.7075661459616,-39.0041167790461,20.));
#90295=CARTESIAN_POINT('Ctrl Pts',(24.6783906201452,-39.019086099931,0.));
#90296=CARTESIAN_POINT('Ctrl Pts',(24.6783906201452,-39.019086099931,20.));
#90297=CARTESIAN_POINT('Ctrl Pts',(24.6492055065285,-39.0340342705498,0.));
#90298=CARTESIAN_POINT('Ctrl Pts',(24.6492055065285,-39.0340342705498,20.));
#90299=CARTESIAN_POINT('Ctrl Pts',(24.6200108201182,-39.0489612842096,0.));
#90300=CARTESIAN_POINT('Ctrl Pts',(24.6200108201182,-39.0489612842096,20.));
#90301=CARTESIAN_POINT('Ctrl Pts',(24.5908065759258,-39.0638671342286,0.));
#90302=CARTESIAN_POINT('Ctrl Pts',(24.5908065759258,-39.0638671342286,20.));
#90303=CARTESIAN_POINT('Ctrl Pts',(24.5615927889669,-39.0787518139362,0.));
#90304=CARTESIAN_POINT('Ctrl Pts',(24.5615927889669,-39.0787518139362,20.));
#90305=CARTESIAN_POINT('Ctrl Pts',(24.5323694742616,-39.0936153166722,0.));
#90306=CARTESIAN_POINT('Ctrl Pts',(24.5323694742616,-39.0936153166722,20.));
#90307=CARTESIAN_POINT('Ctrl Pts',(24.5031366468345,-39.1084576357872,0.));
#90308=CARTESIAN_POINT('Ctrl Pts',(24.5031366468345,-39.1084576357872,20.));
#90309=CARTESIAN_POINT('Ctrl Pts',(24.4738943217155,-39.1232787646414,0.));
#90310=CARTESIAN_POINT('Ctrl Pts',(24.4738943217155,-39.1232787646414,20.));
#90311=CARTESIAN_POINT('Ctrl Pts',(24.4446425139409,-39.1380786966047,0.));
#90312=CARTESIAN_POINT('Ctrl Pts',(24.4446425139409,-39.1380786966047,20.));
#90313=CARTESIAN_POINT('Ctrl Pts',(24.4153812385543,-39.1528574250569,0.));
#90314=CARTESIAN_POINT('Ctrl Pts',(24.4153812385543,-39.1528574250569,20.));
#90315=CARTESIAN_POINT('Ctrl Pts',(24.3861105106067,-39.1676149433869,0.));
#90316=CARTESIAN_POINT('Ctrl Pts',(24.3861105106067,-39.1676149433869,20.));
#90317=CARTESIAN_POINT('Ctrl Pts',(24.3568303451549,-39.1823512449951,0.));
#90318=CARTESIAN_POINT('Ctrl Pts',(24.3568303451549,-39.1823512449951,20.));
#90319=CARTESIAN_POINT('Ctrl Pts',(24.3275407572587,-39.197066323292,0.));
#90320=CARTESIAN_POINT('Ctrl Pts',(24.3275407572587,-39.197066323292,20.));
#90321=CARTESIAN_POINT('Ctrl Pts',(24.2982417619806,-39.2117601717005,0.));
#90322=CARTESIAN_POINT('Ctrl Pts',(24.2982417619806,-39.2117601717005,20.));
#90323=CARTESIAN_POINT('Ctrl Pts',(24.2689333743822,-39.2264327836562,0.));
#90324=CARTESIAN_POINT('Ctrl Pts',(24.2689333743822,-39.2264327836562,20.));
#90325=CARTESIAN_POINT('Ctrl Pts',(24.239615609526,-39.2410841526078,0.));
#90326=CARTESIAN_POINT('Ctrl Pts',(24.239615609526,-39.2410841526078,20.));
#90327=CARTESIAN_POINT('Ctrl Pts',(24.2102884824784,-39.2557142720138,0.));
#90328=CARTESIAN_POINT('Ctrl Pts',(24.2102884824784,-39.2557142720138,20.));
#90329=CARTESIAN_POINT('Ctrl Pts',(24.1809520083146,-39.2703231353422,0.));
#90330=CARTESIAN_POINT('Ctrl Pts',(24.1809520083146,-39.2703231353422,20.));
#90331=CARTESIAN_POINT('Ctrl Pts',(24.1516062021224,-39.2849107360681,0.));
#90332=CARTESIAN_POINT('Ctrl Pts',(24.1516062021224,-39.2849107360681,20.));
#90333=CARTESIAN_POINT('Ctrl Pts',(24.1222510790066,-39.2994770676712,0.));
#90334=CARTESIAN_POINT('Ctrl Pts',(24.1222510790066,-39.2994770676712,20.));
#90335=CARTESIAN_POINT('Ctrl Pts',(24.0928866540881,-39.3140221236369,0.));
#90336=CARTESIAN_POINT('Ctrl Pts',(24.0928866540881,-39.3140221236369,20.));
#90337=CARTESIAN_POINT('Ctrl Pts',(24.0635129424931,-39.3285458974613,0.));
#90338=CARTESIAN_POINT('Ctrl Pts',(24.0635129424931,-39.3285458974613,20.));
#90339=CARTESIAN_POINT('Ctrl Pts',(24.0341299593437,-39.3430483826555,0.));
#90340=CARTESIAN_POINT('Ctrl Pts',(24.0341299593437,-39.3430483826555,20.));
#90341=CARTESIAN_POINT('Ctrl Pts',(24.0047377197503,-39.3575295727493,0.));
#90342=CARTESIAN_POINT('Ctrl Pts',(24.0047377197503,-39.3575295727493,20.));
#90343=CARTESIAN_POINT('Ctrl Pts',(23.9753362387978,-39.3719894612957,0.));
#90344=CARTESIAN_POINT('Ctrl Pts',(23.9753362387978,-39.3719894612957,20.));
#90345=CARTESIAN_POINT('Ctrl Pts',(23.9459255315518,-39.3864280418676,0.));
#90346=CARTESIAN_POINT('Ctrl Pts',(23.9459255315518,-39.3864280418676,20.));
#90347=CARTESIAN_POINT('Ctrl Pts',(23.9165056130837,-39.4008453080481,0.));
#90348=CARTESIAN_POINT('Ctrl Pts',(23.9165056130837,-39.4008453080481,20.));
#90349=CARTESIAN_POINT('Ctrl Pts',(23.8870764984925,-39.4152412534209,0.));
#90350=CARTESIAN_POINT('Ctrl Pts',(23.8870764984925,-39.4152412534209,20.));
#90351=CARTESIAN_POINT('Ctrl Pts',(23.8576382029237,-39.4296158715627,0.));
#90352=CARTESIAN_POINT('Ctrl Pts',(23.8576382029237,-39.4296158715627,20.));
#90353=CARTESIAN_POINT('Ctrl Pts',(23.8281907416004,-39.4439691560298,0.));
#90354=CARTESIAN_POINT('Ctrl Pts',(23.8281907416004,-39.4439691560298,20.));
#90355=CARTESIAN_POINT('Ctrl Pts',(23.7987341298022,-39.4583011003674,0.));
#90356=CARTESIAN_POINT('Ctrl Pts',(23.7987341298022,-39.4583011003674,20.));
#90357=CARTESIAN_POINT('Ctrl Pts',(23.769268382808,-39.4726116981337,0.));
#90358=CARTESIAN_POINT('Ctrl Pts',(23.769268382808,-39.4726116981337,20.));
#90359=CARTESIAN_POINT('Ctrl Pts',(23.7397935158457,-39.4869009429217,0.));
#90360=CARTESIAN_POINT('Ctrl Pts',(23.7397935158457,-39.4869009429217,20.));
#90361=CARTESIAN_POINT('Ctrl Pts',(23.7103095440476,-39.5011688283778,0.));
#90362=CARTESIAN_POINT('Ctrl Pts',(23.7103095440476,-39.5011688283778,20.));
#90363=CARTESIAN_POINT('Ctrl Pts',(23.6808164823786,-39.5154153482324,0.));
#90364=CARTESIAN_POINT('Ctrl Pts',(23.6808164823786,-39.5154153482324,20.));
#90365=CARTESIAN_POINT('Ctrl Pts',(23.651314345698,-39.5296404962722,0.));
#90366=CARTESIAN_POINT('Ctrl Pts',(23.651314345698,-39.5296404962722,20.));
#90367=CARTESIAN_POINT('Ctrl Pts',(23.6218031488904,-39.5438442662853,0.));
#90368=CARTESIAN_POINT('Ctrl Pts',(23.6218031488904,-39.5438442662853,20.));
#90369=CARTESIAN_POINT('Ctrl Pts',(23.5922829069852,-39.5580266520107,0.));
#90370=CARTESIAN_POINT('Ctrl Pts',(23.5922829069852,-39.5580266520107,20.));
#90371=CARTESIAN_POINT('Ctrl Pts',(23.5627536352592,-39.5721876470956,0.));
#90372=CARTESIAN_POINT('Ctrl Pts',(23.5627536352592,-39.5721876470956,20.));
#90373=CARTESIAN_POINT('Ctrl Pts',(23.5332153494019,-39.5863272450268,0.));
#90374=CARTESIAN_POINT('Ctrl Pts',(23.5332153494019,-39.5863272450268,20.));
#90375=CARTESIAN_POINT('Ctrl Pts',(23.5036680653391,-39.6004454392038,0.));
#90376=CARTESIAN_POINT('Ctrl Pts',(23.5036680653391,-39.6004454392038,20.));
#90377=CARTESIAN_POINT('Ctrl Pts',(23.4741117989348,-39.6145422230651,0.));
#90378=CARTESIAN_POINT('Ctrl Pts',(23.4741117989348,-39.6145422230651,20.));
#90379=CARTESIAN_POINT('Ctrl Pts',(23.4445465657147,-39.6286175902046,0.));
#90380=CARTESIAN_POINT('Ctrl Pts',(23.4445465657147,-39.6286175902046,20.));
#90381=CARTESIAN_POINT('Ctrl Pts',(23.414972380622,-39.6426715344742,0.));
#90382=CARTESIAN_POINT('Ctrl Pts',(23.414972380622,-39.6426715344742,20.));
#90383=CARTESIAN_POINT('Ctrl Pts',(23.385389257652,-39.6567040501382,0.));
#90384=CARTESIAN_POINT('Ctrl Pts',(23.385389257652,-39.6567040501382,20.));
#90385=CARTESIAN_POINT('Ctrl Pts',(23.3557972103217,-39.6707151316771,0.));
#90386=CARTESIAN_POINT('Ctrl Pts',(23.3557972103217,-39.6707151316771,20.));
#90387=CARTESIAN_POINT('Ctrl Pts',(23.3261962523444,-39.6847047735001,0.));
#90388=CARTESIAN_POINT('Ctrl Pts',(23.3261962523444,-39.6847047735001,20.));
#90389=CARTESIAN_POINT('Ctrl Pts',(23.2965863982648,-39.6986729696788,0.));
#90390=CARTESIAN_POINT('Ctrl Pts',(23.2965863982648,-39.6986729696788,20.));
#90391=CARTESIAN_POINT('Ctrl Pts',(23.2669676640418,-39.7126197136991,0.));
#90392=CARTESIAN_POINT('Ctrl Pts',(23.2669676640418,-39.7126197136991,20.));
#90393=CARTESIAN_POINT('Ctrl Pts',(23.2373400678346,-39.7265449981305,0.));
#90394=CARTESIAN_POINT('Ctrl Pts',(23.2373400678346,-39.7265449981305,20.));
#90395=CARTESIAN_POINT('Ctrl Pts',(23.2077036288597,-39.7404488151086,0.));
#90396=CARTESIAN_POINT('Ctrl Pts',(23.2077036288597,-39.7404488151086,20.));
#90397=CARTESIAN_POINT('Ctrl Pts',(23.1780583659508,-39.7543311569459,0.));
#90398=CARTESIAN_POINT('Ctrl Pts',(23.1780583659508,-39.7543311569459,20.));
#90399=CARTESIAN_POINT('Ctrl Pts',(23.1484042962029,-39.7681920167058,0.));
#90400=CARTESIAN_POINT('Ctrl Pts',(23.1484042962029,-39.7681920167058,20.));
#90401=CARTESIAN_POINT('Ctrl Pts',(23.118741433625,-39.7820313887737,0.));
#90402=CARTESIAN_POINT('Ctrl Pts',(23.118741433625,-39.7820313887737,20.));
#90403=CARTESIAN_POINT('Ctrl Pts',(23.089069787673,-39.7958492694787,0.));
#90404=CARTESIAN_POINT('Ctrl Pts',(23.089069787673,-39.7958492694787,20.));
#90405=CARTESIAN_POINT('Ctrl Pts',(23.0593893640427,-39.8096456567259,0.));
#90406=CARTESIAN_POINT('Ctrl Pts',(23.0593893640427,-39.8096456567259,20.));
#90407=CARTESIAN_POINT('Ctrl Pts',(23.0356380053138,-39.8206655709904,0.));
#90408=CARTESIAN_POINT('Ctrl Pts',(23.0356380053138,-39.8206655709904,20.));
#90409=CARTESIAN_POINT('Ctrl Pts',(23.0178205380655,-39.8289208340947,0.));
#90410=CARTESIAN_POINT('Ctrl Pts',(23.0178205380655,-39.8289208340947,20.));
#90411=CARTESIAN_POINT('Ctrl Pts',(23.0059404718139,-39.8344200439082,0.));
#90412=CARTESIAN_POINT('Ctrl Pts',(23.0059404718139,-39.8344200439082,20.));
#90413=CARTESIAN_POINT('Ctrl Pts',(23.,-39.8371685740842,0.));
#90414=CARTESIAN_POINT('Ctrl Pts',(23.,-39.8371685740842,20.));
#90415=CARTESIAN_POINT('Origin',(43.2258605561518,-15.7329265929808,0.));
#90416=CARTESIAN_POINT('',(44.1555553153094,-16.0713078122675,0.));
#90417=CARTESIAN_POINT('Origin',(44.4975754586351,-15.1316151914816,0.));
#90418=CARTESIAN_POINT('',(43.5508185339833,-14.8096659320883,0.));
#90419=CARTESIAN_POINT('Origin',(1.83021655258307E-13,-3.27857114887026E-14,
0.));
#90420=CARTESIAN_POINT('',(46.,0.,0.));
#90421=CARTESIAN_POINT('Ctrl Pts',(37.5361777128299,31.4965928746404,0.));
#90422=CARTESIAN_POINT('Ctrl Pts',(37.5361777128299,31.4965928746404,20.));
#90423=CARTESIAN_POINT('Ctrl Pts',(37.5400435810124,31.4910366171629,0.));
#90424=CARTESIAN_POINT('Ctrl Pts',(37.5400435810124,31.4910366171629,20.));
#90425=CARTESIAN_POINT('Ctrl Pts',(37.5477733397938,31.4799228688318,0.));
#90426=CARTESIAN_POINT('Ctrl Pts',(37.5477733397938,31.4799228688318,20.));
#90427=CARTESIAN_POINT('Ctrl Pts',(37.5593620452151,31.4632485462068,0.));
#90428=CARTESIAN_POINT('Ctrl Pts',(37.5593620452151,31.4632485462068,20.));
#90429=CARTESIAN_POINT('Ctrl Pts',(37.574801786924,31.4410087157717,0.));
#90430=CARTESIAN_POINT('Ctrl Pts',(37.574801786924,31.4410087157717,20.));
#90431=CARTESIAN_POINT('Ctrl Pts',(37.5940816876034,31.4131965946731,0.));
#90432=CARTESIAN_POINT('Ctrl Pts',(37.5940816876034,31.4131965946731,20.));
#90433=CARTESIAN_POINT('Ctrl Pts',(37.6133418102375,31.3853721428083,0.));
#90434=CARTESIAN_POINT('Ctrl Pts',(37.6133418102375,31.3853721428083,20.));
#90435=CARTESIAN_POINT('Ctrl Pts',(37.6325821517747,31.3575353648538,0.));
#90436=CARTESIAN_POINT('Ctrl Pts',(37.6325821517747,31.3575353648538,20.));
#90437=CARTESIAN_POINT('Ctrl Pts',(37.6518027072643,31.3296862686536,0.));
#90438=CARTESIAN_POINT('Ctrl Pts',(37.6518027072643,31.3296862686536,20.));
#90439=CARTESIAN_POINT('Ctrl Pts',(37.6710034693473,31.3018248661211,0.));
#90440=CARTESIAN_POINT('Ctrl Pts',(37.6710034693473,31.3018248661211,20.));
#90441=CARTESIAN_POINT('Ctrl Pts',(37.6901844288974,31.2739511721649,0.));
#90442=CARTESIAN_POINT('Ctrl Pts',(37.6901844288974,31.2739511721649,20.));
#90443=CARTESIAN_POINT('Ctrl Pts',(37.7093455757381,31.2460652034827,0.));
#90444=CARTESIAN_POINT('Ctrl Pts',(37.7093455757381,31.2460652034827,20.));
#90445=CARTESIAN_POINT('Ctrl Pts',(37.7284868993471,31.2181669773772,0.));
#90446=CARTESIAN_POINT('Ctrl Pts',(37.7284868993471,31.2181669773772,20.));
#90447=CARTESIAN_POINT('Ctrl Pts',(37.7476083895316,31.1902565106222,0.));
#90448=CARTESIAN_POINT('Ctrl Pts',(37.7476083895316,31.1902565106222,20.));
#90449=CARTESIAN_POINT('Ctrl Pts',(37.7667100372089,31.1623338181506,0.));
#90450=CARTESIAN_POINT('Ctrl Pts',(37.7667100372089,31.1623338181506,20.));
#90451=CARTESIAN_POINT('Ctrl Pts',(37.7857918342009,31.1343989133989,0.));
#90452=CARTESIAN_POINT('Ctrl Pts',(37.7857918342009,31.1343989133989,20.));
#90453=CARTESIAN_POINT('Ctrl Pts',(37.8048537728749,31.1064518089103,0.));
#90454=CARTESIAN_POINT('Ctrl Pts',(37.8048537728749,31.1064518089103,20.));
#90455=CARTESIAN_POINT('Ctrl Pts',(37.8238958458276,31.0784925168637,0.));
#90456=CARTESIAN_POINT('Ctrl Pts',(37.8238958458276,31.0784925168637,20.));
#90457=CARTESIAN_POINT('Ctrl Pts',(37.8429180455734,31.0505210495984,0.));
#90458=CARTESIAN_POINT('Ctrl Pts',(37.8429180455734,31.0505210495984,20.));
#90459=CARTESIAN_POINT('Ctrl Pts',(37.861920364175,31.0225374202321,0.));
#90460=CARTESIAN_POINT('Ctrl Pts',(37.861920364175,31.0225374202321,20.));
#90461=CARTESIAN_POINT('Ctrl Pts',(37.8809027932971,30.9945416425721,0.));
#90462=CARTESIAN_POINT('Ctrl Pts',(37.8809027932971,30.9945416425721,20.));
#90463=CARTESIAN_POINT('Ctrl Pts',(37.8998653243731,30.9665337308352,0.));
#90464=CARTESIAN_POINT('Ctrl Pts',(37.8998653243731,30.9665337308352,20.));
#90465=CARTESIAN_POINT('Ctrl Pts',(37.9188079487378,30.9385136994261,0.));
#90466=CARTESIAN_POINT('Ctrl Pts',(37.9188079487378,30.9385136994261,20.));
#90467=CARTESIAN_POINT('Ctrl Pts',(37.9377306577632,30.9104815627079,0.));
#90468=CARTESIAN_POINT('Ctrl Pts',(37.9377306577632,30.9104815627079,20.));
#90469=CARTESIAN_POINT('Ctrl Pts',(37.9566334430211,30.882437334731,0.));
#90470=CARTESIAN_POINT('Ctrl Pts',(37.9566334430211,30.882437334731,20.));
#90471=CARTESIAN_POINT('Ctrl Pts',(37.9755162962752,30.8543810292446,0.));
#90472=CARTESIAN_POINT('Ctrl Pts',(37.9755162962752,30.8543810292446,20.));
#90473=CARTESIAN_POINT('Ctrl Pts',(37.9943792094053,30.8263126598247,0.));
#90474=CARTESIAN_POINT('Ctrl Pts',(37.9943792094053,30.8263126598247,20.));
#90475=CARTESIAN_POINT('Ctrl Pts',(38.0132221743517,30.7982322399668,0.));
#90476=CARTESIAN_POINT('Ctrl Pts',(38.0132221743517,30.7982322399668,20.));
#90477=CARTESIAN_POINT('Ctrl Pts',(38.0320451830565,30.7701397831859,0.));
#90478=CARTESIAN_POINT('Ctrl Pts',(38.0320451830565,30.7701397831859,20.));
#90479=CARTESIAN_POINT('Ctrl Pts',(38.0508482273931,30.7420353031339,0.));
#90480=CARTESIAN_POINT('Ctrl Pts',(38.0508482273931,30.7420353031339,20.));
#90481=CARTESIAN_POINT('Ctrl Pts',(38.0696312991626,30.7139188136053,0.));
#90482=CARTESIAN_POINT('Ctrl Pts',(38.0696312991626,30.7139188136053,20.));
#90483=CARTESIAN_POINT('Ctrl Pts',(38.088394390128,30.6857903284809,0.));
#90484=CARTESIAN_POINT('Ctrl Pts',(38.088394390128,30.6857903284809,20.));
#90485=CARTESIAN_POINT('Ctrl Pts',(38.1071374920373,30.6576498616875,0.));
#90486=CARTESIAN_POINT('Ctrl Pts',(38.1071374920373,30.6576498616875,20.));
#90487=CARTESIAN_POINT('Ctrl Pts',(38.125860596649,30.6294974271553,0.));
#90488=CARTESIAN_POINT('Ctrl Pts',(38.125860596649,30.6294974271553,20.));
#90489=CARTESIAN_POINT('Ctrl Pts',(38.1445636957629,30.6013330387675,0.));
#90490=CARTESIAN_POINT('Ctrl Pts',(38.1445636957629,30.6013330387675,20.));
#90491=CARTESIAN_POINT('Ctrl Pts',(38.1632467812242,30.5731567103519,0.));
#90492=CARTESIAN_POINT('Ctrl Pts',(38.1632467812242,30.5731567103519,20.));
#90493=CARTESIAN_POINT('Ctrl Pts',(38.1819098449085,30.5449684557073,0.));
#90494=CARTESIAN_POINT('Ctrl Pts',(38.1819098449085,30.5449684557073,20.));
#90495=CARTESIAN_POINT('Ctrl Pts',(38.2005528787125,30.5167682886194,0.));
#90496=CARTESIAN_POINT('Ctrl Pts',(38.2005528787125,30.5167682886194,20.));
#90497=CARTESIAN_POINT('Ctrl Pts',(38.2191758745422,30.4885562228796,0.));
#90498=CARTESIAN_POINT('Ctrl Pts',(38.2191758745422,30.4885562228796,20.));
#90499=CARTESIAN_POINT('Ctrl Pts',(38.2377788243005,30.460332272307,0.));
#90500=CARTESIAN_POINT('Ctrl Pts',(38.2377788243005,30.460332272307,20.));
#90501=CARTESIAN_POINT('Ctrl Pts',(38.2563617198829,30.4320964507535,0.));
#90502=CARTESIAN_POINT('Ctrl Pts',(38.2563617198829,30.4320964507535,20.));
#90503=CARTESIAN_POINT('Ctrl Pts',(38.2749245531853,30.4038487720928,0.));
#90504=CARTESIAN_POINT('Ctrl Pts',(38.2749245531853,30.4038487720928,20.));
#90505=CARTESIAN_POINT('Ctrl Pts',(38.2934673161074,30.3755892502132,0.));
#90506=CARTESIAN_POINT('Ctrl Pts',(38.2934673161074,30.3755892502132,20.));
#90507=CARTESIAN_POINT('Ctrl Pts',(38.3119900005578,30.3473178990095,0.));
#90508=CARTESIAN_POINT('Ctrl Pts',(38.3119900005578,30.3473178990095,20.));
#90509=CARTESIAN_POINT('Ctrl Pts',(38.3304925984593,30.3190347323738,0.));
#90510=CARTESIAN_POINT('Ctrl Pts',(38.3304925984593,30.3190347323738,20.));
#90511=CARTESIAN_POINT('Ctrl Pts',(38.3489751017513,30.2907397641919,0.));
#90512=CARTESIAN_POINT('Ctrl Pts',(38.3489751017513,30.2907397641919,20.));
#90513=CARTESIAN_POINT('Ctrl Pts',(38.3674375023871,30.2624330083488,0.));
#90514=CARTESIAN_POINT('Ctrl Pts',(38.3674375023871,30.2624330083488,20.));
#90515=CARTESIAN_POINT('Ctrl Pts',(38.3858797923318,30.2341144787313,0.));
#90516=CARTESIAN_POINT('Ctrl Pts',(38.3858797923318,30.2341144787313,20.));
#90517=CARTESIAN_POINT('Ctrl Pts',(38.4043019635603,30.2057841892317,0.));
#90518=CARTESIAN_POINT('Ctrl Pts',(38.4043019635603,30.2057841892317,20.));
#90519=CARTESIAN_POINT('Ctrl Pts',(38.4227040080549,30.1774421537519,0.));
#90520=CARTESIAN_POINT('Ctrl Pts',(38.4227040080549,30.1774421537519,20.));
#90521=CARTESIAN_POINT('Ctrl Pts',(38.4410859178038,30.1490883862047,0.));
#90522=CARTESIAN_POINT('Ctrl Pts',(38.4410859178038,30.1490883862047,20.));
#90523=CARTESIAN_POINT('Ctrl Pts',(38.4594476848032,30.1207229005118,0.));
#90524=CARTESIAN_POINT('Ctrl Pts',(38.4594476848032,30.1207229005118,20.));
#90525=CARTESIAN_POINT('Ctrl Pts',(38.4777893010568,30.0923457106027,0.));
#90526=CARTESIAN_POINT('Ctrl Pts',(38.4777893010568,30.0923457106027,20.));
#90527=CARTESIAN_POINT('Ctrl Pts',(38.4961107585777,30.0639568304126,0.));
#90528=CARTESIAN_POINT('Ctrl Pts',(38.4961107585777,30.0639568304126,20.));
#90529=CARTESIAN_POINT('Ctrl Pts',(38.5144120493894,30.0355562738816,0.));
#90530=CARTESIAN_POINT('Ctrl Pts',(38.5144120493894,30.0355562738816,20.));
#90531=CARTESIAN_POINT('Ctrl Pts',(38.532693165526,30.0071440549534,0.));
#90532=CARTESIAN_POINT('Ctrl Pts',(38.532693165526,30.0071440549534,20.));
#90533=CARTESIAN_POINT('Ctrl Pts',(38.5509540990321,29.978720187576,0.));
#90534=CARTESIAN_POINT('Ctrl Pts',(38.5509540990321,29.978720187576,20.));
#90535=CARTESIAN_POINT('Ctrl Pts',(38.5691948419622,29.9502846857025,0.));
#90536=CARTESIAN_POINT('Ctrl Pts',(38.5691948419622,29.9502846857025,20.));
#90537=CARTESIAN_POINT('Ctrl Pts',(38.5874153863803,29.9218375632918,0.));
#90538=CARTESIAN_POINT('Ctrl Pts',(38.5874153863803,29.9218375632918,20.));
#90539=CARTESIAN_POINT('Ctrl Pts',(38.6056157243597,29.8933788343089,0.));
#90540=CARTESIAN_POINT('Ctrl Pts',(38.6056157243597,29.8933788343089,20.));
#90541=CARTESIAN_POINT('Ctrl Pts',(38.6237958479822,29.864908512726,0.));
#90542=CARTESIAN_POINT('Ctrl Pts',(38.6237958479822,29.864908512726,20.));
#90543=CARTESIAN_POINT('Ctrl Pts',(38.6419557493389,29.8364266125215,0.));
#90544=CARTESIAN_POINT('Ctrl Pts',(38.6419557493389,29.8364266125215,20.));
#90545=CARTESIAN_POINT('Ctrl Pts',(38.66009542053,29.8079331476799,0.));
#90546=CARTESIAN_POINT('Ctrl Pts',(38.66009542053,29.8079331476799,20.));
#90547=CARTESIAN_POINT('Ctrl Pts',(38.6782148536649,29.7794281321916,0.));
#90548=CARTESIAN_POINT('Ctrl Pts',(38.6782148536649,29.7794281321916,20.));
#90549=CARTESIAN_POINT('Ctrl Pts',(38.6963140408627,29.7509115800524,0.));
#90550=CARTESIAN_POINT('Ctrl Pts',(38.6963140408627,29.7509115800524,20.));
#90551=CARTESIAN_POINT('Ctrl Pts',(38.7143929742521,29.7223835052637,0.));
#90552=CARTESIAN_POINT('Ctrl Pts',(38.7143929742521,29.7223835052637,20.));
#90553=CARTESIAN_POINT('Ctrl Pts',(38.7324516459718,29.6938439218325,0.));
#90554=CARTESIAN_POINT('Ctrl Pts',(38.7324516459718,29.6938439218325,20.));
#90555=CARTESIAN_POINT('Ctrl Pts',(38.7504900481697,29.6652928437714,0.));
#90556=CARTESIAN_POINT('Ctrl Pts',(38.7504900481697,29.6652928437714,20.));
#90557=CARTESIAN_POINT('Ctrl Pts',(38.7685081730036,29.6367302850988,0.));
#90558=CARTESIAN_POINT('Ctrl Pts',(38.7685081730036,29.6367302850988,20.));
#90559=CARTESIAN_POINT('Ctrl Pts',(38.7865060126402,29.6081562598384,0.));
#90560=CARTESIAN_POINT('Ctrl Pts',(38.7865060126402,29.6081562598384,20.));
#90561=CARTESIAN_POINT('Ctrl Pts',(38.8044835592559,29.5795707820205,0.));
#90562=CARTESIAN_POINT('Ctrl Pts',(38.8044835592559,29.5795707820205,20.));
#90563=CARTESIAN_POINT('Ctrl Pts',(38.8224408050366,29.5509738656807,0.));
#90564=CARTESIAN_POINT('Ctrl Pts',(38.8224408050366,29.5509738656807,20.));
#90565=CARTESIAN_POINT('Ctrl Pts',(38.8403777421773,29.5223655248609,0.));
#90566=CARTESIAN_POINT('Ctrl Pts',(38.8403777421773,29.5223655248609,20.));
#90567=CARTESIAN_POINT('Ctrl Pts',(38.8582943628826,29.4937457736083,0.));
#90568=CARTESIAN_POINT('Ctrl Pts',(38.8582943628826,29.4937457736083,20.));
#90569=CARTESIAN_POINT('Ctrl Pts',(38.8761906593666,29.4651146259764,0.));
#90570=CARTESIAN_POINT('Ctrl Pts',(38.8761906593666,29.4651146259764,20.));
#90571=CARTESIAN_POINT('Ctrl Pts',(38.8940666238532,29.4364720960241,0.));
#90572=CARTESIAN_POINT('Ctrl Pts',(38.8940666238532,29.4364720960241,20.));
#90573=CARTESIAN_POINT('Ctrl Pts',(38.9119222485755,29.4078181978158,0.));
#90574=CARTESIAN_POINT('Ctrl Pts',(38.9119222485755,29.4078181978158,20.));
#90575=CARTESIAN_POINT('Ctrl Pts',(38.9297575257761,29.3791529454216,0.));
#90576=CARTESIAN_POINT('Ctrl Pts',(38.9297575257761,29.3791529454216,20.));
#90577=CARTESIAN_POINT('Ctrl Pts',(38.9475724477072,29.3504763529173,0.));
#90578=CARTESIAN_POINT('Ctrl Pts',(38.9475724477072,29.3504763529173,20.));
#90579=CARTESIAN_POINT('Ctrl Pts',(38.9653670066308,29.3217884343845,0.));
#90580=CARTESIAN_POINT('Ctrl Pts',(38.9653670066308,29.3217884343845,20.));
#90581=CARTESIAN_POINT('Ctrl Pts',(38.9831411948182,29.2930892039104,0.));
#90582=CARTESIAN_POINT('Ctrl Pts',(38.9831411948182,29.2930892039104,20.));
#90583=CARTESIAN_POINT('Ctrl Pts',(39.0008950045502,29.2643786755883,0.));
#90584=CARTESIAN_POINT('Ctrl Pts',(39.0008950045502,29.2643786755883,20.));
#90585=CARTESIAN_POINT('Ctrl Pts',(39.0186284281173,29.2356568635168,0.));
#90586=CARTESIAN_POINT('Ctrl Pts',(39.0186284281173,29.2356568635168,20.));
#90587=CARTESIAN_POINT('Ctrl Pts',(39.0363414578191,29.2069237818005,0.));
#90588=CARTESIAN_POINT('Ctrl Pts',(39.0363414578191,29.2069237818005,20.));
#90589=CARTESIAN_POINT('Ctrl Pts',(39.054034085965,29.1781794445493,0.));
#90590=CARTESIAN_POINT('Ctrl Pts',(39.054034085965,29.1781794445493,20.));
#90591=CARTESIAN_POINT('Ctrl Pts',(39.0717063048737,29.1494238658788,0.));
#90592=CARTESIAN_POINT('Ctrl Pts',(39.0717063048737,29.1494238658788,20.));
#90593=CARTESIAN_POINT('Ctrl Pts',(39.0893581068737,29.1206570599103,0.));
#90594=CARTESIAN_POINT('Ctrl Pts',(39.0893581068737,29.1206570599103,20.));
#90595=CARTESIAN_POINT('Ctrl Pts',(39.106989484303,29.0918790407708,0.));
#90596=CARTESIAN_POINT('Ctrl Pts',(39.106989484303,29.0918790407708,20.));
#90597=CARTESIAN_POINT('Ctrl Pts',(39.1246004295092,29.0630898225929,0.));
#90598=CARTESIAN_POINT('Ctrl Pts',(39.1246004295092,29.0630898225929,20.));
#90599=CARTESIAN_POINT('Ctrl Pts',(39.1421909348497,29.034289419515,0.));
#90600=CARTESIAN_POINT('Ctrl Pts',(39.1421909348497,29.034289419515,20.));
#90601=CARTESIAN_POINT('Ctrl Pts',(39.1597609926911,29.0054778456813,0.));
#90602=CARTESIAN_POINT('Ctrl Pts',(39.1597609926911,29.0054778456813,20.));
#90603=CARTESIAN_POINT('Ctrl Pts',(39.1773105954099,28.9766551152413,0.));
#90604=CARTESIAN_POINT('Ctrl Pts',(39.1773105954099,28.9766551152413,20.));
#90605=CARTESIAN_POINT('Ctrl Pts',(39.1948397353916,28.9478212423503,0.));
#90606=CARTESIAN_POINT('Ctrl Pts',(39.1948397353916,28.9478212423503,20.));
#90607=CARTESIAN_POINT('Ctrl Pts',(39.2123484050317,28.9189762411689,0.));
#90608=CARTESIAN_POINT('Ctrl Pts',(39.2123484050317,28.9189762411689,20.));
#90609=CARTESIAN_POINT('Ctrl Pts',(39.2298365967351,28.8901201258634,0.));
#90610=CARTESIAN_POINT('Ctrl Pts',(39.2298365967351,28.8901201258634,20.));
#90611=CARTESIAN_POINT('Ctrl Pts',(39.2473043029163,28.8612529106058,0.));
#90612=CARTESIAN_POINT('Ctrl Pts',(39.2473043029163,28.8612529106058,20.));
#90613=CARTESIAN_POINT('Ctrl Pts',(39.2647515159997,28.8323746095736,0.));
#90614=CARTESIAN_POINT('Ctrl Pts',(39.2647515159997,28.8323746095736,20.));
#90615=CARTESIAN_POINT('Ctrl Pts',(39.2821782284193,28.80348523695,0.));
#90616=CARTESIAN_POINT('Ctrl Pts',(39.2821782284193,28.80348523695,20.));
#90617=CARTESIAN_POINT('Ctrl Pts',(39.2995844326181,28.7745848069238,0.));
#90618=CARTESIAN_POINT('Ctrl Pts',(39.2995844326181,28.7745848069238,20.));
#90619=CARTESIAN_POINT('Ctrl Pts',(39.316970121049,28.7456733336894,0.));
#90620=CARTESIAN_POINT('Ctrl Pts',(39.316970121049,28.7456733336894,20.));
#90621=CARTESIAN_POINT('Ctrl Pts',(39.3343352861746,28.7167508314468,0.));
#90622=CARTESIAN_POINT('Ctrl Pts',(39.3343352861746,28.7167508314468,20.));
#90623=CARTESIAN_POINT('Ctrl Pts',(39.3516799204672,28.6878173144015,0.));
#90624=CARTESIAN_POINT('Ctrl Pts',(39.3516799204672,28.6878173144015,20.));
#90625=CARTESIAN_POINT('Ctrl Pts',(39.3690040164086,28.6588727967647,0.));
#90626=CARTESIAN_POINT('Ctrl Pts',(39.3690040164086,28.6588727967647,20.));
#90627=CARTESIAN_POINT('Ctrl Pts',(39.3863075664906,28.6299172927529,0.));
#90628=CARTESIAN_POINT('Ctrl Pts',(39.3863075664906,28.6299172927529,20.));
#90629=CARTESIAN_POINT('Ctrl Pts',(39.4035905632141,28.600950816588,0.));
#90630=CARTESIAN_POINT('Ctrl Pts',(39.4035905632141,28.600950816588,20.));
#90631=CARTESIAN_POINT('Ctrl Pts',(39.4208529990894,28.5719733824975,0.));
#90632=CARTESIAN_POINT('Ctrl Pts',(39.4208529990894,28.5719733824975,20.));
#90633=CARTESIAN_POINT('Ctrl Pts',(39.4380948666368,28.5429850047148,0.));
#90634=CARTESIAN_POINT('Ctrl Pts',(39.4380948666368,28.5429850047148,20.));
#90635=CARTESIAN_POINT('Ctrl Pts',(39.4553161583861,28.5139856974786,0.));
#90636=CARTESIAN_POINT('Ctrl Pts',(39.4553161583861,28.5139856974786,20.));
#90637=CARTESIAN_POINT('Ctrl Pts',(39.472516866877,28.4849754750331,0.));
#90638=CARTESIAN_POINT('Ctrl Pts',(39.472516866877,28.4849754750331,20.));
#90639=CARTESIAN_POINT('Ctrl Pts',(39.4896969846589,28.455954351628,0.));
#90640=CARTESIAN_POINT('Ctrl Pts',(39.4896969846589,28.455954351628,20.));
#90641=CARTESIAN_POINT('Ctrl Pts',(39.5068565042907,28.4269223415187,0.));
#90642=CARTESIAN_POINT('Ctrl Pts',(39.5068565042907,28.4269223415187,20.));
#90643=CARTESIAN_POINT('Ctrl Pts',(39.5239954183412,28.3978794589661,0.));
#90644=CARTESIAN_POINT('Ctrl Pts',(39.5239954183412,28.3978794589661,20.));
#90645=CARTESIAN_POINT('Ctrl Pts',(39.5411137193887,28.3688257182364,0.));
#90646=CARTESIAN_POINT('Ctrl Pts',(39.5411137193887,28.3688257182364,20.));
#90647=CARTESIAN_POINT('Ctrl Pts',(39.5582114000212,28.3397611336014,0.));
#90648=CARTESIAN_POINT('Ctrl Pts',(39.5582114000212,28.3397611336014,20.));
#90649=CARTESIAN_POINT('Ctrl Pts',(39.5752884528361,28.3106857193381,0.));
#90650=CARTESIAN_POINT('Ctrl Pts',(39.5752884528361,28.3106857193381,20.));
#90651=CARTESIAN_POINT('Ctrl Pts',(39.5923448704403,28.2815994897291,0.));
#90652=CARTESIAN_POINT('Ctrl Pts',(39.5923448704403,28.2815994897291,20.));
#90653=CARTESIAN_POINT('Ctrl Pts',(39.6093806454502,28.2525024590626,0.));
#90654=CARTESIAN_POINT('Ctrl Pts',(39.6093806454502,28.2525024590626,20.));
#90655=CARTESIAN_POINT('Ctrl Pts',(39.6263957704923,28.2233946416323,0.));
#90656=CARTESIAN_POINT('Ctrl Pts',(39.6263957704923,28.2233946416323,20.));
#90657=CARTESIAN_POINT('Ctrl Pts',(39.6433902382029,28.1942760517371,0.));
#90658=CARTESIAN_POINT('Ctrl Pts',(39.6433902382029,28.1942760517371,20.));
#90659=CARTESIAN_POINT('Ctrl Pts',(39.6603640412281,28.1651467036817,0.));
#90660=CARTESIAN_POINT('Ctrl Pts',(39.6603640412281,28.1651467036817,20.));
#90661=CARTESIAN_POINT('Ctrl Pts',(39.6773171722241,28.136006611776,0.));
#90662=CARTESIAN_POINT('Ctrl Pts',(39.6773171722241,28.136006611776,20.));
#90663=CARTESIAN_POINT('Ctrl Pts',(39.6942496238565,28.1068557903356,0.));
#90664=CARTESIAN_POINT('Ctrl Pts',(39.6942496238565,28.1068557903356,20.));
#90665=CARTESIAN_POINT('Ctrl Pts',(39.7111613888006,28.0776942536814,0.));
#90666=CARTESIAN_POINT('Ctrl Pts',(39.7111613888006,28.0776942536814,20.));
#90667=CARTESIAN_POINT('Ctrl Pts',(39.728052459741,28.0485220161395,0.));
#90668=CARTESIAN_POINT('Ctrl Pts',(39.728052459741,28.0485220161395,20.));
#90669=CARTESIAN_POINT('Ctrl Pts',(39.7449228293718,28.0193390920415,0.));
#90670=CARTESIAN_POINT('Ctrl Pts',(39.7449228293718,28.0193390920415,20.));
#90671=CARTESIAN_POINT('Ctrl Pts',(39.7617724903968,27.9901454957246,0.));
#90672=CARTESIAN_POINT('Ctrl Pts',(39.7617724903968,27.9901454957246,20.));
#90673=CARTESIAN_POINT('Ctrl Pts',(39.7786014355293,27.960941241531,0.));
#90674=CARTESIAN_POINT('Ctrl Pts',(39.7786014355293,27.960941241531,20.));
#90675=CARTESIAN_POINT('Ctrl Pts',(39.795409657493,27.9317263438086,0.));
#90676=CARTESIAN_POINT('Ctrl Pts',(39.795409657493,27.9317263438086,20.));
#90677=CARTESIAN_POINT('Ctrl Pts',(39.8121971490214,27.9025008169107,0.));
#90678=CARTESIAN_POINT('Ctrl Pts',(39.8121971490214,27.9025008169107,20.));
#90679=CARTESIAN_POINT('Ctrl Pts',(39.828963902858,27.8732646751959,0.));
#90680=CARTESIAN_POINT('Ctrl Pts',(39.828963902858,27.8732646751959,20.));
#90681=CARTESIAN_POINT('Ctrl Pts',(39.8457099117559,27.8440179330284,0.));
#90682=CARTESIAN_POINT('Ctrl Pts',(39.8457099117559,27.8440179330284,20.));
#90683=CARTESIAN_POINT('Ctrl Pts',(39.862435168478,27.8147606047778,0.));
#90684=CARTESIAN_POINT('Ctrl Pts',(39.862435168478,27.8147606047778,20.));
#90685=CARTESIAN_POINT('Ctrl Pts',(39.8791396657966,27.785492704819,0.));
#90686=CARTESIAN_POINT('Ctrl Pts',(39.8791396657966,27.785492704819,20.));
#90687=CARTESIAN_POINT('Ctrl Pts',(39.8958233964934,27.7562142475319,0.));
#90688=CARTESIAN_POINT('Ctrl Pts',(39.8958233964934,27.7562142475319,20.));
#90689=CARTESIAN_POINT('Ctrl Pts',(39.9124863533599,27.726925247302,0.));
#90690=CARTESIAN_POINT('Ctrl Pts',(39.9124863533599,27.726925247302,20.));
#90691=CARTESIAN_POINT('Ctrl Pts',(39.9291285291975,27.6976257185198,0.));
#90692=CARTESIAN_POINT('Ctrl Pts',(39.9291285291975,27.6976257185198,20.));
#90693=CARTESIAN_POINT('Ctrl Pts',(39.9457499168175,27.6683156755815,0.));
#90694=CARTESIAN_POINT('Ctrl Pts',(39.9457499168175,27.6683156755815,20.));
#90695=CARTESIAN_POINT('Ctrl Pts',(39.9623505090412,27.6389951328887,0.));
#90696=CARTESIAN_POINT('Ctrl Pts',(39.9623505090412,27.6389951328887,20.));
#90697=CARTESIAN_POINT('Ctrl Pts',(39.9789302986995,27.6096641048483,0.));
#90698=CARTESIAN_POINT('Ctrl Pts',(39.9789302986995,27.6096641048483,20.));
#90699=CARTESIAN_POINT('Ctrl Pts',(39.9954892786331,27.5803226058725,0.));
#90700=CARTESIAN_POINT('Ctrl Pts',(39.9954892786331,27.5803226058725,20.));
#90701=CARTESIAN_POINT('Ctrl Pts',(40.0120274416924,27.5509706503786,0.));
#90702=CARTESIAN_POINT('Ctrl Pts',(40.0120274416924,27.5509706503786,20.));
#90703=CARTESIAN_POINT('Ctrl Pts',(40.0285447807378,27.5216082527897,0.));
#90704=CARTESIAN_POINT('Ctrl Pts',(40.0285447807378,27.5216082527897,20.));
#90705=CARTESIAN_POINT('Ctrl Pts',(40.045041288639,27.4922354275335,0.));
#90706=CARTESIAN_POINT('Ctrl Pts',(40.045041288639,27.4922354275335,20.));
#90707=CARTESIAN_POINT('Ctrl Pts',(40.0615169582759,27.4628521890436,0.));
#90708=CARTESIAN_POINT('Ctrl Pts',(40.0615169582759,27.4628521890436,20.));
#90709=CARTESIAN_POINT('Ctrl Pts',(40.077971782538,27.4334585517582,0.));
#90710=CARTESIAN_POINT('Ctrl Pts',(40.077971782538,27.4334585517582,20.));
#90711=CARTESIAN_POINT('Ctrl Pts',(40.0944057543248,27.4040545301216,0.));
#90712=CARTESIAN_POINT('Ctrl Pts',(40.0944057543248,27.4040545301216,20.));
#90713=CARTESIAN_POINT('Ctrl Pts',(40.1108188665452,27.374640138583,0.));
#90714=CARTESIAN_POINT('Ctrl Pts',(40.1108188665452,27.374640138583,20.));
#90715=CARTESIAN_POINT('Ctrl Pts',(40.1272111121183,27.3452153915969,0.));
#90716=CARTESIAN_POINT('Ctrl Pts',(40.1272111121183,27.3452153915969,20.));
#90717=CARTESIAN_POINT('Ctrl Pts',(40.1435824839731,27.3157803036231,0.));
#90718=CARTESIAN_POINT('Ctrl Pts',(40.1435824839731,27.3157803036231,20.));
#90719=CARTESIAN_POINT('Ctrl Pts',(40.1599329750483,27.2863348891265,0.));
#90720=CARTESIAN_POINT('Ctrl Pts',(40.1599329750483,27.2863348891265,20.));
#90721=CARTESIAN_POINT('Ctrl Pts',(40.1762625782924,27.2568791625774,0.));
#90722=CARTESIAN_POINT('Ctrl Pts',(40.1762625782924,27.2568791625774,20.));
#90723=CARTESIAN_POINT('Ctrl Pts',(40.1925712866631,27.2274131384508,0.));
#90724=CARTESIAN_POINT('Ctrl Pts',(40.1925712866631,27.2274131384508,20.));
#90725=CARTESIAN_POINT('Ctrl Pts',(40.2088590931287,27.1979368312277,0.));
#90726=CARTESIAN_POINT('Ctrl Pts',(40.2088590931287,27.1979368312277,20.));
#90727=CARTESIAN_POINT('Ctrl Pts',(40.2251259906669,27.1684502553939,0.));
#90728=CARTESIAN_POINT('Ctrl Pts',(40.2251259906669,27.1684502553939,20.));
#90729=CARTESIAN_POINT('Ctrl Pts',(40.2413719722657,27.1389534254409,0.));
#90730=CARTESIAN_POINT('Ctrl Pts',(40.2413719722657,27.1389534254409,20.));
#90731=CARTESIAN_POINT('Ctrl Pts',(40.2575970309226,27.1094463558649,0.));
#90732=CARTESIAN_POINT('Ctrl Pts',(40.2575970309226,27.1094463558649,20.));
#90733=CARTESIAN_POINT('Ctrl Pts',(40.2738011596454,27.0799290611676,0.));
#90734=CARTESIAN_POINT('Ctrl Pts',(40.2738011596454,27.0799290611676,20.));
#90735=CARTESIAN_POINT('Ctrl Pts',(40.2899843514517,27.0504015558557,0.));
#90736=CARTESIAN_POINT('Ctrl Pts',(40.2899843514517,27.0504015558557,20.));
#90737=CARTESIAN_POINT('Ctrl Pts',(40.3061465993685,27.0208638544413,0.));
#90738=CARTESIAN_POINT('Ctrl Pts',(40.3061465993685,27.0208638544413,20.));
#90739=CARTESIAN_POINT('Ctrl Pts',(40.3222878964329,26.9913159714415,0.));
#90740=CARTESIAN_POINT('Ctrl Pts',(40.3222878964329,26.9913159714415,20.));
#90741=CARTESIAN_POINT('Ctrl Pts',(40.3384082356913,26.9617579213786,0.));
#90742=CARTESIAN_POINT('Ctrl Pts',(40.3384082356913,26.9617579213786,20.));
#90743=CARTESIAN_POINT('Ctrl Pts',(40.3545076102003,26.9321897187802,0.));
#90744=CARTESIAN_POINT('Ctrl Pts',(40.3545076102003,26.9321897187802,20.));
#90745=CARTESIAN_POINT('Ctrl Pts',(40.3705860130263,26.9026113781788,0.));
#90746=CARTESIAN_POINT('Ctrl Pts',(40.3705860130263,26.9026113781788,20.));
#90747=CARTESIAN_POINT('Ctrl Pts',(40.386643437246,26.8730229141124,0.));
#90748=CARTESIAN_POINT('Ctrl Pts',(40.386643437246,26.8730229141124,20.));
#90749=CARTESIAN_POINT('Ctrl Pts',(40.4026798759458,26.8434243411241,0.));
#90750=CARTESIAN_POINT('Ctrl Pts',(40.4026798759458,26.8434243411241,20.));
#90751=CARTESIAN_POINT('Ctrl Pts',(40.4186953222224,26.8138156737619,0.));
#90752=CARTESIAN_POINT('Ctrl Pts',(40.4186953222224,26.8138156737619,20.));
#90753=CARTESIAN_POINT('Ctrl Pts',(40.4346897691821,26.7841969265794,0.));
#90754=CARTESIAN_POINT('Ctrl Pts',(40.4346897691821,26.7841969265794,20.));
#90755=CARTESIAN_POINT('Ctrl Pts',(40.4506632099408,26.754568114135,0.));
#90756=CARTESIAN_POINT('Ctrl Pts',(40.4506632099408,26.754568114135,20.));
#90757=CARTESIAN_POINT('Ctrl Pts',(40.4666156376241,26.7249292509923,0.));
#90758=CARTESIAN_POINT('Ctrl Pts',(40.4666156376241,26.7249292509923,20.));
#90759=CARTESIAN_POINT('Ctrl Pts',(40.4825470453679,26.6952803517197,0.));
#90760=CARTESIAN_POINT('Ctrl Pts',(40.4825470453679,26.6952803517197,20.));
#90761=CARTESIAN_POINT('Ctrl Pts',(40.4984574263178,26.6656214308914,0.));
#90762=CARTESIAN_POINT('Ctrl Pts',(40.4984574263178,26.6656214308914,20.));
#90763=CARTESIAN_POINT('Ctrl Pts',(40.5143467736295,26.6359525030862,0.));
#90764=CARTESIAN_POINT('Ctrl Pts',(40.5143467736295,26.6359525030862,20.));
#90765=CARTESIAN_POINT('Ctrl Pts',(40.5302150804687,26.606273582888,0.));
#90766=CARTESIAN_POINT('Ctrl Pts',(40.5302150804687,26.606273582888,20.));
#90767=CARTESIAN_POINT('Ctrl Pts',(40.546062340011,26.5765846848862,0.));
#90768=CARTESIAN_POINT('Ctrl Pts',(40.546062340011,26.5765846848862,20.));
#90769=CARTESIAN_POINT('Ctrl Pts',(40.5618885454414,26.5468858236748,0.));
#90770=CARTESIAN_POINT('Ctrl Pts',(40.5618885454414,26.5468858236748,20.));
#90771=CARTESIAN_POINT('Ctrl Pts',(40.5776936899555,26.5171770138532,0.));
#90772=CARTESIAN_POINT('Ctrl Pts',(40.5776936899555,26.5171770138532,20.));
#90773=CARTESIAN_POINT('Ctrl Pts',(40.5934777667583,26.4874582700259,0.));
#90774=CARTESIAN_POINT('Ctrl Pts',(40.5934777667583,26.4874582700259,20.));
#90775=CARTESIAN_POINT('Ctrl Pts',(40.6092407690651,26.4577296068023,0.));
#90776=CARTESIAN_POINT('Ctrl Pts',(40.6092407690651,26.4577296068023,20.));
#90777=CARTESIAN_POINT('Ctrl Pts',(40.6249826901011,26.4279910387971,0.));
#90778=CARTESIAN_POINT('Ctrl Pts',(40.6249826901011,26.4279910387971,20.));
#90779=CARTESIAN_POINT('Ctrl Pts',(40.6407035231015,26.3982425806297,0.));
#90780=CARTESIAN_POINT('Ctrl Pts',(40.6407035231015,26.3982425806297,20.));
#90781=CARTESIAN_POINT('Ctrl Pts',(40.6564032613109,26.3684842469248,0.));
#90782=CARTESIAN_POINT('Ctrl Pts',(40.6564032613109,26.3684842469248,20.));
#90783=CARTESIAN_POINT('Ctrl Pts',(40.6720818979844,26.338716052312,0.));
#90784=CARTESIAN_POINT('Ctrl Pts',(40.6720818979844,26.338716052312,20.));
#90785=CARTESIAN_POINT('Ctrl Pts',(40.6877394263869,26.308938011426,0.));
#90786=CARTESIAN_POINT('Ctrl Pts',(40.6877394263869,26.308938011426,20.));
#90787=CARTESIAN_POINT('Ctrl Pts',(40.7033758397932,26.2791501389067,0.));
#90788=CARTESIAN_POINT('Ctrl Pts',(40.7033758397932,26.2791501389067,20.));
#90789=CARTESIAN_POINT('Ctrl Pts',(40.7189911314882,26.2493524493989,0.));
#90790=CARTESIAN_POINT('Ctrl Pts',(40.7189911314882,26.2493524493989,20.));
#90791=CARTESIAN_POINT('Ctrl Pts',(40.7345852947663,26.2195449575524,0.));
#90792=CARTESIAN_POINT('Ctrl Pts',(40.7345852947663,26.2195449575524,20.));
#90793=CARTESIAN_POINT('Ctrl Pts',(40.7501583229328,26.1897276780219,0.));
#90794=CARTESIAN_POINT('Ctrl Pts',(40.7501583229328,26.1897276780219,20.));
#90795=CARTESIAN_POINT('Ctrl Pts',(40.7657102093021,26.1599006254674,0.));
#90796=CARTESIAN_POINT('Ctrl Pts',(40.7657102093021,26.1599006254674,20.));
#90797=CARTESIAN_POINT('Ctrl Pts',(40.7812409471992,26.1300638145535,0.));
#90798=CARTESIAN_POINT('Ctrl Pts',(40.7812409471992,26.1300638145535,20.));
#90799=CARTESIAN_POINT('Ctrl Pts',(40.7967505299588,26.1002172599501,0.));
#90800=CARTESIAN_POINT('Ctrl Pts',(40.7967505299588,26.1002172599501,20.));
#90801=CARTESIAN_POINT('Ctrl Pts',(40.8122389509256,26.0703609763318,0.));
#90802=CARTESIAN_POINT('Ctrl Pts',(40.8122389509256,26.0703609763318,20.));
#90803=CARTESIAN_POINT('Ctrl Pts',(40.8277062034539,26.0404949783787,0.));
#90804=CARTESIAN_POINT('Ctrl Pts',(40.8277062034539,26.0404949783787,20.));
#90805=CARTESIAN_POINT('Ctrl Pts',(40.843152280908,26.0106192807756,0.));
#90806=CARTESIAN_POINT('Ctrl Pts',(40.843152280908,26.0106192807756,20.));
#90807=CARTESIAN_POINT('Ctrl Pts',(40.8585771766627,25.9807338982121,0.));
#90808=CARTESIAN_POINT('Ctrl Pts',(40.8585771766627,25.9807338982121,20.));
#90809=CARTESIAN_POINT('Ctrl Pts',(40.8739808841024,25.9508388453831,0.));
#90810=CARTESIAN_POINT('Ctrl Pts',(40.8739808841024,25.9508388453831,20.));
#90811=CARTESIAN_POINT('Ctrl Pts',(40.8893633966224,25.9209341369879,0.));
#90812=CARTESIAN_POINT('Ctrl Pts',(40.8893633966224,25.9209341369879,20.));
#90813=CARTESIAN_POINT('Ctrl Pts',(40.9047247076274,25.891019787731,0.));
#90814=CARTESIAN_POINT('Ctrl Pts',(40.9047247076274,25.891019787731,20.));
#90815=CARTESIAN_POINT('Ctrl Pts',(40.9200648105322,25.861095812322,0.));
#90816=CARTESIAN_POINT('Ctrl Pts',(40.9200648105322,25.861095812322,20.));
#90817=CARTESIAN_POINT('Ctrl Pts',(40.9353836987613,25.8311622254754,0.));
#90818=CARTESIAN_POINT('Ctrl Pts',(40.9353836987613,25.8311622254754,20.));
#90819=CARTESIAN_POINT('Ctrl Pts',(40.9506813657491,25.8012190419102,0.));
#90820=CARTESIAN_POINT('Ctrl Pts',(40.9506813657491,25.8012190419102,20.));
#90821=CARTESIAN_POINT('Ctrl Pts',(40.9659578049399,25.7712662763511,0.));
#90822=CARTESIAN_POINT('Ctrl Pts',(40.9659578049399,25.7712662763511,20.));
#90823=CARTESIAN_POINT('Ctrl Pts',(40.981213009789,25.7413039435271,0.));
#90824=CARTESIAN_POINT('Ctrl Pts',(40.981213009789,25.7413039435271,20.));
#90825=CARTESIAN_POINT('Ctrl Pts',(40.9964469737612,25.7113320581728,0.));
#90826=CARTESIAN_POINT('Ctrl Pts',(40.9964469737612,25.7113320581728,20.));
#90827=CARTESIAN_POINT('Ctrl Pts',(41.0116596903316,25.6813506350271,0.));
#90828=CARTESIAN_POINT('Ctrl Pts',(41.0116596903316,25.6813506350271,20.));
#90829=CARTESIAN_POINT('Ctrl Pts',(41.0268511529852,25.6513596888338,0.));
#90830=CARTESIAN_POINT('Ctrl Pts',(41.0268511529852,25.6513596888338,20.));
#90831=CARTESIAN_POINT('Ctrl Pts',(41.0420213552163,25.6213592343415,0.));
#90832=CARTESIAN_POINT('Ctrl Pts',(41.0420213552163,25.6213592343415,20.));
#90833=CARTESIAN_POINT('Ctrl Pts',(41.05717029053,25.5913492863038,0.));
#90834=CARTESIAN_POINT('Ctrl Pts',(41.05717029053,25.5913492863038,20.));
#90835=CARTESIAN_POINT('Ctrl Pts',(41.072297952441,25.5613298594791,0.));
#90836=CARTESIAN_POINT('Ctrl Pts',(41.072297952441,25.5613298594791,20.));
#90837=CARTESIAN_POINT('Ctrl Pts',(41.0874043344745,25.5313009686309,0.));
#90838=CARTESIAN_POINT('Ctrl Pts',(41.0874043344745,25.5313009686309,20.));
#90839=CARTESIAN_POINT('Ctrl Pts',(41.1024894301655,25.5012626285275,0.));
#90840=CARTESIAN_POINT('Ctrl Pts',(41.1024894301655,25.5012626285275,20.));
#90841=CARTESIAN_POINT('Ctrl Pts',(41.1175532330596,25.4712148539422,0.));
#90842=CARTESIAN_POINT('Ctrl Pts',(41.1175532330596,25.4712148539422,20.));
#90843=CARTESIAN_POINT('Ctrl Pts',(41.1325957367119,25.4411576596529,0.));
#90844=CARTESIAN_POINT('Ctrl Pts',(41.1325957367119,25.4411576596529,20.));
#90845=CARTESIAN_POINT('Ctrl Pts',(41.1476169346881,25.4110910604425,0.));
#90846=CARTESIAN_POINT('Ctrl Pts',(41.1476169346881,25.4110910604425,20.));
#90847=CARTESIAN_POINT('Ctrl Pts',(41.1626168205634,25.3810150710984,0.));
#90848=CARTESIAN_POINT('Ctrl Pts',(41.1626168205634,25.3810150710984,20.));
#90849=CARTESIAN_POINT('Ctrl Pts',(41.1775953879232,25.3509297064131,0.));
#90850=CARTESIAN_POINT('Ctrl Pts',(41.1775953879232,25.3509297064131,20.));
#90851=CARTESIAN_POINT('Ctrl Pts',(41.1925526303629,25.3208349811839,0.));
#90852=CARTESIAN_POINT('Ctrl Pts',(41.1925526303629,25.3208349811839,20.));
#90853=CARTESIAN_POINT('Ctrl Pts',(41.2074885414881,25.2907309102128,0.));
#90854=CARTESIAN_POINT('Ctrl Pts',(41.2074885414881,25.2907309102128,20.));
#90855=CARTESIAN_POINT('Ctrl Pts',(41.2224031149147,25.2606175083067,0.));
#90856=CARTESIAN_POINT('Ctrl Pts',(41.2224031149147,25.2606175083067,20.));
#90857=CARTESIAN_POINT('Ctrl Pts',(41.2372963442684,25.2304947902774,0.));
#90858=CARTESIAN_POINT('Ctrl Pts',(41.2372963442684,25.2304947902774,20.));
#90859=CARTESIAN_POINT('Ctrl Pts',(41.2521682231854,25.2003627709414,0.));
#90860=CARTESIAN_POINT('Ctrl Pts',(41.2521682231854,25.2003627709414,20.));
#90861=CARTESIAN_POINT('Ctrl Pts',(41.2670187453114,25.1702214651198,0.));
#90862=CARTESIAN_POINT('Ctrl Pts',(41.2670187453114,25.1702214651198,20.));
#90863=CARTESIAN_POINT('Ctrl Pts',(41.2818479043026,25.1400708876386,0.));
#90864=CARTESIAN_POINT('Ctrl Pts',(41.2818479043026,25.1400708876386,20.));
#90865=CARTESIAN_POINT('Ctrl Pts',(41.2966556938255,25.1099110533288,0.));
#90866=CARTESIAN_POINT('Ctrl Pts',(41.2966556938255,25.1099110533288,20.));
#90867=CARTESIAN_POINT('Ctrl Pts',(41.3114421075567,25.0797419770258,0.));
#90868=CARTESIAN_POINT('Ctrl Pts',(41.3114421075567,25.0797419770258,20.));
#90869=CARTESIAN_POINT('Ctrl Pts',(41.3262071391823,25.0495636735701,0.));
#90870=CARTESIAN_POINT('Ctrl Pts',(41.3262071391823,25.0495636735701,20.));
#90871=CARTESIAN_POINT('Ctrl Pts',(41.3409507823989,25.0193761578067,0.));
#90872=CARTESIAN_POINT('Ctrl Pts',(41.3409507823989,25.0193761578067,20.));
#90873=CARTESIAN_POINT('Ctrl Pts',(41.3556730309131,24.9891794445855,0.));
#90874=CARTESIAN_POINT('Ctrl Pts',(41.3556730309131,24.9891794445855,20.));
#90875=CARTESIAN_POINT('Ctrl Pts',(41.3703738784418,24.9589735487609,0.));
#90876=CARTESIAN_POINT('Ctrl Pts',(41.3703738784418,24.9589735487609,20.));
#90877=CARTESIAN_POINT('Ctrl Pts',(41.3850533187123,24.9287584851923,0.));
#90878=CARTESIAN_POINT('Ctrl Pts',(41.3850533187123,24.9287584851923,20.));
#90879=CARTESIAN_POINT('Ctrl Pts',(41.3997113454618,24.8985342687436,0.));
#90880=CARTESIAN_POINT('Ctrl Pts',(41.3997113454618,24.8985342687436,20.));
#90881=CARTESIAN_POINT('Ctrl Pts',(41.4143479524375,24.8683009142837,0.));
#90882=CARTESIAN_POINT('Ctrl Pts',(41.4143479524375,24.8683009142837,20.));
#90883=CARTESIAN_POINT('Ctrl Pts',(41.4289631333969,24.8380584366859,0.));
#90884=CARTESIAN_POINT('Ctrl Pts',(41.4289631333969,24.8380584366859,20.));
#90885=CARTESIAN_POINT('Ctrl Pts',(41.443556882107,24.8078068508284,0.));
#90886=CARTESIAN_POINT('Ctrl Pts',(41.443556882107,24.8078068508284,20.));
#90887=CARTESIAN_POINT('Ctrl Pts',(41.4581291923457,24.7775461715943,0.));
#90888=CARTESIAN_POINT('Ctrl Pts',(41.4581291923457,24.7775461715943,20.));
#90889=CARTESIAN_POINT('Ctrl Pts',(41.4726800579006,24.7472764138709,0.));
#90890=CARTESIAN_POINT('Ctrl Pts',(41.4726800579006,24.7472764138709,20.));
#90891=CARTESIAN_POINT('Ctrl Pts',(41.4872094725701,24.7169975925505,0.));
#90892=CARTESIAN_POINT('Ctrl Pts',(41.4872094725701,24.7169975925505,20.));
#90893=CARTESIAN_POINT('Ctrl Pts',(41.5017174301628,24.68670972253,0.));
#90894=CARTESIAN_POINT('Ctrl Pts',(41.5017174301628,24.68670972253,20.));
#90895=CARTESIAN_POINT('Ctrl Pts',(41.516203924497,24.6564128187107,0.));
#90896=CARTESIAN_POINT('Ctrl Pts',(41.516203924497,24.6564128187107,20.));
#90897=CARTESIAN_POINT('Ctrl Pts',(41.5306689494012,24.626106895999,0.));
#90898=CARTESIAN_POINT('Ctrl Pts',(41.5306689494012,24.626106895999,20.));
#90899=CARTESIAN_POINT('Ctrl Pts',(41.545112498714,24.5957919693057,0.));
#90900=CARTESIAN_POINT('Ctrl Pts',(41.545112498714,24.5957919693057,20.));
#90901=CARTESIAN_POINT('Ctrl Pts',(41.5595345662842,24.5654680535465,0.));
#90902=CARTESIAN_POINT('Ctrl Pts',(41.5595345662842,24.5654680535465,20.));
#90903=CARTESIAN_POINT('Ctrl Pts',(41.5739351459709,24.5351351636416,0.));
#90904=CARTESIAN_POINT('Ctrl Pts',(41.5739351459709,24.5351351636416,20.));
#90905=CARTESIAN_POINT('Ctrl Pts',(41.5883142316433,24.5047933145158,0.));
#90906=CARTESIAN_POINT('Ctrl Pts',(41.5883142316433,24.5047933145158,20.));
#90907=CARTESIAN_POINT('Ctrl Pts',(41.6026718171809,24.4744425210985,0.));
#90908=CARTESIAN_POINT('Ctrl Pts',(41.6026718171809,24.4744425210985,20.));
#90909=CARTESIAN_POINT('Ctrl Pts',(41.6170078964732,24.4440827983238,0.));
#90910=CARTESIAN_POINT('Ctrl Pts',(41.6170078964732,24.4440827983238,20.));
#90911=CARTESIAN_POINT('Ctrl Pts',(41.6313224634201,24.4137141611302,0.));
#90912=CARTESIAN_POINT('Ctrl Pts',(41.6313224634201,24.4137141611302,20.));
#90913=CARTESIAN_POINT('Ctrl Pts',(41.6456155119319,24.3833366244611,0.));
#90914=CARTESIAN_POINT('Ctrl Pts',(41.6456155119319,24.3833366244611,20.));
#90915=CARTESIAN_POINT('Ctrl Pts',(41.6598870359289,24.3529502032644,0.));
#90916=CARTESIAN_POINT('Ctrl Pts',(41.6598870359289,24.3529502032644,20.));
#90917=CARTESIAN_POINT('Ctrl Pts',(41.6741370293416,24.3225549124927,0.));
#90918=CARTESIAN_POINT('Ctrl Pts',(41.6741370293416,24.3225549124927,20.));
#90919=CARTESIAN_POINT('Ctrl Pts',(41.6883654861106,24.292150767103,0.));
#90920=CARTESIAN_POINT('Ctrl Pts',(41.6883654861106,24.292150767103,20.));
#90921=CARTESIAN_POINT('Ctrl Pts',(41.7025724001866,24.2617377820568,0.));
#90922=CARTESIAN_POINT('Ctrl Pts',(41.7025724001866,24.2617377820568,20.));
#90923=CARTESIAN_POINT('Ctrl Pts',(41.7167577655309,24.2313159723205,0.));
#90924=CARTESIAN_POINT('Ctrl Pts',(41.7167577655309,24.2313159723205,20.));
#90925=CARTESIAN_POINT('Ctrl Pts',(41.7309215761147,24.2008853528648,0.));
#90926=CARTESIAN_POINT('Ctrl Pts',(41.7309215761147,24.2008853528648,20.));
#90927=CARTESIAN_POINT('Ctrl Pts',(41.7450638259196,24.1704459386651,0.));
#90928=CARTESIAN_POINT('Ctrl Pts',(41.7450638259196,24.1704459386651,20.));
#90929=CARTESIAN_POINT('Ctrl Pts',(41.7591845089374,24.1399977447013,0.));
#90930=CARTESIAN_POINT('Ctrl Pts',(41.7591845089374,24.1399977447013,20.));
#90931=CARTESIAN_POINT('Ctrl Pts',(41.7732836191701,24.1095407859578,0.));
#90932=CARTESIAN_POINT('Ctrl Pts',(41.7732836191701,24.1095407859578,20.));
#90933=CARTESIAN_POINT('Ctrl Pts',(41.78736115063,24.0790750774236,0.));
#90934=CARTESIAN_POINT('Ctrl Pts',(41.78736115063,24.0790750774236,20.));
#90935=CARTESIAN_POINT('Ctrl Pts',(41.8014170973399,24.0486006340924,0.));
#90936=CARTESIAN_POINT('Ctrl Pts',(41.8014170973399,24.0486006340924,20.));
#90937=CARTESIAN_POINT('Ctrl Pts',(41.8154514533324,24.0181174709622,0.));
#90938=CARTESIAN_POINT('Ctrl Pts',(41.8154514533324,24.0181174709622,20.));
#90939=CARTESIAN_POINT('Ctrl Pts',(41.8294642126506,23.9876256030355,0.));
#90940=CARTESIAN_POINT('Ctrl Pts',(41.8294642126506,23.9876256030355,20.));
#90941=CARTESIAN_POINT('Ctrl Pts',(41.8434553693478,23.9571250453194,0.));
#90942=CARTESIAN_POINT('Ctrl Pts',(41.8434553693478,23.9571250453194,20.));
#90943=CARTESIAN_POINT('Ctrl Pts',(41.8574249174873,23.9266158128252,0.));
#90944=CARTESIAN_POINT('Ctrl Pts',(41.8574249174873,23.9266158128252,20.));
#90945=CARTESIAN_POINT('Ctrl Pts',(41.8713728511429,23.8960979205694,0.));
#90946=CARTESIAN_POINT('Ctrl Pts',(41.8713728511429,23.8960979205694,20.));
#90947=CARTESIAN_POINT('Ctrl Pts',(41.8852991643986,23.8655713835725,0.));
#90948=CARTESIAN_POINT('Ctrl Pts',(41.8852991643986,23.8655713835725,20.));
#90949=CARTESIAN_POINT('Ctrl Pts',(41.8992038513488,23.8350362168598,0.));
#90950=CARTESIAN_POINT('Ctrl Pts',(41.8992038513488,23.8350362168598,20.));
#90951=CARTESIAN_POINT('Ctrl Pts',(41.9130869060982,23.8044924354607,0.));
#90952=CARTESIAN_POINT('Ctrl Pts',(41.9130869060982,23.8044924354607,20.));
#90953=CARTESIAN_POINT('Ctrl Pts',(41.9269483227618,23.7739400544092,0.));
#90954=CARTESIAN_POINT('Ctrl Pts',(41.9269483227618,23.7739400544092,20.));
#90955=CARTESIAN_POINT('Ctrl Pts',(41.9407880954647,23.7433790887435,0.));
#90956=CARTESIAN_POINT('Ctrl Pts',(41.9407880954647,23.7433790887435,20.));
#90957=CARTESIAN_POINT('Ctrl Pts',(41.9546062183422,23.7128095535066,0.));
#90958=CARTESIAN_POINT('Ctrl Pts',(41.9546062183422,23.7128095535066,20.));
#90959=CARTESIAN_POINT('Ctrl Pts',(41.9684026855399,23.6822314637457,0.));
#90960=CARTESIAN_POINT('Ctrl Pts',(41.9684026855399,23.6822314637457,20.));
#90961=CARTESIAN_POINT('Ctrl Pts',(41.9821774912141,23.651644834513,0.));
#90962=CARTESIAN_POINT('Ctrl Pts',(41.9821774912141,23.651644834513,20.));
#90963=CARTESIAN_POINT('Ctrl Pts',(41.9959306295311,23.6210496808648,0.));
#90964=CARTESIAN_POINT('Ctrl Pts',(41.9959306295311,23.6210496808648,20.));
#90965=CARTESIAN_POINT('Ctrl Pts',(42.0096620946675,23.5904460178619,0.));
#90966=CARTESIAN_POINT('Ctrl Pts',(42.0096620946675,23.5904460178619,20.));
#90967=CARTESIAN_POINT('Ctrl Pts',(42.02337188081,23.5598338605694,0.));
#90968=CARTESIAN_POINT('Ctrl Pts',(42.02337188081,23.5598338605694,20.));
#90969=CARTESIAN_POINT('Ctrl Pts',(42.0370599821558,23.5292132240567,0.));
#90970=CARTESIAN_POINT('Ctrl Pts',(42.0370599821558,23.5292132240567,20.));
#90971=CARTESIAN_POINT('Ctrl Pts',(42.0507263929126,23.4985841233977,0.));
#90972=CARTESIAN_POINT('Ctrl Pts',(42.0507263929126,23.4985841233977,20.));
#90973=CARTESIAN_POINT('Ctrl Pts',(42.0643711072981,23.4679465736707,0.));
#90974=CARTESIAN_POINT('Ctrl Pts',(42.0643711072981,23.4679465736707,20.));
#90975=CARTESIAN_POINT('Ctrl Pts',(42.0779941195407,23.4373005899585,0.));
#90976=CARTESIAN_POINT('Ctrl Pts',(42.0779941195407,23.4373005899585,20.));
#90977=CARTESIAN_POINT('Ctrl Pts',(42.0915954238788,23.4066461873484,0.));
#90978=CARTESIAN_POINT('Ctrl Pts',(42.0915954238788,23.4066461873484,20.));
#90979=CARTESIAN_POINT('Ctrl Pts',(42.1051750145614,23.3759833809318,0.));
#90980=CARTESIAN_POINT('Ctrl Pts',(42.1051750145614,23.3759833809318,20.));
#90981=CARTESIAN_POINT('Ctrl Pts',(42.1187328858474,23.3453121858047,0.));
#90982=CARTESIAN_POINT('Ctrl Pts',(42.1187328858474,23.3453121858047,20.));
#90983=CARTESIAN_POINT('Ctrl Pts',(42.1322690320059,23.3146326170671,0.));
#90984=CARTESIAN_POINT('Ctrl Pts',(42.1322690320059,23.3146326170671,20.));
#90985=CARTESIAN_POINT('Ctrl Pts',(42.1457834473169,23.2839446898238,0.));
#90986=CARTESIAN_POINT('Ctrl Pts',(42.1457834473169,23.2839446898238,20.));
#90987=CARTESIAN_POINT('Ctrl Pts',(42.1592761260708,23.2532484191837,0.));
#90988=CARTESIAN_POINT('Ctrl Pts',(42.1592761260708,23.2532484191837,20.));
#90989=CARTESIAN_POINT('Ctrl Pts',(42.1727470625681,23.2225438202604,0.));
#90990=CARTESIAN_POINT('Ctrl Pts',(42.1727470625681,23.2225438202604,20.));
#90991=CARTESIAN_POINT('Ctrl Pts',(42.1861962511195,23.1918309081713,0.));
#90992=CARTESIAN_POINT('Ctrl Pts',(42.1861962511195,23.1918309081713,20.));
#90993=CARTESIAN_POINT('Ctrl Pts',(42.1996236860461,23.1611096980384,0.));
#90994=CARTESIAN_POINT('Ctrl Pts',(42.1996236860461,23.1611096980384,20.));
#90995=CARTESIAN_POINT('Ctrl Pts',(42.2130293616794,23.1303802049881,0.));
#90996=CARTESIAN_POINT('Ctrl Pts',(42.2130293616794,23.1303802049881,20.));
#90997=CARTESIAN_POINT('Ctrl Pts',(42.2264132723611,23.0996424441509,0.));
#90998=CARTESIAN_POINT('Ctrl Pts',(42.2264132723611,23.0996424441509,20.));
#90999=CARTESIAN_POINT('Ctrl Pts',(42.2397754124437,23.0688964306618,0.));
#91000=CARTESIAN_POINT('Ctrl Pts',(42.2397754124437,23.0688964306618,20.));
#91001=CARTESIAN_POINT('Ctrl Pts',(42.2531157762897,23.0381421796601,0.));
#91002=CARTESIAN_POINT('Ctrl Pts',(42.2531157762897,23.0381421796601,20.));
#91003=CARTESIAN_POINT('Ctrl Pts',(42.2664343582719,23.0073797062893,0.));
#91004=CARTESIAN_POINT('Ctrl Pts',(42.2664343582719,23.0073797062893,20.));
#91005=CARTESIAN_POINT('Ctrl Pts',(42.2797311527738,22.9766090256973,0.));
#91006=CARTESIAN_POINT('Ctrl Pts',(42.2797311527738,22.9766090256973,20.));
#91007=CARTESIAN_POINT('Ctrl Pts',(42.2930061541893,22.9458301530364,0.));
#91008=CARTESIAN_POINT('Ctrl Pts',(42.2930061541893,22.9458301530364,20.));
#91009=CARTESIAN_POINT('Ctrl Pts',(42.3062593569225,22.9150431034629,0.));
#91010=CARTESIAN_POINT('Ctrl Pts',(42.3062593569225,22.9150431034629,20.));
#91011=CARTESIAN_POINT('Ctrl Pts',(42.3194907553882,22.8842478921374,0.));
#91012=CARTESIAN_POINT('Ctrl Pts',(42.3194907553882,22.8842478921374,20.));
#91013=CARTESIAN_POINT('Ctrl Pts',(42.3327003440108,22.8534445342249,0.));
#91014=CARTESIAN_POINT('Ctrl Pts',(42.3327003440108,22.8534445342249,20.));
#91015=CARTESIAN_POINT('Ctrl Pts',(42.3458881172255,22.8226330448945,0.));
#91016=CARTESIAN_POINT('Ctrl Pts',(42.3458881172255,22.8226330448945,20.));
#91017=CARTESIAN_POINT('Ctrl Pts',(42.3590540694774,22.7918134393197,0.));
#91018=CARTESIAN_POINT('Ctrl Pts',(42.3590540694774,22.7918134393197,20.));
#91019=CARTESIAN_POINT('Ctrl Pts',(42.3721981952224,22.7609857326781,0.));
#91020=CARTESIAN_POINT('Ctrl Pts',(42.3721981952224,22.7609857326781,20.));
#91021=CARTESIAN_POINT('Ctrl Pts',(42.3853204889273,22.7301499401517,0.));
#91022=CARTESIAN_POINT('Ctrl Pts',(42.3853204889273,22.7301499401517,20.));
#91023=CARTESIAN_POINT('Ctrl Pts',(42.398420945069,22.6993060769268,0.));
#91024=CARTESIAN_POINT('Ctrl Pts',(42.398420945069,22.6993060769268,20.));
#91025=CARTESIAN_POINT('Ctrl Pts',(42.411499558135,22.6684541581936,0.));
#91026=CARTESIAN_POINT('Ctrl Pts',(42.411499558135,22.6684541581936,20.));
#91027=CARTESIAN_POINT('Ctrl Pts',(42.4245563226236,22.6375941991468,0.));
#91028=CARTESIAN_POINT('Ctrl Pts',(42.4245563226236,22.6375941991468,20.));
#91029=CARTESIAN_POINT('Ctrl Pts',(42.4375912330427,22.6067262149851,0.));
#91030=CARTESIAN_POINT('Ctrl Pts',(42.4375912330427,22.6067262149851,20.));
#91031=CARTESIAN_POINT('Ctrl Pts',(42.4506042839107,22.5758502209116,0.));
#91032=CARTESIAN_POINT('Ctrl Pts',(42.4506042839107,22.5758502209116,20.));
#91033=CARTESIAN_POINT('Ctrl Pts',(42.4635954697559,22.5449662321334,0.));
#91034=CARTESIAN_POINT('Ctrl Pts',(42.4635954697559,22.5449662321334,20.));
#91035=CARTESIAN_POINT('Ctrl Pts',(42.4765647851171,22.5140742638619,0.));
#91036=CARTESIAN_POINT('Ctrl Pts',(42.4765647851171,22.5140742638619,20.));
#91037=CARTESIAN_POINT('Ctrl Pts',(42.4895122245441,22.4831743313126,0.));
#91038=CARTESIAN_POINT('Ctrl Pts',(42.4895122245441,22.4831743313126,20.));
#91039=CARTESIAN_POINT('Ctrl Pts',(42.502437782597,22.4522664497054,0.));
#91040=CARTESIAN_POINT('Ctrl Pts',(42.502437782597,22.4522664497054,20.));
#91041=CARTESIAN_POINT('Ctrl Pts',(42.5153414538467,22.4213506342639,0.));
#91042=CARTESIAN_POINT('Ctrl Pts',(42.5153414538467,22.4213506342639,20.));
#91043=CARTESIAN_POINT('Ctrl Pts',(42.5282232328747,22.3904269002165,0.));
#91044=CARTESIAN_POINT('Ctrl Pts',(42.5282232328747,22.3904269002165,20.));
#91045=CARTESIAN_POINT('Ctrl Pts',(42.5410831142726,22.3594952627952,0.));
#91046=CARTESIAN_POINT('Ctrl Pts',(42.5410831142726,22.3594952627952,20.));
#91047=CARTESIAN_POINT('Ctrl Pts',(42.5539210926424,22.3285557372364,0.));
#91048=CARTESIAN_POINT('Ctrl Pts',(42.5539210926424,22.3285557372364,20.));
#91049=CARTESIAN_POINT('Ctrl Pts',(42.5667371625962,22.2976083387805,0.));
#91050=CARTESIAN_POINT('Ctrl Pts',(42.5667371625962,22.2976083387805,20.));
#91051=CARTESIAN_POINT('Ctrl Pts',(42.5795313187569,22.2666530826722,0.));
#91052=CARTESIAN_POINT('Ctrl Pts',(42.5795313187569,22.2666530826722,20.));
#91053=CARTESIAN_POINT('Ctrl Pts',(42.5923035557573,22.2356899841602,0.));
#91054=CARTESIAN_POINT('Ctrl Pts',(42.5923035557573,22.2356899841602,20.));
#91055=CARTESIAN_POINT('Ctrl Pts',(42.6050538682411,22.2047190584974,0.));
#91056=CARTESIAN_POINT('Ctrl Pts',(42.6050538682411,22.2047190584974,20.));
#91057=CARTESIAN_POINT('Ctrl Pts',(42.6177822508627,22.1737403209406,0.));
#91058=CARTESIAN_POINT('Ctrl Pts',(42.6177822508627,22.1737403209406,20.));
#91059=CARTESIAN_POINT('Ctrl Pts',(42.6304886982869,22.1427537867512,0.));
#91060=CARTESIAN_POINT('Ctrl Pts',(42.6304886982869,22.1427537867512,20.));
#91061=CARTESIAN_POINT('Ctrl Pts',(42.6431732051887,22.1117594711942,0.));
#91062=CARTESIAN_POINT('Ctrl Pts',(42.6431732051887,22.1117594711942,20.));
#91063=CARTESIAN_POINT('Ctrl Pts',(42.6558357662536,22.0807573895388,0.));
#91064=CARTESIAN_POINT('Ctrl Pts',(42.6558357662536,22.0807573895388,20.));
#91065=CARTESIAN_POINT('Ctrl Pts',(42.6684763761777,22.0497475570584,0.));
#91066=CARTESIAN_POINT('Ctrl Pts',(42.6684763761777,22.0497475570584,20.));
#91067=CARTESIAN_POINT('Ctrl Pts',(42.6810950296678,22.0187299890302,0.));
#91068=CARTESIAN_POINT('Ctrl Pts',(42.6810950296678,22.0187299890302,20.));
#91069=CARTESIAN_POINT('Ctrl Pts',(42.6936917214411,21.9877047007357,0.));
#91070=CARTESIAN_POINT('Ctrl Pts',(42.6936917214411,21.9877047007357,20.));
#91071=CARTESIAN_POINT('Ctrl Pts',(42.7062664462249,21.9566717074606,0.));
#91072=CARTESIAN_POINT('Ctrl Pts',(42.7062664462249,21.9566717074606,20.));
#91073=CARTESIAN_POINT('Ctrl Pts',(42.7188191987573,21.9256310244944,0.));
#91074=CARTESIAN_POINT('Ctrl Pts',(42.7188191987573,21.9256310244944,20.));
#91075=CARTESIAN_POINT('Ctrl Pts',(42.7313499737866,21.8945826671308,0.));
#91076=CARTESIAN_POINT('Ctrl Pts',(42.7313499737866,21.8945826671308,20.));
#91077=CARTESIAN_POINT('Ctrl Pts',(42.7438587660714,21.8635266506674,0.));
#91078=CARTESIAN_POINT('Ctrl Pts',(42.7438587660714,21.8635266506674,20.));
#91079=CARTESIAN_POINT('Ctrl Pts',(42.7563455703812,21.832462990406,0.));
#91080=CARTESIAN_POINT('Ctrl Pts',(42.7563455703812,21.832462990406,20.));
#91081=CARTESIAN_POINT('Ctrl Pts',(42.7688103814962,21.8013917016521,0.));
#91082=CARTESIAN_POINT('Ctrl Pts',(42.7688103814962,21.8013917016521,20.));
#91083=CARTESIAN_POINT('Ctrl Pts',(42.7812531942069,21.7703127997157,0.));
#91084=CARTESIAN_POINT('Ctrl Pts',(42.7812531942069,21.7703127997157,20.));
#91085=CARTESIAN_POINT('Ctrl Pts',(42.7936740033148,21.7392262999104,0.));
#91086=CARTESIAN_POINT('Ctrl Pts',(42.7936740033148,21.7392262999104,20.));
#91087=CARTESIAN_POINT('Ctrl Pts',(42.8060728036313,21.7081322175539,0.));
#91088=CARTESIAN_POINT('Ctrl Pts',(42.8060728036313,21.7081322175539,20.));
#91089=CARTESIAN_POINT('Ctrl Pts',(42.8184495899785,21.677030567968,0.));
#91090=CARTESIAN_POINT('Ctrl Pts',(42.8184495899785,21.677030567968,20.));
#91091=CARTESIAN_POINT('Ctrl Pts',(42.8308043571886,21.6459213664784,0.));
#91092=CARTESIAN_POINT('Ctrl Pts',(42.8308043571886,21.6459213664784,20.));
#91093=CARTESIAN_POINT('Ctrl Pts',(42.8431371001047,21.6148046284149,0.));
#91094=CARTESIAN_POINT('Ctrl Pts',(42.8431371001047,21.6148046284149,20.));
#91095=CARTESIAN_POINT('Ctrl Pts',(42.8554478135801,21.5836803691112,0.));
#91096=CARTESIAN_POINT('Ctrl Pts',(42.8554478135801,21.5836803691112,20.));
#91097=CARTESIAN_POINT('Ctrl Pts',(42.8677364924793,21.5525486039049,0.));
#91098=CARTESIAN_POINT('Ctrl Pts',(42.8677364924793,21.5525486039049,20.));
#91099=CARTESIAN_POINT('Ctrl Pts',(42.8800031316769,21.5214093481377,0.));
#91100=CARTESIAN_POINT('Ctrl Pts',(42.8800031316769,21.5214093481377,20.));
#91101=CARTESIAN_POINT('Ctrl Pts',(42.8922477260581,21.490262617155,0.));
#91102=CARTESIAN_POINT('Ctrl Pts',(42.8922477260581,21.490262617155,20.));
#91103=CARTESIAN_POINT('Ctrl Pts',(42.9044702705183,21.4591084263065,0.));
#91104=CARTESIAN_POINT('Ctrl Pts',(42.9044702705183,21.4591084263065,20.));
#91105=CARTESIAN_POINT('Ctrl Pts',(42.916670759964,21.4279467909454,0.));
#91106=CARTESIAN_POINT('Ctrl Pts',(42.916670759964,21.4279467909454,20.));
#91107=CARTESIAN_POINT('Ctrl Pts',(42.9288491893122,21.3967777264295,0.));
#91108=CARTESIAN_POINT('Ctrl Pts',(42.9288491893122,21.3967777264295,20.));
#91109=CARTESIAN_POINT('Ctrl Pts',(42.9410055534907,21.3656012481199,0.));
#91110=CARTESIAN_POINT('Ctrl Pts',(42.9410055534907,21.3656012481199,20.));
#91111=CARTESIAN_POINT('Ctrl Pts',(42.9531398474371,21.3344173713818,0.));
#91112=CARTESIAN_POINT('Ctrl Pts',(42.9531398474371,21.3344173713818,20.));
#91113=CARTESIAN_POINT('Ctrl Pts',(42.9652520660998,21.3032261115844,0.));
#91114=CARTESIAN_POINT('Ctrl Pts',(42.9652520660998,21.3032261115844,20.));
#91115=CARTESIAN_POINT('Ctrl Pts',(42.9773422044374,21.2720274841006,0.));
#91116=CARTESIAN_POINT('Ctrl Pts',(42.9773422044374,21.2720274841006,20.));
#91117=CARTESIAN_POINT('Ctrl Pts',(42.9894102574195,21.2408215043074,0.));
#91118=CARTESIAN_POINT('Ctrl Pts',(42.9894102574195,21.2408215043074,20.));
#91119=CARTESIAN_POINT('Ctrl Pts',(43.0014562200264,21.2096081875857,0.));
#91120=CARTESIAN_POINT('Ctrl Pts',(43.0014562200264,21.2096081875857,20.));
#91121=CARTESIAN_POINT('Ctrl Pts',(43.0134800872489,21.1783875493205,0.));
#91122=CARTESIAN_POINT('Ctrl Pts',(43.0134800872489,21.1783875493205,20.));
#91123=CARTESIAN_POINT('Ctrl Pts',(43.0254818540885,21.1471596049,0.));
#91124=CARTESIAN_POINT('Ctrl Pts',(43.0254818540885,21.1471596049,20.));
#91125=CARTESIAN_POINT('Ctrl Pts',(43.037461515557,21.1159243697169,0.));
#91126=CARTESIAN_POINT('Ctrl Pts',(43.037461515557,21.1159243697169,20.));
#91127=CARTESIAN_POINT('Ctrl Pts',(43.049419066677,21.0846818591673,0.));
#91128=CARTESIAN_POINT('Ctrl Pts',(43.049419066677,21.0846818591673,20.));
#91129=CARTESIAN_POINT('Ctrl Pts',(43.0613545024815,21.0534320886512,0.));
#91130=CARTESIAN_POINT('Ctrl Pts',(43.0613545024815,21.0534320886512,20.));
#91131=CARTESIAN_POINT('Ctrl Pts',(43.0732678180139,21.0221750735727,0.));
#91132=CARTESIAN_POINT('Ctrl Pts',(43.0732678180139,21.0221750735727,20.));
#91133=CARTESIAN_POINT('Ctrl Pts',(43.0851590083283,20.9909108293397,0.));
#91134=CARTESIAN_POINT('Ctrl Pts',(43.0851590083283,20.9909108293397,20.));
#91135=CARTESIAN_POINT('Ctrl Pts',(43.0970280684896,20.959639371364,0.));
#91136=CARTESIAN_POINT('Ctrl Pts',(43.0970280684896,20.959639371364,20.));
#91137=CARTESIAN_POINT('Ctrl Pts',(43.1088749935734,20.9283607150615,0.));
#91138=CARTESIAN_POINT('Ctrl Pts',(43.1088749935734,20.9283607150615,20.));
#91139=CARTESIAN_POINT('Ctrl Pts',(43.1206997786656,20.8970748758512,0.));
#91140=CARTESIAN_POINT('Ctrl Pts',(43.1206997786656,20.8970748758512,20.));
#91141=CARTESIAN_POINT('Ctrl Pts',(43.132502418863,20.8657818691565,0.));
#91142=CARTESIAN_POINT('Ctrl Pts',(43.132502418863,20.8657818691565,20.));
#91143=CARTESIAN_POINT('Ctrl Pts',(43.1442829092724,20.8344817104039,0.));
#91144=CARTESIAN_POINT('Ctrl Pts',(43.1442829092724,20.8344817104039,20.));
#91145=CARTESIAN_POINT('Ctrl Pts',(43.1560412450117,20.8031744150242,0.));
#91146=CARTESIAN_POINT('Ctrl Pts',(43.1560412450117,20.8031744150242,20.));
#91147=CARTESIAN_POINT('Ctrl Pts',(43.1677774212093,20.7718599984519,0.));
#91148=CARTESIAN_POINT('Ctrl Pts',(43.1677774212093,20.7718599984519,20.));
#91149=CARTESIAN_POINT('Ctrl Pts',(43.1794914330045,20.7405384761252,0.));
#91150=CARTESIAN_POINT('Ctrl Pts',(43.1794914330045,20.7405384761252,20.));
#91151=CARTESIAN_POINT('Ctrl Pts',(43.1911832755467,20.7092098634864,0.));
#91152=CARTESIAN_POINT('Ctrl Pts',(43.1911832755467,20.7092098634864,20.));
#91153=CARTESIAN_POINT('Ctrl Pts',(43.202852943996,20.6778741759814,0.));
#91154=CARTESIAN_POINT('Ctrl Pts',(43.202852943996,20.6778741759814,20.));
#91155=CARTESIAN_POINT('Ctrl Pts',(43.2145004335236,20.6465314290598,0.));
#91156=CARTESIAN_POINT('Ctrl Pts',(43.2145004335236,20.6465314290598,20.));
#91157=CARTESIAN_POINT('Ctrl Pts',(43.2261257393109,20.615181638175,0.));
#91158=CARTESIAN_POINT('Ctrl Pts',(43.2261257393109,20.615181638175,20.));
#91159=CARTESIAN_POINT('Ctrl Pts',(43.2377288565503,20.5838248187841,0.));
#91160=CARTESIAN_POINT('Ctrl Pts',(43.2377288565503,20.5838248187841,20.));
#91161=CARTESIAN_POINT('Ctrl Pts',(43.2493097804445,20.5524609863481,0.));
#91162=CARTESIAN_POINT('Ctrl Pts',(43.2493097804445,20.5524609863481,20.));
#91163=CARTESIAN_POINT('Ctrl Pts',(43.2608685062069,20.5210901563314,0.));
#91164=CARTESIAN_POINT('Ctrl Pts',(43.2608685062069,20.5210901563314,20.));
#91165=CARTESIAN_POINT('Ctrl Pts',(43.2724050290617,20.4897123442023,0.));
#91166=CARTESIAN_POINT('Ctrl Pts',(43.2724050290617,20.4897123442023,20.));
#91167=CARTESIAN_POINT('Ctrl Pts',(43.283919344243,20.4583275654327,0.));
#91168=CARTESIAN_POINT('Ctrl Pts',(43.283919344243,20.4583275654327,20.));
#91169=CARTESIAN_POINT('Ctrl Pts',(43.2954114469964,20.4269358354984,0.));
#91170=CARTESIAN_POINT('Ctrl Pts',(43.2954114469964,20.4269358354984,20.));
#91171=CARTESIAN_POINT('Ctrl Pts',(43.3068813325774,20.3955371698787,0.));
#91172=CARTESIAN_POINT('Ctrl Pts',(43.3068813325774,20.3955371698787,20.));
#91173=CARTESIAN_POINT('Ctrl Pts',(43.3183289962528,20.3641315840566,0.));
#91174=CARTESIAN_POINT('Ctrl Pts',(43.3183289962528,20.3641315840566,20.));
#91175=CARTESIAN_POINT('Ctrl Pts',(43.3297544333003,20.3327190935193,0.));
#91176=CARTESIAN_POINT('Ctrl Pts',(43.3297544333003,20.3327190935193,20.));
#91177=CARTESIAN_POINT('Ctrl Pts',(43.3411576390085,20.3012997137575,0.));
#91178=CARTESIAN_POINT('Ctrl Pts',(43.3411576390085,20.3012997137575,20.));
#91179=CARTESIAN_POINT('Ctrl Pts',(43.3525386086763,20.2698734602656,0.));
#91180=CARTESIAN_POINT('Ctrl Pts',(43.3525386086763,20.2698734602656,20.));
#91181=CARTESIAN_POINT('Ctrl Pts',(43.3638973376125,20.2384403485411,0.));
#91182=CARTESIAN_POINT('Ctrl Pts',(43.3638973376125,20.2384403485411,20.));
#91183=CARTESIAN_POINT('Ctrl Pts',(43.3752338211368,20.2070003940853,0.));
#91184=CARTESIAN_POINT('Ctrl Pts',(43.3752338211368,20.2070003940853,20.));
#91185=CARTESIAN_POINT('Ctrl Pts',(43.3865480545792,20.1755536124033,0.));
#91186=CARTESIAN_POINT('Ctrl Pts',(43.3865480545792,20.1755536124033,20.));
#91187=CARTESIAN_POINT('Ctrl Pts',(43.3978400332808,20.1441000190037,0.));
#91188=CARTESIAN_POINT('Ctrl Pts',(43.3978400332808,20.1441000190037,20.));
#91189=CARTESIAN_POINT('Ctrl Pts',(43.409109752594,20.1126396293992,0.));
#91190=CARTESIAN_POINT('Ctrl Pts',(43.409109752594,20.1126396293992,20.));
#91191=CARTESIAN_POINT('Ctrl Pts',(43.4203572078819,20.0811724591059,0.));
#91192=CARTESIAN_POINT('Ctrl Pts',(43.4203572078819,20.0811724591059,20.));
#91193=CARTESIAN_POINT('Ctrl Pts',(43.4315823945181,20.0496985236436,0.));
#91194=CARTESIAN_POINT('Ctrl Pts',(43.4315823945181,20.0496985236436,20.));
#91195=CARTESIAN_POINT('Ctrl Pts',(43.4427853078868,20.0182178385356,0.));
#91196=CARTESIAN_POINT('Ctrl Pts',(43.4427853078868,20.0182178385356,20.));
#91197=CARTESIAN_POINT('Ctrl Pts',(43.4539659433821,19.9867304193089,0.));
#91198=CARTESIAN_POINT('Ctrl Pts',(43.4539659433821,19.9867304193089,20.));
#91199=CARTESIAN_POINT('Ctrl Pts',(43.4651242964088,19.9552362814936,0.));
#91200=CARTESIAN_POINT('Ctrl Pts',(43.4651242964088,19.9552362814936,20.));
#91201=CARTESIAN_POINT('Ctrl Pts',(43.4762603623832,19.923735440624,0.));
#91202=CARTESIAN_POINT('Ctrl Pts',(43.4762603623832,19.923735440624,20.));
#91203=CARTESIAN_POINT('Ctrl Pts',(43.4873741367321,19.8922279122378,0.));
#91204=CARTESIAN_POINT('Ctrl Pts',(43.4873741367321,19.8922279122378,20.));
#91205=CARTESIAN_POINT('Ctrl Pts',(43.4984656148935,19.8607137118763,0.));
#91206=CARTESIAN_POINT('Ctrl Pts',(43.4984656148935,19.8607137118763,20.));
#91207=CARTESIAN_POINT('Ctrl Pts',(43.5095347923164,19.8291928550844,0.));
#91208=CARTESIAN_POINT('Ctrl Pts',(43.5095347923164,19.8291928550844,20.));
#91209=CARTESIAN_POINT('Ctrl Pts',(43.5205816644596,19.7976653574108,0.));
#91210=CARTESIAN_POINT('Ctrl Pts',(43.5205816644596,19.7976653574108,20.));
#91211=CARTESIAN_POINT('Ctrl Pts',(43.5316062267925,19.7661312344072,0.));
#91212=CARTESIAN_POINT('Ctrl Pts',(43.5316062267925,19.7661312344072,20.));
#91213=CARTESIAN_POINT('Ctrl Pts',(43.542608474795,19.734590501629,0.));
#91214=CARTESIAN_POINT('Ctrl Pts',(43.542608474795,19.734590501629,20.));
#91215=CARTESIAN_POINT('Ctrl Pts',(43.5535884039576,19.7030431746352,0.));
#91216=CARTESIAN_POINT('Ctrl Pts',(43.5535884039576,19.7030431746352,20.));
#91217=CARTESIAN_POINT('Ctrl Pts',(43.5645460097823,19.6714892689885,0.));
#91218=CARTESIAN_POINT('Ctrl Pts',(43.5645460097823,19.6714892689885,20.));
#91219=CARTESIAN_POINT('Ctrl Pts',(43.5754812877819,19.639928800255,0.));
#91220=CARTESIAN_POINT('Ctrl Pts',(43.5754812877819,19.639928800255,20.));
#91221=CARTESIAN_POINT('Ctrl Pts',(43.5863942334797,19.6083617840046,0.));
#91222=CARTESIAN_POINT('Ctrl Pts',(43.5863942334797,19.6083617840046,20.));
#91223=CARTESIAN_POINT('Ctrl Pts',(43.5972848424097,19.5767882358104,0.));
#91224=CARTESIAN_POINT('Ctrl Pts',(43.5972848424097,19.5767882358104,20.));
#91225=CARTESIAN_POINT('Ctrl Pts',(43.6081531101168,19.545208171249,0.));
#91226=CARTESIAN_POINT('Ctrl Pts',(43.6081531101168,19.545208171249,20.));
#91227=CARTESIAN_POINT('Ctrl Pts',(43.6189990321561,19.5136216059004,0.));
#91228=CARTESIAN_POINT('Ctrl Pts',(43.6189990321561,19.5136216059004,20.));
#91229=CARTESIAN_POINT('Ctrl Pts',(43.629822604094,19.4820285553483,0.));
#91230=CARTESIAN_POINT('Ctrl Pts',(43.629822604094,19.4820285553483,20.));
#91231=CARTESIAN_POINT('Ctrl Pts',(43.6406238215078,19.4504290351799,0.));
#91232=CARTESIAN_POINT('Ctrl Pts',(43.6406238215078,19.4504290351799,20.));
#91233=CARTESIAN_POINT('Ctrl Pts',(43.6514026799849,19.4188230609858,0.));
#91234=CARTESIAN_POINT('Ctrl Pts',(43.6514026799849,19.4188230609858,20.));
#91235=CARTESIAN_POINT('Ctrl Pts',(43.6621591751234,19.3872106483603,0.));
#91236=CARTESIAN_POINT('Ctrl Pts',(43.6621591751234,19.3872106483603,20.));
#91237=CARTESIAN_POINT('Ctrl Pts',(43.6728933025325,19.3555918129009,0.));
#91238=CARTESIAN_POINT('Ctrl Pts',(43.6728933025325,19.3555918129009,20.));
#91239=CARTESIAN_POINT('Ctrl Pts',(43.6836050578319,19.3239665702086,0.));
#91240=CARTESIAN_POINT('Ctrl Pts',(43.6836050578319,19.3239665702086,20.));
#91241=CARTESIAN_POINT('Ctrl Pts',(43.6942944366523,19.2923349358879,0.));
#91242=CARTESIAN_POINT('Ctrl Pts',(43.6942944366523,19.2923349358879,20.));
#91243=CARTESIAN_POINT('Ctrl Pts',(43.7049614346349,19.2606969255464,0.));
#91244=CARTESIAN_POINT('Ctrl Pts',(43.7049614346349,19.2606969255464,20.));
#91245=CARTESIAN_POINT('Ctrl Pts',(43.7156060474324,19.2290525547956,0.));
#91246=CARTESIAN_POINT('Ctrl Pts',(43.7156060474324,19.2290525547956,20.));
#91247=CARTESIAN_POINT('Ctrl Pts',(43.7262282707082,19.1974018392505,0.));
#91248=CARTESIAN_POINT('Ctrl Pts',(43.7262282707082,19.1974018392505,20.));
#91249=CARTESIAN_POINT('Ctrl Pts',(43.7368281001363,19.1657447945291,0.));
#91250=CARTESIAN_POINT('Ctrl Pts',(43.7368281001363,19.1657447945291,20.));
#91251=CARTESIAN_POINT('Ctrl Pts',(43.747405531401,19.1340814362531,0.));
#91252=CARTESIAN_POINT('Ctrl Pts',(43.747405531401,19.1340814362531,20.));
#91253=CARTESIAN_POINT('Ctrl Pts',(43.7579605601976,19.1024117800474,0.));
#91254=CARTESIAN_POINT('Ctrl Pts',(43.7579605601976,19.1024117800474,20.));
#91255=CARTESIAN_POINT('Ctrl Pts',(43.7684931822314,19.0707358415405,0.));
#91256=CARTESIAN_POINT('Ctrl Pts',(43.7684931822314,19.0707358415405,20.));
#91257=CARTESIAN_POINT('Ctrl Pts',(43.779003393219,19.039053636364,0.));
#91258=CARTESIAN_POINT('Ctrl Pts',(43.779003393219,19.039053636364,20.));
#91259=CARTESIAN_POINT('Ctrl Pts',(43.7894911888877,19.0073651801531,0.));
#91260=CARTESIAN_POINT('Ctrl Pts',(43.7894911888877,19.0073651801531,20.));
#91261=CARTESIAN_POINT('Ctrl Pts',(43.7999565649762,18.9756704885464,0.));
#91262=CARTESIAN_POINT('Ctrl Pts',(43.7999565649762,18.9756704885464,20.));
#91263=CARTESIAN_POINT('Ctrl Pts',(43.8103995172341,18.9439695771858,0.));
#91264=CARTESIAN_POINT('Ctrl Pts',(43.8103995172341,18.9439695771858,20.));
#91265=CARTESIAN_POINT('Ctrl Pts',(43.8208200414219,18.9122624617166,0.));
#91266=CARTESIAN_POINT('Ctrl Pts',(43.8208200414219,18.9122624617166,20.));
#91267=CARTESIAN_POINT('Ctrl Pts',(43.8312181333106,18.8805491577876,0.));
#91268=CARTESIAN_POINT('Ctrl Pts',(43.8312181333106,18.8805491577876,20.));
#91269=CARTESIAN_POINT('Ctrl Pts',(43.8415937886817,18.8488296810507,0.));
#91270=CARTESIAN_POINT('Ctrl Pts',(43.8415937886817,18.8488296810507,20.));
#91271=CARTESIAN_POINT('Ctrl Pts',(43.8519470033272,18.8171040471611,0.));
#91272=CARTESIAN_POINT('Ctrl Pts',(43.8519470033272,18.8171040471611,20.));
#91273=CARTESIAN_POINT('Ctrl Pts',(43.8622777730502,18.7853722717774,0.));
#91274=CARTESIAN_POINT('Ctrl Pts',(43.8622777730502,18.7853722717774,20.));
#91275=CARTESIAN_POINT('Ctrl Pts',(43.8725860936644,18.7536343705616,0.));
#91276=CARTESIAN_POINT('Ctrl Pts',(43.8725860936644,18.7536343705616,20.));
#91277=CARTESIAN_POINT('Ctrl Pts',(43.8828719609947,18.721890359179,0.));
#91278=CARTESIAN_POINT('Ctrl Pts',(43.8828719609947,18.721890359179,20.));
#91279=CARTESIAN_POINT('Ctrl Pts',(43.8931353708767,18.6901402532984,0.));
#91280=CARTESIAN_POINT('Ctrl Pts',(43.8931353708767,18.6901402532984,20.));
#91281=CARTESIAN_POINT('Ctrl Pts',(43.903376319157,18.6583840685915,0.));
#91282=CARTESIAN_POINT('Ctrl Pts',(43.903376319157,18.6583840685915,20.));
#91283=CARTESIAN_POINT('Ctrl Pts',(43.913594801693,18.6266218207337,0.));
#91284=CARTESIAN_POINT('Ctrl Pts',(43.913594801693,18.6266218207337,20.));
#91285=CARTESIAN_POINT('Ctrl Pts',(43.9237908143526,18.5948535254034,0.));
#91286=CARTESIAN_POINT('Ctrl Pts',(43.9237908143526,18.5948535254034,20.));
#91287=CARTESIAN_POINT('Ctrl Pts',(43.9339643530151,18.5630791982821,0.));
#91288=CARTESIAN_POINT('Ctrl Pts',(43.9339643530151,18.5630791982821,20.));
#91289=CARTESIAN_POINT('Ctrl Pts',(43.94411541357,18.5312988550549,0.));
#91290=CARTESIAN_POINT('Ctrl Pts',(43.94411541357,18.5312988550549,20.));
#91291=CARTESIAN_POINT('Ctrl Pts',(43.9542439919177,18.4995125114099,0.));
#91292=CARTESIAN_POINT('Ctrl Pts',(43.9542439919177,18.4995125114099,20.));
#91293=CARTESIAN_POINT('Ctrl Pts',(43.9643500839697,18.4677201830388,0.));
#91294=CARTESIAN_POINT('Ctrl Pts',(43.9643500839697,18.4677201830388,20.));
#91295=CARTESIAN_POINT('Ctrl Pts',(43.9744336856481,18.4359218856365,0.));
#91296=CARTESIAN_POINT('Ctrl Pts',(43.9744336856481,18.4359218856365,20.));
#91297=CARTESIAN_POINT('Ctrl Pts',(43.9844947928861,18.4041176349014,0.));
#91298=CARTESIAN_POINT('Ctrl Pts',(43.9844947928861,18.4041176349014,20.));
#91299=CARTESIAN_POINT('Ctrl Pts',(43.9945334016277,18.3723074465347,0.));
#91300=CARTESIAN_POINT('Ctrl Pts',(43.9945334016277,18.3723074465347,20.));
#91301=CARTESIAN_POINT('Ctrl Pts',(44.0045495078276,18.3404913362408,0.));
#91302=CARTESIAN_POINT('Ctrl Pts',(44.0045495078276,18.3404913362408,20.));
#91303=CARTESIAN_POINT('Ctrl Pts',(44.0145431074514,18.3086693197275,0.));
#91304=CARTESIAN_POINT('Ctrl Pts',(44.0145431074514,18.3086693197275,20.));
#91305=CARTESIAN_POINT('Ctrl Pts',(44.0245141964756,18.2768414127056,0.));
#91306=CARTESIAN_POINT('Ctrl Pts',(44.0245141964756,18.2768414127056,20.));
#91307=CARTESIAN_POINT('Ctrl Pts',(44.0344627708874,18.245007630889,0.));
#91308=CARTESIAN_POINT('Ctrl Pts',(44.0344627708874,18.245007630889,20.));
#91309=CARTESIAN_POINT('Ctrl Pts',(44.044388826685,18.2131679899948,0.));
#91310=CARTESIAN_POINT('Ctrl Pts',(44.044388826685,18.2131679899948,20.));
#91311=CARTESIAN_POINT('Ctrl Pts',(44.0542923598772,18.1813225057438,0.));
#91312=CARTESIAN_POINT('Ctrl Pts',(44.0542923598772,18.1813225057438,20.));
#91313=CARTESIAN_POINT('Ctrl Pts',(44.0641733664839,18.1494711938598,0.));
#91314=CARTESIAN_POINT('Ctrl Pts',(44.0641733664839,18.1494711938598,20.));
#91315=CARTESIAN_POINT('Ctrl Pts',(44.0740318425361,18.1176140700699,0.));
#91316=CARTESIAN_POINT('Ctrl Pts',(44.0740318425361,18.1176140700699,20.));
#91317=CARTESIAN_POINT('Ctrl Pts',(44.0838677840754,18.0857511501043,0.));
#91318=CARTESIAN_POINT('Ctrl Pts',(44.0838677840754,18.0857511501043,20.));
#91319=CARTESIAN_POINT('Ctrl Pts',(44.0936811871546,18.0538824496962,0.));
#91320=CARTESIAN_POINT('Ctrl Pts',(44.0936811871546,18.0538824496962,20.));
#91321=CARTESIAN_POINT('Ctrl Pts',(44.1034720478372,18.0220079845822,0.));
#91322=CARTESIAN_POINT('Ctrl Pts',(44.1034720478372,18.0220079845822,20.));
#91323=CARTESIAN_POINT('Ctrl Pts',(44.1132403621971,17.9901277705015,0.));
#91324=CARTESIAN_POINT('Ctrl Pts',(44.1132403621971,17.9901277705015,20.));
#91325=CARTESIAN_POINT('Ctrl Pts',(44.1229861263191,17.9582418231966,0.));
#91326=CARTESIAN_POINT('Ctrl Pts',(44.1229861263191,17.9582418231966,20.));
#91327=CARTESIAN_POINT('Ctrl Pts',(44.1327093362991,17.9263501584131,0.));
#91328=CARTESIAN_POINT('Ctrl Pts',(44.1327093362991,17.9263501584131,20.));
#91329=CARTESIAN_POINT('Ctrl Pts',(44.1424099882439,17.8944527919,0.));
#91330=CARTESIAN_POINT('Ctrl Pts',(44.1424099882439,17.8944527919,20.));
#91331=CARTESIAN_POINT('Ctrl Pts',(44.1520880782717,17.8625497394092,0.));
#91332=CARTESIAN_POINT('Ctrl Pts',(44.1520880782717,17.8625497394092,20.));
#91333=CARTESIAN_POINT('Ctrl Pts',(44.1617436025112,17.8306410166963,0.));
#91334=CARTESIAN_POINT('Ctrl Pts',(44.1617436025112,17.8306410166963,20.));
#91335=CARTESIAN_POINT('Ctrl Pts',(44.1713765571021,17.7987266395196,0.));
#91336=CARTESIAN_POINT('Ctrl Pts',(44.1713765571021,17.7987266395196,20.));
#91337=CARTESIAN_POINT('Ctrl Pts',(44.1809869381949,17.7668066236405,0.));
#91338=CARTESIAN_POINT('Ctrl Pts',(44.1809869381949,17.7668066236405,20.));
#91339=CARTESIAN_POINT('Ctrl Pts',(44.1905747419505,17.7348809848234,0.));
#91340=CARTESIAN_POINT('Ctrl Pts',(44.1905747419505,17.7348809848234,20.));
#91341=CARTESIAN_POINT('Ctrl Pts',(44.2001399645408,17.7029497388358,0.));
#91342=CARTESIAN_POINT('Ctrl Pts',(44.2001399645408,17.7029497388358,20.));
#91343=CARTESIAN_POINT('Ctrl Pts',(44.2096826021493,17.6710129014481,0.));
#91344=CARTESIAN_POINT('Ctrl Pts',(44.2096826021493,17.6710129014481,20.));
#91345=CARTESIAN_POINT('Ctrl Pts',(44.2192026509705,17.6390704884341,0.));
#91346=CARTESIAN_POINT('Ctrl Pts',(44.2192026509705,17.6390704884341,20.));
#91347=CARTESIAN_POINT('Ctrl Pts',(44.2287001072093,17.6071225155702,0.));
#91348=CARTESIAN_POINT('Ctrl Pts',(44.2287001072093,17.6071225155702,20.));
#91349=CARTESIAN_POINT('Ctrl Pts',(44.2381749670816,17.5751689986363,0.));
#91350=CARTESIAN_POINT('Ctrl Pts',(44.2381749670816,17.5751689986363,20.));
#91351=CARTESIAN_POINT('Ctrl Pts',(44.2476272268138,17.5432099534151,0.));
#91352=CARTESIAN_POINT('Ctrl Pts',(44.2476272268138,17.5432099534151,20.));
#91353=CARTESIAN_POINT('Ctrl Pts',(44.2570568826434,17.5112453956925,0.));
#91354=CARTESIAN_POINT('Ctrl Pts',(44.2570568826434,17.5112453956925,20.));
#91355=CARTESIAN_POINT('Ctrl Pts',(44.2664639308191,17.4792753412574,0.));
#91356=CARTESIAN_POINT('Ctrl Pts',(44.2664639308191,17.4792753412574,20.));
#91357=CARTESIAN_POINT('Ctrl Pts',(44.2758483676008,17.447299805902,0.));
#91358=CARTESIAN_POINT('Ctrl Pts',(44.2758483676008,17.447299805902,20.));
#91359=CARTESIAN_POINT('Ctrl Pts',(44.2852101892593,17.4153188054211,0.));
#91360=CARTESIAN_POINT('Ctrl Pts',(44.2852101892593,17.4153188054211,20.));
#91361=CARTESIAN_POINT('Ctrl Pts',(44.294549392076,17.3833323556128,0.));
#91362=CARTESIAN_POINT('Ctrl Pts',(44.294549392076,17.3833323556128,20.));
#91363=CARTESIAN_POINT('Ctrl Pts',(44.3038659723435,17.3513404722779,0.));
#91364=CARTESIAN_POINT('Ctrl Pts',(44.3038659723435,17.3513404722779,20.));
#91365=CARTESIAN_POINT('Ctrl Pts',(44.3131599263642,17.3193431712198,0.));
#91366=CARTESIAN_POINT('Ctrl Pts',(44.3131599263642,17.3193431712198,20.));
#91367=CARTESIAN_POINT('Ctrl Pts',(44.3224312504523,17.2873404682456,0.));
#91368=CARTESIAN_POINT('Ctrl Pts',(44.3224312504523,17.2873404682456,20.));
#91369=CARTESIAN_POINT('Ctrl Pts',(44.3316799409325,17.2553323791649,0.));
#91370=CARTESIAN_POINT('Ctrl Pts',(44.3316799409325,17.2553323791649,20.));
#91371=CARTESIAN_POINT('Ctrl Pts',(44.340905994141,17.2233189197905,0.));
#91372=CARTESIAN_POINT('Ctrl Pts',(44.340905994141,17.2233189197905,20.));
#91373=CARTESIAN_POINT('Ctrl Pts',(44.3501094064252,17.1913001059384,0.));
#91374=CARTESIAN_POINT('Ctrl Pts',(44.3501094064252,17.1913001059384,20.));
#91375=CARTESIAN_POINT('Ctrl Pts',(44.3592901741436,17.1592759534275,0.));
#91376=CARTESIAN_POINT('Ctrl Pts',(44.3592901741436,17.1592759534275,20.));
#91377=CARTESIAN_POINT('Ctrl Pts',(44.3684482936655,17.1272464780797,0.));
#91378=CARTESIAN_POINT('Ctrl Pts',(44.3684482936655,17.1272464780797,20.));
#91379=CARTESIAN_POINT('Ctrl Pts',(44.3775837613707,17.0952116957196,0.));
#91380=CARTESIAN_POINT('Ctrl Pts',(44.3775837613707,17.0952116957196,20.));
#91381=CARTESIAN_POINT('Ctrl Pts',(44.3866965736492,17.0631716221745,0.));
#91382=CARTESIAN_POINT('Ctrl Pts',(44.3866965736492,17.0631716221745,20.));
#91383=CARTESIAN_POINT('Ctrl Pts',(44.3957867269024,17.0311262732746,0.));
#91384=CARTESIAN_POINT('Ctrl Pts',(44.3957867269024,17.0311262732746,20.));
#91385=CARTESIAN_POINT('Ctrl Pts',(44.404854217543,16.9990756648532,0.));
#91386=CARTESIAN_POINT('Ctrl Pts',(44.404854217543,16.9990756648532,20.));
#91387=CARTESIAN_POINT('Ctrl Pts',(44.4138990419958,16.967019812747,0.));
#91388=CARTESIAN_POINT('Ctrl Pts',(44.4138990419958,16.967019812747,20.));
#91389=CARTESIAN_POINT('Ctrl Pts',(44.4229211966955,16.9349587327952,0.));
#91390=CARTESIAN_POINT('Ctrl Pts',(44.4229211966955,16.9349587327952,20.));
#91391=CARTESIAN_POINT('Ctrl Pts',(44.4319206780879,16.9028924408399,0.));
#91392=CARTESIAN_POINT('Ctrl Pts',(44.4319206780879,16.9028924408399,20.));
#91393=CARTESIAN_POINT('Ctrl Pts',(44.4408974826293,16.870820952726,0.));
#91394=CARTESIAN_POINT('Ctrl Pts',(44.4408974826293,16.870820952726,20.));
#91395=CARTESIAN_POINT('Ctrl Pts',(44.4498516067869,16.8387442843012,0.));
#91396=CARTESIAN_POINT('Ctrl Pts',(44.4498516067869,16.8387442843012,20.));
#91397=CARTESIAN_POINT('Ctrl Pts',(44.4587830470388,16.8066624514163,0.));
#91398=CARTESIAN_POINT('Ctrl Pts',(44.4587830470388,16.8066624514163,20.));
#91399=CARTESIAN_POINT('Ctrl Pts',(44.4676917998748,16.7745754699247,0.));
#91400=CARTESIAN_POINT('Ctrl Pts',(44.4676917998748,16.7745754699247,20.));
#91401=CARTESIAN_POINT('Ctrl Pts',(44.4765778617956,16.742483355683,0.));
#91402=CARTESIAN_POINT('Ctrl Pts',(44.4765778617956,16.742483355683,20.));
#91403=CARTESIAN_POINT('Ctrl Pts',(44.4854412293128,16.7103861245505,0.));
#91404=CARTESIAN_POINT('Ctrl Pts',(44.4854412293128,16.7103861245505,20.));
#91405=CARTESIAN_POINT('Ctrl Pts',(44.4942818989491,16.6782837923893,0.));
#91406=CARTESIAN_POINT('Ctrl Pts',(44.4942818989491,16.6782837923893,20.));
#91407=CARTESIAN_POINT('Ctrl Pts',(44.503099867238,16.6461763750644,0.));
#91408=CARTESIAN_POINT('Ctrl Pts',(44.503099867238,16.6461763750644,20.));
#91409=CARTESIAN_POINT('Ctrl Pts',(44.5118951307243,16.6140638884438,0.));
#91410=CARTESIAN_POINT('Ctrl Pts',(44.5118951307243,16.6140638884438,20.));
#91411=CARTESIAN_POINT('Ctrl Pts',(44.5206676859632,16.581946348398,0.));
#91412=CARTESIAN_POINT('Ctrl Pts',(44.5206676859632,16.581946348398,20.));
#91413=CARTESIAN_POINT('Ctrl Pts',(44.5294175295214,16.5498237708003,0.));
#91414=CARTESIAN_POINT('Ctrl Pts',(44.5294175295214,16.5498237708003,20.));
#91415=CARTESIAN_POINT('Ctrl Pts',(44.5381446579761,16.5176961715269,0.));
#91416=CARTESIAN_POINT('Ctrl Pts',(44.5381446579761,16.5176961715269,20.));
#91417=CARTESIAN_POINT('Ctrl Pts',(44.5468490679154,16.4855635664567,0.));
#91418=CARTESIAN_POINT('Ctrl Pts',(44.5468490679154,16.4855635664567,20.));
#91419=CARTESIAN_POINT('Ctrl Pts',(44.5555307559385,16.4534259714715,0.));
#91420=CARTESIAN_POINT('Ctrl Pts',(44.5555307559385,16.4534259714715,20.));
#91421=CARTESIAN_POINT('Ctrl Pts',(44.5641897186557,16.4212834024559,0.));
#91422=CARTESIAN_POINT('Ctrl Pts',(44.5641897186557,16.4212834024559,20.));
#91423=CARTESIAN_POINT('Ctrl Pts',(44.5728259526889,16.3891358752972,0.));
#91424=CARTESIAN_POINT('Ctrl Pts',(44.5728259526889,16.3891358752972,20.));
#91425=CARTESIAN_POINT('Ctrl Pts',(44.581439454671,16.3569834058857,0.));
#91426=CARTESIAN_POINT('Ctrl Pts',(44.581439454671,16.3569834058857,20.));
#91427=CARTESIAN_POINT('Ctrl Pts',(44.5900302212458,16.3248260101143,0.));
#91428=CARTESIAN_POINT('Ctrl Pts',(44.5900302212458,16.3248260101143,20.));
#91429=CARTESIAN_POINT('Ctrl Pts',(44.5985982490682,16.2926637038787,0.));
#91430=CARTESIAN_POINT('Ctrl Pts',(44.5985982490682,16.2926637038787,20.));
#91431=CARTESIAN_POINT('Ctrl Pts',(44.6071435348036,16.2604965030773,0.));
#91432=CARTESIAN_POINT('Ctrl Pts',(44.6071435348036,16.2604965030773,20.));
#91433=CARTESIAN_POINT('Ctrl Pts',(44.6156660751288,16.2283244236112,0.));
#91434=CARTESIAN_POINT('Ctrl Pts',(44.6156660751288,16.2283244236112,20.));
#91435=CARTESIAN_POINT('Ctrl Pts',(44.6241658667307,16.196147481384,0.));
#91436=CARTESIAN_POINT('Ctrl Pts',(44.6241658667307,16.196147481384,20.));
#91437=CARTESIAN_POINT('Ctrl Pts',(44.6326429063072,16.1639656923023,0.));
#91438=CARTESIAN_POINT('Ctrl Pts',(44.6326429063072,16.1639656923023,20.));
#91439=CARTESIAN_POINT('Ctrl Pts',(44.6410971905673,16.131779072275,0.));
#91440=CARTESIAN_POINT('Ctrl Pts',(44.6410971905673,16.131779072275,20.));
#91441=CARTESIAN_POINT('Ctrl Pts',(44.649528716232,16.0995876372141,0.));
#91442=CARTESIAN_POINT('Ctrl Pts',(44.649528716232,16.0995876372141,20.));
#91443=CARTESIAN_POINT('Ctrl Pts',(44.6579374800339,16.0673914030343,0.));
#91444=CARTESIAN_POINT('Ctrl Pts',(44.6579374800339,16.0673914030343,20.));
#91445=CARTESIAN_POINT('Ctrl Pts',(44.6663234787169,16.0351903856534,0.));
#91446=CARTESIAN_POINT('Ctrl Pts',(44.6663234787169,16.0351903856534,20.));
#91447=CARTESIAN_POINT('Ctrl Pts',(44.6746867090345,16.0029846009915,0.));
#91448=CARTESIAN_POINT('Ctrl Pts',(44.6746867090345,16.0029846009915,20.));
#91449=CARTESIAN_POINT('Ctrl Pts',(44.6830271677516,15.9707740649715,0.));
#91450=CARTESIAN_POINT('Ctrl Pts',(44.6830271677516,15.9707740649715,20.));
#91451=CARTESIAN_POINT('Ctrl Pts',(44.691344851643,15.9385587935186,0.));
#91452=CARTESIAN_POINT('Ctrl Pts',(44.691344851643,15.9385587935186,20.));
#91453=CARTESIAN_POINT('Ctrl Pts',(44.6996397574952,15.9063388025603,0.));
#91454=CARTESIAN_POINT('Ctrl Pts',(44.6996397574952,15.9063388025603,20.));
#91455=CARTESIAN_POINT('Ctrl Pts',(44.7079118821065,15.8741141080272,0.));
#91456=CARTESIAN_POINT('Ctrl Pts',(44.7079118821065,15.8741141080272,20.));
#91457=CARTESIAN_POINT('Ctrl Pts',(44.7161612222865,15.8418847258528,0.));
#91458=CARTESIAN_POINT('Ctrl Pts',(44.7161612222865,15.8418847258528,20.));
#91459=CARTESIAN_POINT('Ctrl Pts',(44.7243877748558,15.8096506719735,0.));
#91460=CARTESIAN_POINT('Ctrl Pts',(44.7243877748558,15.8096506719735,20.));
#91461=CARTESIAN_POINT('Ctrl Pts',(44.7325915366458,15.7774119623278,0.));
#91462=CARTESIAN_POINT('Ctrl Pts',(44.7325915366458,15.7774119623278,20.));
#91463=CARTESIAN_POINT('Ctrl Pts',(44.7407725044985,15.745168612857,0.));
#91464=CARTESIAN_POINT('Ctrl Pts',(44.7407725044985,15.745168612857,20.));
#91465=CARTESIAN_POINT('Ctrl Pts',(44.7489306752664,15.7129206395047,0.));
#91466=CARTESIAN_POINT('Ctrl Pts',(44.7489306752664,15.7129206395047,20.));
#91467=CARTESIAN_POINT('Ctrl Pts',(44.7570660458133,15.6806680582172,0.));
#91468=CARTESIAN_POINT('Ctrl Pts',(44.7570660458133,15.6806680582172,20.));
#91469=CARTESIAN_POINT('Ctrl Pts',(44.7651786130144,15.6484108849434,0.));
#91470=CARTESIAN_POINT('Ctrl Pts',(44.7651786130144,15.6484108849434,20.));
#91471=CARTESIAN_POINT('Ctrl Pts',(44.7732683737566,15.6161491356348,0.));
#91472=CARTESIAN_POINT('Ctrl Pts',(44.7732683737566,15.6161491356348,20.));
#91473=CARTESIAN_POINT('Ctrl Pts',(44.7813353249379,15.583882826246,0.));
#91474=CARTESIAN_POINT('Ctrl Pts',(44.7813353249379,15.583882826246,20.));
#91475=CARTESIAN_POINT('Ctrl Pts',(44.7893794634672,15.5516119727338,0.));
#91476=CARTESIAN_POINT('Ctrl Pts',(44.7893794634672,15.5516119727338,20.));
#91477=CARTESIAN_POINT('Ctrl Pts',(44.7974007862643,15.5193365910578,0.));
#91478=CARTESIAN_POINT('Ctrl Pts',(44.7974007862643,15.5193365910578,20.));
#91479=CARTESIAN_POINT('Ctrl Pts',(44.8053992902599,15.4870566971799,0.));
#91480=CARTESIAN_POINT('Ctrl Pts',(44.8053992902599,15.4870566971799,20.));
#91481=CARTESIAN_POINT('Ctrl Pts',(44.8133749723964,15.4547723070643,0.));
#91482=CARTESIAN_POINT('Ctrl Pts',(44.8133749723964,15.4547723070643,20.));
#91483=CARTESIAN_POINT('Ctrl Pts',(44.8213278296263,15.4224834366782,0.));
#91484=CARTESIAN_POINT('Ctrl Pts',(44.8213278296263,15.4224834366782,20.));
#91485=CARTESIAN_POINT('Ctrl Pts',(44.8292578589132,15.3901901019906,0.));
#91486=CARTESIAN_POINT('Ctrl Pts',(44.8292578589132,15.3901901019906,20.));
#91487=CARTESIAN_POINT('Ctrl Pts',(44.8371650572316,15.3578923189739,0.));
#91488=CARTESIAN_POINT('Ctrl Pts',(44.8371650572316,15.3578923189739,20.));
#91489=CARTESIAN_POINT('Ctrl Pts',(44.8450494215678,15.3255901036026,0.));
#91490=CARTESIAN_POINT('Ctrl Pts',(44.8450494215678,15.3255901036026,20.));
#91491=CARTESIAN_POINT('Ctrl Pts',(44.8529109489191,15.2932834718541,0.));
#91492=CARTESIAN_POINT('Ctrl Pts',(44.8529109489191,15.2932834718541,20.));
#91493=CARTESIAN_POINT('Ctrl Pts',(44.8607496362943,15.2609724397079,0.));
#91494=CARTESIAN_POINT('Ctrl Pts',(44.8607496362943,15.2609724397079,20.));
#91495=CARTESIAN_POINT('Ctrl Pts',(44.8685654807131,15.2286570231461,0.));
#91496=CARTESIAN_POINT('Ctrl Pts',(44.8685654807131,15.2286570231461,20.));
#91497=CARTESIAN_POINT('Ctrl Pts',(44.8763584792064,15.1963372381533,0.));
#91498=CARTESIAN_POINT('Ctrl Pts',(44.8763584792064,15.1963372381533,20.));
#91499=CARTESIAN_POINT('Ctrl Pts',(44.8841286288163,15.1640131007166,0.));
#91500=CARTESIAN_POINT('Ctrl Pts',(44.8841286288163,15.1640131007166,20.));
#91501=CARTESIAN_POINT('Ctrl Pts',(44.8918759265956,15.1316846268256,0.));
#91502=CARTESIAN_POINT('Ctrl Pts',(44.8918759265956,15.1316846268256,20.));
#91503=CARTESIAN_POINT('Ctrl Pts',(44.8996003696078,15.0993518324721,0.));
#91504=CARTESIAN_POINT('Ctrl Pts',(44.8996003696078,15.0993518324721,20.));
#91505=CARTESIAN_POINT('Ctrl Pts',(44.9073019549277,15.0670147336509,0.));
#91506=CARTESIAN_POINT('Ctrl Pts',(44.9073019549277,15.0670147336509,20.));
#91507=CARTESIAN_POINT('Ctrl Pts',(44.9149806796409,15.034673346359,0.));
#91508=CARTESIAN_POINT('Ctrl Pts',(44.9149806796409,15.034673346359,20.));
#91509=CARTESIAN_POINT('Ctrl Pts',(44.9226365408441,15.0023276865958,0.));
#91510=CARTESIAN_POINT('Ctrl Pts',(44.9226365408441,15.0023276865958,20.));
#91511=CARTESIAN_POINT('Ctrl Pts',(44.9302695356455,14.969977770363,0.));
#91512=CARTESIAN_POINT('Ctrl Pts',(44.9302695356455,14.969977770363,20.));
#91513=CARTESIAN_POINT('Ctrl Pts',(44.9378796611651,14.9376236136649,0.));
#91514=CARTESIAN_POINT('Ctrl Pts',(44.9378796611651,14.9376236136649,20.));
#91515=CARTESIAN_POINT('Ctrl Pts',(44.9454669145344,14.9052652325081,0.));
#91516=CARTESIAN_POINT('Ctrl Pts',(44.9454669145344,14.9052652325081,20.));
#91517=CARTESIAN_POINT('Ctrl Pts',(44.9530312928957,14.8729026429019,0.));
#91518=CARTESIAN_POINT('Ctrl Pts',(44.9530312928957,14.8729026429019,20.));
#91519=CARTESIAN_POINT('Ctrl Pts',(44.9605727934022,14.8405358608577,0.));
#91520=CARTESIAN_POINT('Ctrl Pts',(44.9605727934022,14.8405358608577,20.));
#91521=CARTESIAN_POINT('Ctrl Pts',(44.9680914132176,14.8081649023895,0.));
#91522=CARTESIAN_POINT('Ctrl Pts',(44.9680914132176,14.8081649023895,20.));
#91523=CARTESIAN_POINT('Ctrl Pts',(44.9755871495162,14.7757897835134,0.));
#91524=CARTESIAN_POINT('Ctrl Pts',(44.9755871495162,14.7757897835134,20.));
#91525=CARTESIAN_POINT('Ctrl Pts',(44.9830599994838,14.7434105202483,0.));
#91526=CARTESIAN_POINT('Ctrl Pts',(44.9830599994838,14.7434105202483,20.));
#91527=CARTESIAN_POINT('Ctrl Pts',(44.9905099603172,14.7110271286153,0.));
#91528=CARTESIAN_POINT('Ctrl Pts',(44.9905099603172,14.7110271286153,20.));
#91529=CARTESIAN_POINT('Ctrl Pts',(44.9979370292252,14.6786396246378,0.));
#91530=CARTESIAN_POINT('Ctrl Pts',(44.9979370292252,14.6786396246378,20.));
#91531=CARTESIAN_POINT('Ctrl Pts',(45.0053412034276,14.6462480243418,0.));
#91532=CARTESIAN_POINT('Ctrl Pts',(45.0053412034276,14.6462480243418,20.));
#91533=CARTESIAN_POINT('Ctrl Pts',(45.0127224801553,14.6138523437553,0.));
#91534=CARTESIAN_POINT('Ctrl Pts',(45.0127224801553,14.6138523437553,20.));
#91535=CARTESIAN_POINT('Ctrl Pts',(45.020080856651,14.5814525989087,0.));
#91536=CARTESIAN_POINT('Ctrl Pts',(45.020080856651,14.5814525989087,20.));
#91537=CARTESIAN_POINT('Ctrl Pts',(45.0274163301681,14.5490488058349,0.));
#91538=CARTESIAN_POINT('Ctrl Pts',(45.0274163301681,14.5490488058349,20.));
#91539=CARTESIAN_POINT('Ctrl Pts',(45.0347288979708,14.516640980569,0.));
#91540=CARTESIAN_POINT('Ctrl Pts',(45.0347288979708,14.516640980569,20.));
#91541=CARTESIAN_POINT('Ctrl Pts',(45.0420185573341,14.4842291391484,0.));
#91542=CARTESIAN_POINT('Ctrl Pts',(45.0420185573341,14.4842291391484,20.));
#91543=CARTESIAN_POINT('Ctrl Pts',(45.0492853055441,14.451813297613,0.));
#91544=CARTESIAN_POINT('Ctrl Pts',(45.0492853055441,14.451813297613,20.));
#91545=CARTESIAN_POINT('Ctrl Pts',(45.0565291398984,14.4193934720051,0.));
#91546=CARTESIAN_POINT('Ctrl Pts',(45.0565291398984,14.4193934720051,20.));
#91547=CARTESIAN_POINT('Ctrl Pts',(45.0637500577056,14.3869696783692,0.));
#91548=CARTESIAN_POINT('Ctrl Pts',(45.0637500577056,14.3869696783692,20.));
#91549=CARTESIAN_POINT('Ctrl Pts',(45.0709480562863,14.354541932752,0.));
#91550=CARTESIAN_POINT('Ctrl Pts',(45.0709480562863,14.354541932752,20.));
#91551=CARTESIAN_POINT('Ctrl Pts',(45.0781231329719,14.3221102512025,0.));
#91552=CARTESIAN_POINT('Ctrl Pts',(45.0781231329719,14.3221102512025,20.));
#91553=CARTESIAN_POINT('Ctrl Pts',(45.0852752851048,14.2896746497719,0.));
#91554=CARTESIAN_POINT('Ctrl Pts',(45.0852752851048,14.2896746497719,20.));
#91555=CARTESIAN_POINT('Ctrl Pts',(45.0924045100383,14.2572351445137,0.));
#91556=CARTESIAN_POINT('Ctrl Pts',(45.0924045100383,14.2572351445137,20.));
#91557=CARTESIAN_POINT('Ctrl Pts',(45.0995108051367,14.2247917514836,0.));
#91558=CARTESIAN_POINT('Ctrl Pts',(45.0995108051367,14.2247917514836,20.));
#91559=CARTESIAN_POINT('Ctrl Pts',(45.1065941677758,14.1923444867396,0.));
#91560=CARTESIAN_POINT('Ctrl Pts',(45.1065941677758,14.1923444867396,20.));
#91561=CARTESIAN_POINT('Ctrl Pts',(45.1136545953429,14.1598933663423,0.));
#91562=CARTESIAN_POINT('Ctrl Pts',(45.1136545953429,14.1598933663423,20.));
#91563=CARTESIAN_POINT('Ctrl Pts',(45.1206920852361,14.127438406354,0.));
#91564=CARTESIAN_POINT('Ctrl Pts',(45.1206920852361,14.127438406354,20.));
#91565=CARTESIAN_POINT('Ctrl Pts',(45.127706634865,14.0949796228398,0.));
#91566=CARTESIAN_POINT('Ctrl Pts',(45.127706634865,14.0949796228398,20.));
#91567=CARTESIAN_POINT('Ctrl Pts',(45.1346982416501,14.0625170318665,0.));
#91568=CARTESIAN_POINT('Ctrl Pts',(45.1346982416501,14.0625170318665,20.));
#91569=CARTESIAN_POINT('Ctrl Pts',(45.1416669030232,14.0300506495033,0.));
#91570=CARTESIAN_POINT('Ctrl Pts',(45.1416669030232,14.0300506495033,20.));
#91571=CARTESIAN_POINT('Ctrl Pts',(45.1486126164275,13.997580491822,0.));
#91572=CARTESIAN_POINT('Ctrl Pts',(45.1486126164275,13.997580491822,20.));
#91573=CARTESIAN_POINT('Ctrl Pts',(45.1555353793172,13.9651065748961,0.));
#91574=CARTESIAN_POINT('Ctrl Pts',(45.1555353793172,13.9651065748961,20.));
#91575=CARTESIAN_POINT('Ctrl Pts',(45.1624351891574,13.9326289148012,0.));
#91576=CARTESIAN_POINT('Ctrl Pts',(45.1624351891574,13.9326289148012,20.));
#91577=CARTESIAN_POINT('Ctrl Pts',(45.1693120434241,13.9001475276153,0.));
#91578=CARTESIAN_POINT('Ctrl Pts',(45.1693120434241,13.9001475276153,20.));
#91579=CARTESIAN_POINT('Ctrl Pts',(45.1761659396043,13.8676624294184,0.));
#91580=CARTESIAN_POINT('Ctrl Pts',(45.1761659396043,13.8676624294184,20.));
#91581=CARTESIAN_POINT('Ctrl Pts',(45.1829968751969,13.8351736362929,0.));
#91582=CARTESIAN_POINT('Ctrl Pts',(45.1829968751969,13.8351736362929,20.));
#91583=CARTESIAN_POINT('Ctrl Pts',(45.1898048477123,13.8026811643234,0.));
#91584=CARTESIAN_POINT('Ctrl Pts',(45.1898048477123,13.8026811643234,20.));
#91585=CARTESIAN_POINT('Ctrl Pts',(45.1965898546723,13.7701850295968,0.));
#91586=CARTESIAN_POINT('Ctrl Pts',(45.1965898546723,13.7701850295968,20.));
#91587=CARTESIAN_POINT('Ctrl Pts',(45.2033518936101,13.7376852482019,0.));
#91588=CARTESIAN_POINT('Ctrl Pts',(45.2033518936101,13.7376852482019,20.));
#91589=CARTESIAN_POINT('Ctrl Pts',(45.2100909620697,13.7051818362299,0.));
#91590=CARTESIAN_POINT('Ctrl Pts',(45.2100909620697,13.7051818362299,20.));
#91591=CARTESIAN_POINT('Ctrl Pts',(45.2168070576061,13.6726748097738,0.));
#91592=CARTESIAN_POINT('Ctrl Pts',(45.2168070576061,13.6726748097738,20.));
#91593=CARTESIAN_POINT('Ctrl Pts',(45.2235001777847,13.6401641849286,0.));
#91594=CARTESIAN_POINT('Ctrl Pts',(45.2235001777847,13.6401641849286,20.));
#91595=CARTESIAN_POINT('Ctrl Pts',(45.2301703201819,13.6076499777915,0.));
#91596=CARTESIAN_POINT('Ctrl Pts',(45.2301703201819,13.6076499777915,20.));
#91597=CARTESIAN_POINT('Ctrl Pts',(45.2368174823856,13.5751322044618,0.));
#91598=CARTESIAN_POINT('Ctrl Pts',(45.2368174823856,13.5751322044618,20.));
#91599=CARTESIAN_POINT('Ctrl Pts',(45.2434416619952,13.542610881041,0.));
#91600=CARTESIAN_POINT('Ctrl Pts',(45.2434416619952,13.542610881041,20.));
#91601=CARTESIAN_POINT('Ctrl Pts',(45.2500428566225,13.5100860236329,0.));
#91602=CARTESIAN_POINT('Ctrl Pts',(45.2500428566225,13.5100860236329,20.));
#91603=CARTESIAN_POINT('Ctrl Pts',(45.2566210638904,13.4775576483433,0.));
#91604=CARTESIAN_POINT('Ctrl Pts',(45.2566210638904,13.4775576483433,20.));
#91605=CARTESIAN_POINT('Ctrl Pts',(45.2631762814325,13.44502577128,0.));
#91606=CARTESIAN_POINT('Ctrl Pts',(45.2631762814325,13.44502577128,20.));
#91607=CARTESIAN_POINT('Ctrl Pts',(45.2697085068935,13.4124904085531,0.));
#91608=CARTESIAN_POINT('Ctrl Pts',(45.2697085068935,13.4124904085531,20.));
#91609=CARTESIAN_POINT('Ctrl Pts',(45.276217737929,13.3799515762744,0.));
#91610=CARTESIAN_POINT('Ctrl Pts',(45.276217737929,13.3799515762744,20.));
#91611=CARTESIAN_POINT('Ctrl Pts',(45.2827039722059,13.3474092905576,0.));
#91612=CARTESIAN_POINT('Ctrl Pts',(45.2827039722059,13.3474092905576,20.));
#91613=CARTESIAN_POINT('Ctrl Pts',(45.2891672074022,13.3148635675188,0.));
#91614=CARTESIAN_POINT('Ctrl Pts',(45.2891672074022,13.3148635675188,20.));
#91615=CARTESIAN_POINT('Ctrl Pts',(45.2956074412073,13.282314423276,0.));
#91616=CARTESIAN_POINT('Ctrl Pts',(45.2956074412073,13.282314423276,20.));
#91617=CARTESIAN_POINT('Ctrl Pts',(45.3020246713218,13.2497618739494,0.));
#91618=CARTESIAN_POINT('Ctrl Pts',(45.3020246713218,13.2497618739494,20.));
#91619=CARTESIAN_POINT('Ctrl Pts',(45.3084188954577,13.217205935661,0.));
#91620=CARTESIAN_POINT('Ctrl Pts',(45.3084188954577,13.217205935661,20.));
#91621=CARTESIAN_POINT('Ctrl Pts',(45.3147901113387,13.1846466245352,0.));
#91622=CARTESIAN_POINT('Ctrl Pts',(45.3147901113387,13.1846466245352,20.));
#91623=CARTESIAN_POINT('Ctrl Pts',(45.321138316699,13.1520839566979,0.));
#91624=CARTESIAN_POINT('Ctrl Pts',(45.321138316699,13.1520839566979,20.));
#91625=CARTESIAN_POINT('Ctrl Pts',(45.3274635092846,13.1195179482773,0.));
#91626=CARTESIAN_POINT('Ctrl Pts',(45.3274635092846,13.1195179482773,20.));
#91627=CARTESIAN_POINT('Ctrl Pts',(45.3337656868523,13.0869486154035,0.));
#91628=CARTESIAN_POINT('Ctrl Pts',(45.3337656868523,13.0869486154035,20.));
#91629=CARTESIAN_POINT('Ctrl Pts',(45.3400448471699,13.0543759742083,0.));
#91630=CARTESIAN_POINT('Ctrl Pts',(45.3400448471699,13.0543759742083,20.));
#91631=CARTESIAN_POINT('Ctrl Pts',(45.3463009880171,13.021800040826,0.));
#91632=CARTESIAN_POINT('Ctrl Pts',(45.3463009880171,13.021800040826,20.));
#91633=CARTESIAN_POINT('Ctrl Pts',(45.3525341071849,12.9892208313927,0.));
#91634=CARTESIAN_POINT('Ctrl Pts',(45.3525341071849,12.9892208313927,20.));
#91635=CARTESIAN_POINT('Ctrl Pts',(45.3587442024753,12.9566383620464,0.));
#91636=CARTESIAN_POINT('Ctrl Pts',(45.3587442024753,12.9566383620464,20.));
#91637=CARTESIAN_POINT('Ctrl Pts',(45.364931271701,12.9240526489273,0.));
#91638=CARTESIAN_POINT('Ctrl Pts',(45.364931271701,12.9240526489273,20.));
#91639=CARTESIAN_POINT('Ctrl Pts',(45.371095312686,12.8914637081769,0.));
#91640=CARTESIAN_POINT('Ctrl Pts',(45.371095312686,12.8914637081769,20.));
#91641=CARTESIAN_POINT('Ctrl Pts',(45.3772363232658,12.8588715559393,0.));
#91642=CARTESIAN_POINT('Ctrl Pts',(45.3772363232658,12.8588715559393,20.));
#91643=CARTESIAN_POINT('Ctrl Pts',(45.3833543012877,12.82627620836,0.));
#91644=CARTESIAN_POINT('Ctrl Pts',(45.3833543012877,12.82627620836,20.));
#91645=CARTESIAN_POINT('Ctrl Pts',(45.3894492446102,12.7936776815868,0.));
#91646=CARTESIAN_POINT('Ctrl Pts',(45.3894492446102,12.7936776815868,20.));
#91647=CARTESIAN_POINT('Ctrl Pts',(45.3955211511033,12.7610759917694,0.));
#91648=CARTESIAN_POINT('Ctrl Pts',(45.3955211511033,12.7610759917694,20.));
#91649=CARTESIAN_POINT('Ctrl Pts',(45.4015700186485,12.7284711550592,0.));
#91650=CARTESIAN_POINT('Ctrl Pts',(45.4015700186485,12.7284711550592,20.));
#91651=CARTESIAN_POINT('Ctrl Pts',(45.407595845137,12.6958631876099,0.));
#91652=CARTESIAN_POINT('Ctrl Pts',(45.407595845137,12.6958631876099,20.));
#91653=CARTESIAN_POINT('Ctrl Pts',(45.4135986284717,12.6632521055766,0.));
#91654=CARTESIAN_POINT('Ctrl Pts',(45.4135986284717,12.6632521055766,20.));
#91655=CARTESIAN_POINT('Ctrl Pts',(45.4195783665665,12.6306379251165,0.));
#91656=CARTESIAN_POINT('Ctrl Pts',(45.4195783665665,12.6306379251165,20.));
#91657=CARTESIAN_POINT('Ctrl Pts',(45.4255350573473,12.5980206623884,0.));
#91658=CARTESIAN_POINT('Ctrl Pts',(45.4255350573473,12.5980206623884,20.));
#91659=CARTESIAN_POINT('Ctrl Pts',(45.4314686987515,12.5654003335533,0.));
#91660=CARTESIAN_POINT('Ctrl Pts',(45.4314686987515,12.5654003335533,20.));
#91661=CARTESIAN_POINT('Ctrl Pts',(45.4373792887274,12.5327769547739,0.));
#91662=CARTESIAN_POINT('Ctrl Pts',(45.4373792887274,12.5327769547739,20.));
#91663=CARTESIAN_POINT('Ctrl Pts',(45.4432668252347,12.500150542215,0.));
#91664=CARTESIAN_POINT('Ctrl Pts',(45.4432668252347,12.500150542215,20.));
#91665=CARTESIAN_POINT('Ctrl Pts',(45.4491313062444,12.4675211120431,0.));
#91666=CARTESIAN_POINT('Ctrl Pts',(45.4491313062444,12.4675211120431,20.));
#91667=CARTESIAN_POINT('Ctrl Pts',(45.4549727297392,12.4348886804266,0.));
#91668=CARTESIAN_POINT('Ctrl Pts',(45.4549727297392,12.4348886804266,20.));
#91669=CARTESIAN_POINT('Ctrl Pts',(45.4607910937128,12.4022532635357,0.));
#91670=CARTESIAN_POINT('Ctrl Pts',(45.4607910937128,12.4022532635357,20.));
#91671=CARTESIAN_POINT('Ctrl Pts',(45.4665863961701,12.3696148775423,0.));
#91672=CARTESIAN_POINT('Ctrl Pts',(45.4665863961701,12.3696148775423,20.));
#91673=CARTESIAN_POINT('Ctrl Pts',(45.4723586351267,12.3369735386201,0.));
#91674=CARTESIAN_POINT('Ctrl Pts',(45.4723586351267,12.3369735386201,20.));
#91675=CARTESIAN_POINT('Ctrl Pts',(45.4781078086095,12.3043292629445,0.));
#91676=CARTESIAN_POINT('Ctrl Pts',(45.4781078086095,12.3043292629445,20.));
#91677=CARTESIAN_POINT('Ctrl Pts',(45.483833914657,12.2716820666929,0.));
#91678=CARTESIAN_POINT('Ctrl Pts',(45.483833914657,12.2716820666929,20.));
#91679=CARTESIAN_POINT('Ctrl Pts',(45.4895369513189,12.2390319660445,0.));
#91680=CARTESIAN_POINT('Ctrl Pts',(45.4895369513189,12.2390319660445,20.));
#91681=CARTESIAN_POINT('Ctrl Pts',(45.4952169166561,12.2063789771801,0.));
#91682=CARTESIAN_POINT('Ctrl Pts',(45.4952169166561,12.2063789771801,20.));
#91683=CARTESIAN_POINT('Ctrl Pts',(45.5008738087416,12.1737231162825,0.));
#91684=CARTESIAN_POINT('Ctrl Pts',(45.5008738087416,12.1737231162825,20.));
#91685=CARTESIAN_POINT('Ctrl Pts',(45.5065076256599,12.1410643995363,0.));
#91686=CARTESIAN_POINT('Ctrl Pts',(45.5065076256599,12.1410643995363,20.));
#91687=CARTESIAN_POINT('Ctrl Pts',(45.5121183655068,12.1084028431278,0.));
#91688=CARTESIAN_POINT('Ctrl Pts',(45.5121183655068,12.1084028431278,20.));
#91689=CARTESIAN_POINT('Ctrl Pts',(45.5177060263888,12.0757384632451,0.));
#91690=CARTESIAN_POINT('Ctrl Pts',(45.5177060263888,12.0757384632451,20.));
#91691=CARTESIAN_POINT('Ctrl Pts',(45.5232706064237,12.0430712760779,0.));
#91692=CARTESIAN_POINT('Ctrl Pts',(45.5232706064237,12.0430712760779,20.));
#91693=CARTESIAN_POINT('Ctrl Pts',(45.5288121037394,12.0104012978174,0.));
#91694=CARTESIAN_POINT('Ctrl Pts',(45.5288121037394,12.0104012978174,20.));
#91695=CARTESIAN_POINT('Ctrl Pts',(45.5343305164759,11.9777285446569,0.));
#91696=CARTESIAN_POINT('Ctrl Pts',(45.5343305164759,11.9777285446569,20.));
#91697=CARTESIAN_POINT('Ctrl Pts',(45.5398258427844,11.9450530327911,0.));
#91698=CARTESIAN_POINT('Ctrl Pts',(45.5398258427844,11.9450530327911,20.));
#91699=CARTESIAN_POINT('Ctrl Pts',(45.5452980808284,11.9123747784165,0.));
#91700=CARTESIAN_POINT('Ctrl Pts',(45.5452980808284,11.9123747784165,20.));
#91701=CARTESIAN_POINT('Ctrl Pts',(45.5507472287824,11.8796937977314,0.));
#91702=CARTESIAN_POINT('Ctrl Pts',(45.5507472287824,11.8796937977314,20.));
#91703=CARTESIAN_POINT('Ctrl Pts',(45.5561732848327,11.8470101069358,0.));
#91704=CARTESIAN_POINT('Ctrl Pts',(45.5561732848327,11.8470101069358,20.));
#91705=CARTESIAN_POINT('Ctrl Pts',(45.5615762471761,11.8143237222317,0.));
#91706=CARTESIAN_POINT('Ctrl Pts',(45.5615762471761,11.8143237222317,20.));
#91707=CARTESIAN_POINT('Ctrl Pts',(45.5669561140206,11.7816346598227,0.));
#91708=CARTESIAN_POINT('Ctrl Pts',(45.5669561140206,11.7816346598227,20.));
#91709=CARTESIAN_POINT('Ctrl Pts',(45.5723128835857,11.748942935914,0.));
#91710=CARTESIAN_POINT('Ctrl Pts',(45.5723128835857,11.748942935914,20.));
#91711=CARTESIAN_POINT('Ctrl Pts',(45.5776465541021,11.7162485667124,0.));
#91712=CARTESIAN_POINT('Ctrl Pts',(45.5776465541021,11.7162485667124,20.));
#91713=CARTESIAN_POINT('Ctrl Pts',(45.5829571238122,11.6835515684258,0.));
#91714=CARTESIAN_POINT('Ctrl Pts',(45.5829571238122,11.6835515684258,20.));
#91715=CARTESIAN_POINT('Ctrl Pts',(45.5882445909695,11.6508519572639,0.));
#91716=CARTESIAN_POINT('Ctrl Pts',(45.5882445909695,11.6508519572639,20.));
#91717=CARTESIAN_POINT('Ctrl Pts',(45.5935089538387,11.6181497494382,0.));
#91718=CARTESIAN_POINT('Ctrl Pts',(45.5935089538387,11.6181497494382,20.));
#91719=CARTESIAN_POINT('Ctrl Pts',(45.598750210696,11.5854449611619,0.));
#91720=CARTESIAN_POINT('Ctrl Pts',(45.598750210696,11.5854449611619,20.));
#91721=CARTESIAN_POINT('Ctrl Pts',(45.6039683598295,11.5527376086502,0.));
#91722=CARTESIAN_POINT('Ctrl Pts',(45.6039683598295,11.5527376086502,20.));
#91723=CARTESIAN_POINT('Ctrl Pts',(45.6091633995383,11.5200277081201,0.));
#91724=CARTESIAN_POINT('Ctrl Pts',(45.6091633995383,11.5200277081201,20.));
#91725=CARTESIAN_POINT('Ctrl Pts',(45.6143353281323,11.4873152757897,0.));
#91726=CARTESIAN_POINT('Ctrl Pts',(45.6143353281323,11.4873152757897,20.));
#91727=CARTESIAN_POINT('Ctrl Pts',(45.6194841439321,11.4546003278786,0.));
#91728=CARTESIAN_POINT('Ctrl Pts',(45.6194841439321,11.4546003278786,20.));
#91729=CARTESIAN_POINT('Ctrl Pts',(45.6246098452703,11.421882880608,0.));
#91730=CARTESIAN_POINT('Ctrl Pts',(45.6246098452703,11.421882880608,20.));
#91731=CARTESIAN_POINT('Ctrl Pts',(45.6297124304911,11.3891629502006,0.));
#91732=CARTESIAN_POINT('Ctrl Pts',(45.6297124304911,11.3891629502006,20.));
#91733=CARTESIAN_POINT('Ctrl Pts',(45.6347918979506,11.3564405528809,0.));
#91734=CARTESIAN_POINT('Ctrl Pts',(45.6347918979506,11.3564405528809,20.));
#91735=CARTESIAN_POINT('Ctrl Pts',(45.6398482460165,11.3237157048751,0.));
#91736=CARTESIAN_POINT('Ctrl Pts',(45.6398482460165,11.3237157048751,20.));
#91737=CARTESIAN_POINT('Ctrl Pts',(45.6448814730676,11.290988422411,0.));
#91738=CARTESIAN_POINT('Ctrl Pts',(45.6448814730676,11.290988422411,20.));
#91739=CARTESIAN_POINT('Ctrl Pts',(45.6498915774933,11.2582587217178,0.));
#91740=CARTESIAN_POINT('Ctrl Pts',(45.6498915774933,11.2582587217178,20.));
#91741=CARTESIAN_POINT('Ctrl Pts',(45.6548785576938,11.2255266190259,0.));
#91742=CARTESIAN_POINT('Ctrl Pts',(45.6548785576938,11.2255266190259,20.));
#91743=CARTESIAN_POINT('Ctrl Pts',(45.6598424120808,11.1927921305675,0.));
#91744=CARTESIAN_POINT('Ctrl Pts',(45.6598424120808,11.1927921305675,20.));
#91745=CARTESIAN_POINT('Ctrl Pts',(45.6647831390778,11.1600552725764,0.));
#91746=CARTESIAN_POINT('Ctrl Pts',(45.6647831390778,11.1600552725764,20.));
#91747=CARTESIAN_POINT('Ctrl Pts',(45.6697007371202,11.1273160612881,0.));
#91748=CARTESIAN_POINT('Ctrl Pts',(45.6697007371202,11.1273160612881,20.));
#91749=CARTESIAN_POINT('Ctrl Pts',(45.6745952046549,11.0945745129393,0.));
#91750=CARTESIAN_POINT('Ctrl Pts',(45.6745952046549,11.0945745129393,20.));
#91751=CARTESIAN_POINT('Ctrl Pts',(45.6794665401395,11.0618306437685,0.));
#91752=CARTESIAN_POINT('Ctrl Pts',(45.6794665401395,11.0618306437685,20.));
#91753=CARTESIAN_POINT('Ctrl Pts',(45.684314742043,11.0290844700154,0.));
#91754=CARTESIAN_POINT('Ctrl Pts',(45.684314742043,11.0290844700154,20.));
#91755=CARTESIAN_POINT('Ctrl Pts',(45.6891398088456,10.9963360079212,0.));
#91756=CARTESIAN_POINT('Ctrl Pts',(45.6891398088456,10.9963360079212,20.));
#91757=CARTESIAN_POINT('Ctrl Pts',(45.6939417390393,10.9635852737287,0.));
#91758=CARTESIAN_POINT('Ctrl Pts',(45.6939417390393,10.9635852737287,20.));
#91759=CARTESIAN_POINT('Ctrl Pts',(45.698720531127,10.930832283682,0.));
#91760=CARTESIAN_POINT('Ctrl Pts',(45.698720531127,10.930832283682,20.));
#91761=CARTESIAN_POINT('Ctrl Pts',(45.7034761836229,10.898077054027,0.));
#91762=CARTESIAN_POINT('Ctrl Pts',(45.7034761836229,10.898077054027,20.));
#91763=CARTESIAN_POINT('Ctrl Pts',(45.7082086950532,10.8653196010107,0.));
#91764=CARTESIAN_POINT('Ctrl Pts',(45.7082086950532,10.8653196010107,20.));
#91765=CARTESIAN_POINT('Ctrl Pts',(45.7129180639558,10.832559940882,0.));
#91766=CARTESIAN_POINT('Ctrl Pts',(45.7129180639558,10.832559940882,20.));
#91767=CARTESIAN_POINT('Ctrl Pts',(45.7176042888794,10.7997980898913,0.));
#91768=CARTESIAN_POINT('Ctrl Pts',(45.7176042888794,10.7997980898913,20.));
#91769=CARTESIAN_POINT('Ctrl Pts',(45.7222673683833,10.7670340642896,0.));
#91770=CARTESIAN_POINT('Ctrl Pts',(45.7222673683833,10.7670340642896,20.));
#91771=CARTESIAN_POINT('Ctrl Pts',(45.7269073010391,10.73426788033,0.));
#91772=CARTESIAN_POINT('Ctrl Pts',(45.7269073010391,10.73426788033,20.));
#91773=CARTESIAN_POINT('Ctrl Pts',(45.7315240854293,10.7014995542666,0.));
#91774=CARTESIAN_POINT('Ctrl Pts',(45.7315240854293,10.7014995542666,20.));
#91775=CARTESIAN_POINT('Ctrl Pts',(45.7361177201484,10.6687291023553,0.));
#91776=CARTESIAN_POINT('Ctrl Pts',(45.7361177201484,10.6687291023553,20.));
#91777=CARTESIAN_POINT('Ctrl Pts',(45.7406882038015,10.6359565408533,0.));
#91778=CARTESIAN_POINT('Ctrl Pts',(45.7406882038015,10.6359565408533,20.));
#91779=CARTESIAN_POINT('Ctrl Pts',(45.745235535006,10.6031818860194,0.));
#91780=CARTESIAN_POINT('Ctrl Pts',(45.745235535006,10.6031818860194,20.));
#91781=CARTESIAN_POINT('Ctrl Pts',(45.7497597123901,10.5704051541135,0.));
#91782=CARTESIAN_POINT('Ctrl Pts',(45.7497597123901,10.5704051541135,20.));
#91783=CARTESIAN_POINT('Ctrl Pts',(45.7542607345937,10.5376263613969,0.));
#91784=CARTESIAN_POINT('Ctrl Pts',(45.7542607345937,10.5376263613969,20.));
#91785=CARTESIAN_POINT('Ctrl Pts',(45.7587386002674,10.504845524132,0.));
#91786=CARTESIAN_POINT('Ctrl Pts',(45.7587386002674,10.504845524132,20.));
#91787=CARTESIAN_POINT('Ctrl Pts',(45.7631933080735,10.4720626585828,0.));
#91788=CARTESIAN_POINT('Ctrl Pts',(45.7631933080735,10.4720626585828,20.));
#91789=CARTESIAN_POINT('Ctrl Pts',(45.7676248566855,10.4392777810149,0.));
#91790=CARTESIAN_POINT('Ctrl Pts',(45.7676248566855,10.4392777810149,20.));
#91791=CARTESIAN_POINT('Ctrl Pts',(45.772033244789,10.406490907695,0.));
#91792=CARTESIAN_POINT('Ctrl Pts',(45.772033244789,10.406490907695,20.));
#91793=CARTESIAN_POINT('Ctrl Pts',(45.7764184710811,10.3737020548914,0.));
#91794=CARTESIAN_POINT('Ctrl Pts',(45.7764184710811,10.3737020548914,20.));
#91795=CARTESIAN_POINT('Ctrl Pts',(45.7807805342697,10.3409112388736,0.));
#91796=CARTESIAN_POINT('Ctrl Pts',(45.7807805342697,10.3409112388736,20.));
#91797=CARTESIAN_POINT('Ctrl Pts',(45.7851194330743,10.3081184759123,0.));
#91798=CARTESIAN_POINT('Ctrl Pts',(45.7851194330743,10.3081184759123,20.));
#91799=CARTESIAN_POINT('Ctrl Pts',(45.7894351662253,10.2753237822796,0.));
#91800=CARTESIAN_POINT('Ctrl Pts',(45.7894351662253,10.2753237822796,20.));
#91801=CARTESIAN_POINT('Ctrl Pts',(45.7937277324642,10.2425271742485,0.));
#91802=CARTESIAN_POINT('Ctrl Pts',(45.7937277324642,10.2425271742485,20.));
#91803=CARTESIAN_POINT('Ctrl Pts',(45.7979971305449,10.2097286680937,0.));
#91804=CARTESIAN_POINT('Ctrl Pts',(45.7979971305449,10.2097286680937,20.));
#91805=CARTESIAN_POINT('Ctrl Pts',(45.8022433592327,10.1769282800914,0.));
#91806=CARTESIAN_POINT('Ctrl Pts',(45.8022433592327,10.1769282800914,20.));
#91807=CARTESIAN_POINT('Ctrl Pts',(45.8064664173048,10.1441260265191,0.));
#91808=CARTESIAN_POINT('Ctrl Pts',(45.8064664173048,10.1441260265191,20.));
#91809=CARTESIAN_POINT('Ctrl Pts',(45.8106663035491,10.1113219236554,0.));
#91810=CARTESIAN_POINT('Ctrl Pts',(45.8106663035491,10.1113219236554,20.));
#91811=CARTESIAN_POINT('Ctrl Pts',(45.8148430167647,10.0785159877801,0.));
#91812=CARTESIAN_POINT('Ctrl Pts',(45.8148430167647,10.0785159877801,20.));
#91813=CARTESIAN_POINT('Ctrl Pts',(45.8189965557614,10.0457082351741,0.));
#91814=CARTESIAN_POINT('Ctrl Pts',(45.8189965557614,10.0457082351741,20.));
#91815=CARTESIAN_POINT('Ctrl Pts',(45.8231269193611,10.0128986821194,0.));
#91816=CARTESIAN_POINT('Ctrl Pts',(45.8231269193611,10.0128986821194,20.));
#91817=CARTESIAN_POINT('Ctrl Pts',(45.8272341063969,9.98008734489948,0.));
#91818=CARTESIAN_POINT('Ctrl Pts',(45.8272341063969,9.98008734489948,20.));
#91819=CARTESIAN_POINT('Ctrl Pts',(45.8313181157134,9.94727423979906,0.));
#91820=CARTESIAN_POINT('Ctrl Pts',(45.8313181157134,9.94727423979906,20.));
#91821=CARTESIAN_POINT('Ctrl Pts',(45.8353789461673,9.91445938310424,0.));
#91822=CARTESIAN_POINT('Ctrl Pts',(45.8353789461673,9.91445938310424,20.));
#91823=CARTESIAN_POINT('Ctrl Pts',(45.8394165966264,9.88164279110241,0.));
#91824=CARTESIAN_POINT('Ctrl Pts',(45.8394165966264,9.88164279110241,20.));
#91825=CARTESIAN_POINT('Ctrl Pts',(45.84343106597,9.84882448008225,0.));
#91826=CARTESIAN_POINT('Ctrl Pts',(45.84343106597,9.84882448008225,20.));
#91827=CARTESIAN_POINT('Ctrl Pts',(45.8474223530896,9.81600446633368,0.));
#91828=CARTESIAN_POINT('Ctrl Pts',(45.8474223530896,9.81600446633368,20.));
#91829=CARTESIAN_POINT('Ctrl Pts',(45.8513904568872,9.78318276614762,0.));
#91830=CARTESIAN_POINT('Ctrl Pts',(45.8513904568872,9.78318276614762,20.));
#91831=CARTESIAN_POINT('Ctrl Pts',(45.8553353762765,9.75035939581619,0.));
#91832=CARTESIAN_POINT('Ctrl Pts',(45.8553353762765,9.75035939581619,20.));
#91833=CARTESIAN_POINT('Ctrl Pts',(45.8592571101812,9.71753437163221,0.));
#91834=CARTESIAN_POINT('Ctrl Pts',(45.8592571101812,9.71753437163221,20.));
#91835=CARTESIAN_POINT('Ctrl Pts',(45.8631556575366,9.68470770988976,0.));
#91836=CARTESIAN_POINT('Ctrl Pts',(45.8631556575366,9.68470770988976,20.));
#91837=CARTESIAN_POINT('Ctrl Pts',(45.8670310172895,9.65187942688401,0.));
#91838=CARTESIAN_POINT('Ctrl Pts',(45.8670310172895,9.65187942688401,20.));
#91839=CARTESIAN_POINT('Ctrl Pts',(45.870883188399,9.61904953891161,0.));
#91840=CARTESIAN_POINT('Ctrl Pts',(45.870883188399,9.61904953891161,20.));
#91841=CARTESIAN_POINT('Ctrl Pts',(45.8747121698355,9.58621806227057,0.));
#91842=CARTESIAN_POINT('Ctrl Pts',(45.8747121698355,9.58621806227057,20.));
#91843=CARTESIAN_POINT('Ctrl Pts',(45.8785179605829,9.55338501326048,0.));
#91844=CARTESIAN_POINT('Ctrl Pts',(45.8785179605829,9.55338501326048,20.));
#91845=CARTESIAN_POINT('Ctrl Pts',(45.882300559635,9.52055040818185,0.));
#91846=CARTESIAN_POINT('Ctrl Pts',(45.882300559635,9.52055040818185,20.));
#91847=CARTESIAN_POINT('Ctrl Pts',(45.8860599659967,9.4877142633361,0.));
#91848=CARTESIAN_POINT('Ctrl Pts',(45.8860599659967,9.4877142633361,20.));
#91849=CARTESIAN_POINT('Ctrl Pts',(45.8897961786838,9.45487659502548,0.));
#91850=CARTESIAN_POINT('Ctrl Pts',(45.8897961786838,9.45487659502548,20.));
#91851=CARTESIAN_POINT('Ctrl Pts',(45.8935091967241,9.42203741955325,0.));
#91852=CARTESIAN_POINT('Ctrl Pts',(45.8935091967241,9.42203741955325,20.));
#91853=CARTESIAN_POINT('Ctrl Pts',(45.8971990191563,9.38919675322381,0.));
#91854=CARTESIAN_POINT('Ctrl Pts',(45.8971990191563,9.38919675322381,20.));
#91855=CARTESIAN_POINT('Ctrl Pts',(45.90086564503,9.35635461234246,0.));
#91856=CARTESIAN_POINT('Ctrl Pts',(45.90086564503,9.35635461234246,20.));
#91857=CARTESIAN_POINT('Ctrl Pts',(45.9045090734063,9.3235110132158,0.));
#91858=CARTESIAN_POINT('Ctrl Pts',(45.9045090734063,9.3235110132158,20.));
#91859=CARTESIAN_POINT('Ctrl Pts',(45.9081293033576,9.29066597215163,0.));
#91860=CARTESIAN_POINT('Ctrl Pts',(45.9081293033576,9.29066597215163,20.));
#91861=CARTESIAN_POINT('Ctrl Pts',(45.9117263339694,9.25781950545902,0.));
#91862=CARTESIAN_POINT('Ctrl Pts',(45.9117263339694,9.25781950545902,20.));
#91863=CARTESIAN_POINT('Ctrl Pts',(45.9153001643391,9.22497162944821,0.));
#91864=CARTESIAN_POINT('Ctrl Pts',(45.9153001643391,9.22497162944821,20.));
#91865=CARTESIAN_POINT('Ctrl Pts',(45.9188507935764,9.19212236043074,0.));
#91866=CARTESIAN_POINT('Ctrl Pts',(45.9188507935764,9.19212236043074,20.));
#91867=CARTESIAN_POINT('Ctrl Pts',(45.9223782208015,9.15927171471892,0.));
#91868=CARTESIAN_POINT('Ctrl Pts',(45.9223782208015,9.15927171471892,20.));
#91869=CARTESIAN_POINT('Ctrl Pts',(45.9258824451441,9.12641970862567,0.));
#91870=CARTESIAN_POINT('Ctrl Pts',(45.9258824451441,9.12641970862567,20.));
#91871=CARTESIAN_POINT('Ctrl Pts',(45.9293634657451,9.09356635846486,0.));
#91872=CARTESIAN_POINT('Ctrl Pts',(45.9293634657451,9.09356635846486,20.));
#91873=CARTESIAN_POINT('Ctrl Pts',(45.9328212817567,9.06071168055121,0.));
#91874=CARTESIAN_POINT('Ctrl Pts',(45.9328212817567,9.06071168055121,20.));
#91875=CARTESIAN_POINT('Ctrl Pts',(45.9362558923428,9.02785569120062,0.));
#91876=CARTESIAN_POINT('Ctrl Pts',(45.9362558923428,9.02785569120062,20.));
#91877=CARTESIAN_POINT('Ctrl Pts',(45.939667296681,8.99499840673047,0.));
#91878=CARTESIAN_POINT('Ctrl Pts',(45.939667296681,8.99499840673047,20.));
#91879=CARTESIAN_POINT('Ctrl Pts',(45.9430554939595,8.96213984345905,0.));
#91880=CARTESIAN_POINT('Ctrl Pts',(45.9430554939595,8.96213984345905,20.));
#91881=CARTESIAN_POINT('Ctrl Pts',(45.9464204833787,8.92928001770576,0.));
#91882=CARTESIAN_POINT('Ctrl Pts',(45.9464204833787,8.92928001770576,20.));
#91883=CARTESIAN_POINT('Ctrl Pts',(45.9497622641496,8.89641894579083,0.));
#91884=CARTESIAN_POINT('Ctrl Pts',(45.9497622641496,8.89641894579083,20.));
#91885=CARTESIAN_POINT('Ctrl Pts',(45.9530808354938,8.86355664403535,0.));
#91886=CARTESIAN_POINT('Ctrl Pts',(45.9530808354938,8.86355664403535,20.));
#91887=CARTESIAN_POINT('Ctrl Pts',(45.9563761966444,8.83069312876128,0.));
#91888=CARTESIAN_POINT('Ctrl Pts',(45.9563761966444,8.83069312876128,20.));
#91889=CARTESIAN_POINT('Ctrl Pts',(45.9596483468462,8.79782841629148,0.));
#91890=CARTESIAN_POINT('Ctrl Pts',(45.9596483468462,8.79782841629148,20.));
#91891=CARTESIAN_POINT('Ctrl Pts',(45.9628972853566,8.76496252295002,0.));
#91892=CARTESIAN_POINT('Ctrl Pts',(45.9628972853566,8.76496252295002,20.));
#91893=CARTESIAN_POINT('Ctrl Pts',(45.9661230114446,8.732095465062,0.));
#91894=CARTESIAN_POINT('Ctrl Pts',(45.9661230114446,8.732095465062,20.));
#91895=CARTESIAN_POINT('Ctrl Pts',(45.9693255243897,8.69922725895329,0.));
#91896=CARTESIAN_POINT('Ctrl Pts',(45.9693255243897,8.69922725895329,20.));
#91897=CARTESIAN_POINT('Ctrl Pts',(45.9725048234817,8.66635792095044,0.));
#91898=CARTESIAN_POINT('Ctrl Pts',(45.9725048234817,8.66635792095044,20.));
#91899=CARTESIAN_POINT('Ctrl Pts',(45.9756609080225,8.633487467381,0.));
#91900=CARTESIAN_POINT('Ctrl Pts',(45.9756609080225,8.633487467381,20.));
#91901=CARTESIAN_POINT('Ctrl Pts',(45.9787937773254,8.6006159145734,0.));
#91902=CARTESIAN_POINT('Ctrl Pts',(45.9787937773254,8.6006159145734,20.));
#91903=CARTESIAN_POINT('Ctrl Pts',(45.9819034307166,8.56774327885726,0.));
#91904=CARTESIAN_POINT('Ctrl Pts',(45.9819034307166,8.56774327885726,20.));
#91905=CARTESIAN_POINT('Ctrl Pts',(45.9849898675351,8.53486957656348,0.));
#91906=CARTESIAN_POINT('Ctrl Pts',(45.9849898675351,8.53486957656348,20.));
#91907=CARTESIAN_POINT('Ctrl Pts',(45.9880530871298,8.50199482402355,0.));
#91908=CARTESIAN_POINT('Ctrl Pts',(45.9880530871298,8.50199482402355,20.));
#91909=CARTESIAN_POINT('Ctrl Pts',(45.991093088861,8.46911903756974,0.));
#91910=CARTESIAN_POINT('Ctrl Pts',(45.991093088861,8.46911903756974,20.));
#91911=CARTESIAN_POINT('Ctrl Pts',(45.9941098720982,8.43624223353472,0.));
#91912=CARTESIAN_POINT('Ctrl Pts',(45.9941098720982,8.43624223353472,20.));
#91913=CARTESIAN_POINT('Ctrl Pts',(45.9971034362229,8.403364428252,0.));
#91914=CARTESIAN_POINT('Ctrl Pts',(45.9971034362229,8.403364428252,20.));
#91915=CARTESIAN_POINT('Ctrl Pts',(46.000073780629,8.37048563805606,0.));
#91916=CARTESIAN_POINT('Ctrl Pts',(46.000073780629,8.37048563805606,20.));
#91917=CARTESIAN_POINT('Ctrl Pts',(46.0030209047226,8.33760587928254,0.));
#91918=CARTESIAN_POINT('Ctrl Pts',(46.0030209047226,8.33760587928254,20.));
#91919=CARTESIAN_POINT('Ctrl Pts',(46.0059448079215,8.30472516826798,0.));
#91920=CARTESIAN_POINT('Ctrl Pts',(46.0059448079215,8.30472516826798,20.));
#91921=CARTESIAN_POINT('Ctrl Pts',(46.0088454896554,8.27184352134995,0.));
#91922=CARTESIAN_POINT('Ctrl Pts',(46.0088454896554,8.27184352134995,20.));
#91923=CARTESIAN_POINT('Ctrl Pts',(46.0117229493647,8.2389609548667,0.));
#91924=CARTESIAN_POINT('Ctrl Pts',(46.0117229493647,8.2389609548667,20.));
#91925=CARTESIAN_POINT('Ctrl Pts',(46.0145771865005,8.20607748515696,0.));
#91926=CARTESIAN_POINT('Ctrl Pts',(46.0145771865005,8.20607748515696,20.));
#91927=CARTESIAN_POINT('Ctrl Pts',(46.0174082005262,8.17319312856043,0.));
#91928=CARTESIAN_POINT('Ctrl Pts',(46.0174082005262,8.17319312856043,20.));
#91929=CARTESIAN_POINT('Ctrl Pts',(46.0202159909161,8.1403079014174,0.));
#91930=CARTESIAN_POINT('Ctrl Pts',(46.0202159909161,8.1403079014174,20.));
#91931=CARTESIAN_POINT('Ctrl Pts',(46.0230005571558,8.10742182006901,0.));
#91932=CARTESIAN_POINT('Ctrl Pts',(46.0230005571558,8.10742182006901,20.));
#91933=CARTESIAN_POINT('Ctrl Pts',(46.025761898743,8.07453490085737,0.));
#91934=CARTESIAN_POINT('Ctrl Pts',(46.025761898743,8.07453490085737,20.));
#91935=CARTESIAN_POINT('Ctrl Pts',(46.0285000151874,8.04164716012546,0.));
#91936=CARTESIAN_POINT('Ctrl Pts',(46.0285000151874,8.04164716012546,20.));
#91937=CARTESIAN_POINT('Ctrl Pts',(46.0312149060105,8.00875861421695,0.));
#91938=CARTESIAN_POINT('Ctrl Pts',(46.0312149060105,8.00875861421695,20.));
#91939=CARTESIAN_POINT('Ctrl Pts',(46.0339065707442,7.97586927947621,0.));
#91940=CARTESIAN_POINT('Ctrl Pts',(46.0339065707442,7.97586927947621,20.));
#91941=CARTESIAN_POINT('Ctrl Pts',(46.0365750089318,7.94297917224816,0.));
#91942=CARTESIAN_POINT('Ctrl Pts',(46.0365750089318,7.94297917224816,20.));
#91943=CARTESIAN_POINT('Ctrl Pts',(46.0392202201278,7.91008830887856,0.));
#91944=CARTESIAN_POINT('Ctrl Pts',(46.0392202201278,7.91008830887856,20.));
#91945=CARTESIAN_POINT('Ctrl Pts',(46.0418422038989,7.87719670571401,0.));
#91946=CARTESIAN_POINT('Ctrl Pts',(46.0418422038989,7.87719670571401,20.));
#91947=CARTESIAN_POINT('Ctrl Pts',(46.0444409598224,7.84430437910167,0.));
#91948=CARTESIAN_POINT('Ctrl Pts',(46.0444409598224,7.84430437910167,20.));
#91949=CARTESIAN_POINT('Ctrl Pts',(46.0470164874882,7.81141134538955,0.));
#91950=CARTESIAN_POINT('Ctrl Pts',(46.0470164874882,7.81141134538955,20.));
#91951=CARTESIAN_POINT('Ctrl Pts',(46.0495687864972,7.77851762092637,0.));
#91952=CARTESIAN_POINT('Ctrl Pts',(46.0495687864972,7.77851762092637,20.));
#91953=CARTESIAN_POINT('Ctrl Pts',(46.052097856463,7.74562322206168,0.));
#91954=CARTESIAN_POINT('Ctrl Pts',(46.052097856463,7.74562322206168,20.));
#91955=CARTESIAN_POINT('Ctrl Pts',(46.0546036970108,7.71272816514572,0.));
#91956=CARTESIAN_POINT('Ctrl Pts',(46.0546036970108,7.71272816514572,20.));
#91957=CARTESIAN_POINT('Ctrl Pts',(46.0570863077758,7.67983246652918,0.));
#91958=CARTESIAN_POINT('Ctrl Pts',(46.0570863077758,7.67983246652918,20.));
#91959=CARTESIAN_POINT('Ctrl Pts',(46.0595456884042,7.64693614256336,0.));
#91960=CARTESIAN_POINT('Ctrl Pts',(46.0595456884042,7.64693614256336,20.));
#91961=CARTESIAN_POINT('Ctrl Pts',(46.0619818385541,7.61403920960036,0.));
#91962=CARTESIAN_POINT('Ctrl Pts',(46.0619818385541,7.61403920960036,20.));
#91963=CARTESIAN_POINT('Ctrl Pts',(46.0643947578955,7.58114168399302,0.));
#91964=CARTESIAN_POINT('Ctrl Pts',(46.0643947578955,7.58114168399302,20.));
#91965=CARTESIAN_POINT('Ctrl Pts',(46.0667844461104,7.54824358209485,0.));
#91966=CARTESIAN_POINT('Ctrl Pts',(46.0667844461104,7.54824358209485,20.));
#91967=CARTESIAN_POINT('Ctrl Pts',(46.0691509028928,7.51534492025983,0.));
#91968=CARTESIAN_POINT('Ctrl Pts',(46.0691509028928,7.51534492025983,20.));
#91969=CARTESIAN_POINT('Ctrl Pts',(46.0714941279471,7.48244571484251,0.));
#91970=CARTESIAN_POINT('Ctrl Pts',(46.0714941279471,7.48244571484251,20.));
#91971=CARTESIAN_POINT('Ctrl Pts',(46.0738141209885,7.4495459821981,0.));
#91972=CARTESIAN_POINT('Ctrl Pts',(46.0738141209885,7.4495459821981,20.));
#91973=CARTESIAN_POINT('Ctrl Pts',(46.0761108817447,7.41664573868261,0.));
#91974=CARTESIAN_POINT('Ctrl Pts',(46.0761108817447,7.41664573868261,20.));
#91975=CARTESIAN_POINT('Ctrl Pts',(46.0783844099553,7.38374500065295,0.));
#91976=CARTESIAN_POINT('Ctrl Pts',(46.0783844099553,7.38374500065295,20.));
#91977=CARTESIAN_POINT('Ctrl Pts',(46.0806347053718,7.35084378446662,0.));
#91978=CARTESIAN_POINT('Ctrl Pts',(46.0806347053718,7.35084378446662,20.));
#91979=CARTESIAN_POINT('Ctrl Pts',(46.0828617677561,7.3179421064814,0.));
#91980=CARTESIAN_POINT('Ctrl Pts',(46.0828617677561,7.3179421064814,20.));
#91981=CARTESIAN_POINT('Ctrl Pts',(46.0850655968817,7.28503998305551,0.));
#91982=CARTESIAN_POINT('Ctrl Pts',(46.0850655968817,7.28503998305551,20.));
#91983=CARTESIAN_POINT('Ctrl Pts',(46.0872461925336,7.2521374305475,0.));
#91984=CARTESIAN_POINT('Ctrl Pts',(46.0872461925336,7.2521374305475,20.));
#91985=CARTESIAN_POINT('Ctrl Pts',(46.0894035545083,7.21923446531641,0.));
#91986=CARTESIAN_POINT('Ctrl Pts',(46.0894035545083,7.21923446531641,20.));
#91987=CARTESIAN_POINT('Ctrl Pts',(46.0915376826137,7.18633110372212,0.));
#91988=CARTESIAN_POINT('Ctrl Pts',(46.0915376826137,7.18633110372212,20.));
#91989=CARTESIAN_POINT('Ctrl Pts',(46.0936485766695,7.1534273621253,0.));
#91990=CARTESIAN_POINT('Ctrl Pts',(46.0936485766695,7.1534273621253,20.));
#91991=CARTESIAN_POINT('Ctrl Pts',(46.0957362365075,7.12052325688753,0.));
#91992=CARTESIAN_POINT('Ctrl Pts',(46.0957362365075,7.12052325688753,20.));
#91993=CARTESIAN_POINT('Ctrl Pts',(46.097800661971,7.08761880437094,0.));
#91994=CARTESIAN_POINT('Ctrl Pts',(46.097800661971,7.08761880437094,20.));
#91995=CARTESIAN_POINT('Ctrl Pts',(46.0998418529147,7.05471402093802,0.));
#91996=CARTESIAN_POINT('Ctrl Pts',(46.0998418529147,7.05471402093802,20.));
#91997=CARTESIAN_POINT('Ctrl Pts',(46.1018598092046,7.02180892295148,0.));
#91998=CARTESIAN_POINT('Ctrl Pts',(46.1018598092046,7.02180892295148,20.));
#91999=CARTESIAN_POINT('Ctrl Pts',(46.103854530718,6.98890352677439,0.));
#92000=CARTESIAN_POINT('Ctrl Pts',(46.103854530718,6.98890352677439,20.));
#92001=CARTESIAN_POINT('Ctrl Pts',(46.1058260173429,6.95599784877019,0.));
#92002=CARTESIAN_POINT('Ctrl Pts',(46.1058260173429,6.95599784877019,20.));
#92003=CARTESIAN_POINT('Ctrl Pts',(46.1077742689797,6.92309190530285,0.));
#92004=CARTESIAN_POINT('Ctrl Pts',(46.1077742689797,6.92309190530285,20.));
#92005=CARTESIAN_POINT('Ctrl Pts',(46.1096992855399,6.8901857127369,0.));
#92006=CARTESIAN_POINT('Ctrl Pts',(46.1096992855399,6.8901857127369,20.));
#92007=CARTESIAN_POINT('Ctrl Pts',(46.111601066948,6.85727928743788,0.));
#92008=CARTESIAN_POINT('Ctrl Pts',(46.111601066948,6.85727928743788,20.));
#92009=CARTESIAN_POINT('Ctrl Pts',(46.1134796131392,6.82437264577169,0.));
#92010=CARTESIAN_POINT('Ctrl Pts',(46.1134796131392,6.82437264577169,20.));
#92011=CARTESIAN_POINT('Ctrl Pts',(46.1153349240611,6.7914658041047,0.));
#92012=CARTESIAN_POINT('Ctrl Pts',(46.1153349240611,6.7914658041047,20.));
#92013=CARTESIAN_POINT('Ctrl Pts',(46.1171669996709,6.75855877880357,0.));
#92014=CARTESIAN_POINT('Ctrl Pts',(46.1171669996709,6.75855877880357,20.));
#92015=CARTESIAN_POINT('Ctrl Pts',(46.1189758399374,6.72565158623521,0.));
#92016=CARTESIAN_POINT('Ctrl Pts',(46.1189758399374,6.72565158623521,20.));
#92017=CARTESIAN_POINT('Ctrl Pts',(46.1207614448407,6.69274424276688,0.));
#92018=CARTESIAN_POINT('Ctrl Pts',(46.1207614448407,6.69274424276688,20.));
#92019=CARTESIAN_POINT('Ctrl Pts',(46.122523814374,6.65983676476652,0.));
#92020=CARTESIAN_POINT('Ctrl Pts',(46.122523814374,6.65983676476652,20.));
#92021=CARTESIAN_POINT('Ctrl Pts',(46.124262948542,6.62692916860258,0.));
#92022=CARTESIAN_POINT('Ctrl Pts',(46.124262948542,6.62692916860258,20.));
#92023=CARTESIAN_POINT('Ctrl Pts',(46.1259788473615,6.594021470644,0.));
#92024=CARTESIAN_POINT('Ctrl Pts',(46.1259788473615,6.594021470644,20.));
#92025=CARTESIAN_POINT('Ctrl Pts',(46.1276715108604,6.5611136872601,0.));
#92026=CARTESIAN_POINT('Ctrl Pts',(46.1276715108604,6.5611136872601,20.));
#92027=CARTESIAN_POINT('Ctrl Pts',(46.1293409390781,6.5282058348205,0.));
#92028=CARTESIAN_POINT('Ctrl Pts',(46.1293409390781,6.5282058348205,20.));
#92029=CARTESIAN_POINT('Ctrl Pts',(46.1309871320644,6.49529792969509,0.));
#92030=CARTESIAN_POINT('Ctrl Pts',(46.1309871320644,6.49529792969509,20.));
#92031=CARTESIAN_POINT('Ctrl Pts',(46.1326100898806,6.46238998825408,0.));
#92032=CARTESIAN_POINT('Ctrl Pts',(46.1326100898806,6.46238998825408,20.));
#92033=CARTESIAN_POINT('Ctrl Pts',(46.134209812599,6.42948202686814,0.));
#92034=CARTESIAN_POINT('Ctrl Pts',(46.134209812599,6.42948202686814,20.));
#92035=CARTESIAN_POINT('Ctrl Pts',(46.1357863003044,6.39657406190845,0.));
#92036=CARTESIAN_POINT('Ctrl Pts',(46.1357863003044,6.39657406190845,20.));
#92037=CARTESIAN_POINT('Ctrl Pts',(46.1373395530931,6.36366610974648,0.));
#92038=CARTESIAN_POINT('Ctrl Pts',(46.1373395530931,6.36366610974648,20.));
#92039=CARTESIAN_POINT('Ctrl Pts',(46.138869571074,6.3307581867542,0.));
#92040=CARTESIAN_POINT('Ctrl Pts',(46.138869571074,6.3307581867542,20.));
#92041=CARTESIAN_POINT('Ctrl Pts',(46.1403763543673,6.29785030930382,0.));
#92042=CARTESIAN_POINT('Ctrl Pts',(46.1403763543673,6.29785030930382,20.));
#92043=CARTESIAN_POINT('Ctrl Pts',(46.141859903105,6.26494249376778,0.));
#92044=CARTESIAN_POINT('Ctrl Pts',(46.141859903105,6.26494249376778,20.));
#92045=CARTESIAN_POINT('Ctrl Pts',(46.1433202174297,6.23203475651883,0.));
#92046=CARTESIAN_POINT('Ctrl Pts',(46.1433202174297,6.23203475651883,20.));
#92047=CARTESIAN_POINT('Ctrl Pts',(46.1447572974959,6.19912711393004,0.));
#92048=CARTESIAN_POINT('Ctrl Pts',(46.1447572974959,6.19912711393004,20.));
#92049=CARTESIAN_POINT('Ctrl Pts',(46.1461711434687,6.16621958237488,0.));
#92050=CARTESIAN_POINT('Ctrl Pts',(46.1461711434687,6.16621958237488,20.));
#92051=CARTESIAN_POINT('Ctrl Pts',(46.1475617555249,6.1333121782271,0.));
#92052=CARTESIAN_POINT('Ctrl Pts',(46.1475617555249,6.1333121782271,20.));
#92053=CARTESIAN_POINT('Ctrl Pts',(46.1489291338532,6.10040491786086,0.));
#92054=CARTESIAN_POINT('Ctrl Pts',(46.1489291338532,6.10040491786086,20.));
#92055=CARTESIAN_POINT('Ctrl Pts',(46.1502732786543,6.06749781765058,0.));
#92056=CARTESIAN_POINT('Ctrl Pts',(46.1502732786543,6.06749781765058,20.));
#92057=CARTESIAN_POINT('Ctrl Pts',(46.151594190141,6.03459089397104,0.));
#92058=CARTESIAN_POINT('Ctrl Pts',(46.151594190141,6.03459089397104,20.));
#92059=CARTESIAN_POINT('Ctrl Pts',(46.1528918685373,6.0016841631972,0.));
#92060=CARTESIAN_POINT('Ctrl Pts',(46.1528918685373,6.0016841631972,20.));
#92061=CARTESIAN_POINT('Ctrl Pts',(46.1541663140783,5.96877764170412,0.));
#92062=CARTESIAN_POINT('Ctrl Pts',(46.1541663140783,5.96877764170412,20.));
#92063=CARTESIAN_POINT('Ctrl Pts',(46.1554175270101,5.9358713458669,0.));
#92064=CARTESIAN_POINT('Ctrl Pts',(46.1554175270101,5.9358713458669,20.));
#92065=CARTESIAN_POINT('Ctrl Pts',(46.1566455075904,5.90296529206097,0.));
#92066=CARTESIAN_POINT('Ctrl Pts',(46.1566455075904,5.90296529206097,20.));
#92067=CARTESIAN_POINT('Ctrl Pts',(46.1578502560886,5.87005949666212,0.));
#92068=CARTESIAN_POINT('Ctrl Pts',(46.1578502560886,5.87005949666212,20.));
#92069=CARTESIAN_POINT('Ctrl Pts',(46.1590317727861,5.83715397604653,0.));
#92070=CARTESIAN_POINT('Ctrl Pts',(46.1590317727861,5.83715397604653,20.));
#92071=CARTESIAN_POINT('Ctrl Pts',(46.160190057976,5.80424874659071,0.));
#92072=CARTESIAN_POINT('Ctrl Pts',(46.160190057976,5.80424874659071,20.));
#92073=CARTESIAN_POINT('Ctrl Pts',(46.1613251119636,5.77134382467173,0.));
#92074=CARTESIAN_POINT('Ctrl Pts',(46.1613251119636,5.77134382467173,20.));
#92075=CARTESIAN_POINT('Ctrl Pts',(46.1624369350662,5.73843922666648,0.));
#92076=CARTESIAN_POINT('Ctrl Pts',(46.1624369350662,5.73843922666648,20.));
#92077=CARTESIAN_POINT('Ctrl Pts',(46.1635255276116,5.70553496895185,0.));
#92078=CARTESIAN_POINT('Ctrl Pts',(46.1635255276116,5.70553496895185,20.));
#92079=CARTESIAN_POINT('Ctrl Pts',(46.1645908899393,5.67263106790479,0.));
#92080=CARTESIAN_POINT('Ctrl Pts',(46.1645908899393,5.67263106790479,20.));
#92081=CARTESIAN_POINT('Ctrl Pts',(46.1656330223979,5.63972753990236,0.));
#92082=CARTESIAN_POINT('Ctrl Pts',(46.1656330223979,5.63972753990236,20.));
#92083=CARTESIAN_POINT('Ctrl Pts',(46.166651925349,5.60682440132182,0.));
#92084=CARTESIAN_POINT('Ctrl Pts',(46.166651925349,5.60682440132182,20.));
#92085=CARTESIAN_POINT('Ctrl Pts',(46.1676475991657,5.57392166854075,0.));
#92086=CARTESIAN_POINT('Ctrl Pts',(46.1676475991657,5.57392166854075,20.));
#92087=CARTESIAN_POINT('Ctrl Pts',(46.1686200442337,5.5410193579371,0.));
#92088=CARTESIAN_POINT('Ctrl Pts',(46.1686200442337,5.5410193579371,20.));
#92089=CARTESIAN_POINT('Ctrl Pts',(46.1695692609505,5.50811748588894,0.));
#92090=CARTESIAN_POINT('Ctrl Pts',(46.1695692609505,5.50811748588894,20.));
#92091=CARTESIAN_POINT('Ctrl Pts',(46.170495249726,5.4752160687746,0.));
#92092=CARTESIAN_POINT('Ctrl Pts',(46.170495249726,5.4752160687746,20.));
#92093=CARTESIAN_POINT('Ctrl Pts',(46.1713980109807,5.44231512297239,0.));
#92094=CARTESIAN_POINT('Ctrl Pts',(46.1713980109807,5.44231512297239,20.));
#92095=CARTESIAN_POINT('Ctrl Pts',(46.1722775451467,5.40941466486069,0.));
#92096=CARTESIAN_POINT('Ctrl Pts',(46.1722775451467,5.40941466486069,20.));
#92097=CARTESIAN_POINT('Ctrl Pts',(46.1731338526667,5.37651471081787,0.));
#92098=CARTESIAN_POINT('Ctrl Pts',(46.1731338526667,5.37651471081787,20.));
#92099=CARTESIAN_POINT('Ctrl Pts',(46.1739669339953,5.3436152772224,0.));
#92100=CARTESIAN_POINT('Ctrl Pts',(46.1739669339953,5.3436152772224,20.));
#92101=CARTESIAN_POINT('Ctrl Pts',(46.1747767895978,5.31071638045279,0.));
#92102=CARTESIAN_POINT('Ctrl Pts',(46.1747767895978,5.31071638045279,20.));
#92103=CARTESIAN_POINT('Ctrl Pts',(46.1755634199519,5.27781803688791,0.));
#92104=CARTESIAN_POINT('Ctrl Pts',(46.1755634199519,5.27781803688791,20.));
#92105=CARTESIAN_POINT('Ctrl Pts',(46.1763268255471,5.24492026290663,0.));
#92106=CARTESIAN_POINT('Ctrl Pts',(46.1763268255471,5.24492026290663,20.));
#92107=CARTESIAN_POINT('Ctrl Pts',(46.1770670068854,5.21202307488802,0.));
#92108=CARTESIAN_POINT('Ctrl Pts',(46.1770670068854,5.21202307488802,20.));
#92109=CARTESIAN_POINT('Ctrl Pts',(46.1777839644797,5.17912648921102,0.));
#92110=CARTESIAN_POINT('Ctrl Pts',(46.1777839644797,5.17912648921102,20.));
#92111=CARTESIAN_POINT('Ctrl Pts',(46.1784776988548,5.14623052225472,0.));
#92112=CARTESIAN_POINT('Ctrl Pts',(46.1784776988548,5.14623052225472,20.));
#92113=CARTESIAN_POINT('Ctrl Pts',(46.1791482105459,5.11333519039809,0.));
#92114=CARTESIAN_POINT('Ctrl Pts',(46.1791482105459,5.11333519039809,20.));
#92115=CARTESIAN_POINT('Ctrl Pts',(46.1797955000997,5.08044051002026,0.));
#92116=CARTESIAN_POINT('Ctrl Pts',(46.1797955000997,5.08044051002026,20.));
#92117=CARTESIAN_POINT('Ctrl Pts',(46.1804195680748,5.04754649750031,0.));
#92118=CARTESIAN_POINT('Ctrl Pts',(46.1804195680748,5.04754649750031,20.));
#92119=CARTESIAN_POINT('Ctrl Pts',(46.1810204150412,5.01465316921749,0.));
#92120=CARTESIAN_POINT('Ctrl Pts',(46.1810204150412,5.01465316921749,20.));
#92121=CARTESIAN_POINT('Ctrl Pts',(46.1815980415817,4.98176054155101,0.));
#92122=CARTESIAN_POINT('Ctrl Pts',(46.1815980415817,4.98176054155101,20.));
#92123=CARTESIAN_POINT('Ctrl Pts',(46.182152448291,4.94886863088032,0.));
#92124=CARTESIAN_POINT('Ctrl Pts',(46.182152448291,4.94886863088032,20.));
#92125=CARTESIAN_POINT('Ctrl Pts',(46.1826836357763,4.91597745358481,0.));
#92126=CARTESIAN_POINT('Ctrl Pts',(46.1826836357763,4.91597745358481,20.));
#92127=CARTESIAN_POINT('Ctrl Pts',(46.1831916046531,4.8830870260435,0.));
#92128=CARTESIAN_POINT('Ctrl Pts',(46.1831916046531,4.8830870260435,20.));
#92129=CARTESIAN_POINT('Ctrl Pts',(46.1836763555496,4.85019736463544,0.));
#92130=CARTESIAN_POINT('Ctrl Pts',(46.1836763555496,4.85019736463544,20.));
#92131=CARTESIAN_POINT('Ctrl Pts',(46.1841378891039,4.81730848573954,0.));
#92132=CARTESIAN_POINT('Ctrl Pts',(46.1841378891039,4.81730848573954,20.));
#92133=CARTESIAN_POINT('Ctrl Pts',(46.1845762059678,4.78442040573515,0.));
#92134=CARTESIAN_POINT('Ctrl Pts',(46.1845762059678,4.78442040573515,20.));
#92135=CARTESIAN_POINT('Ctrl Pts',(46.1849913068043,4.75153314100161,0.));
#92136=CARTESIAN_POINT('Ctrl Pts',(46.1849913068043,4.75153314100161,20.));
#92137=CARTESIAN_POINT('Ctrl Pts',(46.1853831922891,4.71864670791826,0.));
#92138=CARTESIAN_POINT('Ctrl Pts',(46.1853831922891,4.71864670791826,20.));
#92139=CARTESIAN_POINT('Ctrl Pts',(46.1857518631086,4.68576112286394,0.));
#92140=CARTESIAN_POINT('Ctrl Pts',(46.1857518631086,4.68576112286394,20.));
#92141=CARTESIAN_POINT('Ctrl Pts',(46.1860973199616,4.65287640221748,0.));
#92142=CARTESIAN_POINT('Ctrl Pts',(46.1860973199616,4.65287640221748,20.));
#92143=CARTESIAN_POINT('Ctrl Pts',(46.1864195635571,4.61999256235741,0.));
#92144=CARTESIAN_POINT('Ctrl Pts',(46.1864195635571,4.61999256235741,20.));
#92145=CARTESIAN_POINT('Ctrl Pts',(46.1867185946155,4.58710961966233,0.));
#92146=CARTESIAN_POINT('Ctrl Pts',(46.1867185946155,4.58710961966233,20.));
#92147=CARTESIAN_POINT('Ctrl Pts',(46.1869944138693,4.55422759051101,0.));
#92148=CARTESIAN_POINT('Ctrl Pts',(46.1869944138693,4.55422759051101,20.));
#92149=CARTESIAN_POINT('Ctrl Pts',(46.1872470220627,4.52134649128218,0.));
#92150=CARTESIAN_POINT('Ctrl Pts',(46.1872470220627,4.52134649128218,20.));
#92151=CARTESIAN_POINT('Ctrl Pts',(46.1874764199521,4.48846633835459,0.));
#92152=CARTESIAN_POINT('Ctrl Pts',(46.1874764199521,4.48846633835459,20.));
#92153=CARTESIAN_POINT('Ctrl Pts',(46.1876826083051,4.45558714810681,0.));
#92154=CARTESIAN_POINT('Ctrl Pts',(46.1876826083051,4.45558714810681,20.));
#92155=CARTESIAN_POINT('Ctrl Pts',(46.1878655879008,4.42270893691724,0.));
#92156=CARTESIAN_POINT('Ctrl Pts',(46.1878655879008,4.42270893691724,20.));
#92157=CARTESIAN_POINT('Ctrl Pts',(46.1880253595296,4.38983172116389,0.));
#92158=CARTESIAN_POINT('Ctrl Pts',(46.1880253595296,4.38983172116389,20.));
#92159=CARTESIAN_POINT('Ctrl Pts',(46.1881619239926,4.35695551722447,0.));
#92160=CARTESIAN_POINT('Ctrl Pts',(46.1881619239926,4.35695551722447,20.));
#92161=CARTESIAN_POINT('Ctrl Pts',(46.1882752821036,4.32408034147655,0.));
#92162=CARTESIAN_POINT('Ctrl Pts',(46.1882752821036,4.32408034147655,20.));
#92163=CARTESIAN_POINT('Ctrl Pts',(46.1883654346888,4.29120621029777,0.));
#92164=CARTESIAN_POINT('Ctrl Pts',(46.1883654346888,4.29120621029777,20.));
#92165=CARTESIAN_POINT('Ctrl Pts',(46.1884323825857,4.25833314006578,0.));
#92166=CARTESIAN_POINT('Ctrl Pts',(46.1884323825857,4.25833314006578,20.));
#92167=CARTESIAN_POINT('Ctrl Pts',(46.1884761266433,4.22546114715825,0.));
#92168=CARTESIAN_POINT('Ctrl Pts',(46.1884761266433,4.22546114715825,20.));
#92169=CARTESIAN_POINT('Ctrl Pts',(46.1884966677209,4.19259024795239,0.));
#92170=CARTESIAN_POINT('Ctrl Pts',(46.1884966677209,4.19259024795239,20.));
#92171=CARTESIAN_POINT('Ctrl Pts',(46.1884940066895,4.15972045882509,0.));
#92172=CARTESIAN_POINT('Ctrl Pts',(46.1884940066895,4.15972045882509,20.));
#92173=CARTESIAN_POINT('Ctrl Pts',(46.1884681444317,4.12685179615294,0.));
#92174=CARTESIAN_POINT('Ctrl Pts',(46.1884681444317,4.12685179615294,20.));
#92175=CARTESIAN_POINT('Ctrl Pts',(46.188419081843,4.09398427631255,0.));
#92176=CARTESIAN_POINT('Ctrl Pts',(46.188419081843,4.09398427631255,20.));
#92177=CARTESIAN_POINT('Ctrl Pts',(46.18834681983,4.06111791568023,0.));
#92178=CARTESIAN_POINT('Ctrl Pts',(46.18834681983,4.06111791568023,20.));
#92179=CARTESIAN_POINT('Ctrl Pts',(46.1882513593113,4.02825273063218,0.));
#92180=CARTESIAN_POINT('Ctrl Pts',(46.1882513593113,4.02825273063218,20.));
#92181=CARTESIAN_POINT('Ctrl Pts',(46.1881327012171,3.99538873754443,0.));
#92182=CARTESIAN_POINT('Ctrl Pts',(46.1881327012171,3.99538873754443,20.));
#92183=CARTESIAN_POINT('Ctrl Pts',(46.1879908464881,3.96252595279274,0.));
#92184=CARTESIAN_POINT('Ctrl Pts',(46.1879908464881,3.96252595279274,20.));
#92185=CARTESIAN_POINT('Ctrl Pts',(46.1878257960766,3.92966439275257,0.));
#92186=CARTESIAN_POINT('Ctrl Pts',(46.1878257960766,3.92966439275257,20.));
#92187=CARTESIAN_POINT('Ctrl Pts',(46.1876375509469,3.89680407379914,0.));
#92188=CARTESIAN_POINT('Ctrl Pts',(46.1876375509469,3.89680407379914,20.));
#92189=CARTESIAN_POINT('Ctrl Pts',(46.1874261120751,3.86394501230744,0.));
#92190=CARTESIAN_POINT('Ctrl Pts',(46.1874261120751,3.86394501230744,20.));
#92191=CARTESIAN_POINT('Ctrl Pts',(46.1871914804492,3.83108722465199,0.));
#92192=CARTESIAN_POINT('Ctrl Pts',(46.1871914804492,3.83108722465199,20.));
#92193=CARTESIAN_POINT('Ctrl Pts',(46.1869336570686,3.79823072720685,0.));
#92194=CARTESIAN_POINT('Ctrl Pts',(46.1869336570686,3.79823072720685,20.));
#92195=CARTESIAN_POINT('Ctrl Pts',(46.1866526429445,3.76537553634596,0.));
#92196=CARTESIAN_POINT('Ctrl Pts',(46.1866526429445,3.76537553634596,20.));
#92197=CARTESIAN_POINT('Ctrl Pts',(46.1863484390996,3.73252166844328,0.));
#92198=CARTESIAN_POINT('Ctrl Pts',(46.1863484390996,3.73252166844328,20.));
#92199=CARTESIAN_POINT('Ctrl Pts',(46.1860210465678,3.69966913987253,0.));
#92200=CARTESIAN_POINT('Ctrl Pts',(46.1860210465678,3.69966913987253,20.));
#92201=CARTESIAN_POINT('Ctrl Pts',(46.185670466394,3.6668179670071,0.));
#92202=CARTESIAN_POINT('Ctrl Pts',(46.185670466394,3.6668179670071,20.));
#92203=CARTESIAN_POINT('Ctrl Pts',(46.1852966996347,3.6339681662199,0.));
#92204=CARTESIAN_POINT('Ctrl Pts',(46.1852966996347,3.6339681662199,20.));
#92205=CARTESIAN_POINT('Ctrl Pts',(46.1848997473582,3.60111975388339,0.));
#92206=CARTESIAN_POINT('Ctrl Pts',(46.1848997473582,3.60111975388339,20.));
#92207=CARTESIAN_POINT('Ctrl Pts',(46.1844796106451,3.56827274636958,0.));
#92208=CARTESIAN_POINT('Ctrl Pts',(46.1844796106451,3.56827274636958,20.));
#92209=CARTESIAN_POINT('Ctrl Pts',(46.1840362905882,3.53542716005025,0.));
#92210=CARTESIAN_POINT('Ctrl Pts',(46.1840362905882,3.53542716005025,20.));
#92211=CARTESIAN_POINT('Ctrl Pts',(46.1835697882921,3.50258301129689,0.));
#92212=CARTESIAN_POINT('Ctrl Pts',(46.1835697882921,3.50258301129689,20.));
#92213=CARTESIAN_POINT('Ctrl Pts',(46.1830801048722,3.4697403164807,0.));
#92214=CARTESIAN_POINT('Ctrl Pts',(46.1830801048722,3.4697403164807,20.));
#92215=CARTESIAN_POINT('Ctrl Pts',(46.1825672414553,3.43689909197262,0.));
#92216=CARTESIAN_POINT('Ctrl Pts',(46.1825672414553,3.43689909197262,20.));
#92217=CARTESIAN_POINT('Ctrl Pts',(46.1820311991793,3.40405935414302,0.));
#92218=CARTESIAN_POINT('Ctrl Pts',(46.1820311991793,3.40405935414302,20.));
#92219=CARTESIAN_POINT('Ctrl Pts',(46.1814719791936,3.37122111936182,0.));
#92220=CARTESIAN_POINT('Ctrl Pts',(46.1814719791936,3.37122111936182,20.));
#92221=CARTESIAN_POINT('Ctrl Pts',(46.1808895826591,3.33838440399861,0.));
#92222=CARTESIAN_POINT('Ctrl Pts',(46.1808895826591,3.33838440399861,20.));
#92223=CARTESIAN_POINT('Ctrl Pts',(46.1802840107495,3.30554922442266,0.));
#92224=CARTESIAN_POINT('Ctrl Pts',(46.1802840107495,3.30554922442266,20.));
#92225=CARTESIAN_POINT('Ctrl Pts',(46.1796552646498,3.27271559700279,0.));
#92226=CARTESIAN_POINT('Ctrl Pts',(46.1796552646498,3.27271559700279,20.));
#92227=CARTESIAN_POINT('Ctrl Pts',(46.1790033455572,3.23988353810748,0.));
#92228=CARTESIAN_POINT('Ctrl Pts',(46.1790033455572,3.23988353810748,20.));
#92229=CARTESIAN_POINT('Ctrl Pts',(46.1783282546796,3.20705306410471,0.));
#92230=CARTESIAN_POINT('Ctrl Pts',(46.1783282546796,3.20705306410471,20.));
#92231=CARTESIAN_POINT('Ctrl Pts',(46.1776299932363,3.17422419136187,0.));
#92232=CARTESIAN_POINT('Ctrl Pts',(46.1776299932363,3.17422419136187,20.));
#92233=CARTESIAN_POINT('Ctrl Pts',(46.1769085624582,3.14139693624605,0.));
#92234=CARTESIAN_POINT('Ctrl Pts',(46.1769085624582,3.14139693624605,20.));
#92235=CARTESIAN_POINT('Ctrl Pts',(46.1761639635878,3.10857131512384,0.));
#92236=CARTESIAN_POINT('Ctrl Pts',(46.1761639635878,3.10857131512384,20.));
#92237=CARTESIAN_POINT('Ctrl Pts',(46.1753961978798,3.0757473443616,0.));
#92238=CARTESIAN_POINT('Ctrl Pts',(46.1753961978798,3.0757473443616,20.));
#92239=CARTESIAN_POINT('Ctrl Pts',(46.1746052665999,3.04292504032497,0.));
#92240=CARTESIAN_POINT('Ctrl Pts',(46.1746052665999,3.04292504032497,20.));
#92241=CARTESIAN_POINT('Ctrl Pts',(46.1737911710261,3.01010441937913,0.));
#92242=CARTESIAN_POINT('Ctrl Pts',(46.1737911710261,3.01010441937913,20.));
#92243=CARTESIAN_POINT('Ctrl Pts',(46.1729539124487,2.9772854978889,0.));
#92244=CARTESIAN_POINT('Ctrl Pts',(46.1729539124487,2.9772854978889,20.));
#92245=CARTESIAN_POINT('Ctrl Pts',(46.172093492169,2.94446829221865,0.));
#92246=CARTESIAN_POINT('Ctrl Pts',(46.172093492169,2.94446829221865,20.));
#92247=CARTESIAN_POINT('Ctrl Pts',(46.1712099114993,2.91165281873225,0.));
#92248=CARTESIAN_POINT('Ctrl Pts',(46.1712099114993,2.91165281873225,20.));
#92249=CARTESIAN_POINT('Ctrl Pts',(46.1703031717627,2.87883909379287,0.));
#92250=CARTESIAN_POINT('Ctrl Pts',(46.1703031717627,2.87883909379287,20.));
#92251=CARTESIAN_POINT('Ctrl Pts',(46.169373274294,2.84602713376309,0.));
#92252=CARTESIAN_POINT('Ctrl Pts',(46.169373274294,2.84602713376309,20.));
#92253=CARTESIAN_POINT('Ctrl Pts',(46.1684202204402,2.81321695500492,0.));
#92254=CARTESIAN_POINT('Ctrl Pts',(46.1684202204402,2.81321695500492,20.));
#92255=CARTESIAN_POINT('Ctrl Pts',(46.1674440115603,2.78040857388008,0.));
#92256=CARTESIAN_POINT('Ctrl Pts',(46.1674440115603,2.78040857388008,20.));
#92257=CARTESIAN_POINT('Ctrl Pts',(46.1664446490252,2.7476020067498,0.));
#92258=CARTESIAN_POINT('Ctrl Pts',(46.1664446490252,2.7476020067498,20.));
#92259=CARTESIAN_POINT('Ctrl Pts',(46.1654221342175,2.71479726997479,0.));
#92260=CARTESIAN_POINT('Ctrl Pts',(46.1654221342175,2.71479726997479,20.));
#92261=CARTESIAN_POINT('Ctrl Pts',(46.1643764685316,2.68199437991524,0.));
#92262=CARTESIAN_POINT('Ctrl Pts',(46.1643764685316,2.68199437991524,20.));
#92263=CARTESIAN_POINT('Ctrl Pts',(46.163307653373,2.64919335293067,0.));
#92264=CARTESIAN_POINT('Ctrl Pts',(46.163307653373,2.64919335293067,20.));
#92265=CARTESIAN_POINT('Ctrl Pts',(46.1622156901587,2.61639420537995,0.));
#92266=CARTESIAN_POINT('Ctrl Pts',(46.1622156901587,2.61639420537995,20.));
#92267=CARTESIAN_POINT('Ctrl Pts',(46.1611005803162,2.58359695362108,0.));
#92268=CARTESIAN_POINT('Ctrl Pts',(46.1611005803162,2.58359695362108,20.));
#92269=CARTESIAN_POINT('Ctrl Pts',(46.1599623252856,2.55080161401166,0.));
#92270=CARTESIAN_POINT('Ctrl Pts',(46.1599623252856,2.55080161401166,20.));
#92271=CARTESIAN_POINT('Ctrl Pts',(46.1588009265184,2.51800820290892,0.));
#92272=CARTESIAN_POINT('Ctrl Pts',(46.1588009265184,2.51800820290892,20.));
#92273=CARTESIAN_POINT('Ctrl Pts',(46.1576163854777,2.48521673666957,0.));
#92274=CARTESIAN_POINT('Ctrl Pts',(46.1576163854777,2.48521673666957,20.));
#92275=CARTESIAN_POINT('Ctrl Pts',(46.1564087036389,2.4524272316497,0.));
#92276=CARTESIAN_POINT('Ctrl Pts',(46.1564087036389,2.4524272316497,20.));
#92277=CARTESIAN_POINT('Ctrl Pts',(46.155177882489,2.41963970420458,0.));
#92278=CARTESIAN_POINT('Ctrl Pts',(46.155177882489,2.41963970420458,20.));
#92279=CARTESIAN_POINT('Ctrl Pts',(46.1539239235264,2.38685417068871,0.));
#92280=CARTESIAN_POINT('Ctrl Pts',(46.1539239235264,2.38685417068871,20.));
#92281=CARTESIAN_POINT('Ctrl Pts',(46.1526468282603,2.35407064745589,0.));
#92282=CARTESIAN_POINT('Ctrl Pts',(46.1526468282603,2.35407064745589,20.));
#92283=CARTESIAN_POINT('Ctrl Pts',(46.1513465982124,2.3212891508592,0.));
#92284=CARTESIAN_POINT('Ctrl Pts',(46.1513465982124,2.3212891508592,20.));
#92285=CARTESIAN_POINT('Ctrl Pts',(46.1500232349155,2.28850969725138,0.));
#92286=CARTESIAN_POINT('Ctrl Pts',(46.1500232349155,2.28850969725138,20.));
#92287=CARTESIAN_POINT('Ctrl Pts',(46.1486767399146,2.25573230298459,0.));
#92288=CARTESIAN_POINT('Ctrl Pts',(46.1486767399146,2.25573230298459,20.));
#92289=CARTESIAN_POINT('Ctrl Pts',(46.147307114766,2.2229569844105,0.));
#92290=CARTESIAN_POINT('Ctrl Pts',(46.147307114766,2.2229569844105,20.));
#92291=CARTESIAN_POINT('Ctrl Pts',(46.1459143610377,2.19018375787987,0.));
#92292=CARTESIAN_POINT('Ctrl Pts',(46.1459143610377,2.19018375787987,20.));
#92293=CARTESIAN_POINT('Ctrl Pts',(46.1444984803082,2.15741263974263,0.));
#92294=CARTESIAN_POINT('Ctrl Pts',(46.1444984803082,2.15741263974263,20.));
#92295=CARTESIAN_POINT('Ctrl Pts',(46.1430594741682,2.12464364634813,0.));
#92296=CARTESIAN_POINT('Ctrl Pts',(46.1430594741682,2.12464364634813,20.));
#92297=CARTESIAN_POINT('Ctrl Pts',(46.1415973442202,2.09187679404497,0.));
#92298=CARTESIAN_POINT('Ctrl Pts',(46.1415973442202,2.09187679404497,20.));
#92299=CARTESIAN_POINT('Ctrl Pts',(46.1401120920793,2.05911209918102,0.));
#92300=CARTESIAN_POINT('Ctrl Pts',(46.1401120920793,2.05911209918102,20.));
#92301=CARTESIAN_POINT('Ctrl Pts',(46.1386037193727,2.02634957810318,0.));
#92302=CARTESIAN_POINT('Ctrl Pts',(46.1386037193727,2.02634957810318,20.));
#92303=CARTESIAN_POINT('Ctrl Pts',(46.1370722277379,1.99358924715754,0.));
#92304=CARTESIAN_POINT('Ctrl Pts',(46.1370722277379,1.99358924715754,20.));
#92305=CARTESIAN_POINT('Ctrl Pts',(46.1355176188236,1.96083112268931,0.));
#92306=CARTESIAN_POINT('Ctrl Pts',(46.1355176188236,1.96083112268931,20.));
#92307=CARTESIAN_POINT('Ctrl Pts',(46.1339398942902,1.9280752210434,0.));
#92308=CARTESIAN_POINT('Ctrl Pts',(46.1339398942902,1.9280752210434,20.));
#92309=CARTESIAN_POINT('Ctrl Pts',(46.1323390558096,1.89532155856415,0.));
#92310=CARTESIAN_POINT('Ctrl Pts',(46.1323390558096,1.89532155856415,20.));
#92311=CARTESIAN_POINT('Ctrl Pts',(46.1307151050651,1.86257015159583,0.));
#92312=CARTESIAN_POINT('Ctrl Pts',(46.1307151050651,1.86257015159583,20.));
#92313=CARTESIAN_POINT('Ctrl Pts',(46.1290680437528,1.82982101648207,0.));
#92314=CARTESIAN_POINT('Ctrl Pts',(46.1290680437528,1.82982101648207,20.));
#92315=CARTESIAN_POINT('Ctrl Pts',(46.1273978735796,1.79707416956535,0.));
#92316=CARTESIAN_POINT('Ctrl Pts',(46.1273978735796,1.79707416956535,20.));
#92317=CARTESIAN_POINT('Ctrl Pts',(46.1257045962649,1.76432962718686,0.));
#92318=CARTESIAN_POINT('Ctrl Pts',(46.1257045962649,1.76432962718686,20.));
#92319=CARTESIAN_POINT('Ctrl Pts',(46.1239882135394,1.73158740568598,0.));
#92320=CARTESIAN_POINT('Ctrl Pts',(46.1239882135394,1.73158740568598,20.));
#92321=CARTESIAN_POINT('Ctrl Pts',(46.1222487271454,1.6988475214004,0.));
#92322=CARTESIAN_POINT('Ctrl Pts',(46.1222487271454,1.6988475214004,20.));
#92323=CARTESIAN_POINT('Ctrl Pts',(46.1204861388364,1.66610999066656,0.));
#92324=CARTESIAN_POINT('Ctrl Pts',(46.1204861388364,1.66610999066656,20.));
#92325=CARTESIAN_POINT('Ctrl Pts',(46.1187004503775,1.63337482982071,0.));
#92326=CARTESIAN_POINT('Ctrl Pts',(46.1187004503775,1.63337482982071,20.));
#92327=CARTESIAN_POINT('Ctrl Pts',(46.1168916635447,1.60064205519959,0.));
#92328=CARTESIAN_POINT('Ctrl Pts',(46.1168916635447,1.60064205519959,20.));
#92329=CARTESIAN_POINT('Ctrl Pts',(46.1150597801266,1.56791168314158,0.));
#92330=CARTESIAN_POINT('Ctrl Pts',(46.1150597801266,1.56791168314158,20.));
#92331=CARTESIAN_POINT('Ctrl Pts',(46.1132048019234,1.53518372998667,0.));
#92332=CARTESIAN_POINT('Ctrl Pts',(46.1132048019234,1.53518372998667,20.));
#92333=CARTESIAN_POINT('Ctrl Pts',(46.111326730748,1.50245821207431,0.));
#92334=CARTESIAN_POINT('Ctrl Pts',(46.111326730748,1.50245821207431,20.));
#92335=CARTESIAN_POINT('Ctrl Pts',(46.1094255684237,1.46973514574144,0.));
#92336=CARTESIAN_POINT('Ctrl Pts',(46.1094255684237,1.46973514574144,20.));
#92337=CARTESIAN_POINT('Ctrl Pts',(46.1075013167858,1.43701454732091,0.));
#92338=CARTESIAN_POINT('Ctrl Pts',(46.1075013167858,1.43701454732091,20.));
#92339=CARTESIAN_POINT('Ctrl Pts',(46.1055539776801,1.40429643313894,0.));
#92340=CARTESIAN_POINT('Ctrl Pts',(46.1055539776801,1.40429643313894,20.));
#92341=CARTESIAN_POINT('Ctrl Pts',(46.1035835529643,1.37158081951552,0.));
#92342=CARTESIAN_POINT('Ctrl Pts',(46.1035835529643,1.37158081951552,20.));
#92343=CARTESIAN_POINT('Ctrl Pts',(46.1015900445065,1.33886772276919,0.));
#92344=CARTESIAN_POINT('Ctrl Pts',(46.1015900445065,1.33886772276919,20.));
#92345=CARTESIAN_POINT('Ctrl Pts',(46.0995734541875,1.30615715922173,0.));
#92346=CARTESIAN_POINT('Ctrl Pts',(46.0995734541875,1.30615715922173,20.));
#92347=CARTESIAN_POINT('Ctrl Pts',(46.0975337839002,1.27344914520176,0.));
#92348=CARTESIAN_POINT('Ctrl Pts',(46.0975337839002,1.27344914520176,20.));
#92349=CARTESIAN_POINT('Ctrl Pts',(46.0954710355506,1.24074369705073,0.));
#92350=CARTESIAN_POINT('Ctrl Pts',(46.0954710355506,1.24074369705073,20.));
#92351=CARTESIAN_POINT('Ctrl Pts',(46.0933852110571,1.20804083112097,0.));
#92352=CARTESIAN_POINT('Ctrl Pts',(46.0933852110571,1.20804083112097,20.));
#92353=CARTESIAN_POINT('Ctrl Pts',(46.0912763123502,1.17534056376402,0.));
#92354=CARTESIAN_POINT('Ctrl Pts',(46.0912763123502,1.17534056376402,20.));
#92355=CARTESIAN_POINT('Ctrl Pts',(46.0891443413718,1.14264291132053,0.));
#92356=CARTESIAN_POINT('Ctrl Pts',(46.0891443413718,1.14264291132053,20.));
#92357=CARTESIAN_POINT('Ctrl Pts',(46.0869893000733,1.10994789011163,0.));
#92358=CARTESIAN_POINT('Ctrl Pts',(46.0869893000733,1.10994789011163,20.));
#92359=CARTESIAN_POINT('Ctrl Pts',(46.0848111904142,1.07725551642471,0.));
#92360=CARTESIAN_POINT('Ctrl Pts',(46.0848111904142,1.07725551642471,20.));
#92361=CARTESIAN_POINT('Ctrl Pts',(46.0826100143611,1.04456580652048,0.));
#92362=CARTESIAN_POINT('Ctrl Pts',(46.0826100143611,1.04456580652048,20.));
#92363=CARTESIAN_POINT('Ctrl Pts',(46.0803857738924,1.01187877665955,0.));
#92364=CARTESIAN_POINT('Ctrl Pts',(46.0803857738924,1.01187877665955,20.));
#92365=CARTESIAN_POINT('Ctrl Pts',(46.0781384710012,0.979194443126295,0.));
#92366=CARTESIAN_POINT('Ctrl Pts',(46.0781384710012,0.979194443126295,20.));
#92367=CARTESIAN_POINT('Ctrl Pts',(46.0758681076973,0.946512822248755,0.));
#92368=CARTESIAN_POINT('Ctrl Pts',(46.0758681076973,0.946512822248755,20.));
#92369=CARTESIAN_POINT('Ctrl Pts',(46.0735746860119,0.913833930432277,0.));
#92370=CARTESIAN_POINT('Ctrl Pts',(46.0735746860119,0.913833930432277,20.));
#92371=CARTESIAN_POINT('Ctrl Pts',(46.0712582079948,0.881157784136745,0.));
#92372=CARTESIAN_POINT('Ctrl Pts',(46.0712582079948,0.881157784136745,20.));
#92373=CARTESIAN_POINT('Ctrl Pts',(46.0689186757066,0.848484399815189,0.));
#92374=CARTESIAN_POINT('Ctrl Pts',(46.0689186757066,0.848484399815189,20.));
#92375=CARTESIAN_POINT('Ctrl Pts',(46.0665560912128,0.815813793858643,0.));
#92376=CARTESIAN_POINT('Ctrl Pts',(46.0665560912128,0.815813793858643,20.));
#92377=CARTESIAN_POINT('Ctrl Pts',(46.064170456577,0.783145982548935,0.));
#92378=CARTESIAN_POINT('Ctrl Pts',(46.064170456577,0.783145982548935,20.));
#92379=CARTESIAN_POINT('Ctrl Pts',(46.0617617738521,0.750480981980926,0.));
#92380=CARTESIAN_POINT('Ctrl Pts',(46.0617617738521,0.750480981980926,20.));
#92381=CARTESIAN_POINT('Ctrl Pts',(46.0593300450868,0.71781880812973,0.));
#92382=CARTESIAN_POINT('Ctrl Pts',(46.0593300450868,0.71781880812973,20.));
#92383=CARTESIAN_POINT('Ctrl Pts',(46.0568752723439,0.685159476991768,0.));
#92384=CARTESIAN_POINT('Ctrl Pts',(46.0568752723439,0.685159476991768,20.));
#92385=CARTESIAN_POINT('Ctrl Pts',(46.0543974577158,0.652503004713265,0.));
#92386=CARTESIAN_POINT('Ctrl Pts',(46.0543974577158,0.652503004713265,20.));
#92387=CARTESIAN_POINT('Ctrl Pts',(46.0518966033391,0.619849407700868,0.));
#92388=CARTESIAN_POINT('Ctrl Pts',(46.0518966033391,0.619849407700868,20.));
#92389=CARTESIAN_POINT('Ctrl Pts',(46.0493727114182,0.587198702798626,0.));
#92390=CARTESIAN_POINT('Ctrl Pts',(46.0493727114182,0.587198702798626,20.));
#92391=CARTESIAN_POINT('Ctrl Pts',(46.0468257841997,0.554550907098833,0.));
#92392=CARTESIAN_POINT('Ctrl Pts',(46.0468257841997,0.554550907098833,20.));
#92393=CARTESIAN_POINT('Ctrl Pts',(46.044255823933,0.521906037621051,0.));
#92394=CARTESIAN_POINT('Ctrl Pts',(46.044255823933,0.521906037621051,20.));
#92395=CARTESIAN_POINT('Ctrl Pts',(46.0416628328334,0.489264111013841,0.));
#92396=CARTESIAN_POINT('Ctrl Pts',(46.0416628328334,0.489264111013841,20.));
#92397=CARTESIAN_POINT('Ctrl Pts',(46.0390468130479,0.456625143292617,0.));
#92398=CARTESIAN_POINT('Ctrl Pts',(46.0390468130479,0.456625143292617,20.));
#92399=CARTESIAN_POINT('Ctrl Pts',(46.0364077666069,0.42398914944525,0.));
#92400=CARTESIAN_POINT('Ctrl Pts',(46.0364077666069,0.42398914944525,20.));
#92401=CARTESIAN_POINT('Ctrl Pts',(46.0337456954889,0.391356143937839,0.));
#92402=CARTESIAN_POINT('Ctrl Pts',(46.0337456954889,0.391356143937839,20.));
#92403=CARTESIAN_POINT('Ctrl Pts',(46.0310606017089,0.358726141441572,0.));
#92404=CARTESIAN_POINT('Ctrl Pts',(46.0310606017089,0.358726141441572,20.));
#92405=CARTESIAN_POINT('Ctrl Pts',(46.0283524874048,0.32609915751696,0.));
#92406=CARTESIAN_POINT('Ctrl Pts',(46.0283524874048,0.32609915751696,20.));
#92407=CARTESIAN_POINT('Ctrl Pts',(46.025621354915,0.293475209241793,0.));
#92408=CARTESIAN_POINT('Ctrl Pts',(46.025621354915,0.293475209241793,20.));
#92409=CARTESIAN_POINT('Ctrl Pts',(46.022867206884,0.260854316057536,0.));
#92410=CARTESIAN_POINT('Ctrl Pts',(46.022867206884,0.260854316057536,20.));
#92411=CARTESIAN_POINT('Ctrl Pts',(46.0200900461091,0.228236498538563,0.));
#92412=CARTESIAN_POINT('Ctrl Pts',(46.0200900461091,0.228236498538563,20.));
#92413=CARTESIAN_POINT('Ctrl Pts',(46.0172898753497,0.195621776838885,0.));
#92414=CARTESIAN_POINT('Ctrl Pts',(46.0172898753497,0.195621776838885,20.));
#92415=CARTESIAN_POINT('Ctrl Pts',(46.0144666971462,0.163010169231708,0.));
#92416=CARTESIAN_POINT('Ctrl Pts',(46.0144666971462,0.163010169231708,20.));
#92417=CARTESIAN_POINT('Ctrl Pts',(46.0116205136405,0.130401690656321,0.));
#92418=CARTESIAN_POINT('Ctrl Pts',(46.0116205136405,0.130401690656321,20.));
#92419=CARTESIAN_POINT('Ctrl Pts',(46.0087513263814,0.0977963511372851,
0.));
#92420=CARTESIAN_POINT('Ctrl Pts',(46.0087513263814,0.0977963511372851,
20.));
#92421=CARTESIAN_POINT('Ctrl Pts',(46.0058591364029,0.0651941566547578,
0.));
#92422=CARTESIAN_POINT('Ctrl Pts',(46.0058591364029,0.0651941566547578,
20.));
#92423=CARTESIAN_POINT('Ctrl Pts',(46.0035269827389,0.0391149194889428,
0.));
#92424=CARTESIAN_POINT('Ctrl Pts',(46.0035269827389,0.0391149194889428,
20.));
#92425=CARTESIAN_POINT('Ctrl Pts',(46.0017675166781,0.0195569086685896,
0.));
#92426=CARTESIAN_POINT('Ctrl Pts',(46.0017675166781,0.0195569086685896,
20.));
#92427=CARTESIAN_POINT('Ctrl Pts',(46.0005899389515,0.0065188645893676,
0.));
#92428=CARTESIAN_POINT('Ctrl Pts',(46.0005899389515,0.0065188645893676,
20.));
#92429=CARTESIAN_POINT('Ctrl Pts',(46.,0.,0.));
#92430=CARTESIAN_POINT('Ctrl Pts',(46.,0.,20.));
#92431=CARTESIAN_POINT('Origin',(35.238044383473,29.5682300455808,0.));
#92432=CARTESIAN_POINT('',(35.9959384951176,30.2041787151333,0.));
#92433=CARTESIAN_POINT('Ctrl Pts',(-8.50876070567958,48.2555798975982,0.));
#92434=CARTESIAN_POINT('Ctrl Pts',(-8.50876070567958,48.2555798975982,20.));
#92435=CARTESIAN_POINT('Ctrl Pts',(-8.50201591146282,48.2561497089132,0.));
#92436=CARTESIAN_POINT('Ctrl Pts',(-8.50201591146282,48.2561497089132,20.));
#92437=CARTESIAN_POINT('Ctrl Pts',(-8.48852624368609,48.2572870022174,0.));
#92438=CARTESIAN_POINT('Ctrl Pts',(-8.48852624368609,48.2572870022174,20.));
#92439=CARTESIAN_POINT('Ctrl Pts',(-8.46829150399134,48.2589859541967,0.));
#92440=CARTESIAN_POINT('Ctrl Pts',(-8.46829150399134,48.2589859541967,20.));
#92441=CARTESIAN_POINT('Ctrl Pts',(-8.44131137500422,48.2612372475269,0.));
#92442=CARTESIAN_POINT('Ctrl Pts',(-8.44131137500422,48.2612372475269,20.));
#92443=CARTESIAN_POINT('Ctrl Pts',(-8.40758542126,48.2640280707484,0.));
#92444=CARTESIAN_POINT('Ctrl Pts',(-8.40758542126,48.2640280707484,20.));
#92445=CARTESIAN_POINT('Ctrl Pts',(-8.37385867778171,48.2667956002972,0.));
#92446=CARTESIAN_POINT('Ctrl Pts',(-8.37385867778171,48.2667956002972,20.));
#92447=CARTESIAN_POINT('Ctrl Pts',(-8.34013115014498,48.2695398358687,0.));
#92448=CARTESIAN_POINT('Ctrl Pts',(-8.34013115014498,48.2695398358687,20.));
#92449=CARTESIAN_POINT('Ctrl Pts',(-8.30640284761837,48.2722607770974,0.));
#92450=CARTESIAN_POINT('Ctrl Pts',(-8.30640284761837,48.2722607770974,20.));
#92451=CARTESIAN_POINT('Ctrl Pts',(-8.2726737841987,48.274958423567,0.));
#92452=CARTESIAN_POINT('Ctrl Pts',(-8.2726737841987,48.274958423567,20.));
#92453=CARTESIAN_POINT('Ctrl Pts',(-8.23894397736023,48.2776327748283,0.));
#92454=CARTESIAN_POINT('Ctrl Pts',(-8.23894397736023,48.2776327748283,20.));
#92455=CARTESIAN_POINT('Ctrl Pts',(-8.20521344665195,48.2802838304168,0.));
#92456=CARTESIAN_POINT('Ctrl Pts',(-8.20521344665195,48.2802838304168,20.));
#92457=CARTESIAN_POINT('Ctrl Pts',(-8.17148221231955,48.2829115898716,0.));
#92458=CARTESIAN_POINT('Ctrl Pts',(-8.17148221231955,48.2829115898716,20.));
#92459=CARTESIAN_POINT('Ctrl Pts',(-8.13775029398595,48.2855160527521,0.));
#92460=CARTESIAN_POINT('Ctrl Pts',(-8.13775029398595,48.2855160527521,20.));
#92461=CARTESIAN_POINT('Ctrl Pts',(-8.10401770912493,48.288097218659,0.));
#92462=CARTESIAN_POINT('Ctrl Pts',(-8.10401770912493,48.288097218659,20.));
#92463=CARTESIAN_POINT('Ctrl Pts',(-8.07028447346159,48.2906550872281,0.));
#92464=CARTESIAN_POINT('Ctrl Pts',(-8.07028447346159,48.2906550872281,20.));
#92465=CARTESIAN_POINT('Ctrl Pts',(-8.03655060167525,48.2931896581208,0.));
#92466=CARTESIAN_POINT('Ctrl Pts',(-8.03655060167525,48.2931896581208,20.));
#92467=CARTESIAN_POINT('Ctrl Pts',(-8.00281610801474,48.2957009310153,0.));
#92468=CARTESIAN_POINT('Ctrl Pts',(-8.00281610801474,48.2957009310153,20.));
#92469=CARTESIAN_POINT('Ctrl Pts',(-7.96908100690894,48.2981889055984,0.));
#92470=CARTESIAN_POINT('Ctrl Pts',(-7.96908100690894,48.2981889055984,20.));
#92471=CARTESIAN_POINT('Ctrl Pts',(-7.93534531368691,48.300653581555,0.));
#92472=CARTESIAN_POINT('Ctrl Pts',(-7.93534531368691,48.300653581555,20.));
#92473=CARTESIAN_POINT('Ctrl Pts',(-7.90160904447353,48.3030949585702,0.));
#92474=CARTESIAN_POINT('Ctrl Pts',(-7.90160904447353,48.3030949585702,20.));
#92475=CARTESIAN_POINT('Ctrl Pts',(-7.86787221586447,48.3055130363337,0.));
#92476=CARTESIAN_POINT('Ctrl Pts',(-7.86787221586447,48.3055130363337,20.));
#92477=CARTESIAN_POINT('Ctrl Pts',(-7.83413484466695,48.3079078145432,0.));
#92478=CARTESIAN_POINT('Ctrl Pts',(-7.83413484466695,48.3079078145432,20.));
#92479=CARTESIAN_POINT('Ctrl Pts',(-7.80039694763398,48.3102792929086,0.));
#92480=CARTESIAN_POINT('Ctrl Pts',(-7.80039694763398,48.3102792929086,20.));
#92481=CARTESIAN_POINT('Ctrl Pts',(-7.76665854114747,48.3126274711557,0.));
#92482=CARTESIAN_POINT('Ctrl Pts',(-7.76665854114747,48.3126274711557,20.));
#92483=CARTESIAN_POINT('Ctrl Pts',(-7.7329196412329,48.3149523490266,0.));
#92484=CARTESIAN_POINT('Ctrl Pts',(-7.7329196412329,48.3149523490266,20.));
#92485=CARTESIAN_POINT('Ctrl Pts',(-7.69918026370737,48.3172539262766,0.));
#92486=CARTESIAN_POINT('Ctrl Pts',(-7.69918026370737,48.3172539262766,20.));
#92487=CARTESIAN_POINT('Ctrl Pts',(-7.66544042428834,48.3195322026739,0.));
#92488=CARTESIAN_POINT('Ctrl Pts',(-7.66544042428834,48.3195322026739,20.));
#92489=CARTESIAN_POINT('Ctrl Pts',(-7.63170013870894,48.3217871779975,0.));
#92490=CARTESIAN_POINT('Ctrl Pts',(-7.63170013870894,48.3217871779975,20.));
#92491=CARTESIAN_POINT('Ctrl Pts',(-7.59795942285541,48.3240188520354,0.));
#92492=CARTESIAN_POINT('Ctrl Pts',(-7.59795942285541,48.3240188520354,20.));
#92493=CARTESIAN_POINT('Ctrl Pts',(-7.56421829277371,48.3262272245847,0.));
#92494=CARTESIAN_POINT('Ctrl Pts',(-7.56421829277371,48.3262272245847,20.));
#92495=CARTESIAN_POINT('Ctrl Pts',(-7.53047676460328,48.328412295452,0.));
#92496=CARTESIAN_POINT('Ctrl Pts',(-7.53047676460328,48.328412295452,20.));
#92497=CARTESIAN_POINT('Ctrl Pts',(-7.4967348545312,48.3305740644544,0.));
#92498=CARTESIAN_POINT('Ctrl Pts',(-7.4967348545312,48.3305740644544,20.));
#92499=CARTESIAN_POINT('Ctrl Pts',(-7.4629925787421,48.3327125314199,0.));
#92500=CARTESIAN_POINT('Ctrl Pts',(-7.4629925787421,48.3327125314199,20.));
#92501=CARTESIAN_POINT('Ctrl Pts',(-7.42924995335919,48.3348276961881,0.));
#92502=CARTESIAN_POINT('Ctrl Pts',(-7.42924995335919,48.3348276961881,20.));
#92503=CARTESIAN_POINT('Ctrl Pts',(-7.39550699443534,48.3369195586108,0.));
#92504=CARTESIAN_POINT('Ctrl Pts',(-7.39550699443534,48.3369195586108,20.));
#92505=CARTESIAN_POINT('Ctrl Pts',(-7.36176371798263,48.3389881185516,0.));
#92506=CARTESIAN_POINT('Ctrl Pts',(-7.36176371798263,48.3389881185516,20.));
#92507=CARTESIAN_POINT('Ctrl Pts',(-7.32802013999148,48.3410333758855,0.));
#92508=CARTESIAN_POINT('Ctrl Pts',(-7.32802013999148,48.3410333758855,20.));
#92509=CARTESIAN_POINT('Ctrl Pts',(-7.2942762764527,48.3430553304987,0.));
#92510=CARTESIAN_POINT('Ctrl Pts',(-7.2942762764527,48.3430553304987,20.));
#92511=CARTESIAN_POINT('Ctrl Pts',(-7.26053214338257,48.3450539822883,0.));
#92512=CARTESIAN_POINT('Ctrl Pts',(-7.26053214338257,48.3450539822883,20.));
#92513=CARTESIAN_POINT('Ctrl Pts',(-7.22678775682933,48.3470293311619,0.));
#92514=CARTESIAN_POINT('Ctrl Pts',(-7.22678775682933,48.3470293311619,20.));
#92515=CARTESIAN_POINT('Ctrl Pts',(-7.19304313285999,48.3489813770376,0.));
#92516=CARTESIAN_POINT('Ctrl Pts',(-7.19304313285999,48.3489813770376,20.));
#92517=CARTESIAN_POINT('Ctrl Pts',(-7.15929828755241,48.3509101198447,0.));
#92518=CARTESIAN_POINT('Ctrl Pts',(-7.15929828755241,48.3509101198447,20.));
#92519=CARTESIAN_POINT('Ctrl Pts',(-7.12555323698551,48.3528155595232,0.));
#92520=CARTESIAN_POINT('Ctrl Pts',(-7.12555323698551,48.3528155595232,20.));
#92521=CARTESIAN_POINT('Ctrl Pts',(-7.09180799722882,48.354697696024,0.));
#92522=CARTESIAN_POINT('Ctrl Pts',(-7.09180799722882,48.354697696024,20.));
#92523=CARTESIAN_POINT('Ctrl Pts',(-7.05806258433803,48.3565565293095,0.));
#92524=CARTESIAN_POINT('Ctrl Pts',(-7.05806258433803,48.3565565293095,20.));
#92525=CARTESIAN_POINT('Ctrl Pts',(-7.02431701436127,48.3583920593534,0.));
#92526=CARTESIAN_POINT('Ctrl Pts',(-7.02431701436127,48.3583920593534,20.));
#92527=CARTESIAN_POINT('Ctrl Pts',(-6.99057130334228,48.3602042861407,0.));
#92528=CARTESIAN_POINT('Ctrl Pts',(-6.99057130334228,48.3602042861407,20.));
#92529=CARTESIAN_POINT('Ctrl Pts',(-6.95682546732485,48.3619932096677,0.));
#92530=CARTESIAN_POINT('Ctrl Pts',(-6.95682546732485,48.3619932096677,20.));
#92531=CARTESIAN_POINT('Ctrl Pts',(-6.9230795223571,48.3637588299416,0.));
#92532=CARTESIAN_POINT('Ctrl Pts',(-6.9230795223571,48.3637588299416,20.));
#92533=CARTESIAN_POINT('Ctrl Pts',(-6.88933348449371,48.3655011469807,0.));
#92534=CARTESIAN_POINT('Ctrl Pts',(-6.88933348449371,48.3655011469807,20.));
#92535=CARTESIAN_POINT('Ctrl Pts',(-6.8555873697933,48.3672201608141,0.));
#92536=CARTESIAN_POINT('Ctrl Pts',(-6.8555873697933,48.3672201608141,20.));
#92537=CARTESIAN_POINT('Ctrl Pts',(-6.82184119431719,48.3689158714816,0.));
#92538=CARTESIAN_POINT('Ctrl Pts',(-6.82184119431719,48.3689158714816,20.));
#92539=CARTESIAN_POINT('Ctrl Pts',(-6.78809497412715,48.370588279034,0.));
#92540=CARTESIAN_POINT('Ctrl Pts',(-6.78809497412715,48.370588279034,20.));
#92541=CARTESIAN_POINT('Ctrl Pts',(-6.75434872528386,48.3722373835335,0.));
#92542=CARTESIAN_POINT('Ctrl Pts',(-6.75434872528386,48.3722373835335,20.));
#92543=CARTESIAN_POINT('Ctrl Pts',(-6.72060246384581,48.3738631850533,0.));
#92544=CARTESIAN_POINT('Ctrl Pts',(-6.72060246384581,48.3738631850533,20.));
#92545=CARTESIAN_POINT('Ctrl Pts',(-6.68685620587016,48.3754656836776,0.));
#92546=CARTESIAN_POINT('Ctrl Pts',(-6.68685620587016,48.3754656836776,20.));
#92547=CARTESIAN_POINT('Ctrl Pts',(-6.65310996741334,48.3770448795022,0.));
#92548=CARTESIAN_POINT('Ctrl Pts',(-6.65310996741334,48.3770448795022,20.));
#92549=CARTESIAN_POINT('Ctrl Pts',(-6.61936376453196,48.3786007726338,0.));
#92550=CARTESIAN_POINT('Ctrl Pts',(-6.61936376453196,48.3786007726338,20.));
#92551=CARTESIAN_POINT('Ctrl Pts',(-6.58561761328368,48.3801333631899,0.));
#92552=CARTESIAN_POINT('Ctrl Pts',(-6.58561761328368,48.3801333631899,20.));
#92553=CARTESIAN_POINT('Ctrl Pts',(-6.55187152972773,48.3816426512994,0.));
#92554=CARTESIAN_POINT('Ctrl Pts',(-6.55187152972773,48.3816426512994,20.));
#92555=CARTESIAN_POINT('Ctrl Pts',(-6.51812552992425,48.3831286371024,0.));
#92556=CARTESIAN_POINT('Ctrl Pts',(-6.51812552992425,48.3831286371024,20.));
#92557=CARTESIAN_POINT('Ctrl Pts',(-6.48437962993407,48.3845913207494,0.));
#92558=CARTESIAN_POINT('Ctrl Pts',(-6.48437962993407,48.3845913207494,20.));
#92559=CARTESIAN_POINT('Ctrl Pts',(-6.45063384581846,48.3860307024022,0.));
#92560=CARTESIAN_POINT('Ctrl Pts',(-6.45063384581846,48.3860307024022,20.));
#92561=CARTESIAN_POINT('Ctrl Pts',(-6.41688819363866,48.3874467822337,0.));
#92562=CARTESIAN_POINT('Ctrl Pts',(-6.41688819363866,48.3874467822337,20.));
#92563=CARTESIAN_POINT('Ctrl Pts',(-6.38314268945589,48.388839560428,0.));
#92564=CARTESIAN_POINT('Ctrl Pts',(-6.38314268945589,48.388839560428,20.));
#92565=CARTESIAN_POINT('Ctrl Pts',(-6.34939734933123,48.3902090371802,0.));
#92566=CARTESIAN_POINT('Ctrl Pts',(-6.34939734933123,48.3902090371802,20.));
#92567=CARTESIAN_POINT('Ctrl Pts',(-6.3156521893259,48.3915552126968,0.));
#92568=CARTESIAN_POINT('Ctrl Pts',(-6.3156521893259,48.3915552126968,20.));
#92569=CARTESIAN_POINT('Ctrl Pts',(-6.28190722550134,48.3928780871951,0.));
#92570=CARTESIAN_POINT('Ctrl Pts',(-6.28190722550134,48.3928780871951,20.));
#92571=CARTESIAN_POINT('Ctrl Pts',(-6.24816247391921,48.3941776609035,0.));
#92572=CARTESIAN_POINT('Ctrl Pts',(-6.24816247391921,48.3941776609035,20.));
#92573=CARTESIAN_POINT('Ctrl Pts',(-6.21441795064169,48.3954539340615,0.));
#92574=CARTESIAN_POINT('Ctrl Pts',(-6.21441795064169,48.3954539340615,20.));
#92575=CARTESIAN_POINT('Ctrl Pts',(-6.18067367173125,48.3967069069196,0.));
#92576=CARTESIAN_POINT('Ctrl Pts',(-6.18067367173125,48.3967069069196,20.));
#92577=CARTESIAN_POINT('Ctrl Pts',(-6.1469296532508,48.3979365797396,0.));
#92578=CARTESIAN_POINT('Ctrl Pts',(-6.1469296532508,48.3979365797396,20.));
#92579=CARTESIAN_POINT('Ctrl Pts',(-6.11318591126344,48.3991429527941,0.));
#92580=CARTESIAN_POINT('Ctrl Pts',(-6.11318591126344,48.3991429527941,20.));
#92581=CARTESIAN_POINT('Ctrl Pts',(-6.07944246183268,48.400326026367,0.));
#92582=CARTESIAN_POINT('Ctrl Pts',(-6.07944246183268,48.400326026367,20.));
#92583=CARTESIAN_POINT('Ctrl Pts',(-6.04569932102201,48.4014858007534,0.));
#92584=CARTESIAN_POINT('Ctrl Pts',(-6.04569932102201,48.4014858007534,20.));
#92585=CARTESIAN_POINT('Ctrl Pts',(-6.01195650489506,48.4026222762592,0.));
#92586=CARTESIAN_POINT('Ctrl Pts',(-6.01195650489506,48.4026222762592,20.));
#92587=CARTESIAN_POINT('Ctrl Pts',(-5.97821402951549,48.4037354532013,0.));
#92588=CARTESIAN_POINT('Ctrl Pts',(-5.97821402951549,48.4037354532013,20.));
#92589=CARTESIAN_POINT('Ctrl Pts',(-5.94447191094723,48.404825331908,0.));
#92590=CARTESIAN_POINT('Ctrl Pts',(-5.94447191094723,48.404825331908,20.));
#92591=CARTESIAN_POINT('Ctrl Pts',(-5.91073016525427,48.4058919127185,0.));
#92592=CARTESIAN_POINT('Ctrl Pts',(-5.91073016525427,48.4058919127185,20.));
#92593=CARTESIAN_POINT('Ctrl Pts',(-5.87698880850096,48.4069351959835,0.));
#92594=CARTESIAN_POINT('Ctrl Pts',(-5.87698880850096,48.4069351959835,20.));
#92595=CARTESIAN_POINT('Ctrl Pts',(-5.8432478567519,48.4079551820642,0.));
#92596=CARTESIAN_POINT('Ctrl Pts',(-5.8432478567519,48.4079551820642,20.));
#92597=CARTESIAN_POINT('Ctrl Pts',(-5.80950732607179,48.4089518713336,0.));
#92598=CARTESIAN_POINT('Ctrl Pts',(-5.80950732607179,48.4089518713336,20.));
#92599=CARTESIAN_POINT('Ctrl Pts',(-5.77576723252553,48.4099252641753,0.));
#92600=CARTESIAN_POINT('Ctrl Pts',(-5.77576723252553,48.4099252641753,20.));
#92601=CARTESIAN_POINT('Ctrl Pts',(-5.74202759217814,48.4108753609837,0.));
#92602=CARTESIAN_POINT('Ctrl Pts',(-5.74202759217814,48.4108753609837,20.));
#92603=CARTESIAN_POINT('Ctrl Pts',(-5.70828842109461,48.4118021621647,0.));
#92604=CARTESIAN_POINT('Ctrl Pts',(-5.70828842109461,48.4118021621647,20.));
#92605=CARTESIAN_POINT('Ctrl Pts',(-5.67454973534015,48.412705668135,0.));
#92606=CARTESIAN_POINT('Ctrl Pts',(-5.67454973534015,48.412705668135,20.));
#92607=CARTESIAN_POINT('Ctrl Pts',(-5.64081155098006,48.4135858793227,0.));
#92608=CARTESIAN_POINT('Ctrl Pts',(-5.64081155098006,48.4135858793227,20.));
#92609=CARTESIAN_POINT('Ctrl Pts',(-5.60707388407982,48.414442796167,0.));
#92610=CARTESIAN_POINT('Ctrl Pts',(-5.60707388407982,48.414442796167,20.));
#92611=CARTESIAN_POINT('Ctrl Pts',(-5.57333675070493,48.4152764191183,0.));
#92612=CARTESIAN_POINT('Ctrl Pts',(-5.57333675070493,48.4152764191183,20.));
#92613=CARTESIAN_POINT('Ctrl Pts',(-5.53960016692118,48.4160867486381,0.));
#92614=CARTESIAN_POINT('Ctrl Pts',(-5.53960016692118,48.4160867486381,20.));
#92615=CARTESIAN_POINT('Ctrl Pts',(-5.50586414879431,48.4168737851989,0.));
#92616=CARTESIAN_POINT('Ctrl Pts',(-5.50586414879431,48.4168737851989,20.));
#92617=CARTESIAN_POINT('Ctrl Pts',(-5.47212871239031,48.417637529284,0.));
#92618=CARTESIAN_POINT('Ctrl Pts',(-5.47212871239031,48.417637529284,20.));
#92619=CARTESIAN_POINT('Ctrl Pts',(-5.43839387377499,48.4183779813881,0.));
#92620=CARTESIAN_POINT('Ctrl Pts',(-5.43839387377499,48.4183779813881,20.));
#92621=CARTESIAN_POINT('Ctrl Pts',(-5.40465964901426,48.4190951420167,0.));
#92622=CARTESIAN_POINT('Ctrl Pts',(-5.40465964901426,48.4190951420167,20.));
#92623=CARTESIAN_POINT('Ctrl Pts',(-5.37092605417403,48.4197890116867,0.));
#92624=CARTESIAN_POINT('Ctrl Pts',(-5.37092605417403,48.4197890116867,20.));
#92625=CARTESIAN_POINT('Ctrl Pts',(-5.33719310532028,48.4204595909261,0.));
#92626=CARTESIAN_POINT('Ctrl Pts',(-5.33719310532028,48.4204595909261,20.));
#92627=CARTESIAN_POINT('Ctrl Pts',(-5.3034608185191,48.4211068802741,0.));
#92628=CARTESIAN_POINT('Ctrl Pts',(-5.3034608185191,48.4211068802741,20.));
#92629=CARTESIAN_POINT('Ctrl Pts',(-5.26972920983671,48.4217308802807,0.));
#92630=CARTESIAN_POINT('Ctrl Pts',(-5.26972920983671,48.4217308802807,20.));
#92631=CARTESIAN_POINT('Ctrl Pts',(-5.23599829533945,48.4223315915069,0.));
#92632=CARTESIAN_POINT('Ctrl Pts',(-5.23599829533945,48.4223315915069,20.));
#92633=CARTESIAN_POINT('Ctrl Pts',(-5.20226809109352,48.4229090145253,0.));
#92634=CARTESIAN_POINT('Ctrl Pts',(-5.20226809109352,48.4229090145253,20.));
#92635=CARTESIAN_POINT('Ctrl Pts',(-5.16853861316522,48.4234631499193,0.));
#92636=CARTESIAN_POINT('Ctrl Pts',(-5.16853861316522,48.4234631499193,20.));
#92637=CARTESIAN_POINT('Ctrl Pts',(-5.13480987762072,48.4239939982838,0.));
#92638=CARTESIAN_POINT('Ctrl Pts',(-5.13480987762072,48.4239939982838,20.));
#92639=CARTESIAN_POINT('Ctrl Pts',(-5.10108190052608,48.4245015602246,0.));
#92640=CARTESIAN_POINT('Ctrl Pts',(-5.10108190052608,48.4245015602246,20.));
#92641=CARTESIAN_POINT('Ctrl Pts',(-5.06735469794743,48.4249858363582,0.));
#92642=CARTESIAN_POINT('Ctrl Pts',(-5.06735469794743,48.4249858363582,20.));
#92643=CARTESIAN_POINT('Ctrl Pts',(-5.03362828595094,48.4254468273122,0.));
#92644=CARTESIAN_POINT('Ctrl Pts',(-5.03362828595094,48.4254468273122,20.));
#92645=CARTESIAN_POINT('Ctrl Pts',(-4.99990268060293,48.4258845337255,0.));
#92646=CARTESIAN_POINT('Ctrl Pts',(-4.99990268060293,48.4258845337255,20.));
#92647=CARTESIAN_POINT('Ctrl Pts',(-4.96617789796954,48.4262989562483,0.));
#92648=CARTESIAN_POINT('Ctrl Pts',(-4.96617789796954,48.4262989562483,20.));
#92649=CARTESIAN_POINT('Ctrl Pts',(-4.93245395411686,48.4266900955418,0.));
#92650=CARTESIAN_POINT('Ctrl Pts',(-4.93245395411686,48.4266900955418,20.));
#92651=CARTESIAN_POINT('Ctrl Pts',(-4.89873086511077,48.4270579522784,0.));
#92652=CARTESIAN_POINT('Ctrl Pts',(-4.89873086511077,48.4270579522784,20.));
#92653=CARTESIAN_POINT('Ctrl Pts',(-4.86500864701731,48.4274025271416,0.));
#92654=CARTESIAN_POINT('Ctrl Pts',(-4.86500864701731,48.4274025271416,20.));
#92655=CARTESIAN_POINT('Ctrl Pts',(-4.8312873159023,48.4277238208263,0.));
#92656=CARTESIAN_POINT('Ctrl Pts',(-4.8312873159023,48.4277238208263,20.));
#92657=CARTESIAN_POINT('Ctrl Pts',(-4.79756688783169,48.4280218340382,0.));
#92658=CARTESIAN_POINT('Ctrl Pts',(-4.79756688783169,48.4280218340382,20.));
#92659=CARTESIAN_POINT('Ctrl Pts',(-4.76384737887107,48.4282965674942,0.));
#92660=CARTESIAN_POINT('Ctrl Pts',(-4.76384737887107,48.4282965674942,20.));
#92661=CARTESIAN_POINT('Ctrl Pts',(-4.73012880508602,48.4285480219221,0.));
#92662=CARTESIAN_POINT('Ctrl Pts',(-4.73012880508602,48.4285480219221,20.));
#92663=CARTESIAN_POINT('Ctrl Pts',(-4.69641118254227,48.4287761980604,0.));
#92664=CARTESIAN_POINT('Ctrl Pts',(-4.69641118254227,48.4287761980604,20.));
#92665=CARTESIAN_POINT('Ctrl Pts',(-4.66269452730544,48.4289810966589,0.));
#92666=CARTESIAN_POINT('Ctrl Pts',(-4.66269452730544,48.4289810966589,20.));
#92667=CARTESIAN_POINT('Ctrl Pts',(-4.62897885544098,48.4291627184787,0.));
#92668=CARTESIAN_POINT('Ctrl Pts',(-4.62897885544098,48.4291627184787,20.));
#92669=CARTESIAN_POINT('Ctrl Pts',(-4.5952641830141,48.4293210642923,0.));
#92670=CARTESIAN_POINT('Ctrl Pts',(-4.5952641830141,48.4293210642923,20.));
#92671=CARTESIAN_POINT('Ctrl Pts',(-4.56155052608981,48.4294561348833,0.));
#92672=CARTESIAN_POINT('Ctrl Pts',(-4.56155052608981,48.4294561348833,20.));
#92673=CARTESIAN_POINT('Ctrl Pts',(-4.52783790073295,48.4295679310466,0.));
#92674=CARTESIAN_POINT('Ctrl Pts',(-4.52783790073295,48.4295679310466,20.));
#92675=CARTESIAN_POINT('Ctrl Pts',(-4.49412632300816,48.4296564535884,0.));
#92676=CARTESIAN_POINT('Ctrl Pts',(-4.49412632300816,48.4296564535884,20.));
#92677=CARTESIAN_POINT('Ctrl Pts',(-4.46041580898013,48.4297217033257,0.));
#92678=CARTESIAN_POINT('Ctrl Pts',(-4.46041580898013,48.4297217033257,20.));
#92679=CARTESIAN_POINT('Ctrl Pts',(-4.42670637471342,48.4297636810863,0.));
#92680=CARTESIAN_POINT('Ctrl Pts',(-4.42670637471342,48.4297636810863,20.));
#92681=CARTESIAN_POINT('Ctrl Pts',(-4.39299803627247,48.4297823877088,0.));
#92682=CARTESIAN_POINT('Ctrl Pts',(-4.39299803627247,48.4297823877088,20.));
#92683=CARTESIAN_POINT('Ctrl Pts',(-4.35929080972167,48.4297778240431,0.));
#92684=CARTESIAN_POINT('Ctrl Pts',(-4.35929080972167,48.4297778240431,20.));
#92685=CARTESIAN_POINT('Ctrl Pts',(-4.32558471112518,48.42974999095,0.));
#92686=CARTESIAN_POINT('Ctrl Pts',(-4.32558471112518,48.42974999095,20.));
#92687=CARTESIAN_POINT('Ctrl Pts',(-4.29187975654678,48.4296988893018,0.));
#92688=CARTESIAN_POINT('Ctrl Pts',(-4.29187975654678,48.4296988893018,20.));
#92689=CARTESIAN_POINT('Ctrl Pts',(-4.25817596205002,48.4296245199823,0.));
#92690=CARTESIAN_POINT('Ctrl Pts',(-4.25817596205002,48.4296245199823,20.));
#92691=CARTESIAN_POINT('Ctrl Pts',(-4.22447334369802,48.4295268838864,0.));
#92692=CARTESIAN_POINT('Ctrl Pts',(-4.22447334369802,48.4295268838864,20.));
#92693=CARTESIAN_POINT('Ctrl Pts',(-4.19077191755407,48.4294059819202,0.));
#92694=CARTESIAN_POINT('Ctrl Pts',(-4.19077191755407,48.4294059819202,20.));
#92695=CARTESIAN_POINT('Ctrl Pts',(-4.15707169968116,48.4292618150011,0.));
#92696=CARTESIAN_POINT('Ctrl Pts',(-4.15707169968116,48.4292618150011,20.));
#92697=CARTESIAN_POINT('Ctrl Pts',(-4.12337270614212,48.429094384057,0.));
#92698=CARTESIAN_POINT('Ctrl Pts',(-4.12337270614212,48.429094384057,20.));
#92699=CARTESIAN_POINT('Ctrl Pts',(-4.08967495299953,48.4289036900268,0.));
#92700=CARTESIAN_POINT('Ctrl Pts',(-4.08967495299953,48.4289036900268,20.));
#92701=CARTESIAN_POINT('Ctrl Pts',(-4.0559784563157,48.4286897338604,0.));
#92702=CARTESIAN_POINT('Ctrl Pts',(-4.0559784563157,48.4286897338604,20.));
#92703=CARTESIAN_POINT('Ctrl Pts',(-4.02228323215261,48.4284525165189,0.));
#92704=CARTESIAN_POINT('Ctrl Pts',(-4.02228323215261,48.4284525165189,20.));
#92705=CARTESIAN_POINT('Ctrl Pts',(-3.98858929657202,48.4281920389749,0.));
#92706=CARTESIAN_POINT('Ctrl Pts',(-3.98858929657202,48.4281920389749,20.));
#92707=CARTESIAN_POINT('Ctrl Pts',(-3.9548966656355,48.427908302212,0.));
#92708=CARTESIAN_POINT('Ctrl Pts',(-3.9548966656355,48.427908302212,20.));
#92709=CARTESIAN_POINT('Ctrl Pts',(-3.92120535540421,48.4276013072253,0.));
#92710=CARTESIAN_POINT('Ctrl Pts',(-3.92120535540421,48.4276013072253,20.));
#92711=CARTESIAN_POINT('Ctrl Pts',(-3.88751538193921,48.4272710550206,0.));
#92712=CARTESIAN_POINT('Ctrl Pts',(-3.88751538193921,48.4272710550206,20.));
#92713=CARTESIAN_POINT('Ctrl Pts',(-3.85382676130116,48.4269175466151,0.));
#92714=CARTESIAN_POINT('Ctrl Pts',(-3.85382676130116,48.4269175466151,20.));
#92715=CARTESIAN_POINT('Ctrl Pts',(-3.82013950955044,48.4265407830367,0.));
#92716=CARTESIAN_POINT('Ctrl Pts',(-3.82013950955044,48.4265407830367,20.));
#92717=CARTESIAN_POINT('Ctrl Pts',(-3.78645364274707,48.4261407653249,0.));
#92718=CARTESIAN_POINT('Ctrl Pts',(-3.78645364274707,48.4261407653249,20.));
#92719=CARTESIAN_POINT('Ctrl Pts',(-3.75276917695086,48.4257174945299,0.));
#92720=CARTESIAN_POINT('Ctrl Pts',(-3.75276917695086,48.4257174945299,20.));
#92721=CARTESIAN_POINT('Ctrl Pts',(-3.7190861282211,48.4252709717129,0.));
#92722=CARTESIAN_POINT('Ctrl Pts',(-3.7190861282211,48.4252709717129,20.));
#92723=CARTESIAN_POINT('Ctrl Pts',(-3.68540451261697,48.424801197947,0.));
#92724=CARTESIAN_POINT('Ctrl Pts',(-3.68540451261697,48.424801197947,20.));
#92725=CARTESIAN_POINT('Ctrl Pts',(-3.65172434619742,48.4243081743158,0.));
#92726=CARTESIAN_POINT('Ctrl Pts',(-3.65172434619742,48.4243081743158,20.));
#92727=CARTESIAN_POINT('Ctrl Pts',(-3.61804564502098,48.4237919019141,0.));
#92728=CARTESIAN_POINT('Ctrl Pts',(-3.61804564502098,48.4237919019141,20.));
#92729=CARTESIAN_POINT('Ctrl Pts',(-3.58436842514565,48.4232523818483,0.));
#92730=CARTESIAN_POINT('Ctrl Pts',(-3.58436842514565,48.4232523818483,20.));
#92731=CARTESIAN_POINT('Ctrl Pts',(-3.55069270262909,48.4226896152354,0.));
#92732=CARTESIAN_POINT('Ctrl Pts',(-3.55069270262909,48.4226896152354,20.));
#92733=CARTESIAN_POINT('Ctrl Pts',(-3.51701849352855,48.422103603204,0.));
#92734=CARTESIAN_POINT('Ctrl Pts',(-3.51701849352855,48.422103603204,20.));
#92735=CARTESIAN_POINT('Ctrl Pts',(-3.48334581390102,48.4214943468927,0.));
#92736=CARTESIAN_POINT('Ctrl Pts',(-3.48334581390102,48.4214943468927,20.));
#92737=CARTESIAN_POINT('Ctrl Pts',(-3.44967467980324,48.4208618474523,0.));
#92738=CARTESIAN_POINT('Ctrl Pts',(-3.44967467980324,48.4208618474523,20.));
#92739=CARTESIAN_POINT('Ctrl Pts',(-3.4160051072915,48.4202061060442,0.));
#92740=CARTESIAN_POINT('Ctrl Pts',(-3.4160051072915,48.4202061060442,20.));
#92741=CARTESIAN_POINT('Ctrl Pts',(-3.38233711242168,48.4195271238417,0.));
#92742=CARTESIAN_POINT('Ctrl Pts',(-3.38233711242168,48.4195271238417,20.));
#92743=CARTESIAN_POINT('Ctrl Pts',(-3.34867071124919,48.4188249020284,0.));
#92744=CARTESIAN_POINT('Ctrl Pts',(-3.34867071124919,48.4188249020284,20.));
#92745=CARTESIAN_POINT('Ctrl Pts',(-3.31500591982889,48.4180994417999,0.));
#92746=CARTESIAN_POINT('Ctrl Pts',(-3.31500591982889,48.4180994417999,20.));
#92747=CARTESIAN_POINT('Ctrl Pts',(-3.28134275421533,48.4173507443625,0.));
#92748=CARTESIAN_POINT('Ctrl Pts',(-3.28134275421533,48.4173507443625,20.));
#92749=CARTESIAN_POINT('Ctrl Pts',(-3.24768123046267,48.4165788109335,0.));
#92750=CARTESIAN_POINT('Ctrl Pts',(-3.24768123046267,48.4165788109335,20.));
#92751=CARTESIAN_POINT('Ctrl Pts',(-3.21402136462459,48.4157836427414,0.));
#92752=CARTESIAN_POINT('Ctrl Pts',(-3.21402136462459,48.4157836427414,20.));
#92753=CARTESIAN_POINT('Ctrl Pts',(-3.18036317275455,48.4149652410254,0.));
#92754=CARTESIAN_POINT('Ctrl Pts',(-3.18036317275455,48.4149652410254,20.));
#92755=CARTESIAN_POINT('Ctrl Pts',(-3.14670667090557,48.414123607036,0.));
#92756=CARTESIAN_POINT('Ctrl Pts',(-3.14670667090557,48.414123607036,20.));
#92757=CARTESIAN_POINT('Ctrl Pts',(-3.11305187513001,48.4132587420349,0.));
#92758=CARTESIAN_POINT('Ctrl Pts',(-3.11305187513001,48.4132587420349,20.));
#92759=CARTESIAN_POINT('Ctrl Pts',(-3.0793988014797,48.4123706472953,0.));
#92760=CARTESIAN_POINT('Ctrl Pts',(-3.0793988014797,48.4123706472953,20.));
#92761=CARTESIAN_POINT('Ctrl Pts',(-3.04574746600609,48.4114593241014,0.));
#92762=CARTESIAN_POINT('Ctrl Pts',(-3.04574746600609,48.4114593241014,20.));
#92763=CARTESIAN_POINT('Ctrl Pts',(-3.01209788475996,48.4105247737488,0.));
#92764=CARTESIAN_POINT('Ctrl Pts',(-3.01209788475996,48.4105247737488,20.));
#92765=CARTESIAN_POINT('Ctrl Pts',(-2.97845007379182,48.4095669975441,0.));
#92766=CARTESIAN_POINT('Ctrl Pts',(-2.97845007379182,48.4095669975441,20.));
#92767=CARTESIAN_POINT('Ctrl Pts',(-2.94480404915165,48.4085859968048,0.));
#92768=CARTESIAN_POINT('Ctrl Pts',(-2.94480404915165,48.4085859968048,20.));
#92769=CARTESIAN_POINT('Ctrl Pts',(-2.91115982688905,48.4075817728593,0.));
#92770=CARTESIAN_POINT('Ctrl Pts',(-2.91115982688905,48.4075817728593,20.));
#92771=CARTESIAN_POINT('Ctrl Pts',(-2.87751742305295,48.4065543270471,0.));
#92772=CARTESIAN_POINT('Ctrl Pts',(-2.87751742305295,48.4065543270471,20.));
#92773=CARTESIAN_POINT('Ctrl Pts',(-2.84387685369182,48.4055036607195,0.));
#92774=CARTESIAN_POINT('Ctrl Pts',(-2.84387685369182,48.4055036607195,20.));
#92775=CARTESIAN_POINT('Ctrl Pts',(-2.81023813485357,48.4044297752383,0.));
#92776=CARTESIAN_POINT('Ctrl Pts',(-2.81023813485357,48.4044297752383,20.));
#92777=CARTESIAN_POINT('Ctrl Pts',(-2.77660128258548,48.4033326719771,0.));
#92778=CARTESIAN_POINT('Ctrl Pts',(-2.77660128258548,48.4033326719771,20.));
#92779=CARTESIAN_POINT('Ctrl Pts',(-2.74296631293438,48.4022123523201,0.));
#92780=CARTESIAN_POINT('Ctrl Pts',(-2.74296631293438,48.4022123523201,20.));
#92781=CARTESIAN_POINT('Ctrl Pts',(-2.70933324194662,48.4010688176627,0.));
#92782=CARTESIAN_POINT('Ctrl Pts',(-2.70933324194662,48.4010688176627,20.));
#92783=CARTESIAN_POINT('Ctrl Pts',(-2.67570208566795,48.3999020694116,0.));
#92784=CARTESIAN_POINT('Ctrl Pts',(-2.67570208566795,48.3999020694116,20.));
#92785=CARTESIAN_POINT('Ctrl Pts',(-2.64207286014351,48.3987121089844,0.));
#92786=CARTESIAN_POINT('Ctrl Pts',(-2.64207286014351,48.3987121089844,20.));
#92787=CARTESIAN_POINT('Ctrl Pts',(-2.60844558141791,48.3974989378103,0.));
#92788=CARTESIAN_POINT('Ctrl Pts',(-2.60844558141791,48.3974989378103,20.));
#92789=CARTESIAN_POINT('Ctrl Pts',(-2.57482026553517,48.3962625573292,0.));
#92790=CARTESIAN_POINT('Ctrl Pts',(-2.57482026553517,48.3962625573292,20.));
#92791=CARTESIAN_POINT('Ctrl Pts',(-2.54119692853862,48.3950029689925,0.));
#92792=CARTESIAN_POINT('Ctrl Pts',(-2.54119692853862,48.3950029689925,20.));
#92793=CARTESIAN_POINT('Ctrl Pts',(-2.50757558647122,48.3937201742621,0.));
#92794=CARTESIAN_POINT('Ctrl Pts',(-2.50757558647122,48.3937201742621,20.));
#92795=CARTESIAN_POINT('Ctrl Pts',(-2.47395625537496,48.3924141746117,0.));
#92796=CARTESIAN_POINT('Ctrl Pts',(-2.47395625537496,48.3924141746117,20.));
#92797=CARTESIAN_POINT('Ctrl Pts',(-2.44033895129154,48.3910849715258,0.));
#92798=CARTESIAN_POINT('Ctrl Pts',(-2.44033895129154,48.3910849715258,20.));
#92799=CARTESIAN_POINT('Ctrl Pts',(-2.40672369026198,48.3897325665,0.));
#92800=CARTESIAN_POINT('Ctrl Pts',(-2.40672369026198,48.3897325665,20.));
#92801=CARTESIAN_POINT('Ctrl Pts',(-2.37311048832666,48.3883569610415,0.));
#92802=CARTESIAN_POINT('Ctrl Pts',(-2.37311048832666,48.3883569610415,20.));
#92803=CARTESIAN_POINT('Ctrl Pts',(-2.33949936152535,48.3869581566679,0.));
#92804=CARTESIAN_POINT('Ctrl Pts',(-2.33949936152535,48.3869581566679,20.));
#92805=CARTESIAN_POINT('Ctrl Pts',(-2.30589032589701,48.3855361549086,0.));
#92806=CARTESIAN_POINT('Ctrl Pts',(-2.30589032589701,48.3855361549086,20.));
#92807=CARTESIAN_POINT('Ctrl Pts',(-2.2722833974801,48.3840909573039,0.));
#92808=CARTESIAN_POINT('Ctrl Pts',(-2.2722833974801,48.3840909573039,20.));
#92809=CARTESIAN_POINT('Ctrl Pts',(-2.23867859231222,48.3826225654055,0.));
#92810=CARTESIAN_POINT('Ctrl Pts',(-2.23867859231222,48.3826225654055,20.));
#92811=CARTESIAN_POINT('Ctrl Pts',(-2.20507592643043,48.3811309807756,0.));
#92812=CARTESIAN_POINT('Ctrl Pts',(-2.20507592643043,48.3811309807756,20.));
#92813=CARTESIAN_POINT('Ctrl Pts',(-2.17147541587105,48.3796162049883,0.));
#92814=CARTESIAN_POINT('Ctrl Pts',(-2.17147541587105,48.3796162049883,20.));
#92815=CARTESIAN_POINT('Ctrl Pts',(-2.13787707667014,48.3780782396279,0.));
#92816=CARTESIAN_POINT('Ctrl Pts',(-2.13787707667014,48.3780782396279,20.));
#92817=CARTESIAN_POINT('Ctrl Pts',(-2.10428092486295,48.3765170862905,0.));
#92818=CARTESIAN_POINT('Ctrl Pts',(-2.10428092486295,48.3765170862905,20.));
#92819=CARTESIAN_POINT('Ctrl Pts',(-2.07068697648389,48.374932746583,0.));
#92820=CARTESIAN_POINT('Ctrl Pts',(-2.07068697648389,48.374932746583,20.));
#92821=CARTESIAN_POINT('Ctrl Pts',(-2.03709524756656,48.3733252221237,0.));
#92822=CARTESIAN_POINT('Ctrl Pts',(-2.03709524756656,48.3733252221237,20.));
#92823=CARTESIAN_POINT('Ctrl Pts',(-2.00350575414356,48.3716945145424,0.));
#92824=CARTESIAN_POINT('Ctrl Pts',(-2.00350575414356,48.3716945145424,20.));
#92825=CARTESIAN_POINT('Ctrl Pts',(-1.96991851224693,48.3700406254798,0.));
#92826=CARTESIAN_POINT('Ctrl Pts',(-1.96991851224693,48.3700406254798,20.));
#92827=CARTESIAN_POINT('Ctrl Pts',(-1.93633353790814,48.3683635565876,0.));
#92828=CARTESIAN_POINT('Ctrl Pts',(-1.93633353790814,48.3683635565876,20.));
#92829=CARTESIAN_POINT('Ctrl Pts',(-1.90275084715797,48.3666633095284,0.));
#92830=CARTESIAN_POINT('Ctrl Pts',(-1.90275084715797,48.3666633095284,20.));
#92831=CARTESIAN_POINT('Ctrl Pts',(-1.86917045602653,48.3649398859758,0.));
#92832=CARTESIAN_POINT('Ctrl Pts',(-1.86917045602653,48.3649398859758,20.));
#92833=CARTESIAN_POINT('Ctrl Pts',(-1.83559238054324,48.3631932876149,0.));
#92834=CARTESIAN_POINT('Ctrl Pts',(-1.83559238054324,48.3631932876149,20.));
#92835=CARTESIAN_POINT('Ctrl Pts',(-1.80201663673657,48.3614235161422,0.));
#92836=CARTESIAN_POINT('Ctrl Pts',(-1.80201663673657,48.3614235161422,20.));
#92837=CARTESIAN_POINT('Ctrl Pts',(-1.76844324063427,48.3596305732653,0.));
#92838=CARTESIAN_POINT('Ctrl Pts',(-1.76844324063427,48.3596305732653,20.));
#92839=CARTESIAN_POINT('Ctrl Pts',(-1.73487220826327,48.357814460703,0.));
#92840=CARTESIAN_POINT('Ctrl Pts',(-1.73487220826327,48.357814460703,20.));
#92841=CARTESIAN_POINT('Ctrl Pts',(-1.70130355564958,48.3559751801849,0.));
#92842=CARTESIAN_POINT('Ctrl Pts',(-1.70130355564958,48.3559751801849,20.));
#92843=CARTESIAN_POINT('Ctrl Pts',(-1.66773729881857,48.3541127334515,0.));
#92844=CARTESIAN_POINT('Ctrl Pts',(-1.66773729881857,48.3541127334515,20.));
#92845=CARTESIAN_POINT('Ctrl Pts',(-1.63417345379483,48.3522271222546,0.));
#92846=CARTESIAN_POINT('Ctrl Pts',(-1.63417345379483,48.3522271222546,20.));
#92847=CARTESIAN_POINT('Ctrl Pts',(-1.60061203660208,48.350318348357,0.));
#92848=CARTESIAN_POINT('Ctrl Pts',(-1.60061203660208,48.350318348357,20.));
#92849=CARTESIAN_POINT('Ctrl Pts',(-1.56705306326333,48.3483864135332,0.));
#92850=CARTESIAN_POINT('Ctrl Pts',(-1.56705306326333,48.3483864135332,20.));
#92851=CARTESIAN_POINT('Ctrl Pts',(-1.53349654980078,48.3464313195685,0.));
#92852=CARTESIAN_POINT('Ctrl Pts',(-1.53349654980078,48.3464313195685,20.));
#92853=CARTESIAN_POINT('Ctrl Pts',(-1.49994251223572,48.3444530682597,0.));
#92854=CARTESIAN_POINT('Ctrl Pts',(-1.49994251223572,48.3444530682597,20.));
#92855=CARTESIAN_POINT('Ctrl Pts',(-1.46639096658853,48.3424516614145,0.));
#92856=CARTESIAN_POINT('Ctrl Pts',(-1.46639096658853,48.3424516614145,20.));
#92857=CARTESIAN_POINT('Ctrl Pts',(-1.4328419288788,48.3404271008519,0.));
#92858=CARTESIAN_POINT('Ctrl Pts',(-1.4328419288788,48.3404271008519,20.));
#92859=CARTESIAN_POINT('Ctrl Pts',(-1.39929541512521,48.3383793884017,0.));
#92860=CARTESIAN_POINT('Ctrl Pts',(-1.39929541512521,48.3383793884017,20.));
#92861=CARTESIAN_POINT('Ctrl Pts',(-1.36575144134572,48.336308525905,0.));
#92862=CARTESIAN_POINT('Ctrl Pts',(-1.36575144134572,48.336308525905,20.));
#92863=CARTESIAN_POINT('Ctrl Pts',(-1.33221002355744,48.3342145152137,0.));
#92864=CARTESIAN_POINT('Ctrl Pts',(-1.33221002355744,48.3342145152137,20.));
#92865=CARTESIAN_POINT('Ctrl Pts',(-1.29867117777653,48.3320973581913,0.));
#92866=CARTESIAN_POINT('Ctrl Pts',(-1.29867117777653,48.3320973581913,20.));
#92867=CARTESIAN_POINT('Ctrl Pts',(-1.26513492001823,48.3299570567123,0.));
#92868=CARTESIAN_POINT('Ctrl Pts',(-1.26513492001823,48.3299570567123,20.));
#92869=CARTESIAN_POINT('Ctrl Pts',(-1.23160126629694,48.3277936126623,0.));
#92870=CARTESIAN_POINT('Ctrl Pts',(-1.23160126629694,48.3277936126623,20.));
#92871=CARTESIAN_POINT('Ctrl Pts',(-1.19807023262612,48.3256070279384,0.));
#92872=CARTESIAN_POINT('Ctrl Pts',(-1.19807023262612,48.3256070279384,20.));
#92873=CARTESIAN_POINT('Ctrl Pts',(-1.1645418350184,48.3233973044482,0.));
#92874=CARTESIAN_POINT('Ctrl Pts',(-1.1645418350184,48.3233973044482,20.));
#92875=CARTESIAN_POINT('Ctrl Pts',(-1.13101608948536,48.3211644441107,0.));
#92876=CARTESIAN_POINT('Ctrl Pts',(-1.13101608948536,48.3211644441107,20.));
#92877=CARTESIAN_POINT('Ctrl Pts',(-1.09749301203764,48.3189084488565,0.));
#92878=CARTESIAN_POINT('Ctrl Pts',(-1.09749301203764,48.3189084488565,20.));
#92879=CARTESIAN_POINT('Ctrl Pts',(-1.06397261868501,48.3166293206271,0.));
#92880=CARTESIAN_POINT('Ctrl Pts',(-1.06397261868501,48.3166293206271,20.));
#92881=CARTESIAN_POINT('Ctrl Pts',(-1.03045492543642,48.3143270613748,0.));
#92882=CARTESIAN_POINT('Ctrl Pts',(-1.03045492543642,48.3143270613748,20.));
#92883=CARTESIAN_POINT('Ctrl Pts',(-0.996939948299871,48.312001673063,0.));
#92884=CARTESIAN_POINT('Ctrl Pts',(-0.996939948299871,48.312001673063,20.));
#92885=CARTESIAN_POINT('Ctrl Pts',(-0.963427703282371,48.3096531576664,
0.));
#92886=CARTESIAN_POINT('Ctrl Pts',(-0.963427703282371,48.3096531576664,
20.));
#92887=CARTESIAN_POINT('Ctrl Pts',(-0.929918206389844,48.3072815171712,
0.));
#92888=CARTESIAN_POINT('Ctrl Pts',(-0.929918206389844,48.3072815171712,
20.));
#92889=CARTESIAN_POINT('Ctrl Pts',(-0.896411473627245,48.3048867535745,
0.));
#92890=CARTESIAN_POINT('Ctrl Pts',(-0.896411473627245,48.3048867535745,
20.));
#92891=CARTESIAN_POINT('Ctrl Pts',(-0.862907520998508,48.3024688688845,
0.));
#92892=CARTESIAN_POINT('Ctrl Pts',(-0.862907520998508,48.3024688688845,
20.));
#92893=CARTESIAN_POINT('Ctrl Pts',(-0.829406364506684,48.3000278651208,
0.));
#92894=CARTESIAN_POINT('Ctrl Pts',(-0.829406364506684,48.3000278651208,
20.));
#92895=CARTESIAN_POINT('Ctrl Pts',(-0.79590802015391,48.2975637443136,0.));
#92896=CARTESIAN_POINT('Ctrl Pts',(-0.79590802015391,48.2975637443136,20.));
#92897=CARTESIAN_POINT('Ctrl Pts',(-0.762412503941543,48.2950765085043,
0.));
#92898=CARTESIAN_POINT('Ctrl Pts',(-0.762412503941543,48.2950765085043,
20.));
#92899=CARTESIAN_POINT('Ctrl Pts',(-0.728919831869663,48.2925661597457,
0.));
#92900=CARTESIAN_POINT('Ctrl Pts',(-0.728919831869663,48.2925661597457,
20.));
#92901=CARTESIAN_POINT('Ctrl Pts',(-0.695430019937358,48.2900327001016,
0.));
#92902=CARTESIAN_POINT('Ctrl Pts',(-0.695430019937358,48.2900327001016,
20.));
#92903=CARTESIAN_POINT('Ctrl Pts',(-0.66194308414246,48.2874761316474,0.));
#92904=CARTESIAN_POINT('Ctrl Pts',(-0.66194308414246,48.2874761316474,20.));
#92905=CARTESIAN_POINT('Ctrl Pts',(-0.628459040481846,48.2848964564694,
0.));
#92906=CARTESIAN_POINT('Ctrl Pts',(-0.628459040481846,48.2848964564694,
20.));
#92907=CARTESIAN_POINT('Ctrl Pts',(-0.594977904951284,48.282293676665,0.));
#92908=CARTESIAN_POINT('Ctrl Pts',(-0.594977904951284,48.282293676665,20.));
#92909=CARTESIAN_POINT('Ctrl Pts',(-0.561499693545691,48.2796677943426,
0.));
#92910=CARTESIAN_POINT('Ctrl Pts',(-0.561499693545691,48.2796677943426,
20.));
#92911=CARTESIAN_POINT('Ctrl Pts',(-0.528024422259037,48.2770188116216,
0.));
#92912=CARTESIAN_POINT('Ctrl Pts',(-0.528024422259037,48.2770188116216,
20.));
#92913=CARTESIAN_POINT('Ctrl Pts',(-0.494552107084227,48.2743467306329,
0.));
#92914=CARTESIAN_POINT('Ctrl Pts',(-0.494552107084227,48.2743467306329,
20.));
#92915=CARTESIAN_POINT('Ctrl Pts',(-0.461082764013003,48.2716515535183,
0.));
#92916=CARTESIAN_POINT('Ctrl Pts',(-0.461082764013003,48.2716515535183,
20.));
#92917=CARTESIAN_POINT('Ctrl Pts',(-0.427616409036058,48.2689332824309,
0.));
#92918=CARTESIAN_POINT('Ctrl Pts',(-0.427616409036058,48.2689332824309,
20.));
#92919=CARTESIAN_POINT('Ctrl Pts',(-0.394153058142925,48.2661919195348,
0.));
#92920=CARTESIAN_POINT('Ctrl Pts',(-0.394153058142925,48.2661919195348,
20.));
#92921=CARTESIAN_POINT('Ctrl Pts',(-0.360692727322003,48.2634274670053,
0.));
#92922=CARTESIAN_POINT('Ctrl Pts',(-0.360692727322003,48.2634274670053,
20.));
#92923=CARTESIAN_POINT('Ctrl Pts',(-0.327235432560555,48.2606399270286,
0.));
#92924=CARTESIAN_POINT('Ctrl Pts',(-0.327235432560555,48.2606399270286,
20.));
#92925=CARTESIAN_POINT('Ctrl Pts',(-0.293781189844835,48.2578293018028,
0.));
#92926=CARTESIAN_POINT('Ctrl Pts',(-0.293781189844835,48.2578293018028,
20.));
#92927=CARTESIAN_POINT('Ctrl Pts',(-0.260330015159953,48.2549955935366,
0.));
#92928=CARTESIAN_POINT('Ctrl Pts',(-0.260330015159953,48.2549955935366,
20.));
#92929=CARTESIAN_POINT('Ctrl Pts',(-0.22688192448987,48.2521388044499,0.));
#92930=CARTESIAN_POINT('Ctrl Pts',(-0.22688192448987,48.2521388044499,20.));
#92931=CARTESIAN_POINT('Ctrl Pts',(-0.193436933817472,48.2492589367737,
0.));
#92932=CARTESIAN_POINT('Ctrl Pts',(-0.193436933817472,48.2492589367737,
20.));
#92933=CARTESIAN_POINT('Ctrl Pts',(-0.159995059124576,48.2463559927498,
0.));
#92934=CARTESIAN_POINT('Ctrl Pts',(-0.159995059124576,48.2463559927498,
20.));
#92935=CARTESIAN_POINT('Ctrl Pts',(-0.126556316391682,48.2434299746318,
0.));
#92936=CARTESIAN_POINT('Ctrl Pts',(-0.126556316391682,48.2434299746318,
20.));
#92937=CARTESIAN_POINT('Ctrl Pts',(-0.0931207215982832,48.2404808846839,
0.));
#92938=CARTESIAN_POINT('Ctrl Pts',(-0.0931207215982832,48.2404808846839,
20.));
#92939=CARTESIAN_POINT('Ctrl Pts',(-0.0596882907225993,48.2375087251817,
0.));
#92940=CARTESIAN_POINT('Ctrl Pts',(-0.0596882907225993,48.2375087251817,
20.));
#92941=CARTESIAN_POINT('Ctrl Pts',(-0.0262590397416762,48.234513498412,
0.));
#92942=CARTESIAN_POINT('Ctrl Pts',(-0.0262590397416762,48.234513498412,
20.));
#92943=CARTESIAN_POINT('Ctrl Pts',(0.00716701536856768,48.2314952066725,
0.));
#92944=CARTESIAN_POINT('Ctrl Pts',(0.00716701536856768,48.2314952066725,
20.));
#92945=CARTESIAN_POINT('Ctrl Pts',(0.0405898586334352,48.2284538522724,
0.));
#92946=CARTESIAN_POINT('Ctrl Pts',(0.0405898586334352,48.2284538522724,
20.));
#92947=CARTESIAN_POINT('Ctrl Pts',(0.0740094740793884,48.2253894375317,
0.));
#92948=CARTESIAN_POINT('Ctrl Pts',(0.0740094740793884,48.2253894375317,
20.));
#92949=CARTESIAN_POINT('Ctrl Pts',(0.107425845734119,48.2223019647818,0.));
#92950=CARTESIAN_POINT('Ctrl Pts',(0.107425845734119,48.2223019647818,20.));
#92951=CARTESIAN_POINT('Ctrl Pts',(0.140838957626541,48.2191914363652,0.));
#92952=CARTESIAN_POINT('Ctrl Pts',(0.140838957626541,48.2191914363652,20.));
#92953=CARTESIAN_POINT('Ctrl Pts',(0.174248793786895,48.2160578546352,0.));
#92954=CARTESIAN_POINT('Ctrl Pts',(0.174248793786895,48.2160578546352,20.));
#92955=CARTESIAN_POINT('Ctrl Pts',(0.207655338246555,48.2129012219564,0.));
#92956=CARTESIAN_POINT('Ctrl Pts',(0.207655338246555,48.2129012219564,20.));
#92957=CARTESIAN_POINT('Ctrl Pts',(0.241058575037867,48.2097215407045,0.));
#92958=CARTESIAN_POINT('Ctrl Pts',(0.241058575037867,48.2097215407045,20.));
#92959=CARTESIAN_POINT('Ctrl Pts',(0.274458488194584,48.2065188132665,0.));
#92960=CARTESIAN_POINT('Ctrl Pts',(0.274458488194584,48.2065188132665,20.));
#92961=CARTESIAN_POINT('Ctrl Pts',(0.30785506175171,48.2032930420408,0.));
#92962=CARTESIAN_POINT('Ctrl Pts',(0.30785506175171,48.2032930420408,20.));
#92963=CARTESIAN_POINT('Ctrl Pts',(0.341248279745643,48.2000442294364,0.));
#92964=CARTESIAN_POINT('Ctrl Pts',(0.341248279745643,48.2000442294364,20.));
#92965=CARTESIAN_POINT('Ctrl Pts',(0.374638126214095,48.1967723778737,0.));
#92966=CARTESIAN_POINT('Ctrl Pts',(0.374638126214095,48.1967723778737,20.));
#92967=CARTESIAN_POINT('Ctrl Pts',(0.408024585196225,48.1934774897842,0.));
#92968=CARTESIAN_POINT('Ctrl Pts',(0.408024585196225,48.1934774897842,20.));
#92969=CARTESIAN_POINT('Ctrl Pts',(0.441407640732092,48.1901595676102,0.));
#92970=CARTESIAN_POINT('Ctrl Pts',(0.441407640732092,48.1901595676102,20.));
#92971=CARTESIAN_POINT('Ctrl Pts',(0.474787276863071,48.1868186138054,0.));
#92972=CARTESIAN_POINT('Ctrl Pts',(0.474787276863071,48.1868186138054,20.));
#92973=CARTESIAN_POINT('Ctrl Pts',(0.508163477631851,48.1834546308352,0.));
#92974=CARTESIAN_POINT('Ctrl Pts',(0.508163477631851,48.1834546308352,20.));
#92975=CARTESIAN_POINT('Ctrl Pts',(0.541536227082355,48.1800676211754,0.));
#92976=CARTESIAN_POINT('Ctrl Pts',(0.541536227082355,48.1800676211754,20.));
#92977=CARTESIAN_POINT('Ctrl Pts',(0.574905509259889,48.1766575873132,0.));
#92978=CARTESIAN_POINT('Ctrl Pts',(0.574905509259889,48.1766575873132,20.));
#92979=CARTESIAN_POINT('Ctrl Pts',(0.608271308211097,48.1732245317468,0.));
#92980=CARTESIAN_POINT('Ctrl Pts',(0.608271308211097,48.1732245317468,20.));
#92981=CARTESIAN_POINT('Ctrl Pts',(0.6416336079841,48.1697684569855,0.));
#92982=CARTESIAN_POINT('Ctrl Pts',(0.6416336079841,48.1697684569855,20.));
#92983=CARTESIAN_POINT('Ctrl Pts',(0.674992392628235,48.16628936555,0.));
#92984=CARTESIAN_POINT('Ctrl Pts',(0.674992392628235,48.16628936555,20.));
#92985=CARTESIAN_POINT('Ctrl Pts',(0.708347646194278,48.1627872599717,0.));
#92986=CARTESIAN_POINT('Ctrl Pts',(0.708347646194278,48.1627872599717,20.));
#92987=CARTESIAN_POINT('Ctrl Pts',(0.741699352734257,48.1592621427937,0.));
#92988=CARTESIAN_POINT('Ctrl Pts',(0.741699352734257,48.1592621427937,20.));
#92989=CARTESIAN_POINT('Ctrl Pts',(0.775047496301533,48.1557140165701,0.));
#92990=CARTESIAN_POINT('Ctrl Pts',(0.775047496301533,48.1557140165701,20.));
#92991=CARTESIAN_POINT('Ctrl Pts',(0.808392060950864,48.1521428838659,0.));
#92992=CARTESIAN_POINT('Ctrl Pts',(0.808392060950864,48.1521428838659,20.));
#92993=CARTESIAN_POINT('Ctrl Pts',(0.841733030738387,48.1485487472572,0.));
#92994=CARTESIAN_POINT('Ctrl Pts',(0.841733030738387,48.1485487472572,20.));
#92995=CARTESIAN_POINT('Ctrl Pts',(0.875070389721522,48.144931609331,0.));
#92996=CARTESIAN_POINT('Ctrl Pts',(0.875070389721522,48.144931609331,20.));
#92997=CARTESIAN_POINT('Ctrl Pts',(0.908404121959285,48.1412914726861,0.));
#92998=CARTESIAN_POINT('Ctrl Pts',(0.908404121959285,48.1412914726861,20.));
#92999=CARTESIAN_POINT('Ctrl Pts',(0.941734211511944,48.137628339932,0.));
#93000=CARTESIAN_POINT('Ctrl Pts',(0.941734211511944,48.137628339932,20.));
#93001=CARTESIAN_POINT('Ctrl Pts',(0.975060642441243,48.1339422136897,0.));
#93002=CARTESIAN_POINT('Ctrl Pts',(0.975060642441243,48.1339422136897,20.));
#93003=CARTESIAN_POINT('Ctrl Pts',(1.00838339881032,48.130233096591,0.));
#93004=CARTESIAN_POINT('Ctrl Pts',(1.00838339881032,48.130233096591,20.));
#93005=CARTESIAN_POINT('Ctrl Pts',(1.04170246468365,48.1265009912787,0.));
#93006=CARTESIAN_POINT('Ctrl Pts',(1.04170246468365,48.1265009912787,20.));
#93007=CARTESIAN_POINT('Ctrl Pts',(1.07501782412728,48.1227459004068,0.));
#93008=CARTESIAN_POINT('Ctrl Pts',(1.07501782412728,48.1227459004068,20.));
#93009=CARTESIAN_POINT('Ctrl Pts',(1.10832946120861,48.1189678266406,0.));
#93010=CARTESIAN_POINT('Ctrl Pts',(1.10832946120861,48.1189678266406,20.));
#93011=CARTESIAN_POINT('Ctrl Pts',(1.14163735999657,48.1151667726565,0.));
#93012=CARTESIAN_POINT('Ctrl Pts',(1.14163735999657,48.1151667726565,20.));
#93013=CARTESIAN_POINT('Ctrl Pts',(1.17494150456145,48.111342741142,0.));
#93014=CARTESIAN_POINT('Ctrl Pts',(1.17494150456145,48.111342741142,20.));
#93015=CARTESIAN_POINT('Ctrl Pts',(1.20824187897489,48.1074957347955,0.));
#93016=CARTESIAN_POINT('Ctrl Pts',(1.20824187897489,48.1074957347955,20.));
#93017=CARTESIAN_POINT('Ctrl Pts',(1.24153846731022,48.1036257563271,0.));
#93018=CARTESIAN_POINT('Ctrl Pts',(1.24153846731022,48.1036257563271,20.));
#93019=CARTESIAN_POINT('Ctrl Pts',(1.27483125364215,48.0997328084577,0.));
#93020=CARTESIAN_POINT('Ctrl Pts',(1.27483125364215,48.0997328084577,20.));
#93021=CARTESIAN_POINT('Ctrl Pts',(1.30812022204704,48.0958168939195,0.));
#93022=CARTESIAN_POINT('Ctrl Pts',(1.30812022204704,48.0958168939195,20.));
#93023=CARTESIAN_POINT('Ctrl Pts',(1.3414053566026,48.0918780154556,0.));
#93024=CARTESIAN_POINT('Ctrl Pts',(1.3414053566026,48.0918780154556,20.));
#93025=CARTESIAN_POINT('Ctrl Pts',(1.37468664138801,48.0879161758201,0.));
#93026=CARTESIAN_POINT('Ctrl Pts',(1.37468664138801,48.0879161758201,20.));
#93027=CARTESIAN_POINT('Ctrl Pts',(1.40796406048387,48.0839313777781,0.));
#93028=CARTESIAN_POINT('Ctrl Pts',(1.40796406048387,48.0839313777781,20.));
#93029=CARTESIAN_POINT('Ctrl Pts',(1.44123759797224,48.0799236241059,0.));
#93030=CARTESIAN_POINT('Ctrl Pts',(1.44123759797224,48.0799236241059,20.));
#93031=CARTESIAN_POINT('Ctrl Pts',(1.47450723793681,48.0758929175908,0.));
#93032=CARTESIAN_POINT('Ctrl Pts',(1.47450723793681,48.0758929175908,20.));
#93033=CARTESIAN_POINT('Ctrl Pts',(1.50777296446291,48.071839261032,0.));
#93034=CARTESIAN_POINT('Ctrl Pts',(1.50777296446291,48.071839261032,20.));
#93035=CARTESIAN_POINT('Ctrl Pts',(1.54103476163743,48.0677626572394,0.));
#93036=CARTESIAN_POINT('Ctrl Pts',(1.54103476163743,48.0677626572394,20.));
#93037=CARTESIAN_POINT('Ctrl Pts',(1.57429261354889,48.0636631090342,0.));
#93038=CARTESIAN_POINT('Ctrl Pts',(1.57429261354889,48.0636631090342,20.));
#93039=CARTESIAN_POINT('Ctrl Pts',(1.60754650428745,48.0595406192492,0.));
#93040=CARTESIAN_POINT('Ctrl Pts',(1.60754650428745,48.0595406192492,20.));
#93041=CARTESIAN_POINT('Ctrl Pts',(1.64079641794461,48.0553951907273,0.));
#93042=CARTESIAN_POINT('Ctrl Pts',(1.64079641794461,48.0553951907273,20.));
#93043=CARTESIAN_POINT('Ctrl Pts',(1.67404233861337,48.0512268263229,0.));
#93044=CARTESIAN_POINT('Ctrl Pts',(1.67404233861337,48.0512268263229,20.));
#93045=CARTESIAN_POINT('Ctrl Pts',(1.70728425038804,48.0470355289011,0.));
#93046=CARTESIAN_POINT('Ctrl Pts',(1.70728425038804,48.0470355289011,20.));
#93047=CARTESIAN_POINT('Ctrl Pts',(1.74052213736471,48.0428213013379,0.));
#93048=CARTESIAN_POINT('Ctrl Pts',(1.74052213736471,48.0428213013379,20.));
#93049=CARTESIAN_POINT('Ctrl Pts',(1.77375598364109,48.038584146521,0.));
#93050=CARTESIAN_POINT('Ctrl Pts',(1.77375598364109,48.038584146521,20.));
#93051=CARTESIAN_POINT('Ctrl Pts',(1.80698577331663,48.0343240673492,0.));
#93052=CARTESIAN_POINT('Ctrl Pts',(1.80698577331663,48.0343240673492,20.));
#93053=CARTESIAN_POINT('Ctrl Pts',(1.84021149049245,48.0300410667328,0.));
#93054=CARTESIAN_POINT('Ctrl Pts',(1.84021149049245,48.0300410667328,20.));
#93055=CARTESIAN_POINT('Ctrl Pts',(1.87343311927141,48.0257351475934,0.));
#93056=CARTESIAN_POINT('Ctrl Pts',(1.87343311927141,48.0257351475934,20.));
#93057=CARTESIAN_POINT('Ctrl Pts',(1.90665064375786,48.0214063128629,0.));
#93058=CARTESIAN_POINT('Ctrl Pts',(1.90665064375786,48.0214063128629,20.));
#93059=CARTESIAN_POINT('Ctrl Pts',(1.93986404805772,48.0170545654849,0.));
#93060=CARTESIAN_POINT('Ctrl Pts',(1.93986404805772,48.0170545654849,20.));
#93061=CARTESIAN_POINT('Ctrl Pts',(1.97307331627849,48.0126799084137,0.));
#93062=CARTESIAN_POINT('Ctrl Pts',(1.97307331627849,48.0126799084137,20.));
#93063=CARTESIAN_POINT('Ctrl Pts',(2.00627843252925,48.0082823446147,0.));
#93064=CARTESIAN_POINT('Ctrl Pts',(2.00627843252925,48.0082823446147,20.));
#93065=CARTESIAN_POINT('Ctrl Pts',(2.03947938092067,48.0038618770642,0.));
#93066=CARTESIAN_POINT('Ctrl Pts',(2.03947938092067,48.0038618770642,20.));
#93067=CARTESIAN_POINT('Ctrl Pts',(2.07267614556536,47.9994185087499,0.));
#93068=CARTESIAN_POINT('Ctrl Pts',(2.07267614556536,47.9994185087499,20.));
#93069=CARTESIAN_POINT('Ctrl Pts',(2.10586871057748,47.994952242671,0.));
#93070=CARTESIAN_POINT('Ctrl Pts',(2.10586871057748,47.994952242671,20.));
#93071=CARTESIAN_POINT('Ctrl Pts',(2.13905706007285,47.9904630818375,0.));
#93072=CARTESIAN_POINT('Ctrl Pts',(2.13905706007285,47.9904630818375,20.));
#93073=CARTESIAN_POINT('Ctrl Pts',(2.17224117816898,47.9859510292704,0.));
#93074=CARTESIAN_POINT('Ctrl Pts',(2.17224117816898,47.9859510292704,20.));
#93075=CARTESIAN_POINT('Ctrl Pts',(2.2054210489852,47.9814160880019,0.));
#93076=CARTESIAN_POINT('Ctrl Pts',(2.2054210489852,47.9814160880019,20.));
#93077=CARTESIAN_POINT('Ctrl Pts',(2.23859665664239,47.9768582610752,0.));
#93078=CARTESIAN_POINT('Ctrl Pts',(2.23859665664239,47.9768582610752,20.));
#93079=CARTESIAN_POINT('Ctrl Pts',(2.27176798526352,47.9722775515452,0.));
#93080=CARTESIAN_POINT('Ctrl Pts',(2.27176798526352,47.9722775515452,20.));
#93081=CARTESIAN_POINT('Ctrl Pts',(2.30493501897294,47.9676739624772,0.));
#93082=CARTESIAN_POINT('Ctrl Pts',(2.30493501897294,47.9676739624772,20.));
#93083=CARTESIAN_POINT('Ctrl Pts',(2.33809774189657,47.9630474969481,0.));
#93084=CARTESIAN_POINT('Ctrl Pts',(2.33809774189657,47.9630474969481,20.));
#93085=CARTESIAN_POINT('Ctrl Pts',(2.3712561381623,47.9583981580454,0.));
#93086=CARTESIAN_POINT('Ctrl Pts',(2.3712561381623,47.9583981580454,20.));
#93087=CARTESIAN_POINT('Ctrl Pts',(2.40441019189959,47.9537259488681,0.));
#93088=CARTESIAN_POINT('Ctrl Pts',(2.40441019189959,47.9537259488681,20.));
#93089=CARTESIAN_POINT('Ctrl Pts',(2.43755988723965,47.9490308725257,0.));
#93090=CARTESIAN_POINT('Ctrl Pts',(2.43755988723965,47.9490308725257,20.));
#93091=CARTESIAN_POINT('Ctrl Pts',(2.47070520831548,47.9443129321394,0.));
#93092=CARTESIAN_POINT('Ctrl Pts',(2.47070520831548,47.9443129321394,20.));
#93093=CARTESIAN_POINT('Ctrl Pts',(2.50384613926209,47.9395721308414,0.));
#93094=CARTESIAN_POINT('Ctrl Pts',(2.50384613926209,47.9395721308414,20.));
#93095=CARTESIAN_POINT('Ctrl Pts',(2.53698266421613,47.9348084717752,0.));
#93096=CARTESIAN_POINT('Ctrl Pts',(2.53698266421613,47.9348084717752,20.));
#93097=CARTESIAN_POINT('Ctrl Pts',(2.57011476731622,47.9300219580955,0.));
#93098=CARTESIAN_POINT('Ctrl Pts',(2.57011476731622,47.9300219580955,20.));
#93099=CARTESIAN_POINT('Ctrl Pts',(2.60324243270257,47.9252125929679,0.));
#93100=CARTESIAN_POINT('Ctrl Pts',(2.60324243270257,47.9252125929679,20.));
#93101=CARTESIAN_POINT('Ctrl Pts',(2.63636564451718,47.9203803795688,0.));
#93102=CARTESIAN_POINT('Ctrl Pts',(2.63636564451718,47.9203803795688,20.));
#93103=CARTESIAN_POINT('Ctrl Pts',(2.66948438690365,47.9155253210858,0.));
#93104=CARTESIAN_POINT('Ctrl Pts',(2.66948438690365,47.9155253210858,20.));
#93105=CARTESIAN_POINT('Ctrl Pts',(2.70259864400757,47.9106474207177,0.));
#93106=CARTESIAN_POINT('Ctrl Pts',(2.70259864400757,47.9106474207177,20.));
#93107=CARTESIAN_POINT('Ctrl Pts',(2.73570839997628,47.9057466816743,0.));
#93108=CARTESIAN_POINT('Ctrl Pts',(2.73570839997628,47.9057466816743,20.));
#93109=CARTESIAN_POINT('Ctrl Pts',(2.76881363895917,47.9008231071768,0.));
#93110=CARTESIAN_POINT('Ctrl Pts',(2.76881363895917,47.9008231071768,20.));
#93111=CARTESIAN_POINT('Ctrl Pts',(2.80191434510733,47.8958767004573,0.));
#93112=CARTESIAN_POINT('Ctrl Pts',(2.80191434510733,47.8958767004573,20.));
#93113=CARTESIAN_POINT('Ctrl Pts',(2.83501050257375,47.8909074647592,0.));
#93114=CARTESIAN_POINT('Ctrl Pts',(2.83501050257375,47.8909074647592,20.));
#93115=CARTESIAN_POINT('Ctrl Pts',(2.86810209551307,47.8859154033363,0.));
#93116=CARTESIAN_POINT('Ctrl Pts',(2.86810209551307,47.8859154033363,20.));
#93117=CARTESIAN_POINT('Ctrl Pts',(2.90118910808199,47.8809005194543,0.));
#93118=CARTESIAN_POINT('Ctrl Pts',(2.90118910808199,47.8809005194543,20.));
#93119=CARTESIAN_POINT('Ctrl Pts',(2.93427152443917,47.8758628163901,0.));
#93120=CARTESIAN_POINT('Ctrl Pts',(2.93427152443917,47.8758628163901,20.));
#93121=CARTESIAN_POINT('Ctrl Pts',(2.96734932874504,47.8708022974315,0.));
#93122=CARTESIAN_POINT('Ctrl Pts',(2.96734932874504,47.8708022974315,20.));
#93123=CARTESIAN_POINT('Ctrl Pts',(3.00042250516192,47.8657189658771,0.));
#93124=CARTESIAN_POINT('Ctrl Pts',(3.00042250516192,47.8657189658771,20.));
#93125=CARTESIAN_POINT('Ctrl Pts',(3.03349103785388,47.8606128250365,0.));
#93126=CARTESIAN_POINT('Ctrl Pts',(3.03349103785388,47.8606128250365,20.));
#93127=CARTESIAN_POINT('Ctrl Pts',(3.06655491098681,47.8554838782302,0.));
#93128=CARTESIAN_POINT('Ctrl Pts',(3.06655491098681,47.8554838782302,20.));
#93129=CARTESIAN_POINT('Ctrl Pts',(3.09961410872875,47.8503321287903,0.));
#93130=CARTESIAN_POINT('Ctrl Pts',(3.09961410872875,47.8503321287903,20.));
#93131=CARTESIAN_POINT('Ctrl Pts',(3.13266861524953,47.8451575800601,0.));
#93132=CARTESIAN_POINT('Ctrl Pts',(3.13266861524953,47.8451575800601,20.));
#93133=CARTESIAN_POINT('Ctrl Pts',(3.16571841472089,47.8399602353939,0.));
#93134=CARTESIAN_POINT('Ctrl Pts',(3.16571841472089,47.8399602353939,20.));
#93135=CARTESIAN_POINT('Ctrl Pts',(3.19876349131674,47.834740098157,0.));
#93136=CARTESIAN_POINT('Ctrl Pts',(3.19876349131674,47.834740098157,20.));
#93137=CARTESIAN_POINT('Ctrl Pts',(3.23180382921272,47.829497171726,0.));
#93138=CARTESIAN_POINT('Ctrl Pts',(3.23180382921272,47.829497171726,20.));
#93139=CARTESIAN_POINT('Ctrl Pts',(3.26483941258676,47.8242314594881,0.));
#93140=CARTESIAN_POINT('Ctrl Pts',(3.26483941258676,47.8242314594881,20.));
#93141=CARTESIAN_POINT('Ctrl Pts',(3.29787022561835,47.818942964842,0.));
#93142=CARTESIAN_POINT('Ctrl Pts',(3.29787022561835,47.818942964842,20.));
#93143=CARTESIAN_POINT('Ctrl Pts',(3.33089625248902,47.813631691197,0.));
#93144=CARTESIAN_POINT('Ctrl Pts',(3.33089625248902,47.813631691197,20.));
#93145=CARTESIAN_POINT('Ctrl Pts',(3.36391747738213,47.8082976419741,0.));
#93146=CARTESIAN_POINT('Ctrl Pts',(3.36391747738213,47.8082976419741,20.));
#93147=CARTESIAN_POINT('Ctrl Pts',(3.39693388448305,47.802940820605,0.));
#93148=CARTESIAN_POINT('Ctrl Pts',(3.39693388448305,47.802940820605,20.));
#93149=CARTESIAN_POINT('Ctrl Pts',(3.42994545797921,47.797561230533,0.));
#93150=CARTESIAN_POINT('Ctrl Pts',(3.42994545797921,47.797561230533,20.));
#93151=CARTESIAN_POINT('Ctrl Pts',(3.46295218206011,47.7921588752121,0.));
#93152=CARTESIAN_POINT('Ctrl Pts',(3.46295218206011,47.7921588752121,20.));
#93153=CARTESIAN_POINT('Ctrl Pts',(3.49595404091727,47.7867337581073,0.));
#93154=CARTESIAN_POINT('Ctrl Pts',(3.49595404091727,47.7867337581073,20.));
#93155=CARTESIAN_POINT('Ctrl Pts',(3.52895101874414,47.7812858826946,0.));
#93156=CARTESIAN_POINT('Ctrl Pts',(3.52895101874414,47.7812858826946,20.));
#93157=CARTESIAN_POINT('Ctrl Pts',(3.56194309973641,47.7758152524613,0.));
#93158=CARTESIAN_POINT('Ctrl Pts',(3.56194309973641,47.7758152524613,20.));
#93159=CARTESIAN_POINT('Ctrl Pts',(3.59493026809157,47.7703218709055,0.));
#93160=CARTESIAN_POINT('Ctrl Pts',(3.59493026809157,47.7703218709055,20.));
#93161=CARTESIAN_POINT('Ctrl Pts',(3.62791250800923,47.764805741537,0.));
#93162=CARTESIAN_POINT('Ctrl Pts',(3.62791250800923,47.764805741537,20.));
#93163=CARTESIAN_POINT('Ctrl Pts',(3.66088980369083,47.7592668678762,0.));
#93164=CARTESIAN_POINT('Ctrl Pts',(3.66088980369083,47.7592668678762,20.));
#93165=CARTESIAN_POINT('Ctrl Pts',(3.69386213933993,47.7537052534546,0.));
#93166=CARTESIAN_POINT('Ctrl Pts',(3.69386213933993,47.7537052534546,20.));
#93167=CARTESIAN_POINT('Ctrl Pts',(3.72682949916222,47.7481209018149,0.));
#93168=CARTESIAN_POINT('Ctrl Pts',(3.72682949916222,47.7481209018149,20.));
#93169=CARTESIAN_POINT('Ctrl Pts',(3.75979186736544,47.7425138165111,0.));
#93170=CARTESIAN_POINT('Ctrl Pts',(3.75979186736544,47.7425138165111,20.));
#93171=CARTESIAN_POINT('Ctrl Pts',(3.79274922815948,47.7368840011081,0.));
#93172=CARTESIAN_POINT('Ctrl Pts',(3.79274922815948,47.7368840011081,20.));
#93173=CARTESIAN_POINT('Ctrl Pts',(3.82570156575622,47.7312314591817,0.));
#93174=CARTESIAN_POINT('Ctrl Pts',(3.82570156575622,47.7312314591817,20.));
#93175=CARTESIAN_POINT('Ctrl Pts',(3.85864886436973,47.7255561943191,0.));
#93176=CARTESIAN_POINT('Ctrl Pts',(3.85864886436973,47.7255561943191,20.));
#93177=CARTESIAN_POINT('Ctrl Pts',(3.89159110821604,47.719858210118,0.));
#93178=CARTESIAN_POINT('Ctrl Pts',(3.89159110821604,47.719858210118,20.));
#93179=CARTESIAN_POINT('Ctrl Pts',(3.92452828151332,47.7141375101875,0.));
#93180=CARTESIAN_POINT('Ctrl Pts',(3.92452828151332,47.7141375101875,20.));
#93181=CARTESIAN_POINT('Ctrl Pts',(3.95746036848186,47.7083940981477,0.));
#93182=CARTESIAN_POINT('Ctrl Pts',(3.95746036848186,47.7083940981477,20.));
#93183=CARTESIAN_POINT('Ctrl Pts',(3.990387353344,47.7026279776294,0.));
#93184=CARTESIAN_POINT('Ctrl Pts',(3.990387353344,47.7026279776294,20.));
#93185=CARTESIAN_POINT('Ctrl Pts',(4.02330922032433,47.6968391522753,0.));
#93186=CARTESIAN_POINT('Ctrl Pts',(4.02330922032433,47.6968391522753,20.));
#93187=CARTESIAN_POINT('Ctrl Pts',(4.05622595364951,47.6910276257391,0.));
#93188=CARTESIAN_POINT('Ctrl Pts',(4.05622595364951,47.6910276257391,20.));
#93189=CARTESIAN_POINT('Ctrl Pts',(4.08913753754848,47.6851934016861,0.));
#93190=CARTESIAN_POINT('Ctrl Pts',(4.08913753754848,47.6851934016861,20.));
#93191=CARTESIAN_POINT('Ctrl Pts',(4.12204395625218,47.6793364837921,0.));
#93192=CARTESIAN_POINT('Ctrl Pts',(4.12204395625218,47.6793364837921,20.));
#93193=CARTESIAN_POINT('Ctrl Pts',(4.15494519399369,47.6734568757434,0.));
#93194=CARTESIAN_POINT('Ctrl Pts',(4.15494519399369,47.6734568757434,20.));
#93195=CARTESIAN_POINT('Ctrl Pts',(4.18784123500835,47.6675545812371,0.));
#93196=CARTESIAN_POINT('Ctrl Pts',(4.18784123500835,47.6675545812371,20.));
#93197=CARTESIAN_POINT('Ctrl Pts',(4.22073206353344,47.6616296039816,0.));
#93198=CARTESIAN_POINT('Ctrl Pts',(4.22073206353344,47.6616296039816,20.));
#93199=CARTESIAN_POINT('Ctrl Pts',(4.25361766380859,47.6556819476964,0.));
#93200=CARTESIAN_POINT('Ctrl Pts',(4.25361766380859,47.6556819476964,20.));
#93201=CARTESIAN_POINT('Ctrl Pts',(4.28649802007566,47.6497116161128,0.));
#93202=CARTESIAN_POINT('Ctrl Pts',(4.28649802007566,47.6497116161128,20.));
#93203=CARTESIAN_POINT('Ctrl Pts',(4.31937311657885,47.6437186129734,0.));
#93204=CARTESIAN_POINT('Ctrl Pts',(4.31937311657885,47.6437186129734,20.));
#93205=CARTESIAN_POINT('Ctrl Pts',(4.35224293756439,47.6377029420315,0.));
#93206=CARTESIAN_POINT('Ctrl Pts',(4.35224293756439,47.6377029420315,20.));
#93207=CARTESIAN_POINT('Ctrl Pts',(4.38510746728074,47.6316646070511,0.));
#93208=CARTESIAN_POINT('Ctrl Pts',(4.38510746728074,47.6316646070511,20.));
#93209=CARTESIAN_POINT('Ctrl Pts',(4.41796668997835,47.6256036118071,0.));
#93210=CARTESIAN_POINT('Ctrl Pts',(4.41796668997835,47.6256036118071,20.));
#93211=CARTESIAN_POINT('Ctrl Pts',(4.45082058991003,47.6195199600851,0.));
#93212=CARTESIAN_POINT('Ctrl Pts',(4.45082058991003,47.6195199600851,20.));
#93213=CARTESIAN_POINT('Ctrl Pts',(4.48366915133083,47.6134136556823,0.));
#93214=CARTESIAN_POINT('Ctrl Pts',(4.48366915133083,47.6134136556823,20.));
#93215=CARTESIAN_POINT('Ctrl Pts',(4.51651235849822,47.6072847024073,0.));
#93216=CARTESIAN_POINT('Ctrl Pts',(4.51651235849822,47.6072847024073,20.));
#93217=CARTESIAN_POINT('Ctrl Pts',(4.54935019567197,47.6011331040799,0.));
#93218=CARTESIAN_POINT('Ctrl Pts',(4.54935019567197,47.6011331040799,20.));
#93219=CARTESIAN_POINT('Ctrl Pts',(4.58218264711418,47.5949588645311,0.));
#93220=CARTESIAN_POINT('Ctrl Pts',(4.58218264711418,47.5949588645311,20.));
#93221=CARTESIAN_POINT('Ctrl Pts',(4.61500969708895,47.5887619876026,0.));
#93222=CARTESIAN_POINT('Ctrl Pts',(4.61500969708895,47.5887619876026,20.));
#93223=CARTESIAN_POINT('Ctrl Pts',(4.64783132986259,47.5825424771468,0.));
#93224=CARTESIAN_POINT('Ctrl Pts',(4.64783132986259,47.5825424771468,20.));
#93225=CARTESIAN_POINT('Ctrl Pts',(4.68064752970369,47.5763003370265,0.));
#93226=CARTESIAN_POINT('Ctrl Pts',(4.68064752970369,47.5763003370265,20.));
#93227=CARTESIAN_POINT('Ctrl Pts',(4.71345828088308,47.5700355711162,0.));
#93228=CARTESIAN_POINT('Ctrl Pts',(4.71345828088308,47.5700355711162,20.));
#93229=CARTESIAN_POINT('Ctrl Pts',(4.74626356767412,47.5637481833017,0.));
#93230=CARTESIAN_POINT('Ctrl Pts',(4.74626356767412,47.5637481833017,20.));
#93231=CARTESIAN_POINT('Ctrl Pts',(4.77906337435243,47.5574381774801,0.));
#93232=CARTESIAN_POINT('Ctrl Pts',(4.77906337435243,47.5574381774801,20.));
#93233=CARTESIAN_POINT('Ctrl Pts',(4.81185768519588,47.5511055575593,0.));
#93234=CARTESIAN_POINT('Ctrl Pts',(4.81185768519588,47.5511055575593,20.));
#93235=CARTESIAN_POINT('Ctrl Pts',(4.84464648448474,47.5447503274583,0.));
#93236=CARTESIAN_POINT('Ctrl Pts',(4.84464648448474,47.5447503274583,20.));
#93237=CARTESIAN_POINT('Ctrl Pts',(4.87742975650161,47.538372491107,0.));
#93238=CARTESIAN_POINT('Ctrl Pts',(4.87742975650161,47.538372491107,20.));
#93239=CARTESIAN_POINT('Ctrl Pts',(4.91020748553144,47.5319720524462,0.));
#93240=CARTESIAN_POINT('Ctrl Pts',(4.91020748553144,47.5319720524462,20.));
#93241=CARTESIAN_POINT('Ctrl Pts',(4.94297965586156,47.5255490154281,0.));
#93242=CARTESIAN_POINT('Ctrl Pts',(4.94297965586156,47.5255490154281,20.));
#93243=CARTESIAN_POINT('Ctrl Pts',(4.97574625178169,47.519103384016,0.));
#93244=CARTESIAN_POINT('Ctrl Pts',(4.97574625178169,47.519103384016,20.));
#93245=CARTESIAN_POINT('Ctrl Pts',(5.00850725758367,47.5126351621839,0.));
#93246=CARTESIAN_POINT('Ctrl Pts',(5.00850725758367,47.5126351621839,20.));
#93247=CARTESIAN_POINT('Ctrl Pts',(5.04126265756154,47.5061443539168,0.));
#93248=CARTESIAN_POINT('Ctrl Pts',(5.04126265756154,47.5061443539168,20.));
#93249=CARTESIAN_POINT('Ctrl Pts',(5.07401243601198,47.4996309632108,0.));
#93250=CARTESIAN_POINT('Ctrl Pts',(5.07401243601198,47.4996309632108,20.));
#93251=CARTESIAN_POINT('Ctrl Pts',(5.10675657723402,47.4930949940731,0.));
#93252=CARTESIAN_POINT('Ctrl Pts',(5.10675657723402,47.4930949940731,20.));
#93253=CARTESIAN_POINT('Ctrl Pts',(5.13949506552922,47.4865364505219,0.));
#93254=CARTESIAN_POINT('Ctrl Pts',(5.13949506552922,47.4865364505219,20.));
#93255=CARTESIAN_POINT('Ctrl Pts',(5.17222788520144,47.4799553365862,0.));
#93256=CARTESIAN_POINT('Ctrl Pts',(5.17222788520144,47.4799553365862,20.));
#93257=CARTESIAN_POINT('Ctrl Pts',(5.20495502055713,47.4733516563069,0.));
#93258=CARTESIAN_POINT('Ctrl Pts',(5.20495502055713,47.4733516563069,20.));
#93259=CARTESIAN_POINT('Ctrl Pts',(5.2376764559051,47.4667254137359,0.));
#93260=CARTESIAN_POINT('Ctrl Pts',(5.2376764559051,47.4667254137359,20.));
#93261=CARTESIAN_POINT('Ctrl Pts',(5.27039217555655,47.4600766129357,0.));
#93262=CARTESIAN_POINT('Ctrl Pts',(5.27039217555655,47.4600766129357,20.));
#93263=CARTESIAN_POINT('Ctrl Pts',(5.30310216382505,47.4534052579797,0.));
#93264=CARTESIAN_POINT('Ctrl Pts',(5.30310216382505,47.4534052579797,20.));
#93265=CARTESIAN_POINT('Ctrl Pts',(5.3358064050266,47.4467113529523,0.));
#93266=CARTESIAN_POINT('Ctrl Pts',(5.3358064050266,47.4467113529523,20.));
#93267=CARTESIAN_POINT('Ctrl Pts',(5.36850488347923,47.4399949019487,0.));
#93268=CARTESIAN_POINT('Ctrl Pts',(5.36850488347923,47.4399949019487,20.));
#93269=CARTESIAN_POINT('Ctrl Pts',(5.40119758350378,47.4332559090748,0.));
#93270=CARTESIAN_POINT('Ctrl Pts',(5.40119758350378,47.4332559090748,20.));
#93271=CARTESIAN_POINT('Ctrl Pts',(5.43388448942349,47.4264943784481,0.));
#93272=CARTESIAN_POINT('Ctrl Pts',(5.43388448942349,47.4264943784481,20.));
#93273=CARTESIAN_POINT('Ctrl Pts',(5.46656558556425,47.4197103141976,0.));
#93274=CARTESIAN_POINT('Ctrl Pts',(5.46656558556425,47.4197103141976,20.));
#93275=CARTESIAN_POINT('Ctrl Pts',(5.49924085625463,47.4129037204631,0.));
#93276=CARTESIAN_POINT('Ctrl Pts',(5.49924085625463,47.4129037204631,20.));
#93277=CARTESIAN_POINT('Ctrl Pts',(5.53191028582554,47.4060746013959,0.));
#93278=CARTESIAN_POINT('Ctrl Pts',(5.53191028582554,47.4060746013959,20.));
#93279=CARTESIAN_POINT('Ctrl Pts',(5.56457385861036,47.3992229611579,0.));
#93280=CARTESIAN_POINT('Ctrl Pts',(5.56457385861036,47.3992229611579,20.));
#93281=CARTESIAN_POINT('Ctrl Pts',(5.59723155894482,47.3923488039217,0.));
#93282=CARTESIAN_POINT('Ctrl Pts',(5.59723155894482,47.3923488039217,20.));
#93283=CARTESIAN_POINT('Ctrl Pts',(5.62988337116714,47.3854521338708,0.));
#93284=CARTESIAN_POINT('Ctrl Pts',(5.62988337116714,47.3854521338708,20.));
#93285=CARTESIAN_POINT('Ctrl Pts',(5.6625292796181,47.3785329551997,0.));
#93286=CARTESIAN_POINT('Ctrl Pts',(5.6625292796181,47.3785329551997,20.));
#93287=CARTESIAN_POINT('Ctrl Pts',(5.69516926864087,47.3715912721141,0.));
#93288=CARTESIAN_POINT('Ctrl Pts',(5.69516926864087,47.3715912721141,20.));
#93289=CARTESIAN_POINT('Ctrl Pts',(5.72780332258134,47.3646270888308,0.));
#93290=CARTESIAN_POINT('Ctrl Pts',(5.72780332258134,47.3646270888308,20.));
#93291=CARTESIAN_POINT('Ctrl Pts',(5.76043142578785,47.3576404095778,0.));
#93292=CARTESIAN_POINT('Ctrl Pts',(5.76043142578785,47.3576404095778,20.));
#93293=CARTESIAN_POINT('Ctrl Pts',(5.79305356261141,47.3506312385939,0.));
#93294=CARTESIAN_POINT('Ctrl Pts',(5.79305356261141,47.3506312385939,20.));
#93295=CARTESIAN_POINT('Ctrl Pts',(5.82566971740555,47.3435995801292,0.));
#93296=CARTESIAN_POINT('Ctrl Pts',(5.82566971740555,47.3435995801292,20.));
#93297=CARTESIAN_POINT('Ctrl Pts',(5.85827987452639,47.3365454384446,0.));
#93298=CARTESIAN_POINT('Ctrl Pts',(5.85827987452639,47.3365454384446,20.));
#93299=CARTESIAN_POINT('Ctrl Pts',(5.89088401833276,47.3294688178121,0.));
#93300=CARTESIAN_POINT('Ctrl Pts',(5.89088401833276,47.3294688178121,20.));
#93301=CARTESIAN_POINT('Ctrl Pts',(5.92348213318597,47.3223697225143,0.));
#93302=CARTESIAN_POINT('Ctrl Pts',(5.92348213318597,47.3223697225143,20.));
#93303=CARTESIAN_POINT('Ctrl Pts',(5.95607420344985,47.3152481568452,0.));
#93304=CARTESIAN_POINT('Ctrl Pts',(5.95607420344985,47.3152481568452,20.));
#93305=CARTESIAN_POINT('Ctrl Pts',(5.98866021349066,47.3081041251096,0.));
#93306=CARTESIAN_POINT('Ctrl Pts',(5.98866021349066,47.3081041251096,20.));
#93307=CARTESIAN_POINT('Ctrl Pts',(6.02124014767729,47.3009376316237,0.));
#93308=CARTESIAN_POINT('Ctrl Pts',(6.02124014767729,47.3009376316237,20.));
#93309=CARTESIAN_POINT('Ctrl Pts',(6.05381399038128,47.2937486807145,0.));
#93310=CARTESIAN_POINT('Ctrl Pts',(6.05381399038128,47.2937486807145,20.));
#93311=CARTESIAN_POINT('Ctrl Pts',(6.08638172597683,47.2865372767199,0.));
#93312=CARTESIAN_POINT('Ctrl Pts',(6.08638172597683,47.2865372767199,20.));
#93313=CARTESIAN_POINT('Ctrl Pts',(6.11894333884087,47.2793034239892,0.));
#93314=CARTESIAN_POINT('Ctrl Pts',(6.11894333884087,47.2793034239892,20.));
#93315=CARTESIAN_POINT('Ctrl Pts',(6.15149881335289,47.272047126882,0.));
#93316=CARTESIAN_POINT('Ctrl Pts',(6.15149881335289,47.272047126882,20.));
#93317=CARTESIAN_POINT('Ctrl Pts',(6.18404813389528,47.2647683897693,0.));
#93318=CARTESIAN_POINT('Ctrl Pts',(6.18404813389528,47.2647683897693,20.));
#93319=CARTESIAN_POINT('Ctrl Pts',(6.21659128485295,47.2574672170331,0.));
#93320=CARTESIAN_POINT('Ctrl Pts',(6.21659128485295,47.2574672170331,20.));
#93321=CARTESIAN_POINT('Ctrl Pts',(6.24912825061342,47.2501436130661,0.));
#93322=CARTESIAN_POINT('Ctrl Pts',(6.24912825061342,47.2501436130661,20.));
#93323=CARTESIAN_POINT('Ctrl Pts',(6.28165901556675,47.2427975822723,0.));
#93324=CARTESIAN_POINT('Ctrl Pts',(6.28165901556675,47.2427975822723,20.));
#93325=CARTESIAN_POINT('Ctrl Pts',(6.31418356410549,47.2354291290667,0.));
#93326=CARTESIAN_POINT('Ctrl Pts',(6.31418356410549,47.2354291290667,20.));
#93327=CARTESIAN_POINT('Ctrl Pts',(6.34670188062515,47.2280382578755,0.));
#93328=CARTESIAN_POINT('Ctrl Pts',(6.34670188062515,47.2280382578755,20.));
#93329=CARTESIAN_POINT('Ctrl Pts',(6.37921394952379,47.2206249731358,0.));
#93330=CARTESIAN_POINT('Ctrl Pts',(6.37921394952379,47.2206249731358,20.));
#93331=CARTESIAN_POINT('Ctrl Pts',(6.41171975520233,47.213189279296,0.));
#93332=CARTESIAN_POINT('Ctrl Pts',(6.41171975520233,47.213189279296,20.));
#93333=CARTESIAN_POINT('Ctrl Pts',(6.44421928206445,47.205731180815,0.));
#93334=CARTESIAN_POINT('Ctrl Pts',(6.44421928206445,47.205731180815,20.));
#93335=CARTESIAN_POINT('Ctrl Pts',(6.47671251451637,47.1982506821625,0.));
#93336=CARTESIAN_POINT('Ctrl Pts',(6.47671251451637,47.1982506821625,20.));
#93337=CARTESIAN_POINT('Ctrl Pts',(6.50919943696717,47.190747787819,0.));
#93338=CARTESIAN_POINT('Ctrl Pts',(6.50919943696717,47.190747787819,20.));
#93339=CARTESIAN_POINT('Ctrl Pts',(6.54168003382861,47.1832225022762,0.));
#93340=CARTESIAN_POINT('Ctrl Pts',(6.54168003382861,47.1832225022762,20.));
#93341=CARTESIAN_POINT('Ctrl Pts',(6.57415428951524,47.1756748300372,0.));
#93342=CARTESIAN_POINT('Ctrl Pts',(6.57415428951524,47.1756748300372,20.));
#93343=CARTESIAN_POINT('Ctrl Pts',(6.60662218844434,47.168104775616,0.));
#93344=CARTESIAN_POINT('Ctrl Pts',(6.60662218844434,47.168104775616,20.));
#93345=CARTESIAN_POINT('Ctrl Pts',(6.63908371503577,47.1605123435378,0.));
#93346=CARTESIAN_POINT('Ctrl Pts',(6.63908371503577,47.1605123435378,20.));
#93347=CARTESIAN_POINT('Ctrl Pts',(6.67153885371226,47.1528975383387,0.));
#93348=CARTESIAN_POINT('Ctrl Pts',(6.67153885371226,47.1528975383387,20.));
#93349=CARTESIAN_POINT('Ctrl Pts',(6.70398758889916,47.1452603645656,0.));
#93350=CARTESIAN_POINT('Ctrl Pts',(6.70398758889916,47.1452603645656,20.));
#93351=CARTESIAN_POINT('Ctrl Pts',(6.73642990502458,47.1376008267758,0.));
#93352=CARTESIAN_POINT('Ctrl Pts',(6.73642990502458,47.1376008267758,20.));
#93353=CARTESIAN_POINT('Ctrl Pts',(6.76886578651954,47.129918929538,0.));
#93354=CARTESIAN_POINT('Ctrl Pts',(6.76886578651954,47.129918929538,20.));
#93355=CARTESIAN_POINT('Ctrl Pts',(6.80129521781808,47.1222146774323,0.));
#93356=CARTESIAN_POINT('Ctrl Pts',(6.80129521781808,47.1222146774323,20.));
#93357=CARTESIAN_POINT('Ctrl Pts',(6.83371818335697,47.1144880750497,0.));
#93358=CARTESIAN_POINT('Ctrl Pts',(6.83371818335697,47.1144880750497,20.));
#93359=CARTESIAN_POINT('Ctrl Pts',(6.86613466757588,47.1067391269919,0.));
#93360=CARTESIAN_POINT('Ctrl Pts',(6.86613466757588,47.1067391269919,20.));
#93361=CARTESIAN_POINT('Ctrl Pts',(6.89854465491702,47.0989678378717,0.));
#93362=CARTESIAN_POINT('Ctrl Pts',(6.89854465491702,47.0989678378717,20.));
#93363=CARTESIAN_POINT('Ctrl Pts',(6.93094812982541,47.0911742123123,0.));
#93364=CARTESIAN_POINT('Ctrl Pts',(6.93094812982541,47.0911742123123,20.));
#93365=CARTESIAN_POINT('Ctrl Pts',(6.96334507674873,47.0833582549484,0.));
#93366=CARTESIAN_POINT('Ctrl Pts',(6.96334507674873,47.0833582549484,20.));
#93367=CARTESIAN_POINT('Ctrl Pts',(6.99573548013776,47.0755199704256,0.));
#93368=CARTESIAN_POINT('Ctrl Pts',(6.99573548013776,47.0755199704256,20.));
#93369=CARTESIAN_POINT('Ctrl Pts',(7.02811932444601,47.0676593634011,0.));
#93370=CARTESIAN_POINT('Ctrl Pts',(7.02811932444601,47.0676593634011,20.));
#93371=CARTESIAN_POINT('Ctrl Pts',(7.06049659413007,47.0597764385426,0.));
#93372=CARTESIAN_POINT('Ctrl Pts',(7.06049659413007,47.0597764385426,20.));
#93373=CARTESIAN_POINT('Ctrl Pts',(7.09286727364932,47.0518712005288,0.));
#93374=CARTESIAN_POINT('Ctrl Pts',(7.09286727364932,47.0518712005288,20.));
#93375=CARTESIAN_POINT('Ctrl Pts',(7.12523134746603,47.0439436540493,0.));
#93376=CARTESIAN_POINT('Ctrl Pts',(7.12523134746603,47.0439436540493,20.));
#93377=CARTESIAN_POINT('Ctrl Pts',(7.15758880004521,47.0359938038039,0.));
#93378=CARTESIAN_POINT('Ctrl Pts',(7.15758880004521,47.0359938038039,20.));
#93379=CARTESIAN_POINT('Ctrl Pts',(7.18993961585469,47.0280216545038,0.));
#93380=CARTESIAN_POINT('Ctrl Pts',(7.18993961585469,47.0280216545038,20.));
#93381=CARTESIAN_POINT('Ctrl Pts',(7.22228377936529,47.020027210871,0.));
#93382=CARTESIAN_POINT('Ctrl Pts',(7.22228377936529,47.020027210871,20.));
#93383=CARTESIAN_POINT('Ctrl Pts',(7.25462127505076,47.012010477639,0.));
#93384=CARTESIAN_POINT('Ctrl Pts',(7.25462127505076,47.012010477639,20.));
#93385=CARTESIAN_POINT('Ctrl Pts',(7.28695208738784,47.0039714595526,0.));
#93386=CARTESIAN_POINT('Ctrl Pts',(7.28695208738784,47.0039714595526,20.));
#93387=CARTESIAN_POINT('Ctrl Pts',(7.31927620085613,46.9959101613675,0.));
#93388=CARTESIAN_POINT('Ctrl Pts',(7.31927620085613,46.9959101613675,20.));
#93389=CARTESIAN_POINT('Ctrl Pts',(7.35159359993817,46.9878265878505,0.));
#93390=CARTESIAN_POINT('Ctrl Pts',(7.35159359993817,46.9878265878505,20.));
#93391=CARTESIAN_POINT('Ctrl Pts',(7.38390426911931,46.9797207437786,0.));
#93392=CARTESIAN_POINT('Ctrl Pts',(7.38390426911931,46.9797207437786,20.));
#93393=CARTESIAN_POINT('Ctrl Pts',(7.41620819288777,46.9715926339391,0.));
#93394=CARTESIAN_POINT('Ctrl Pts',(7.41620819288777,46.9715926339391,20.));
#93395=CARTESIAN_POINT('Ctrl Pts',(7.44850535573481,46.9634422631307,0.));
#93396=CARTESIAN_POINT('Ctrl Pts',(7.44850535573481,46.9634422631307,20.));
#93397=CARTESIAN_POINT('Ctrl Pts',(7.48079574215478,46.9552696361634,0.));
#93398=CARTESIAN_POINT('Ctrl Pts',(7.48079574215478,46.9552696361634,20.));
#93399=CARTESIAN_POINT('Ctrl Pts',(7.51307933664511,46.9470747578592,0.));
#93400=CARTESIAN_POINT('Ctrl Pts',(7.51307933664511,46.9470747578592,20.));
#93401=CARTESIAN_POINT('Ctrl Pts',(7.54535612370601,46.9388576330501,0.));
#93402=CARTESIAN_POINT('Ctrl Pts',(7.54535612370601,46.9388576330501,20.));
#93403=CARTESIAN_POINT('Ctrl Pts',(7.57762608784068,46.9306182665792,0.));
#93404=CARTESIAN_POINT('Ctrl Pts',(7.57762608784068,46.9306182665792,20.));
#93405=CARTESIAN_POINT('Ctrl Pts',(7.6098892135552,46.9223566632999,0.));
#93406=CARTESIAN_POINT('Ctrl Pts',(7.6098892135552,46.9223566632999,20.));
#93407=CARTESIAN_POINT('Ctrl Pts',(7.64214548535856,46.9140728280766,0.));
#93408=CARTESIAN_POINT('Ctrl Pts',(7.64214548535856,46.9140728280766,20.));
#93409=CARTESIAN_POINT('Ctrl Pts',(7.67439488776287,46.9057667657847,0.));
#93410=CARTESIAN_POINT('Ctrl Pts',(7.67439488776287,46.9057667657847,20.));
#93411=CARTESIAN_POINT('Ctrl Pts',(7.7066374052833,46.8974384813109,0.));
#93412=CARTESIAN_POINT('Ctrl Pts',(7.7066374052833,46.8974384813109,20.));
#93413=CARTESIAN_POINT('Ctrl Pts',(7.73887302243815,46.8890879795531,0.));
#93414=CARTESIAN_POINT('Ctrl Pts',(7.73887302243815,46.8890879795531,20.));
#93415=CARTESIAN_POINT('Ctrl Pts',(7.77110172374868,46.8807152654198,0.));
#93416=CARTESIAN_POINT('Ctrl Pts',(7.77110172374868,46.8807152654198,20.));
#93417=CARTESIAN_POINT('Ctrl Pts',(7.80332349373917,46.8723203438306,0.));
#93418=CARTESIAN_POINT('Ctrl Pts',(7.80332349373917,46.8723203438306,20.));
#93419=CARTESIAN_POINT('Ctrl Pts',(7.83553831693686,46.8639032197162,0.));
#93420=CARTESIAN_POINT('Ctrl Pts',(7.83553831693686,46.8639032197162,20.));
#93421=CARTESIAN_POINT('Ctrl Pts',(7.86774617787212,46.855463898018,0.));
#93422=CARTESIAN_POINT('Ctrl Pts',(7.86774617787212,46.855463898018,20.));
#93423=CARTESIAN_POINT('Ctrl Pts',(7.89994706107838,46.8470023836881,0.));
#93424=CARTESIAN_POINT('Ctrl Pts',(7.89994706107838,46.8470023836881,20.));
#93425=CARTESIAN_POINT('Ctrl Pts',(7.9321409510921,46.8385186816898,0.));
#93426=CARTESIAN_POINT('Ctrl Pts',(7.9321409510921,46.8385186816898,20.));
#93427=CARTESIAN_POINT('Ctrl Pts',(7.96432783245285,46.8300127969969,0.));
#93428=CARTESIAN_POINT('Ctrl Pts',(7.96432783245285,46.8300127969969,20.));
#93429=CARTESIAN_POINT('Ctrl Pts',(7.99650768970303,46.8214847345942,0.));
#93430=CARTESIAN_POINT('Ctrl Pts',(7.99650768970303,46.8214847345942,20.));
#93431=CARTESIAN_POINT('Ctrl Pts',(8.02868050738827,46.8129344994773,0.));
#93432=CARTESIAN_POINT('Ctrl Pts',(8.02868050738827,46.8129344994773,20.));
#93433=CARTESIAN_POINT('Ctrl Pts',(8.06084627005728,46.8043620966531,0.));
#93434=CARTESIAN_POINT('Ctrl Pts',(8.06084627005728,46.8043620966531,20.));
#93435=CARTESIAN_POINT('Ctrl Pts',(8.09300496226219,46.7957675311395,0.));
#93436=CARTESIAN_POINT('Ctrl Pts',(8.09300496226219,46.7957675311395,20.));
#93437=CARTESIAN_POINT('Ctrl Pts',(8.125156568558,46.7871508079658,0.));
#93438=CARTESIAN_POINT('Ctrl Pts',(8.125156568558,46.7871508079658,20.));
#93439=CARTESIAN_POINT('Ctrl Pts',(8.15730107350294,46.7785119321719,0.));
#93440=CARTESIAN_POINT('Ctrl Pts',(8.15730107350294,46.7785119321719,20.));
#93441=CARTESIAN_POINT('Ctrl Pts',(8.18943846165844,46.7698509088086,0.));
#93442=CARTESIAN_POINT('Ctrl Pts',(8.18943846165844,46.7698509088086,20.));
#93443=CARTESIAN_POINT('Ctrl Pts',(8.22156871758881,46.7611677429374,0.));
#93444=CARTESIAN_POINT('Ctrl Pts',(8.22156871758881,46.7611677429374,20.));
#93445=CARTESIAN_POINT('Ctrl Pts',(8.25369182586168,46.7524624396307,0.));
#93446=CARTESIAN_POINT('Ctrl Pts',(8.25369182586168,46.7524624396307,20.));
#93447=CARTESIAN_POINT('Ctrl Pts',(8.28580777104744,46.7437350039712,0.));
#93448=CARTESIAN_POINT('Ctrl Pts',(8.28580777104744,46.7437350039712,20.));
#93449=CARTESIAN_POINT('Ctrl Pts',(8.31791653771973,46.7349854410525,0.));
#93450=CARTESIAN_POINT('Ctrl Pts',(8.31791653771973,46.7349854410525,20.));
#93451=CARTESIAN_POINT('Ctrl Pts',(8.35001811045535,46.7262137559789,0.));
#93452=CARTESIAN_POINT('Ctrl Pts',(8.35001811045535,46.7262137559789,20.));
#93453=CARTESIAN_POINT('Ctrl Pts',(8.38211247383476,46.7174199538668,0.));
#93454=CARTESIAN_POINT('Ctrl Pts',(8.38211247383476,46.7174199538668,20.));
#93455=CARTESIAN_POINT('Ctrl Pts',(8.41419961244154,46.7086040398438,0.));
#93456=CARTESIAN_POINT('Ctrl Pts',(8.41419961244154,46.7086040398438,20.));
#93457=CARTESIAN_POINT('Ctrl Pts',(8.44627951086261,46.6997660190488,0.));
#93458=CARTESIAN_POINT('Ctrl Pts',(8.44627951086261,46.6997660190488,20.));
#93459=CARTESIAN_POINT('Ctrl Pts',(8.47835215368743,46.6909058966306,0.));
#93460=CARTESIAN_POINT('Ctrl Pts',(8.47835215368743,46.6909058966306,20.));
#93461=CARTESIAN_POINT('Ctrl Pts',(8.5104175255088,46.6820236777489,0.));
#93462=CARTESIAN_POINT('Ctrl Pts',(8.5104175255088,46.6820236777489,20.));
#93463=CARTESIAN_POINT('Ctrl Pts',(8.54247561092257,46.673119367573,0.));
#93464=CARTESIAN_POINT('Ctrl Pts',(8.54247561092257,46.673119367573,20.));
#93465=CARTESIAN_POINT('Ctrl Pts',(8.57452639452827,46.6641929712839,0.));
#93466=CARTESIAN_POINT('Ctrl Pts',(8.57452639452827,46.6641929712839,20.));
#93467=CARTESIAN_POINT('Ctrl Pts',(8.60656986092877,46.6552444940739,0.));
#93468=CARTESIAN_POINT('Ctrl Pts',(8.60656986092877,46.6552444940739,20.));
#93469=CARTESIAN_POINT('Ctrl Pts',(8.63860599473002,46.6462739411471,0.));
#93470=CARTESIAN_POINT('Ctrl Pts',(8.63860599473002,46.6462739411471,20.));
#93471=CARTESIAN_POINT('Ctrl Pts',(8.67063478054115,46.6372813177181,0.));
#93472=CARTESIAN_POINT('Ctrl Pts',(8.67063478054115,46.6372813177181,20.));
#93473=CARTESIAN_POINT('Ctrl Pts',(8.70265620297453,46.6282666290119,0.));
#93474=CARTESIAN_POINT('Ctrl Pts',(8.70265620297453,46.6282666290119,20.));
#93475=CARTESIAN_POINT('Ctrl Pts',(8.73467024664569,46.6192298802645,0.));
#93476=CARTESIAN_POINT('Ctrl Pts',(8.73467024664569,46.6192298802645,20.));
#93477=CARTESIAN_POINT('Ctrl Pts',(8.76667689617329,46.6101710767218,0.));
#93478=CARTESIAN_POINT('Ctrl Pts',(8.76667689617329,46.6101710767218,20.));
#93479=CARTESIAN_POINT('Ctrl Pts',(8.79867613617932,46.6010902236408,0.));
#93480=CARTESIAN_POINT('Ctrl Pts',(8.79867613617932,46.6010902236408,20.));
#93481=CARTESIAN_POINT('Ctrl Pts',(8.83066795128933,46.59198732629,0.));
#93482=CARTESIAN_POINT('Ctrl Pts',(8.83066795128933,46.59198732629,20.));
#93483=CARTESIAN_POINT('Ctrl Pts',(8.86265232613214,46.582862389949,0.));
#93484=CARTESIAN_POINT('Ctrl Pts',(8.86265232613214,46.582862389949,20.));
#93485=CARTESIAN_POINT('Ctrl Pts',(8.89462924533988,46.5737154199087,0.));
#93486=CARTESIAN_POINT('Ctrl Pts',(8.89462924533988,46.5737154199087,20.));
#93487=CARTESIAN_POINT('Ctrl Pts',(8.92659869354787,46.5645464214705,0.));
#93488=CARTESIAN_POINT('Ctrl Pts',(8.92659869354787,46.5645464214705,20.));
#93489=CARTESIAN_POINT('Ctrl Pts',(8.9585606553947,46.5553553999467,0.));
#93490=CARTESIAN_POINT('Ctrl Pts',(8.9585606553947,46.5553553999467,20.));
#93491=CARTESIAN_POINT('Ctrl Pts',(8.99051511552228,46.5461423606602,0.));
#93492=CARTESIAN_POINT('Ctrl Pts',(8.99051511552228,46.5461423606602,20.));
#93493=CARTESIAN_POINT('Ctrl Pts',(9.02246205857627,46.5369073089453,0.));
#93494=CARTESIAN_POINT('Ctrl Pts',(9.02246205857627,46.5369073089453,20.));
#93495=CARTESIAN_POINT('Ctrl Pts',(9.05440146920514,46.5276502501459,0.));
#93496=CARTESIAN_POINT('Ctrl Pts',(9.05440146920514,46.5276502501459,20.));
#93497=CARTESIAN_POINT('Ctrl Pts',(9.08633333206089,46.5183711896174,0.));
#93498=CARTESIAN_POINT('Ctrl Pts',(9.08633333206089,46.5183711896174,20.));
#93499=CARTESIAN_POINT('Ctrl Pts',(9.11825763179851,46.5090701327255,0.));
#93500=CARTESIAN_POINT('Ctrl Pts',(9.11825763179851,46.5090701327255,20.));
#93501=CARTESIAN_POINT('Ctrl Pts',(9.15017435307665,46.4997470848477,0.));
#93502=CARTESIAN_POINT('Ctrl Pts',(9.15017435307665,46.4997470848477,20.));
#93503=CARTESIAN_POINT('Ctrl Pts',(9.18208348055724,46.4904020513722,0.));
#93504=CARTESIAN_POINT('Ctrl Pts',(9.18208348055724,46.4904020513722,20.));
#93505=CARTESIAN_POINT('Ctrl Pts',(9.21398499890591,46.4810350376983,0.));
#93506=CARTESIAN_POINT('Ctrl Pts',(9.21398499890591,46.4810350376983,20.));
#93507=CARTESIAN_POINT('Ctrl Pts',(9.2458788927917,46.4716460492361,0.));
#93508=CARTESIAN_POINT('Ctrl Pts',(9.2458788927917,46.4716460492361,20.));
#93509=CARTESIAN_POINT('Ctrl Pts',(9.27776514688698,46.4622350914066,0.));
#93510=CARTESIAN_POINT('Ctrl Pts',(9.27776514688698,46.4622350914066,20.));
#93511=CARTESIAN_POINT('Ctrl Pts',(9.30964374586751,46.4528021696416,0.));
#93512=CARTESIAN_POINT('Ctrl Pts',(9.30964374586751,46.4528021696416,20.));
#93513=CARTESIAN_POINT('Ctrl Pts',(9.3415146744124,46.4433472893837,0.));
#93514=CARTESIAN_POINT('Ctrl Pts',(9.3415146744124,46.4433472893837,20.));
#93515=CARTESIAN_POINT('Ctrl Pts',(9.37337791720392,46.4338704560856,0.));
#93516=CARTESIAN_POINT('Ctrl Pts',(9.37337791720392,46.4338704560856,20.));
#93517=CARTESIAN_POINT('Ctrl Pts',(9.40523345892773,46.4243716752115,0.));
#93518=CARTESIAN_POINT('Ctrl Pts',(9.40523345892773,46.4243716752115,20.));
#93519=CARTESIAN_POINT('Ctrl Pts',(9.43708128427273,46.4148509522358,0.));
#93520=CARTESIAN_POINT('Ctrl Pts',(9.43708128427273,46.4148509522358,20.));
#93521=CARTESIAN_POINT('Ctrl Pts',(9.46892137793147,46.405308292644,0.));
#93522=CARTESIAN_POINT('Ctrl Pts',(9.46892137793147,46.405308292644,20.));
#93523=CARTESIAN_POINT('Ctrl Pts',(9.50075372460008,46.3957437019326,0.));
#93524=CARTESIAN_POINT('Ctrl Pts',(9.50075372460008,46.3957437019326,20.));
#93525=CARTESIAN_POINT('Ctrl Pts',(9.5325783089785,46.3861571856095,0.));
#93526=CARTESIAN_POINT('Ctrl Pts',(9.5325783089785,46.3861571856095,20.));
#93527=CARTESIAN_POINT('Ctrl Pts',(9.56439511577022,46.3765487491938,0.));
#93528=CARTESIAN_POINT('Ctrl Pts',(9.56439511577022,46.3765487491938,20.));
#93529=CARTESIAN_POINT('Ctrl Pts',(9.59620412968212,46.3669183982155,0.));
#93530=CARTESIAN_POINT('Ctrl Pts',(9.59620412968212,46.3669183982155,20.));
#93531=CARTESIAN_POINT('Ctrl Pts',(9.62800533542435,46.3572661382147,0.));
#93532=CARTESIAN_POINT('Ctrl Pts',(9.62800533542435,46.3572661382147,20.));
#93533=CARTESIAN_POINT('Ctrl Pts',(9.65979871771038,46.347591974742,0.));
#93534=CARTESIAN_POINT('Ctrl Pts',(9.65979871771038,46.347591974742,20.));
#93535=CARTESIAN_POINT('Ctrl Pts',(9.69158426125691,46.3378959133587,0.));
#93536=CARTESIAN_POINT('Ctrl Pts',(9.69158426125691,46.3378959133587,20.));
#93537=CARTESIAN_POINT('Ctrl Pts',(9.72336195078413,46.3281779596367,0.));
#93538=CARTESIAN_POINT('Ctrl Pts',(9.72336195078413,46.3281779596367,20.));
#93539=CARTESIAN_POINT('Ctrl Pts',(9.75513177101576,46.3184381191592,0.));
#93540=CARTESIAN_POINT('Ctrl Pts',(9.75513177101576,46.3184381191592,20.));
#93541=CARTESIAN_POINT('Ctrl Pts',(9.78689370667939,46.3086763975205,0.));
#93542=CARTESIAN_POINT('Ctrl Pts',(9.78689370667939,46.3086763975205,20.));
#93543=CARTESIAN_POINT('Ctrl Pts',(9.81864774250618,46.2988928003257,0.));
#93544=CARTESIAN_POINT('Ctrl Pts',(9.81864774250618,46.2988928003257,20.));
#93545=CARTESIAN_POINT('Ctrl Pts',(9.85039386323084,46.289087333191,0.));
#93546=CARTESIAN_POINT('Ctrl Pts',(9.85039386323084,46.289087333191,20.));
#93547=CARTESIAN_POINT('Ctrl Pts',(9.8821320535919,46.2792600017436,0.));
#93548=CARTESIAN_POINT('Ctrl Pts',(9.8821320535919,46.2792600017436,20.));
#93549=CARTESIAN_POINT('Ctrl Pts',(9.91386229833136,46.2694108116213,0.));
#93550=CARTESIAN_POINT('Ctrl Pts',(9.91386229833136,46.2694108116213,20.));
#93551=CARTESIAN_POINT('Ctrl Pts',(9.94558458219445,46.2595397684724,0.));
#93552=CARTESIAN_POINT('Ctrl Pts',(9.94558458219445,46.2595397684724,20.));
#93553=CARTESIAN_POINT('Ctrl Pts',(9.97729888992979,46.2496468779557,0.));
#93554=CARTESIAN_POINT('Ctrl Pts',(9.97729888992979,46.2496468779557,20.));
#93555=CARTESIAN_POINT('Ctrl Pts',(10.0090052062894,46.2397321457408,0.));
#93556=CARTESIAN_POINT('Ctrl Pts',(10.0090052062894,46.2397321457408,20.));
#93557=CARTESIAN_POINT('Ctrl Pts',(10.0407035160292,46.2297955775084,0.));
#93558=CARTESIAN_POINT('Ctrl Pts',(10.0407035160292,46.2297955775084,20.));
#93559=CARTESIAN_POINT('Ctrl Pts',(10.0723938039086,46.2198371789501,0.));
#93560=CARTESIAN_POINT('Ctrl Pts',(10.0723938039086,46.2198371789501,20.));
#93561=CARTESIAN_POINT('Ctrl Pts',(10.1040760546909,46.2098569557688,0.));
#93562=CARTESIAN_POINT('Ctrl Pts',(10.1040760546909,46.2098569557688,20.));
#93563=CARTESIAN_POINT('Ctrl Pts',(10.1357502531431,46.1998549136779,0.));
#93564=CARTESIAN_POINT('Ctrl Pts',(10.1357502531431,46.1998549136779,20.));
#93565=CARTESIAN_POINT('Ctrl Pts',(10.1674163840354,46.1898310584014,0.));
#93566=CARTESIAN_POINT('Ctrl Pts',(10.1674163840354,46.1898310584014,20.));
#93567=CARTESIAN_POINT('Ctrl Pts',(10.199074432142,46.179785395674,0.));
#93568=CARTESIAN_POINT('Ctrl Pts',(10.199074432142,46.179785395674,20.));
#93569=CARTESIAN_POINT('Ctrl Pts',(10.2307243822402,46.169717931241,0.));
#93570=CARTESIAN_POINT('Ctrl Pts',(10.2307243822402,46.169717931241,20.));
#93571=CARTESIAN_POINT('Ctrl Pts',(10.2623662191113,46.1596286708586,0.));
#93572=CARTESIAN_POINT('Ctrl Pts',(10.2623662191113,46.1596286708586,20.));
#93573=CARTESIAN_POINT('Ctrl Pts',(10.2939999275403,46.1495176202946,0.));
#93574=CARTESIAN_POINT('Ctrl Pts',(10.2939999275403,46.1495176202946,20.));
#93575=CARTESIAN_POINT('Ctrl Pts',(10.3256254923155,46.139384785327,0.));
#93576=CARTESIAN_POINT('Ctrl Pts',(10.3256254923155,46.139384785327,20.));
#93577=CARTESIAN_POINT('Ctrl Pts',(10.3572428982293,46.1292301717445,0.));
#93578=CARTESIAN_POINT('Ctrl Pts',(10.3572428982293,46.1292301717445,20.));
#93579=CARTESIAN_POINT('Ctrl Pts',(10.3888521300773,46.119053785347,0.));
#93580=CARTESIAN_POINT('Ctrl Pts',(10.3888521300773,46.119053785347,20.));
#93581=CARTESIAN_POINT('Ctrl Pts',(10.4204531726593,46.1088556319449,0.));
#93582=CARTESIAN_POINT('Ctrl Pts',(10.4204531726593,46.1088556319449,20.));
#93583=CARTESIAN_POINT('Ctrl Pts',(10.4520460107784,46.0986357173598,0.));
#93584=CARTESIAN_POINT('Ctrl Pts',(10.4520460107784,46.0986357173598,20.));
#93585=CARTESIAN_POINT('Ctrl Pts',(10.4836306292415,46.0883940474237,0.));
#93586=CARTESIAN_POINT('Ctrl Pts',(10.4836306292415,46.0883940474237,20.));
#93587=CARTESIAN_POINT('Ctrl Pts',(10.5152070128592,46.0781306279792,0.));
#93588=CARTESIAN_POINT('Ctrl Pts',(10.5152070128592,46.0781306279792,20.));
#93589=CARTESIAN_POINT('Ctrl Pts',(10.5467751464457,46.0678454648793,0.));
#93590=CARTESIAN_POINT('Ctrl Pts',(10.5467751464457,46.0678454648793,20.));
#93591=CARTESIAN_POINT('Ctrl Pts',(10.5783350148187,46.0575385639878,0.));
#93592=CARTESIAN_POINT('Ctrl Pts',(10.5783350148187,46.0575385639878,20.));
#93593=CARTESIAN_POINT('Ctrl Pts',(10.6098866028001,46.0472099311799,0.));
#93594=CARTESIAN_POINT('Ctrl Pts',(10.6098866028001,46.0472099311799,20.));
#93595=CARTESIAN_POINT('Ctrl Pts',(10.6414298952151,46.0368595723418,0.));
#93596=CARTESIAN_POINT('Ctrl Pts',(10.6414298952151,46.0368595723418,20.));
#93597=CARTESIAN_POINT('Ctrl Pts',(10.6729648768932,46.0264874933706,0.));
#93598=CARTESIAN_POINT('Ctrl Pts',(10.6729648768932,46.0264874933706,20.));
#93599=CARTESIAN_POINT('Ctrl Pts',(10.7044915326674,46.0160937001747,0.));
#93600=CARTESIAN_POINT('Ctrl Pts',(10.7044915326674,46.0160937001747,20.));
#93601=CARTESIAN_POINT('Ctrl Pts',(10.7360098473747,46.0056781986726,0.));
#93602=CARTESIAN_POINT('Ctrl Pts',(10.7360098473747,46.0056781986726,20.));
#93603=CARTESIAN_POINT('Ctrl Pts',(10.7675198058554,45.9952409947932,0.));
#93604=CARTESIAN_POINT('Ctrl Pts',(10.7675198058554,45.9952409947932,20.));
#93605=CARTESIAN_POINT('Ctrl Pts',(10.7990213929536,45.9847820944759,0.));
#93606=CARTESIAN_POINT('Ctrl Pts',(10.7990213929536,45.9847820944759,20.));
#93607=CARTESIAN_POINT('Ctrl Pts',(10.8305145935168,45.9743015036702,0.));
#93608=CARTESIAN_POINT('Ctrl Pts',(10.8305145935168,45.9743015036702,20.));
#93609=CARTESIAN_POINT('Ctrl Pts',(10.8619993923966,45.9637992283368,0.));
#93610=CARTESIAN_POINT('Ctrl Pts',(10.8619993923966,45.9637992283368,20.));
#93611=CARTESIAN_POINT('Ctrl Pts',(10.8934757744485,45.9532752744476,0.));
#93612=CARTESIAN_POINT('Ctrl Pts',(10.8934757744485,45.9532752744476,20.));
#93613=CARTESIAN_POINT('Ctrl Pts',(10.9249437245321,45.9427296479861,0.));
#93614=CARTESIAN_POINT('Ctrl Pts',(10.9249437245321,45.9427296479861,20.));
#93615=CARTESIAN_POINT('Ctrl Pts',(10.9564032275107,45.9321623549466,0.));
#93616=CARTESIAN_POINT('Ctrl Pts',(10.9564032275107,45.9321623549466,20.));
#93617=CARTESIAN_POINT('Ctrl Pts',(10.9878542682513,45.9215734013338,0.));
#93618=CARTESIAN_POINT('Ctrl Pts',(10.9878542682513,45.9215734013338,20.));
#93619=CARTESIAN_POINT('Ctrl Pts',(11.0192968316246,45.9109627931629,0.));
#93620=CARTESIAN_POINT('Ctrl Pts',(11.0192968316246,45.9109627931629,20.));
#93621=CARTESIAN_POINT('Ctrl Pts',(11.0507309025052,45.9003305364593,0.));
#93622=CARTESIAN_POINT('Ctrl Pts',(11.0507309025052,45.9003305364593,20.));
#93623=CARTESIAN_POINT('Ctrl Pts',(11.0821564657716,45.8896766372596,0.));
#93624=CARTESIAN_POINT('Ctrl Pts',(11.0821564657716,45.8896766372596,20.));
#93625=CARTESIAN_POINT('Ctrl Pts',(11.1135735063059,45.8790011016108,0.));
#93626=CARTESIAN_POINT('Ctrl Pts',(11.1135735063059,45.8790011016108,20.));
#93627=CARTESIAN_POINT('Ctrl Pts',(11.1449820089942,45.868303935571,0.));
#93628=CARTESIAN_POINT('Ctrl Pts',(11.1449820089942,45.868303935571,20.));
#93629=CARTESIAN_POINT('Ctrl Pts',(11.1763819587262,45.8575851452088,0.));
#93630=CARTESIAN_POINT('Ctrl Pts',(11.1763819587262,45.8575851452088,20.));
#93631=CARTESIAN_POINT('Ctrl Pts',(11.2077733403959,45.8468447366038,0.));
#93632=CARTESIAN_POINT('Ctrl Pts',(11.2077733403959,45.8468447366038,20.));
#93633=CARTESIAN_POINT('Ctrl Pts',(11.2391561389011,45.8360827158468,0.));
#93634=CARTESIAN_POINT('Ctrl Pts',(11.2391561389011,45.8360827158468,20.));
#93635=CARTESIAN_POINT('Ctrl Pts',(11.2705303391434,45.8252990890386,0.));
#93636=CARTESIAN_POINT('Ctrl Pts',(11.2705303391434,45.8252990890386,20.));
#93637=CARTESIAN_POINT('Ctrl Pts',(11.3018959260282,45.8144938622913,0.));
#93638=CARTESIAN_POINT('Ctrl Pts',(11.3018959260282,45.8144938622913,20.));
#93639=CARTESIAN_POINT('Ctrl Pts',(11.3332528844652,45.8036670417272,0.));
#93640=CARTESIAN_POINT('Ctrl Pts',(11.3332528844652,45.8036670417272,20.));
#93641=CARTESIAN_POINT('Ctrl Pts',(11.3646011993673,45.7928186334791,0.));
#93642=CARTESIAN_POINT('Ctrl Pts',(11.3646011993673,45.7928186334791,20.));
#93643=CARTESIAN_POINT('Ctrl Pts',(11.395940855652,45.7819486436912,0.));
#93644=CARTESIAN_POINT('Ctrl Pts',(11.395940855652,45.7819486436912,20.));
#93645=CARTESIAN_POINT('Ctrl Pts',(11.4272718382403,45.7710570785186,0.));
#93646=CARTESIAN_POINT('Ctrl Pts',(11.4272718382403,45.7710570785186,20.));
#93647=CARTESIAN_POINT('Ctrl Pts',(11.4585941320574,45.760143944127,0.));
#93648=CARTESIAN_POINT('Ctrl Pts',(11.4585941320574,45.760143944127,20.));
#93649=CARTESIAN_POINT('Ctrl Pts',(11.489907722032,45.7492092466918,0.));
#93650=CARTESIAN_POINT('Ctrl Pts',(11.489907722032,45.7492092466918,20.));
#93651=CARTESIAN_POINT('Ctrl Pts',(11.5212125930966,45.7382529923996,0.));
#93652=CARTESIAN_POINT('Ctrl Pts',(11.5212125930966,45.7382529923996,20.));
#93653=CARTESIAN_POINT('Ctrl Pts',(11.5525087301884,45.7272751874478,0.));
#93654=CARTESIAN_POINT('Ctrl Pts',(11.5525087301884,45.7272751874478,20.));
#93655=CARTESIAN_POINT('Ctrl Pts',(11.5837961182481,45.7162758380449,0.));
#93656=CARTESIAN_POINT('Ctrl Pts',(11.5837961182481,45.7162758380449,20.));
#93657=CARTESIAN_POINT('Ctrl Pts',(11.6150747422209,45.7052549504103,0.));
#93658=CARTESIAN_POINT('Ctrl Pts',(11.6150747422209,45.7052549504103,20.));
#93659=CARTESIAN_POINT('Ctrl Pts',(11.6463445870557,45.694212530774,0.));
#93660=CARTESIAN_POINT('Ctrl Pts',(11.6463445870557,45.694212530774,20.));
#93661=CARTESIAN_POINT('Ctrl Pts',(11.6776056377055,45.6831485853771,0.));
#93662=CARTESIAN_POINT('Ctrl Pts',(11.6776056377055,45.6831485853771,20.));
#93663=CARTESIAN_POINT('Ctrl Pts',(11.7088578791266,45.6720631204703,0.));
#93664=CARTESIAN_POINT('Ctrl Pts',(11.7088578791266,45.6720631204703,20.));
#93665=CARTESIAN_POINT('Ctrl Pts',(11.7401012962797,45.6609561423149,0.));
#93666=CARTESIAN_POINT('Ctrl Pts',(11.7401012962797,45.6609561423149,20.));
#93667=CARTESIAN_POINT('Ctrl Pts',(11.7713358741292,45.6498276571829,0.));
#93668=CARTESIAN_POINT('Ctrl Pts',(11.7713358741292,45.6498276571829,20.));
#93669=CARTESIAN_POINT('Ctrl Pts',(11.8025615976441,45.6386776713575,0.));
#93670=CARTESIAN_POINT('Ctrl Pts',(11.8025615976441,45.6386776713575,20.));
#93671=CARTESIAN_POINT('Ctrl Pts',(11.8337784517972,45.627506191133,0.));
#93672=CARTESIAN_POINT('Ctrl Pts',(11.8337784517972,45.627506191133,20.));
#93673=CARTESIAN_POINT('Ctrl Pts',(11.8649864215653,45.6163132228138,0.));
#93674=CARTESIAN_POINT('Ctrl Pts',(11.8649864215653,45.6163132228138,20.));
#93675=CARTESIAN_POINT('Ctrl Pts',(11.8961854919293,45.6050987727153,0.));
#93676=CARTESIAN_POINT('Ctrl Pts',(11.8961854919293,45.6050987727153,20.));
#93677=CARTESIAN_POINT('Ctrl Pts',(11.9273756478741,45.5938628471638,0.));
#93678=CARTESIAN_POINT('Ctrl Pts',(11.9273756478741,45.5938628471638,20.));
#93679=CARTESIAN_POINT('Ctrl Pts',(11.9585568743886,45.5826054524963,0.));
#93680=CARTESIAN_POINT('Ctrl Pts',(11.9585568743886,45.5826054524963,20.));
#93681=CARTESIAN_POINT('Ctrl Pts',(11.989729156466,45.5713265950605,0.));
#93682=CARTESIAN_POINT('Ctrl Pts',(11.989729156466,45.5713265950605,20.));
#93683=CARTESIAN_POINT('Ctrl Pts',(12.0208924791034,45.5600262812144,0.));
#93684=CARTESIAN_POINT('Ctrl Pts',(12.0208924791034,45.5600262812144,20.));
#93685=CARTESIAN_POINT('Ctrl Pts',(12.0520468273019,45.5487045173265,0.));
#93686=CARTESIAN_POINT('Ctrl Pts',(12.0520468273019,45.5487045173265,20.));
#93687=CARTESIAN_POINT('Ctrl Pts',(12.0831921860665,45.5373613097755,0.));
#93688=CARTESIAN_POINT('Ctrl Pts',(12.0831921860665,45.5373613097755,20.));
#93689=CARTESIAN_POINT('Ctrl Pts',(12.1143285404065,45.5259966649516,0.));
#93690=CARTESIAN_POINT('Ctrl Pts',(12.1143285404065,45.5259966649516,20.));
#93691=CARTESIAN_POINT('Ctrl Pts',(12.1454558753351,45.5146105892553,0.));
#93692=CARTESIAN_POINT('Ctrl Pts',(12.1454558753351,45.5146105892553,20.));
#93693=CARTESIAN_POINT('Ctrl Pts',(12.1765741758697,45.5032030890978,0.));
#93694=CARTESIAN_POINT('Ctrl Pts',(12.1765741758697,45.5032030890978,20.));
#93695=CARTESIAN_POINT('Ctrl Pts',(12.2076834270323,45.4917741709015,0.));
#93696=CARTESIAN_POINT('Ctrl Pts',(12.2076834270323,45.4917741709015,20.));
#93697=CARTESIAN_POINT('Ctrl Pts',(12.2387836138487,45.4803238410999,0.));
#93698=CARTESIAN_POINT('Ctrl Pts',(12.2387836138487,45.4803238410999,20.));
#93699=CARTESIAN_POINT('Ctrl Pts',(12.269874721349,45.4688521061371,0.));
#93700=CARTESIAN_POINT('Ctrl Pts',(12.269874721349,45.4688521061371,20.));
#93701=CARTESIAN_POINT('Ctrl Pts',(12.3009567345673,45.4573589724673,0.));
#93702=CARTESIAN_POINT('Ctrl Pts',(12.3009567345673,45.4573589724673,20.));
#93703=CARTESIAN_POINT('Ctrl Pts',(12.3320296385417,45.4458444465552,0.));
#93704=CARTESIAN_POINT('Ctrl Pts',(12.3320296385417,45.4458444465552,20.));
#93705=CARTESIAN_POINT('Ctrl Pts',(12.3630934183142,45.4343085348755,0.));
#93706=CARTESIAN_POINT('Ctrl Pts',(12.3630934183142,45.4343085348755,20.));
#93707=CARTESIAN_POINT('Ctrl Pts',(12.3941480589311,45.4227512439136,0.));
#93708=CARTESIAN_POINT('Ctrl Pts',(12.3941480589311,45.4227512439136,20.));
#93709=CARTESIAN_POINT('Ctrl Pts',(12.4251935454428,45.4111725801659,0.));
#93710=CARTESIAN_POINT('Ctrl Pts',(12.4251935454428,45.4111725801659,20.));
#93711=CARTESIAN_POINT('Ctrl Pts',(12.4562298629045,45.3995725501402,0.));
#93712=CARTESIAN_POINT('Ctrl Pts',(12.4562298629045,45.3995725501402,20.));
#93713=CARTESIAN_POINT('Ctrl Pts',(12.4872569963754,45.3879511603549,0.));
#93714=CARTESIAN_POINT('Ctrl Pts',(12.4872569963754,45.3879511603549,20.));
#93715=CARTESIAN_POINT('Ctrl Pts',(12.5182749309189,45.376308417339,0.));
#93716=CARTESIAN_POINT('Ctrl Pts',(12.5182749309189,45.376308417339,20.));
#93717=CARTESIAN_POINT('Ctrl Pts',(12.5492836516023,45.364644327632,0.));
#93718=CARTESIAN_POINT('Ctrl Pts',(12.5492836516023,45.364644327632,20.));
#93719=CARTESIAN_POINT('Ctrl Pts',(12.5802831434966,45.3529588977839,0.));
#93720=CARTESIAN_POINT('Ctrl Pts',(12.5802831434966,45.3529588977839,20.));
#93721=CARTESIAN_POINT('Ctrl Pts',(12.6112733916776,45.3412521343551,0.));
#93722=CARTESIAN_POINT('Ctrl Pts',(12.6112733916776,45.3412521343551,20.));
#93723=CARTESIAN_POINT('Ctrl Pts',(12.6422543812251,45.3295240439169,0.));
#93724=CARTESIAN_POINT('Ctrl Pts',(12.6422543812251,45.3295240439169,20.));
#93725=CARTESIAN_POINT('Ctrl Pts',(12.6732260972239,45.3177746330512,0.));
#93726=CARTESIAN_POINT('Ctrl Pts',(12.6732260972239,45.3177746330512,20.));
#93727=CARTESIAN_POINT('Ctrl Pts',(12.7041885247626,45.3060039083501,0.));
#93728=CARTESIAN_POINT('Ctrl Pts',(12.7041885247626,45.3060039083501,20.));
#93729=CARTESIAN_POINT('Ctrl Pts',(12.7351416489341,45.2942118764167,0.));
#93730=CARTESIAN_POINT('Ctrl Pts',(12.7351416489341,45.2942118764167,20.));
#93731=CARTESIAN_POINT('Ctrl Pts',(12.7660854548354,45.2823985438647,0.));
#93732=CARTESIAN_POINT('Ctrl Pts',(12.7660854548354,45.2823985438647,20.));
#93733=CARTESIAN_POINT('Ctrl Pts',(12.7970199275678,45.2705639173192,0.));
#93734=CARTESIAN_POINT('Ctrl Pts',(12.7970199275678,45.2705639173192,20.));
#93735=CARTESIAN_POINT('Ctrl Pts',(12.8279450522365,45.2587080034157,0.));
#93736=CARTESIAN_POINT('Ctrl Pts',(12.8279450522365,45.2587080034157,20.));
#93737=CARTESIAN_POINT('Ctrl Pts',(12.8588608139512,45.2468308087994,0.));
#93738=CARTESIAN_POINT('Ctrl Pts',(12.8588608139512,45.2468308087994,20.));
#93739=CARTESIAN_POINT('Ctrl Pts',(12.8897671978256,45.2349323401259,0.));
#93740=CARTESIAN_POINT('Ctrl Pts',(12.8897671978256,45.2349323401259,20.));
#93741=CARTESIAN_POINT('Ctrl Pts',(12.9206641889781,45.2230126040617,0.));
#93742=CARTESIAN_POINT('Ctrl Pts',(12.9206641889781,45.2230126040617,20.));
#93743=CARTESIAN_POINT('Ctrl Pts',(12.9515517725313,45.2110716072841,0.));
#93744=CARTESIAN_POINT('Ctrl Pts',(12.9515517725313,45.2110716072841,20.));
#93745=CARTESIAN_POINT('Ctrl Pts',(12.9824299336127,45.199109356482,0.));
#93746=CARTESIAN_POINT('Ctrl Pts',(12.9824299336127,45.199109356482,20.));
#93747=CARTESIAN_POINT('Ctrl Pts',(13.0132986573536,45.1871258583545,0.));
#93748=CARTESIAN_POINT('Ctrl Pts',(13.0132986573536,45.1871258583545,20.));
#93749=CARTESIAN_POINT('Ctrl Pts',(13.0441579288899,45.1751211196118,0.));
#93750=CARTESIAN_POINT('Ctrl Pts',(13.0441579288899,45.1751211196118,20.));
#93751=CARTESIAN_POINT('Ctrl Pts',(13.0750077333613,45.1630951469734,0.));
#93752=CARTESIAN_POINT('Ctrl Pts',(13.0750077333613,45.1630951469734,20.));
#93753=CARTESIAN_POINT('Ctrl Pts',(13.105848055912,45.1510479471692,0.));
#93754=CARTESIAN_POINT('Ctrl Pts',(13.105848055912,45.1510479471692,20.));
#93755=CARTESIAN_POINT('Ctrl Pts',(13.1366788816904,45.1389795269399,0.));
#93756=CARTESIAN_POINT('Ctrl Pts',(13.1366788816904,45.1389795269399,20.));
#93757=CARTESIAN_POINT('Ctrl Pts',(13.1675001958492,45.1268898930368,0.));
#93758=CARTESIAN_POINT('Ctrl Pts',(13.1675001958492,45.1268898930368,20.));
#93759=CARTESIAN_POINT('Ctrl Pts',(13.198311983546,45.114779052223,0.));
#93760=CARTESIAN_POINT('Ctrl Pts',(13.198311983546,45.114779052223,20.));
#93761=CARTESIAN_POINT('Ctrl Pts',(13.2291142299426,45.1026470112717,0.));
#93762=CARTESIAN_POINT('Ctrl Pts',(13.2291142299426,45.1026470112717,20.));
#93763=CARTESIAN_POINT('Ctrl Pts',(13.259906920205,45.0904937769663,0.));
#93764=CARTESIAN_POINT('Ctrl Pts',(13.259906920205,45.0904937769663,20.));
#93765=CARTESIAN_POINT('Ctrl Pts',(13.2906900395037,45.0783193561008,0.));
#93766=CARTESIAN_POINT('Ctrl Pts',(13.2906900395037,45.0783193561008,20.));
#93767=CARTESIAN_POINT('Ctrl Pts',(13.3214635730135,45.0661237554798,0.));
#93768=CARTESIAN_POINT('Ctrl Pts',(13.3214635730135,45.0661237554798,20.));
#93769=CARTESIAN_POINT('Ctrl Pts',(13.3522275059137,45.0539069819185,0.));
#93770=CARTESIAN_POINT('Ctrl Pts',(13.3522275059137,45.0539069819185,20.));
#93771=CARTESIAN_POINT('Ctrl Pts',(13.3829818233878,45.0416690422424,0.));
#93772=CARTESIAN_POINT('Ctrl Pts',(13.3829818233878,45.0416690422424,20.));
#93773=CARTESIAN_POINT('Ctrl Pts',(13.4137265106238,45.029409943288,0.));
#93774=CARTESIAN_POINT('Ctrl Pts',(13.4137265106238,45.029409943288,20.));
#93775=CARTESIAN_POINT('Ctrl Pts',(13.4444615528144,45.0171296919022,0.));
#93776=CARTESIAN_POINT('Ctrl Pts',(13.4444615528144,45.0171296919022,20.));
#93777=CARTESIAN_POINT('Ctrl Pts',(13.4751869351564,45.0048282949433,0.));
#93778=CARTESIAN_POINT('Ctrl Pts',(13.4751869351564,45.0048282949433,20.));
#93779=CARTESIAN_POINT('Ctrl Pts',(13.5059026428512,44.9925057592796,0.));
#93780=CARTESIAN_POINT('Ctrl Pts',(13.5059026428512,44.9925057592796,20.));
#93781=CARTESIAN_POINT('Ctrl Pts',(13.5366086611044,44.9801620917891,0.));
#93782=CARTESIAN_POINT('Ctrl Pts',(13.5366086611044,44.9801620917891,20.));
#93783=CARTESIAN_POINT('Ctrl Pts',(13.5673049751264,44.967797299361,0.));
#93784=CARTESIAN_POINT('Ctrl Pts',(13.5673049751264,44.967797299361,20.));
#93785=CARTESIAN_POINT('Ctrl Pts',(13.5979915701319,44.955411388895,0.));
#93786=CARTESIAN_POINT('Ctrl Pts',(13.5979915701319,44.955411388895,20.));
#93787=CARTESIAN_POINT('Ctrl Pts',(13.6286684313401,44.9430043673018,0.));
#93788=CARTESIAN_POINT('Ctrl Pts',(13.6286684313401,44.9430043673018,20.));
#93789=CARTESIAN_POINT('Ctrl Pts',(13.6593355439745,44.930576241502,0.));
#93790=CARTESIAN_POINT('Ctrl Pts',(13.6593355439745,44.930576241502,20.));
#93791=CARTESIAN_POINT('Ctrl Pts',(13.6899928932632,44.9181270184275,0.));
#93792=CARTESIAN_POINT('Ctrl Pts',(13.6899928932632,44.9181270184275,20.));
#93793=CARTESIAN_POINT('Ctrl Pts',(13.7206404644388,44.9056567050204,0.));
#93794=CARTESIAN_POINT('Ctrl Pts',(13.7206404644388,44.9056567050204,20.));
#93795=CARTESIAN_POINT('Ctrl Pts',(13.7512782427386,44.8931653082334,0.));
#93796=CARTESIAN_POINT('Ctrl Pts',(13.7512782427386,44.8931653082334,20.));
#93797=CARTESIAN_POINT('Ctrl Pts',(13.7819062134042,44.8806528350291,0.));
#93798=CARTESIAN_POINT('Ctrl Pts',(13.7819062134042,44.8806528350291,20.));
#93799=CARTESIAN_POINT('Ctrl Pts',(13.8125243616816,44.8681192923811,0.));
#93800=CARTESIAN_POINT('Ctrl Pts',(13.8125243616816,44.8681192923811,20.));
#93801=CARTESIAN_POINT('Ctrl Pts',(13.8431326728214,44.8555646872732,0.));
#93802=CARTESIAN_POINT('Ctrl Pts',(13.8431326728214,44.8555646872732,20.));
#93803=CARTESIAN_POINT('Ctrl Pts',(13.8737311320789,44.8429890267007,0.));
#93804=CARTESIAN_POINT('Ctrl Pts',(13.8737311320789,44.8429890267007,20.));
#93805=CARTESIAN_POINT('Ctrl Pts',(13.9043197247138,44.8303923176691,0.));
#93806=CARTESIAN_POINT('Ctrl Pts',(13.9043197247138,44.8303923176691,20.));
#93807=CARTESIAN_POINT('Ctrl Pts',(13.9348984359903,44.8177745671945,0.));
#93808=CARTESIAN_POINT('Ctrl Pts',(13.9348984359903,44.8177745671945,20.));
#93809=CARTESIAN_POINT('Ctrl Pts',(13.9654672511774,44.8051357823031,0.));
#93810=CARTESIAN_POINT('Ctrl Pts',(13.9654672511774,44.8051357823031,20.));
#93811=CARTESIAN_POINT('Ctrl Pts',(13.9960261555481,44.7924759700314,0.));
#93812=CARTESIAN_POINT('Ctrl Pts',(13.9960261555481,44.7924759700314,20.));
#93813=CARTESIAN_POINT('Ctrl Pts',(14.0265751343805,44.7797951374262,0.));
#93814=CARTESIAN_POINT('Ctrl Pts',(14.0265751343805,44.7797951374262,20.));
#93815=CARTESIAN_POINT('Ctrl Pts',(14.057114172957,44.7670932915455,0.));
#93816=CARTESIAN_POINT('Ctrl Pts',(14.057114172957,44.7670932915455,20.));
#93817=CARTESIAN_POINT('Ctrl Pts',(14.0876432565649,44.7543704394583,0.));
#93818=CARTESIAN_POINT('Ctrl Pts',(14.0876432565649,44.7543704394583,20.));
#93819=CARTESIAN_POINT('Ctrl Pts',(14.118162370496,44.7416265882443,0.));
#93820=CARTESIAN_POINT('Ctrl Pts',(14.118162370496,44.7416265882443,20.));
#93821=CARTESIAN_POINT('Ctrl Pts',(14.1486715000464,44.728861744993,0.));
#93822=CARTESIAN_POINT('Ctrl Pts',(14.1486715000464,44.728861744993,20.));
#93823=CARTESIAN_POINT('Ctrl Pts',(14.1791706305171,44.7160759168044,0.));
#93824=CARTESIAN_POINT('Ctrl Pts',(14.1791706305171,44.7160759168044,20.));
#93825=CARTESIAN_POINT('Ctrl Pts',(14.2096597472134,44.7032691107881,0.));
#93826=CARTESIAN_POINT('Ctrl Pts',(14.2096597472134,44.7032691107881,20.));
#93827=CARTESIAN_POINT('Ctrl Pts',(14.2401388354454,44.690441334065,0.));
#93828=CARTESIAN_POINT('Ctrl Pts',(14.2401388354454,44.690441334065,20.));
#93829=CARTESIAN_POINT('Ctrl Pts',(14.2706078805279,44.6775925937661,0.));
#93830=CARTESIAN_POINT('Ctrl Pts',(14.2706078805279,44.6775925937661,20.));
#93831=CARTESIAN_POINT('Ctrl Pts',(14.3010668677802,44.6647228970333,0.));
#93832=CARTESIAN_POINT('Ctrl Pts',(14.3010668677802,44.6647228970333,20.));
#93833=CARTESIAN_POINT('Ctrl Pts',(14.3315157825264,44.6518322510194,0.));
#93834=CARTESIAN_POINT('Ctrl Pts',(14.3315157825264,44.6518322510194,20.));
#93835=CARTESIAN_POINT('Ctrl Pts',(14.3619546100951,44.6389206628876,0.));
#93836=CARTESIAN_POINT('Ctrl Pts',(14.3619546100951,44.6389206628876,20.));
#93837=CARTESIAN_POINT('Ctrl Pts',(14.3923833358197,44.6259881398119,0.));
#93838=CARTESIAN_POINT('Ctrl Pts',(14.3923833358197,44.6259881398119,20.));
#93839=CARTESIAN_POINT('Ctrl Pts',(14.4228019450383,44.613034688977,0.));
#93840=CARTESIAN_POINT('Ctrl Pts',(14.4228019450383,44.613034688977,20.));
#93841=CARTESIAN_POINT('Ctrl Pts',(14.4532104230936,44.6000603175775,0.));
#93842=CARTESIAN_POINT('Ctrl Pts',(14.4532104230936,44.6000603175775,20.));
#93843=CARTESIAN_POINT('Ctrl Pts',(14.4836087553332,44.5870650328188,0.));
#93844=CARTESIAN_POINT('Ctrl Pts',(14.4836087553332,44.5870650328188,20.));
#93845=CARTESIAN_POINT('Ctrl Pts',(14.5139969271087,44.5740488419152,0.));
#93846=CARTESIAN_POINT('Ctrl Pts',(14.5139969271087,44.5740488419152,20.));
#93847=CARTESIAN_POINT('Ctrl Pts',(14.5443749237767,44.5610117520915,0.));
#93848=CARTESIAN_POINT('Ctrl Pts',(14.5443749237767,44.5610117520915,20.));
#93849=CARTESIAN_POINT('Ctrl Pts',(14.5747427306988,44.5479537705835,0.));
#93850=CARTESIAN_POINT('Ctrl Pts',(14.5747427306988,44.5479537705835,20.));
#93851=CARTESIAN_POINT('Ctrl Pts',(14.6051003332411,44.5348749046379,0.));
#93852=CARTESIAN_POINT('Ctrl Pts',(14.6051003332411,44.5348749046379,20.));
#93853=CARTESIAN_POINT('Ctrl Pts',(14.6354477167742,44.521775161512,0.));
#93854=CARTESIAN_POINT('Ctrl Pts',(14.6354477167742,44.521775161512,20.));
#93855=CARTESIAN_POINT('Ctrl Pts',(14.6657848666743,44.5086545484757,0.));
#93856=CARTESIAN_POINT('Ctrl Pts',(14.6657848666743,44.5086545484757,20.));
#93857=CARTESIAN_POINT('Ctrl Pts',(14.6961117683217,44.4955130728078,0.));
#93858=CARTESIAN_POINT('Ctrl Pts',(14.6961117683217,44.4955130728078,20.));
#93859=CARTESIAN_POINT('Ctrl Pts',(14.7264284071013,44.4823507417973,0.));
#93860=CARTESIAN_POINT('Ctrl Pts',(14.7264284071013,44.4823507417973,20.));
#93861=CARTESIAN_POINT('Ctrl Pts',(14.7567347684029,44.469167562743,0.));
#93862=CARTESIAN_POINT('Ctrl Pts',(14.7567347684029,44.469167562743,20.));
#93863=CARTESIAN_POINT('Ctrl Pts',(14.7870308376214,44.4559635429545,0.));
#93864=CARTESIAN_POINT('Ctrl Pts',(14.7870308376214,44.4559635429545,20.));
#93865=CARTESIAN_POINT('Ctrl Pts',(14.817316600156,44.4427386897515,0.));
#93866=CARTESIAN_POINT('Ctrl Pts',(14.817316600156,44.4427386897515,20.));
#93867=CARTESIAN_POINT('Ctrl Pts',(14.8475920414107,44.4294930104636,0.));
#93868=CARTESIAN_POINT('Ctrl Pts',(14.8475920414107,44.4294930104636,20.));
#93869=CARTESIAN_POINT('Ctrl Pts',(14.8778571467943,44.416226512431,0.));
#93870=CARTESIAN_POINT('Ctrl Pts',(14.8778571467943,44.416226512431,20.));
#93871=CARTESIAN_POINT('Ctrl Pts',(14.9081119017199,44.4029392030043,0.));
#93872=CARTESIAN_POINT('Ctrl Pts',(14.9081119017199,44.4029392030043,20.));
#93873=CARTESIAN_POINT('Ctrl Pts',(14.9383562916061,44.389631089546,0.));
#93874=CARTESIAN_POINT('Ctrl Pts',(14.9383562916061,44.389631089546,20.));
#93875=CARTESIAN_POINT('Ctrl Pts',(14.9685903018767,44.3763021794296,0.));
#93876=CARTESIAN_POINT('Ctrl Pts',(14.9685903018767,44.3763021794296,20.));
#93877=CARTESIAN_POINT('Ctrl Pts',(14.9988139179602,44.3629524800397,0.));
#93878=CARTESIAN_POINT('Ctrl Pts',(14.9988139179602,44.3629524800397,20.));
#93879=CARTESIAN_POINT('Ctrl Pts',(15.0290271252899,44.3495819987708,0.));
#93880=CARTESIAN_POINT('Ctrl Pts',(15.0290271252899,44.3495819987708,20.));
#93881=CARTESIAN_POINT('Ctrl Pts',(15.0592299093032,44.3361907430254,0.));
#93882=CARTESIAN_POINT('Ctrl Pts',(15.0592299093032,44.3361907430254,20.));
#93883=CARTESIAN_POINT('Ctrl Pts',(15.0894222554424,44.3227787202166,0.));
#93884=CARTESIAN_POINT('Ctrl Pts',(15.0894222554424,44.3227787202166,20.));
#93885=CARTESIAN_POINT('Ctrl Pts',(15.1196041491546,44.3093459377674,0.));
#93886=CARTESIAN_POINT('Ctrl Pts',(15.1196041491546,44.3093459377674,20.));
#93887=CARTESIAN_POINT('Ctrl Pts',(15.1497755758917,44.2958924031118,0.));
#93888=CARTESIAN_POINT('Ctrl Pts',(15.1497755758917,44.2958924031118,20.));
#93889=CARTESIAN_POINT('Ctrl Pts',(15.1799365211113,44.2824181236961,0.));
#93890=CARTESIAN_POINT('Ctrl Pts',(15.1799365211113,44.2824181236961,20.));
#93891=CARTESIAN_POINT('Ctrl Pts',(15.2100869702755,44.2689231069767,0.));
#93892=CARTESIAN_POINT('Ctrl Pts',(15.2100869702755,44.2689231069767,20.));
#93893=CARTESIAN_POINT('Ctrl Pts',(15.2402269088514,44.2554073604206,0.));
#93894=CARTESIAN_POINT('Ctrl Pts',(15.2402269088514,44.2554073604206,20.));
#93895=CARTESIAN_POINT('Ctrl Pts',(15.2703563223108,44.2418708915045,0.));
#93896=CARTESIAN_POINT('Ctrl Pts',(15.2703563223108,44.2418708915045,20.));
#93897=CARTESIAN_POINT('Ctrl Pts',(15.30047519613,44.2283137077152,0.));
#93898=CARTESIAN_POINT('Ctrl Pts',(15.30047519613,44.2283137077152,20.));
#93899=CARTESIAN_POINT('Ctrl Pts',(15.3305835157903,44.2147358165492,0.));
#93900=CARTESIAN_POINT('Ctrl Pts',(15.3305835157903,44.2147358165492,20.));
#93901=CARTESIAN_POINT('Ctrl Pts',(15.3606812667781,44.201137225514,0.));
#93902=CARTESIAN_POINT('Ctrl Pts',(15.3606812667781,44.201137225514,20.));
#93903=CARTESIAN_POINT('Ctrl Pts',(15.390768434585,44.1875179421286,0.));
#93904=CARTESIAN_POINT('Ctrl Pts',(15.390768434585,44.1875179421286,20.));
#93905=CARTESIAN_POINT('Ctrl Pts',(15.4208450047077,44.1738779739225,0.));
#93906=CARTESIAN_POINT('Ctrl Pts',(15.4208450047077,44.1738779739225,20.));
#93907=CARTESIAN_POINT('Ctrl Pts',(15.4509109626472,44.1602173284345,0.));
#93908=CARTESIAN_POINT('Ctrl Pts',(15.4509109626472,44.1602173284345,20.));
#93909=CARTESIAN_POINT('Ctrl Pts',(15.4809662939093,44.146536013213,0.));
#93910=CARTESIAN_POINT('Ctrl Pts',(15.4809662939093,44.146536013213,20.));
#93911=CARTESIAN_POINT('Ctrl Pts',(15.5110109840047,44.1328340358171,0.));
#93912=CARTESIAN_POINT('Ctrl Pts',(15.5110109840047,44.1328340358171,20.));
#93913=CARTESIAN_POINT('Ctrl Pts',(15.5410450184494,44.1191114038164,0.));
#93914=CARTESIAN_POINT('Ctrl Pts',(15.5410450184494,44.1191114038164,20.));
#93915=CARTESIAN_POINT('Ctrl Pts',(15.5710683827645,44.1053681247921,0.));
#93916=CARTESIAN_POINT('Ctrl Pts',(15.5710683827645,44.1053681247921,20.));
#93917=CARTESIAN_POINT('Ctrl Pts',(15.6010810624766,44.0916042063371,0.));
#93918=CARTESIAN_POINT('Ctrl Pts',(15.6010810624766,44.0916042063371,20.));
#93919=CARTESIAN_POINT('Ctrl Pts',(15.6310830431167,44.0778196560536,0.));
#93920=CARTESIAN_POINT('Ctrl Pts',(15.6310830431167,44.0778196560536,20.));
#93921=CARTESIAN_POINT('Ctrl Pts',(15.6610743102207,44.0640144815534,0.));
#93922=CARTESIAN_POINT('Ctrl Pts',(15.6610743102207,44.0640144815534,20.));
#93923=CARTESIAN_POINT('Ctrl Pts',(15.6910548493288,44.050188690457,0.));
#93924=CARTESIAN_POINT('Ctrl Pts',(15.6910548493288,44.050188690457,20.));
#93925=CARTESIAN_POINT('Ctrl Pts',(15.7210246459867,44.0363422903955,0.));
#93926=CARTESIAN_POINT('Ctrl Pts',(15.7210246459867,44.0363422903955,20.));
#93927=CARTESIAN_POINT('Ctrl Pts',(15.7509836857452,44.0224752890112,0.));
#93928=CARTESIAN_POINT('Ctrl Pts',(15.7509836857452,44.0224752890112,20.));
#93929=CARTESIAN_POINT('Ctrl Pts',(15.7809319541601,44.0085876939576,0.));
#93930=CARTESIAN_POINT('Ctrl Pts',(15.7809319541601,44.0085876939576,20.));
#93931=CARTESIAN_POINT('Ctrl Pts',(15.8108694367927,43.9946795128988,0.));
#93932=CARTESIAN_POINT('Ctrl Pts',(15.8108694367927,43.9946795128988,20.));
#93933=CARTESIAN_POINT('Ctrl Pts',(15.8407961192089,43.9807507535097,0.));
#93934=CARTESIAN_POINT('Ctrl Pts',(15.8407961192089,43.9807507535097,20.));
#93935=CARTESIAN_POINT('Ctrl Pts',(15.8707119869797,43.9668014234746,0.));
#93936=CARTESIAN_POINT('Ctrl Pts',(15.8707119869797,43.9668014234746,20.));
#93937=CARTESIAN_POINT('Ctrl Pts',(15.9006170256808,43.9528315304878,0.));
#93938=CARTESIAN_POINT('Ctrl Pts',(15.9006170256808,43.9528315304878,20.));
#93939=CARTESIAN_POINT('Ctrl Pts',(15.9305112208934,43.9388410822542,0.));
#93940=CARTESIAN_POINT('Ctrl Pts',(15.9305112208934,43.9388410822542,20.));
#93941=CARTESIAN_POINT('Ctrl Pts',(15.9603945582034,43.9248300864889,0.));
#93942=CARTESIAN_POINT('Ctrl Pts',(15.9603945582034,43.9248300864889,20.));
#93943=CARTESIAN_POINT('Ctrl Pts',(15.9902670232019,43.9107985509168,0.));
#93944=CARTESIAN_POINT('Ctrl Pts',(15.9902670232019,43.9107985509168,20.));
#93945=CARTESIAN_POINT('Ctrl Pts',(16.0201286014849,43.896746483274,0.));
#93946=CARTESIAN_POINT('Ctrl Pts',(16.0201286014849,43.896746483274,20.));
#93947=CARTESIAN_POINT('Ctrl Pts',(16.0499792786541,43.8826738913074,0.));
#93948=CARTESIAN_POINT('Ctrl Pts',(16.0499792786541,43.8826738913074,20.));
#93949=CARTESIAN_POINT('Ctrl Pts',(16.0798190403159,43.8685807827745,0.));
#93950=CARTESIAN_POINT('Ctrl Pts',(16.0798190403159,43.8685807827745,20.));
#93951=CARTESIAN_POINT('Ctrl Pts',(16.1096478720818,43.854467165442,0.));
#93952=CARTESIAN_POINT('Ctrl Pts',(16.1096478720818,43.854467165442,20.));
#93953=CARTESIAN_POINT('Ctrl Pts',(16.1394657595683,43.8403330470868,0.));
#93954=CARTESIAN_POINT('Ctrl Pts',(16.1394657595683,43.8403330470868,20.));
#93955=CARTESIAN_POINT('Ctrl Pts',(16.1692726883968,43.8261784354962,0.));
#93956=CARTESIAN_POINT('Ctrl Pts',(16.1692726883968,43.8261784354962,20.));
#93957=CARTESIAN_POINT('Ctrl Pts',(16.199068644194,43.8120033384679,0.));
#93958=CARTESIAN_POINT('Ctrl Pts',(16.199068644194,43.8120033384679,20.));
#93959=CARTESIAN_POINT('Ctrl Pts',(16.2288536125916,43.7978077638098,0.));
#93960=CARTESIAN_POINT('Ctrl Pts',(16.2288536125916,43.7978077638098,20.));
#93961=CARTESIAN_POINT('Ctrl Pts',(16.2586275792268,43.7835917193404,0.));
#93962=CARTESIAN_POINT('Ctrl Pts',(16.2586275792268,43.7835917193404,20.));
#93963=CARTESIAN_POINT('Ctrl Pts',(16.2883905297415,43.7693552128887,0.));
#93964=CARTESIAN_POINT('Ctrl Pts',(16.2883905297415,43.7693552128887,20.));
#93965=CARTESIAN_POINT('Ctrl Pts',(16.3181424497834,43.7550982522947,0.));
#93966=CARTESIAN_POINT('Ctrl Pts',(16.3181424497834,43.7550982522947,20.));
#93967=CARTESIAN_POINT('Ctrl Pts',(16.3478833250055,43.7408208454089,0.));
#93968=CARTESIAN_POINT('Ctrl Pts',(16.3478833250055,43.7408208454089,20.));
#93969=CARTESIAN_POINT('Ctrl Pts',(16.3776131410651,43.7265230000909,0.));
#93970=CARTESIAN_POINT('Ctrl Pts',(16.3776131410651,43.7265230000909,20.));
#93971=CARTESIAN_POINT('Ctrl Pts',(16.4073318836249,43.7122047242097,0.));
#93972=CARTESIAN_POINT('Ctrl Pts',(16.4073318836249,43.7122047242097,20.));
#93973=CARTESIAN_POINT('Ctrl Pts',(16.4370395383523,43.6978660256455,0.));
#93974=CARTESIAN_POINT('Ctrl Pts',(16.4370395383523,43.6978660256455,20.));
#93975=CARTESIAN_POINT('Ctrl Pts',(16.4667360909206,43.6835069122887,0.));
#93976=CARTESIAN_POINT('Ctrl Pts',(16.4667360909206,43.6835069122887,20.));
#93977=CARTESIAN_POINT('Ctrl Pts',(16.4964215270082,43.6691273920409,0.));
#93978=CARTESIAN_POINT('Ctrl Pts',(16.4964215270082,43.6691273920409,20.));
#93979=CARTESIAN_POINT('Ctrl Pts',(16.5260958322991,43.6547274728139,0.));
#93980=CARTESIAN_POINT('Ctrl Pts',(16.5260958322991,43.6547274728139,20.));
#93981=CARTESIAN_POINT('Ctrl Pts',(16.5557589924819,43.640307162529,0.));
#93982=CARTESIAN_POINT('Ctrl Pts',(16.5557589924819,43.640307162529,20.));
#93983=CARTESIAN_POINT('Ctrl Pts',(16.5854109932504,43.6258664691173,0.));
#93984=CARTESIAN_POINT('Ctrl Pts',(16.5854109932504,43.6258664691173,20.));
#93985=CARTESIAN_POINT('Ctrl Pts',(16.6150518203036,43.6114054005208,0.));
#93986=CARTESIAN_POINT('Ctrl Pts',(16.6150518203036,43.6114054005208,20.));
#93987=CARTESIAN_POINT('Ctrl Pts',(16.6446814593458,43.5969239646926,0.));
#93988=CARTESIAN_POINT('Ctrl Pts',(16.6446814593458,43.5969239646926,20.));
#93989=CARTESIAN_POINT('Ctrl Pts',(16.6742998960869,43.5824221695961,0.));
#93990=CARTESIAN_POINT('Ctrl Pts',(16.6742998960869,43.5824221695961,20.));
#93991=CARTESIAN_POINT('Ctrl Pts',(16.7039071162413,43.5679000232041,0.));
#93992=CARTESIAN_POINT('Ctrl Pts',(16.7039071162413,43.5679000232041,20.));
#93993=CARTESIAN_POINT('Ctrl Pts',(16.7335031055294,43.5533575334996,0.));
#93994=CARTESIAN_POINT('Ctrl Pts',(16.7335031055294,43.5533575334996,20.));
#93995=CARTESIAN_POINT('Ctrl Pts',(16.7630878496767,43.5387947084755,0.));
#93996=CARTESIAN_POINT('Ctrl Pts',(16.7630878496767,43.5387947084755,20.));
#93997=CARTESIAN_POINT('Ctrl Pts',(16.792661334414,43.5242115561352,0.));
#93998=CARTESIAN_POINT('Ctrl Pts',(16.792661334414,43.5242115561352,20.));
#93999=CARTESIAN_POINT('Ctrl Pts',(16.8222235454772,43.5096080844922,0.));
#94000=CARTESIAN_POINT('Ctrl Pts',(16.8222235454772,43.5096080844922,20.));
#94001=CARTESIAN_POINT('Ctrl Pts',(16.8517744686076,43.4949843015709,0.));
#94002=CARTESIAN_POINT('Ctrl Pts',(16.8517744686076,43.4949843015709,20.));
#94003=CARTESIAN_POINT('Ctrl Pts',(16.8813140895513,43.4803402154062,0.));
#94004=CARTESIAN_POINT('Ctrl Pts',(16.8813140895513,43.4803402154062,20.));
#94005=CARTESIAN_POINT('Ctrl Pts',(16.91084239406,43.4656758340435,0.));
#94006=CARTESIAN_POINT('Ctrl Pts',(16.91084239406,43.4656758340435,20.));
#94007=CARTESIAN_POINT('Ctrl Pts',(16.9403593678908,43.4509911655382,0.));
#94008=CARTESIAN_POINT('Ctrl Pts',(16.9403593678908,43.4509911655382,20.));
#94009=CARTESIAN_POINT('Ctrl Pts',(16.9698649968061,43.4362862179557,0.));
#94010=CARTESIAN_POINT('Ctrl Pts',(16.9698649968061,43.4362862179557,20.));
#94011=CARTESIAN_POINT('Ctrl Pts',(16.9993592665737,43.4215609993712,0.));
#94012=CARTESIAN_POINT('Ctrl Pts',(16.9993592665737,43.4215609993712,20.));
#94013=CARTESIAN_POINT('Ctrl Pts',(17.0288421629666,43.4068155178696,0.));
#94014=CARTESIAN_POINT('Ctrl Pts',(17.0288421629666,43.4068155178696,20.));
#94015=CARTESIAN_POINT('Ctrl Pts',(17.0583136717632,43.3920497815463,0.));
#94016=CARTESIAN_POINT('Ctrl Pts',(17.0583136717632,43.3920497815463,20.));
#94017=CARTESIAN_POINT('Ctrl Pts',(17.0877737787472,43.3772637985072,0.));
#94018=CARTESIAN_POINT('Ctrl Pts',(17.0877737787472,43.3772637985072,20.));
#94019=CARTESIAN_POINT('Ctrl Pts',(17.1172224697079,43.3624575768695,0.));
#94020=CARTESIAN_POINT('Ctrl Pts',(17.1172224697079,43.3624575768695,20.));
#94021=CARTESIAN_POINT('Ctrl Pts',(17.1466597304397,43.3476311247602,0.));
#94022=CARTESIAN_POINT('Ctrl Pts',(17.1466597304397,43.3476311247602,20.));
#94023=CARTESIAN_POINT('Ctrl Pts',(17.1760855467426,43.332784450317,0.));
#94024=CARTESIAN_POINT('Ctrl Pts',(17.1760855467426,43.332784450317,20.));
#94025=CARTESIAN_POINT('Ctrl Pts',(17.2054999044212,43.3179175616862,0.));
#94026=CARTESIAN_POINT('Ctrl Pts',(17.2054999044212,43.3179175616862,20.));
#94027=CARTESIAN_POINT('Ctrl Pts',(17.2349027892859,43.3030304670242,0.));
#94028=CARTESIAN_POINT('Ctrl Pts',(17.2349027892859,43.3030304670242,20.));
#94029=CARTESIAN_POINT('Ctrl Pts',(17.2642941871522,43.2881231744974,0.));
#94030=CARTESIAN_POINT('Ctrl Pts',(17.2642941871522,43.2881231744974,20.));
#94031=CARTESIAN_POINT('Ctrl Pts',(17.2936740838416,43.2731956922839,0.));
#94032=CARTESIAN_POINT('Ctrl Pts',(17.2936740838416,43.2731956922839,20.));
#94033=CARTESIAN_POINT('Ctrl Pts',(17.3230424651811,43.258248028572,0.));
#94034=CARTESIAN_POINT('Ctrl Pts',(17.3230424651811,43.258248028572,20.));
#94035=CARTESIAN_POINT('Ctrl Pts',(17.352399317003,43.2432801915607,0.));
#94036=CARTESIAN_POINT('Ctrl Pts',(17.352399317003,43.2432801915607,20.));
#94037=CARTESIAN_POINT('Ctrl Pts',(17.3817446251452,43.2282921894589,0.));
#94038=CARTESIAN_POINT('Ctrl Pts',(17.3817446251452,43.2282921894589,20.));
#94039=CARTESIAN_POINT('Ctrl Pts',(17.4110783754507,43.2132840304854,0.));
#94040=CARTESIAN_POINT('Ctrl Pts',(17.4110783754507,43.2132840304854,20.));
#94041=CARTESIAN_POINT('Ctrl Pts',(17.4404005537678,43.1982557228684,0.));
#94042=CARTESIAN_POINT('Ctrl Pts',(17.4404005537678,43.1982557228684,20.));
#94043=CARTESIAN_POINT('Ctrl Pts',(17.46971114595,43.1832072748459,0.));
#94044=CARTESIAN_POINT('Ctrl Pts',(17.46971114595,43.1832072748459,20.));
#94045=CARTESIAN_POINT('Ctrl Pts',(17.4990101378563,43.1681386946662,0.));
#94046=CARTESIAN_POINT('Ctrl Pts',(17.4990101378563,43.1681386946662,20.));
#94047=CARTESIAN_POINT('Ctrl Pts',(17.5282975153509,43.1530499905879,0.));
#94048=CARTESIAN_POINT('Ctrl Pts',(17.5282975153509,43.1530499905879,20.));
#94049=CARTESIAN_POINT('Ctrl Pts',(17.557573264304,43.1379411708804,0.));
#94050=CARTESIAN_POINT('Ctrl Pts',(17.557573264304,43.1379411708804,20.));
#94051=CARTESIAN_POINT('Ctrl Pts',(17.5868373705916,43.122812243824,0.));
#94052=CARTESIAN_POINT('Ctrl Pts',(17.5868373705916,43.122812243824,20.));
#94053=CARTESIAN_POINT('Ctrl Pts',(17.6160898200949,43.1076632177089,0.));
#94054=CARTESIAN_POINT('Ctrl Pts',(17.6160898200949,43.1076632177089,20.));
#94055=CARTESIAN_POINT('Ctrl Pts',(17.645330598701,43.0924941008354,0.));
#94056=CARTESIAN_POINT('Ctrl Pts',(17.645330598701,43.0924941008354,20.));
#94057=CARTESIAN_POINT('Ctrl Pts',(17.674559692302,43.0773049015137,0.));
#94058=CARTESIAN_POINT('Ctrl Pts',(17.674559692302,43.0773049015137,20.));
#94059=CARTESIAN_POINT('Ctrl Pts',(17.7037770867956,43.0620956280638,0.));
#94060=CARTESIAN_POINT('Ctrl Pts',(17.7037770867956,43.0620956280638,20.));
#94061=CARTESIAN_POINT('Ctrl Pts',(17.7329827680846,43.0468662888157,0.));
#94062=CARTESIAN_POINT('Ctrl Pts',(17.7329827680846,43.0468662888157,20.));
#94063=CARTESIAN_POINT('Ctrl Pts',(17.7621767220773,43.0316168921093,0.));
#94064=CARTESIAN_POINT('Ctrl Pts',(17.7621767220773,43.0316168921093,20.));
#94065=CARTESIAN_POINT('Ctrl Pts',(17.7913589346876,43.0163474462951,0.));
#94066=CARTESIAN_POINT('Ctrl Pts',(17.7913589346876,43.0163474462951,20.));
#94067=CARTESIAN_POINT('Ctrl Pts',(17.8205293918351,43.0010579597341,0.));
#94068=CARTESIAN_POINT('Ctrl Pts',(17.8205293918351,43.0010579597341,20.));
#94069=CARTESIAN_POINT('Ctrl Pts',(17.8496880794454,42.985748440798,0.));
#94070=CARTESIAN_POINT('Ctrl Pts',(17.8496880794454,42.985748440798,20.));
#94071=CARTESIAN_POINT('Ctrl Pts',(17.8788349834491,42.9704188978681,0.));
#94072=CARTESIAN_POINT('Ctrl Pts',(17.8788349834491,42.9704188978681,20.));
#94073=CARTESIAN_POINT('Ctrl Pts',(17.9079700897828,42.9550693393359,0.));
#94074=CARTESIAN_POINT('Ctrl Pts',(17.9079700897828,42.9550693393359,20.));
#94075=CARTESIAN_POINT('Ctrl Pts',(17.9370933843882,42.9396997736018,0.));
#94076=CARTESIAN_POINT('Ctrl Pts',(17.9370933843882,42.9396997736018,20.));
#94077=CARTESIAN_POINT('Ctrl Pts',(17.9662048532126,42.9243102090766,0.));
#94078=CARTESIAN_POINT('Ctrl Pts',(17.9662048532126,42.9243102090766,20.));
#94079=CARTESIAN_POINT('Ctrl Pts',(17.9953044822088,42.9089006541818,0.));
#94080=CARTESIAN_POINT('Ctrl Pts',(17.9953044822088,42.9089006541818,20.));
#94081=CARTESIAN_POINT('Ctrl Pts',(18.0243922573354,42.8934711173491,0.));
#94082=CARTESIAN_POINT('Ctrl Pts',(18.0243922573354,42.8934711173491,20.));
#94083=CARTESIAN_POINT('Ctrl Pts',(18.0534681645565,42.8780216070205,0.));
#94084=CARTESIAN_POINT('Ctrl Pts',(18.0534681645565,42.8780216070205,20.));
#94085=CARTESIAN_POINT('Ctrl Pts',(18.0825321898416,42.8625521316489,0.));
#94086=CARTESIAN_POINT('Ctrl Pts',(18.0825321898416,42.8625521316489,20.));
#94087=CARTESIAN_POINT('Ctrl Pts',(18.1115843191668,42.8470626996976,0.));
#94088=CARTESIAN_POINT('Ctrl Pts',(18.1115843191668,42.8470626996976,20.));
#94089=CARTESIAN_POINT('Ctrl Pts',(18.1406245385131,42.831553319639,0.));
#94090=CARTESIAN_POINT('Ctrl Pts',(18.1406245385131,42.831553319639,20.));
#94091=CARTESIAN_POINT('Ctrl Pts',(18.1696528338673,42.8160239999555,0.));
#94092=CARTESIAN_POINT('Ctrl Pts',(18.1696528338673,42.8160239999555,20.));
#94093=CARTESIAN_POINT('Ctrl Pts',(18.1986691912208,42.8004747491375,0.));
#94094=CARTESIAN_POINT('Ctrl Pts',(18.1986691912208,42.8004747491375,20.));
#94095=CARTESIAN_POINT('Ctrl Pts',(18.2276735965714,42.7849055756869,0.));
#94096=CARTESIAN_POINT('Ctrl Pts',(18.2276735965714,42.7849055756869,20.));
#94097=CARTESIAN_POINT('Ctrl Pts',(18.256666035922,42.7693164881155,0.));
#94098=CARTESIAN_POINT('Ctrl Pts',(18.256666035922,42.7693164881155,20.));
#94099=CARTESIAN_POINT('Ctrl Pts',(18.285646495282,42.7537074949463,0.));
#94100=CARTESIAN_POINT('Ctrl Pts',(18.285646495282,42.7537074949463,20.));
#94101=CARTESIAN_POINT('Ctrl Pts',(18.3146149606662,42.7380786047127,0.));
#94102=CARTESIAN_POINT('Ctrl Pts',(18.3146149606662,42.7380786047127,20.));
#94103=CARTESIAN_POINT('Ctrl Pts',(18.3435714180954,42.7224298259587,0.));
#94104=CARTESIAN_POINT('Ctrl Pts',(18.3435714180954,42.7224298259587,20.));
#94105=CARTESIAN_POINT('Ctrl Pts',(18.372515853596,42.7067611672378,0.));
#94106=CARTESIAN_POINT('Ctrl Pts',(18.372515853596,42.7067611672378,20.));
#94107=CARTESIAN_POINT('Ctrl Pts',(18.4014482531999,42.6910726371132,0.));
#94108=CARTESIAN_POINT('Ctrl Pts',(18.4014482531999,42.6910726371132,20.));
#94109=CARTESIAN_POINT('Ctrl Pts',(18.4303686029443,42.6753642441576,0.));
#94110=CARTESIAN_POINT('Ctrl Pts',(18.4303686029443,42.6753642441576,20.));
#94111=CARTESIAN_POINT('Ctrl Pts',(18.4592768888724,42.6596359969538,0.));
#94112=CARTESIAN_POINT('Ctrl Pts',(18.4592768888724,42.6596359969538,20.));
#94113=CARTESIAN_POINT('Ctrl Pts',(18.4881730970326,42.6438879040941,0.));
#94114=CARTESIAN_POINT('Ctrl Pts',(18.4881730970326,42.6438879040941,20.));
#94115=CARTESIAN_POINT('Ctrl Pts',(18.5170572134793,42.6281199741818,0.));
#94116=CARTESIAN_POINT('Ctrl Pts',(18.5170572134793,42.6281199741818,20.));
#94117=CARTESIAN_POINT('Ctrl Pts',(18.5459292242727,42.61233221583,0.));
#94118=CARTESIAN_POINT('Ctrl Pts',(18.5459292242727,42.61233221583,20.));
#94119=CARTESIAN_POINT('Ctrl Pts',(18.574789115479,42.596524637663,0.));
#94120=CARTESIAN_POINT('Ctrl Pts',(18.574789115479,42.596524637663,20.));
#94121=CARTESIAN_POINT('Ctrl Pts',(18.6036368731702,42.5806972483146,0.));
#94122=CARTESIAN_POINT('Ctrl Pts',(18.6036368731702,42.5806972483146,20.));
#94123=CARTESIAN_POINT('Ctrl Pts',(18.6324724834239,42.5648500564287,0.));
#94124=CARTESIAN_POINT('Ctrl Pts',(18.6324724834239,42.5648500564287,20.));
#94125=CARTESIAN_POINT('Ctrl Pts',(18.6612959323233,42.5489830706585,0.));
#94126=CARTESIAN_POINT('Ctrl Pts',(18.6612959323233,42.5489830706585,20.));
#94127=CARTESIAN_POINT('Ctrl Pts',(18.6901072059567,42.5330962996668,0.));
#94128=CARTESIAN_POINT('Ctrl Pts',(18.6901072059567,42.5330962996668,20.));
#94129=CARTESIAN_POINT('Ctrl Pts',(18.718906290419,42.517189752127,0.));
#94130=CARTESIAN_POINT('Ctrl Pts',(18.718906290419,42.517189752127,20.));
#94131=CARTESIAN_POINT('Ctrl Pts',(18.7476931718101,42.5012634367222,0.));
#94132=CARTESIAN_POINT('Ctrl Pts',(18.7476931718101,42.5012634367222,20.));
#94133=CARTESIAN_POINT('Ctrl Pts',(18.7764678362367,42.4853173621469,0.));
#94134=CARTESIAN_POINT('Ctrl Pts',(18.7764678362367,42.4853173621469,20.));
#94135=CARTESIAN_POINT('Ctrl Pts',(18.8052302698113,42.4693515371059,0.));
#94136=CARTESIAN_POINT('Ctrl Pts',(18.8052302698113,42.4693515371059,20.));
#94137=CARTESIAN_POINT('Ctrl Pts',(18.8339804586522,42.4533659703145,0.));
#94138=CARTESIAN_POINT('Ctrl Pts',(18.8339804586522,42.4533659703145,20.));
#94139=CARTESIAN_POINT('Ctrl Pts',(18.8627183888827,42.4373606704956,0.));
#94140=CARTESIAN_POINT('Ctrl Pts',(18.8627183888827,42.4373606704956,20.));
#94141=CARTESIAN_POINT('Ctrl Pts',(18.8914440466322,42.4213356463824,0.));
#94142=CARTESIAN_POINT('Ctrl Pts',(18.8914440466322,42.4213356463824,20.));
#94143=CARTESIAN_POINT('Ctrl Pts',(18.9201574180352,42.4052909067172,0.));
#94144=CARTESIAN_POINT('Ctrl Pts',(18.9201574180352,42.4052909067172,20.));
#94145=CARTESIAN_POINT('Ctrl Pts',(18.9488584892326,42.389226460254,0.));
#94146=CARTESIAN_POINT('Ctrl Pts',(18.9488584892326,42.389226460254,20.));
#94147=CARTESIAN_POINT('Ctrl Pts',(18.9775472463711,42.3731423157568,0.));
#94148=CARTESIAN_POINT('Ctrl Pts',(18.9775472463711,42.3731423157568,20.));
#94149=CARTESIAN_POINT('Ctrl Pts',(19.0062236756035,42.3570384820003,0.));
#94150=CARTESIAN_POINT('Ctrl Pts',(19.0062236756035,42.3570384820003,20.));
#94151=CARTESIAN_POINT('Ctrl Pts',(19.0348877630887,42.3409149677685,0.));
#94152=CARTESIAN_POINT('Ctrl Pts',(19.0348877630887,42.3409149677685,20.));
#94153=CARTESIAN_POINT('Ctrl Pts',(19.0635394949913,42.3247717818558,0.));
#94154=CARTESIAN_POINT('Ctrl Pts',(19.0635394949913,42.3247717818558,20.));
#94155=CARTESIAN_POINT('Ctrl Pts',(19.0921788574819,42.3086089330658,0.));
#94156=CARTESIAN_POINT('Ctrl Pts',(19.0921788574819,42.3086089330658,20.));
#94157=CARTESIAN_POINT('Ctrl Pts',(19.1208058367362,42.2924264302113,0.));
#94158=CARTESIAN_POINT('Ctrl Pts',(19.1208058367362,42.2924264302113,20.));
#94159=CARTESIAN_POINT('Ctrl Pts',(19.1494204189361,42.2762242821163,0.));
#94160=CARTESIAN_POINT('Ctrl Pts',(19.1494204189361,42.2762242821163,20.));
#94161=CARTESIAN_POINT('Ctrl Pts',(19.1780225902694,42.2600024976146,0.));
#94162=CARTESIAN_POINT('Ctrl Pts',(19.1780225902694,42.2600024976146,20.));
#94163=CARTESIAN_POINT('Ctrl Pts',(19.2066123369297,42.2437610855506,0.));
#94164=CARTESIAN_POINT('Ctrl Pts',(19.2066123369297,42.2437610855506,20.));
#94165=CARTESIAN_POINT('Ctrl Pts',(19.2351896451166,42.2275000547783,0.));
#94166=CARTESIAN_POINT('Ctrl Pts',(19.2351896451166,42.2275000547783,20.));
#94167=CARTESIAN_POINT('Ctrl Pts',(19.2637545010356,42.2112194141618,0.));
#94168=CARTESIAN_POINT('Ctrl Pts',(19.2637545010356,42.2112194141618,20.));
#94169=CARTESIAN_POINT('Ctrl Pts',(19.2923068908981,42.1949191725745,0.));
#94170=CARTESIAN_POINT('Ctrl Pts',(19.2923068908981,42.1949191725745,20.));
#94171=CARTESIAN_POINT('Ctrl Pts',(19.3208468009211,42.1785993388989,0.));
#94172=CARTESIAN_POINT('Ctrl Pts',(19.3208468009211,42.1785993388989,20.));
#94173=CARTESIAN_POINT('Ctrl Pts',(19.3493742173282,42.1622599220289,0.));
#94174=CARTESIAN_POINT('Ctrl Pts',(19.3493742173282,42.1622599220289,20.));
#94175=CARTESIAN_POINT('Ctrl Pts',(19.377889126349,42.1459009308685,0.));
#94176=CARTESIAN_POINT('Ctrl Pts',(19.377889126349,42.1459009308685,20.));
#94177=CARTESIAN_POINT('Ctrl Pts',(19.4063915142187,42.1295223743319,0.));
#94178=CARTESIAN_POINT('Ctrl Pts',(19.4063915142187,42.1295223743319,20.));
#94179=CARTESIAN_POINT('Ctrl Pts',(19.4348813671784,42.1131242613432,0.));
#94180=CARTESIAN_POINT('Ctrl Pts',(19.4348813671784,42.1131242613432,20.));
#94181=CARTESIAN_POINT('Ctrl Pts',(19.4633586714748,42.0967066008354,0.));
#94182=CARTESIAN_POINT('Ctrl Pts',(19.4633586714748,42.0967066008354,20.));
#94183=CARTESIAN_POINT('Ctrl Pts',(19.4918234133604,42.080269401751,0.));
#94184=CARTESIAN_POINT('Ctrl Pts',(19.4918234133604,42.080269401751,20.));
#94185=CARTESIAN_POINT('Ctrl Pts',(19.5202755790939,42.0638126730426,0.));
#94186=CARTESIAN_POINT('Ctrl Pts',(19.5202755790939,42.0638126730426,20.));
#94187=CARTESIAN_POINT('Ctrl Pts',(19.5487151549408,42.0473364236742,0.));
#94188=CARTESIAN_POINT('Ctrl Pts',(19.5487151549408,42.0473364236742,20.));
#94189=CARTESIAN_POINT('Ctrl Pts',(19.5771421271718,42.0308406626191,0.));
#94190=CARTESIAN_POINT('Ctrl Pts',(19.5771421271718,42.0308406626191,20.));
#94191=CARTESIAN_POINT('Ctrl Pts',(19.6055564820642,42.0143253988608,0.));
#94192=CARTESIAN_POINT('Ctrl Pts',(19.6055564820642,42.0143253988608,20.));
#94193=CARTESIAN_POINT('Ctrl Pts',(19.6339582059008,41.997790641393,0.));
#94194=CARTESIAN_POINT('Ctrl Pts',(19.6339582059008,41.997790641393,20.));
#94195=CARTESIAN_POINT('Ctrl Pts',(19.6623472849704,41.9812363992182,0.));
#94196=CARTESIAN_POINT('Ctrl Pts',(19.6623472849704,41.9812363992182,20.));
#94197=CARTESIAN_POINT('Ctrl Pts',(19.6907237055674,41.9646626813489,0.));
#94198=CARTESIAN_POINT('Ctrl Pts',(19.6907237055674,41.9646626813489,20.));
#94199=CARTESIAN_POINT('Ctrl Pts',(19.7190874539927,41.9480694968077,0.));
#94200=CARTESIAN_POINT('Ctrl Pts',(19.7190874539927,41.9480694968077,20.));
#94201=CARTESIAN_POINT('Ctrl Pts',(19.7474385165531,41.9314568546275,0.));
#94202=CARTESIAN_POINT('Ctrl Pts',(19.7474385165531,41.9314568546275,20.));
#94203=CARTESIAN_POINT('Ctrl Pts',(19.7757768795619,41.9148247638512,0.));
#94204=CARTESIAN_POINT('Ctrl Pts',(19.7757768795619,41.9148247638512,20.));
#94205=CARTESIAN_POINT('Ctrl Pts',(19.8041025293385,41.8981732335313,0.));
#94206=CARTESIAN_POINT('Ctrl Pts',(19.8041025293385,41.8981732335313,20.));
#94207=CARTESIAN_POINT('Ctrl Pts',(19.8324154522082,41.8815022727306,0.));
#94208=CARTESIAN_POINT('Ctrl Pts',(19.8324154522082,41.8815022727306,20.));
#94209=CARTESIAN_POINT('Ctrl Pts',(19.8607156345021,41.8648118905217,0.));
#94210=CARTESIAN_POINT('Ctrl Pts',(19.8607156345021,41.8648118905217,20.));
#94211=CARTESIAN_POINT('Ctrl Pts',(19.889003062557,41.8481020959867,0.));
#94212=CARTESIAN_POINT('Ctrl Pts',(19.889003062557,41.8481020959867,20.));
#94213=CARTESIAN_POINT('Ctrl Pts',(19.9172777227157,41.8313728982175,0.));
#94214=CARTESIAN_POINT('Ctrl Pts',(19.9172777227157,41.8313728982175,20.));
#94215=CARTESIAN_POINT('Ctrl Pts',(19.9455396013269,41.8146243063152,0.));
#94216=CARTESIAN_POINT('Ctrl Pts',(19.9455396013269,41.8146243063152,20.));
#94217=CARTESIAN_POINT('Ctrl Pts',(19.9737886847461,41.7978563293914,0.));
#94218=CARTESIAN_POINT('Ctrl Pts',(19.9737886847461,41.7978563293914,20.));
#94219=CARTESIAN_POINT('Ctrl Pts',(20.0020249593348,41.7810689765679,0.));
#94220=CARTESIAN_POINT('Ctrl Pts',(20.0020249593348,41.7810689765679,20.));
#94221=CARTESIAN_POINT('Ctrl Pts',(20.0302484114611,41.7642622569769,0.));
#94222=CARTESIAN_POINT('Ctrl Pts',(20.0302484114611,41.7642622569769,20.));
#94223=CARTESIAN_POINT('Ctrl Pts',(20.0584590274991,41.7474361797609,0.));
#94224=CARTESIAN_POINT('Ctrl Pts',(20.0584590274991,41.7474361797609,20.));
#94225=CARTESIAN_POINT('Ctrl Pts',(20.0866567938287,41.7305907540713,0.));
#94226=CARTESIAN_POINT('Ctrl Pts',(20.0866567938287,41.7305907540713,20.));
#94227=CARTESIAN_POINT('Ctrl Pts',(20.1148416968357,41.7137259890696,0.));
#94228=CARTESIAN_POINT('Ctrl Pts',(20.1148416968357,41.7137259890696,20.));
#94229=CARTESIAN_POINT('Ctrl Pts',(20.1430137229118,41.6968418939263,0.));
#94230=CARTESIAN_POINT('Ctrl Pts',(20.1430137229118,41.6968418939263,20.));
#94231=CARTESIAN_POINT('Ctrl Pts',(20.1711728584548,41.6799384778218,0.));
#94232=CARTESIAN_POINT('Ctrl Pts',(20.1711728584548,41.6799384778218,20.));
#94233=CARTESIAN_POINT('Ctrl Pts',(20.199319089869,41.6630157499462,0.));
#94234=CARTESIAN_POINT('Ctrl Pts',(20.199319089869,41.6630157499462,20.));
#94235=CARTESIAN_POINT('Ctrl Pts',(20.2274524035648,41.6460737195007,0.));
#94236=CARTESIAN_POINT('Ctrl Pts',(20.2274524035648,41.6460737195007,20.));
#94237=CARTESIAN_POINT('Ctrl Pts',(20.2555727859589,41.6291123956959,0.));
#94238=CARTESIAN_POINT('Ctrl Pts',(20.2555727859589,41.6291123956959,20.));
#94239=CARTESIAN_POINT('Ctrl Pts',(20.2836802234745,41.6121317877528,0.));
#94240=CARTESIAN_POINT('Ctrl Pts',(20.2836802234745,41.6121317877528,20.));
#94241=CARTESIAN_POINT('Ctrl Pts',(20.3117747025404,41.5951319049016,0.));
#94242=CARTESIAN_POINT('Ctrl Pts',(20.3117747025404,41.5951319049016,20.));
#94243=CARTESIAN_POINT('Ctrl Pts',(20.3398562095916,41.5781127563818,0.));
#94244=CARTESIAN_POINT('Ctrl Pts',(20.3398562095916,41.5781127563818,20.));
#94245=CARTESIAN_POINT('Ctrl Pts',(20.3679247310694,41.561074351443,0.));
#94246=CARTESIAN_POINT('Ctrl Pts',(20.3679247310694,41.561074351443,20.));
#94247=CARTESIAN_POINT('Ctrl Pts',(20.395980253421,41.5440166993445,0.));
#94248=CARTESIAN_POINT('Ctrl Pts',(20.395980253421,41.5440166993445,20.));
#94249=CARTESIAN_POINT('Ctrl Pts',(20.4240227631002,41.5269398093561,0.));
#94250=CARTESIAN_POINT('Ctrl Pts',(20.4240227631002,41.5269398093561,20.));
#94251=CARTESIAN_POINT('Ctrl Pts',(20.4520522465668,41.5098436907568,0.));
#94252=CARTESIAN_POINT('Ctrl Pts',(20.4520522465668,41.5098436907568,20.));
#94253=CARTESIAN_POINT('Ctrl Pts',(20.4800686902869,41.4927283528358,0.));
#94254=CARTESIAN_POINT('Ctrl Pts',(20.4800686902869,41.4927283528358,20.));
#94255=CARTESIAN_POINT('Ctrl Pts',(20.5080720807336,41.4755938048931,0.));
#94256=CARTESIAN_POINT('Ctrl Pts',(20.5080720807336,41.4755938048931,20.));
#94257=CARTESIAN_POINT('Ctrl Pts',(20.5360624043854,41.4584400562379,0.));
#94258=CARTESIAN_POINT('Ctrl Pts',(20.5360624043854,41.4584400562379,20.));
#94259=CARTESIAN_POINT('Ctrl Pts',(20.5640396477269,41.4412671161883,0.));
#94260=CARTESIAN_POINT('Ctrl Pts',(20.5640396477269,41.4412671161883,20.));
#94261=CARTESIAN_POINT('Ctrl Pts',(20.5920037972489,41.4240749940722,0.));
#94262=CARTESIAN_POINT('Ctrl Pts',(20.5920037972489,41.4240749940722,20.));
#94263=CARTESIAN_POINT('Ctrl Pts',(20.6199548394484,41.4068636992265,0.));
#94264=CARTESIAN_POINT('Ctrl Pts',(20.6199548394484,41.4068636992265,20.));
#94265=CARTESIAN_POINT('Ctrl Pts',(20.6478927608288,41.3896332409988,0.));
#94266=CARTESIAN_POINT('Ctrl Pts',(20.6478927608288,41.3896332409988,20.));
#94267=CARTESIAN_POINT('Ctrl Pts',(20.6758175479,41.3723836287471,0.));
#94268=CARTESIAN_POINT('Ctrl Pts',(20.6758175479,41.3723836287471,20.));
#94269=CARTESIAN_POINT('Ctrl Pts',(20.7037291871782,41.3551148718389,0.));
#94270=CARTESIAN_POINT('Ctrl Pts',(20.7037291871782,41.3551148718389,20.));
#94271=CARTESIAN_POINT('Ctrl Pts',(20.731627665186,41.3378269796522,0.));
#94272=CARTESIAN_POINT('Ctrl Pts',(20.731627665186,41.3378269796522,20.));
#94273=CARTESIAN_POINT('Ctrl Pts',(20.7595129684521,41.3205199615745,0.));
#94274=CARTESIAN_POINT('Ctrl Pts',(20.7595129684521,41.3205199615745,20.));
#94275=CARTESIAN_POINT('Ctrl Pts',(20.7873850835117,41.303193827003,0.));
#94276=CARTESIAN_POINT('Ctrl Pts',(20.7873850835117,41.303193827003,20.));
#94277=CARTESIAN_POINT('Ctrl Pts',(20.8152439969059,41.285848585344,0.));
#94278=CARTESIAN_POINT('Ctrl Pts',(20.8152439969059,41.285848585344,20.));
#94279=CARTESIAN_POINT('Ctrl Pts',(20.8430896951822,41.268484246013,0.));
#94280=CARTESIAN_POINT('Ctrl Pts',(20.8430896951822,41.268484246013,20.));
#94281=CARTESIAN_POINT('Ctrl Pts',(20.8709221648944,41.2511008184358,0.));
#94282=CARTESIAN_POINT('Ctrl Pts',(20.8709221648944,41.2511008184358,20.));
#94283=CARTESIAN_POINT('Ctrl Pts',(20.8987413926025,41.2336983120481,0.));
#94284=CARTESIAN_POINT('Ctrl Pts',(20.8987413926025,41.2336983120481,20.));
#94285=CARTESIAN_POINT('Ctrl Pts',(20.9265473648728,41.2162767362953,0.));
#94286=CARTESIAN_POINT('Ctrl Pts',(20.9265473648728,41.2162767362953,20.));
#94287=CARTESIAN_POINT('Ctrl Pts',(20.9543400682781,41.1988361006333,0.));
#94288=CARTESIAN_POINT('Ctrl Pts',(20.9543400682781,41.1988361006333,20.));
#94289=CARTESIAN_POINT('Ctrl Pts',(20.9821194893979,41.1813764145274,0.));
#94290=CARTESIAN_POINT('Ctrl Pts',(20.9821194893979,41.1813764145274,20.));
#94291=CARTESIAN_POINT('Ctrl Pts',(21.009885614818,41.1638976874526,0.));
#94292=CARTESIAN_POINT('Ctrl Pts',(21.009885614818,41.1638976874526,20.));
#94293=CARTESIAN_POINT('Ctrl Pts',(21.0376384311301,41.1463999288927,0.));
#94294=CARTESIAN_POINT('Ctrl Pts',(21.0376384311301,41.1463999288927,20.));
#94295=CARTESIAN_POINT('Ctrl Pts',(21.0653779249329,41.128883148342,0.));
#94296=CARTESIAN_POINT('Ctrl Pts',(21.0653779249329,41.128883148342,20.));
#94297=CARTESIAN_POINT('Ctrl Pts',(21.093104082831,41.1113473553046,0.));
#94298=CARTESIAN_POINT('Ctrl Pts',(21.093104082831,41.1113473553046,20.));
#94299=CARTESIAN_POINT('Ctrl Pts',(21.1208168914355,41.0937925592944,0.));
#94300=CARTESIAN_POINT('Ctrl Pts',(21.1208168914355,41.0937925592944,20.));
#94301=CARTESIAN_POINT('Ctrl Pts',(21.1485163373635,41.076218769835,0.));
#94302=CARTESIAN_POINT('Ctrl Pts',(21.1485163373635,41.076218769835,20.));
#94303=CARTESIAN_POINT('Ctrl Pts',(21.1762024072388,41.0586259964597,0.));
#94304=CARTESIAN_POINT('Ctrl Pts',(21.1762024072388,41.0586259964597,20.));
#94305=CARTESIAN_POINT('Ctrl Pts',(21.2038750876913,41.0410142487106,0.));
#94306=CARTESIAN_POINT('Ctrl Pts',(21.2038750876913,41.0410142487106,20.));
#94307=CARTESIAN_POINT('Ctrl Pts',(21.2315343653574,41.0233835361399,0.));
#94308=CARTESIAN_POINT('Ctrl Pts',(21.2315343653574,41.0233835361399,20.));
#94309=CARTESIAN_POINT('Ctrl Pts',(21.25918022688,41.0057338683097,0.));
#94310=CARTESIAN_POINT('Ctrl Pts',(21.25918022688,41.0057338683097,20.));
#94311=CARTESIAN_POINT('Ctrl Pts',(21.286812658909,40.9880652547928,0.));
#94312=CARTESIAN_POINT('Ctrl Pts',(21.286812658909,40.9880652547928,20.));
#94313=CARTESIAN_POINT('Ctrl Pts',(21.3144316481011,40.9703777051716,0.));
#94314=CARTESIAN_POINT('Ctrl Pts',(21.3144316481011,40.9703777051716,20.));
#94315=CARTESIAN_POINT('Ctrl Pts',(21.342037181119,40.9526712290373,0.));
#94316=CARTESIAN_POINT('Ctrl Pts',(21.342037181119,40.9526712290373,20.));
#94317=CARTESIAN_POINT('Ctrl Pts',(21.3696292446317,40.9349458359905,0.));
#94318=CARTESIAN_POINT('Ctrl Pts',(21.3696292446317,40.9349458359905,20.));
#94319=CARTESIAN_POINT('Ctrl Pts',(21.3972078253142,40.9172015356414,0.));
#94320=CARTESIAN_POINT('Ctrl Pts',(21.3972078253142,40.9172015356414,20.));
#94321=CARTESIAN_POINT('Ctrl Pts',(21.4247729098479,40.8994383376102,0.));
#94322=CARTESIAN_POINT('Ctrl Pts',(21.4247729098479,40.8994383376102,20.));
#94323=CARTESIAN_POINT('Ctrl Pts',(21.4523244849199,40.8816562515268,0.));
#94324=CARTESIAN_POINT('Ctrl Pts',(21.4523244849199,40.8816562515268,20.));
#94325=CARTESIAN_POINT('Ctrl Pts',(21.4798625372243,40.8638552870319,0.));
#94326=CARTESIAN_POINT('Ctrl Pts',(21.4798625372243,40.8638552870319,20.));
#94327=CARTESIAN_POINT('Ctrl Pts',(21.5073870534614,40.8460354537749,0.));
#94328=CARTESIAN_POINT('Ctrl Pts',(21.5073870534614,40.8460354537749,20.));
#94329=CARTESIAN_POINT('Ctrl Pts',(21.5348980203391,40.8281967614155,0.));
#94330=CARTESIAN_POINT('Ctrl Pts',(21.5348980203391,40.8281967614155,20.));
#94331=CARTESIAN_POINT('Ctrl Pts',(21.5623954245725,40.8103392196221,0.));
#94332=CARTESIAN_POINT('Ctrl Pts',(21.5623954245725,40.8103392196221,20.));
#94333=CARTESIAN_POINT('Ctrl Pts',(21.5898792528837,40.7924628380726,0.));
#94334=CARTESIAN_POINT('Ctrl Pts',(21.5898792528837,40.7924628380726,20.));
#94335=CARTESIAN_POINT('Ctrl Pts',(21.6173494920019,40.7745676264537,0.));
#94336=CARTESIAN_POINT('Ctrl Pts',(21.6173494920019,40.7745676264537,20.));
#94337=CARTESIAN_POINT('Ctrl Pts',(21.6448061286619,40.7566535944621,0.));
#94338=CARTESIAN_POINT('Ctrl Pts',(21.6448061286619,40.7566535944621,20.));
#94339=CARTESIAN_POINT('Ctrl Pts',(21.6722491496038,40.7387207518043,0.));
#94340=CARTESIAN_POINT('Ctrl Pts',(21.6722491496038,40.7387207518043,20.));
#94341=CARTESIAN_POINT('Ctrl Pts',(21.6996785415723,40.7207691081984,0.));
#94342=CARTESIAN_POINT('Ctrl Pts',(21.6996785415723,40.7207691081984,20.));
#94343=CARTESIAN_POINT('Ctrl Pts',(21.7270942913167,40.7027986733736,0.));
#94344=CARTESIAN_POINT('Ctrl Pts',(21.7270942913167,40.7027986733736,20.));
#94345=CARTESIAN_POINT('Ctrl Pts',(21.7544963855931,40.6848094570694,0.));
#94346=CARTESIAN_POINT('Ctrl Pts',(21.7544963855931,40.6848094570694,20.));
#94347=CARTESIAN_POINT('Ctrl Pts',(21.781884811165,40.6668014690334,0.));
#94348=CARTESIAN_POINT('Ctrl Pts',(21.781884811165,40.6668014690334,20.));
#94349=CARTESIAN_POINT('Ctrl Pts',(21.8092595548052,40.6487747190214,0.));
#94350=CARTESIAN_POINT('Ctrl Pts',(21.8092595548052,40.6487747190214,20.));
#94351=CARTESIAN_POINT('Ctrl Pts',(21.8366206032979,40.6307292167951,0.));
#94352=CARTESIAN_POINT('Ctrl Pts',(21.8366206032979,40.6307292167951,20.));
#94353=CARTESIAN_POINT('Ctrl Pts',(21.8639679434382,40.6126649721233,0.));
#94354=CARTESIAN_POINT('Ctrl Pts',(21.8639679434382,40.6126649721233,20.));
#94355=CARTESIAN_POINT('Ctrl Pts',(21.8913015620281,40.594581994783,0.));
#94356=CARTESIAN_POINT('Ctrl Pts',(21.8913015620281,40.594581994783,20.));
#94357=CARTESIAN_POINT('Ctrl Pts',(21.9186214458728,40.5764802945639,0.));
#94358=CARTESIAN_POINT('Ctrl Pts',(21.9186214458728,40.5764802945639,20.));
#94359=CARTESIAN_POINT('Ctrl Pts',(21.9459275817778,40.5583598812699,0.));
#94360=CARTESIAN_POINT('Ctrl Pts',(21.9459275817778,40.5583598812699,20.));
#94361=CARTESIAN_POINT('Ctrl Pts',(21.9732199565439,40.5402207647219,0.));
#94362=CARTESIAN_POINT('Ctrl Pts',(21.9732199565439,40.5402207647219,20.));
#94363=CARTESIAN_POINT('Ctrl Pts',(22.0004985569689,40.5220629547578,0.));
#94364=CARTESIAN_POINT('Ctrl Pts',(22.0004985569689,40.5220629547578,20.));
#94365=CARTESIAN_POINT('Ctrl Pts',(22.0277633698572,40.5038864612253,0.));
#94366=CARTESIAN_POINT('Ctrl Pts',(22.0277633698572,40.5038864612253,20.));
#94367=CARTESIAN_POINT('Ctrl Pts',(22.0550143820281,40.485691293976,0.));
#94368=CARTESIAN_POINT('Ctrl Pts',(22.0550143820281,40.485691293976,20.));
#94369=CARTESIAN_POINT('Ctrl Pts',(22.0822515803231,40.4674774628609,0.));
#94370=CARTESIAN_POINT('Ctrl Pts',(22.0822515803231,40.4674774628609,20.));
#94371=CARTESIAN_POINT('Ctrl Pts',(22.1094749516164,40.4492449777204,0.));
#94372=CARTESIAN_POINT('Ctrl Pts',(22.1094749516164,40.4492449777204,20.));
#94373=CARTESIAN_POINT('Ctrl Pts',(22.1366844828092,40.4309938483881,0.));
#94374=CARTESIAN_POINT('Ctrl Pts',(22.1366844828092,40.4309938483881,20.));
#94375=CARTESIAN_POINT('Ctrl Pts',(22.1638801608087,40.4127240847076,0.));
#94376=CARTESIAN_POINT('Ctrl Pts',(22.1638801608087,40.4127240847076,20.));
#94377=CARTESIAN_POINT('Ctrl Pts',(22.1910619725087,40.3944356965472,0.));
#94378=CARTESIAN_POINT('Ctrl Pts',(22.1910619725087,40.3944356965472,20.));
#94379=CARTESIAN_POINT('Ctrl Pts',(22.2182299047735,40.3761286938115,0.));
#94380=CARTESIAN_POINT('Ctrl Pts',(22.2182299047735,40.3761286938115,20.));
#94381=CARTESIAN_POINT('Ctrl Pts',(22.2453839444114,40.357803086462,0.));
#94382=CARTESIAN_POINT('Ctrl Pts',(22.2453839444114,40.357803086462,20.));
#94383=CARTESIAN_POINT('Ctrl Pts',(22.2725240781926,40.3394588845042,0.));
#94384=CARTESIAN_POINT('Ctrl Pts',(22.2725240781926,40.3394588845042,20.));
#94385=CARTESIAN_POINT('Ctrl Pts',(22.2996502928986,40.3210960979489,0.));
#94386=CARTESIAN_POINT('Ctrl Pts',(22.2996502928986,40.3210960979489,20.));
#94387=CARTESIAN_POINT('Ctrl Pts',(22.326762575367,40.3027147367804,0.));
#94388=CARTESIAN_POINT('Ctrl Pts',(22.326762575367,40.3027147367804,20.));
#94389=CARTESIAN_POINT('Ctrl Pts',(22.3538609125294,40.2843148109268,0.));
#94390=CARTESIAN_POINT('Ctrl Pts',(22.3538609125294,40.2843148109268,20.));
#94391=CARTESIAN_POINT('Ctrl Pts',(22.3809452914735,40.2658963302133,0.));
#94392=CARTESIAN_POINT('Ctrl Pts',(22.3809452914735,40.2658963302133,20.));
#94393=CARTESIAN_POINT('Ctrl Pts',(22.4080156993888,40.2474593044019,0.));
#94394=CARTESIAN_POINT('Ctrl Pts',(22.4080156993888,40.2474593044019,20.));
#94395=CARTESIAN_POINT('Ctrl Pts',(22.4350721234534,40.229003743277,0.));
#94396=CARTESIAN_POINT('Ctrl Pts',(22.4350721234534,40.229003743277,20.));
#94397=CARTESIAN_POINT('Ctrl Pts',(22.4621145507305,40.210529656724,0.));
#94398=CARTESIAN_POINT('Ctrl Pts',(22.4621145507305,40.210529656724,20.));
#94399=CARTESIAN_POINT('Ctrl Pts',(22.4891429680799,40.1920370547964,0.));
#94400=CARTESIAN_POINT('Ctrl Pts',(22.4891429680799,40.1920370547964,20.));
#94401=CARTESIAN_POINT('Ctrl Pts',(22.5161573620162,40.1735259478254,0.));
#94402=CARTESIAN_POINT('Ctrl Pts',(22.5161573620162,40.1735259478254,20.));
#94403=CARTESIAN_POINT('Ctrl Pts',(22.5431577188605,40.1549963463026,0.));
#94404=CARTESIAN_POINT('Ctrl Pts',(22.5431577188605,40.1549963463026,20.));
#94405=CARTESIAN_POINT('Ctrl Pts',(22.5701440249982,40.1364482606861,0.));
#94406=CARTESIAN_POINT('Ctrl Pts',(22.5701440249982,40.1364482606861,20.));
#94407=CARTESIAN_POINT('Ctrl Pts',(22.5971162671187,40.1178817012184,0.));
#94408=CARTESIAN_POINT('Ctrl Pts',(22.5971162671187,40.1178817012184,20.));
#94409=CARTESIAN_POINT('Ctrl Pts',(22.6240744324258,40.0992966777668,0.));
#94410=CARTESIAN_POINT('Ctrl Pts',(22.6240744324258,40.0992966777668,20.));
#94411=CARTESIAN_POINT('Ctrl Pts',(22.6510185089549,40.0806931995834,0.));
#94412=CARTESIAN_POINT('Ctrl Pts',(22.6510185089549,40.0806931995834,20.));
#94413=CARTESIAN_POINT('Ctrl Pts',(22.6779484851672,40.0620712756149,0.));
#94414=CARTESIAN_POINT('Ctrl Pts',(22.6779484851672,40.0620712756149,20.));
#94415=CARTESIAN_POINT('Ctrl Pts',(22.7048643493645,40.0434309149417,0.));
#94416=CARTESIAN_POINT('Ctrl Pts',(22.7048643493645,40.0434309149417,20.));
#94417=CARTESIAN_POINT('Ctrl Pts',(22.73176608914,40.0247721271957,0.));
#94418=CARTESIAN_POINT('Ctrl Pts',(22.73176608914,40.0247721271957,20.));
#94419=CARTESIAN_POINT('Ctrl Pts',(22.7586536908731,40.0060949229408,0.));
#94420=CARTESIAN_POINT('Ctrl Pts',(22.7586536908731,40.0060949229408,20.));
#94421=CARTESIAN_POINT('Ctrl Pts',(22.7855271390493,39.9873993141881,0.));
#94422=CARTESIAN_POINT('Ctrl Pts',(22.7855271390493,39.9873993141881,20.));
#94423=CARTESIAN_POINT('Ctrl Pts',(22.8123864172494,39.9686853136472,0.));
#94424=CARTESIAN_POINT('Ctrl Pts',(22.8123864172494,39.9686853136472,20.));
#94425=CARTESIAN_POINT('Ctrl Pts',(22.8392315093989,39.9499529337848,0.));
#94426=CARTESIAN_POINT('Ctrl Pts',(22.8392315093989,39.9499529337848,20.));
#94427=CARTESIAN_POINT('Ctrl Pts',(22.8660624009432,39.9312021859375,0.));
#94428=CARTESIAN_POINT('Ctrl Pts',(22.8660624009432,39.9312021859375,20.));
#94429=CARTESIAN_POINT('Ctrl Pts',(22.8928790800154,39.91243307943,0.));
#94430=CARTESIAN_POINT('Ctrl Pts',(22.8928790800154,39.91243307943,20.));
#94431=CARTESIAN_POINT('Ctrl Pts',(22.9196815387084,39.8936456206159,0.));
#94432=CARTESIAN_POINT('Ctrl Pts',(22.9196815387084,39.8936456206159,20.));
#94433=CARTESIAN_POINT('Ctrl Pts',(22.9464697723601,39.8748398133807,0.));
#94434=CARTESIAN_POINT('Ctrl Pts',(22.9464697723601,39.8748398133807,20.));
#94435=CARTESIAN_POINT('Ctrl Pts',(22.9678889774251,39.8597804904793,0.));
#94436=CARTESIAN_POINT('Ctrl Pts',(22.9678889774251,39.8597804904793,20.));
#94437=CARTESIAN_POINT('Ctrl Pts',(22.9839469786125,39.8484777427633,0.));
#94438=CARTESIAN_POINT('Ctrl Pts',(22.9839469786125,39.8484777427633,20.));
#94439=CARTESIAN_POINT('Ctrl Pts',(22.9946494671375,39.8409389084975,0.));
#94440=CARTESIAN_POINT('Ctrl Pts',(22.9946494671375,39.8409389084975,20.));
#94441=CARTESIAN_POINT('Ctrl Pts',(23.,39.8371685740842,0.));
#94442=CARTESIAN_POINT('Ctrl Pts',(23.,39.8371685740842,20.));
#94443=CARTESIAN_POINT('',(23.,39.8371685740842,0.));
#94444=CARTESIAN_POINT('Origin',(35.3531508854311,30.9702231582522,0.));
#94445=CARTESIAN_POINT('',(34.6009561857411,30.3112822399915,0.));
#94446=CARTESIAN_POINT('Origin',(1.19904086659517E-13,1.4210854715202E-13,
0.));
#94447=CARTESIAN_POINT('Origin',(0.,0.,0.));
#99493=UNCERTAINTY_MEASURE_WITH_UNIT(LENGTH_MEASURE(0.01),#99527,
'DISTANCE_ACCURACY_VALUE',
'Maximum model space distance between geometric entities at asserted c
onnectivities');
#99508=UNCERTAINTY_MEASURE_WITH_UNIT(LENGTH_MEASURE(0.01),#99527,
'DISTANCE_ACCURACY_VALUE',
'Maximum model space distance between geometric entities at asserted c
onnectivities');
#99511=(
GEOMETRIC_REPRESENTATION_CONTEXT(3)
GLOBAL_UNCERTAINTY_ASSIGNED_CONTEXT((#99493))
GLOBAL_UNIT_ASSIGNED_CONTEXT((#99527,#99529,#99530))
REPRESENTATION_CONTEXT('','3D')
);
#99526=(
GEOMETRIC_REPRESENTATION_CONTEXT(3)
GLOBAL_UNCERTAINTY_ASSIGNED_CONTEXT((#99508))
GLOBAL_UNIT_ASSIGNED_CONTEXT((#99527,#99529,#99530))
REPRESENTATION_CONTEXT('','3D')
);
#99527=(
LENGTH_UNIT()
NAMED_UNIT(*)
SI_UNIT(.MILLI.,.METRE.)
);
#99529=(
NAMED_UNIT(*)
PLANE_ANGLE_UNIT()
SI_UNIT($,.RADIAN.)
);
#99530=(
NAMED_UNIT(*)
SI_UNIT($,.STERADIAN.)
SOLID_ANGLE_UNIT()
);
#99533=SHAPE_DEFINITION_REPRESENTATION(#99550,#99626);
#99550=PRODUCT_DEFINITION_SHAPE('',$,#99644);
#99626=SHAPE_REPRESENTATION('',(#18965),#99511);
#99641=PRODUCT_DEFINITION_CONTEXT('part definition',#99694,'design');
#99644=PRODUCT_DEFINITION('Ramp hub','Ramp hub',#99661,#99641);
#99661=PRODUCT_DEFINITION_FORMATION('',$,#99698);
#99694=APPLICATION_CONTEXT(
'Core Data for Automotive Mechanical Design Process');
#99695=PRODUCT_CONTEXT('part definition',#99694,'mechanical');
#99698=PRODUCT('Ramp hub','Ramp hub',
'Turn OD and bore; cut gear teeth in the assembly-specific design.',(#99695));
#99715=PRESENTATION_STYLE_ASSIGNMENT((#99728));
#99728=SURFACE_STYLE_USAGE(.BOTH.,#99741);
#99741=SURFACE_SIDE_STYLE('',(#99754));
#99754=SURFACE_STYLE_FILL_AREA(#99767);
#99767=FILL_AREA_STYLE('Light blue',(#99780));
#99780=FILL_AREA_STYLE_COLOUR('Light blue',#99793);
#99793=COLOUR_RGB('Light blue',0.662745098039216,0.831372549019608,0.949019607843137);
ENDSEC;
END-ISO-10303-21;
